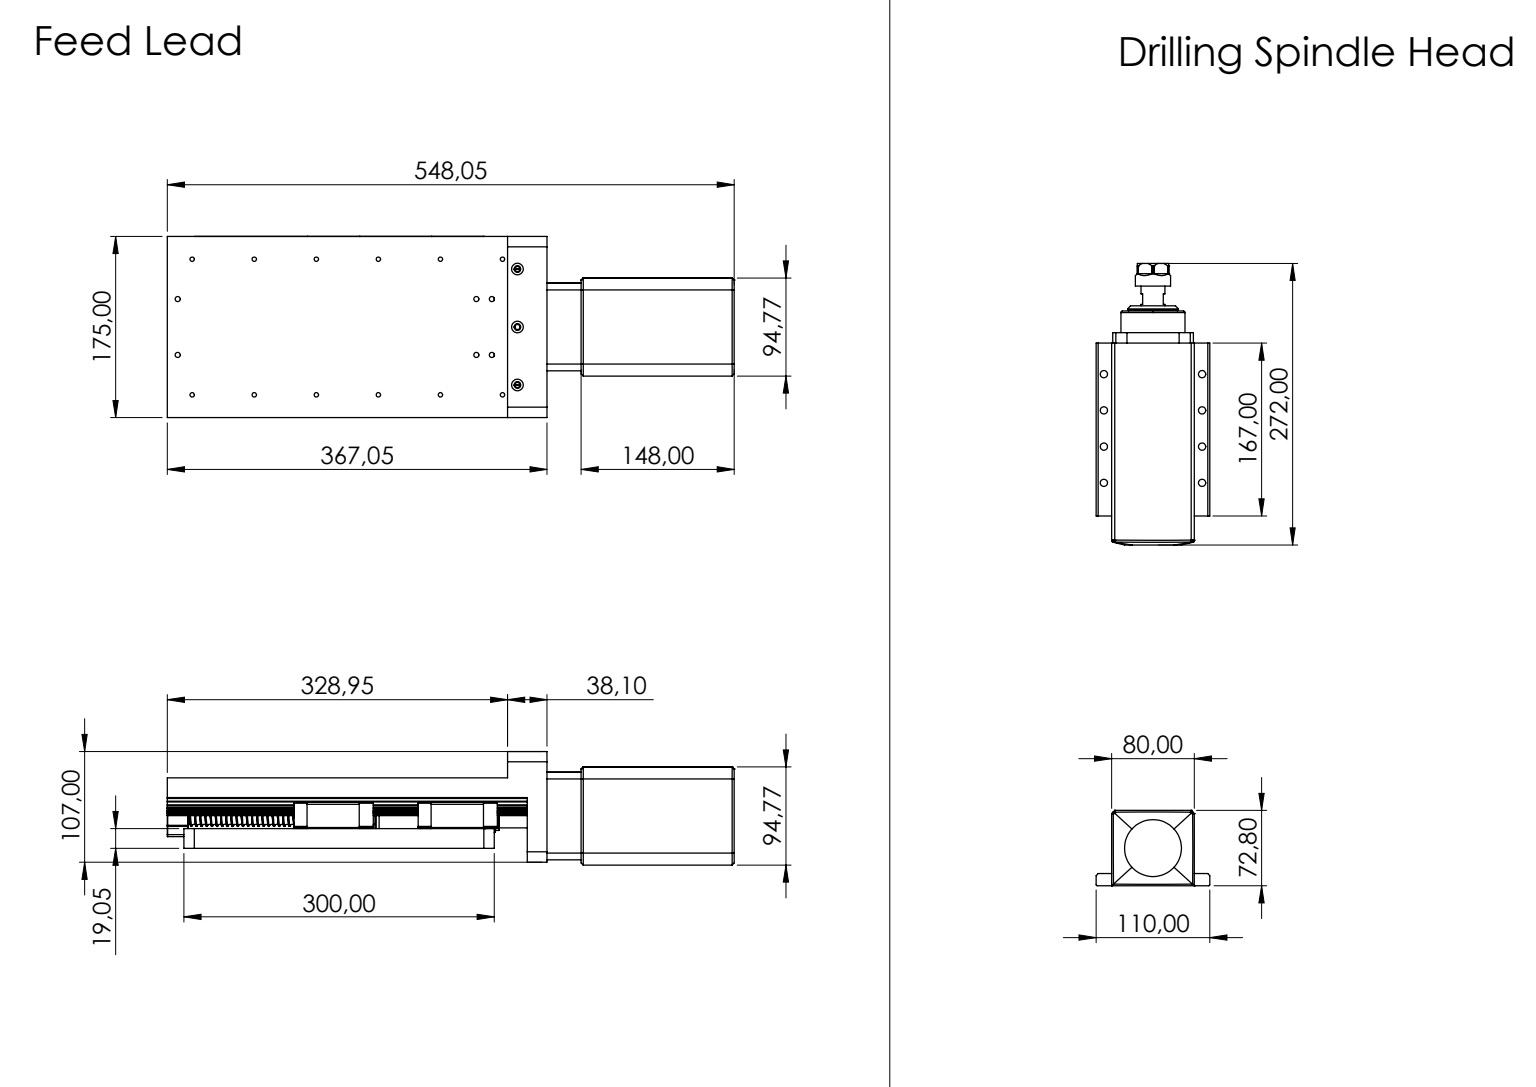
ISO-10303-21;
HEADER;
FILE_DESCRIPTION (('STEP AP214'),
    '1' );
FILE_NAME ('Feed Lead.step',
    '2026-10-07T11:37:37',
    ( '' ),
    ( '' ),
    'SwSTEP 2.0',
    'SolidWorks 2020',
    '' );
FILE_SCHEMA (( 'AUTOMOTIVE_DESIGN' ));
ENDSEC;

DATA;
#1=CARTESIAN_POINT ( 'NONE',  ( 98.82205551832399237, -39.36200594543229414, 279.3785665600675543 ) ) ;
#2=VECTOR ( 'NONE', #11114, 1000.000000000000000 ) ;
#4=CARTESIAN_POINT ( 'NONE',  ( 105.4244293397738659, -47.72525222749325735, 147.4584824187689662 ) ) ;
#7=DIRECTION ( 'NONE',  ( 0.000000000000000000, 1.000000000000000000, 0.000000000000000000 ) ) ;
#10=CARTESIAN_POINT ( 'NONE',  ( 112.4341072229889136, -46.44469865882210513, 248.9661014663869878 ) ) ;
#13=ORIENTED_EDGE ( 'NONE', *, *, #80261, .T. ) ;
#16=CARTESIAN_POINT ( 'NONE',  ( 97.53157056845665807, -31.04763954905634193, 126.9108633711489915 ) ) ;
#17=CARTESIAN_POINT ( 'NONE',  ( 83.56670559755357885, -36.73837296219067383, 249.5838068554176630 ) ) ;
#20=ORIENTED_EDGE ( 'NONE', *, *, #86122, .T. ) ;
#22=DIRECTION ( 'NONE',  ( 0.000000000000000000, 0.000000000000000000, -1.000000000000000000 ) ) ;
#23=LINE ( 'NONE', #20915, #47197 ) ;
#25=CARTESIAN_POINT ( 'NONE',  ( 179.7974245136208253, -36.32844715993472562, 237.4678068554150059 ) ) ;
#26=CARTESIAN_POINT ( 'NONE',  ( 108.8610815749077574, -28.26302276435299987, 182.7404713219719667 ) ) ;
#27=CARTESIAN_POINT ( 'NONE',  ( 118.1260584382194025, -36.12034675239389259, 269.8822919425776945 ) ) ;
#28=DIRECTION ( 'NONE',  ( 0.7071067811865491270, -0.7071067811865459074, 7.071067811865492096E-16 ) ) ;
#29=EDGE_LOOP ( 'NONE', ( #51270, #35552, #65434, #23515 ) ) ;
#34=ORIENTED_EDGE ( 'NONE', *, *, #61854, .T. ) ;
#35=EDGE_CURVE ( 'NONE', #22057, #40854, #8280, .T. ) ;
#37=DIRECTION ( 'NONE',  ( 0.000000000000000000, 0.000000000000000000, 1.000000000000000000 ) ) ;
#38=LINE ( 'NONE', #47715, #64581 ) ;
#39=CARTESIAN_POINT ( 'NONE',  ( 20.03715912545644073, -24.42818131006202265, 129.9678068554150627 ) ) ;
#42=CARTESIAN_POINT ( 'NONE',  ( 112.8494018163660968, -30.44343212223953543, 198.9067055423629711 ) ) ;
#43=CARTESIAN_POINT ( 'NONE',  ( 116.1621043582934902, -29.05491297703968101, 74.38419670448293175 ) ) ;
#44=CARTESIAN_POINT ( 'NONE',  ( 140.9629299006807059, -46.47944715994099596, -5.074374724088994704 ) ) ;
#45=VERTEX_POINT ( 'NONE', #80264 ) ;
#46=DIRECTION ( 'NONE',  ( 0.000000000000000000, 0.000000000000000000, -1.000000000000000000 ) ) ;
#47=ORIENTED_EDGE ( 'NONE', *, *, #89162, .T. ) ;
#50=LINE ( 'NONE', #6413, #88589 ) ;
#51=CARTESIAN_POINT ( 'NONE',  ( 151.0371591254573502, -24.42818131005592974, 249.9678068554149490 ) ) ;
#52=DIRECTION ( 'NONE',  ( 0.000000000000000000, 0.000000000000000000, -1.000000000000000000 ) ) ;
#53=AXIS2_PLACEMENT_3D ( 'NONE', #43663, #9164, #36861 ) ;
#54=CARTESIAN_POINT ( 'NONE',  ( 50.56670390244699576, -22.48495420874030515, 342.9256252759119548 ) ) ;
#56=CARTESIAN_POINT ( 'NONE',  ( 117.9477513149503523, -41.48675964724572651, 58.49848241876792798 ) ) ;
#59=LINE ( 'NONE', #15039, #77144 ) ;
#60=CARTESIAN_POINT ( 'NONE',  ( 131.4961476553978912, -17.75123073100106552, 2.855912073278314534 ) ) ;
#63=CIRCLE ( 'NONE', #39212, 3.250000000000002665 ) ;
#68=CIRCLE ( 'NONE', #26139, 0.1499999999999965528 ) ;
#69=CARTESIAN_POINT ( 'NONE',  ( 163.2449138992999735, -32.11662333284611748, -5.074374724088000832 ) ) ;
#70=VERTEX_POINT ( 'NONE', #52061 ) ;
#71=CARTESIAN_POINT ( 'NONE',  ( 98.28804800891427362, -28.73186473263583807, 76.73848241876795839 ) ) ;
#74=CARTESIAN_POINT ( 'NONE',  ( 151.0371591254582881, -46.82818131005593187, 249.9678068554149490 ) ) ;
#78=ORIENTED_EDGE ( 'NONE', *, *, #28035, .F. ) ;
#79=CARTESIAN_POINT ( 'NONE',  ( 116.1942131220465768, -33.21547736372282600, 135.1184824187679396 ) ) ;
#81=VECTOR ( 'NONE', #81815, 1000.000000000000000 ) ;
#82=PLANE ( 'NONE',  #68963 ) ;
#83=ORIENTED_EDGE ( 'NONE', *, *, #76173, .T. ) ;
#84=CARTESIAN_POINT ( 'NONE',  ( 95.25611604350974915, -37.33230102880721546, 267.3670538473395482 ) ) ;
#89=CARTESIAN_POINT ( 'NONE',  ( 19.56648329127400032, 0.2215528400590013880, 342.9256252759119548 ) ) ;
#90=DIRECTION ( 'NONE',  ( 0.000000000000000000, 0.000000000000000000, 1.000000000000000000 ) ) ;
#92=VECTOR ( 'NONE', #88319, 1000.000000000000000 ) ;
#93=CARTESIAN_POINT ( 'NONE',  ( 102.2986265273211188, -45.30740241592388884, 187.1727681330549729 ) ) ;
#94=ORIENTED_EDGE ( 'NONE', *, *, #21602, .F. ) ;
#96=CARTESIAN_POINT ( 'NONE',  ( 102.7360552222912418, -45.06754756083040547, 163.6149166392309837 ) ) ;
#97=CARTESIAN_POINT ( 'NONE',  ( 41.56648329127398966, -27.82844715994070484, 78.92562527591199739 ) ) ;
#98=CARTESIAN_POINT ( 'NONE',  ( 110.5196960824274868, -45.46740155661881033, 19.31967854399191253 ) ) ;
#100=VECTOR ( 'NONE', #56288, 1000.000000000000000 ) ;
#101=CARTESIAN_POINT ( 'NONE',  ( 97.80969231062213964, -40.51824920587227297, 266.6357212253427633 ) ) ;
#102=CARTESIAN_POINT ( 'NONE',  ( 107.3303934170485405, -25.27334761448656764, 321.8751915430112263 ) ) ;
#103=CIRCLE ( 'NONE', #55178, 11.45913725231036118 ) ;
#106=CARTESIAN_POINT ( 'NONE',  ( 117.3910620576583312, -35.19077923515891371, 218.9441967044829482 ) ) ;
#112=CARTESIAN_POINT ( 'NONE',  ( 98.04125204931517601, -41.04130019950920172, 122.6806003489451342 ) ) ;
#114=VECTOR ( 'NONE', #52134, 1000.000000000000114 ) ;
#115=ADVANCED_FACE ( 'NONE', ( #66606 ), #81165, .T. ) ;
#118=CARTESIAN_POINT ( 'NONE',  ( 109.6225776363756950, -25.10716277166327615, 25.90419670448196143 ) ) ;
#120=CARTESIAN_POINT ( 'NONE',  ( 116.8850244782298091, -41.80638879970206290, 243.4346728949589647 ) ) ;
#123=CARTESIAN_POINT ( 'NONE',  ( 48.16670390244701139, -28.27351298637280408, 342.9256252759109884 ) ) ;
#124=CARTESIAN_POINT ( 'NONE',  ( 116.9882021585877823, -35.34044312313820058, 168.9370952240663257 ) ) ;
#125=CARTESIAN_POINT ( 'NONE',  ( 103.0685998583681311, -29.61280089403793525, 58.30237608387695047 ) ) ;
#126=CARTESIAN_POINT ( 'NONE',  ( 103.0413726597163446, -26.41035368485499646, 166.3603871806729444 ) ) ;
#128=DIRECTION ( 'NONE',  ( 1.000000000000000000, 4.163336342344333240E-14, 0.000000000000000000 ) ) ;
#131=ORIENTED_EDGE ( 'NONE', *, *, #64159, .T. ) ;
#133=ORIENTED_EDGE ( 'NONE', *, *, #51168, .F. ) ;
#137=VERTEX_POINT ( 'NONE', #67956 ) ;
#138=DIRECTION ( 'NONE',  ( 0.000000000000000000, 0.000000000000000000, -1.000000000000000000 ) ) ;
#139=CARTESIAN_POINT ( 'NONE',  ( 114.8228036748933079, -33.15234975719755539, 103.5924198280769843 ) ) ;
#140=VECTOR ( 'NONE', #87504, 1000.000000000000000 ) ;
#141=CARTESIAN_POINT ( 'NONE',  ( 96.49566810458604493, -31.31724962161759507, 245.9499109901969689 ) ) ;
#142=CARTESIAN_POINT ( 'NONE',  ( 116.8369567342160451, -40.30247308064095790, 218.5470538473399529 ) ) ;
#143=CARTESIAN_POINT ( 'NONE',  ( 114.8031991714176741, -43.68443766454699073, 34.24419670448197905 ) ) ;
#145=CARTESIAN_POINT ( 'NONE',  ( 116.7940250750810804, -39.39174829627296504, 94.61447052041835093 ) ) ;
#146=VECTOR ( 'NONE', #83071, 1000.000000000000000 ) ;
#147=EDGE_CURVE ( 'NONE', #87632, #64364, #18910, .T. ) ;
#148=ORIENTED_EDGE ( 'NONE', *, *, #76335, .T. ) ;
#150=CARTESIAN_POINT ( 'NONE',  ( 98.15811136316399654, -31.42099212808717468, 130.9108633711499863 ) ) ;
#151=CARTESIAN_POINT ( 'NONE',  ( 106.8402339230401452, -48.62808610490878891, 77.56133956162491927 ) ) ;
#152=CARTESIAN_POINT ( 'NONE',  ( 104.8318391505165010, -26.46503486849124087, 260.2470538473397710 ) ) ;
#154=CARTESIAN_POINT ( 'NONE',  ( 115.5175571194294122, -29.60495148624196204, 224.3718157521009573 ) ) ;
#156=CARTESIAN_POINT ( 'NONE',  ( 107.0664832912739399, -36.72944715994095333, 293.9356252759109793 ) ) ;
#158=DIRECTION ( 'NONE',  ( -1.000000000000000078E-15, 0.000000000000000000, 1.000000000000000000 ) ) ;
#159=CARTESIAN_POINT ( 'NONE',  ( 167.2371591254543262, -47.82818131005522844, 249.9678068554149775 ) ) ;
#160=CARTESIAN_POINT ( 'NONE',  ( 41.56670390244777735, -36.32844715994104234, 300.4678068554150059 ) ) ;
#164=CARTESIAN_POINT ( 'NONE',  ( 88.17226027475679473, -58.72944715994100306, 239.5838068554174924 ) ) ;
#169=ORIENTED_EDGE ( 'NONE', *, *, #32648, .T. ) ;
#171=CARTESIAN_POINT ( 'NONE',  ( 96.89273651078235616, -34.20293982824353662, 276.1327681330536734 ) ) ;
#172=CARTESIAN_POINT ( 'NONE',  ( 117.0331605330187728, -30.31849857022486816, 140.2813395616249750 ) ) ;
#173=CARTESIAN_POINT ( 'NONE',  ( 106.2234015700748699, -47.79681864418333959, 263.5280062282922131 ) ) ;
#174=CARTESIAN_POINT ( 'NONE',  ( 51.56670390244799762, -33.35206098992650681, -5.074374724088000832 ) ) ;
#175=CIRCLE ( 'NONE', #23415, 3.000000000000002665 ) ;
#177=LINE ( 'NONE', #49653, #51558 ) ;
#178=CARTESIAN_POINT ( 'NONE',  ( 164.9212702847350158, -29.73316016639540749, -5.074374724088000832 ) ) ;
#179=CARTESIAN_POINT ( 'NONE',  ( 84.06648329127399677, -18.82844715994099971, 93.42562527591199739 ) ) ;
#180=VECTOR ( 'NONE', #42235, 1000.000000000000000 ) ;
#181=ORIENTED_EDGE ( 'NONE', *, *, #13082, .F. ) ;
#183=EDGE_LOOP ( 'NONE', ( #41737, #81659, #77262, #76610 ) ) ;
#184=CARTESIAN_POINT ( 'NONE',  ( 104.1791519563360993, -28.66003454886012136, 189.7724198280769770 ) ) ;
#185=EDGE_CURVE ( 'NONE', #48213, #31965, #19881, .T. ) ;
#186=CARTESIAN_POINT ( 'NONE',  ( 112.0622504009905356, -45.49043716283868832, 187.9900270775093247 ) ) ;
#187=ORIENTED_EDGE ( 'NONE', *, *, #67758, .F. ) ;
#189=CARTESIAN_POINT ( 'NONE',  ( 103.8142050530422864, -26.84757730287823563, 161.3299109901969643 ) ) ;
#190=DIRECTION ( 'NONE',  ( 0.000000000000000000, 1.000000000000000000, 0.000000000000000000 ) ) ;
#192=DIRECTION ( 'NONE',  ( 1.000000000000000000, 0.000000000000000000, 2.283216351027200160E-14 ) ) ;
#193=DIRECTION ( 'NONE',  ( 0.7071067811865779928, -0.7071067811865171526, 7.071067811865786933E-16 ) ) ;
#195=LINE ( 'NONE', #54679, #27346 ) ;
#196=CARTESIAN_POINT ( 'NONE',  ( 31.78666935232898894, -29.62846900982320264, -5.074374724088000832 ) ) ;
#197=CARTESIAN_POINT ( 'NONE',  ( 97.28369645613162220, -37.51102008256657427, 101.3899109901979472 ) ) ;
#199=ORIENTED_EDGE ( 'NONE', *, *, #77128, .T. ) ;
#202=CARTESIAN_POINT ( 'NONE',  ( 106.1501016865858844, -27.91533782510476058, 46.59015473446797984 ) ) ;
#203=DIRECTION ( 'NONE',  ( 5.512527431108029424E-15, -1.000000000000000000, 0.000000000000000000 ) ) ;
#204=CARTESIAN_POINT ( 'NONE',  ( 104.6152064257953640, -27.26083179018629465, 196.2784824187679362 ) ) ;
#206=DIRECTION ( 'NONE',  ( 0.000000000000000000, 0.000000000000000000, -1.000000000000000000 ) ) ;
#208=VECTOR ( 'NONE', #84296, 1000.000000000000000 ) ;
#209=CARTESIAN_POINT ( 'NONE',  ( 37.06648329127298780, 12.92155284005730387, 361.9756252759109998 ) ) ;
#210=CARTESIAN_POINT ( 'NONE',  ( 41.56670390244777735, -36.32844715994104234, 300.4678068554150059 ) ) ;
#212=CARTESIAN_POINT ( 'NONE',  ( 107.3333893024683903, -26.32957087652219741, 120.0556252759109555 ) ) ;
#213=EDGE_LOOP ( 'NONE', ( #60741, #6929, #76892, #6396, #4910, #86505 ) ) ;
#215=ORIENTED_EDGE ( 'NONE', *, *, #58002, .F. ) ;
#219=CARTESIAN_POINT ( 'NONE',  ( 98.44383420958352815, -35.98725590436672661, 184.0642808457819797 ) ) ;
#221=CARTESIAN_POINT ( 'NONE',  ( 104.4907063090252848, -26.97860099647315835, 26.28081536904196014 ) ) ;
#223=VERTEX_POINT ( 'NONE', #60677 ) ;
#224=ORIENTED_EDGE ( 'NONE', *, *, #76975, .F. ) ;
#225=AXIS2_PLACEMENT_3D ( 'NONE', #81195, #12130, #54323 ) ;
#226=CARTESIAN_POINT ( 'NONE',  ( 136.6090958654750978, -19.77717416134860073, 2.822018739140460308 ) ) ;
#227=ORIENTED_EDGE ( 'NONE', *, *, #86908, .T. ) ;
#228=VERTEX_POINT ( 'NONE', #75677 ) ;
#229=DIRECTION ( 'NONE',  ( 0.7071067811989784069, -0.7071067811741166276, 2.899137802813994686E-29 ) ) ;
#230=CARTESIAN_POINT ( 'NONE',  ( 115.9278856700424143, -36.79130581669468825, 260.2530118773256049 ) ) ;
#231=VERTEX_POINT ( 'NONE', #46142 ) ;
#232=VECTOR ( 'NONE', #61372, 1000.000000000000000 ) ;
#233=DIRECTION ( 'NONE',  ( 0.000000000000000000, 0.000000000000000000, 1.000000000000000000 ) ) ;
#235=ORIENTED_EDGE ( 'NONE', *, *, #62757, .T. ) ;
#236=ORIENTED_EDGE ( 'NONE', *, *, #27432, .F. ) ;
#239=FACE_OUTER_BOUND ( 'NONE', #13018, .T. ) ;
#240=ORIENTED_EDGE ( 'NONE', *, *, #81916, .T. ) ;
#241=VERTEX_POINT ( 'NONE', #73874 ) ;
#243=CARTESIAN_POINT ( 'NONE',  ( 102.1978417368446657, -43.31572210571547998, 254.8880903695915947 ) ) ;
#245=CARTESIAN_POINT ( 'NONE',  ( 117.7016330746719035, -39.82606306527180351, 138.5889586092439743 ) ) ;
#246=CARTESIAN_POINT ( 'NONE',  ( 109.7644292386350457, -47.42453529627131559, 92.78514908543495210 ) ) ;
#248=DIRECTION ( 'NONE',  ( 0.000000000000000000, 1.000000000000000000, 0.000000000000000000 ) ) ;
#249=CARTESIAN_POINT ( 'NONE',  ( 118.0406971908402340, -35.41012545131285094, 234.9337205140059552 ) ) ;
#250=PLANE ( 'NONE',  #16765 ) ;
#251=CARTESIAN_POINT ( 'NONE',  ( 97.07202379341690346, -35.37891260357572776, 127.2189961379345533 ) ) ;
#252=ORIENTED_EDGE ( 'NONE', *, *, #45616, .F. ) ;
#257=EDGE_CURVE ( 'NONE', #42008, #10149, #60224, .T. ) ;
#258=EDGE_LOOP ( 'NONE', ( #12072, #35059, #37559, #82671 ) ) ;
#260=EDGE_CURVE ( 'NONE', #76240, #83594, #40692, .T. ) ;
#261=EDGE_CURVE ( 'NONE', #85910, #25889, #5287, .T. ) ;
#263=AXIS2_PLACEMENT_3D ( 'NONE', #9661, #10113, #65519 ) ;
#264=CARTESIAN_POINT ( 'NONE',  ( 113.9865487620526920, -28.11017913222394071, 119.5261014663869474 ) ) ;
#266=ADVANCED_FACE ( 'NONE', ( #53845 ), #12696, .T. ) ;
#270=CARTESIAN_POINT ( 'NONE',  ( 97.84728005659533778, -40.60342492179871954, 56.64262628539218269 ) ) ;
#271=CARTESIAN_POINT ( 'NONE',  ( 107.2427983594548948, -47.16656068249876910, 208.5899109901969837 ) ) ;
#272=LINE ( 'NONE', #64302, #50971 ) ;
#273=CARTESIAN_POINT ( 'NONE',  ( 73.06648329127396835, -8.729447159941065237, 14.67562527591093513 ) ) ;
#276=CARTESIAN_POINT ( 'NONE',  ( 25.56670390244797275, -62.87844715994099687, 262.0928068554150059 ) ) ;
#277=EDGE_CURVE ( 'NONE', #55396, #20871, #38896, .T. ) ;
#279=CARTESIAN_POINT ( 'NONE',  ( 25.56670390244797275, -62.87844715994099687, 173.2178068554149775 ) ) ;
#282=CARTESIAN_POINT ( 'NONE',  ( 97.18209604296552584, -40.28622700274314639, 266.6013395616253661 ) ) ;
#283=EDGE_LOOP ( 'NONE', ( #66370, #22379, #4924, #25013 ) ) ;
#285=CARTESIAN_POINT ( 'NONE',  ( 102.0403423364015509, -46.60028036886249225, 172.2137205140059564 ) ) ;
#286=CARTESIAN_POINT ( 'NONE',  ( 96.65901483881968659, -33.00673566691533978, 22.06514908543494258 ) ) ;
#287=CARTESIAN_POINT ( 'NONE',  ( 102.8263616157396854, -46.30098559033366001, 173.2441967044829596 ) ) ;
#288=DIRECTION ( 'NONE',  ( 0.000000000000000000, 1.000000000000000000, 1.541976423090495239E-15 ) ) ;
#289=CARTESIAN_POINT ( 'NONE',  ( 194.0667039024482392, -40.32844715993407192, 129.9678068554150343 ) ) ;
#290=DIRECTION ( 'NONE',  ( 1.000000000000000000, 6.897260540483778545E-11, 0.000000000000000000 ) ) ;
#291=DIRECTION ( 'NONE',  ( -0.9254794337955623007, -0.3787978585227819162, 0.000000000000000000 ) ) ;
#292=CARTESIAN_POINT ( 'NONE',  ( 102.0670550211478940, -27.97049802524514561, 190.4897919370553723 ) ) ;
#294=ORIENTED_EDGE ( 'NONE', *, *, #45450, .F. ) ;
#297=ORIENTED_EDGE ( 'NONE', *, *, #22548, .T. ) ;
#298=EDGE_CURVE ( 'NONE', #22750, #69972, #67790, .T. ) ;
#300=CARTESIAN_POINT ( 'NONE',  ( 108.9812119692459049, -46.95502683147942236, 78.72419670448194040 ) ) ;
#302=EDGE_CURVE ( 'NONE', #30540, #70341, #82951, .T. ) ;
#304=CARTESIAN_POINT ( 'NONE',  ( 113.7066566934868348, -44.24661119772650864, 118.1542348793510797 ) ) ;
#305=CARTESIAN_POINT ( 'NONE',  ( 114.3743266858445935, -29.18402207539437399, 170.4641967044829585 ) ) ;
#306=EDGE_CURVE ( 'NONE', #30320, #66948, #55191, .T. ) ;
#307=CIRCLE ( 'NONE', #48127, 2.500000000000002220 ) ;
#308=CARTESIAN_POINT ( 'NONE',  ( 106.3786087989843736, -45.75936958534449417, 266.9505150661723860 ) ) ;
#310=EDGE_LOOP ( 'NONE', ( #10446, #4525, #31738, #66778 ) ) ;
#311=VERTEX_POINT ( 'NONE', #89763 ) ;
#315=CARTESIAN_POINT ( 'NONE',  ( 105.8005616001767919, -26.72389448867465589, 20.17631252315041124 ) ) ;
#317=LINE ( 'NONE', #34380, #47959 ) ;
#318=FACE_OUTER_BOUND ( 'NONE', #73984, .T. ) ;
#319=DIRECTION ( 'NONE',  ( 0.000000000000000000, 0.000000000000000000, -1.000000000000000000 ) ) ;
#320=CARTESIAN_POINT ( 'NONE',  ( 116.7068942081672276, -31.36975501082240569, 29.24229194257799236 ) ) ;
#322=AXIS2_PLACEMENT_3D ( 'NONE', #12515, #67464, #82472 ) ;
#323=EDGE_LOOP ( 'NONE', ( #9517, #37915, #44390, #42427, #11200 ) ) ;
#325=DIRECTION ( 'NONE',  ( 0.000000000000000000, 0.000000000000000000, 1.000000000000000000 ) ) ;
#326=CARTESIAN_POINT ( 'NONE',  ( 115.3104451506078192, -40.98773602117310588, 91.26523322673496352 ) ) ;
#329=CARTESIAN_POINT ( 'NONE',  ( 188.5667039024483529, -48.82844715993431350, 293.2178068554150059 ) ) ;
#331=DIRECTION ( 'NONE',  ( -1.000000000000000000, -4.299999999999999979E-14, -1.000000000000000078E-15 ) ) ;
#332=ORIENTED_EDGE ( 'NONE', *, *, #80901, .T. ) ;
#336=ORIENTED_EDGE ( 'NONE', *, *, #71330, .T. ) ;
#338=CARTESIAN_POINT ( 'NONE',  ( 105.5787418010314695, -46.69191849206237066, 143.8901547344689789 ) ) ;
#339=DIRECTION ( 'NONE',  ( 0.000000000000000000, 0.000000000000000000, -1.000000000000000000 ) ) ;
#340=CARTESIAN_POINT ( 'NONE',  ( 108.5410322698540853, -26.38715707682645117, 100.9641967044829727 ) ) ;
#342=ORIENTED_EDGE ( 'NONE', *, *, #66737, .T. ) ;
#344=( BOUNDED_CURVE ( )  B_SPLINE_CURVE ( 3, ( #44, #89538, #6404, #82288 ),
 .UNSPECIFIED., .F., .F. ) 
 B_SPLINE_CURVE_WITH_KNOTS ( ( 4, 4 ),
 ( 1.570796326796012332, 3.141592653591100071 ),
 .UNSPECIFIED. ) 
 CURVE ( )  GEOMETRIC_REPRESENTATION_ITEM ( )  RATIONAL_B_SPLINE_CURVE ( ( 1.000000000000000000, 0.8047378541243199734, 0.8047378541243199734, 1.000000000000000000 ) ) 
 REPRESENTATION_ITEM ( '' )  );
#347=EDGE_CURVE ( 'NONE', #71530, #74616, #28405, .T. ) ;
#348=EDGE_CURVE ( 'NONE', #63582, #58541, #14803, .T. ) ;
#349=EDGE_CURVE ( 'NONE', #47011, #27495, #88110, .T. ) ;
#350=AXIS2_PLACEMENT_3D ( 'NONE', #71260, #57605, #29916 ) ;
#353=CARTESIAN_POINT ( 'NONE',  ( 99.85651329992167291, -30.12038005267077878, 275.7356252759109907 ) ) ;
#354=CARTESIAN_POINT ( 'NONE',  ( 102.3028228262999164, -26.72980997527264790, 136.4422919425779526 ) ) ;
#355=DIRECTION ( 'NONE',  ( 1.000000000000000078E-15, 1.000000000000000083E-30, -1.000000000000000000 ) ) ;
#357=CARTESIAN_POINT ( 'NONE',  ( 103.8413319783160489, -46.68031304110885316, 78.32705384733995402 ) ) ;
#358=CARTESIAN_POINT ( 'NONE',  ( 113.1782937855189175, -44.75186858143347024, 263.0939586106779871 ) ) ;
#359=ORIENTED_EDGE ( 'NONE', *, *, #83740, .T. ) ;
#362=ADVANCED_FACE ( 'NONE', ( #20710 ), #6627, .T. ) ;
#363=CYLINDRICAL_SURFACE ( 'NONE', #49100, 2.517500000000005844 ) ;
#368=CARTESIAN_POINT ( 'NONE',  ( 106.5180884070038161, -25.68959433010697779, 45.12800622829193742 ) ) ;
#372=CARTESIAN_POINT ( 'NONE',  ( 115.7849560329669316, -41.79918665415381440, 93.40735705935379940 ) ) ;
#373=CARTESIAN_POINT ( 'NONE',  ( 113.6564618781686704, -45.68400828401192371, 33.08133956162595268 ) ) ;
#374=CARTESIAN_POINT ( 'NONE',  ( 123.6837132603319560, -55.86395651782485317, 239.5838068554170377 ) ) ;
#375=CARTESIAN_POINT ( 'NONE',  ( 116.9011659702703270, -33.23038410113878882, 110.0984824187679578 ) ) ;
#380=LINE ( 'NONE', #54868, #23274 ) ;
#383=AXIS2_PLACEMENT_3D ( 'NONE', #79227, #30612, #36545 ) ;
#384=EDGE_CURVE ( 'NONE', #62636, #60868, #42469, .T. ) ;
#385=CARTESIAN_POINT ( 'NONE',  ( 97.81305373959743577, -40.51655628150228949, 62.63606721061723448 ) ) ;
#386=CARTESIAN_POINT ( 'NONE',  ( 113.7136498174399577, -45.61921998050937077, 188.0994347997199725 ) ) ;
#388=DIRECTION ( 'NONE',  ( 0.000000000000000000, 0.000000000000000000, 1.000000000000000000 ) ) ;
#389=CARTESIAN_POINT ( 'NONE',  ( 116.3968524479345348, -41.42853965253563331, 199.4556252759109611 ) ) ;
#392=ADVANCED_FACE ( 'NONE', ( #48831 ), #55637, .F. ) ;
#394=VERTEX_POINT ( 'NONE', #62925 ) ;
#395=CIRCLE ( 'NONE', #51150, 2.029999999999997140 ) ;
#397=VERTEX_POINT ( 'NONE', #70200 ) ;
#398=EDGE_LOOP ( 'NONE', ( #88242, #56816, #40923, #15353 ) ) ;
#400=B_SPLINE_CURVE_WITH_KNOTS ( 'NONE', 3,
 ( #74384, #34379, #5797, #83006, #53452, #62087, #20761, #48432, #41187, #82114, #19868, #6241, #39844, #69366, #89822, #68914, #6681, #20327 ),
 .UNSPECIFIED., .F., .F.,
 ( 4, 2, 2, 2, 2, 2, 2, 2, 4 ),
 ( 0.000000000000000000, 0.06249223058255102409, 0.1249844611651020482, 0.1874766917476530792, 0.2499689223302040963, 0.3124611529127551135, 0.3749533834953061584, 0.4374456140778571478, 0.4999378446604081927 ),
 .UNSPECIFIED. ) ;
#401=ORIENTED_EDGE ( 'NONE', *, *, #80513, .F. ) ;
#403=CARTESIAN_POINT ( 'NONE',  ( 100.7501737310821994, -45.80018108968007340, 233.0803871806729717 ) ) ;
#404=CARTESIAN_POINT ( 'NONE',  ( 107.0664832912739399, -36.72944715994095333, 293.6356252759106837 ) ) ;
#406=EDGE_CURVE ( 'NONE', #68641, #20681, #82800, .T. ) ;
#410=LINE ( 'NONE', #49435, #25440 ) ;
#411=CARTESIAN_POINT ( 'NONE',  ( 96.66715014961923202, -32.91509328854561289, 21.03467289495897319 ) ) ;
#414=CARTESIAN_POINT ( 'NONE',  ( 89.10937460273881072, -56.62589376934804619, 14.92562527591089072 ) ) ;
#416=CARTESIAN_POINT ( 'NONE',  ( 104.3638673426610950, -27.29495504168068365, 221.2984824187679465 ) ) ;
#420=CARTESIAN_POINT ( 'NONE',  ( 112.4472966703648780, -46.45872411559670212, 98.97848241876694431 ) ) ;
#421=CARTESIAN_POINT ( 'NONE',  ( 97.81193015299326987, -40.51731617131004271, 31.63594527021773573 ) ) ;
#422=CARTESIAN_POINT ( 'NONE',  ( 99.09526974470551863, -30.55101700259475095, 21.80228081981730526 ) ) ;
#423=ORIENTED_EDGE ( 'NONE', *, *, #49489, .T. ) ;
#427=EDGE_LOOP ( 'NONE', ( #4062, #28838, #78754, #43787 ) ) ;
#429=CARTESIAN_POINT ( 'NONE',  ( 114.5810018449060834, -31.08954144758037685, 260.7825356868496556 ) ) ;
#432=CARTESIAN_POINT ( 'NONE',  ( 164.7830935719630361, -29.99615139349950965, 193.9678068554150059 ) ) ;
#433=DIRECTION ( 'NONE',  ( 0.000000000000000000, 0.000000000000000000, -1.000000000000000000 ) ) ;
#434=CARTESIAN_POINT ( 'NONE',  ( 105.8694971003958614, -26.37070548771162493, 321.6188579224977389 ) ) ;
#437=DIRECTION ( 'NONE',  ( 3.999999999999999995E-14, -1.000000000000000000, 4.100000000000000342E-29 ) ) ;
#438=CARTESIAN_POINT ( 'NONE',  ( 101.9929361239610586, -45.44564905068737914, 183.1569278323868275 ) ) ;
#439=ORIENTED_EDGE ( 'NONE', *, *, #54997, .F. ) ;
#440=CARTESIAN_POINT ( 'NONE',  ( 103.5987056385471448, -46.56110768157568458, 57.30705384733997221 ) ) ;
#441=ORIENTED_EDGE ( 'NONE', *, *, #18893, .T. ) ;
#442=CARTESIAN_POINT ( 'NONE',  ( 110.7250417795893611, -29.43255185136001728, 277.5252332267342581 ) ) ;
#443=DIRECTION ( 'NONE',  ( 0.000000000000000000, 0.000000000000000000, -1.000000000000000000 ) ) ;
#444=CARTESIAN_POINT ( 'NONE',  ( 113.3375292005774639, -44.23527279707086279, 193.1299109901969757 ) ) ;
#446=DIRECTION ( 'NONE',  ( 1.000000000000000000, 8.843517682682131024E-16, 1.000000000000000078E-15 ) ) ;
#448=CARTESIAN_POINT ( 'NONE',  ( 57.56670390244832447, -48.82844715994039575, 257.2178068554150627 ) ) ;
#449=EDGE_CURVE ( 'NONE', #89731, #57212, #70727, .T. ) ;
#450=CARTESIAN_POINT ( 'NONE',  ( 100.8224507837568638, -45.17634439094529597, 253.0699109901969450 ) ) ;
#451=CARTESIAN_POINT ( 'NONE',  ( 108.4288913835557935, -46.66050271621784873, 117.6868369591917798 ) ) ;
#452=ORIENTED_EDGE ( 'NONE', *, *, #80459, .T. ) ;
#455=CARTESIAN_POINT ( 'NONE',  ( 117.6520138419322734, -33.39117794972031561, 125.0575300378149706 ) ) ;
#457=AXIS2_PLACEMENT_3D ( 'NONE', #40016, #13662, #12778 ) ;
#460=EDGE_CURVE ( 'NONE', #23716, #59746, #25705, .T. ) ;
#462=VERTEX_POINT ( 'NONE', #5128 ) ;
#463=LINE ( 'NONE', #21362, #81231 ) ;
#464=ADVANCED_FACE ( 'NONE', ( #20109, #60985 ), #12393, .T. ) ;
#465=DIRECTION ( 'NONE',  ( 1.000000000000000078E-15, -1.000000000000000083E-30, -1.000000000000000000 ) ) ;
#466=DIRECTION ( 'NONE',  ( 9.351236661543306751E-17, -3.725950533538267725E-29, -1.000000000000000000 ) ) ;
#467=CARTESIAN_POINT ( 'NONE',  ( 46.03715912545432332, -48.62818131006086020, 249.9678068554150343 ) ) ;
#468=CARTESIAN_POINT ( 'NONE',  ( 165.2748236753145079, -30.08671355699731720, 313.9678068554149490 ) ) ;
#469=CARTESIAN_POINT ( 'NONE',  ( 114.5787023362084085, -39.92261033116096058, 166.3252332267339852 ) ) ;
#470=CARTESIAN_POINT ( 'NONE',  ( 99.31704471179752147, -28.81544643672065220, 266.7051490854347549 ) ) ;
#471=CARTESIAN_POINT ( 'NONE',  ( 181.9694315774339941, -34.03355364505720360, -5.074374724088000832 ) ) ;
#472=ORIENTED_EDGE ( 'NONE', *, *, #66905, .F. ) ;
#474=EDGE_CURVE ( 'NONE', #57694, #54558, #12854, .T. ) ;
#475=DIRECTION ( 'NONE',  ( 0.000000000000000000, 1.000000000000000000, 0.000000000000000000 ) ) ;
#476=ORIENTED_EDGE ( 'NONE', *, *, #40956, .T. ) ;
#477=ORIENTED_EDGE ( 'NONE', *, *, #19060, .T. ) ;
#478=ADVANCED_FACE ( 'NONE', ( #33732 ), #15616, .T. ) ;
#483=LINE ( 'NONE', #35438, #14390 ) ;
#484=CARTESIAN_POINT ( 'NONE',  ( 125.0664851986225159, -56.72944715994101728, 14.67562527591098842 ) ) ;
#485=EDGE_CURVE ( 'NONE', #9163, #84782, #46440, .T. ) ;
#486=CARTESIAN_POINT ( 'NONE',  ( 113.4141308401190287, -30.97102092343966007, 208.8352769709339896 ) ) ;
#487=CARTESIAN_POINT ( 'NONE',  ( 115.7653496281367325, -43.62456195820889349, 48.30514908543492680 ) ) ;
#488=ORIENTED_EDGE ( 'NONE', *, *, #73147, .F. ) ;
#491=AXIS2_PLACEMENT_3D ( 'NONE', #81875, #41838, #63202 ) ;
#494=CARTESIAN_POINT ( 'NONE',  ( 100.9540432847708757, -28.70751825035962668, 261.5939957165031728 ) ) ;
#495=ORIENTED_EDGE ( 'NONE', *, *, #3649, .T. ) ;
#496=DIRECTION ( 'NONE',  ( 0.000000000000000000, 1.000000000000000000, 0.000000000000000000 ) ) ;
#497=DIRECTION ( 'NONE',  ( 0.7071067811864661934, 0.7071067811866289521, 7.071067811864654918E-16 ) ) ;
#500=DIRECTION ( 'NONE',  ( 0.000000000000000000, 0.000000000000000000, 1.000000000000000000 ) ) ;
#502=CARTESIAN_POINT ( 'NONE',  ( 117.0750736332619937, -31.98354782443029620, 64.19086337114899266 ) ) ;
#505=CARTESIAN_POINT ( 'NONE',  ( 123.0664832912757021, -36.72944715993921960, 13.92562527591098487 ) ) ;
#506=CARTESIAN_POINT ( 'NONE',  ( 132.5731111080376081, -16.41810224486803449, 1.981704920701433448 ) ) ;
#507=ORIENTED_EDGE ( 'NONE', *, *, #40768, .T. ) ;
#512=CARTESIAN_POINT ( 'NONE',  ( 114.0955628336689500, -44.50577255156974843, 129.1613395616249704 ) ) ;
#515=EDGE_CURVE ( 'NONE', #85162, #7841, #6469, .T. ) ;
#516=DIRECTION ( 'NONE',  ( 0.000000000000000000, -1.000000000000000000, 0.000000000000000000 ) ) ;
#518=CARTESIAN_POINT ( 'NONE',  ( 162.8595971212720031, -23.19206098994050436, -5.074374724088000832 ) ) ;
#519=CARTESIAN_POINT ( 'NONE',  ( 97.33998274022617636, -37.75834089694784979, 122.4099109901959679 ) ) ;
#522=CARTESIAN_POINT ( 'NONE',  ( 115.0380569359701326, -30.04493676975927485, 265.3813395616251682 ) ) ;
#524=FACE_OUTER_BOUND ( 'NONE', #14285, .T. ) ;
#527=CARTESIAN_POINT ( 'NONE',  ( 48.16670390244701139, -26.71338133339251542, -5.074374724088000832 ) ) ;
#528=DIRECTION ( 'NONE',  ( 0.000000000000000000, 0.000000000000000000, 1.000000000000000000 ) ) ;
#529=CARTESIAN_POINT ( 'NONE',  ( 108.1128363339379632, -46.45408497333518483, 202.6613395616259652 ) ) ;
#530=ORIENTED_EDGE ( 'NONE', *, *, #45775, .T. ) ;
#532=CARTESIAN_POINT ( 'NONE',  ( 113.1755435565086998, -43.14875213554007161, 154.6130118773249649 ) ) ;
#533=EDGE_CURVE ( 'NONE', #28842, #89511, #38792, .T. ) ;
#535=CARTESIAN_POINT ( 'NONE',  ( 31.89136050872263439, -31.76306994223845948, 237.4678068554150059 ) ) ;
#536=CARTESIAN_POINT ( 'NONE',  ( 98.24278011039416469, -41.58876472015902692, 23.15872616303999010 ) ) ;
#538=CARTESIAN_POINT ( 'NONE',  ( 69.26949937496598864, -71.54137415153812185, 361.9756252759101471 ) ) ;
#539=DIRECTION ( 'NONE',  ( 1.000000000000000078E-15, 1.000000000000000083E-30, -1.000000000000000000 ) ) ;
#541=AXIS2_PLACEMENT_3D ( 'NONE', #19415, #46652, #5344 ) ;
#542=CARTESIAN_POINT ( 'NONE',  ( 193.0371591254572934, -23.42818131005411786, 237.4678068554150059 ) ) ;
#543=CYLINDRICAL_SURFACE ( 'NONE', #74912, 9.999999999999998224 ) ;
#544=CARTESIAN_POINT ( 'NONE',  ( 115.4997179687694882, -29.61999039777954579, 224.3718157521009573 ) ) ;
#546=ORIENTED_EDGE ( 'NONE', *, *, #43939, .F. ) ;
#548=CARTESIAN_POINT ( 'NONE',  ( 98.30753417703368768, -41.72887546760895106, 86.73979194043660357 ) ) ;
#549=CARTESIAN_POINT ( 'NONE',  ( 82.81647637678409524, -18.77596264856125430, 6.749779334551668342 ) ) ;
#550=CARTESIAN_POINT ( 'NONE',  ( 113.1793785465512201, -44.75106650107741046, 124.0924085711809965 ) ) ;
#551=CARTESIAN_POINT ( 'NONE',  ( 25.56670390244797275, -67.87844715994100397, 262.0928068554150059 ) ) ;
#554=FACE_OUTER_BOUND ( 'NONE', #32275, .T. ) ;
#555=CARTESIAN_POINT ( 'NONE',  ( 118.1077515449285613, -36.21032982800684152, 268.8518157521015723 ) ) ;
#556=EDGE_CURVE ( 'NONE', #40009, #71950, #88711, .T. ) ;
#558=EDGE_CURVE ( 'NONE', #50481, #68206, #62341, .T. ) ;
#559=CARTESIAN_POINT ( 'NONE',  ( 107.0664832912739968, -36.72944715994100306, 287.6356252759109680 ) ) ;
#560=FACE_BOUND ( 'NONE', #57673, .T. ) ;
#561=ADVANCED_FACE ( 'NONE', ( #55484, #43213 ), #64129, .F. ) ;
#563=CARTESIAN_POINT ( 'NONE',  ( 107.1962421797556289, -28.07588791089852265, 77.89475703625792846 ) ) ;
#564=CARTESIAN_POINT ( 'NONE',  ( 113.5786777234211939, -44.94349119991360197, 164.1099109901969655 ) ) ;
#565=LINE ( 'NONE', #61440, #85629 ) ;
#567=EDGE_CURVE ( 'NONE', #27001, #32371, #2511, .T. ) ;
#568=DIRECTION ( 'NONE',  ( 4.237773401492740281E-14, -1.000000000000000000, 0.000000000000000000 ) ) ;
#569=EDGE_LOOP ( 'NONE', ( #65281, #35010, #45549, #63195, #36234, #78377 ) ) ;
#570=ORIENTED_EDGE ( 'NONE', *, *, #83826, .F. ) ;
#573=ORIENTED_EDGE ( 'NONE', *, *, #24287, .F. ) ;
#576=AXIS2_PLACEMENT_3D ( 'NONE', #61805, #46, #41357 ) ;
#577=CARTESIAN_POINT ( 'NONE',  ( 106.9471680199217332, -25.26948335760882713, 320.5674069059367639 ) ) ;
#578=EDGE_CURVE ( 'NONE', #82390, #82238, #27804, .T. ) ;
#579=CARTESIAN_POINT ( 'NONE',  ( 113.7032067727884197, -42.10625226631949403, 87.70670554236198768 ) ) ;
#580=CARTESIAN_POINT ( 'NONE',  ( 106.8511556536399780, -47.80415145147887301, 227.5489586092439538 ) ) ;
#581=CARTESIAN_POINT ( 'NONE',  ( 103.3114313307233658, -27.02747569519249993, 215.3699109901969848 ) ) ;
#582=CARTESIAN_POINT ( 'NONE',  ( 112.1705331031350283, -27.62378402076942763, 30.66991099019694644 ) ) ;
#583=CARTESIAN_POINT ( 'NONE',  ( 41.56648329127399677, 0.2215528400590013880, 76.80862527591200717 ) ) ;
#585=EDGE_LOOP ( 'NONE', ( #73914, #36571, #16667, #18856, #51645, #20721, #25049, #39551, #67761, #8021, #890, #9072, #69488, #83607, #32589, #87543 ) ) ;
#589=CARTESIAN_POINT ( 'NONE',  ( 96.20363159075253634, -34.36081134307595164, 106.1556252759109640 ) ) ;
#590=CARTESIAN_POINT ( 'NONE',  ( 101.6881215347969345, -27.70586588967184483, 85.50419670448295051 ) ) ;
#591=CARTESIAN_POINT ( 'NONE',  ( 106.8354617269136497, -47.19621815579884583, 272.5584824187680510 ) ) ;
#592=VECTOR ( 'NONE', #33740, 1000.000000000000000 ) ;
#593=VERTEX_POINT ( 'NONE', #57292 ) ;
#594=UNCERTAINTY_MEASURE_WITH_UNIT (LENGTH_MEASURE( 1.000000000000000082E-05 ), #15036, 'distance_accuracy_value', 'NONE');
#595=CARTESIAN_POINT ( 'NONE',  ( 101.6505379212622699, -45.63756515480785225, 247.1413395616249602 ) ) ;
#596=DIRECTION ( 'NONE',  ( 0.000000000000000000, 0.000000000000000000, 1.000000000000000000 ) ) ;
#597=VECTOR ( 'NONE', #60325, 1000.000000000000000 ) ;
#600=CARTESIAN_POINT ( 'NONE',  ( 49.16670390244654243, -28.27351298637376686, 193.9678068554150911 ) ) ;
#601=DIRECTION ( 'NONE',  ( 0.000000000000000000, 0.000000000000000000, 1.000000000000000000 ) ) ;
#603=DIRECTION ( 'NONE',  ( 1.000000000000000078E-15, -1.000000000000000083E-30, -1.000000000000000000 ) ) ;
#606=VECTOR ( 'NONE', #21628, 1000.000000000000000 ) ;
#608=LINE ( 'NONE', #29227, #58991 ) ;
#610=CARTESIAN_POINT ( 'NONE',  ( 98.34985889676497095, -31.65658483615705521, 260.9064586116816145 ) ) ;
#611=VERTEX_POINT ( 'NONE', #50480 ) ;
#613=CARTESIAN_POINT ( 'NONE',  ( 96.99510461011969653, -33.95209312647379818, 251.1127681330538337 ) ) ;
#614=CARTESIAN_POINT ( 'NONE',  ( 99.10138041440774259, -45.50374834597938900, 152.9899109901969894 ) ) ;
#615=CARTESIAN_POINT ( 'NONE',  ( 101.3723308891022157, -27.97080072976544685, 21.53562527591096298 ) ) ;
#616=LINE ( 'NONE', #21531, #83843 ) ;
#617=DIRECTION ( 'NONE',  ( 0.000000000000000000, 0.000000000000000000, -1.000000000000000000 ) ) ;
#618=CARTESIAN_POINT ( 'NONE',  ( 82.31780288914308130, -35.14744377621693161, 7.339349742403836530 ) ) ;
#619=EDGE_CURVE ( 'NONE', #6607, #89473, #22352, .T. ) ;
#620=CARTESIAN_POINT ( 'NONE',  ( 116.3231543710223121, -32.93883412237410369, 190.1356252759109680 ) ) ;
#623=VERTEX_POINT ( 'NONE', #20999 ) ;
#626=CARTESIAN_POINT ( 'NONE',  ( 102.7266122873206768, -44.08618886718738139, 161.5752769709339702 ) ) ;
#627=CARTESIAN_POINT ( 'NONE',  ( 193.5667039024483529, -48.82844715993410034, 300.4678068554149490 ) ) ;
#628=VERTEX_POINT ( 'NONE', #14642 ) ;
#630=CARTESIAN_POINT ( 'NONE',  ( 116.9962961068553113, -33.62662860631130712, 170.0670538473399631 ) ) ;
#631=CARTESIAN_POINT ( 'NONE',  ( 162.7131505118551047, -33.70561438051486647, 313.9678068554149490 ) ) ;
#633=CARTESIAN_POINT ( 'NONE',  ( 111.4434818239271436, -27.72135023051140834, 85.71645798515046977 ) ) ;
#636=CARTESIAN_POINT ( 'NONE',  ( 112.1775644307544013, -28.39036538331624726, 94.63848241876893042 ) ) ;
#637=ORIENTED_EDGE ( 'NONE', *, *, #20066, .T. ) ;
#640=VECTOR ( 'NONE', #25417, 1000.000000000000000 ) ;
#641=CARTESIAN_POINT ( 'NONE',  ( 115.2933828064165311, -33.43605939358163681, 50.56158330589693861 ) ) ;
#642=EDGE_CURVE ( 'NONE', #45558, #61357, #53228, .T. ) ;
#644=CARTESIAN_POINT ( 'NONE',  ( 107.5349099188610893, -47.08895302312297559, 188.6003871806719587 ) ) ;
#648=DIRECTION ( 'NONE',  ( 3.999999999999999995E-14, -1.000000000000000000, 4.100000000000000342E-29 ) ) ;
#649=DIRECTION ( 'NONE',  ( -2.900000000000000265E-14, 2.000000000000000155E-15, -1.000000000000000000 ) ) ;
#652=CARTESIAN_POINT ( 'NONE',  ( 114.0075736764523100, -28.98025818340840942, 114.4956252759109816 ) ) ;
#653=ORIENTED_EDGE ( 'NONE', *, *, #73659, .T. ) ;
#654=ORIENTED_EDGE ( 'NONE', *, *, #48753, .F. ) ;
#658=CARTESIAN_POINT ( 'NONE',  ( 102.0659489093014685, -27.97114065885338263, 130.4898948659551365 ) ) ;
#659=DIRECTION ( 'NONE',  ( 1.000000000000000000, 3.930900487435134677E-14, 0.000000000000000000 ) ) ;
#660=CARTESIAN_POINT ( 'NONE',  ( 112.1932604131138760, -43.70204218538222563, 180.8871379886389832 ) ) ;
#664=VECTOR ( 'NONE', #62185, 1000.000000000000000 ) ;
#666=CARTESIAN_POINT ( 'NONE',  ( 83.06670390244796920, -61.87844715994100397, 204.3338068554149913 ) ) ;
#667=VERTEX_POINT ( 'NONE', #62769 ) ;
#668=ORIENTED_EDGE ( 'NONE', *, *, #40170, .F. ) ;
#669=ORIENTED_EDGE ( 'NONE', *, *, #45253, .F. ) ;
#670=VECTOR ( 'NONE', #88324, 1000.000000000000000 ) ;
#671=CIRCLE ( 'NONE', #54333, 1.000000000000000888 ) ;
#674=EDGE_LOOP ( 'NONE', ( #44663, #41328, #16227, #43214 ) ) ;
#677=CARTESIAN_POINT ( 'NONE',  ( 104.8088860400571463, -27.60915219823615985, 236.6892023535159808 ) ) ;
#680=CYLINDRICAL_SURFACE ( 'NONE', #60979, 2.750000000000002665 ) ;
#682=ORIENTED_EDGE ( 'NONE', *, *, #19511, .F. ) ;
#685=EDGE_LOOP ( 'NONE', ( #78794, #39701 ) ) ;
#686=VERTEX_POINT ( 'NONE', #72289 ) ;
#689=CARTESIAN_POINT ( 'NONE',  ( 106.1481202089414637, -44.86820639808929201, 280.3052332267342877 ) ) ;
#690=CARTESIAN_POINT ( 'NONE',  ( 102.3026241189005532, -26.72939285866361914, 140.4422919425769578 ) ) ;
#691=CARTESIAN_POINT ( 'NONE',  ( 98.47671751366513604, -30.86049585540210671, 120.8499109901969604 ) ) ;
#692=CARTESIAN_POINT ( 'NONE',  ( 97.81168895331838087, -40.51742574516882200, 287.6356252759109680 ) ) ;
#693=ADVANCED_FACE ( 'NONE', ( #58200 ), #71402, .F. ) ;
#695=CARTESIAN_POINT ( 'NONE',  ( 109.9601702690906677, -48.22123515106449787, 238.7727681330539724 ) ) ;
#697=CARTESIAN_POINT ( 'NONE',  ( 142.8698897858160706, -0.9167816978817300289, 542.9756252759101471 ) ) ;
#699=DIRECTION ( 'NONE',  ( -1.000000000000000000, -4.299999999999999979E-14, -1.000000000000000078E-15 ) ) ;
#700=ORIENTED_EDGE ( 'NONE', *, *, #62620, .T. ) ;
#704=CARTESIAN_POINT ( 'NONE',  ( 115.7771187221315898, -31.78005509801509021, 135.2375939364552266 ) ) ;
#705=ORIENTED_EDGE ( 'NONE', *, *, #10479, .F. ) ;
#706=CARTESIAN_POINT ( 'NONE',  ( 98.45613130301506999, -42.66979608177781813, 126.8070538473389490 ) ) ;
#707=CARTESIAN_POINT ( 'NONE',  ( 120.6562317954107328, -37.89495061977655155, 302.6356252759109680 ) ) ;
#708=AXIS2_PLACEMENT_3D ( 'NONE', #61591, #89328, #88881 ) ;
#709=FACE_OUTER_BOUND ( 'NONE', #24326, .T. ) ;
#712=CARTESIAN_POINT ( 'NONE',  ( 102.0553424010809351, -45.40300992569917327, 57.15924359062986326 ) ) ;
#713=CARTESIAN_POINT ( 'NONE',  ( 100.8363305107023820, -45.83159080358277748, 238.1108633711489517 ) ) ;
#715=DIRECTION ( 'NONE',  ( 1.000000000000000078E-15, -1.000000000000000083E-30, -1.000000000000000000 ) ) ;
#718=FACE_OUTER_BOUND ( 'NONE', #75674, .T. ) ;
#721=CARTESIAN_POINT ( 'NONE',  ( 172.5664832912740110, 0.2215528400590013880, 318.9256252759120116 ) ) ;
#722=EDGE_LOOP ( 'NONE', ( #23623, #15028, #2356, #87724 ) ) ;
#724=CARTESIAN_POINT ( 'NONE',  ( 101.9611696646907433, -46.55956485693801028, 167.1832443235299763 ) ) ;
#725=CARTESIAN_POINT ( 'NONE',  ( 115.7285985590555129, -43.59543139906921283, 44.30514908543492680 ) ) ;
#726=CARTESIAN_POINT ( 'NONE',  ( 109.8676264040644526, -26.64249633179236909, 170.8613395616249591 ) ) ;
#727=CARTESIAN_POINT ( 'NONE',  ( 97.33784125381592389, -34.07106473404611080, 32.11479195932787434 ) ) ;
#728=DIRECTION ( 'NONE',  ( 1.000000000000000000, 0.000000000000000000, 9.462128050782575008E-16 ) ) ;
#731=DIRECTION ( 'NONE',  ( -0.000000000000000000, -0.000000000000000000, 1.000000000000000000 ) ) ;
#732=DIRECTION ( 'NONE',  ( 0.000000000000000000, 0.000000000000000000, 1.000000000000000000 ) ) ;
#733=VERTEX_POINT ( 'NONE', #85930 ) ;
#735=CIRCLE ( 'NONE', #25428, 2.117000000000000881 ) ;
#736=VECTOR ( 'NONE', #34922, 1000.000000000000000 ) ;
#741=ORIENTED_EDGE ( 'NONE', *, *, #80273, .F. ) ;
#743=CIRCLE ( 'NONE', #67453, 0.5000000000000004441 ) ;
#744=DIRECTION ( 'NONE',  ( 0.000000000000000000, -1.000000000000000000, 0.000000000000000000 ) ) ;
#746=CARTESIAN_POINT ( 'NONE',  ( 112.7479404651553949, -27.97242311821442584, 65.61848241876793963 ) ) ;
#747=DIRECTION ( 'NONE',  ( -0.9068632946707808618, 0.4214249218767877059, 0.000000000000000000 ) ) ;
#748=CARTESIAN_POINT ( 'NONE',  ( 165.6738106836045006, -28.98061976758433289, 237.4678068554150059 ) ) ;
#749=CARTESIAN_POINT ( 'NONE',  ( 113.7785824165150643, -44.76317014998476651, 189.1299109901969757 ) ) ;
#750=AXIS2_PLACEMENT_3D ( 'NONE', #24215, #59157, #1983 ) ;
#751=CARTESIAN_POINT ( 'NONE',  ( 97.36980136507975203, -37.22440909395530184, 270.7895626852197779 ) ) ;
#752=VERTEX_POINT ( 'NONE', #65897 ) ;
#757=DIRECTION ( 'NONE',  ( -2.999999999999999839E-15, 1.000000000000000000, -2.999999999999999900E-30 ) ) ;
#758=DIRECTION ( 'NONE',  ( -4.237773401492740281E-14, 1.000000000000000000, 0.000000000000000000 ) ) ;
#759=CARTESIAN_POINT ( 'NONE',  ( 97.31585577103271589, -39.30600539877234922, 162.5314611377484084 ) ) ;
#760=CARTESIAN_POINT ( 'NONE',  ( 112.1393456390005952, -28.01282277954388888, 74.65645860948981749 ) ) ;
#761=VECTOR ( 'NONE', #1970, 1000.000000000000000 ) ;
#763=CYLINDRICAL_SURFACE ( 'NONE', #81462, 13.16666666666669627 ) ;
#764=EDGE_CURVE ( 'NONE', #26493, #14667, #50932, .T. ) ;
#767=CARTESIAN_POINT ( 'NONE',  ( 96.71096103112829212, -32.93116260832594122, 21.03467289495897319 ) ) ;
#770=VERTEX_POINT ( 'NONE', #57750 ) ;
#772=DIRECTION ( 'NONE',  ( 0.000000000000000000, 1.000000000000000000, 0.000000000000000000 ) ) ;
#773=CARTESIAN_POINT ( 'NONE',  ( 41.56648329127398966, -18.82844715994071194, 258.9256252759120116 ) ) ;
#774=CARTESIAN_POINT ( 'NONE',  ( 100.6392880577574687, -41.80624237711439406, 89.67666179816296790 ) ) ;
#775=ADVANCED_FACE ( 'NONE', ( #86365 ), #65018, .T. ) ;
#776=B_SPLINE_CURVE_WITH_KNOTS ( 'NONE', 3,
 ( #76928, #55545, #48739, #1068, #42379, #61936, #14706, #7433, #21978, #76474, #29230, #13800, #610, #13359, #49645, #42826, #76023, #34679 ),
 .UNSPECIFIED., .F., .F.,
 ( 4, 2, 2, 2, 2, 2, 2, 2, 4 ),
 ( 0.000000000000000000, 0.06250000008602163426, 0.1250000001720432685, 0.1875000002580649028, 0.2500000003440865370, 0.3125000004301081713, 0.3750000005161298056, 0.4375000006021514398, 0.5000000006881730741 ),
 .UNSPECIFIED. ) ;
#777=AXIS2_PLACEMENT_3D ( 'NONE', #25052, #40017, #47268 ) ;
#778=VECTOR ( 'NONE', #6983, 1000.000000000000000 ) ;
#781=CARTESIAN_POINT ( 'NONE',  ( 116.3212776292271258, -32.94146857470711609, 44.13562527591097506 ) ) ;
#782=ORIENTED_EDGE ( 'NONE', *, *, #58682, .T. ) ;
#783=VERTEX_POINT ( 'NONE', #55463 ) ;
#784=DIRECTION ( 'NONE',  ( 1.000000000000000000, -1.000000000000000078E-15, 0.000000000000000000 ) ) ;
#788=CARTESIAN_POINT ( 'NONE',  ( 104.0080147226004925, -45.04654038386073012, 138.7272975916119435 ) ) ;
#790=CARTESIAN_POINT ( 'NONE',  ( 117.8979321085648877, -39.04567734339117635, 104.6708633711489824 ) ) ;
#791=DIRECTION ( 'NONE',  ( -0.7071067811865779928, 0.7071067811865171526, -7.071067811865785947E-16 ) ) ;
#792=EDGE_LOOP ( 'NONE', ( #87956, #8143, #70608, #66324, #45131 ) ) ;
#794=VECTOR ( 'NONE', #12046, 1000.000000000000000 ) ;
#795=TOROIDAL_SURFACE ( 'NONE', #87816, 11.75000000000000000, 2.125000000000000000 ) ;
#796=ORIENTED_EDGE ( 'NONE', *, *, #68724, .F. ) ;
#798=CIRCLE ( 'NONE', #70252, 3.000000000000002665 ) ;
#800=FACE_OUTER_BOUND ( 'NONE', #89670, .T. ) ;
#801=ORIENTED_EDGE ( 'NONE', *, *, #59322, .T. ) ;
#802=CARTESIAN_POINT ( 'NONE',  ( 97.51798386322114709, -31.03399775848789233, 280.8984824187687082 ) ) ;
#803=CARTESIAN_POINT ( 'NONE',  ( 106.9748050991984059, -47.17592283179411083, 183.5699109901969734 ) ) ;
#806=CARTESIAN_POINT ( 'NONE',  ( 101.9928297044944543, -45.44558343088166907, 128.1563855231297850 ) ) ;
#807=CARTESIAN_POINT ( 'NONE',  ( 113.8434436840914117, -28.76112614263219669, 135.5156252759109634 ) ) ;
#808=CYLINDRICAL_SURFACE ( 'NONE', #21880, 9.999999999999998224 ) ;
#809=EDGE_CURVE ( 'NONE', #84681, #23299, #69575, .T. ) ;
#810=VERTEX_POINT ( 'NONE', #35943 ) ;
#812=CARTESIAN_POINT ( 'NONE',  ( 144.8664832912740223, -71.52944715994085811, 394.9756252759100903 ) ) ;
#814=DIRECTION ( 'NONE',  ( 0.000000000000000000, 0.000000000000000000, 1.000000000000000000 ) ) ;
#815=AXIS2_PLACEMENT_3D ( 'NONE', #55356, #35825, #83549 ) ;
#816=ORIENTED_EDGE ( 'NONE', *, *, #29499, .T. ) ;
#819=CARTESIAN_POINT ( 'NONE',  ( 99.76197604230684135, -44.21744263965017296, 21.96133956162593748 ) ) ;
#821=CIRCLE ( 'NONE', #18255, 0.4999999999999976685 ) ;
#822=PLANE ( 'NONE',  #31862 ) ;
#823=CARTESIAN_POINT ( 'NONE',  ( 105.7154773393596372, -46.72385839336168090, 73.46895860995762462 ) ) ;
#824=CARTESIAN_POINT ( 'NONE',  ( 104.7983354006062058, -46.84845355260645761, 27.38895860924495196 ) ) ;
#825=CARTESIAN_POINT ( 'NONE',  ( 97.53201903585136279, -39.74950769135491413, 111.5705769356003287 ) ) ;
#826=CARTESIAN_POINT ( 'NONE',  ( 117.5859182825551983, -33.41202194707546624, 125.0575300378149706 ) ) ;
#828=CARTESIAN_POINT ( 'NONE',  ( 172.5664832912740110, -9.303447159940999356, 201.0426252759120018 ) ) ;
#829=VERTEX_POINT ( 'NONE', #27783 ) ;
#831=FACE_BOUND ( 'NONE', #32263, .T. ) ;
#833=VECTOR ( 'NONE', #85571, 1000.000000000000000 ) ;
#834=VERTEX_POINT ( 'NONE', #56373 ) ;
#836=CARTESIAN_POINT ( 'NONE',  ( 108.3716159000525039, -47.75258262280652843, 162.6822919425769669 ) ) ;
#837=VERTEX_POINT ( 'NONE', #15063 ) ;
#838=CARTESIAN_POINT ( 'NONE',  ( 41.56670390244688207, -36.32844715994109208, 193.9678068554150911 ) ) ;
#839=CARTESIAN_POINT ( 'NONE',  ( 114.6212291911790402, -29.51397259194560263, 230.4327681330539690 ) ) ;
#840=CARTESIAN_POINT ( 'NONE',  ( 99.26130681012091372, -43.75918647830361863, 52.90991099019698396 ) ) ;
#842=DIRECTION ( 'NONE',  ( -1.000000000000000000, -4.299999999999999979E-14, 1.230419385187874527E-43 ) ) ;
#843=VECTOR ( 'NONE', #71770, 1000.000000000000000 ) ;
#844=FACE_OUTER_BOUND ( 'NONE', #84054, .T. ) ;
#846=AXIS2_PLACEMENT_3D ( 'NONE', #32859, #19245, #80142 ) ;
#848=ORIENTED_EDGE ( 'NONE', *, *, #1891, .F. ) ;
#850=CARTESIAN_POINT ( 'NONE',  ( 41.56648329127499153, -27.82844715994070484, 83.67562527591201160 ) ) ;
#851=CARTESIAN_POINT ( 'NONE',  ( 115.7761331719916171, -31.00018137778016936, 250.2899109901966028 ) ) ;
#852=CARTESIAN_POINT ( 'NONE',  ( 33.91903122894440514, -35.91149509761246605, 193.9678068554150911 ) ) ;
#853=CARTESIAN_POINT ( 'NONE',  ( 136.1684221027214790, -16.94667169169761678, 2.376609173410517695 ) ) ;
#854=CARTESIAN_POINT ( 'NONE',  ( 125.0664851986225159, -56.72944715994101728, 14.92562527591098842 ) ) ;
#855=DIRECTION ( 'NONE',  ( -1.000000000000000000, 0.000000000000000000, 0.000000000000000000 ) ) ;
#856=DIRECTION ( 'NONE',  ( -7.723290606088049820E-15, 0.000000000000000000, -1.000000000000000000 ) ) ;
#857=CARTESIAN_POINT ( 'NONE',  ( 109.6484814735558189, -46.85267042889636002, 47.77562527591094721 ) ) ;
#858=ORIENTED_EDGE ( 'NONE', *, *, #68817, .T. ) ;
#859=AXIS2_PLACEMENT_3D ( 'NONE', #84695, #41975, #69709 ) ;
#860=ORIENTED_EDGE ( 'NONE', *, *, #37022, .F. ) ;
#861=VECTOR ( 'NONE', #43079, 1000.000000000000000 ) ;
#862=EDGE_CURVE ( 'NONE', #52251, #6347, #68681, .T. ) ;
#863=DIRECTION ( 'NONE',  ( 1.000000000000000000, 4.237773401492740281E-14, 0.000000000000000000 ) ) ;
#864=AXIS2_PLACEMENT_3D ( 'NONE', #1232, #17420, #79664 ) ;
#865=CARTESIAN_POINT ( 'NONE',  ( 97.81483072311490901, -40.51614641965803543, 17.63529977666319937 ) ) ;
#867=CARTESIAN_POINT ( 'NONE',  ( 101.6507727546967743, -27.01955209951630010, 251.4813395616246510 ) ) ;
#868=CARTESIAN_POINT ( 'NONE',  ( 193.0371591254586860, -47.82818131005411999, 117.4678068554150627 ) ) ;
#870=CARTESIAN_POINT ( 'NONE',  ( 116.7039036015865037, -32.90075090702275418, 95.13943479971997874 ) ) ;
#872=CARTESIAN_POINT ( 'NONE',  ( 103.2786946225953244, -27.47457500332495783, 21.38560984476657367 ) ) ;
#873=EDGE_CURVE ( 'NONE', #43897, #27298, #82327, .T. ) ;
#876=ADVANCED_FACE ( 'NONE', ( #524 ), #35485, .F. ) ;
#878=ORIENTED_EDGE ( 'NONE', *, *, #89050, .T. ) ;
#882=CARTESIAN_POINT ( 'NONE',  ( 106.2775494337459037, -46.09182447052010190, 258.9292023535161889 ) ) ;
#884=CARTESIAN_POINT ( 'NONE',  ( 116.7951252649886555, -39.38782981628543922, 193.6147919404536992 ) ) ;
#888=DIRECTION ( 'NONE',  ( 1.000000000000000000, -1.000000000000000078E-15, 0.000000000000000000 ) ) ;
#890=ORIENTED_EDGE ( 'NONE', *, *, #36462, .T. ) ;
#891=DIRECTION ( 'NONE',  ( 0.1858654558203195195, -0.9825752044157765042, 0.000000000000000000 ) ) ;
#893=VERTEX_POINT ( 'NONE', #76385 ) ;
#894=CARTESIAN_POINT ( 'NONE',  ( 110.3719962439868425, -47.27708535874812412, 52.80610146638697699 ) ) ;
#895=ORIENTED_EDGE ( 'NONE', *, *, #68923, .F. ) ;
#896=CARTESIAN_POINT ( 'NONE',  ( 101.0819131387675611, -42.86434890131523900, 21.38384839950496641 ) ) ;
#897=ADVANCED_FACE ( 'NONE', ( #76834 ), #14164, .T. ) ;
#898=CYLINDRICAL_SURFACE ( 'NONE', #14088, 4.749999999999976907 ) ;
#899=CARTESIAN_POINT ( 'NONE',  ( 116.4500618263486444, -39.48841239489308919, 183.5984824187689526 ) ) ;
#902=DIRECTION ( 'NONE',  ( 1.000000000000000000, 4.163336342344333240E-14, 0.000000000000000000 ) ) ;
#904=CARTESIAN_POINT ( 'NONE',  ( 109.2209341577003698, -48.43284210327079364, 273.7213395616253706 ) ) ;
#906=ORIENTED_EDGE ( 'NONE', *, *, #59103, .T. ) ;
#907=CARTESIAN_POINT ( 'NONE',  ( 48.45959712129000252, -28.98061976758940617, -5.074374724088000832 ) ) ;
#909=CARTESIAN_POINT ( 'NONE',  ( 117.9015171282527916, -39.13767059441630636, 99.64038718067195077 ) ) ;
#912=DIRECTION ( 'NONE',  ( 0.000000000000000000, 0.000000000000000000, -1.000000000000000000 ) ) ;
#914=VERTEX_POINT ( 'NONE', #980 ) ;
#915=DIRECTION ( 'NONE',  ( -0.7071067811865475727, 0.7071067811865475727, 0.000000000000000000 ) ) ;
#918=CARTESIAN_POINT ( 'NONE',  ( 50.56670390244759972, -18.82844715994099971, -5.074374724088000832 ) ) ;
#919=FACE_OUTER_BOUND ( 'NONE', #24563, .T. ) ;
#920=CARTESIAN_POINT ( 'NONE',  ( 100.4792253034169960, -27.85352395805916359, 31.59657765686396758 ) ) ;
#923=ORIENTED_EDGE ( 'NONE', *, *, #29698, .F. ) ;
#926=VECTOR ( 'NONE', #24690, 1000.000000000000000 ) ;
#927=DIRECTION ( 'NONE',  ( 1.000000000000000000, 4.299999999999999979E-14, 1.000000000000000078E-15 ) ) ;
#928=ORIENTED_EDGE ( 'NONE', *, *, #2414, .T. ) ;
#929=EDGE_LOOP ( 'NONE', ( #3602, #48230, #57007, #56048 ) ) ;
#932=CARTESIAN_POINT ( 'NONE',  ( 25.56670390244797275, -48.82844715994099971, 293.2178068554150627 ) ) ;
#933=VECTOR ( 'NONE', #68373, 1000.000000000000000 ) ;
#934=CARTESIAN_POINT ( 'NONE',  ( 19.56648329127400032, 0.2215528400590083269, 323.8756252759109202 ) ) ;
#935=CARTESIAN_POINT ( 'NONE',  ( 97.12554568906318764, -37.99677948043573394, 16.42730063705512578 ) ) ;
#939=CARTESIAN_POINT ( 'NONE',  ( 98.04376085404715013, -35.95281974173802553, 185.6686103042669629 ) ) ;
#941=CARTESIAN_POINT ( 'NONE',  ( 102.5390659930443746, -27.28968240376552501, 95.43276813305395478 ) ) ;
#943=CARTESIAN_POINT ( 'NONE',  ( 132.1198940698264153, -20.67261125153088841, 7.590611884327144843 ) ) ;
#944=VERTEX_POINT ( 'NONE', #22782 ) ;
#946=ORIENTED_EDGE ( 'NONE', *, *, #71953, .T. ) ;
#947=CARTESIAN_POINT ( 'NONE',  ( 116.3212776292270973, -32.94146857470704504, 49.13562527591097506 ) ) ;
#948=EDGE_LOOP ( 'NONE', ( #39295, #50309, #44340, #82075, #28155, #33375, #36970, #41977, #80232, #84882, #47381, #79009, #7396, #61225 ) ) ;
#955=CARTESIAN_POINT ( 'NONE',  ( 110.4638204314202881, -47.27238515144596676, 57.83657765686300678 ) ) ;
#956=CARTESIAN_POINT ( 'NONE',  ( 116.3201356630459884, -32.94258242523766711, 69.13562527591093954 ) ) ;
#959=CARTESIAN_POINT ( 'NONE',  ( 131.8592257737627449, -17.08568546291111190, 2.471387922376312218 ) ) ;
#961=CARTESIAN_POINT ( 'NONE',  ( 77.31648329127399677, -36.72944715994107412, 14.92562527591094046 ) ) ;
#962=CARTESIAN_POINT ( 'NONE',  ( 104.4899545134221910, -26.97880756921290413, 155.2814586042531459 ) ) ;
#963=CARTESIAN_POINT ( 'NONE',  ( 107.0664832912739399, -49.89611382660763184, 308.7195067599733420 ) ) ;
#964=CARTESIAN_POINT ( 'NONE',  ( 103.1973475860487639, -46.47157139977531415, 113.2756252759109827 ) ) ;
#965=CARTESIAN_POINT ( 'NONE',  ( 162.9033555647770015, -33.89581943344391135, -5.074374724088000832 ) ) ;
#966=CARTESIAN_POINT ( 'NONE',  ( 48.86082318535700608, -35.55794170701751256, -5.074374724088000832 ) ) ;
#971=EDGE_CURVE ( 'NONE', #54474, #73652, #20012, .T. ) ;
#973=EDGE_CURVE ( 'NONE', #19682, #50715, #60572, .T. ) ;
#974=CARTESIAN_POINT ( 'NONE',  ( 98.36735121233628831, -42.37464764417345719, 142.7965776568629508 ) ) ;
#976=VERTEX_POINT ( 'NONE', #80758 ) ;
#977=EDGE_CURVE ( 'NONE', #57623, #62556, #57271, .T. ) ;
#978=CARTESIAN_POINT ( 'NONE',  ( 115.6373213143783545, -30.77082676042347487, 275.3099109901965562 ) ) ;
#979=CARTESIAN_POINT ( 'NONE',  ( 194.0371591254572934, -24.42818131005417825, 300.4678068554149490 ) ) ;
#980=CARTESIAN_POINT ( 'NONE',  ( 51.03742451361310373, -23.42844715994068849, 193.9678068554150911 ) ) ;
#982=CARTESIAN_POINT ( 'NONE',  ( 80.06648329127399677, -8.350947159940998787, 293.6356252759119911 ) ) ;
#986=VECTOR ( 'NONE', #84387, 1000.000000000000000 ) ;
#987=CARTESIAN_POINT ( 'NONE',  ( 116.1939227058878714, -40.33550099034470549, 193.5270538473399426 ) ) ;
#988=ORIENTED_EDGE ( 'NONE', *, *, #73179, .F. ) ;
#989=ORIENTED_EDGE ( 'NONE', *, *, #13021, .F. ) ;
#990=CARTESIAN_POINT ( 'NONE',  ( 107.8658914883948512, -27.90296577952642210, 151.4358690201829631 ) ) ;
#992=VECTOR ( 'NONE', #4749, 1000.000000000000000 ) ;
#993=CARTESIAN_POINT ( 'NONE',  ( 51.42025729302798709, -31.94127993907680718, -5.074374724088000832 ) ) ;
#994=AXIS2_PLACEMENT_3D ( 'NONE', #60875, #53588, #6362 ) ;
#995=CARTESIAN_POINT ( 'NONE',  ( 117.6440909798951253, -33.30491947301820232, 280.0756252759109657 ) ) ;
#997=ADVANCED_FACE ( 'NONE', ( #45744 ), #73028, .F. ) ;
#999=CARTESIAN_POINT ( 'NONE',  ( 107.3241674272228892, -25.27320757387406402, 321.5865679059475610 ) ) ;
#1001=CARTESIAN_POINT ( 'NONE',  ( 131.0667039024480118, -67.87844715994100397, 207.5838068554149913 ) ) ;
#1002=CARTESIAN_POINT ( 'NONE',  ( 112.4430884738663821, -45.67687932769439385, 238.0070538473389377 ) ) ;
#1003=DIRECTION ( 'NONE',  ( 1.000000000000000078E-15, -1.000000000000000083E-30, -1.000000000000000000 ) ) ;
#1007=CARTESIAN_POINT ( 'NONE',  ( 99.04406184276894010, -42.84125761936532939, 86.84395860719635607 ) ) ;
#1008=CARTESIAN_POINT ( 'NONE',  ( 82.81058719979510840, -18.91414947189774409, 6.758631288823465866 ) ) ;
#1009=DIRECTION ( 'NONE',  ( -0.9254794337955620787, -0.3787978585227822492, 0.000000000000000000 ) ) ;
#1010=FACE_OUTER_BOUND ( 'NONE', #74696, .T. ) ;
#1011=VECTOR ( 'NONE', #20035, 1000.000000000000000 ) ;
#1012=CARTESIAN_POINT ( 'NONE',  ( 114.3402351757609097, -43.26825200597433962, 34.24419670448197905 ) ) ;
#1014=CLOSED_SHELL ( 'NONE', ( #3243, #64982, #6193, #64038, #15469, #48042, #25476 ) ) ;
#1015=ORIENTED_EDGE ( 'NONE', *, *, #78887, .F. ) ;
#1016=CARTESIAN_POINT ( 'NONE',  ( 112.1383799374394670, -26.85658479980368440, 15.71086337114896381 ) ) ;
#1017=DIRECTION ( 'NONE',  ( 0.000000000000000000, 1.000000000000000000, 0.000000000000000000 ) ) ;
#1019=CARTESIAN_POINT ( 'NONE',  ( 112.4118754778678380, -46.40445981238691076, 252.9661014663871583 ) ) ;
#1021=B_SPLINE_CURVE_WITH_KNOTS ( 'NONE', 3,
 ( #71671, #64846, #73436, #24410, #51194, #87082, #18468, #18022, #72989, #59353, #45705, #3069, #87525, #9885, #58898, #73886, #65723, #17148 ),
 .UNSPECIFIED., .F., .F.,
 ( 4, 2, 2, 2, 2, 2, 2, 2, 4 ),
 ( 0.000000000000000000, 0.06249843191113654828, 0.1249968638222730966, 0.1874952957334096448, 0.2499937276445461931, 0.3124921595556827691, 0.3749905914668192897, 0.4374890233779558102, 0.4999874552890923862 ),
 .UNSPECIFIED. ) ;
#1022=CARTESIAN_POINT ( 'NONE',  ( 77.74802179993278628, -38.20859666167125113, 7.273989459505274091 ) ) ;
#1024=DIRECTION ( 'NONE',  ( -4.237773401492740281E-14, 1.000000000000000000, 0.000000000000000000 ) ) ;
#1025=CARTESIAN_POINT ( 'NONE',  ( 98.46239236780679960, -37.66247686286469332, 79.21856656006798403 ) ) ;
#1026=CARTESIAN_POINT ( 'NONE',  ( 102.0405519839503086, -46.59986864225058412, 168.2137205140059564 ) ) ;
#1030=FACE_OUTER_BOUND ( 'NONE', #20809, .T. ) ;
#1031=ORIENTED_EDGE ( 'NONE', *, *, #56201, .F. ) ;
#1032=ORIENTED_EDGE ( 'NONE', *, *, #44128, .F. ) ;
#1033=CARTESIAN_POINT ( 'NONE',  ( 107.0667039024482818, -36.72944715994103149, 249.5838068554170093 ) ) ;
#1037=CARTESIAN_POINT ( 'NONE',  ( 112.1857315011839802, -29.85591823435125747, 103.9895626852199655 ) ) ;
#1038=CARTESIAN_POINT ( 'NONE',  ( 118.1310582692406257, -36.20923403681121044, 268.8518157521014587 ) ) ;
#1039=CARTESIAN_POINT ( 'NONE',  ( 194.5667039024482960, -47.82844715993405771, 300.4678068554149490 ) ) ;
#1040=DIRECTION ( 'NONE',  ( 0.000000000000000000, 0.000000000000000000, -1.000000000000000000 ) ) ;
#1041=ADVANCED_FACE ( 'NONE', ( #85016 ), #1147, .F. ) ;
#1044=DIRECTION ( 'NONE',  ( -1.000000000000000000, -2.756263715554006823E-15, 0.000000000000000000 ) ) ;
#1046=CYLINDRICAL_SURFACE ( 'NONE', #15910, 2.999999999999999112 ) ;
#1048=CARTESIAN_POINT ( 'NONE',  ( 117.2073019650709256, -38.89799087863980276, 108.6708633711499772 ) ) ;
#1049=EDGE_CURVE ( 'NONE', #77857, #70798, #9839, .T. ) ;
#1050=CARTESIAN_POINT ( 'NONE',  ( 98.26918992425659383, -28.71468409831775404, 80.73848241876795839 ) ) ;
#1052=CARTESIAN_POINT ( 'NONE',  ( 99.30039714715974242, -28.79844535499942637, 270.7051490854347549 ) ) ;
#1055=CARTESIAN_POINT ( 'NONE',  ( 98.83914287153486100, -29.34771585412822859, 235.7565776568629872 ) ) ;
#1057=CIRCLE ( 'NONE', #69269, 2.500000000000002220 ) ;
#1059=PLANE ( 'NONE',  #8576 ) ;
#1061=DIRECTION ( 'NONE',  ( 0.000000000000000000, 0.000000000000000000, 1.000000000000000000 ) ) ;
#1066=DIRECTION ( 'NONE',  ( 0.000000000000000000, 0.000000000000000000, 1.000000000000000000 ) ) ;
#1068=CARTESIAN_POINT ( 'NONE',  ( 113.2454986924611831, -28.75867294014850017, 259.5522919431510331 ) ) ;
#1069=VERTEX_POINT ( 'NONE', #73932 ) ;
#1070=CARTESIAN_POINT ( 'NONE',  ( 116.3212776292296127, -32.94146857471318413, 9.635625275910941312 ) ) ;
#1071=CARTESIAN_POINT ( 'NONE',  ( 110.9007760261032871, -26.97308707819648887, 269.7784824187680783 ) ) ;
#1072=CARTESIAN_POINT ( 'NONE',  ( 113.8434436840914117, -28.76112614263219669, 135.5156252759109634 ) ) ;
#1073=CARTESIAN_POINT ( 'NONE',  ( 97.08395347075709481, -39.80944164022105980, 17.56419670448195092 ) ) ;
#1075=DIRECTION ( 'NONE',  ( 0.000000000000000000, 0.000000000000000000, -1.000000000000000000 ) ) ;
#1077=CARTESIAN_POINT ( 'NONE',  ( 82.81181082189971221, -36.54506369576082392, 6.756870619999560290 ) ) ;
#1078=CARTESIAN_POINT ( 'NONE',  ( 80.06648329127399677, -8.729447159940999512, 308.6356252759119911 ) ) ;
#1081=EDGE_CURVE ( 'NONE', #311, #15646, #50008, .T. ) ;
#1083=ORIENTED_EDGE ( 'NONE', *, *, #51612, .F. ) ;
#1084=EDGE_CURVE ( 'NONE', #81584, #10240, #66415, .T. ) ;
#1085=CARTESIAN_POINT ( 'NONE',  ( 115.8434954054525292, -34.49858887834006538, 168.4590864947439854 ) ) ;
#1086=DIRECTION ( 'NONE',  ( -4.299999999999999979E-14, 1.000000000000000000, -4.400000000000000367E-29 ) ) ;
#1087=ORIENTED_EDGE ( 'NONE', *, *, #37246, .T. ) ;
#1088=CARTESIAN_POINT ( 'NONE',  ( 69.25757238336807120, -1.944390235229864539, 361.9756252759101471 ) ) ;
#1089=EDGE_CURVE ( 'NONE', #82238, #52360, #8707, .T. ) ;
#1090=CARTESIAN_POINT ( 'NONE',  ( 107.6517678568360452, -47.10594642807011923, 148.6213395616249784 ) ) ;
#1092=CARTESIAN_POINT ( 'NONE',  ( 100.9550073947607416, -28.70676405461405878, 150.5943758343188676 ) ) ;
#1095=EDGE_CURVE ( 'NONE', #23005, #54148, #34462, .T. ) ;
#1097=CARTESIAN_POINT ( 'NONE',  ( 97.87212830949604836, -31.93334231290197067, 90.93181575210196854 ) ) ;
#1098=AXIS2_PLACEMENT_3D ( 'NONE', #46225, #82143, #67591 ) ;
#1100=EDGE_LOOP ( 'NONE', ( #17602, #31733, #14707, #68615 ) ) ;
#1101=VECTOR ( 'NONE', #3865, 1000.000000000000000 ) ;
#1103=CARTESIAN_POINT ( 'NONE',  ( 104.4962338114797262, -45.76661171243296877, 63.79967854399193072 ) ) ;
#1105=CARTESIAN_POINT ( 'NONE',  ( 97.38117110781249153, -35.36630255995241612, 177.2156252759109805 ) ) ;
#1106=CARTESIAN_POINT ( 'NONE',  ( 117.0718954832505148, -35.46248234554022360, 38.92729194342982879 ) ) ;
#1107=CARTESIAN_POINT ( 'NONE',  ( 98.35008263532775175, -31.65619168214967871, 55.90512834145738452 ) ) ;
#1109=ADVANCED_FACE ( 'NONE', ( #1881 ), #58941, .F. ) ;
#1111=DIRECTION ( 'NONE',  ( 0.000000000000000000, 0.000000000000000000, 1.000000000000000000 ) ) ;
#1112=DIRECTION ( 'NONE',  ( 4.299999999999999979E-14, -1.000000000000000000, 0.000000000000000000 ) ) ;
#1113=CARTESIAN_POINT ( 'NONE',  ( 96.05093434719793777, -37.29646042206077539, 121.3794347997209684 ) ) ;
#1114=ORIENTED_EDGE ( 'NONE', *, *, #42132, .T. ) ;
#1115=EDGE_LOOP ( 'NONE', ( #85274, #9415 ) ) ;
#1120=FACE_OUTER_BOUND ( 'NONE', #51217, .T. ) ;
#1122=CARTESIAN_POINT ( 'NONE',  ( 102.0328030160422230, -28.93470572416599751, 218.3509475124479593 ) ) ;
#1123=VECTOR ( 'NONE', #70345, 1000.000000000000000 ) ;
#1126=CARTESIAN_POINT ( 'NONE',  ( 116.3283240494693160, -32.94276334974209419, 64.13562527591099638 ) ) ;
#1127=CARTESIAN_POINT ( 'NONE',  ( 128.2586590417343473, -60.54728653293321372, 394.9756252759100903 ) ) ;
#1128=ORIENTED_EDGE ( 'NONE', *, *, #82632, .T. ) ;
#1132=CARTESIAN_POINT ( 'NONE',  ( 172.5664832912740110, 0.2215528400590013880, 261.0426252759119734 ) ) ;
#1133=ORIENTED_EDGE ( 'NONE', *, *, #3086, .T. ) ;
#1134=VERTEX_POINT ( 'NONE', #61189 ) ;
#1135=CARTESIAN_POINT ( 'NONE',  ( 80.06648281188262217, -21.47944715903999224, 8.225259175037979986 ) ) ;
#1136=CARTESIAN_POINT ( 'NONE',  ( 105.1749981762835802, -28.04127050161159218, 256.6787261630399826 ) ) ;
#1138=CARTESIAN_POINT ( 'NONE',  ( 105.7154763623905325, -46.72385826930020158, 272.4689585321721097 ) ) ;
#1139=ORIENTED_EDGE ( 'NONE', *, *, #52392, .F. ) ;
#1140=VECTOR ( 'NONE', #9711, 1000.000000000000000 ) ;
#1142=EDGE_CURVE ( 'NONE', #55592, #16504, #81665, .T. ) ;
#1143=FACE_OUTER_BOUND ( 'NONE', #20323, .T. ) ;
#1145=VERTEX_POINT ( 'NONE', #33486 ) ;
#1146=ORIENTED_EDGE ( 'NONE', *, *, #46506, .T. ) ;
#1147=CONICAL_SURFACE ( 'NONE', #80912, 1.571100913904360796, 1.047197551196591414 ) ;
#1148=DIRECTION ( 'NONE',  ( 1.000000000000000078E-15, 1.000000000000000083E-30, -1.000000000000000000 ) ) ;
#1149=EDGE_LOOP ( 'NONE', ( #68518, #70003, #30605, #37059 ) ) ;
#1151=EDGE_CURVE ( 'NONE', #29300, #69198, #38864, .T. ) ;
#1152=CARTESIAN_POINT ( 'NONE',  ( 98.99928044157054785, -35.48447157832033128, 264.0223760838769635 ) ) ;
#1153=CARTESIAN_POINT ( 'NONE',  ( 101.9737040637596124, -45.89197751792076474, 187.1727681330539781 ) ) ;
#1154=CARTESIAN_POINT ( 'NONE',  ( 102.3122812202564376, -27.43633205498510108, 120.4527681330539792 ) ) ;
#1155=LINE ( 'NONE', #58661, #6547 ) ;
#1156=CARTESIAN_POINT ( 'NONE',  ( 193.0371591254586008, -47.82818131005421236, 193.9678068554150343 ) ) ;
#1157=CARTESIAN_POINT ( 'NONE',  ( 117.4126858048608000, -35.18755665659306686, 214.9441967044829767 ) ) ;
#1161=DIRECTION ( 'NONE',  ( 0.000000000000000000, 0.000000000000000000, -1.000000000000000000 ) ) ;
#1163=EDGE_LOOP ( 'NONE', ( #74376, #83384, #75990, #89814 ) ) ;
#1166=CIRCLE ( 'NONE', #18523, 2.117000000000000881 ) ;
#1167=DIRECTION ( 'NONE',  ( 1.000000000000000000, 4.443626637970137948E-14, 0.000000000000000000 ) ) ;
#1169=ORIENTED_EDGE ( 'NONE', *, *, #25991, .T. ) ;
#1170=CARTESIAN_POINT ( 'NONE',  ( 117.2382404677042729, -39.01746902538002360, 148.6499109901969859 ) ) ;
#1173=DIRECTION ( 'NONE',  ( 0.000000000000000000, 0.000000000000000000, -1.000000000000000000 ) ) ;
#1174=CARTESIAN_POINT ( 'NONE',  ( 142.8824340801165249, -74.11588153691421610, 540.9756252759101471 ) ) ;
#1176=CARTESIAN_POINT ( 'NONE',  ( 115.7579298488886224, -31.01215564512775558, 250.2899109901966028 ) ) ;
#1183=DIRECTION ( 'NONE',  ( -0.9254794337955620787, -0.3787978585227822492, 0.000000000000000000 ) ) ;
#1184=CARTESIAN_POINT ( 'NONE',  ( 110.9088526855213388, -26.95253601363527807, 269.7784824187680783 ) ) ;
#1186=PLANE ( 'NONE',  #3121 ) ;
#1187=CARTESIAN_POINT ( 'NONE',  ( 97.65468660891812647, -41.26425114427870255, 171.6841967044819626 ) ) ;
#1188=CARTESIAN_POINT ( 'NONE',  ( 115.6731346838618464, -43.66482979471727077, 39.27467289495895386 ) ) ;
#1189=CARTESIAN_POINT ( 'NONE',  ( 112.2265052985635236, -45.83807782717671131, 208.9870538473389558 ) ) ;
#1190=VECTOR ( 'NONE', #44932, 1000.000000000000000 ) ;
#1191=CARTESIAN_POINT ( 'NONE',  ( 105.7995183767597211, -26.72403497849174059, 31.17729195139352427 ) ) ;
#1192=FACE_OUTER_BOUND ( 'NONE', #57543, .T. ) ;
#1193=CYLINDRICAL_SURFACE ( 'NONE', #21742, 2.030000000001311644 ) ;
#1194=CARTESIAN_POINT ( 'NONE',  ( 51.06670390244799762, -33.35206098992630075, -5.074374724088000832 ) ) ;
#1195=DIRECTION ( 'NONE',  ( -3.999999999999999995E-14, 1.000000000000000000, -4.100000000000000342E-29 ) ) ;
#1200=CIRCLE ( 'NONE', #15728, 6.571100913904396990 ) ;
#1203=EDGE_CURVE ( 'NONE', #37163, #33963, #54349, .T. ) ;
#1205=CYLINDRICAL_SURFACE ( 'NONE', #12500, 10.00000000000000711 ) ;
#1206=ORIENTED_EDGE ( 'NONE', *, *, #46372, .T. ) ;
#1207=CARTESIAN_POINT ( 'NONE',  ( 101.0787430638809496, -27.46603582566407908, 66.54514908543495721 ) ) ;
#1208=CARTESIAN_POINT ( 'NONE',  ( 63.03715912545643363, -24.42818131006017168, 129.9678068554150911 ) ) ;
#1212=CARTESIAN_POINT ( 'NONE',  ( 117.8238795360118445, -33.99523349031771602, 165.0365776568629315 ) ) ;
#1216=CARTESIAN_POINT ( 'NONE',  ( 116.1088647163993386, -36.23144265813309772, 273.3048007804578674 ) ) ;
#1218=ORIENTED_EDGE ( 'NONE', *, *, #74092, .F. ) ;
#1219=ORIENTED_EDGE ( 'NONE', *, *, #23918, .F. ) ;
#1221=CARTESIAN_POINT ( 'NONE',  ( 116.3212776292267989, -32.94146857470629186, 109.1356252759109680 ) ) ;
#1224=CARTESIAN_POINT ( 'NONE',  ( 109.7248659172085468, -27.00080517855199602, 74.86479194292134309 ) ) ;
#1227=EDGE_CURVE ( 'NONE', #46193, #83432, #400, .T. ) ;
#1228=CARTESIAN_POINT ( 'NONE',  ( 51.42025729304100423, -33.70561438051981185, 313.9678068554150059 ) ) ;
#1229=CARTESIAN_POINT ( 'NONE',  ( 168.0371591254546217, -48.62818131005519007, 129.9678068554150059 ) ) ;
#1230=EDGE_CURVE ( 'NONE', #47280, #23292, #33932, .T. ) ;
#1231=CARTESIAN_POINT ( 'NONE',  ( 114.0759046727996093, -46.25395340493279406, 33.08133956162495792 ) ) ;
#1232=CARTESIAN_POINT ( 'NONE',  ( 41.56648329127499153, -32.07844715994070839, 18.92562527591200094 ) ) ;
#1233=VERTEX_POINT ( 'NONE', #53904 ) ;
#1234=CARTESIAN_POINT ( 'NONE',  ( 109.7248663305506824, -27.00080529972676402, 269.8647919088584786 ) ) ;
#1235=CIRCLE ( 'NONE', #78146, 5.599999999999994316 ) ;
#1237=CARTESIAN_POINT ( 'NONE',  ( 99.02147155855831784, -38.11057432192225747, 89.27951894101998676 ) ) ;
#1238=VECTOR ( 'NONE', #55571, 1000.000000000000000 ) ;
#1239=DIRECTION ( 'NONE',  ( 0.000000000000000000, 0.000000000000000000, -1.000000000000000000 ) ) ;
#1240=FACE_OUTER_BOUND ( 'NONE', #74366, .T. ) ;
#1243=CARTESIAN_POINT ( 'NONE',  ( 116.3195061320206207, -32.94150711290046729, 139.1356252759109680 ) ) ;
#1244=ORIENTED_EDGE ( 'NONE', *, *, #63545, .T. ) ;
#1246=CARTESIAN_POINT ( 'NONE',  ( 113.3535730310440215, -29.74740315656111989, 155.9368214011359726 ) ) ;
#1249=CARTESIAN_POINT ( 'NONE',  ( 117.6173583669683040, -42.17933576662011319, 89.44705384733997278 ) ) ;
#1250=LINE ( 'NONE', #55720, #50250 ) ;
#1253=EDGE_LOOP ( 'NONE', ( #76808, #30804, #21641, #56351 ) ) ;
#1255=ADVANCED_FACE ( 'NONE', ( #13946 ), #5345, .T. ) ;
#1258=ORIENTED_EDGE ( 'NONE', *, *, #10802, .T. ) ;
#1259=CARTESIAN_POINT ( 'NONE',  ( 111.0379167980823496, -47.01981040405703993, 17.85753003781598380 ) ) ;
#1260=CARTESIAN_POINT ( 'NONE',  ( 109.3632651814324817, -25.89385771158341853, 180.9222919425779708 ) ) ;
#1262=LINE ( 'NONE', #28968, #50442 ) ;
#1263=CARTESIAN_POINT ( 'NONE',  ( 117.5808906079046352, -33.32045621506634347, 130.0880062282919880 ) ) ;
#1264=DIRECTION ( 'NONE',  ( -0.04216478779797398074, 0.9991106698809455455, 0.000000000000000000 ) ) ;
#1265=ORIENTED_EDGE ( 'NONE', *, *, #51238, .T. ) ;
#1267=DIRECTION ( 'NONE',  ( -1.000000000000000078E-15, 1.000000000000000083E-30, 1.000000000000000000 ) ) ;
#1269=AXIS2_PLACEMENT_3D ( 'NONE', #52081, #59360, #60251 ) ;
#1270=CARTESIAN_POINT ( 'NONE',  ( 100.8874142568969887, -44.70019346635132962, 133.0531993215868454 ) ) ;
#1271=ORIENTED_EDGE ( 'NONE', *, *, #74088, .F. ) ;
#1272=ORIENTED_EDGE ( 'NONE', *, *, #67656, .T. ) ;
#1275=CARTESIAN_POINT ( 'NONE',  ( 95.25894796463062164, -35.71821259427313322, 36.25848241876794731 ) ) ;
#1276=FACE_OUTER_BOUND ( 'NONE', #42259, .T. ) ;
#1277=CARTESIAN_POINT ( 'NONE',  ( 192.5667039024473013, -23.42844715993434335, 249.9678068554149775 ) ) ;
#1278=CARTESIAN_POINT ( 'NONE',  ( 109.6430121376341731, -46.48008673325654883, 73.78145860982388626 ) ) ;
#1279=CARTESIAN_POINT ( 'NONE',  ( 110.1676348244934616, -46.62498374987622896, 52.80610146638697699 ) ) ;
#1280=CARTESIAN_POINT ( 'NONE',  ( 37.03715912545347777, -48.62818131006128652, 129.9678068554150911 ) ) ;
#1281=CARTESIAN_POINT ( 'NONE',  ( 102.0922439024871551, -27.59239485085799970, 141.4727681330539895 ) ) ;
#1282=FACE_OUTER_BOUND ( 'NONE', #76067, .T. ) ;
#1283=DIRECTION ( 'NONE',  ( -0.08544974978095701279, -0.9963424814100680926, 0.000000000000000000 ) ) ;
#1285=VECTOR ( 'NONE', #59340, 1000.000000000000000 ) ;
#1287=PLANE ( 'NONE',  #62261 ) ;
#1288=LINE ( 'NONE', #22190, #77551 ) ;
#1290=ADVANCED_FACE ( 'NONE', ( #75283 ), #32583, .F. ) ;
#1292=CARTESIAN_POINT ( 'NONE',  ( 101.9629764938643035, -45.91127772325894085, 187.1727681330539781 ) ) ;
#1293=ORIENTED_EDGE ( 'NONE', *, *, #65322, .F. ) ;
#1294=LINE ( 'NONE', #23102, #82825 ) ;
#1295=CARTESIAN_POINT ( 'NONE',  ( 96.65238424151439744, -35.53540495314400260, 202.2356252759109623 ) ) ;
#1296=CARTESIAN_POINT ( 'NONE',  ( 101.7337754387761635, -26.99498644972499051, 96.46324432352997746 ) ) ;
#1297=CARTESIAN_POINT ( 'NONE',  ( 119.5435152932140284, -31.57448135767196362, 293.6356252759107974 ) ) ;
#1298=CARTESIAN_POINT ( 'NONE',  ( 107.0664832912739968, -36.72944715994100306, 287.6356252759109680 ) ) ;
#1299=AXIS2_PLACEMENT_3D ( 'NONE', #44643, #72376, #1552 ) ;
#1302=EDGE_CURVE ( 'NONE', #71592, #61394, #60732, .T. ) ;
#1305=VERTEX_POINT ( 'NONE', #40299 ) ;
#1306=DIRECTION ( 'NONE',  ( 1.907762142705490052E-15, 7.167082501179359715E-16, -1.000000000000000000 ) ) ;
#1307=CARTESIAN_POINT ( 'NONE',  ( 118.6539291974399219, -39.21253252500506647, 254.6584824187681022 ) ) ;
#1308=LINE ( 'NONE', #36273, #19986 ) ;
#1310=ADVANCED_FACE ( 'NONE', ( #70258 ), #78437, .F. ) ;
#1313=CARTESIAN_POINT ( 'NONE',  ( 86.06670390244796920, -58.35344715994099829, 10.91780685541479734 ) ) ;
#1315=CARTESIAN_POINT ( 'NONE',  ( 115.9104104090373539, -31.16785412357883800, 34.27276813305396530 ) ) ;
#1316=ORIENTED_EDGE ( 'NONE', *, *, #15848, .F. ) ;
#1317=CIRCLE ( 'NONE', #82579, 0.5000000000000004441 ) ;
#1318=VECTOR ( 'NONE', #65684, 1000.000000000000000 ) ;
#1319=ORIENTED_EDGE ( 'NONE', *, *, #57624, .F. ) ;
#1320=CARTESIAN_POINT ( 'NONE',  ( 97.07210785868812764, -35.37808982346257380, 17.22062569094285678 ) ) ;
#1321=CARTESIAN_POINT ( 'NONE',  ( 104.7413546109693527, -27.22895552020974108, 281.2670538473389570 ) ) ;
#1322=CARTESIAN_POINT ( 'NONE',  ( 181.5667039024459939, -18.82844715994031048, -5.074374724088000832 ) ) ;
#1323=EDGE_CURVE ( 'NONE', #68582, #48583, #42528, .T. ) ;
#1324=CIRCLE ( 'NONE', #86910, 2.999999999999919176 ) ;
#1325=CARTESIAN_POINT ( 'NONE',  ( 102.6065612795740805, -27.36740250608086100, 136.4422919425769578 ) ) ;
#1328=EDGE_CURVE ( 'NONE', #38211, #27387, #71169, .T. ) ;
#1329=AXIS2_PLACEMENT_3D ( 'NONE', #73383, #39311, #72509 ) ;
#1330=CARTESIAN_POINT ( 'NONE',  ( 108.5946222506355952, -26.81343367791396659, 20.95493592026397778 ) ) ;
#1333=CARTESIAN_POINT ( 'NONE',  ( 134.0664832912740110, -8.729447159940999512, 2.408125275911999097 ) ) ;
#1334=EDGE_CURVE ( 'NONE', #8126, #49439, #57738, .T. ) ;
#1339=CARTESIAN_POINT ( 'NONE',  ( 105.8471956337337190, -45.50678253122700312, 253.8987261630398677 ) ) ;
#1340=DIRECTION ( 'NONE',  ( 0.000000000000000000, 0.000000000000000000, -1.000000000000000000 ) ) ;
#1342=LINE ( 'NONE', #15426, #49019 ) ;
#1343=CIRCLE ( 'NONE', #68054, 13.44999999999999396 ) ;
#1345=VERTEX_POINT ( 'NONE', #4344 ) ;
#1347=FACE_OUTER_BOUND ( 'NONE', #6550, .T. ) ;
#1349=CARTESIAN_POINT ( 'NONE',  ( 112.5143773164265184, -27.84083190490108706, 94.63848241876793566 ) ) ;
#1351=CARTESIAN_POINT ( 'NONE',  ( 105.0857350373783561, -45.56626257478142605, 26.81146744712498275 ) ) ;
#1352=CARTESIAN_POINT ( 'NONE',  ( 116.8165727570488741, -34.15080317556459732, 129.0313754411595824 ) ) ;
#1353=CARTESIAN_POINT ( 'NONE',  ( 116.7860849611261500, -31.33117650353035799, 179.2299109901969700 ) ) ;
#1355=CARTESIAN_POINT ( 'NONE',  ( 87.06648329127403940, -46.72944715994105280, -4.824374724089049771 ) ) ;
#1358=VECTOR ( 'NONE', #26134, 1000.000000000000000 ) ;
#1359=CARTESIAN_POINT ( 'NONE',  ( 116.1774319148507573, -31.53050193741562524, 285.2384824187680579 ) ) ;
#1360=CARTESIAN_POINT ( 'NONE',  ( 110.4730404891439832, -46.15996163262695973, 117.8541770027330529 ) ) ;
#1362=CARTESIAN_POINT ( 'NONE',  ( 136.7660003837311535, -37.25405382162939105, 6.823682607504132136 ) ) ;
#1364=CARTESIAN_POINT ( 'NONE',  ( 101.4776230940428832, -27.87746311998561666, 106.5241967044819944 ) ) ;
#1366=VERTEX_POINT ( 'NONE', #25221 ) ;
#1368=EDGE_CURVE ( 'NONE', #40826, #8807, #66105, .T. ) ;
#1370=CARTESIAN_POINT ( 'NONE',  ( 99.04406175382935373, -42.84125750402932908, 121.8439585956957103 ) ) ;
#1371=LINE ( 'NONE', #6828, #59327 ) ;
#1373=CARTESIAN_POINT ( 'NONE',  ( 179.1667039024476082, -26.71338133338671028, 193.9678068554150059 ) ) ;
#1375=CARTESIAN_POINT ( 'NONE',  ( 116.3364580279229301, -41.54664843801584340, 284.4441967044824082 ) ) ;
#1376=DIRECTION ( 'NONE',  ( -1.000000000000000000, -2.756263715554006823E-15, 0.000000000000000000 ) ) ;
#1377=ORIENTED_EDGE ( 'NONE', *, *, #75271, .F. ) ;
#1378=FACE_OUTER_BOUND ( 'NONE', #72636, .T. ) ;
#1379=CIRCLE ( 'NONE', #11547, 4.750000000000004441 ) ;
#1380=DIRECTION ( 'NONE',  ( -0.7071067811865187069, -0.7071067811865764385, -7.071067811865181482E-16 ) ) ;
#1382=VERTEX_POINT ( 'NONE', #52449 ) ;
#1383=CIRCLE ( 'NONE', #83926, 4.874999999999990230 ) ;
#1385=CARTESIAN_POINT ( 'NONE',  ( 161.4809174648183330, -48.32844715993547879, 300.4678068554149490 ) ) ;
#1387=CARTESIAN_POINT ( 'NONE',  ( 106.5131950068454216, -24.24167068730766417, 320.8164078654934315 ) ) ;
#1390=DIRECTION ( 'NONE',  ( -0.02150753337723538411, -0.0009076677972193728959, -0.9997682742251812194 ) ) ;
#1391=CARTESIAN_POINT ( 'NONE',  ( 100.6939357996894557, -31.04202505589751837, 190.1695626852199439 ) ) ;
#1392=LINE ( 'NONE', #63611, #18562 ) ;
#1394=CARTESIAN_POINT ( 'NONE',  ( 114.5992475275822784, -44.05128143045557465, 98.21276813305395592 ) ) ;
#1396=CARTESIAN_POINT ( 'NONE',  ( 71.24189083761808661, -0.9290567490904538817, 542.9756252759101471 ) ) ;
#1398=AXIS2_PLACEMENT_3D ( 'NONE', #85405, #71315, #36783 ) ;
#1399=EDGE_CURVE ( 'NONE', #84277, #89309, #85337, .T. ) ;
#1401=CARTESIAN_POINT ( 'NONE',  ( 103.2832162603179285, -27.47272535187759956, 276.3852211716737202 ) ) ;
#1402=ORIENTED_EDGE ( 'NONE', *, *, #53008, .T. ) ;
#1404=EDGE_CURVE ( 'NONE', #77239, #78071, #17527, .T. ) ;
#1405=CARTESIAN_POINT ( 'NONE',  ( 152.4532656103850172, -72.54314042502360849, 542.9756252759101471 ) ) ;
#1406=ORIENTED_EDGE ( 'NONE', *, *, #28026, .F. ) ;
#1407=CARTESIAN_POINT ( 'NONE',  ( 188.5667039024484950, -48.82844715993430640, 139.7178068554150059 ) ) ;
#1410=EDGE_CURVE ( 'NONE', #78226, #87811, #22759, .T. ) ;
#1411=CARTESIAN_POINT ( 'NONE',  ( 172.5664832912740110, -36.32844715994070839, 194.1756252759119832 ) ) ;
#1413=CARTESIAN_POINT ( 'NONE',  ( 98.07775226919108036, -31.40506188283435307, 85.90133956162493689 ) ) ;
#1415=CARTESIAN_POINT ( 'NONE',  ( 99.09538940105012728, -30.55084863300459475, 165.8023339492073944 ) ) ;
#1418=CARTESIAN_POINT ( 'NONE',  ( 107.0664832912730020, -36.72944715994189835, 342.9256252759109884 ) ) ;
#1419=ORIENTED_EDGE ( 'NONE', *, *, #29735, .F. ) ;
#1420=ADVANCED_FACE ( 'NONE', ( #38399 ), #3890, .F. ) ;
#1421=CARTESIAN_POINT ( 'NONE',  ( 131.3164832912739826, -36.72944715994100306, 14.92562527591099553 ) ) ;
#1422=DIRECTION ( 'NONE',  ( 0.000000000000000000, 1.000000000000000000, 0.000000000000000000 ) ) ;
#1423=EDGE_CURVE ( 'NONE', #44341, #74855, #9375, .T. ) ;
#1425=CARTESIAN_POINT ( 'NONE',  ( 113.0894857754661587, -28.19359922731340262, 125.5870538473399591 ) ) ;
#1427=CARTESIAN_POINT ( 'NONE',  ( 141.0667039024479834, -50.82844715994100682, 198.9178068554149945 ) ) ;
#1429=VECTOR ( 'NONE', #18753, 1000.000000000000000 ) ;
#1430=VERTEX_POINT ( 'NONE', #64784 ) ;
#1432=CARTESIAN_POINT ( 'NONE',  ( 116.5394839232219510, -34.29517225379352396, 120.0270538473389479 ) ) ;
#1436=EDGE_CURVE ( 'NONE', #65478, #55247, #52010, .T. ) ;
#1437=CARTESIAN_POINT ( 'NONE',  ( 117.5198883501232103, -40.51604253736888950, 19.54991099019698453 ) ) ;
#1438=FACE_OUTER_BOUND ( 'NONE', #32979, .T. ) ;
#1440=CARTESIAN_POINT ( 'NONE',  ( 151.0371591254572934, -24.42818131005592974, 300.4678068554149490 ) ) ;
#1441=EDGE_CURVE ( 'NONE', #36268, #46468, #45639, .T. ) ;
#1442=CARTESIAN_POINT ( 'NONE',  ( 151.0371591254575208, -24.42818131005592264, 180.4678068554149775 ) ) ;
#1443=EDGE_CURVE ( 'NONE', #65895, #81510, #3004, .T. ) ;
#1444=DIRECTION ( 'NONE',  ( -0.7071067811865634489, 0.7071067811865315855, -7.071067811865641980E-16 ) ) ;
#1446=ADVANCED_FACE ( 'NONE', ( #51138, #11142 ), #86131, .T. ) ;
#1447=CARTESIAN_POINT ( 'NONE',  ( 104.1325824198641499, -27.39908484284267587, 250.3184824187684683 ) ) ;
#1449=ORIENTED_EDGE ( 'NONE', *, *, #60949, .F. ) ;
#1450=CARTESIAN_POINT ( 'NONE',  ( 113.3955173535308063, -30.52198670013464010, 145.8758690201829609 ) ) ;
#1451=AXIS2_PLACEMENT_3D ( 'NONE', #77132, #55746, #63036 ) ;
#1453=CARTESIAN_POINT ( 'NONE',  ( 105.0114852080080254, -45.89751720821543302, 23.82063092494396273 ) ) ;
#1455=CARTESIAN_POINT ( 'NONE',  ( 134.0664832912739826, -18.72944715994100306, -5.074374724089001809 ) ) ;
#1458=DIRECTION ( 'NONE',  ( 1.000000000000000078E-15, 0.000000000000000000, -1.000000000000000000 ) ) ;
#1461=CARTESIAN_POINT ( 'NONE',  ( 116.0363244534468805, -41.99923036749497385, 238.4041967044829562 ) ) ;
#1463=VERTEX_POINT ( 'NONE', #58402 ) ;
#1464=ORIENTED_EDGE ( 'NONE', *, *, #37003, .T. ) ;
#1467=VECTOR ( 'NONE', #23210, 1000.000000000000000 ) ;
#1468=CARTESIAN_POINT ( 'NONE',  ( 97.82696674394188108, -40.55455350847689289, 122.6383624784102722 ) ) ;
#1469=DIRECTION ( 'NONE',  ( 0.000000000000000000, 0.000000000000000000, 1.000000000000000000 ) ) ;
#1470=CARTESIAN_POINT ( 'NONE',  ( 106.6352542858682284, -26.36832623700844280, 36.09753003781596448 ) ) ;
#1471=LINE ( 'NONE', #42765, #9304 ) ;
#1473=CARTESIAN_POINT ( 'NONE',  ( 110.2975601020867202, -46.68703778808450267, 8.827053847339950465 ) ) ;
#1474=CARTESIAN_POINT ( 'NONE',  ( 61.56670390244634916, -23.42844715994023375, 180.4678068554151196 ) ) ;
#1475=CARTESIAN_POINT ( 'NONE',  ( 97.61519122654028990, -41.12945951998310790, 256.6727681330537507 ) ) ;
#1478=CARTESIAN_POINT ( 'NONE',  ( 77.40528906089568295, -37.42303004212706696, 6.877070700249887203 ) ) ;
#1479=CARTESIAN_POINT ( 'NONE',  ( 73.06670390244801183, -50.82844715994100682, 10.91780685541510110 ) ) ;
#1480=FACE_OUTER_BOUND ( 'NONE', #2476, .T. ) ;
#1481=CARTESIAN_POINT ( 'NONE',  ( 108.0475348069766284, -44.83298120013808585, 115.4909475124489830 ) ) ;
#1482=CARTESIAN_POINT ( 'NONE',  ( 110.7038792373522824, -48.03394190404919328, 203.8241967044819489 ) ) ;
#1483=CARTESIAN_POINT ( 'NONE',  ( 31.56670390244800828, -32.29483332968611364, -5.074374724088000832 ) ) ;
#1484=VERTEX_POINT ( 'NONE', #23906 ) ;
#1485=CARTESIAN_POINT ( 'NONE',  ( 130.3998166246070127, 12.92155284005802685, 349.2756252759110680 ) ) ;
#1486=VECTOR ( 'NONE', #6356, 1000.000000000000000 ) ;
#1489=CARTESIAN_POINT ( 'NONE',  ( 141.8664832912729992, -1.929447159941394263, 361.9756252759109998 ) ) ;
#1490=EDGE_LOOP ( 'NONE', ( #21592, #40625, #23212, #44186 ) ) ;
#1491=ORIENTED_EDGE ( 'NONE', *, *, #3137, .F. ) ;
#1492=DIRECTION ( 'NONE',  ( 1.000000000000000000, 6.145690160522439356E-16, 0.000000000000000000 ) ) ;
#1496=CARTESIAN_POINT ( 'NONE',  ( 100.3410792892688761, -42.04179533522079026, 91.28099125664796532 ) ) ;
#1497=CARTESIAN_POINT ( 'NONE',  ( 108.0161133123553725, -24.89170165127225332, 265.0127681330534415 ) ) ;
#1498=EDGE_CURVE ( 'NONE', #17889, #3581, #82453, .T. ) ;
#1502=AXIS2_PLACEMENT_3D ( 'NONE', #54107, #67766, #39599 ) ;
#1505=DIRECTION ( 'NONE',  ( 0.000000000000000000, 1.000000000000000000, 0.000000000000000000 ) ) ;
#1509=ADVANCED_FACE ( 'NONE', ( #61970, #32925 ), #67902, .T. ) ;
#1510=CARTESIAN_POINT ( 'NONE',  ( 97.33998274022607688, -37.75834089694785689, 126.4099109901969626 ) ) ;
#1511=CARTESIAN_POINT ( 'NONE',  ( 102.2821109723304431, -27.37735778705684098, 120.4527681330539792 ) ) ;
#1512=CARTESIAN_POINT ( 'NONE',  ( 116.3563860081925725, -41.55700552044970664, 288.4441967044822945 ) ) ;
#1513=ORIENTED_EDGE ( 'NONE', *, *, #16568, .T. ) ;
#1514=CARTESIAN_POINT ( 'NONE',  ( 113.2201423986613520, -45.14488000985961946, 228.0784824187679760 ) ) ;
#1515=CARTESIAN_POINT ( 'NONE',  ( 83.06670390244804025, -42.97311385574013798, 207.5838068554169809 ) ) ;
#1517=DIRECTION ( 'NONE',  ( 1.000000000000000078E-15, -1.000000000000000083E-30, -1.000000000000000000 ) ) ;
#1521=CARTESIAN_POINT ( 'NONE',  ( 141.8545562996768012, -1.932463243632623229, 394.9756252759100903 ) ) ;
#1522=CARTESIAN_POINT ( 'NONE',  ( 131.3881603334745307, -37.35482103167609580, 6.853567712192067951 ) ) ;
#1523=CIRCLE ( 'NONE', #72707, 11.45913725231036118 ) ;
#1526=CARTESIAN_POINT ( 'NONE',  ( 107.0664832912739968, -36.72944715994100306, 287.6356252759109680 ) ) ;
#1527=EDGE_CURVE ( 'NONE', #55604, #83594, #25669, .T. ) ;
#1528=LINE ( 'NONE', #63747, #61685 ) ;
#1529=VERTEX_POINT ( 'NONE', #54239 ) ;
#1530=DIRECTION ( 'NONE',  ( -1.000000000000000000, 0.000000000000000000, 2.900000000000000265E-14 ) ) ;
#1531=CARTESIAN_POINT ( 'NONE',  ( 100.8351866834200337, -45.15911532695984931, 257.0699109901966608 ) ) ;
#1532=CARTESIAN_POINT ( 'NONE',  ( 102.6835365363430981, -27.27046913952221985, 176.4213395616249898 ) ) ;
#1533=CARTESIAN_POINT ( 'NONE',  ( 100.4654578171049337, -27.83497312075872188, 31.59657765686396758 ) ) ;
#1536=CARTESIAN_POINT ( 'NONE',  ( 81.36335724984412821, -34.30134337669328914, 7.962481652686962619 ) ) ;
#1537=CARTESIAN_POINT ( 'NONE',  ( 97.92333446084529669, -40.78093374296712881, 137.6583996970876456 ) ) ;
#1540=FACE_OUTER_BOUND ( 'NONE', #74364, .T. ) ;
#1541=ORIENTED_EDGE ( 'NONE', *, *, #69904, .T. ) ;
#1542=VECTOR ( 'NONE', #76999, 1000.000000000000000 ) ;
#1543=CARTESIAN_POINT ( 'NONE',  ( 115.6043783821399558, -39.74888713174190968, 177.9905150661719802 ) ) ;
#1548=CARTESIAN_POINT ( 'NONE',  ( 102.0615167388205293, -46.55869598106821883, 168.2137205140059564 ) ) ;
#1549=DIRECTION ( 'NONE',  ( 1.000000000000000078E-15, 0.000000000000000000, 1.000000000000000000 ) ) ;
#1550=FACE_BOUND ( 'NONE', #55978, .T. ) ;
#1551=CARTESIAN_POINT ( 'NONE',  ( 110.8974114899633463, -27.49234298998610271, 85.76376216369907013 ) ) ;
#1552=DIRECTION ( 'NONE',  ( 1.000000000000000000, 0.000000000000000000, 0.000000000000000000 ) ) ;
#1553=CARTESIAN_POINT ( 'NONE',  ( 97.82527667066705135, -40.55047884729894747, 96.63846944729883148 ) ) ;
#1554=EDGE_CURVE ( 'NONE', #74158, #31761, #61083, .T. ) ;
#1555=CARTESIAN_POINT ( 'NONE',  ( 96.76615086495793605, -37.93025403122317130, 86.43086337114897333 ) ) ;
#1556=ORIENTED_EDGE ( 'NONE', *, *, #26606, .T. ) ;
#1557=AXIS2_PLACEMENT_3D ( 'NONE', #77427, #56968, #20674 ) ;
#1558=EDGE_LOOP ( 'NONE', ( #88400, #79193, #56424, #64076 ) ) ;
#1559=CARTESIAN_POINT ( 'NONE',  ( 97.94737569220006890, -41.00876738043628222, 58.10729759161198160 ) ) ;
#1560=DIRECTION ( 'NONE',  ( -1.000000000000000078E-15, -1.000000000000000083E-30, 1.000000000000000000 ) ) ;
#1561=CARTESIAN_POINT ( 'NONE',  ( 98.96845470676157674, -30.25173782105014197, 191.7775300378149836 ) ) ;
#1562=CARTESIAN_POINT ( 'NONE',  ( 100.8874679703711195, -44.70022144079540993, 37.05229195109952656 ) ) ;
#1563=LINE ( 'NONE', #29264, #27555 ) ;
#1564=CARTESIAN_POINT ( 'NONE',  ( 46.32460016641643108, -48.34074026909789268, 129.9678068554150911 ) ) ;
#1568=CARTESIAN_POINT ( 'NONE',  ( 108.3168256696638281, -47.05733704442519638, 117.6727681330539639 ) ) ;
#1570=ORIENTED_EDGE ( 'NONE', *, *, #83036, .T. ) ;
#1572=CIRCLE ( 'NONE', #49391, 13.44999999999999396 ) ;
#1575=CARTESIAN_POINT ( 'NONE',  ( 51.24204729617298426, -31.76306994223730840, 237.4678068554150059 ) ) ;
#1576=LINE ( 'NONE', #36087, #46456 ) ;
#1578=CARTESIAN_POINT ( 'NONE',  ( 102.6495774910181780, -44.17201850306531696, 204.9804713219729706 ) ) ;
#1580=ADVANCED_FACE ( 'NONE', ( #61521 ), #47438, .T. ) ;
#1581=PLANE ( 'NONE',  #53701 ) ;
#1582=B_SPLINE_CURVE_WITH_KNOTS ( 'NONE', 3,
 ( #68511, #27613, #81707, #33969, #19908, #40789, #13541, #28053, #41225, #34870, #68955, #6278, #61672, #54394, #20805, #13988, #47590, #34421 ),
 .UNSPECIFIED., .F., .F.,
 ( 4, 2, 2, 2, 2, 2, 2, 2, 4 ),
 ( 0.5000000002310567293, 0.5625000002021746104, 0.6250000001732924915, 0.6875000001444104836, 0.7500000001155283647, 0.8125000000866462457, 0.8750000000577642378, 0.9375000000288821189, 1.000000000000000000 ),
 .UNSPECIFIED. ) ;
#1583=CARTESIAN_POINT ( 'NONE',  ( 97.74620163809125017, -42.67179083687646823, 141.7661014663869707 ) ) ;
#1584=CARTESIAN_POINT ( 'NONE',  ( 165.6738106836043585, -28.98061976758451053, 237.4678068554150059 ) ) ;
#1587=ORIENTED_EDGE ( 'NONE', *, *, #52130, .F. ) ;
#1588=AXIS2_PLACEMENT_3D ( 'NONE', #9865, #37126, #79814 ) ;
#1590=ORIENTED_EDGE ( 'NONE', *, *, #84891, .F. ) ;
#1591=ORIENTED_EDGE ( 'NONE', *, *, #56835, .F. ) ;
#1594=CARTESIAN_POINT ( 'NONE',  ( 98.31940232332729579, -40.15947632561638869, 243.0434880678019738 ) ) ;
#1595=DIRECTION ( 'NONE',  ( -0.000000000000000000, -0.000000000000000000, -1.000000000000000000 ) ) ;
#1596=ORIENTED_EDGE ( 'NONE', *, *, #78100, .F. ) ;
#1597=CARTESIAN_POINT ( 'NONE',  ( 100.0187664783711483, -40.62989960760008046, 9.635625275910943088 ) ) ;
#1598=DIRECTION ( 'NONE',  ( -4.299999999999999979E-14, 1.000000000000000000, -4.400000000000000367E-29 ) ) ;
#1600=ORIENTED_EDGE ( 'NONE', *, *, #21100, .T. ) ;
#1607=CARTESIAN_POINT ( 'NONE',  ( 115.7114656938015429, -36.32299383444259888, 266.6699951314962505 ) ) ;
#1608=CARTESIAN_POINT ( 'NONE',  ( 117.5094658089964241, -40.42262428419060427, 178.5680062282919778 ) ) ;
#1609=AXIS2_PLACEMENT_3D ( 'NONE', #15949, #58595, #43631 ) ;
#1611=CARTESIAN_POINT ( 'NONE',  ( 97.59110611908489830, -31.08311649095515250, 130.9108633711489915 ) ) ;
#1613=CARTESIAN_POINT ( 'NONE',  ( 20.56670390244748603, -48.82844715994200158, 129.9678068554150627 ) ) ;
#1614=CARTESIAN_POINT ( 'NONE',  ( 115.8552077933167794, -44.67884570232850194, 229.2413395616249545 ) ) ;
#1615=DIRECTION ( 'NONE',  ( 1.000000000000000000, 4.299999999999999979E-14, 1.000000000000000078E-15 ) ) ;
#1618=VERTEX_POINT ( 'NONE', #88813 ) ;
#1619=CARTESIAN_POINT ( 'NONE',  ( 164.5667039024479834, -50.82844715994100682, 10.91780685541479734 ) ) ;
#1620=ORIENTED_EDGE ( 'NONE', *, *, #59322, .F. ) ;
#1622=ORIENTED_EDGE ( 'NONE', *, *, #61664, .T. ) ;
#1623=AXIS2_PLACEMENT_3D ( 'NONE', #46896, #47349, #54597 ) ;
#1624=EDGE_CURVE ( 'NONE', #49936, #14756, #19759, .T. ) ;
#1626=CARTESIAN_POINT ( 'NONE',  ( 113.7136498174399577, -45.61921998050937077, 188.0994347997199725 ) ) ;
#1628=CARTESIAN_POINT ( 'NONE',  ( 102.3603858057123972, -46.03211757857948783, 127.2041967044829960 ) ) ;
#1629=CARTESIAN_POINT ( 'NONE',  ( 97.81399847929220925, -40.51646572127298640, 256.6355814287313137 ) ) ;
#1630=CARTESIAN_POINT ( 'NONE',  ( 135.9194882200285690, -34.69035895458431185, 7.660272404649855815 ) ) ;
#1631=DIRECTION ( 'NONE',  ( 0.000000000000000000, 0.000000000000000000, -1.000000000000000000 ) ) ;
#1632=CARTESIAN_POINT ( 'NONE',  ( 143.9834832912729894, -71.52944715994142655, 352.4506252759077825 ) ) ;
#1634=CARTESIAN_POINT ( 'NONE',  ( 113.7851844261089695, -26.99768152489570738, 235.5956252759109759 ) ) ;
#1636=DIRECTION ( 'NONE',  ( -4.299999999999999979E-14, 1.000000000000000000, 0.000000000000000000 ) ) ;
#1637=EDGE_CURVE ( 'NONE', #12195, #79540, #27020, .T. ) ;
#1638=DIRECTION ( 'NONE',  ( -0.7071067811865475727, 0.7071067811865475727, 0.000000000000000000 ) ) ;
#1639=CARTESIAN_POINT ( 'NONE',  ( 134.0664832912740110, -8.729447159940999512, 4.925625275911999168 ) ) ;
#1640=CARTESIAN_POINT ( 'NONE',  ( 117.0608945241952483, -38.08045311458047877, 259.7189586097406391 ) ) ;
#1641=CARTESIAN_POINT ( 'NONE',  ( 107.0664832912740394, -56.47944715994103149, -4.824374724089029343 ) ) ;
#1643=CARTESIAN_POINT ( 'NONE',  ( 117.5355484441921163, -36.80252840376058288, 263.8213395616250523 ) ) ;
#1644=ORIENTED_EDGE ( 'NONE', *, *, #23752, .F. ) ;
#1646=CARTESIAN_POINT ( 'NONE',  ( 99.08440026364779385, -45.52245356036965518, 156.9899109901969609 ) ) ;
#1647=CARTESIAN_POINT ( 'NONE',  ( 97.35162482889903401, -32.85093483786611301, 37.02419670448292521 ) ) ;
#1648=CARTESIAN_POINT ( 'NONE',  ( 117.3342495501102007, -34.51337161069084658, 179.9956252759109532 ) ) ;
#1650=CARTESIAN_POINT ( 'NONE',  ( 152.0368932755770857, -23.42844715993588522, 249.9678068554149490 ) ) ;
#1651=FACE_OUTER_BOUND ( 'NONE', #25600, .T. ) ;
#1652=DIRECTION ( 'NONE',  ( 0.000000000000000000, 0.000000000000000000, 1.000000000000000000 ) ) ;
#1653=DIRECTION ( 'NONE',  ( 0.000000000000000000, 0.000000000000000000, 1.000000000000000000 ) ) ;
#1654=LINE ( 'NONE', #56123, #5955 ) ;
#1655=EDGE_LOOP ( 'NONE', ( #58719, #47475, #58604, #81433 ) ) ;
#1656=AXIS2_PLACEMENT_3D ( 'NONE', #65732, #23978, #4421 ) ;
#1658=EDGE_LOOP ( 'NONE', ( #89720, #70654, #32040, #47006 ) ) ;
#1660=CONICAL_SURFACE ( 'NONE', #16179, 9.571100913904340146, 0.7853981633974539411 ) ;
#1661=CARTESIAN_POINT ( 'NONE',  ( 41.56648329127499153, -27.82844715994070484, 203.6756252759119832 ) ) ;
#1663=CARTESIAN_POINT ( 'NONE',  ( 98.60777729073579678, -43.80857954853289016, 67.86895860924497015 ) ) ;
#1666=CARTESIAN_POINT ( 'NONE',  ( 71.24189083761808661, -0.9290567490904538817, 542.9756252759101471 ) ) ;
#1667=CARTESIAN_POINT ( 'NONE',  ( 96.00793635059680753, -35.77758691827158799, 182.2461014663869889 ) ) ;
#1668=EDGE_CURVE ( 'NONE', #27718, #55509, #54582, .T. ) ;
#1669=CARTESIAN_POINT ( 'NONE',  ( 100.8732324256648951, -44.32512360075851632, 12.03276813305398463 ) ) ;
#1672=VERTEX_POINT ( 'NONE', #14747 ) ;
#1674=FACE_OUTER_BOUND ( 'NONE', #5073, .T. ) ;
#1675=DIRECTION ( 'NONE',  ( 4.299999999999999979E-14, -1.000000000000000000, 4.400000000000000367E-29 ) ) ;
#1680=CARTESIAN_POINT ( 'NONE',  ( 130.3998166246059895, 12.92155284005730387, 358.9756252759109998 ) ) ;
#1681=CARTESIAN_POINT ( 'NONE',  ( 117.4903696573864522, -37.28369426754697002, 18.78419670448294809 ) ) ;
#1682=ORIENTED_EDGE ( 'NONE', *, *, #11573, .T. ) ;
#1686=CARTESIAN_POINT ( 'NONE',  ( 98.42009728606723229, -37.10485906011713553, 114.1671379886389559 ) ) ;
#1687=CIRCLE ( 'NONE', #19050, 10.04999999999999361 ) ;
#1688=ADVANCED_FACE ( 'NONE', ( #70144 ), #28818, .F. ) ;
#1689=CARTESIAN_POINT ( 'NONE',  ( 90.44969454456403923, -17.59493780205715652, 229.5838068554169809 ) ) ;
#1690=CARTESIAN_POINT ( 'NONE',  ( 118.5256205435843526, -36.72944715994100306, 394.9756252759102040 ) ) ;
#1692=ORIENTED_EDGE ( 'NONE', *, *, #42690, .T. ) ;
#1693=CARTESIAN_POINT ( 'NONE',  ( 99.50491052054114505, -43.30599679329080942, 136.8954324092491959 ) ) ;
#1694=ORIENTED_EDGE ( 'NONE', *, *, #55189, .F. ) ;
#1695=ORIENTED_EDGE ( 'NONE', *, *, #73004, .F. ) ;
#1696=CIRCLE ( 'NONE', #74241, 1.499999999999987788 ) ;
#1697=CARTESIAN_POINT ( 'NONE',  ( 103.3528332358002331, -45.35993549251112711, 133.6968214011349403 ) ) ;
#1699=CARTESIAN_POINT ( 'NONE',  ( 117.3602503114455402, -32.64000144215158628, 95.13943479972097350 ) ) ;
#1700=AXIS2_PLACEMENT_3D ( 'NONE', #61047, #54207, #6539 ) ;
#1701=CARTESIAN_POINT ( 'NONE',  ( 112.4304735641928374, -45.18349285385466629, 18.02636112242024424 ) ) ;
#1705=EDGE_CURVE ( 'NONE', #27930, #72137, #18994, .T. ) ;
#1707=CARTESIAN_POINT ( 'NONE',  ( 98.28768183251310120, -28.73153112808589427, 80.73848241876795839 ) ) ;
#1710=CARTESIAN_POINT ( 'NONE',  ( 111.5675350091857325, -45.45035926415926752, 272.9556252759110180 ) ) ;
#1711=CARTESIAN_POINT ( 'NONE',  ( 107.6557286256638264, -47.79009794008123890, 193.6308633711489620 ) ) ;
#1712=DIRECTION ( 'NONE',  ( 0.000000000000000000, 0.000000000000000000, -1.000000000000000000 ) ) ;
#1715=CARTESIAN_POINT ( 'NONE',  ( 98.20239980326637408, -43.33262854484335946, 107.8480062282919647 ) ) ;
#1716=AXIS2_PLACEMENT_3D ( 'NONE', #66058, #16155, #51094 ) ;
#1717=CARTESIAN_POINT ( 'NONE',  ( 107.0664832912739968, -36.72944715994100306, 287.6356252759109680 ) ) ;
#1719=DIRECTION ( 'NONE',  ( -0.7071067811865765496, 0.7071067811865185959, -7.071067811865773128E-16 ) ) ;
#1720=EDGE_CURVE ( 'NONE', #34717, #38575, #50130, .T. ) ;
#1721=EDGE_LOOP ( 'NONE', ( #9907, #28709, #20435, #18619 ) ) ;
#1726=CARTESIAN_POINT ( 'NONE',  ( 79.06648329127300201, -36.72944715994189835, 361.9756252759109998 ) ) ;
#1727=CARTESIAN_POINT ( 'NONE',  ( 115.8917813183058740, -31.17956921574393903, 34.27276813305396530 ) ) ;
#1731=CARTESIAN_POINT ( 'NONE',  ( 112.3909220325769667, -27.83061929752856400, 54.65943479972096242 ) ) ;
#1733=CARTESIAN_POINT ( 'NONE',  ( 99.43809884604152671, -27.69271567064635065, 146.6356252759109395 ) ) ;
#1735=DIRECTION ( 'NONE',  ( 0.000000000000000000, 0.000000000000000000, -1.000000000000000000 ) ) ;
#1737=ORIENTED_EDGE ( 'NONE', *, *, #19258, .F. ) ;
#1739=AXIS2_PLACEMENT_3D ( 'NONE', #45180, #80628, #79299 ) ;
#1740=DIRECTION ( 'NONE',  ( 0.000000000000000000, 0.000000000000000000, 1.000000000000000000 ) ) ;
#1743=CYLINDRICAL_SURFACE ( 'NONE', #8533, 2.500000000000002220 ) ;
#1744=CARTESIAN_POINT ( 'NONE',  ( 113.6419851944692425, -45.67235822675655754, 183.0689586092439640 ) ) ;
#1746=DIRECTION ( 'NONE',  ( 1.000000000000000000, 0.000000000000000000, 9.462128050782575008E-16 ) ) ;
#1747=CARTESIAN_POINT ( 'NONE',  ( 116.5464386332369600, -41.20266105201044127, 224.4756252759109714 ) ) ;
#1748=CARTESIAN_POINT ( 'NONE',  ( 96.04171114508396556, -38.01470880000633201, 82.43086337114895912 ) ) ;
#1749=CARTESIAN_POINT ( 'NONE',  ( 115.0921083526524313, -30.62179339271783007, 250.3457344079624818 ) ) ;
#1750=AXIS2_PLACEMENT_3D ( 'NONE', #28533, #56229, #83979 ) ;
#1752=FACE_OUTER_BOUND ( 'NONE', #52042, .T. ) ;
#1753=ORIENTED_EDGE ( 'NONE', *, *, #85215, .T. ) ;
#1754=AXIS2_PLACEMENT_3D ( 'NONE', #6182, #33870, #20258 ) ;
#1755=ORIENTED_EDGE ( 'NONE', *, *, #60357, .T. ) ;
#1757=VERTEX_POINT ( 'NONE', #62426 ) ;
#1759=CARTESIAN_POINT ( 'NONE',  ( 100.6563598938200812, -44.95093154396422364, 228.0499109901969348 ) ) ;
#1760=CARTESIAN_POINT ( 'NONE',  ( 142.8821648370248170, -72.54478064608022692, 542.9756252759101471 ) ) ;
#1761=DIRECTION ( 'NONE',  ( 1.000000000000000000, 0.000000000000000000, 0.000000000000000000 ) ) ;
#1762=AXIS2_PLACEMENT_3D ( 'NONE', #40307, #88483, #18978 ) ;
#1763=CARTESIAN_POINT ( 'NONE',  ( 192.5667039024474434, -23.42844715993433624, 180.4678068554150343 ) ) ;
#1767=CARTESIAN_POINT ( 'NONE',  ( 102.7461184130007581, -25.66741906146929253, 20.37276813305294354 ) ) ;
#1770=VERTEX_POINT ( 'NONE', #49230 ) ;
#1771=ORIENTED_EDGE ( 'NONE', *, *, #45505, .T. ) ;
#1773=DIRECTION ( 'NONE',  ( 1.000000000000000000, 8.673617379883546378E-16, 9.757819552368989676E-16 ) ) ;
#1774=CARTESIAN_POINT ( 'NONE',  ( 105.7995771162975416, -24.27178701759104840, 322.4846826458744431 ) ) ;
#1776=CARTESIAN_POINT ( 'NONE',  ( 117.4208826025846690, -36.15918394849474282, 269.8822919425771829 ) ) ;
#1778=PLANE ( 'NONE',  #32775 ) ;
#1779=CARTESIAN_POINT ( 'NONE',  ( 116.9564367646782728, -33.61053620760072391, 125.0575300378159795 ) ) ;
#1784=CARTESIAN_POINT ( 'NONE',  ( 97.60787293175452817, -39.98237518918260491, 57.59005031470000091 ) ) ;
#1789=CARTESIAN_POINT ( 'NONE',  ( 115.9514134386872826, -36.57345012324869060, 285.2730118773255867 ) ) ;
#1790=ADVANCED_FACE ( 'NONE', ( #15185 ), #15640, .F. ) ;
#1791=DIRECTION ( 'NONE',  ( 0.000000000000000000, -1.000000000000000000, 0.000000000000000000 ) ) ;
#1792=DIRECTION ( 'NONE',  ( 1.000000000000000078E-15, 1.000000000000000083E-30, -1.000000000000000000 ) ) ;
#1793=CARTESIAN_POINT ( 'NONE',  ( 116.3186249068845939, -32.94868901192853627, 254.1356252759109395 ) ) ;
#1795=CARTESIAN_POINT ( 'NONE',  ( 29.56648329127400388, 15.62155284005900491, 328.6381252759109088 ) ) ;
#1796=CARTESIAN_POINT ( 'NONE',  ( 152.0371591254582881, -47.82818131005588214, 300.4678068554149490 ) ) ;
#1797=CIRCLE ( 'NONE', #52519, 2.517500000000005844 ) ;
#1798=ORIENTED_EDGE ( 'NONE', *, *, #78237, .T. ) ;
#1799=CARTESIAN_POINT ( 'NONE',  ( 97.22546204445637841, -31.69621874537715556, 95.96229194257799122 ) ) ;
#1800=ORIENTED_EDGE ( 'NONE', *, *, #20414, .T. ) ;
#1801=CARTESIAN_POINT ( 'NONE',  ( 110.6296508234850222, -44.49217663217273611, 27.34099125664796048 ) ) ;
#1802=EDGE_CURVE ( 'NONE', #74993, #84792, #81200, .T. ) ;
#1803=CARTESIAN_POINT ( 'NONE',  ( 99.04451456929375297, -42.84186625629031653, 126.8437268382981387 ) ) ;
#1804=CARTESIAN_POINT ( 'NONE',  ( 97.98063455390165188, -41.72806076336413383, 176.7146728949589658 ) ) ;
#1805=LINE ( 'NONE', #30840, #53471 ) ;
#1807=CARTESIAN_POINT ( 'NONE',  ( 116.3212776292296127, -32.94146857471318413, 287.6356252759109680 ) ) ;
#1808=AXIS2_PLACEMENT_3D ( 'NONE', #24429, #39384, #67089 ) ;
#1810=CARTESIAN_POINT ( 'NONE',  ( 116.3557873595856336, -41.55669258580370951, 284.4441967044824082 ) ) ;
#1811=CARTESIAN_POINT ( 'NONE',  ( 106.4460240858017528, -46.73159911271572753, 117.5290179274728075 ) ) ;
#1812=ORIENTED_EDGE ( 'NONE', *, *, #43102, .T. ) ;
#1815=CARTESIAN_POINT ( 'NONE',  ( 117.7233698349432132, -39.83239211553974712, 134.5889586092439743 ) ) ;
#1816=PLANE ( 'NONE',  #74416 ) ;
#1818=ORIENTED_EDGE ( 'NONE', *, *, #12913, .F. ) ;
#1819=EDGE_LOOP ( 'NONE', ( #40428, #80947 ) ) ;
#1821=CARTESIAN_POINT ( 'NONE',  ( 21.03715912545824551, -47.82818131006186491, 300.4678068554150059 ) ) ;
#1824=FACE_OUTER_BOUND ( 'NONE', #7569, .T. ) ;
#1825=DIRECTION ( 'NONE',  ( 0.000000000000000000, 0.000000000000000000, 1.000000000000000000 ) ) ;
#1826=EDGE_CURVE ( 'NONE', #68103, #39224, #1563, .T. ) ;
#1827=CARTESIAN_POINT ( 'NONE',  ( 106.6068465219953794, -25.68577410589699994, 36.09753003781596448 ) ) ;
#1830=VERTEX_POINT ( 'NONE', #17415 ) ;
#1832=CARTESIAN_POINT ( 'NONE',  ( 32.25690895537100289, -33.54226604285010893, -5.074374724088000832 ) ) ;
#1833=EDGE_LOOP ( 'NONE', ( #81821, #34815, #69385, #52376 ) ) ;
#1836=CARTESIAN_POINT ( 'NONE',  ( 80.06648329127399677, -21.47944715994105991, 1.625625275910943746 ) ) ;
#1837=DIRECTION ( 'NONE',  ( -0.7071067811874389708, 0.7071067811856560636, 0.000000000000000000 ) ) ;
#1838=CARTESIAN_POINT ( 'NONE',  ( 162.5667039024470171, -32.29483332968611364, -5.074374724088000832 ) ) ;
#1840=DIRECTION ( 'NONE',  ( -1.000000000000000000, -2.756263715554006823E-15, 0.000000000000000000 ) ) ;
#1841=CARTESIAN_POINT ( 'NONE',  ( 103.9834678596679538, -28.76382429851063449, 214.7924198280769872 ) ) ;
#1843=DIRECTION ( 'NONE',  ( -4.237773401492740281E-14, 1.000000000000000000, 0.000000000000000000 ) ) ;
#1845=CARTESIAN_POINT ( 'NONE',  ( 104.2019728789896078, -25.17854340234507760, 90.26991099019693365 ) ) ;
#1846=ORIENTED_EDGE ( 'NONE', *, *, #60116, .T. ) ;
#1847=CYLINDRICAL_SURFACE ( 'NONE', #68361, 0.4999999999999976685 ) ;
#1849=EDGE_LOOP ( 'NONE', ( #88194, #34939, #52622, #61995 ) ) ;
#1852=LINE ( 'NONE', #29548, #70283 ) ;
#1853=ORIENTED_EDGE ( 'NONE', *, *, #7488, .F. ) ;
#1858=DIRECTION ( 'NONE',  ( 1.000000000000000078E-15, 0.000000000000000000, -1.000000000000000000 ) ) ;
#1860=CARTESIAN_POINT ( 'NONE',  ( 106.8407094991504209, -48.60307516909384873, 77.56133956162491927 ) ) ;
#1861=CARTESIAN_POINT ( 'NONE',  ( 97.75839927879950153, -40.38492254185889863, 166.6242597985468308 ) ) ;
#1862=LINE ( 'NONE', #43169, #22040 ) ;
#1865=AXIS2_PLACEMENT_3D ( 'NONE', #58280, #51884, #79640 ) ;
#1866=CARTESIAN_POINT ( 'NONE',  ( 172.5664832912740110, -36.32844715994070839, 23.67562527591200094 ) ) ;
#1869=CARTESIAN_POINT ( 'NONE',  ( 106.0743987232105212, -48.56321320874933889, 108.5099109901969712 ) ) ;
#1870=DIRECTION ( 'NONE',  ( 1.000000000000000078E-15, -1.000000000000000083E-30, -1.000000000000000000 ) ) ;
#1871=DIRECTION ( 'NONE',  ( -0.7071067811865192621, -0.7071067811865758834, -7.071067811865186413E-16 ) ) ;
#1874=ORIENTED_EDGE ( 'NONE', *, *, #12701, .T. ) ;
#1875=DIRECTION ( 'NONE',  ( 0.000000000000000000, 1.000000000000000000, 0.000000000000000000 ) ) ;
#1876=CARTESIAN_POINT ( 'NONE',  ( 98.02110346605356028, -41.80092515478911963, 177.7451490854339795 ) ) ;
#1877=FACE_OUTER_BOUND ( 'NONE', #3764, .T. ) ;
#1878=ORIENTED_EDGE ( 'NONE', *, *, #63667, .T. ) ;
#1879=CARTESIAN_POINT ( 'NONE',  ( 110.8002664325828164, -46.40403567634503901, 13.85753003781498016 ) ) ;
#1880=CARTESIAN_POINT ( 'NONE',  ( 94.06648329127393993, -36.72944715994095333, 294.6356252759106837 ) ) ;
#1881=FACE_OUTER_BOUND ( 'NONE', #1933, .T. ) ;
#1882=CARTESIAN_POINT ( 'NONE',  ( 163.5667039024460223, -18.82844715994111340, -5.074374724088000832 ) ) ;
#1884=DIRECTION ( 'NONE',  ( -0.000000000000000000, 1.000000000000000000, 0.000000000000000000 ) ) ;
#1885=CARTESIAN_POINT ( 'NONE',  ( 118.0655259830059265, -38.35211242607485360, 223.7099109901979546 ) ) ;
#1886=VERTEX_POINT ( 'NONE', #45098 ) ;
#1888=CARTESIAN_POINT ( 'NONE',  ( 115.7036244402283529, -40.42759782077664710, 209.9482499725639855 ) ) ;
#1889=CONICAL_SURFACE ( 'NONE', #88912, 1.258750000000002922, 1.029744258676650093 ) ;
#1890=DIRECTION ( 'NONE',  ( -2.108538789381372925E-16, 0.5150380749100580413, 0.8571673007021100021 ) ) ;
#1891=EDGE_CURVE ( 'NONE', #43116, #66809, #65233, .T. ) ;
#1892=CARTESIAN_POINT ( 'NONE',  ( 116.2961902049681697, -40.76469377450285947, 54.93015473446794061 ) ) ;
#1894=VECTOR ( 'NONE', #46363, 1000.000000000000000 ) ;
#1896=CARTESIAN_POINT ( 'NONE',  ( 29.56670390244857316, -48.82844715994099971, 300.4678068554149490 ) ) ;
#1897=ADVANCED_FACE ( 'NONE', ( #72386, #45530 ), #51033, .F. ) ;
#1898=CARTESIAN_POINT ( 'NONE',  ( 160.7738106836351051, -48.62134037874900372, 129.9678068554149775 ) ) ;
#1899=CARTESIAN_POINT ( 'NONE',  ( 194.5667039024479834, -67.87844715994100397, 300.9178068554150514 ) ) ;
#1901=CARTESIAN_POINT ( 'NONE',  ( 96.83034234600413015, -40.83861266248845823, 251.6422919425777138 ) ) ;
#1903=ORIENTED_EDGE ( 'NONE', *, *, #34266, .T. ) ;
#1908=CARTESIAN_POINT ( 'NONE',  ( 107.3241674272228892, -25.27320757387406402, 321.5865679059475610 ) ) ;
#1910=CARTESIAN_POINT ( 'NONE',  ( 115.0382812869126923, -42.90717343850143806, 124.3008843337145493 ) ) ;
#1911=LINE ( 'NONE', #44558, #57846 ) ;
#1912=EDGE_CURVE ( 'NONE', #54183, #19039, #23242, .T. ) ;
#1913=CARTESIAN_POINT ( 'NONE',  ( 106.0550521757682816, -27.00111521709629514, 46.15848241876796720 ) ) ;
#1916=CARTESIAN_POINT ( 'NONE',  ( 115.6092852924205943, -42.78035731602705027, 49.33562527591095659 ) ) ;
#1918=TOROIDAL_SURFACE ( 'NONE', #52641, 11.75000000000000000, 2.550000000000000266 ) ;
#1919=EDGE_CURVE ( 'NONE', #28582, #4939, #58727, .T. ) ;
#1920=CARTESIAN_POINT ( 'NONE',  ( 109.9602307476630330, -48.22147533147688847, 242.7727681330539724 ) ) ;
#1921=ORIENTED_EDGE ( 'NONE', *, *, #75931, .T. ) ;
#1922=CIRCLE ( 'NONE', #42546, 4.749999999999976907 ) ;
#1924=CARTESIAN_POINT ( 'NONE',  ( 116.7956705048818833, -39.38589551711255865, 19.61517315323455080 ) ) ;
#1926=ADVANCED_FACE ( 'NONE', ( #30152 ), #2454, .F. ) ;
#1927=CARTESIAN_POINT ( 'NONE',  ( 99.91476266851738330, -32.73750773393640401, 108.7395189410199663 ) ) ;
#1928=CARTESIAN_POINT ( 'NONE',  ( 113.1681127151884141, -26.54159316308081173, 200.6470538473399756 ) ) ;
#1932=VERTEX_POINT ( 'NONE', #22906 ) ;
#1933=EDGE_LOOP ( 'NONE', ( #38657, #38106, #30690, #37524 ) ) ;
#1935=CARTESIAN_POINT ( 'NONE',  ( 83.06670390244808289, -58.72944715994108122, 207.5838068554169809 ) ) ;
#1936=ORIENTED_EDGE ( 'NONE', *, *, #27418, .F. ) ;
#1937=VERTEX_POINT ( 'NONE', #23798 ) ;
#1938=DIRECTION ( 'NONE',  ( -6.524622321627019585E-16, -4.013151879589939944E-16, -1.000000000000000000 ) ) ;
#1939=CARTESIAN_POINT ( 'NONE',  ( 97.12553659991493760, -37.99670770671464481, 42.42725359356597181 ) ) ;
#1940=CARTESIAN_POINT ( 'NONE',  ( 103.4870123794286059, -45.04810440550495798, 136.6876579233149300 ) ) ;
#1941=CARTESIAN_POINT ( 'NONE',  ( 105.6290166497307581, -47.07739640705644035, 257.4670538473392298 ) ) ;
#1942=EDGE_CURVE ( 'NONE', #34565, #32370, #37863, .T. ) ;
#1943=EDGE_CURVE ( 'NONE', #50013, #35318, #85140, .T. ) ;
#1944=CARTESIAN_POINT ( 'NONE',  ( 126.8164832912740110, -46.47944715994101017, 14.92562527591099020 ) ) ;
#1950=DIRECTION ( 'NONE',  ( 0.000000000000000000, 0.000000000000000000, -1.000000000000000000 ) ) ;
#1953=CARTESIAN_POINT ( 'NONE',  ( 114.5992475275822784, -44.05128143045557465, 98.21276813305395592 ) ) ;
#1955=ORIENTED_EDGE ( 'NONE', *, *, #57171, .T. ) ;
#1956=CARTESIAN_POINT ( 'NONE',  ( 96.53679867426635042, -40.09171982297686299, 281.5603871806728762 ) ) ;
#1961=LINE ( 'NONE', #35113, #15568 ) ;
#1962=CARTESIAN_POINT ( 'NONE',  ( 57.56670390244744340, -48.82844715994040286, 170.7178068554150911 ) ) ;
#1963=CARTESIAN_POINT ( 'NONE',  ( 167.6524903400755875, -49.32844715993520879, 180.4678068554150059 ) ) ;
#1964=CARTESIAN_POINT ( 'NONE',  ( 188.5667039024484097, -48.82844715993431350, 257.2178068554150059 ) ) ;
#1966=DIRECTION ( 'NONE',  ( 0.000000000000000000, 0.000000000000000000, 1.000000000000000000 ) ) ;
#1968=CARTESIAN_POINT ( 'NONE',  ( 97.81168843500762478, -40.51741166756562507, 12.63579318495451176 ) ) ;
#1969=CARTESIAN_POINT ( 'NONE',  ( 21.03689327557613709, -23.42844715994197813, 193.9678068554150627 ) ) ;
#1970=DIRECTION ( 'NONE',  ( -0.9254794337955621897, -0.3787978585227821382, 0.000000000000000000 ) ) ;
#1972=CARTESIAN_POINT ( 'NONE',  ( 36.23715912545429063, -47.82818131006125384, 249.9678068554150343 ) ) ;
#1973=CARTESIAN_POINT ( 'NONE',  ( 116.3368571269942464, -41.54685706111320087, 288.4441967044822945 ) ) ;
#1974=CARTESIAN_POINT ( 'NONE',  ( 95.91002759172351944, -32.73343517516348555, 172.0527681330539735 ) ) ;
#1975=CARTESIAN_POINT ( 'NONE',  ( 102.3596500697202174, -47.65578173298946751, 283.2527681330539053 ) ) ;
#1976=DIRECTION ( 'NONE',  ( 1.000000000000000000, 0.000000000000000000, 0.000000000000000000 ) ) ;
#1977=DIRECTION ( 'NONE',  ( 0.000000000000000000, 0.000000000000000000, -1.000000000000000000 ) ) ;
#1979=EDGE_LOOP ( 'NONE', ( #57902, #80804, #1590, #27732, #34775 ) ) ;
#1980=CARTESIAN_POINT ( 'NONE',  ( 71.25614885437424562, -84.12815644128085069, 540.9756252759101471 ) ) ;
#1982=CARTESIAN_POINT ( 'NONE',  ( 98.65123886609836745, -31.74476095556103061, 81.90133956162493689 ) ) ;
#1983=DIRECTION ( 'NONE',  ( 4.299999999999999979E-14, -1.000000000000000000, 4.400000000000000367E-29 ) ) ;
#1985=AXIS2_PLACEMENT_3D ( 'NONE', #70024, #47761, #75044 ) ;
#1987=CARTESIAN_POINT ( 'NONE',  ( 96.87985868497426623, -34.61725761836213167, 212.1641967044819808 ) ) ;
#1988=FACE_OUTER_BOUND ( 'NONE', #21891, .T. ) ;
#1989=CARTESIAN_POINT ( 'NONE',  ( 110.8549113655039378, -45.98405751658768992, 147.8856630510708214 ) ) ;
#1993=CARTESIAN_POINT ( 'NONE',  ( 116.0282290876930773, -41.23944930189807678, 98.45557829630303104 ) ) ;
#1994=CARTESIAN_POINT ( 'NONE',  ( 118.1720832024965802, -36.20253795304678590, 118.8641967044829784 ) ) ;
#1995=VERTEX_POINT ( 'NONE', #9708 ) ;
#1996=ORIENTED_EDGE ( 'NONE', *, *, #71175, .F. ) ;
#1997=AXIS2_PLACEMENT_3D ( 'NONE', #48456, #76195, #47125 ) ;
#1998=CARTESIAN_POINT ( 'NONE',  ( 98.44769980935930676, -38.78975051229773641, 52.94444044875496047 ) ) ;
#1999=CARTESIAN_POINT ( 'NONE',  ( 119.2637946045970097, -42.39761235918182081, 3.024967495036162912 ) ) ;
#2000=CARTESIAN_POINT ( 'NONE',  ( 99.40370404213548738, -29.74227323812501211, 226.7261014663869503 ) ) ;
#2003=DIRECTION ( 'NONE',  ( 1.000000000000000078E-15, -1.000000000000000000, 0.000000000000000000 ) ) ;
#2004=EDGE_CURVE ( 'NONE', #55608, #6226, #43488, .T. ) ;
#2009=CARTESIAN_POINT ( 'NONE',  ( 117.0023065291009061, -39.93004192841232936, 158.5784824187679476 ) ) ;
#2012=VERTEX_POINT ( 'NONE', #80102 ) ;
#2014=EDGE_CURVE ( 'NONE', #42554, #76542, #40577, .T. ) ;
#2017=CARTESIAN_POINT ( 'NONE',  ( 97.70664598133903667, -40.25154286292865891, 131.6128750669620047 ) ) ;
#2018=CARTESIAN_POINT ( 'NONE',  ( 98.15069168346546746, -41.26105110007194554, 102.7006730368125886 ) ) ;
#2019=CARTESIAN_POINT ( 'NONE',  ( 115.6671688226974197, -35.76553148137116267, 231.7214237029249659 ) ) ;
#2020=EDGE_CURVE ( 'NONE', #49604, #54780, #78350, .T. ) ;
#2021=VECTOR ( 'NONE', #60130, 1000.000000000000000 ) ;
#2022=CARTESIAN_POINT ( 'NONE',  ( 76.24325998657069192, -5.906223855237660914, -4.824374724089060429 ) ) ;
#2025=CARTESIAN_POINT ( 'NONE',  ( 102.9133425085070712, -27.12904003091135152, 155.4013395616249795 ) ) ;
#2026=DIRECTION ( 'NONE',  ( 0.000000000000000000, 1.000000000000000000, 0.000000000000000000 ) ) ;
#2028=ORIENTED_EDGE ( 'NONE', *, *, #46820, .T. ) ;
#2034=CARTESIAN_POINT ( 'NONE',  ( 131.5359215223094793, -35.65293368213150416, 7.043713522540487659 ) ) ;
#2035=EDGE_CURVE ( 'NONE', #3324, #86462, #81453, .T. ) ;
#2036=CARTESIAN_POINT ( 'NONE',  ( 110.1825742734413609, -44.80353631977761353, 15.67570941721097100 ) ) ;
#2038=ORIENTED_EDGE ( 'NONE', *, *, #67864, .T. ) ;
#2039=CARTESIAN_POINT ( 'NONE',  ( 116.4162535572406227, -39.30367360901732354, 9.635625275910939536 ) ) ;
#2040=EDGE_CURVE ( 'NONE', #19992, #80451, #49255, .T. ) ;
#2044=CIRCLE ( 'NONE', #42603, 2.517500000000005844 ) ;
#2045=CARTESIAN_POINT ( 'NONE',  ( 109.6431318019857741, -46.48005661577610681, 112.7814924369443048 ) ) ;
#2046=CIRCLE ( 'NONE', #73144, 0.2999999999999943823 ) ;
#2047=ORIENTED_EDGE ( 'NONE', *, *, #41980, .T. ) ;
#2049=VECTOR ( 'NONE', #49400, 999.9999999999998863 ) ;
#2050=CARTESIAN_POINT ( 'NONE',  ( 99.35983957736841887, -39.50259174935074213, 264.4195189410201579 ) ) ;
#2051=AXIS2_PLACEMENT_3D ( 'NONE', #14860, #42527, #7586 ) ;
#2052=CARTESIAN_POINT ( 'NONE',  ( 118.9428397581607442, -36.92852597549882177, 153.8127681330539644 ) ) ;
#2053=CARTESIAN_POINT ( 'NONE',  ( 108.2752786314947429, -47.69320359391970499, 157.6518157521019532 ) ) ;
#2054=LINE ( 'NONE', #1156, #52467 ) ;
#2055=CARTESIAN_POINT ( 'NONE',  ( 98.03678599612689482, -44.40402742967116723, 222.8870538473399563 ) ) ;
#2061=EDGE_CURVE ( 'NONE', #51053, #60205, #12385, .T. ) ;
#2063=ADVANCED_FACE ( 'NONE', ( #20103 ), #73913, .F. ) ;
#2064=CARTESIAN_POINT ( 'NONE',  ( 97.01576029581003979, -41.44069443601846814, 211.6632443235299945 ) ) ;
#2066=CARTESIAN_POINT ( 'NONE',  ( 97.95630822081318456, -30.46975087157407458, 165.8594347997199634 ) ) ;
#2068=DIRECTION ( 'NONE',  ( 0.000000000000000000, 0.000000000000000000, 1.000000000000000000 ) ) ;
#2069=FACE_OUTER_BOUND ( 'NONE', #72844, .T. ) ;
#2070=DIRECTION ( 'NONE',  ( -1.000000000000000000, 1.000000000000000078E-15, 0.000000000000000000 ) ) ;
#2071=CARTESIAN_POINT ( 'NONE',  ( 99.48017111314335637, -43.25549976577509881, 56.89151756084950762 ) ) ;
#2072=CARTESIAN_POINT ( 'NONE',  ( 99.55514648348079731, -29.48070623161996551, 246.7156252759109520 ) ) ;
#2073=DIRECTION ( 'NONE',  ( 0.000000000000000000, 0.000000000000000000, -1.000000000000000000 ) ) ;
#2075=DIRECTION ( 'NONE',  ( 0.000000000000000000, 0.000000000000000000, -1.000000000000000000 ) ) ;
#2078=LINE ( 'NONE', #21180, #28830 ) ;
#2079=CARTESIAN_POINT ( 'NONE',  ( 102.8854998099173628, -43.62190156306392197, 195.5838068554170945 ) ) ;
#2080=ORIENTED_EDGE ( 'NONE', *, *, #9388, .F. ) ;
#2082=CARTESIAN_POINT ( 'NONE',  ( 98.26213988389305598, -31.03978702703054537, 145.8699109901969848 ) ) ;
#2083=CARTESIAN_POINT ( 'NONE',  ( 117.9887704088505274, -38.42580343310776669, 64.69181575210097890 ) ) ;
#2084=CARTESIAN_POINT ( 'NONE',  ( 96.63066398506619237, -35.53291458860860530, 202.2356252759109623 ) ) ;
#2085=CARTESIAN_POINT ( 'NONE',  ( 33.92127028473601769, -29.73316016639540749, 342.9256252759119548 ) ) ;
#2086=CARTESIAN_POINT ( 'NONE',  ( 36.65249034007530327, -49.32844715994124130, 300.4678068554150059 ) ) ;
#2087=DIRECTION ( 'NONE',  ( 0.000000000000000000, 0.000000000000000000, 1.000000000000000000 ) ) ;
#2088=CARTESIAN_POINT ( 'NONE',  ( 163.2569089553700223, -33.54226604285010893, -5.074374724088000832 ) ) ;
#2089=CARTESIAN_POINT ( 'NONE',  ( 107.0664832912739399, -36.72944715994096754, 300.2406250056037038 ) ) ;
#2091=VERTEX_POINT ( 'NONE', #5122 ) ;
#2094=DIRECTION ( 'NONE',  ( 0.000000000000000000, 0.000000000000000000, -1.000000000000000000 ) ) ;
#2097=ORIENTED_EDGE ( 'NONE', *, *, #65777, .F. ) ;
#2099=VERTEX_POINT ( 'NONE', #68251 ) ;
#2100=CARTESIAN_POINT ( 'NONE',  ( 114.0075736764522389, -28.98025818340847692, 110.4956252759109816 ) ) ;
#2101=CARTESIAN_POINT ( 'NONE',  ( 36.65249034007526063, -48.32844715994123419, 300.4678068554150059 ) ) ;
#2103=DIRECTION ( 'NONE',  ( -4.237773401492740281E-14, 1.000000000000000000, 0.000000000000000000 ) ) ;
#2104=CARTESIAN_POINT ( 'NONE',  ( 104.4155842956043614, -46.14412563975625403, 22.35848241876892217 ) ) ;
#2110=AXIS2_PLACEMENT_3D ( 'NONE', #73687, #36936, #64637 ) ;
#2113=CARTESIAN_POINT ( 'NONE',  ( 33.78129701732233059, -35.65087443489924368, 117.4678068554150485 ) ) ;
#2114=CARTESIAN_POINT ( 'NONE',  ( 97.07207206033048408, -35.37844118961633910, 117.2189586084917465 ) ) ;
#2115=AXIS2_PLACEMENT_3D ( 'NONE', #72445, #25624, #25172 ) ;
#2116=FACE_OUTER_BOUND ( 'NONE', #56016, .T. ) ;
#2117=CARTESIAN_POINT ( 'NONE',  ( 161.4809174648185603, -49.32844715993547169, 180.4678068554150059 ) ) ;
#2118=EDGE_CURVE ( 'NONE', #43566, #38211, #79774, .T. ) ;
#2120=ADVANCED_FACE ( 'NONE', ( #74606 ), #13043, .F. ) ;
#2125=CARTESIAN_POINT ( 'NONE',  ( 107.0664832912739968, -36.72944715994100306, 277.6356252759110248 ) ) ;
#2126=CARTESIAN_POINT ( 'NONE',  ( 96.70769389551958284, -42.43415482991314036, 26.72705384733997747 ) ) ;
#2128=EDGE_CURVE ( 'NONE', #83421, #73910, #72499, .T. ) ;
#2129=DIRECTION ( 'NONE',  ( 0.000000000000000000, 0.000000000000000000, 1.000000000000000000 ) ) ;
#2131=CARTESIAN_POINT ( 'NONE',  ( 108.5685384152640864, -45.25263643686804471, 120.5214237029249915 ) ) ;
#2132=EDGE_CURVE ( 'NONE', #7741, #13694, #46432, .T. ) ;
#2133=CARTESIAN_POINT ( 'NONE',  ( 97.53201689872335578, -39.74949948161557955, 96.57057676354683906 ) ) ;
#2134=ADVANCED_FACE ( 'NONE', ( #19203 ), #19642, .F. ) ;
#2135=CARTESIAN_POINT ( 'NONE',  ( 25.56670390244832447, -48.82844715994168183, 257.2178068554150059 ) ) ;
#2137=VERTEX_POINT ( 'NONE', #87793 ) ;
#2138=LINE ( 'NONE', #28949, #75783 ) ;
#2139=ORIENTED_EDGE ( 'NONE', *, *, #23065, .T. ) ;
#2140=VERTEX_POINT ( 'NONE', #25558 ) ;
#2142=CARTESIAN_POINT ( 'NONE',  ( 115.8989637469753831, -39.93316602039875107, 169.9692023535169483 ) ) ;
#2143=DIRECTION ( 'NONE',  ( 0.000000000000000000, 1.000000000000000000, 0.000000000000000000 ) ) ;
#2144=CARTESIAN_POINT ( 'NONE',  ( 102.5487710710870033, -27.30991770518087591, 91.43276813305395478 ) ) ;
#2146=CARTESIAN_POINT ( 'NONE',  ( 111.2589507039926673, -45.80977664277359196, 17.92067989835221553 ) ) ;
#2147=ORIENTED_EDGE ( 'NONE', *, *, #60736, .T. ) ;
#2150=ORIENTED_EDGE ( 'NONE', *, *, #60777, .T. ) ;
#2151=CARTESIAN_POINT ( 'NONE',  ( 100.0385306026334717, -40.93546354753772221, 159.5738046553059917 ) ) ;
#2152=CARTESIAN_POINT ( 'NONE',  ( 117.4695374193713775, -37.69008693337416815, 78.75276813305399060 ) ) ;
#2154=CARTESIAN_POINT ( 'NONE',  ( 104.4960957391109417, -46.84663716100912012, 47.37848241876796607 ) ) ;
#2155=CARTESIAN_POINT ( 'NONE',  ( 102.8351866564443924, -46.28106417705388509, 173.2441967044829596 ) ) ;
#2156=DIRECTION ( 'NONE',  ( -0.000000000000000000, 1.000000000000000000, 0.000000000000000000 ) ) ;
#2158=CARTESIAN_POINT ( 'NONE',  ( 114.0221110621602492, -28.96402831996850225, 110.4956252759109816 ) ) ;
#2159=CARTESIAN_POINT ( 'NONE',  ( 48.45959712127231711, -26.00627455219176554, 313.9678068554150059 ) ) ;
#2163=CARTESIAN_POINT ( 'NONE',  ( 107.0664832912739399, -36.72944715994096754, 300.2406250056037038 ) ) ;
#2167=CONICAL_SURFACE ( 'NONE', #38393, 1.258750000000002922, 1.029744258676650093 ) ;
#2169=AXIS2_PLACEMENT_3D ( 'NONE', #19405, #25766, #87556 ) ;
#2170=VECTOR ( 'NONE', #76166, 1000.000000000000000 ) ;
#2171=CARTESIAN_POINT ( 'NONE',  ( 123.6837132603320413, -56.64645651782490177, 239.5838068554164693 ) ) ;
#2172=CARTESIAN_POINT ( 'NONE',  ( 99.06573214631099233, -44.35618096740151373, 36.92038718067297509 ) ) ;
#2173=CARTESIAN_POINT ( 'NONE',  ( 75.31670390244798341, -50.82844715994100682, 88.43480685541499042 ) ) ;
#2174=AXIS2_PLACEMENT_3D ( 'NONE', #70061, #41881, #83254 ) ;
#2175=CYLINDRICAL_SURFACE ( 'NONE', #5758, 0.5000000000000004441 ) ;
#2177=CARTESIAN_POINT ( 'NONE',  ( 101.5079035968563943, -28.64143341885324290, 50.55562527591095545 ) ) ;
#2179=CARTESIAN_POINT ( 'NONE',  ( 109.1969564574039282, -26.54663071456431211, 135.9127681330539872 ) ) ;
#2180=CYLINDRICAL_SURFACE ( 'NONE', #26274, 0.5000000000000104361 ) ;
#2182=ORIENTED_EDGE ( 'NONE', *, *, #45449, .F. ) ;
#2183=LINE ( 'NONE', #38465, #64338 ) ;
#2187=EDGE_LOOP ( 'NONE', ( #30572, #48799, #30481, #67896 ) ) ;
#2188=LINE ( 'NONE', #29442, #60705 ) ;
#2189=EDGE_CURVE ( 'NONE', #28049, #56291, #13728, .T. ) ;
#2190=CARTESIAN_POINT ( 'NONE',  ( 96.69933951777882442, -35.27033920508573317, 181.2156252759109805 ) ) ;
#2191=ORIENTED_EDGE ( 'NONE', *, *, #58584, .F. ) ;
#2193=CARTESIAN_POINT ( 'NONE',  ( 118.6781471654015689, -39.21772221756580734, 254.6584824187681022 ) ) ;
#2194=CARTESIAN_POINT ( 'NONE',  ( 101.6557087385557736, -27.03816153323032268, 101.4937205140059575 ) ) ;
#2195=CARTESIAN_POINT ( 'NONE',  ( 102.0693260774676077, -27.96916680133194788, 251.4954626382068170 ) ) ;
#2196=DIRECTION ( 'NONE',  ( 4.299999999999999979E-14, -1.000000000000000000, 4.400000000000000367E-29 ) ) ;
#2197=AXIS2_PLACEMENT_3D ( 'NONE', #49101, #70021, #56815 ) ;
#2199=EDGE_LOOP ( 'NONE', ( #46345, #19487, #45707, #60891 ) ) ;
#2200=EDGE_CURVE ( 'NONE', #24293, #72149, #60865, .T. ) ;
#2201=CIRCLE ( 'NONE', #32644, 2.029999999999997140 ) ;
#2202=EDGE_LOOP ( 'NONE', ( #9887, #66284, #10875, #64176 ) ) ;
#2204=ORIENTED_EDGE ( 'NONE', *, *, #24360, .F. ) ;
#2206=CARTESIAN_POINT ( 'NONE',  ( 106.5673366543293383, -47.17799660047543853, 243.5384824187679556 ) ) ;
#2208=CARTESIAN_POINT ( 'NONE',  ( 131.5918432679227692, -35.51852171454133611, 2.740177351677670625 ) ) ;
#2210=DIRECTION ( 'NONE',  ( 0.000000000000000000, 0.000000000000000000, 1.000000000000000000 ) ) ;
#2211=DIRECTION ( 'NONE',  ( 0.9834602067019598826, 0.1811243270069988198, 0.000000000000000000 ) ) ;
#2212=CARTESIAN_POINT ( 'NONE',  ( 99.04884357002234196, -44.37228004027687689, 36.92038718067297509 ) ) ;
#2214=VERTEX_POINT ( 'NONE', #82791 ) ;
#2217=CARTESIAN_POINT ( 'NONE',  ( 107.0664832912739968, -36.72944715994100306, 293.2242906452868851 ) ) ;
#2219=DIRECTION ( 'NONE',  ( 0.8758084860610321210, 0.03696114963002913867, 0.4812414873652411940 ) ) ;
#2220=CARTESIAN_POINT ( 'NONE',  ( 113.3415799102510277, -29.55617248177381740, 285.5032443235294863 ) ) ;
#2223=CARTESIAN_POINT ( 'NONE',  ( 103.4152017835536270, -27.65577212482034497, 126.3813395616249835 ) ) ;
#2225=CARTESIAN_POINT ( 'NONE',  ( 105.7148859710100339, -46.72376874668114510, 27.46891152066978847 ) ) ;
#2227=LINE ( 'NONE', #35832, #3709 ) ;
#2228=EDGE_CURVE ( 'NONE', #8503, #22291, #18794, .T. ) ;
#2229=CARTESIAN_POINT ( 'NONE',  ( 101.1158614047228070, -28.69863163947533735, 195.5838086201111992 ) ) ;
#2232=CARTESIAN_POINT ( 'NONE',  ( 104.9598549460505126, -28.12176414095025834, 281.6987261630399644 ) ) ;
#2233=VECTOR ( 'NONE', #17843, 1000.000000000000114 ) ;
#2235=AXIS2_PLACEMENT_3D ( 'NONE', #81438, #46860, #26447 ) ;
#2236=DIRECTION ( 'NONE',  ( 0.000000000000000000, 0.000000000000000000, 1.000000000000000000 ) ) ;
#2239=EDGE_CURVE ( 'NONE', #23384, #56843, #21449, .T. ) ;
#2240=CYLINDRICAL_SURFACE ( 'NONE', #2429, 2.517500000000005844 ) ;
#2243=CARTESIAN_POINT ( 'NONE',  ( 29.77381068363512995, -48.62134037875389936, 180.4678068554150911 ) ) ;
#2244=DIRECTION ( 'NONE',  ( -1.000000000000000078E-15, -1.000000000000000083E-30, 1.000000000000000000 ) ) ;
#2245=VERTEX_POINT ( 'NONE', #15076 ) ;
#2246=CARTESIAN_POINT ( 'NONE',  ( 98.64717563880898865, -43.89145428829765194, 76.89943479971999807 ) ) ;
#2247=EDGE_LOOP ( 'NONE', ( #64116, #5451, #68628, #29875 ) ) ;
#2248=CARTESIAN_POINT ( 'NONE',  ( 116.6246688045503248, -35.02307164793359107, 48.38956268521998538 ) ) ;
#2250=CARTESIAN_POINT ( 'NONE',  ( 117.1137397764925794, -36.70408575741609525, 89.82803621957074824 ) ) ;
#2251=CARTESIAN_POINT ( 'NONE',  ( 99.76930146980365066, -30.21680002102808515, 190.7470538473399415 ) ) ;
#2252=CARTESIAN_POINT ( 'NONE',  ( 83.56670390244801183, -35.47069715994107497, 218.8274735512160589 ) ) ;
#2253=DIRECTION ( 'NONE',  ( 0.000000000000000000, 0.000000000000000000, 1.000000000000000000 ) ) ;
#2255=VECTOR ( 'NONE', #7789, 1000.000000000000000 ) ;
#2256=CARTESIAN_POINT ( 'NONE',  ( 116.5760347145385367, -42.45360038892302157, 274.3832443235299365 ) ) ;
#2257=VERTEX_POINT ( 'NONE', #538 ) ;
#2258=CYLINDRICAL_SURFACE ( 'NONE', #76327, 0.5000000000000172085 ) ;
#2260=CARTESIAN_POINT ( 'NONE',  ( 108.6553284749260229, -25.75107874774626993, 145.9737205140069420 ) ) ;
#2265=ORIENTED_EDGE ( 'NONE', *, *, #2519, .F. ) ;
#2266=CARTESIAN_POINT ( 'NONE',  ( 107.0664832912739399, -36.72944715994095333, 302.4856252759109907 ) ) ;
#2268=CARTESIAN_POINT ( 'NONE',  ( 117.2610056464983899, -34.82931580038571440, 203.9851490854349549 ) ) ;
#2271=DIRECTION ( 'NONE',  ( 0.000000000000000000, 1.000000000000000000, 0.000000000000000000 ) ) ;
#2272=CARTESIAN_POINT ( 'NONE',  ( 117.5122013968931327, -37.28485508719111863, 14.78419670448294454 ) ) ;
#2275=CARTESIAN_POINT ( 'NONE',  ( 97.39132285814163481, -39.27863230505913350, 172.5314464909690173 ) ) ;
#2277=EDGE_CURVE ( 'NONE', #8532, #10148, #83228, .T. ) ;
#2278=EDGE_LOOP ( 'NONE', ( #26146, #60774, #48811, #5437, #49983, #10714, #79016, #72653, #66355, #63648, #52989, #54495, #41268, #18003 ) ) ;
#2279=ORIENTED_EDGE ( 'NONE', *, *, #48571, .T. ) ;
#2280=CIRCLE ( 'NONE', #86442, 2.117000000000007987 ) ;
#2283=CARTESIAN_POINT ( 'NONE',  ( 110.6887065042383256, -47.98678726807249006, 207.8241967044819489 ) ) ;
#2284=CONICAL_SURFACE ( 'NONE', #26902, 13.31607168056649115, 0.1047197551196538678 ) ;
#2287=CYLINDRICAL_SURFACE ( 'NONE', #65139, 2.117000000000000881 ) ;
#2288=FACE_OUTER_BOUND ( 'NONE', #45660, .T. ) ;
#2289=CARTESIAN_POINT ( 'NONE',  ( 98.10212974493634874, -35.44374275293071008, 225.6476579233149948 ) ) ;
#2291=CARTESIAN_POINT ( 'NONE',  ( 118.7081646409640427, -34.65111545711814500, 44.96705384733895272 ) ) ;
#2293=CARTESIAN_POINT ( 'NONE',  ( 117.4914506980151572, -37.69211045134998272, 78.75276813305399060 ) ) ;
#2294=ORIENTED_EDGE ( 'NONE', *, *, #64461, .F. ) ;
#2295=LINE ( 'NONE', #56326, #17593 ) ;
#2296=VERTEX_POINT ( 'NONE', #76402 ) ;
#2297=DIRECTION ( 'NONE',  ( 0.000000000000000000, 0.000000000000000000, -1.000000000000000000 ) ) ;
#2299=CARTESIAN_POINT ( 'NONE',  ( 100.9524021217529111, -28.70875815854373769, 276.5941401920176190 ) ) ;
#2301=CARTESIAN_POINT ( 'NONE',  ( 71.06648329127399677, -8.729447159940999512, 323.8756252759120002 ) ) ;
#2304=CARTESIAN_POINT ( 'NONE',  ( 163.1639762274590169, -34.03355364505800651, 193.9678068554150059 ) ) ;
#2306=VECTOR ( 'NONE', #60851, 1000.000000000000000 ) ;
#2308=EDGE_CURVE ( 'NONE', #9456, #67515, #7262, .T. ) ;
#2309=CARTESIAN_POINT ( 'NONE',  ( 114.5834136592134200, -44.03589093681723909, 98.21276813305395592 ) ) ;
#2311=VECTOR ( 'NONE', #86354, 1000.000000000000000 ) ;
#2314=CARTESIAN_POINT ( 'NONE',  ( 134.0664832912740110, -46.72944715994100306, 4.925625275910997303 ) ) ;
#2316=CARTESIAN_POINT ( 'NONE',  ( 127.1498166246069985, 12.92155284005802685, 349.2756252759110680 ) ) ;
#2317=VERTEX_POINT ( 'NONE', #76849 ) ;
#2318=CARTESIAN_POINT ( 'NONE',  ( 115.9999835663602425, -32.15690669870756579, 120.2027918068147869 ) ) ;
#2320=DIRECTION ( 'NONE',  ( 0.000000000000000000, 1.000000000000000000, 0.000000000000000000 ) ) ;
#2321=DIRECTION ( 'NONE',  ( 0.000000000000000000, 0.000000000000000000, -1.000000000000000000 ) ) ;
#2322=CYLINDRICAL_SURFACE ( 'NONE', #12343, 9.999999999999998224 ) ;
#2323=FACE_OUTER_BOUND ( 'NONE', #74053, .T. ) ;
#2326=AXIS2_PLACEMENT_3D ( 'NONE', #9134, #51327, #50895 ) ;
#2328=CARTESIAN_POINT ( 'NONE',  ( 112.4269750522866076, -44.91043508143932428, 174.0384824187679556 ) ) ;
#2329=EDGE_CURVE ( 'NONE', #89894, #9402, #88512, .T. ) ;
#2331=ORIENTED_EDGE ( 'NONE', *, *, #77422, .F. ) ;
#2332=CARTESIAN_POINT ( 'NONE',  ( 111.1466539572837320, -45.61852150024213870, 23.91848241876692782 ) ) ;
#2333=LINE ( 'NONE', #57726, #3410 ) ;
#2334=CARTESIAN_POINT ( 'NONE',  ( 110.8544976311862627, -45.98422686449477936, 52.88562747957674048 ) ) ;
#2335=ADVANCED_FACE ( 'NONE', ( #70491 ), #27351, .F. ) ;
#2336=CARTESIAN_POINT ( 'NONE',  ( 168.0371591254543944, -48.62818131005519717, 249.9678068554149775 ) ) ;
#2339=CARTESIAN_POINT ( 'NONE',  ( 98.06605190618643064, -40.64173669134676459, 231.6527681330539679 ) ) ;
#2340=ORIENTED_EDGE ( 'NONE', *, *, #72951, .F. ) ;
#2342=CARTESIAN_POINT ( 'NONE',  ( 102.9614994733801439, -44.58294233512814486, 208.6244404487539725 ) ) ;
#2343=CARTESIAN_POINT ( 'NONE',  ( 117.0713428532484244, -35.45787740602197857, 54.92720707917401768 ) ) ;
#2344=CARTESIAN_POINT ( 'NONE',  ( 114.4295241859595933, -42.56572631025478870, 44.73682140113599814 ) ) ;
#2349=ORIENTED_EDGE ( 'NONE', *, *, #6584, .T. ) ;
#2351=DIRECTION ( 'NONE',  ( 0.000000000000000000, 1.000000000000000000, 0.000000000000000000 ) ) ;
#2353=CARTESIAN_POINT ( 'NONE',  ( 97.63514171170966449, -41.12017164899860688, 256.6727681330537507 ) ) ;
#2355=ORIENTED_EDGE ( 'NONE', *, *, #75957, .T. ) ;
#2356=ORIENTED_EDGE ( 'NONE', *, *, #15049, .T. ) ;
#2357=DIRECTION ( 'NONE',  ( 1.000000000000000000, 3.999999999999999995E-14, 1.000000000000000078E-15 ) ) ;
#2358=DIRECTION ( 'NONE',  ( 0.9999999853157766072, 0.0001713722456143218888, 0.000000000000000000 ) ) ;
#2359=DIRECTION ( 'NONE',  ( 1.000000000000000000, 0.000000000000000000, 0.000000000000000000 ) ) ;
#2360=CARTESIAN_POINT ( 'NONE',  ( 99.99294959284291906, -33.44233276930008714, 9.425625275910963552 ) ) ;
#2361=VECTOR ( 'NONE', #14084, 1000.000000000000000 ) ;
#2362=CARTESIAN_POINT ( 'NONE',  ( 103.0217603822331398, -26.37318333953113836, 16.37276813305293999 ) ) ;
#2364=DIRECTION ( 'NONE',  ( 0.000000000000000000, 1.000000000000000000, 0.000000000000000000 ) ) ;
#2366=CIRCLE ( 'NONE', #31386, 0.5000000000000004441 ) ;
#2367=CARTESIAN_POINT ( 'NONE',  ( 118.7813114821712901, -34.63805691389952557, 44.96705384733895272 ) ) ;
#2368=VECTOR ( 'NONE', #76069, 1000.000000000000000 ) ;
#2369=DIRECTION ( 'NONE',  ( -0.7071067811864676367, -0.7071067811866273978, -7.071067811864669709E-16 ) ) ;
#2370=AXIS2_PLACEMENT_3D ( 'NONE', #51800, #58622, #16865 ) ;
#2371=CARTESIAN_POINT ( 'NONE',  ( 105.0216316738932107, -25.86677467614671500, 280.2365776568631759 ) ) ;
#2372=ORIENTED_EDGE ( 'NONE', *, *, #78459, .F. ) ;
#2373=CARTESIAN_POINT ( 'NONE',  ( 82.57637212004242144, -17.60518726036903203, 2.783021291305785905 ) ) ;
#2374=CARTESIAN_POINT ( 'NONE',  ( 97.81863755922226744, -40.53440256270629760, 17.63675073572146346 ) ) ;
#2375=CARTESIAN_POINT ( 'NONE',  ( 160.7738106836350482, -48.62134037874900372, 180.4678068554150059 ) ) ;
#2376=CARTESIAN_POINT ( 'NONE',  ( 99.60924227704973077, -33.40991670024246218, 98.81094751244894780 ) ) ;
#2377=CARTESIAN_POINT ( 'NONE',  ( 99.06932979199925171, -29.95266829982950441, 211.7670538473399517 ) ) ;
#2378=FACE_OUTER_BOUND ( 'NONE', #26754, .T. ) ;
#2379=ORIENTED_EDGE ( 'NONE', *, *, #6516, .F. ) ;
#2381=DIRECTION ( 'NONE',  ( 0.7071067811861589947, -0.7071067811869361508, 0.000000000000000000 ) ) ;
#2382=ORIENTED_EDGE ( 'NONE', *, *, #13447, .T. ) ;
#2383=EDGE_LOOP ( 'NONE', ( #3491, #12437, #2480, #38867, #9258 ) ) ;
#2384=CARTESIAN_POINT ( 'NONE',  ( 95.60734603896358408, -36.72944715994100306, 300.2406250056037038 ) ) ;
#2385=VERTEX_POINT ( 'NONE', #5011 ) ;
#2386=ORIENTED_EDGE ( 'NONE', *, *, #75745, .F. ) ;
#2391=CARTESIAN_POINT ( 'NONE',  ( 112.1370707133610551, -28.01151978404558207, 24.65666564914236858 ) ) ;
#2392=CARTESIAN_POINT ( 'NONE',  ( 100.0120368033278311, -41.59636475471172901, 126.2295626852199746 ) ) ;
#2393=CARTESIAN_POINT ( 'NONE',  ( 111.7490138926534797, -27.39026733005105640, 279.7070538473396937 ) ) ;
#2398=DIRECTION ( 'NONE',  ( 0.000000000000000000, 1.000000000000000000, 0.000000000000000000 ) ) ;
#2404=PRODUCT_DEFINITION_CONTEXT ( 'detailed design', #26055, 'design' ) ;
#2405=CARTESIAN_POINT ( 'NONE',  ( 108.0141129856239957, -24.91663700320364327, 265.0127681330535552 ) ) ;
#2406=CARTESIAN_POINT ( 'NONE',  ( 96.67145939589113368, -37.96898657530446997, 37.42133956162496844 ) ) ;
#2408=CARTESIAN_POINT ( 'NONE',  ( 123.6837132603318992, -16.81243780205710436, 239.5838068554165545 ) ) ;
#2411=CYLINDRICAL_SURFACE ( 'NONE', #66983, 2.500000000000002220 ) ;
#2413=LINE ( 'NONE', #16050, #15526 ) ;
#2414=EDGE_CURVE ( 'NONE', #34580, #72320, #63, .T. ) ;
#2416=FACE_OUTER_BOUND ( 'NONE', #34062, .T. ) ;
#2417=ADVANCED_FACE ( 'NONE', ( #39969 ), #32256, .T. ) ;
#2418=DIRECTION ( 'NONE',  ( 0.7071067811865187069, 0.7071067811865764385, 7.071067811865181482E-16 ) ) ;
#2419=CARTESIAN_POINT ( 'NONE',  ( 97.19579330311479737, -33.30690068839255957, 286.0613395616251751 ) ) ;
#2420=CARTESIAN_POINT ( 'NONE',  ( 103.5424053135282634, -26.88047730603072694, 186.3499109901969746 ) ) ;
#2421=CARTESIAN_POINT ( 'NONE',  ( 104.6438654950096350, -47.53759819287119370, 23.38895860924494841 ) ) ;
#2422=VECTOR ( 'NONE', #86944, 1000.000000000000000 ) ;
#2423=CARTESIAN_POINT ( 'NONE',  ( 61.56670390244634916, -23.42844715994043270, 180.4678068554151196 ) ) ;
#2425=CARTESIAN_POINT ( 'NONE',  ( 41.56648329127399677, -18.82844715994099971, 16.80862527591200006 ) ) ;
#2426=CIRCLE ( 'NONE', #50253, 3.299999999999997158 ) ;
#2429=AXIS2_PLACEMENT_3D ( 'NONE', #71288, #17648, #29491 ) ;
#2430=EDGE_CURVE ( 'NONE', #52659, #76993, #18186, .T. ) ;
#2434=CARTESIAN_POINT ( 'NONE',  ( 116.8058161338297509, -37.62879752186919546, 74.75276813305298163 ) ) ;
#2435=CARTESIAN_POINT ( 'NONE',  ( 31.90335556477753087, -33.89581943344372661, 117.4678068554150485 ) ) ;
#2436=ORIENTED_EDGE ( 'NONE', *, *, #62322, .T. ) ;
#2437=FACE_OUTER_BOUND ( 'NONE', #38144, .T. ) ;
#2438=CARTESIAN_POINT ( 'NONE',  ( 97.42226921825846375, -40.63044708855864684, 202.6327681330539860 ) ) ;
#2440=CARTESIAN_POINT ( 'NONE',  ( 152.0371591254585155, -47.82818131005588214, 193.9678068554149775 ) ) ;
#2441=DIRECTION ( 'NONE',  ( 1.000000000000000000, 4.299999999999999979E-14, 1.000000000000000078E-15 ) ) ;
#2443=CARTESIAN_POINT ( 'NONE',  ( 107.0664832912739399, -36.72944715994095333, 302.6356252759109680 ) ) ;
#2445=CARTESIAN_POINT ( 'NONE',  ( 101.9926790296990617, -45.44549198893967201, 97.15644839471165994 ) ) ;
#2446=CARTESIAN_POINT ( 'NONE',  ( 114.2951562036313646, -44.16484043540982185, 118.2022919425779719 ) ) ;
#2447=ORIENTED_EDGE ( 'NONE', *, *, #64197, .F. ) ;
#2448=ORIENTED_EDGE ( 'NONE', *, *, #1323, .T. ) ;
#2449=CARTESIAN_POINT ( 'NONE',  ( 98.70151408295986073, -32.45115127476004346, 92.39396425827794701 ) ) ;
#2450=CLOSED_SHELL ( 'NONE', ( #67978, #44873, #65919, #73944, #9506, #75828, #29716, #45419, #66834, #4528 ) ) ;
#2451=DIRECTION ( 'NONE',  ( -1.000000000000000000, -4.299999999999999979E-14, -1.000000000000000078E-15 ) ) ;
#2452=CARTESIAN_POINT ( 'NONE',  ( 104.0204373342842814, -47.42213563049708824, 213.3556252759109668 ) ) ;
#2454=CYLINDRICAL_SURFACE ( 'NONE', #20307, 2.500000000000002220 ) ;
#2457=EDGE_CURVE ( 'NONE', #48113, #52443, #27414, .T. ) ;
#2460=EDGE_CURVE ( 'NONE', #38655, #6628, #78419, .T. ) ;
#2461=CARTESIAN_POINT ( 'NONE',  ( 97.76587557681018836, -42.65924729906321744, 141.7661014663869707 ) ) ;
#2462=VERTEX_POINT ( 'NONE', #84014 ) ;
#2463=ORIENTED_EDGE ( 'NONE', *, *, #46767, .F. ) ;
#2464=ORIENTED_EDGE ( 'NONE', *, *, #38378, .T. ) ;
#2465=ADVANCED_FACE ( 'NONE', ( #40860 ), #14970, .F. ) ;
#2469=CARTESIAN_POINT ( 'NONE',  ( 172.5664832912728457, -27.82844715994070484, 141.9256252759119832 ) ) ;
#2470=CARTESIAN_POINT ( 'NONE',  ( 98.38024141146789248, -41.69495811671281160, 102.7397364358299683 ) ) ;
#2471=CARTESIAN_POINT ( 'NONE',  ( 115.6591437269271694, -35.69643618062379176, 236.7518998934009460 ) ) ;
#2472=TOROIDAL_SURFACE ( 'NONE', #43088, 13.50000000000000000, 0.5000000000000000000 ) ;
#2474=CARTESIAN_POINT ( 'NONE',  ( 104.5625478726873894, -48.31265885861421339, 182.4070538473399665 ) ) ;
#2475=FACE_OUTER_BOUND ( 'NONE', #4820, .T. ) ;
#2476=EDGE_LOOP ( 'NONE', ( #82219, #32746, #88557, #78259, #36525, #35506, #87850, #66493, #83455, #35952, #23042, #13862, #17754, #32156, #54995, #34490 ) ) ;
#2477=EDGE_LOOP ( 'NONE', ( #89283, #43761, #21479, #6064, #55922 ) ) ;
#2478=ORIENTED_EDGE ( 'NONE', *, *, #80459, .F. ) ;
#2480=ORIENTED_EDGE ( 'NONE', *, *, #65974, .F. ) ;
#2483=CARTESIAN_POINT ( 'NONE',  ( 133.6902059199614143, -33.99866847873242648, 8.209451181318698332 ) ) ;
#2484=CARTESIAN_POINT ( 'NONE',  ( 106.3528233092926740, -46.09786297945525035, 263.9596785439923678 ) ) ;
#2485=CARTESIAN_POINT ( 'NONE',  ( 116.3114837287122754, -32.94280867712679850, 274.1356252759109680 ) ) ;
#2488=AXIS2_PLACEMENT_3D ( 'NONE', #42561, #63024, #42126 ) ;
#2489=CARTESIAN_POINT ( 'NONE',  ( 114.0969355440510355, -42.17668752783679054, 9.635625275910941312 ) ) ;
#2490=FACE_BOUND ( 'NONE', #213, .T. ) ;
#2491=VERTEX_POINT ( 'NONE', #20881 ) ;
#2493=VECTOR ( 'NONE', #56354, 1000.000000000000000 ) ;
#2494=VECTOR ( 'NONE', #83577, 1000.000000000000000 ) ;
#2495=DIRECTION ( 'NONE',  ( 0.000000000000000000, 0.000000000000000000, -1.000000000000000000 ) ) ;
#2496=AXIS2_PLACEMENT_3D ( 'NONE', #9728, #36987, #56519 ) ;
#2497=ORIENTED_EDGE ( 'NONE', *, *, #86925, .T. ) ;
#2498=ORIENTED_EDGE ( 'NONE', *, *, #31190, .T. ) ;
#2500=CARTESIAN_POINT ( 'NONE',  ( 114.7745679063646378, -33.04956858091291139, 18.60384839950496172 ) ) ;
#2501=CARTESIAN_POINT ( 'NONE',  ( 117.0895389762686136, -39.67643183956238317, 183.5984824187679578 ) ) ;
#2502=CARTESIAN_POINT ( 'NONE',  ( 97.76587557681018836, -42.65924729906321744, 141.7661014663869707 ) ) ;
#2503=CARTESIAN_POINT ( 'NONE',  ( 182.5667039024459939, -19.82844715994031759, 342.9256252759109884 ) ) ;
#2504=CARTESIAN_POINT ( 'NONE',  ( 115.9598434605651107, -30.16574962093465828, 255.3203871806729524 ) ) ;
#2505=DIRECTION ( 'NONE',  ( 1.000000000000000000, 0.000000000000000000, 0.000000000000000000 ) ) ;
#2509=VERTEX_POINT ( 'NONE', #14062 ) ;
#2510=AXIS2_PLACEMENT_3D ( 'NONE', #86283, #13549, #13115 ) ;
#2511=CIRCLE ( 'NONE', #89528, 0.5000000000000004441 ) ;
#2512=CARTESIAN_POINT ( 'NONE',  ( 109.4554010020096513, -25.88943074854985227, 179.8918157521019339 ) ) ;
#2513=ORIENTED_EDGE ( 'NONE', *, *, #76054, .F. ) ;
#2515=CARTESIAN_POINT ( 'NONE',  ( 111.4173512164996254, -47.75262429423162303, 172.8756252759109771 ) ) ;
#2517=CARTESIAN_POINT ( 'NONE',  ( 136.5173892390752712, -35.48112160756611644, 7.135585143040955813 ) ) ;
#2518=CARTESIAN_POINT ( 'NONE',  ( 51.06648329127330044, -0.7548456658612000547, 331.7756252759120343 ) ) ;
#2519=EDGE_CURVE ( 'NONE', #38575, #4939, #34813, .T. ) ;
#2520=CARTESIAN_POINT ( 'NONE',  ( 98.00595362218291484, -39.44849273793310829, 277.6356252759110248 ) ) ;
#2521=CARTESIAN_POINT ( 'NONE',  ( 90.44969454456413871, -53.34645651782494724, 239.5838068554169809 ) ) ;
#2522=CARTESIAN_POINT ( 'NONE',  ( 96.79764630557892247, -40.75620882907055176, 242.6118157521009664 ) ) ;
#2523=LINE ( 'NONE', #57915, #19075 ) ;
#2524=DIRECTION ( 'NONE',  ( 0.000000000000000000, 0.000000000000000000, 1.000000000000000000 ) ) ;
#2525=DIRECTION ( 'NONE',  ( 0.000000000000000000, 1.000000000000000000, 0.000000000000000000 ) ) ;
#2526=EDGE_CURVE ( 'NONE', #8195, #79540, #13099, .T. ) ;
#2527=CARTESIAN_POINT ( 'NONE',  ( 107.0664832912739399, -36.72944715994096754, 299.5704287327187103 ) ) ;
#2528=CARTESIAN_POINT ( 'NONE',  ( 176.7738106835694225, -48.62134037881071436, 249.9678068554149775 ) ) ;
#2529=EDGE_CURVE ( 'NONE', #54739, #53364, #18864, .T. ) ;
#2530=CARTESIAN_POINT ( 'NONE',  ( 73.06670390244801183, -58.72944715994112386, 198.9178068554149945 ) ) ;
#2531=CARTESIAN_POINT ( 'NONE',  ( 114.8835829893441911, -32.52868086562086347, 195.5838068554168103 ) ) ;
#2535=CARTESIAN_POINT ( 'NONE',  ( 107.5668325082694139, -47.79493819276859057, 192.6003871806729535 ) ) ;
#2536=CARTESIAN_POINT ( 'NONE',  ( 98.64735160015825954, -43.89130460420365409, 72.89943479972099283 ) ) ;
#2537=CARTESIAN_POINT ( 'NONE',  ( 98.34346157482828232, -29.86603762143552032, 196.8080062282919869 ) ) ;
#2538=DIRECTION ( 'NONE',  ( 0.000000000000000000, 0.000000000000000000, 1.000000000000000000 ) ) ;
#2540=LINE ( 'NONE', #62954, #23247 ) ;
#2542=CARTESIAN_POINT ( 'NONE',  ( 115.0889047250496304, -30.61763668164335428, 69.34395860908813347 ) ) ;
#2543=DIRECTION ( 'NONE',  ( -0.000000000000000000, -0.000000000000000000, 1.000000000000000000 ) ) ;
#2545=VECTOR ( 'NONE', #22991, 1000.000000000000000 ) ;
#2546=ADVANCED_FACE ( 'NONE', ( #57172 ), #77642, .F. ) ;
#2547=DIRECTION ( 'NONE',  ( 0.000000000000000000, 0.000000000000000000, 1.000000000000000000 ) ) ;
#2548=EDGE_CURVE ( 'NONE', #85262, #26105, #68216, .T. ) ;
#2549=VERTEX_POINT ( 'NONE', #51694 ) ;
#2551=CARTESIAN_POINT ( 'NONE',  ( 114.8228036748933079, -33.15234975719755539, 103.5924198280769843 ) ) ;
#2554=CARTESIAN_POINT ( 'NONE',  ( 115.2499566122392736, -44.12502604085369029, 79.25372051400697160 ) ) ;
#2555=CARTESIAN_POINT ( 'NONE',  ( 123.6837132603319560, -53.34645651782485487, 229.5838068554170093 ) ) ;
#2556=EDGE_CURVE ( 'NONE', #76619, #84501, #79441, .T. ) ;
#2557=DIRECTION ( 'NONE',  ( 1.000000000000000000, 3.999999999999999995E-14, 1.000000000000000078E-15 ) ) ;
#2558=DIRECTION ( 'NONE',  ( 0.000000000000000000, 0.000000000000000000, 1.000000000000000000 ) ) ;
#2560=CARTESIAN_POINT ( 'NONE',  ( 106.6352542858682284, -26.36832623700835398, 40.09753003781596448 ) ) ;
#2561=ORIENTED_EDGE ( 'NONE', *, *, #35543, .T. ) ;
#2562=ORIENTED_EDGE ( 'NONE', *, *, #7027, .T. ) ;
#2563=ORIENTED_EDGE ( 'NONE', *, *, #89281, .T. ) ;
#2565=AXIS2_PLACEMENT_3D ( 'NONE', #44897, #9954, #78999 ) ;
#2566=LINE ( 'NONE', #87458, #12345 ) ;
#2570=DIRECTION ( 'NONE',  ( 0.7071067811868672059, 0.7071067811862279395, 6.612322855857878503E-17 ) ) ;
#2571=CARTESIAN_POINT ( 'NONE',  ( 97.78477890316482046, -40.45109945164446685, 52.62952827575012549 ) ) ;
#2574=CARTESIAN_POINT ( 'NONE',  ( 114.3378803067696765, -44.16957155219879638, 73.19276813305397411 ) ) ;
#2576=ADVANCED_FACE ( 'NONE', ( #43542 ), #65345, .F. ) ;
#2578=CARTESIAN_POINT ( 'NONE',  ( 102.0670556523651129, -27.97049767320797642, 270.4897918799564422 ) ) ;
#2580=EDGE_CURVE ( 'NONE', #65668, #43936, #65776, .T. ) ;
#2581=VECTOR ( 'NONE', #41232, 1000.000000000000000 ) ;
#2583=CARTESIAN_POINT ( 'NONE',  ( 114.7692409103599687, -39.43078961860824450, 131.3766617981629565 ) ) ;
#2584=AXIS2_PLACEMENT_3D ( 'NONE', #60286, #27574, #40741 ) ;
#2585=CARTESIAN_POINT ( 'NONE',  ( 97.80804003460494300, -40.50849928945232392, 96.63485748601286218 ) ) ;
#2586=DIRECTION ( 'NONE',  ( 0.7071067811739204512, -0.7071067811991745833, 0.000000000000000000 ) ) ;
#2588=ORIENTED_EDGE ( 'NONE', *, *, #74749, .T. ) ;
#2590=ORIENTED_EDGE ( 'NONE', *, *, #8065, .T. ) ;
#2591=VERTEX_POINT ( 'NONE', #16310 ) ;
#2592=CARTESIAN_POINT ( 'NONE',  ( 99.50276801249795255, -32.11225214635365433, 167.3215833058969793 ) ) ;
#2594=CARTESIAN_POINT ( 'NONE',  ( 97.81677459100555438, -31.87350772351088679, 131.9413395616259947 ) ) ;
#2595=CARTESIAN_POINT ( 'NONE',  ( 97.31584367109211087, -39.30597582529259171, 121.5314585950798403 ) ) ;
#2597=CARTESIAN_POINT ( 'NONE',  ( 117.0897445426788295, -37.64026809670689744, 18.75396567128554892 ) ) ;
#2598=ORIENTED_EDGE ( 'NONE', *, *, #57285, .F. ) ;
#2599=ORIENTED_EDGE ( 'NONE', *, *, #69975, .F. ) ;
#2601=CARTESIAN_POINT ( 'NONE',  ( 102.5899018517108772, -44.13627803831183627, 199.9499951314959674 ) ) ;
#2602=CARTESIAN_POINT ( 'NONE',  ( 104.7546666864753320, -46.91776733316893200, 72.39848241876795498 ) ) ;
#2603=VERTEX_POINT ( 'NONE', #29488 ) ;
#2604=CARTESIAN_POINT ( 'NONE',  ( 115.5933672690474765, -28.53551910654237389, 39.43562527591099354 ) ) ;
#2605=CARTESIAN_POINT ( 'NONE',  ( 104.4482647075962518, -26.61598136914473400, 196.2784824187679362 ) ) ;
#2606=DIRECTION ( 'NONE',  ( 0.000000000000000000, -9.999999999999953445E-16, 1.000000000000000000 ) ) ;
#2607=CARTESIAN_POINT ( 'NONE',  ( 97.81168569434709070, -40.51740311210409828, 127.6359003399277441 ) ) ;
#2608=CARTESIAN_POINT ( 'NONE',  ( 108.2766895582742848, -26.33922418024667422, 125.9841967044819597 ) ) ;
#2610=ORIENTED_EDGE ( 'NONE', *, *, #83767, .T. ) ;
#2612=AXIS2_PLACEMENT_3D ( 'NONE', #50412, #86290, #24070 ) ;
#2614=DIRECTION ( 'NONE',  ( 0.000000000000000000, 0.000000000000000000, 1.000000000000000000 ) ) ;
#2618=CARTESIAN_POINT ( 'NONE',  ( 116.3259679314843282, -32.93868236591013243, 264.1356252759109680 ) ) ;
#2619=AXIS2_PLACEMENT_3D ( 'NONE', #65973, #78755, #30135 ) ;
#2620=CARTESIAN_POINT ( 'NONE',  ( 107.0664832912739968, 19.62155284005901024, 330.1506252759110680 ) ) ;
#2621=CARTESIAN_POINT ( 'NONE',  ( 96.92686062739846875, -39.15330414739766240, 56.51276813305394597 ) ) ;
#2622=DIRECTION ( 'NONE',  ( 0.7071067811866516006, -0.7071067811864434338, 0.000000000000000000 ) ) ;
#2624=DIRECTION ( 'NONE',  ( -4.237773401492740281E-14, 1.000000000000000000, 0.000000000000000000 ) ) ;
#2626=ADVANCED_FACE ( 'NONE', ( #43089 ), #43987, .F. ) ;
#2627=CARTESIAN_POINT ( 'NONE',  ( 113.0644005321300511, -46.09090919705352718, 68.02991099019695298 ) ) ;
#2628=CARTESIAN_POINT ( 'NONE',  ( 181.8884939055946575, -32.11662333283960180, 237.4678068554150059 ) ) ;
#2629=CARTESIAN_POINT ( 'NONE',  ( 98.00553567079155926, -41.84099229931889852, 132.7356252759109623 ) ) ;
#2632=ORIENTED_EDGE ( 'NONE', *, *, #298, .T. ) ;
#2633=DIRECTION ( 'NONE',  ( 0.000000000000000000, 0.000000000000000000, -1.000000000000000000 ) ) ;
#2635=EDGE_CURVE ( 'NONE', #72873, #48257, #4414, .T. ) ;
#2637=CARTESIAN_POINT ( 'NONE',  ( 25.56670390244797275, -62.87844715994099687, 137.2178068554150059 ) ) ;
#2638=VECTOR ( 'NONE', #4954, 1000.000000000000000 ) ;
#2639=EDGE_CURVE ( 'NONE', #28741, #49561, #9054, .T. ) ;
#2640=DIRECTION ( 'NONE',  ( -1.000000000000000078E-15, 1.000000000000000083E-30, 1.000000000000000000 ) ) ;
#2641=CARTESIAN_POINT ( 'NONE',  ( 99.05215007911658631, -29.93811023049936892, 215.7670538473399517 ) ) ;
#2642=ORIENTED_EDGE ( 'NONE', *, *, #1443, .F. ) ;
#2643=CARTESIAN_POINT ( 'NONE',  ( 33.78309357196258844, -29.99615139349924675, 342.9256252759109884 ) ) ;
#2644=CARTESIAN_POINT ( 'NONE',  ( 96.75123844313058896, -34.86533355485506291, 237.1841967044819626 ) ) ;
#2645=CARTESIAN_POINT ( 'NONE',  ( 96.74875621672018156, -38.50074266403909462, 87.46133956162493917 ) ) ;
#2646=CIRCLE ( 'NONE', #25835, 4.875000000000017764 ) ;
#2647=CARTESIAN_POINT ( 'NONE',  ( 194.0667039024479834, -40.32844715993407902, 300.4678068554149490 ) ) ;
#2649=CARTESIAN_POINT ( 'NONE',  ( 99.09497285450953541, -30.55141387270104048, 191.8022096076827552 ) ) ;
#2650=CARTESIAN_POINT ( 'NONE',  ( 115.7831076721481764, -41.80230950652948252, 78.40645860958801450 ) ) ;
#2651=ORIENTED_EDGE ( 'NONE', *, *, #41288, .F. ) ;
#2652=EDGE_CURVE ( 'NONE', #77917, #64042, #85371, .T. ) ;
#2653=ORIENTED_EDGE ( 'NONE', *, *, #88370, .F. ) ;
#2654=ADVANCED_FACE ( 'NONE', ( #29943 ), #51246, .T. ) ;
#2655=VERTEX_POINT ( 'NONE', #78554 ) ;
#2657=EDGE_LOOP ( 'NONE', ( #68451, #82652, #40751, #53725 ) ) ;
#2659=CARTESIAN_POINT ( 'NONE',  ( 105.3240584539683482, -26.47319898023377149, 11.20991099019697046 ) ) ;
#2661=CARTESIAN_POINT ( 'NONE',  ( 131.3164832912740110, -36.72944715994100306, 3.101481641215535046 ) ) ;
#2662=EDGE_CURVE ( 'NONE', #35967, #46977, #71833, .T. ) ;
#2663=DIRECTION ( 'NONE',  ( 1.000000000000000000, 4.299999999999999979E-14, 1.000000000000000078E-15 ) ) ;
#2665=CARTESIAN_POINT ( 'NONE',  ( 179.8585841295800094, -30.08671355700241179, -5.074374724088000832 ) ) ;
#2666=CARTESIAN_POINT ( 'NONE',  ( 115.0373743241724327, -39.87857374794037923, 192.9495626852199450 ) ) ;
#2667=ORIENTED_EDGE ( 'NONE', *, *, #22230, .F. ) ;
#2670=VERTEX_POINT ( 'NONE', #86691 ) ;
#2671=CARTESIAN_POINT ( 'NONE',  ( 110.8549203045407978, -45.98405385848638360, 182.8856638173630529 ) ) ;
#2672=CARTESIAN_POINT ( 'NONE',  ( 112.1541913332956284, -45.76570811864959154, 253.9965776568629110 ) ) ;
#2673=CARTESIAN_POINT ( 'NONE',  ( 97.81168895331838087, -40.51742574516882200, 287.6356252759109680 ) ) ;
#2675=ORIENTED_EDGE ( 'NONE', *, *, #74928, .F. ) ;
#2676=AXIS2_PLACEMENT_3D ( 'NONE', #78933, #16698, #44380 ) ;
#2681=CARTESIAN_POINT ( 'NONE',  ( 111.5476492967639359, -29.48535330821865941, 286.0672975916113501 ) ) ;
#2682=CIRCLE ( 'NONE', #50511, 2.500000000000002220 ) ;
#2683=AXIS2_PLACEMENT_3D ( 'NONE', #52529, #5317, #32552 ) ;
#2685=CARTESIAN_POINT ( 'NONE',  ( 25.56670390244797275, -58.35344715994099829, 173.2178068554149775 ) ) ;
#2692=CARTESIAN_POINT ( 'NONE',  ( 109.6839073351967642, -47.46854297047285343, 87.75467289495897205 ) ) ;
#2693=EDGE_LOOP ( 'NONE', ( #48499, #38481 ) ) ;
#2694=CARTESIAN_POINT ( 'NONE',  ( 114.9815630121539272, -32.32897180620768296, 28.66480078045796631 ) ) ;
#2695=CIRCLE ( 'NONE', #66468, 2.500000000000002220 ) ;
#2697=CARTESIAN_POINT ( 'NONE',  ( 112.4011824308993397, -28.99526907646757934, 86.03967854399191140 ) ) ;
#2699=CARTESIAN_POINT ( 'NONE',  ( 116.8176351461798816, -34.15490266430645505, 15.03129702300762638 ) ) ;
#2700=CARTESIAN_POINT ( 'NONE',  ( 91.27445496092437338, -35.37506862591278889, 302.6356252759109680 ) ) ;
#2701=CIRCLE ( 'NONE', #7039, 0.5000000000000004441 ) ;
#2703=CARTESIAN_POINT ( 'NONE',  ( 117.5626006132557535, -36.54510529939036445, 284.8413395616253752 ) ) ;
#2705=VERTEX_POINT ( 'NONE', #19426 ) ;
#2706=EDGE_CURVE ( 'NONE', #5970, #80043, #52218, .T. ) ;
#2708=EDGE_LOOP ( 'NONE', ( #58431, #17831, #43894, #14719 ) ) ;
#2709=CARTESIAN_POINT ( 'NONE',  ( 105.7148016331714757, -24.90641244965552659, 156.1670538473399574 ) ) ;
#2710=CARTESIAN_POINT ( 'NONE',  ( 79.69020591994394920, -21.46022584114962939, 1.641799370505243827 ) ) ;
#2711=EDGE_LOOP ( 'NONE', ( #29510, #40676, #50421, #40816 ) ) ;
#2712=ORIENTED_EDGE ( 'NONE', *, *, #40555, .F. ) ;
#2713=EDGE_LOOP ( 'NONE', ( #7717, #89123 ) ) ;
#2715=DIRECTION ( 'NONE',  ( -0.7071067811865192621, -0.7071067811865758834, -7.071067811865186413E-16 ) ) ;
#2717=CARTESIAN_POINT ( 'NONE',  ( 96.12852455334814294, -38.72269610271991525, 201.4699109901969791 ) ) ;
#2718=CARTESIAN_POINT ( 'NONE',  ( 144.8664832912739939, -71.52944715994085811, 361.9756252759100335 ) ) ;
#2719=DIRECTION ( 'NONE',  ( 0.000000000000000000, 1.000000000000000000, 0.000000000000000000 ) ) ;
#2720=DIRECTION ( 'NONE',  ( 1.000000000000000000, 4.299999999999999979E-14, 1.000000000000000078E-15 ) ) ;
#2721=CARTESIAN_POINT ( 'NONE',  ( 117.5407444095047111, -36.54548251031545192, 284.8413395616252615 ) ) ;
#2722=DIRECTION ( 'NONE',  ( 1.000000000000000000, 4.163336342344333240E-14, 0.000000000000000000 ) ) ;
#2723=VERTEX_POINT ( 'NONE', #18524 ) ;
#2724=CARTESIAN_POINT ( 'NONE',  ( 97.79627733347969354, -40.47956530005762232, 172.6323719911590899 ) ) ;
#2726=VECTOR ( 'NONE', #73705, 1000.000000000000000 ) ;
#2728=DIRECTION ( 'NONE',  ( 0.000000000000000000, 0.000000000000000000, 1.000000000000000000 ) ) ;
#2730=CARTESIAN_POINT ( 'NONE',  ( 112.4780167374716058, -46.34085331822173970, 257.9965776568635647 ) ) ;
#2733=PLANE ( 'NONE',  #44835 ) ;
#2734=CARTESIAN_POINT ( 'NONE',  ( 184.5664832912729878, -81.37844715994266664, 361.9756252759109998 ) ) ;
#2735=ADVANCED_FACE ( 'NONE', ( #88485 ), #26242, .F. ) ;
#2736=CARTESIAN_POINT ( 'NONE',  ( 98.89771913768545630, -40.63891803577419637, 216.1162293518859485 ) ) ;
#2738=CARTESIAN_POINT ( 'NONE',  ( 117.4328057974122714, -37.95573561897357706, 49.73276813305393773 ) ) ;
#2740=CARTESIAN_POINT ( 'NONE',  ( 109.0807882705640139, -47.64528240413121551, 127.7337205140059382 ) ) ;
#2741=ORIENTED_EDGE ( 'NONE', *, *, #83393, .F. ) ;
#2746=CARTESIAN_POINT ( 'NONE',  ( 110.2240687061785707, -27.20640067271266460, 275.8215515107314104 ) ) ;
#2747=EDGE_LOOP ( 'NONE', ( #68008, #47012, #36592, #22120 ) ) ;
#2751=ORIENTED_EDGE ( 'NONE', *, *, #56201, .T. ) ;
#2752=PLANE ( 'NONE',  #5918 ) ;
#2753=DIRECTION ( 'NONE',  ( 4.299999999999999979E-14, -1.000000000000000000, 4.400000000000000367E-29 ) ) ;
#2754=AXIS2_PLACEMENT_3D ( 'NONE', #84563, #50902, #49098 ) ;
#2755=LINE ( 'NONE', #78623, #59670 ) ;
#2757=AXIS2_PLACEMENT_3D ( 'NONE', #23707, #65023, #56851 ) ;
#2758=EDGE_CURVE ( 'NONE', #66915, #46344, #79890, .T. ) ;
#2759=CARTESIAN_POINT ( 'NONE',  ( 95.46334413863738177, -34.19939227723602926, 106.1556252759109640 ) ) ;
#2760=CARTESIAN_POINT ( 'NONE',  ( 97.80795155074446257, -40.50828509696400914, 166.6348390368860635 ) ) ;
#2762=CARTESIAN_POINT ( 'NONE',  ( 104.4081006369549982, -46.45808913368724546, 142.3647919406123208 ) ) ;
#2764=EDGE_CURVE ( 'NONE', #51166, #61833, #7332, .T. ) ;
#2770=CIRCLE ( 'NONE', #60767, 2.517500000000005844 ) ;
#2771=DIRECTION ( 'NONE',  ( 1.000000000000000000, 4.163336342344333240E-14, 0.000000000000000000 ) ) ;
#2773=DIRECTION ( 'NONE',  ( 0.000000000000000000, 0.000000000000000000, 1.000000000000000000 ) ) ;
#2774=ORIENTED_EDGE ( 'NONE', *, *, #57742, .T. ) ;
#2775=CARTESIAN_POINT ( 'NONE',  ( 116.3130905035090876, -32.93898513502411163, 35.13562527591096796 ) ) ;
#2776=CARTESIAN_POINT ( 'NONE',  ( 111.1483613326457629, -47.07112276671751516, 168.8756252759109486 ) ) ;
#2778=FACE_OUTER_BOUND ( 'NONE', #78792, .T. ) ;
#2779=ORIENTED_EDGE ( 'NONE', *, *, #75020, .T. ) ;
#2780=CARTESIAN_POINT ( 'NONE',  ( 97.33063402535807995, -33.15845140301009053, 17.03467289495797132 ) ) ;
#2781=DIRECTION ( 'NONE',  ( 0.000000000000000000, 1.000000000000000000, 0.000000000000000000 ) ) ;
#2782=CARTESIAN_POINT ( 'NONE',  ( 101.9935131536830255, -45.44600547682843938, 52.15652309846547752 ) ) ;
#2784=EDGE_LOOP ( 'NONE', ( #26357, #21741, #19433, #87508 ) ) ;
#2786=CARTESIAN_POINT ( 'NONE',  ( 116.7732407090126827, -35.28285290846962141, 218.9441967044829482 ) ) ;
#2787=VERTEX_POINT ( 'NONE', #50598 ) ;
#2789=EDGE_CURVE ( 'NONE', #9116, #25721, #63798, .T. ) ;
#2790=AXIS2_PLACEMENT_3D ( 'NONE', #76630, #62543, #83010 ) ;
#2791=CARTESIAN_POINT ( 'NONE',  ( 117.1060311394199402, -37.55296641157723769, 185.1930118773259437 ) ) ;
#2793=CARTESIAN_POINT ( 'NONE',  ( 107.5258121372104227, -46.79223613538503912, 39.04444044875393871 ) ) ;
#2795=CARTESIAN_POINT ( 'NONE',  ( 31.78666935232998725, -36.02818131005891189, 342.9256252759119548 ) ) ;
#2800=CARTESIAN_POINT ( 'NONE',  ( 101.3060704567421197, -26.40153104436172526, 255.4813395616251626 ) ) ;
#2802=ORIENTED_EDGE ( 'NONE', *, *, #18081, .T. ) ;
#2803=AXIS2_PLACEMENT_3D ( 'NONE', #76364, #49979, #28655 ) ;
#2804=CARTESIAN_POINT ( 'NONE',  ( 33.96670390244744198, -28.27351298637434240, 313.9678068554150059 ) ) ;
#2806=CARTESIAN_POINT ( 'NONE',  ( 188.5667039024483529, -48.82844715993431350, 290.7178068554150059 ) ) ;
#2808=CARTESIAN_POINT ( 'NONE',  ( 109.4546162266722575, -25.87086512622489920, 25.90419670448196143 ) ) ;
#2811=AXIS2_PLACEMENT_3D ( 'NONE', #73164, #46336, #10941 ) ;
#2813=EDGE_CURVE ( 'NONE', #19234, #64957, #57658, .T. ) ;
#2814=CARTESIAN_POINT ( 'NONE',  ( 110.4707641138770668, -47.29393344369797347, 53.83657765686300678 ) ) ;
#2815=CARTESIAN_POINT ( 'NONE',  ( 118.3411383306134468, -33.07924694129162901, 284.0756252759109657 ) ) ;
#2817=VECTOR ( 'NONE', #5606, 1000.000000000000000 ) ;
#2818=DIRECTION ( 'NONE',  ( -1.000000000000000078E-15, 1.000000000000000083E-30, 1.000000000000000000 ) ) ;
#2819=CARTESIAN_POINT ( 'NONE',  ( 97.82709414970555883, -40.55490225695719175, 17.63852738896761707 ) ) ;
#2822=CARTESIAN_POINT ( 'NONE',  ( 107.4866789999374390, -28.54983079893278486, 92.85380465530596439 ) ) ;
#2823=CARTESIAN_POINT ( 'NONE',  ( 108.1840971438632550, -47.11637154254925974, 198.6613395616249989 ) ) ;
#2824=CARTESIAN_POINT ( 'NONE',  ( 51.06670390244899238, -32.29483332968430886, -5.074374724088000832 ) ) ;
#2825=DIRECTION ( 'NONE',  ( 0.000000000000000000, 0.000000000000000000, 1.000000000000000000 ) ) ;
#2826=EDGE_LOOP ( 'NONE', ( #73856, #10535, #25706, #5708 ) ) ;
#2827=VECTOR ( 'NONE', #16599, 1000.000000000000000 ) ;
#2828=CYLINDRICAL_SURFACE ( 'NONE', #17543, 2.116999999999993776 ) ;
#2829=ORIENTED_EDGE ( 'NONE', *, *, #27986, .T. ) ;
#2830=ORIENTED_EDGE ( 'NONE', *, *, #67015, .T. ) ;
#2832=ORIENTED_EDGE ( 'NONE', *, *, #43523, .T. ) ;
#2835=CARTESIAN_POINT ( 'NONE',  ( 102.0670447425352165, -27.97050339635270788, 41.48976872766033352 ) ) ;
#2836=EDGE_CURVE ( 'NONE', #20875, #48555, #1576, .T. ) ;
#2837=VECTOR ( 'NONE', #22180, 1000.000000000000000 ) ;
#2838=CARTESIAN_POINT ( 'NONE',  ( 99.43039265704440766, -41.59799905411310306, 141.1886103042669731 ) ) ;
#2839=CARTESIAN_POINT ( 'NONE',  ( 118.1265197682042327, -36.12032134488166690, 273.8822919425775808 ) ) ;
#2840=ADVANCED_FACE ( 'NONE', ( #82131 ), #47563, .T. ) ;
#2842=ADVANCED_FACE ( 'NONE', ( #63343, #1120 ), #40759, .F. ) ;
#2844=CARTESIAN_POINT ( 'NONE',  ( 104.5600616111754562, -27.04296758930388833, 136.2779522869518303 ) ) ;
#2845=EDGE_CURVE ( 'NONE', #12768, #20192, #22930, .T. ) ;
#2847=DIRECTION ( 'NONE',  ( 1.000000000000000000, 4.510281037539788691E-14, 0.000000000000000000 ) ) ;
#2851=VERTEX_POINT ( 'NONE', #52353 ) ;
#2852=CARTESIAN_POINT ( 'NONE',  ( 96.80868943730629894, -40.84730494075294871, 251.6422919425777138 ) ) ;
#2853=CARTESIAN_POINT ( 'NONE',  ( 117.5312049024071257, -37.01681686833584450, 39.80419670448193159 ) ) ;
#2854=CARTESIAN_POINT ( 'NONE',  ( 113.1782937674814491, -44.75186859554625585, 119.0939586088680500 ) ) ;
#2855=DIRECTION ( 'NONE',  ( -1.000000000000000078E-15, 0.000000000000000000, 1.000000000000000000 ) ) ;
#2856=DIRECTION ( 'NONE',  ( 0.7071067811866377228, -0.7071067811864573116, 0.000000000000000000 ) ) ;
#2857=DIRECTION ( 'NONE',  ( 1.000000000000000000, -3.885780586187990841E-13, 0.000000000000000000 ) ) ;
#2859=CARTESIAN_POINT ( 'NONE',  ( 131.7480217999342926, -38.20859666167535096, 7.273989459506820410 ) ) ;
#2861=EDGE_CURVE ( 'NONE', #38542, #32624, #25126, .T. ) ;
#2862=DIRECTION ( 'NONE',  ( -0.1858654557293184517, 0.9825752044329902901, 0.000000000000000000 ) ) ;
#2863=CARTESIAN_POINT ( 'NONE',  ( 115.7834167274817503, -41.80178756718994748, 163.4063445344124261 ) ) ;
#2864=DIRECTION ( 'NONE',  ( 0.000000000000000000, 1.000000000000000000, 0.000000000000000000 ) ) ;
#2865=AXIS2_PLACEMENT_3D ( 'NONE', #73796, #80184, #86552 ) ;
#2866=CARTESIAN_POINT ( 'NONE',  ( 49.35031423293201414, -29.99615139349890569, 313.9678068554150059 ) ) ;
#2867=CARTESIAN_POINT ( 'NONE',  ( 116.5566381636777322, -42.44192488244189576, 278.3832443235297660 ) ) ;
#2868=CARTESIAN_POINT ( 'NONE',  ( 103.8073934974285066, -26.82688076304711444, 161.3299109901969643 ) ) ;
#2869=CARTESIAN_POINT ( 'NONE',  ( 96.31605362642591217, -41.77429727756310740, 57.67562527591096710 ) ) ;
#2870=PLANE ( 'NONE',  #50830 ) ;
#2871=DIRECTION ( 'NONE',  ( 0.7071067811865758834, -0.7071067811865192621, 7.071067811865766226E-16 ) ) ;
#2872=CARTESIAN_POINT ( 'NONE',  ( 82.80042800423679239, -36.38432671277497832, 3.076561810303515276 ) ) ;
#2873=AXIS2_PLACEMENT_3D ( 'NONE', #63355, #56978, #84719 ) ;
#2876=VERTEX_POINT ( 'NONE', #66452 ) ;
#2877=CARTESIAN_POINT ( 'NONE',  ( 103.6990349130722677, -26.13358598113153164, 51.32133956162493149 ) ) ;
#2878=AXIS2_PLACEMENT_3D ( 'NONE', #86496, #67361, #11063 ) ;
#2879=DIRECTION ( 'NONE',  ( 1.000000000000000078E-15, -1.000000000000000083E-30, -1.000000000000000000 ) ) ;
#2880=VERTEX_POINT ( 'NONE', #73267 ) ;
#2881=CARTESIAN_POINT ( 'NONE',  ( 99.04401119945882215, -42.84118153451598943, 47.84395147023094097 ) ) ;
#2882=CARTESIAN_POINT ( 'NONE',  ( 110.4916936757735186, -26.90617889774112825, 205.8099109901969541 ) ) ;
#2883=CARTESIAN_POINT ( 'NONE',  ( 32.06670390244764945, -33.35206098992742341, 313.9678068554150059 ) ) ;
#2886=CARTESIAN_POINT ( 'NONE',  ( 97.06107109957150669, -37.99641198294513345, 47.42729194408147464 ) ) ;
#2887=CARTESIAN_POINT ( 'NONE',  ( 194.5667039024479834, -48.82844715994099971, 310.9178068554150514 ) ) ;
#2888=CARTESIAN_POINT ( 'NONE',  ( 99.08956738544915765, -42.79550390363951351, 96.84396446119878021 ) ) ;
#2889=AXIS2_PLACEMENT_3D ( 'NONE', #48360, #76095, #49273 ) ;
#2890=CARTESIAN_POINT ( 'NONE',  ( 111.8077268321493563, -46.78591733285071541, 137.9270538473399768 ) ) ;
#2891=EDGE_LOOP ( 'NONE', ( #4565, #87707, #60253, #39963 ) ) ;
#2894=CARTESIAN_POINT ( 'NONE',  ( 115.7982244386701609, -33.26055366603426933, 95.57110711542094350 ) ) ;
#2895=DIRECTION ( 'NONE',  ( 0.000000000000000000, 1.000000000000000000, 0.000000000000000000 ) ) ;
#2896=CARTESIAN_POINT ( 'NONE',  ( 111.8874393434637682, -45.23954810143637673, 208.9870538473389558 ) ) ;
#2898=DIRECTION ( 'NONE',  ( 9.351236661543306751E-17, -3.725950533538267725E-29, -1.000000000000000000 ) ) ;
#2900=EDGE_CURVE ( 'NONE', #30367, #30159, #57865, .T. ) ;
#2901=AXIS2_PLACEMENT_3D ( 'NONE', #33441, #54750, #19371 ) ;
#2906=CARTESIAN_POINT ( 'NONE',  ( 116.6407469026009238, -40.79910830432095281, 168.5070538473399608 ) ) ;
#2907=ORIENTED_EDGE ( 'NONE', *, *, #43181, .F. ) ;
#2908=VERTEX_POINT ( 'NONE', #31048 ) ;
#2911=DIRECTION ( 'NONE',  ( 0.000000000000000000, 1.000000000000000000, 0.000000000000000000 ) ) ;
#2912=CARTESIAN_POINT ( 'NONE',  ( 97.81186694083565669, -40.51786060332464956, 102.6356630628624060 ) ) ;
#2913=CARTESIAN_POINT ( 'NONE',  ( 116.2459175369934172, -38.08366948007849118, 221.5280903695909842 ) ) ;
#2917=CARTESIAN_POINT ( 'NONE',  ( 98.37959078170875671, -29.89446464491232192, 200.8080062282919869 ) ) ;
#2919=VERTEX_POINT ( 'NONE', #2469 ) ;
#2920=VERTEX_POINT ( 'NONE', #45110 ) ;
#2922=AXIS2_PLACEMENT_3D ( 'NONE', #15425, #58514, #9487 ) ;
#2924=DIRECTION ( 'NONE',  ( -0.9963424814100678706, 0.08544974978095865037, 0.000000000000000000 ) ) ;
#2925=CARTESIAN_POINT ( 'NONE',  ( 172.5664832912740110, -36.32844715994070839, 18.92562527591200094 ) ) ;
#2926=CARTESIAN_POINT ( 'NONE',  ( 114.1852310984691883, -41.65497984893937655, 11.17475703625792072 ) ) ;
#2928=CARTESIAN_POINT ( 'NONE',  ( 115.7831074623854590, -41.80230988274058035, 273.4064585755251642 ) ) ;
#2930=CARTESIAN_POINT ( 'NONE',  ( 116.3422999134539566, -39.38573384602094052, 9.635625275910941312 ) ) ;
#2931=CYLINDRICAL_SURFACE ( 'NONE', #70630, 2.500000000000002220 ) ;
#2932=VERTEX_POINT ( 'NONE', #45541 ) ;
#2933=CIRCLE ( 'NONE', #73985, 0.5000000000000004441 ) ;
#2934=ORIENTED_EDGE ( 'NONE', *, *, #46666, .F. ) ;
#2935=CYLINDRICAL_SURFACE ( 'NONE', #19748, 9.999999999999998224 ) ;
#2936=ORIENTED_EDGE ( 'NONE', *, *, #82900, .T. ) ;
#2938=CARTESIAN_POINT ( 'NONE',  ( 110.3949268851355328, -45.15168757608171290, 22.31051506617198754 ) ) ;
#2939=VECTOR ( 'NONE', #80924, 1000.000000000000000 ) ;
#2940=CARTESIAN_POINT ( 'NONE',  ( 103.0412047595748959, -26.40992324271003966, 170.3603871806729444 ) ) ;
#2941=CARTESIAN_POINT ( 'NONE',  ( 103.1828028919049558, -27.07824557232541807, 130.3813395616259925 ) ) ;
#2942=DIRECTION ( 'NONE',  ( -1.000000000000000078E-15, 1.000000000000000083E-30, 1.000000000000000000 ) ) ;
#2943=CARTESIAN_POINT ( 'NONE',  ( 99.14341341762981585, -43.50528616620496791, 31.88991099019594699 ) ) ;
#2944=CARTESIAN_POINT ( 'NONE',  ( 115.3234718241651535, -45.22984455807579707, 264.1899109901965517 ) ) ;
#2946=EDGE_CURVE ( 'NONE', #42715, #65869, #30164, .T. ) ;
#2947=DIRECTION ( 'NONE',  ( 3.360405532702990443E-14, -1.000000000000000000, 0.000000000000000000 ) ) ;
#2950=VERTEX_POINT ( 'NONE', #78782 ) ;
#2952=CARTESIAN_POINT ( 'NONE',  ( 96.69933951777882442, -35.27033920508573317, 181.2156252759109805 ) ) ;
#2954=CARTESIAN_POINT ( 'NONE',  ( 98.00691293156391737, -30.39673331971502179, 160.8289586092449497 ) ) ;
#2955=CARTESIAN_POINT ( 'NONE',  ( 97.80969231062213964, -40.51824920587227297, 266.6357212253427633 ) ) ;
#2959=FACE_OUTER_BOUND ( 'NONE', #48584, .T. ) ;
#2960=CARTESIAN_POINT ( 'NONE',  ( 110.9847977634195928, -46.36662828626490551, 278.8841967044824059 ) ) ;
#2961=CARTESIAN_POINT ( 'NONE',  ( 33.78309357196401663, -29.99615139349950965, 313.9678068554150059 ) ) ;
#2962=FACE_OUTER_BOUND ( 'NONE', #41421, .T. ) ;
#2963=AXIS2_PLACEMENT_3D ( 'NONE', #80579, #60548, #88735 ) ;
#2964=CARTESIAN_POINT ( 'NONE',  ( 109.7212149768267437, -26.99983785526716318, 270.8646645069375722 ) ) ;
#2966=CARTESIAN_POINT ( 'NONE',  ( 32.25690895537100289, -33.54226604285010893, 342.9256252759119548 ) ) ;
#2967=ADVANCED_FACE ( 'NONE', ( #44669 ), #44213, .F. ) ;
#2968=CARTESIAN_POINT ( 'NONE',  ( 98.30753420875569759, -41.72887552247058096, 257.7397919454337512 ) ) ;
#2969=CARTESIAN_POINT ( 'NONE',  ( 104.1015251979861773, -44.20529628163873781, 195.5838068554170661 ) ) ;
#2971=CARTESIAN_POINT ( 'NONE',  ( 83.56670559755343675, -40.03837296219064967, 239.5838068554176914 ) ) ;
#2972=CARTESIAN_POINT ( 'NONE',  ( 117.3133064751534249, -34.51789172102134984, 183.9956252759109532 ) ) ;
#2973=CARTESIAN_POINT ( 'NONE',  ( 112.7598396812348369, -27.95408244994987967, 65.61848241876793963 ) ) ;
#2974=CARTESIAN_POINT ( 'NONE',  ( 117.9939971868874125, -34.78344139941312108, 194.9546728949589749 ) ) ;
#2976=DIRECTION ( 'NONE',  ( 1.000000000000000000, 4.163336342344333240E-14, 0.000000000000000000 ) ) ;
#2977=CONICAL_SURFACE ( 'NONE', #5894, 1.571100913904333041, 1.047197551196591858 ) ;
#2978=CARTESIAN_POINT ( 'NONE',  ( 80.06648329127402519, -46.42944715994105565, 4.925625275910944012 ) ) ;
#2979=CARTESIAN_POINT ( 'NONE',  ( 116.9975143198770269, -38.00265672266952066, 39.72466762246843786 ) ) ;
#2980=DIRECTION ( 'NONE',  ( 1.000000000000000000, 1.261617073437676668E-15, 9.462128050782575008E-16 ) ) ;
#2981=FACE_OUTER_BOUND ( 'NONE', #28946, .T. ) ;
#2983=CARTESIAN_POINT ( 'NONE',  ( 97.12553845659432739, -37.99676787625246988, 66.42808859729984761 ) ) ;
#2984=ORIENTED_EDGE ( 'NONE', *, *, #3400, .F. ) ;
#2986=CARTESIAN_POINT ( 'NONE',  ( 103.1631342820178929, -29.09950819311272951, 119.8752769709339816 ) ) ;
#2987=VECTOR ( 'NONE', #10602, 1000.000000000000000 ) ;
#2989=ORIENTED_EDGE ( 'NONE', *, *, #21081, .F. ) ;
#2990=CARTESIAN_POINT ( 'NONE',  ( 96.66103594285313250, -37.56076609107801545, 97.38991099019594344 ) ) ;
#2991=DIRECTION ( 'NONE',  ( 1.000000000000000078E-15, -1.000000000000000083E-30, -1.000000000000000000 ) ) ;
#2993=CARTESIAN_POINT ( 'NONE',  ( 77.40046754268362861, -18.03188136815523279, 6.871351212842800926 ) ) ;
#2995=CARTESIAN_POINT ( 'NONE',  ( 105.4283229756613309, -27.08692670426131954, 15.20991099019697401 ) ) ;
#2996=ORIENTED_EDGE ( 'NONE', *, *, #11015, .T. ) ;
#2997=ORIENTED_EDGE ( 'NONE', *, *, #62383, .T. ) ;
#2998=VECTOR ( 'NONE', #39579, 1000.000000000000000 ) ;
#3000=CARTESIAN_POINT ( 'NONE',  ( 125.0235919798090833, -56.62589376934764118, -5.074374724088935196 ) ) ;
#3001=DIRECTION ( 'NONE',  ( 1.000000000000000000, 8.673617379883546378E-16, 9.757819552368989676E-16 ) ) ;
#3004=LINE ( 'NONE', #85694, #39287 ) ;
#3005=CARTESIAN_POINT ( 'NONE',  ( 97.79626992864577062, -40.47954699870867756, 52.63196278063107769 ) ) ;
#3008=CARTESIAN_POINT ( 'NONE',  ( 72.06648329127396835, -9.729447159941065237, 14.92562527591093691 ) ) ;
#3010=CARTESIAN_POINT ( 'NONE',  ( 99.14404768239418786, -44.40400490628097430, 41.95086337114900488 ) ) ;
#3015=CARTESIAN_POINT ( 'NONE',  ( 114.5297761857384415, -31.21626383854846765, 107.1509475124489654 ) ) ;
#3018=CARTESIAN_POINT ( 'NONE',  ( 97.78499608817705280, -40.45164102492867642, 96.62997540673826791 ) ) ;
#3026=ORIENTED_EDGE ( 'NONE', *, *, #12789, .T. ) ;
#3029=CARTESIAN_POINT ( 'NONE',  ( 99.82831888057269509, -43.73513634207608902, 188.3701547344689686 ) ) ;
#3030=EDGE_CURVE ( 'NONE', #45213, #82293, #20566, .T. ) ;
#3033=CARTESIAN_POINT ( 'NONE',  ( 96.00479252368074867, -37.29883552165912874, 117.3794347997199594 ) ) ;
#3034=LINE ( 'NONE', #23930, #39994 ) ;
#3035=EDGE_CURVE ( 'NONE', #54987, #56697, #11507, .T. ) ;
#3036=CARTESIAN_POINT ( 'NONE',  ( 104.4076680213851489, -46.45796240592144244, 17.36483092543189244 ) ) ;
#3037=ORIENTED_EDGE ( 'NONE', *, *, #67402, .T. ) ;
#3038=EDGE_CURVE ( 'NONE', #23716, #49134, #19215, .T. ) ;
#3041=ORIENTED_EDGE ( 'NONE', *, *, #54810, .F. ) ;
#3043=CARTESIAN_POINT ( 'NONE',  ( 109.9085748933103162, -45.56225229135190347, 205.6423760838769681 ) ) ;
#3044=CARTESIAN_POINT ( 'NONE',  ( 100.9280588457464489, -46.89575235069233372, 52.14419670448194921 ) ) ;
#3045=ORIENTED_EDGE ( 'NONE', *, *, #2639, .T. ) ;
#3046=CARTESIAN_POINT ( 'NONE',  ( 97.79189512308828114, -32.01662636557816199, 50.95276813305294183 ) ) ;
#3047=CARTESIAN_POINT ( 'NONE',  ( 98.30744901804703773, -41.72866419761319179, 251.7400428627262272 ) ) ;
#3048=CARTESIAN_POINT ( 'NONE',  ( 107.0664832912739968, 19.62155284005901024, 333.4006252759110112 ) ) ;
#3049=DIRECTION ( 'NONE',  ( 1.000000000000000000, 4.012088370409549976E-14, 0.000000000000000000 ) ) ;
#3050=CARTESIAN_POINT ( 'NONE',  ( 116.8065287754011337, -43.47971597432173496, 159.3441967044829539 ) ) ;
#3051=EDGE_CURVE ( 'NONE', #58818, #51146, #39200, .T. ) ;
#3054=CARTESIAN_POINT ( 'NONE',  ( 184.3595971212631071, -48.62134037874749026, 129.9678068554150059 ) ) ;
#3055=CIRCLE ( 'NONE', #46533, 5.599999999999994316 ) ;
#3057=DIRECTION ( 'NONE',  ( 4.299999999999999979E-14, -1.000000000000000000, 4.400000000000000367E-29 ) ) ;
#3062=CARTESIAN_POINT ( 'NONE',  ( 98.72235591169328472, -42.97945265871884857, 66.83848241876793850 ) ) ;
#3065=DIRECTION ( 'NONE',  ( 0.000000000000000000, 0.000000000000000000, -1.000000000000000000 ) ) ;
#3066=CARTESIAN_POINT ( 'NONE',  ( 98.34688518126456813, -32.29864090244028318, 50.95276813305393659 ) ) ;
#3068=CARTESIAN_POINT ( 'NONE',  ( 114.1099639442525699, -29.07320488188167218, 195.4841967044819739 ) ) ;
#3069=CARTESIAN_POINT ( 'NONE',  ( 99.09461421399829817, -30.55189217855991757, 60.80243564339674833 ) ) ;
#3071=ORIENTED_EDGE ( 'NONE', *, *, #17294, .F. ) ;
#3073=CARTESIAN_POINT ( 'NONE',  ( 134.0664832912739826, -36.72944715994100306, 14.92562527591099908 ) ) ;
#3074=EDGE_CURVE ( 'NONE', #25046, #85174, #31586, .T. ) ;
#3076=EDGE_CURVE ( 'NONE', #39961, #13820, #74179, .T. ) ;
#3080=DIRECTION ( 'NONE',  ( 0.000000000000000000, 1.000000000000000000, 0.000000000000000000 ) ) ;
#3081=CARTESIAN_POINT ( 'NONE',  ( 117.9786848761844453, -34.69554937534774552, 203.9851490854349549 ) ) ;
#3083=CARTESIAN_POINT ( 'NONE',  ( 105.7993243576699740, -26.72405701148164425, 145.1773073154230929 ) ) ;
#3084=CARTESIAN_POINT ( 'NONE',  ( 118.1046235831494755, -32.34975429571041161, 245.1270538473389706 ) ) ;
#3085=CARTESIAN_POINT ( 'NONE',  ( 108.0381942455320967, -25.67262681319542494, 105.9946728949589811 ) ) ;
#3086=EDGE_CURVE ( 'NONE', #59810, #59306, #11959, .T. ) ;
#3087=CARTESIAN_POINT ( 'NONE',  ( 97.33812840985710579, -34.06989766951477350, 252.1185538372223789 ) ) ;
#3090=CARTESIAN_POINT ( 'NONE',  ( 113.1776118851075523, -44.75237816312386485, 264.0940798895346688 ) ) ;
#3091=VERTEX_POINT ( 'NONE', #53698 ) ;
#3092=ORIENTED_EDGE ( 'NONE', *, *, #87930, .T. ) ;
#3093=VERTEX_POINT ( 'NONE', #81465 ) ;
#3094=CIRCLE ( 'NONE', #14702, 2.117000000000000881 ) ;
#3095=ORIENTED_EDGE ( 'NONE', *, *, #80064, .T. ) ;
#3096=CARTESIAN_POINT ( 'NONE',  ( 116.3212776292269837, -32.94146857470673240, 74.13562527591093954 ) ) ;
#3097=CARTESIAN_POINT ( 'NONE',  ( 106.2269110120561635, -47.75074920971118075, 263.5280062282920994 ) ) ;
#3103=AXIS2_PLACEMENT_3D ( 'NONE', #79956, #38152, #4076 ) ;
#3104=CARTESIAN_POINT ( 'NONE',  ( 115.3915529780678781, -40.29397869100746021, 212.9390864947429804 ) ) ;
#3106=ORIENTED_EDGE ( 'NONE', *, *, #1441, .F. ) ;
#3107=VERTEX_POINT ( 'NONE', #74619 ) ;
#3108=AXIS2_PLACEMENT_3D ( 'NONE', #72090, #44361, #64381 ) ;
#3109=FACE_BOUND ( 'NONE', #78919, .T. ) ;
#3110=CARTESIAN_POINT ( 'NONE',  ( 98.38056673804321406, -41.69552625526764444, 181.7398107738224553 ) ) ;
#3111=CARTESIAN_POINT ( 'NONE',  ( 105.2300248619054344, -26.52326248388681051, 271.2061014663865990 ) ) ;
#3112=DIRECTION ( 'NONE',  ( 1.000000000000000078E-15, -1.000000000000000083E-30, -1.000000000000000000 ) ) ;
#3113=DIRECTION ( 'NONE',  ( -1.000000000000000078E-15, 1.000000000000000000, 0.000000000000000000 ) ) ;
#3114=CARTESIAN_POINT ( 'NONE',  ( 141.0667039024479834, -50.82844715994100682, 310.9178068554150514 ) ) ;
#3115=VECTOR ( 'NONE', #25222, 1000.000000000000000 ) ;
#3116=ORIENTED_EDGE ( 'NONE', *, *, #65169, .T. ) ;
#3117=CARTESIAN_POINT ( 'NONE',  ( 97.33759702722761631, -34.07205617727079527, 57.11479585955967764 ) ) ;
#3120=CARTESIAN_POINT ( 'NONE',  ( 110.1825742734413609, -44.80353631977761353, 15.67570941721097100 ) ) ;
#3121=AXIS2_PLACEMENT_3D ( 'NONE', #15266, #48855, #55656 ) ;
#3122=DIRECTION ( 'NONE',  ( 1.000000000000000078E-15, 0.000000000000000000, -1.000000000000000000 ) ) ;
#3124=EDGE_CURVE ( 'NONE', #26617, #74993, #5594, .T. ) ;
#3125=DIRECTION ( 'NONE',  ( 4.299999999999999979E-14, -1.000000000000000000, 4.400000000000000367E-29 ) ) ;
#3127=CARTESIAN_POINT ( 'NONE',  ( 31.90335556477812773, -33.89581943344378345, 342.9256252759109884 ) ) ;
#3129=FACE_OUTER_BOUND ( 'NONE', #76203, .T. ) ;
#3130=EDGE_CURVE ( 'NONE', #73516, #22726, #80355, .T. ) ;
#3131=CARTESIAN_POINT ( 'NONE',  ( 107.0664832912750057, -36.72944715993903486, 3.024967495036150922 ) ) ;
#3132=ORIENTED_EDGE ( 'NONE', *, *, #63384, .F. ) ;
#3133=CARTESIAN_POINT ( 'NONE',  ( 97.28826076399516865, -33.11373220042904109, 66.04419670448297097 ) ) ;
#3134=ORIENTED_EDGE ( 'NONE', *, *, #36753, .F. ) ;
#3135=CARTESIAN_POINT ( 'NONE',  ( 112.8214380862813755, -44.54936551000075440, 32.50384839950498872 ) ) ;
#3137=EDGE_CURVE ( 'NONE', #87926, #55506, #28713, .T. ) ;
#3138=PLANE ( 'NONE',  #51795 ) ;
#3139=CARTESIAN_POINT ( 'NONE',  ( 97.72568451978753501, -37.74236564027221874, 77.83205949637394383 ) ) ;
#3141=ADVANCED_FACE ( 'NONE', ( #63232 ), #49129, .F. ) ;
#3144=CARTESIAN_POINT ( 'NONE',  ( 116.4070807376042609, -31.97209126034463011, 40.20133956162496958 ) ) ;
#3147=ORIENTED_EDGE ( 'NONE', *, *, #23047, .F. ) ;
#3148=DIRECTION ( 'NONE',  ( 0.000000000000000000, 0.000000000000000000, 1.000000000000000000 ) ) ;
#3150=CARTESIAN_POINT ( 'NONE',  ( 111.8139374584311554, -25.81739915606283375, 130.7499109901969518 ) ) ;
#3151=CARTESIAN_POINT ( 'NONE',  ( 79.00802158143517318, -21.26771232012923463, 1.799893082726899740 ) ) ;
#3153=ORIENTED_EDGE ( 'NONE', *, *, #55507, .T. ) ;
#3154=ADVANCED_FACE ( 'NONE', ( #14648 ), #84594, .T. ) ;
#3155=AXIS2_PLACEMENT_3D ( 'NONE', #31336, #37271, #57706 ) ;
#3158=CARTESIAN_POINT ( 'NONE',  ( 109.1965444620390571, -27.18343884754219886, 224.9013395616259459 ) ) ;
#3159=CARTESIAN_POINT ( 'NONE',  ( 172.5664832912740110, -9.303447159940999356, 138.9256252759119832 ) ) ;
#3160=CARTESIAN_POINT ( 'NONE',  ( 130.3998166246070127, 12.92155284005802685, 349.2756252759110680 ) ) ;
#3161=CARTESIAN_POINT ( 'NONE',  ( 97.81170999498195329, -40.51745678363457159, 187.6351607544849287 ) ) ;
#3162=CARTESIAN_POINT ( 'NONE',  ( 97.28846512631339749, -33.11380776793520653, 62.04419670448196911 ) ) ;
#3164=CARTESIAN_POINT ( 'NONE',  ( 98.04129921502178036, -41.04139788470866534, 42.68115173508382298 ) ) ;
#3165=ORIENTED_EDGE ( 'NONE', *, *, #82118, .T. ) ;
#3166=CARTESIAN_POINT ( 'NONE',  ( 105.0192423035563678, -26.92869720746245576, 171.2403743890392320 ) ) ;
#3170=ORIENTED_EDGE ( 'NONE', *, *, #16091, .F. ) ;
#3172=DIRECTION ( 'NONE',  ( 0.7071067811865784369, -0.7071067811865165975, 7.071067811865791864E-16 ) ) ;
#3174=CARTESIAN_POINT ( 'NONE',  ( 104.3301552612371381, -26.04411461992200927, 245.2880062282919482 ) ) ;
#3177=DIRECTION ( 'NONE',  ( -0.04216478779797398074, 0.9991106698809455455, 0.000000000000000000 ) ) ;
#3178=CARTESIAN_POINT ( 'NONE',  ( 100.3258375188005402, -30.68160747159130963, 235.1790864947439559 ) ) ;
#3179=DIRECTION ( 'NONE',  ( -1.000000000000000000, -4.299999999999999979E-14, -1.000000000000000078E-15 ) ) ;
#3180=CARTESIAN_POINT ( 'NONE',  ( 103.9639062230919251, -47.31423993612432355, 58.33753003781600199 ) ) ;
#3182=CARTESIAN_POINT ( 'NONE',  ( 102.6790914627476070, -46.92570513279398625, 137.2651490854349561 ) ) ;
#3184=CARTESIAN_POINT ( 'NONE',  ( 179.7974245136200011, -36.32844715994040996, 342.9256252759119548 ) ) ;
#3185=ORIENTED_EDGE ( 'NONE', *, *, #57679, .F. ) ;
#3187=FACE_OUTER_BOUND ( 'NONE', #7952, .T. ) ;
#3188=CARTESIAN_POINT ( 'NONE',  ( 115.8332703014196312, -31.75044964869108810, 275.2380515835822052 ) ) ;
#3195=EDGE_CURVE ( 'NONE', #66655, #15446, #15088, .T. ) ;
#3196=DIRECTION ( 'NONE',  ( 0.000000000000000000, 0.000000000000000000, 1.000000000000000000 ) ) ;
#3198=CARTESIAN_POINT ( 'NONE',  ( 141.0667039024479834, -48.82844715994099971, 250.9178068554160461 ) ) ;
#3199=ORIENTED_EDGE ( 'NONE', *, *, #89002, .T. ) ;
#3200=VECTOR ( 'NONE', #39348, 1000.000000000000114 ) ;
#3201=CARTESIAN_POINT ( 'NONE',  ( 101.6994268497411724, -27.72483345503921370, 85.50419670448295051 ) ) ;
#3203=CARTESIAN_POINT ( 'NONE',  ( 97.78490694950903617, -40.45141876997547570, 166.6299563115132116 ) ) ;
#3205=CARTESIAN_POINT ( 'NONE',  ( 105.7154773070653704, -46.72385838926080481, 142.4689586073946543 ) ) ;
#3206=ORIENTED_EDGE ( 'NONE', *, *, #39653, .T. ) ;
#3211=CARTESIAN_POINT ( 'NONE',  ( 71.06648329127399677, -8.729447159940999512, -5.074374724088000832 ) ) ;
#3213=CARTESIAN_POINT ( 'NONE',  ( 117.1057691840046147, -37.46862480412959684, 249.7680016665607354 ) ) ;
#3214=PLANE ( 'NONE',  #31191 ) ;
#3217=EDGE_LOOP ( 'NONE', ( #66937, #30175 ) ) ;
#3218=LINE ( 'NONE', #45850, #54897 ) ;
#3219=CARTESIAN_POINT ( 'NONE',  ( 112.1511370651176662, -26.84216853020821958, 165.6984824187679521 ) ) ;
#3220=CARTESIAN_POINT ( 'NONE',  ( 144.4409906766500455, -0.9165124547899898833, 540.9756252759101471 ) ) ;
#3221=EDGE_LOOP ( 'NONE', ( #56278, #7392, #79586 ) ) ;
#3222=CARTESIAN_POINT ( 'NONE',  ( 116.2977993645975232, -41.52656014244012539, 284.4441967044824082 ) ) ;
#3223=CARTESIAN_POINT ( 'NONE',  ( 79.56670390244796920, -50.82844715994100682, 104.9178068554150087 ) ) ;
#3224=CARTESIAN_POINT ( 'NONE',  ( 98.54782847511336286, -41.97726656945443580, 51.76585797866146521 ) ) ;
#3225=FACE_BOUND ( 'NONE', #50152, .T. ) ;
#3227=CARTESIAN_POINT ( 'NONE',  ( 102.0677619940791914, -27.97008352907843687, 30.48995469929853286 ) ) ;
#3228=ORIENTED_EDGE ( 'NONE', *, *, #59103, .F. ) ;
#3229=VECTOR ( 'NONE', #9904, 1000.000000000000000 ) ;
#3231=EDGE_CURVE ( 'NONE', #61365, #36567, #8275, .T. ) ;
#3232=CARTESIAN_POINT ( 'NONE',  ( 109.9841060568515729, -28.36190534590500434, 206.2415833058969667 ) ) ;
#3233=VECTOR ( 'NONE', #6596, 1000.000000000000000 ) ;
#3234=DIRECTION ( 'NONE',  ( -1.000000000000000000, 1.011922027653136551E-15, 0.000000000000000000 ) ) ;
#3235=CARTESIAN_POINT ( 'NONE',  ( 99.19755098026091389, -30.44051964901187191, 42.22158330589692810 ) ) ;
#3237=EDGE_CURVE ( 'NONE', #33634, #13721, #35974, .T. ) ;
#3238=ADVANCED_FACE ( 'NONE', ( #41867 ), #15543, .F. ) ;
#3239=CARTESIAN_POINT ( 'NONE',  ( 108.4174892568073005, -26.73503592836434706, 79.96895860887276797 ) ) ;
#3240=CYLINDRICAL_SURFACE ( 'NONE', #58938, 9.999999999999998224 ) ;
#3241=ORIENTED_EDGE ( 'NONE', *, *, #60322, .F. ) ;
#3243=ADVANCED_FACE ( 'NONE', ( #79113 ), #10501, .F. ) ;
#3245=VERTEX_POINT ( 'NONE', #2806 ) ;
#3246=CARTESIAN_POINT ( 'NONE',  ( 117.4695305279094981, -36.80206755349689729, 263.8213395616251660 ) ) ;
#3248=VERTEX_POINT ( 'NONE', #3687 ) ;
#3251=CARTESIAN_POINT ( 'NONE',  ( 116.8171228667533796, -34.15291832118845150, 84.03145860919784127 ) ) ;
#3255=CARTESIAN_POINT ( 'NONE',  ( 96.60079736239889314, -36.47965167166085365, 192.3070538473399438 ) ) ;
#3258=EDGE_LOOP ( 'NONE', ( #10676, #48610 ) ) ;
#3259=CIRCLE ( 'NONE', #74314, 3.000000000000002665 ) ;
#3260=CARTESIAN_POINT ( 'NONE',  ( 112.9878179797879909, -28.09632633057573159, 40.59848241876795782 ) ) ;
#3261=DIRECTION ( 'NONE',  ( 2.900000000000000265E-14, -2.000000000000000155E-15, 1.000000000000000000 ) ) ;
#3262=CARTESIAN_POINT ( 'NONE',  ( 111.7391504816189212, -27.40993963462091543, 279.7070538473396937 ) ) ;
#3264=ADVANCED_FACE ( 'NONE', ( #51813 ), #9609, .T. ) ;
#3267=CARTESIAN_POINT ( 'NONE',  ( 105.7160904893042783, -46.72395770272043336, 18.46948113466270769 ) ) ;
#3268=DIRECTION ( 'NONE',  ( 0.000000000000000000, 0.000000000000000000, 1.000000000000000000 ) ) ;
#3269=CARTESIAN_POINT ( 'NONE',  ( 114.8246268090051245, -34.19154740317726038, 86.89666179816296676 ) ) ;
#3270=CARTESIAN_POINT ( 'NONE',  ( 98.24294948823698803, -42.32252413779357170, 182.7756252759109543 ) ) ;
#3272=ORIENTED_EDGE ( 'NONE', *, *, #5036, .F. ) ;
#3275=ORIENTED_EDGE ( 'NONE', *, *, #16027, .F. ) ;
#3277=( BOUNDED_CURVE ( )  B_SPLINE_CURVE ( 3, ( #1908, #7374, #21913, #28711 ),
 .UNSPECIFIED., .F., .T. ) 
 B_SPLINE_CURVE_WITH_KNOTS ( ( 4, 4 ),
 ( 1.506129919829842123, 1.572423208257343274 ),
 .UNSPECIFIED. ) 
 CURVE ( )  GEOMETRIC_REPRESENTATION_ITEM ( )  RATIONAL_B_SPLINE_CURVE ( ( 1.000000000000000000, 0.9996338001896092340, 0.9996338001896092340, 1.000000000000000000 ) ) 
 REPRESENTATION_ITEM ( '' )  );
#3278=ORIENTED_EDGE ( 'NONE', *, *, #8194, .F. ) ;
#3280=CARTESIAN_POINT ( 'NONE',  ( 112.0675020739599006, -45.48750542127923779, 168.9906668250784776 ) ) ;
#3281=CARTESIAN_POINT ( 'NONE',  ( 99.09569553996823288, -30.55044851293582653, 41.80222573704838851 ) ) ;
#3282=CARTESIAN_POINT ( 'NONE',  ( 98.01892258562502036, -37.12227740767932715, 115.7714674471239675 ) ) ;
#3283=B_SPLINE_CURVE_WITH_KNOTS ( 'NONE', 3,
 ( #20790, #13973, #42112, #69838, #69391 ),
 .UNSPECIFIED., .F., .F.,
 ( 4, 1, 4 ),
 ( 0.000000000000000000, 0.5713596581863561452, 1.000000000000000000 ),
 .UNSPECIFIED. ) ;
#3284=CARTESIAN_POINT ( 'NONE',  ( 105.4140021367065003, -47.06753073853725056, 37.44991099019695469 ) ) ;
#3285=VECTOR ( 'NONE', #50335, 1000.000000000000000 ) ;
#3287=ORIENTED_EDGE ( 'NONE', *, *, #64697, .T. ) ;
#3288=CARTESIAN_POINT ( 'NONE',  ( 103.2790154487345688, -27.47444377515469682, 136.3855822504286266 ) ) ;
#3290=CARTESIAN_POINT ( 'NONE',  ( 80.06648329127401098, -41.22944715994105280, 4.925625275910944012 ) ) ;
#3291=CARTESIAN_POINT ( 'NONE',  ( 117.0605793477646444, -38.08267519577708526, 33.71899569443299782 ) ) ;
#3292=ADVANCED_FACE ( 'NONE', ( #87259 ), #30504, .F. ) ;
#3293=DIRECTION ( 'NONE',  ( -1.000000000000000000, -3.999999999999999995E-14, -1.000000000000000078E-15 ) ) ;
#3294=VECTOR ( 'NONE', #20015, 1000.000000000000000 ) ;
#3297=CARTESIAN_POINT ( 'NONE',  ( 115.6554515427140473, -30.75822225795367970, 279.3099109901966131 ) ) ;
#3298=CARTESIAN_POINT ( 'NONE',  ( 104.2291421067619694, -46.80627582718438617, 18.35848241876792031 ) ) ;
#3300=CARTESIAN_POINT ( 'NONE',  ( 90.44969454456415292, -53.34645651782494724, 229.5838068554169809 ) ) ;
#3301=CARTESIAN_POINT ( 'NONE',  ( 76.24325998657069192, -5.906223855237660914, -5.074374724089060429 ) ) ;
#3302=DIRECTION ( 'NONE',  ( 0.000000000000000000, 0.000000000000000000, -1.000000000000000000 ) ) ;
#3304=CARTESIAN_POINT ( 'NONE',  ( 83.06670390244796920, -67.87844715994100397, 201.9838068554149970 ) ) ;
#3305=CARTESIAN_POINT ( 'NONE',  ( 51.06670390244799762, -33.35206098992630075, 342.9256252759119548 ) ) ;
#3306=FACE_OUTER_BOUND ( 'NONE', #82321, .T. ) ;
#3307=CARTESIAN_POINT ( 'NONE',  ( 99.04410099017079006, -42.84131659189329611, 161.8437698291777735 ) ) ;
#3308=AXIS2_PLACEMENT_3D ( 'NONE', #22031, #8389, #659 ) ;
#3309=DIRECTION ( 'NONE',  ( 1.000000000000000078E-15, -1.000000000000000083E-30, -1.000000000000000000 ) ) ;
#3310=CARTESIAN_POINT ( 'NONE',  ( 111.7836659179374408, -46.75466717335095268, 287.9146728949587555 ) ) ;
#3311=CARTESIAN_POINT ( 'NONE',  ( 109.3584748782654401, -25.91645705315499981, 180.9222919425779708 ) ) ;
#3312=CARTESIAN_POINT ( 'NONE',  ( 106.6058858729755201, -25.66269263286424263, 36.09753003781596448 ) ) ;
#3314=PLANE ( 'NONE',  #39955 ) ;
#3315=CARTESIAN_POINT ( 'NONE',  ( 81.97596355239819843, -34.74831825238398864, 2.232988539021949492 ) ) ;
#3316=AXIS2_PLACEMENT_3D ( 'NONE', #89644, #6080, #54627 ) ;
#3317=EDGE_CURVE ( 'NONE', #45463, #28588, #11335, .T. ) ;
#3318=ORIENTED_EDGE ( 'NONE', *, *, #88036, .T. ) ;
#3319=FACE_OUTER_BOUND ( 'NONE', #48560, .T. ) ;
#3321=AXIS2_PLACEMENT_3D ( 'NONE', #11100, #2524, #79282 ) ;
#3322=CARTESIAN_POINT ( 'NONE',  ( 114.7602587138392209, -43.68247563549507362, 79.25372051400597684 ) ) ;
#3324=VERTEX_POINT ( 'NONE', #9172 ) ;
#3326=CARTESIAN_POINT ( 'NONE',  ( 101.4371718687638406, -46.21494532752021200, 203.1622919425779514 ) ) ;
#3328=CARTESIAN_POINT ( 'NONE',  ( 105.7153080974451882, -46.72383283222870887, 147.4690131811856872 ) ) ;
#3329=DIRECTION ( 'NONE',  ( 0.000000000000000000, -1.000000000000000000, 0.000000000000000000 ) ) ;
#3330=DIRECTION ( 'NONE',  ( -6.831565154159360295E-14, 1.000000000000000000, 0.000000000000000000 ) ) ;
#3333=CARTESIAN_POINT ( 'NONE',  ( 111.3489484856832235, -45.76813167571804541, 97.92856849314694045 ) ) ;
#3334=CARTESIAN_POINT ( 'NONE',  ( 108.9483104351207317, -46.92736419409159510, 127.7337205140069472 ) ) ;
#3335=ORIENTED_EDGE ( 'NONE', *, *, #973, .T. ) ;
#3336=VERTEX_POINT ( 'NONE', #37770 ) ;
#3337=CARTESIAN_POINT ( 'NONE',  ( 107.2073525216087120, -27.33494443775582639, 76.50824997256394511 ) ) ;
#3338=CARTESIAN_POINT ( 'NONE',  ( 31.56670390244800828, -32.29483332968611364, -5.074374724088000832 ) ) ;
#3339=CARTESIAN_POINT ( 'NONE',  ( 101.2091419812965256, -45.28691980162477648, 238.1108633711489517 ) ) ;
#3340=DIRECTION ( 'NONE',  ( 0.000000000000000000, 0.000000000000000000, -1.000000000000000000 ) ) ;
#3341=CARTESIAN_POINT ( 'NONE',  ( 25.56670390244797275, -62.87844715994099687, 293.2178068554150627 ) ) ;
#3342=CARTESIAN_POINT ( 'NONE',  ( 179.4595971212889935, -28.98061976758940617, -5.074374724088000832 ) ) ;
#3343=B_SPLINE_CURVE_WITH_KNOTS ( 'NONE', 3,
 ( #16058, #84658, #1077, #27878, #76937, #8804, #50100, #15158, #35131, #56469, #71476, #50554, #64206, #14266, #84217, #55553, #42834, #28789, #618, #21987, #9238, #49203, #21073, #43286, #70571, #7443, #41939, #14715, #48749, #57368, #63300, #8345, #1536, #62842, #28315, #77836, #85109 ),
 .UNSPECIFIED., .F., .F.,
 ( 4, 2, 2, 1, 2, 2, 2, 1, 1, 2, 2, 2, 2, 1, 2, 2, 2, 1, 1, 1, 2, 4 ),
 ( 0.6666501603264138875, 0.6874845253060100081, 0.6926931165509091493, 0.6979017077958082904, 0.7083188902856059066, 0.7499876202447992579, 0.7525919158672497167, 0.7551962114897000644, 0.7604048027346009819, 0.7708219852244027059, 0.7916563502040085964, 0.8124907151836144870, 0.8176993064285161816, 0.8229078976734178763, 0.8333250801632203775, 0.8749938101224256082, 0.8775981057448752898, 0.8802024013673249714, 0.8854109926122243346, 0.8958281751020222838, 0.9166625400816181823, 1.000000000000000000 ),
 .UNSPECIFIED. ) ;
#3344=ADVANCED_FACE ( 'NONE', ( #86813 ), #10940, .F. ) ;
#3346=DIRECTION ( 'NONE',  ( -1.387778780781444413E-14, -1.000000000000000000, 0.000000000000000000 ) ) ;
#3349=ADVANCED_FACE ( 'NONE', ( #72732, #43672 ), #85936, .F. ) ;
#3351=CARTESIAN_POINT ( 'NONE',  ( 102.0922439024870982, -27.59239485085791088, 145.4727681330539610 ) ) ;
#3357=CARTESIAN_POINT ( 'NONE',  ( 97.33784134183721903, -34.07106442030320892, 152.1147919335942333 ) ) ;
#3359=CARTESIAN_POINT ( 'NONE',  ( 97.86644802266228282, -40.64892155565895848, 102.6469608634411372 ) ) ;
#3361=CARTESIAN_POINT ( 'NONE',  ( 108.3334346252740517, -46.73486118540429857, 268.6772908713167567 ) ) ;
#3362=CARTESIAN_POINT ( 'NONE',  ( 102.9670468844020235, -26.46427747797763175, 175.3908633711489813 ) ) ;
#3363=CYLINDRICAL_SURFACE ( 'NONE', #34239, 9.999999999999998224 ) ;
#3364=ORIENTED_EDGE ( 'NONE', *, *, #17294, .T. ) ;
#3365=ORIENTED_EDGE ( 'NONE', *, *, #29121, .T. ) ;
#3368=CARTESIAN_POINT ( 'NONE',  ( 97.90457037977253663, -40.73788048421130981, 62.65513217813478519 ) ) ;
#3369=DIRECTION ( 'NONE',  ( 0.000000000000000000, 1.000000000000000000, 0.000000000000000000 ) ) ;
#3371=CARTESIAN_POINT ( 'NONE',  ( 114.0851551000824600, -43.95502333027237540, 264.6215833058971043 ) ) ;
#3372=LINE ( 'NONE', #66469, #46346 ) ;
#3373=ORIENTED_EDGE ( 'NONE', *, *, #13817, .T. ) ;
#3374=CARTESIAN_POINT ( 'NONE',  ( 110.3061846121042464, -44.54875278746831668, 9.635625275910943088 ) ) ;
#3375=CARTESIAN_POINT ( 'NONE',  ( 163.0664832912739826, -0.7548456658610993575, 333.4006252759120343 ) ) ;
#3377=VERTEX_POINT ( 'NONE', #50938 ) ;
#3378=VECTOR ( 'NONE', #53973, 1000.000000000000000 ) ;
#3379=CARTESIAN_POINT ( 'NONE',  ( 116.5693234920293406, -33.54757666135687089, 114.0835099680320468 ) ) ;
#3380=ORIENTED_EDGE ( 'NONE', *, *, #47014, .T. ) ;
#3382=FACE_OUTER_BOUND ( 'NONE', #82012, .T. ) ;
#3383=VECTOR ( 'NONE', #82830, 1000.000000000000000 ) ;
#3384=CARTESIAN_POINT ( 'NONE',  ( 105.7183000297088284, -45.16381338481517815, 36.87241982807598362 ) ) ;
#3385=CARTESIAN_POINT ( 'NONE',  ( 96.16820482414080118, -32.01123326506838396, 211.0013395616249738 ) ) ;
#3386=CARTESIAN_POINT ( 'NONE',  ( 95.33621695423326514, -38.27597901479985865, 151.4299109901969871 ) ) ;
#3388=CARTESIAN_POINT ( 'NONE',  ( 105.1090458072749527, -25.85091697680629608, 271.2061014663872243 ) ) ;
#3389=CARTESIAN_POINT ( 'NONE',  ( 141.8664832912729992, -71.52944715994142655, 352.4506252759077825 ) ) ;
#3392=VERTEX_POINT ( 'NONE', #17764 ) ;
#3394=CARTESIAN_POINT ( 'NONE',  ( 115.0114139542580318, -28.97761122332106964, 194.4537205140059370 ) ) ;
#3395=VERTEX_POINT ( 'NONE', #59523 ) ;
#3396=CARTESIAN_POINT ( 'NONE',  ( 95.90979441981569664, -32.73335165780250122, 176.0527681330539735 ) ) ;
#3397=CARTESIAN_POINT ( 'NONE',  ( 116.3259679314843282, -32.93868236591013243, 264.1356252759109680 ) ) ;
#3400=EDGE_CURVE ( 'NONE', #19567, #38055, #1235, .T. ) ;
#3402=CARTESIAN_POINT ( 'NONE',  ( 32.09598329127712901, -23.42844715994121785, 237.4678068554150059 ) ) ;
#3403=LINE ( 'NONE', #58358, #84123 ) ;
#3405=CARTESIAN_POINT ( 'NONE',  ( 100.1919508713739759, -45.35525880799009713, 268.0289586092443415 ) ) ;
#3406=CARTESIAN_POINT ( 'NONE',  ( 71.25529199314600248, -79.12815651470191369, 394.9756252759101471 ) ) ;
#3407=DIRECTION ( 'NONE',  ( 0.000000000000000000, 0.000000000000000000, -1.000000000000000000 ) ) ;
#3409=CARTESIAN_POINT ( 'NONE',  ( 97.07198150990221563, -35.37932431885204210, 272.2185945074161282 ) ) ;
#3410=VECTOR ( 'NONE', #78654, 1000.000000000000000 ) ;
#3413=CARTESIAN_POINT ( 'NONE',  ( 97.81169182074827972, -40.51741433969252881, 77.63574375254798099 ) ) ;
#3414=CARTESIAN_POINT ( 'NONE',  ( 114.5003034259403876, -40.32092683139836709, 195.5838068554168103 ) ) ;
#3415=ORIENTED_EDGE ( 'NONE', *, *, #59729, .T. ) ;
#3416=CARTESIAN_POINT ( 'NONE',  ( 136.4532669483820086, -20.09809895853697626, 7.205238605735853952 ) ) ;
#3417=CARTESIAN_POINT ( 'NONE',  ( 113.1683672335202431, -26.54116819535108363, 204.6470538473399756 ) ) ;
#3418=CARTESIAN_POINT ( 'NONE',  ( 110.4565933333529699, -47.24995733706104062, 53.83657765686300678 ) ) ;
#3419=CARTESIAN_POINT ( 'NONE',  ( 110.2692182064865420, -26.72542277727598403, 230.8299109901969643 ) ) ;
#3420=CARTESIAN_POINT ( 'NONE',  ( 71.06648329127399677, -18.82844715994099971, -5.074374724088000832 ) ) ;
#3421=FACE_OUTER_BOUND ( 'NONE', #44834, .T. ) ;
#3422=CARTESIAN_POINT ( 'NONE',  ( 37.06648329127400388, 12.92155284005802685, 335.5992267699910485 ) ) ;
#3423=CARTESIAN_POINT ( 'NONE',  ( 99.03269296098446262, -42.71672268585848542, 37.83590083622135580 ) ) ;
#3425=DIRECTION ( 'NONE',  ( 1.000000000000000000, 0.000000000000000000, 0.000000000000000000 ) ) ;
#3426=VECTOR ( 'NONE', #74195, 1000.000000000000000 ) ;
#3427=CARTESIAN_POINT ( 'NONE',  ( 97.53191058446375905, -39.74916629817411717, 66.57112017202103971 ) ) ;
#3428=EDGE_CURVE ( 'NONE', #10086, #80351, #7057, .T. ) ;
#3430=ORIENTED_EDGE ( 'NONE', *, *, #49161, .F. ) ;
#3431=CARTESIAN_POINT ( 'NONE',  ( 115.5032561769494066, -38.06248691838574416, 113.1238483995059596 ) ) ;
#3432=FACE_OUTER_BOUND ( 'NONE', #89510, .T. ) ;
#3434=CARTESIAN_POINT ( 'NONE',  ( 103.3702027031294648, -47.12181610991854086, 98.31657765686297523 ) ) ;
#3436=CARTESIAN_POINT ( 'NONE',  ( 78.64593636902102958, -16.36767598605628393, 7.908804215164068729 ) ) ;
#3438=CARTESIAN_POINT ( 'NONE',  ( 105.5226833586260682, -46.38761039419750176, 37.44991099019695469 ) ) ;
#3440=ORIENTED_EDGE ( 'NONE', *, *, #73892, .F. ) ;
#3441=VERTEX_POINT ( 'NONE', #73616 ) ;
#3444=DIRECTION ( 'NONE',  ( 1.000000000000000078E-15, 1.000000000000000083E-30, -1.000000000000000000 ) ) ;
#3448=CARTESIAN_POINT ( 'NONE',  ( 130.5667039024479834, -36.72944715994100306, 239.5838068554162987 ) ) ;
#3449=CARTESIAN_POINT ( 'NONE',  ( 109.7256116747375785, -27.00100285621926233, 50.86608334895753813 ) ) ;
#3453=CARTESIAN_POINT ( 'NONE',  ( 112.7298150101557894, -27.26422151970076158, 54.65943479971996055 ) ) ;
#3455=EDGE_CURVE ( 'NONE', #79347, #59817, #19546, .T. ) ;
#3456=ORIENTED_EDGE ( 'NONE', *, *, #348, .T. ) ;
#3459=FACE_BOUND ( 'NONE', #49722, .T. ) ;
#3460=CARTESIAN_POINT ( 'NONE',  ( 98.14730025337767927, -34.17130281729839680, 138.9223760838769692 ) ) ;
#3461=VECTOR ( 'NONE', #53125, 1000.000000000000000 ) ;
#3462=AXIS2_PLACEMENT_3D ( 'NONE', #13486, #56133, #747 ) ;
#3463=CARTESIAN_POINT ( 'NONE',  ( 34.27258461953899626, -35.55794170701810941, -5.074374724088000832 ) ) ;
#3466=EDGE_CURVE ( 'NONE', #51387, #71603, #40435, .T. ) ;
#3467=CARTESIAN_POINT ( 'NONE',  ( 151.0371591254575776, -24.42818131005592974, 117.4678068554150485 ) ) ;
#3468=CIRCLE ( 'NONE', #15079, 16.00000000000000000 ) ;
#3470=ORIENTED_EDGE ( 'NONE', *, *, #14907, .F. ) ;
#3473=CARTESIAN_POINT ( 'NONE',  ( 102.8032110495234264, -45.10208326393837552, 168.6453928297069353 ) ) ;
#3474=FACE_OUTER_BOUND ( 'NONE', #11009, .T. ) ;
#3477=VERTEX_POINT ( 'NONE', #5028 ) ;
#3478=ORIENTED_EDGE ( 'NONE', *, *, #38035, .F. ) ;
#3480=CARTESIAN_POINT ( 'NONE',  ( 104.4487311862825578, -28.48030787377049577, 203.1271379886389639 ) ) ;
#3481=CARTESIAN_POINT ( 'NONE',  ( 98.62940354253828446, -43.90657238178356181, 76.89943479971999807 ) ) ;
#3482=CARTESIAN_POINT ( 'NONE',  ( 96.70769389551958284, -42.43415482991314036, 26.72705384733997747 ) ) ;
#3483=CARTESIAN_POINT ( 'NONE',  ( 64.68306507141296890, -72.55818180160879649, 361.9756252759101471 ) ) ;
#3484=CARTESIAN_POINT ( 'NONE',  ( 182.5667039024478413, -32.29483332967956244, 193.9678068554150059 ) ) ;
#3485=CARTESIAN_POINT ( 'NONE',  ( 98.16828830165673025, -31.29763223543249850, 166.8899109901969950 ) ) ;
#3486=LINE ( 'NONE', #30751, #59578 ) ;
#3488=CARTESIAN_POINT ( 'NONE',  ( 116.3212776292270973, -32.94146857470704504, 49.13562527591097506 ) ) ;
#3490=FACE_OUTER_BOUND ( 'NONE', #41059, .T. ) ;
#3491=ORIENTED_EDGE ( 'NONE', *, *, #4004, .F. ) ;
#3492=ORIENTED_EDGE ( 'NONE', *, *, #83767, .F. ) ;
#3494=DIRECTION ( 'NONE',  ( -0.000000000000000000, 0.000000000000000000, -1.000000000000000000 ) ) ;
#3496=CARTESIAN_POINT ( 'NONE',  ( 101.1408812403245747, -27.39851324166288649, 65.51467289495799662 ) ) ;
#3497=CARTESIAN_POINT ( 'NONE',  ( 86.06670390244796920, -48.82844715994099971, 310.9178068554150514 ) ) ;
#3499=EDGE_CURVE ( 'NONE', #67881, #66948, #40876, .T. ) ;
#3500=DIRECTION ( 'NONE',  ( 4.299999999999999979E-14, -1.000000000000000000, 4.400000000000000367E-29 ) ) ;
#3502=CARTESIAN_POINT ( 'NONE',  ( 107.8187922529720026, -26.97765417004747945, 70.01562527591099183 ) ) ;
#3503=FACE_OUTER_BOUND ( 'NONE', #64211, .T. ) ;
#3504=CARTESIAN_POINT ( 'NONE',  ( 116.7748712849171255, -40.56502120445009751, 189.5270538473389479 ) ) ;
#3508=FACE_OUTER_BOUND ( 'NONE', #6204, .T. ) ;
#3509=DIRECTION ( 'NONE',  ( 0.000000000000000000, 0.000000000000000000, -1.000000000000000000 ) ) ;
#3510=CARTESIAN_POINT ( 'NONE',  ( 97.60821144546386563, -39.98336359112931859, 136.5904942992093538 ) ) ;
#3511=CARTESIAN_POINT ( 'NONE',  ( 177.0371591254545365, -48.62818131005479927, 193.9678068554150059 ) ) ;
#3512=CARTESIAN_POINT ( 'NONE',  ( 116.8989603263487567, -40.32514756444775372, 218.5470538473399529 ) ) ;
#3513=ORIENTED_EDGE ( 'NONE', *, *, #36390, .F. ) ;
#3514=CARTESIAN_POINT ( 'NONE',  ( 97.80413494325495094, -40.49892049533512051, 146.6340343114085840 ) ) ;
#3515=CARTESIAN_POINT ( 'NONE',  ( 111.6179861195847849, -46.13269558042843244, 243.9356252759109509 ) ) ;
#3516=CARTESIAN_POINT ( 'NONE',  ( 104.9540660161283370, -25.01839229886434524, 121.2184824187679766 ) ) ;
#3518=CARTESIAN_POINT ( 'NONE',  ( 82.49755700851245876, -38.01506174167302987, 7.157201688890673985 ) ) ;
#3519=CARTESIAN_POINT ( 'NONE',  ( 128.5492039024480277, -51.22944715994093912, 231.5838068554170093 ) ) ;
#3520=DIRECTION ( 'NONE',  ( 1.000000000000000078E-15, -1.000000000000000083E-30, -1.000000000000000000 ) ) ;
#3521=EDGE_LOOP ( 'NONE', ( #36204, #39976, #27229, #43307, #43469 ) ) ;
#3522=VECTOR ( 'NONE', #75529, 999.9999999999998863 ) ;
#3525=AXIS2_PLACEMENT_3D ( 'NONE', #13100, #56185, #40783 ) ;
#3526=AXIS2_PLACEMENT_3D ( 'NONE', #32532, #10753, #86632 ) ;
#3527=VERTEX_POINT ( 'NONE', #39985 ) ;
#3530=CIRCLE ( 'NONE', #26738, 2.117000000000007987 ) ;
#3533=CARTESIAN_POINT ( 'NONE',  ( 97.21679027376985971, -33.31418093018012172, 282.0613395616252888 ) ) ;
#3535=CARTESIAN_POINT ( 'NONE',  ( 131.9692527705847169, -34.94806367531011659, 2.376725340804888731 ) ) ;
#3536=ADVANCED_FACE ( 'NONE', ( #68604 ), #67700, .T. ) ;
#3537=ADVANCED_FACE ( 'NONE', ( #26804 ), #33627, .T. ) ;
#3538=DIRECTION ( 'NONE',  ( 1.000000000000000000, 4.163336342344333240E-14, 0.000000000000000000 ) ) ;
#3540=CARTESIAN_POINT ( 'NONE',  ( 115.9692459539148643, -35.07008363779494431, 203.4076579233149573 ) ) ;
#3541=ORIENTED_EDGE ( 'NONE', *, *, #83553, .T. ) ;
#3542=ORIENTED_EDGE ( 'NONE', *, *, #71061, .T. ) ;
#3544=LINE ( 'NONE', #10796, #16633 ) ;
#3545=CARTESIAN_POINT ( 'NONE',  ( 105.7152538737207834, -46.72382489312290943, 182.4690088981411407 ) ) ;
#3546=ADVANCED_FACE ( 'NONE', ( #87699 ), #13193, .T. ) ;
#3547=DIRECTION ( 'NONE',  ( 1.000000000000000000, 0.000000000000000000, 0.000000000000000000 ) ) ;
#3548=CARTESIAN_POINT ( 'NONE',  ( 116.4309197881342612, -37.49355097060504249, 35.20539282970796791 ) ) ;
#3550=CARTESIAN_POINT ( 'NONE',  ( 193.0371591254585155, -47.82818131005411999, 180.4678068554150343 ) ) ;
#3552=DIRECTION ( 'NONE',  ( 0.000000000000000000, 0.000000000000000000, -1.000000000000000000 ) ) ;
#3555=ORIENTED_EDGE ( 'NONE', *, *, #9128, .T. ) ;
#3556=CARTESIAN_POINT ( 'NONE',  ( 172.5667039024480687, -36.32844715993499563, 129.9678068554150059 ) ) ;
#3557=CARTESIAN_POINT ( 'NONE',  ( 105.2414988608755522, -45.18937368885499950, 30.23761417911497063 ) ) ;
#3559=CARTESIAN_POINT ( 'NONE',  ( 89.06648138392553449, -56.72944715994104570, -5.074374724089047106 ) ) ;
#3561=CARTESIAN_POINT ( 'NONE',  ( 172.5664832912740110, -32.07844715994070839, 194.1756252759119832 ) ) ;
#3562=FACE_OUTER_BOUND ( 'NONE', #19344, .T. ) ;
#3564=CARTESIAN_POINT ( 'NONE',  ( 71.24189083761808661, -0.9290567490904538817, 540.9756252759101471 ) ) ;
#3567=ORIENTED_EDGE ( 'NONE', *, *, #18617, .T. ) ;
#3568=CARTESIAN_POINT ( 'NONE',  ( 117.3389957193927131, -32.64844533837379004, 99.13943479972098771 ) ) ;
#3569=ORIENTED_EDGE ( 'NONE', *, *, #67007, .T. ) ;
#3570=EDGE_CURVE ( 'NONE', #32266, #69245, #75200, .T. ) ;
#3571=CARTESIAN_POINT ( 'NONE',  ( 114.7034172354883168, -32.83980166744527196, 43.62384839950495063 ) ) ;
#3572=EDGE_CURVE ( 'NONE', #54506, #83131, #72295, .T. ) ;
#3573=CARTESIAN_POINT ( 'NONE',  ( 102.0492436467375654, -45.42708556363530192, 88.15966356583727759 ) ) ;
#3574=CARTESIAN_POINT ( 'NONE',  ( 105.1055546886446308, -45.37138199117224957, 68.83015473446796761 ) ) ;
#3579=CARTESIAN_POINT ( 'NONE',  ( 109.6483737747080198, -46.85224817473300618, 43.77562527591094721 ) ) ;
#3580=CARTESIAN_POINT ( 'NONE',  ( 22.49541547940750164, -78.44951497180814215, 342.9256252759109884 ) ) ;
#3581=VERTEX_POINT ( 'NONE', #53591 ) ;
#3585=CARTESIAN_POINT ( 'NONE',  ( 48.79742451362098166, -36.32844715994040996, -5.074374724088000832 ) ) ;
#3586=VECTOR ( 'NONE', #16838, 1000.000000000000000 ) ;
#3590=VERTEX_POINT ( 'NONE', #46335 ) ;
#3591=CIRCLE ( 'NONE', #55758, 1.000000000000000888 ) ;
#3593=AXIS2_PLACEMENT_3D ( 'NONE', #24118, #38620, #37292 ) ;
#3594=CARTESIAN_POINT ( 'NONE',  ( 115.3120223323506792, -44.18753462406608179, 233.2413395616259493 ) ) ;
#3595=CARTESIAN_POINT ( 'NONE',  ( 101.0140741488528846, -28.73402828939939369, 125.5909382567238453 ) ) ;
#3597=CARTESIAN_POINT ( 'NONE',  ( 100.9432064590905469, -28.29215089373294489, 71.57562527591099411 ) ) ;
#3598=CARTESIAN_POINT ( 'NONE',  ( 98.15075042664197724, -41.26116664859105043, 42.70068335180353358 ) ) ;
#3599=ORIENTED_EDGE ( 'NONE', *, *, #13625, .F. ) ;
#3600=CARTESIAN_POINT ( 'NONE',  ( 97.78478760265450376, -40.45112112471975507, 172.6299302010647239 ) ) ;
#3601=CARTESIAN_POINT ( 'NONE',  ( 63.56670390244745050, -47.82844715994014706, 129.9678068554150911 ) ) ;
#3602=ORIENTED_EDGE ( 'NONE', *, *, #89579, .F. ) ;
#3605=CARTESIAN_POINT ( 'NONE',  ( 107.5091008941355994, -47.12332782054438951, 237.6099109901969655 ) ) ;
#3606=CARTESIAN_POINT ( 'NONE',  ( 164.9212702847350158, -29.73316016639540749, -5.074374724088000832 ) ) ;
#3608=LINE ( 'NONE', #58999, #12955 ) ;
#3609=CARTESIAN_POINT ( 'NONE',  ( 97.81413906161476746, -40.51632882248723888, 267.6361360915977343 ) ) ;
#3610=CARTESIAN_POINT ( 'NONE',  ( 114.8173571680961231, -40.38677627709480333, 227.8981341137909453 ) ) ;
#3611=DIRECTION ( 'NONE',  ( 0.7071067811866377228, -0.7071067811864573116, 0.000000000000000000 ) ) ;
#3612=CARTESIAN_POINT ( 'NONE',  ( 104.0490797691970073, -47.33883444496879633, 63.36800622829197494 ) ) ;
#3614=CARTESIAN_POINT ( 'NONE',  ( 114.0157635323931515, -28.07379075743241259, 119.5261014663869474 ) ) ;
#3616=CARTESIAN_POINT ( 'NONE',  ( 133.3151861768397168, -21.40257939794838293, 8.160477455083581688 ) ) ;
#3618=DIRECTION ( 'NONE',  ( -6.524622321627019585E-16, -3.741823817616790462E-31, -1.000000000000000000 ) ) ;
#3619=DIRECTION ( 'NONE',  ( -0.9254794337955623007, -0.3787978585227819162, 0.000000000000000000 ) ) ;
#3620=DIRECTION ( 'NONE',  ( 0.000000000000000000, 0.000000000000000000, -1.000000000000000000 ) ) ;
#3621=ORIENTED_EDGE ( 'NONE', *, *, #78173, .F. ) ;
#3622=CARTESIAN_POINT ( 'NONE',  ( 97.79834681188958712, -40.48468739506365210, 51.63281160315436580 ) ) ;
#3623=CARTESIAN_POINT ( 'NONE',  ( 104.0952645214482430, -46.76829794407347407, 107.3470538473389411 ) ) ;
#3624=ORIENTED_EDGE ( 'NONE', *, *, #67742, .T. ) ;
#3625=LINE ( 'NONE', #25407, #53791 ) ;
#3626=LINE ( 'NONE', #36818, #72255 ) ;
#3627=AXIS2_PLACEMENT_3D ( 'NONE', #24939, #15904, #71322 ) ;
#3629=VERTEX_POINT ( 'NONE', #81360 ) ;
#3630=CARTESIAN_POINT ( 'NONE',  ( 116.9427733469681385, -33.21558069166144378, 114.0984824187679720 ) ) ;
#3631=EDGE_CURVE ( 'NONE', #50606, #71390, #83912, .T. ) ;
#3632=CIRCLE ( 'NONE', #54360, 2.517500000000000071 ) ;
#3635=CARTESIAN_POINT ( 'NONE',  ( 32.09598329127609873, -23.42844715994129956, 193.9678068554150911 ) ) ;
#3637=CARTESIAN_POINT ( 'NONE',  ( 116.3212776292272537, -32.94146857470742162, 144.1356252759109680 ) ) ;
#3638=ORIENTED_EDGE ( 'NONE', *, *, #88566, .F. ) ;
#3640=EDGE_LOOP ( 'NONE', ( #24121, #11356, #56768, #63460 ) ) ;
#3642=DIRECTION ( 'NONE',  ( 1.000000000000000078E-15, 1.000000000000000083E-30, -1.000000000000000000 ) ) ;
#3644=EDGE_CURVE ( 'NONE', #41573, #70760, #28139, .T. ) ;
#3645=ADVANCED_FACE ( 'NONE', ( #55830 ), #67932, .T. ) ;
#3647=CARTESIAN_POINT ( 'NONE',  ( 93.79772160076439036, -35.59147263058779487, 299.5704287327187103 ) ) ;
#3648=DIRECTION ( 'NONE',  ( 9.912705577010326536E-16, 1.000000000000000000, 0.000000000000000000 ) ) ;
#3649=EDGE_CURVE ( 'NONE', #24119, #5757, #31685, .T. ) ;
#3650=EDGE_CURVE ( 'NONE', #623, #79790, #41762, .T. ) ;
#3652=EDGE_LOOP ( 'NONE', ( #65461, #50322, #39157, #72622 ) ) ;
#3653=AXIS2_PLACEMENT_3D ( 'NONE', #38063, #36731, #64432 ) ;
#3654=VECTOR ( 'NONE', #59725, 1000.000000000000000 ) ;
#3655=AXIS2_PLACEMENT_3D ( 'NONE', #13751, #6936, #28260 ) ;
#3656=FACE_OUTER_BOUND ( 'NONE', #37612, .T. ) ;
#3657=EDGE_CURVE ( 'NONE', #35758, #26375, #76305, .T. ) ;
#3658=CARTESIAN_POINT ( 'NONE',  ( 99.36405074150921735, -30.70139697576588134, 151.7984824187679465 ) ) ;
#3659=DIRECTION ( 'NONE',  ( 0.9999999853157766072, 0.0001713722456134502174, 0.000000000000000000 ) ) ;
#3660=ORIENTED_EDGE ( 'NONE', *, *, #21086, .F. ) ;
#3661=CARTESIAN_POINT ( 'NONE',  ( 98.38136461969652657, -29.78821554292439444, 41.78991099019696520 ) ) ;
#3662=DIRECTION ( 'NONE',  ( 1.000000000000000078E-15, -1.000000000000000083E-30, -1.000000000000000000 ) ) ;
#3663=CARTESIAN_POINT ( 'NONE',  ( 172.5664832912729878, -27.82844715994070484, 318.9256252759120116 ) ) ;
#3668=ORIENTED_EDGE ( 'NONE', *, *, #67409, .F. ) ;
#3669=ORIENTED_EDGE ( 'NONE', *, *, #1328, .T. ) ;
#3671=CARTESIAN_POINT ( 'NONE',  ( 112.1289716242999361, -44.03925847519028025, 199.4901547344690016 ) ) ;
#3672=CYLINDRICAL_SURFACE ( 'NONE', #73405, 2.030000000001869864 ) ;
#3674=AXIS2_PLACEMENT_3D ( 'NONE', #56916, #83748, #70562 ) ;
#3677=EDGE_LOOP ( 'NONE', ( #25344, #41434 ) ) ;
#3679=CARTESIAN_POINT ( 'NONE',  ( 116.3130905035090876, -32.93898513502411163, 35.13562527591096796 ) ) ;
#3681=CARTESIAN_POINT ( 'NONE',  ( 106.2286657330468103, -47.72771449247521502, 267.5280062282920994 ) ) ;
#3684=EDGE_CURVE ( 'NONE', #59373, #41311, #73765, .T. ) ;
#3687=CARTESIAN_POINT ( 'NONE',  ( 182.4202572930269923, -31.94127993907680718, -5.074374724088000832 ) ) ;
#3689=EDGE_CURVE ( 'NONE', #31817, #11027, #21806, .T. ) ;
#3691=CARTESIAN_POINT ( 'NONE',  ( 102.2170635254687454, -46.00716819922848799, 208.1927681330539599 ) ) ;
#3694=CARTESIAN_POINT ( 'NONE',  ( 97.03360904796217312, -33.74039811955494628, 27.09562527591097236 ) ) ;
#3695=CARTESIAN_POINT ( 'NONE',  ( 72.06648329127399677, -9.729447159941065237, -4.824374724089063982 ) ) ;
#3696=VECTOR ( 'NONE', #13797, 1000.000000000000000 ) ;
#3697=CARTESIAN_POINT ( 'NONE',  ( 116.5821416419259435, -42.35362450032752690, 283.4137205140060587 ) ) ;
#3698=ORIENTED_EDGE ( 'NONE', *, *, #86343, .T. ) ;
#3699=CARTESIAN_POINT ( 'NONE',  ( 81.12494507884962047, -16.19118199975293848, 1.799893109327372009 ) ) ;
#3700=CARTESIAN_POINT ( 'NONE',  ( 98.04140782067196369, -41.04162603110138718, 17.68090933045322899 ) ) ;
#3702=CARTESIAN_POINT ( 'NONE',  ( 114.7692409103599687, -39.43078961860824450, 131.3766617981629565 ) ) ;
#3703=CARTESIAN_POINT ( 'NONE',  ( 116.6256809191353909, -40.94358996305180654, 249.4956252759109532 ) ) ;
#3705=ORIENTED_EDGE ( 'NONE', *, *, #4708, .F. ) ;
#3706=CARTESIAN_POINT ( 'NONE',  ( 135.5598545223519693, -39.04079274305309610, 1.981704437697082488 ) ) ;
#3708=EDGE_LOOP ( 'NONE', ( #86674, #58448, #5739, #63634 ) ) ;
#3709=VECTOR ( 'NONE', #70823, 1000.000000000000114 ) ;
#3712=AXIS2_PLACEMENT_3D ( 'NONE', #39625, #80999, #88702 ) ;
#3716=VECTOR ( 'NONE', #8640, 1000.000000000000000 ) ;
#3717=CARTESIAN_POINT ( 'NONE',  ( 100.9535868929799989, -28.70787548350885388, 25.59406758372123392 ) ) ;
#3718=CARTESIAN_POINT ( 'NONE',  ( 99.50386058399449496, -32.75919911893461034, 135.3638483995049739 ) ) ;
#3719=VECTOR ( 'NONE', #61055, 1000.000000000000000 ) ;
#3720=CARTESIAN_POINT ( 'NONE',  ( 99.10996421577944204, -43.53389204880360097, 31.88991099019594699 ) ) ;
#3721=VERTEX_POINT ( 'NONE', #69497 ) ;
#3724=AXIS2_PLACEMENT_3D ( 'NONE', #82886, #32914, #40629 ) ;
#3725=FACE_OUTER_BOUND ( 'NONE', #16206, .T. ) ;
#3727=DIRECTION ( 'NONE',  ( 0.000000000000000000, 0.000000000000000000, 1.000000000000000000 ) ) ;
#3728=DIRECTION ( 'NONE',  ( -0.04216478779797398074, 0.9991106698809455455, 0.000000000000000000 ) ) ;
#3729=DIRECTION ( 'NONE',  ( 1.000000000000000078E-15, -1.000000000000000083E-30, -1.000000000000000000 ) ) ;
#3731=EDGE_CURVE ( 'NONE', #26105, #85262, #8497, .T. ) ;
#3732=DIRECTION ( 'NONE',  ( 0.000000000000000000, 0.000000000000000000, -1.000000000000000000 ) ) ;
#3733=VERTEX_POINT ( 'NONE', #69944 ) ;
#3734=CARTESIAN_POINT ( 'NONE',  ( 100.1774089044720881, -45.37350532423673144, 272.0289586092443415 ) ) ;
#3735=CARTESIAN_POINT ( 'NONE',  ( 111.1459338097010914, -47.05202348217205355, 18.88800622829195319 ) ) ;
#3738=EDGE_CURVE ( 'NONE', #68582, #12535, #85414, .T. ) ;
#3740=DIRECTION ( 'NONE',  ( 2.900000000000000265E-14, -2.000000000000000155E-15, 1.000000000000000000 ) ) ;
#3741=CARTESIAN_POINT ( 'NONE',  ( 107.0664832912730020, -36.72944715994189835, 361.9756252759109998 ) ) ;
#3744=CARTESIAN_POINT ( 'NONE',  ( 83.06670390244796920, -64.87844715994098976, 231.5838068554150198 ) ) ;
#3746=PLANE ( 'NONE',  #6882 ) ;
#3748=DIRECTION ( 'NONE',  ( 0.000000000000000000, 0.000000000000000000, -1.000000000000000000 ) ) ;
#3749=EDGE_CURVE ( 'NONE', #86967, #73636, #69045, .T. ) ;
#3750=CARTESIAN_POINT ( 'NONE',  ( 111.1461885285858671, -47.05266801877174032, 22.88800622829195675 ) ) ;
#3751=CARTESIAN_POINT ( 'NONE',  ( 110.1374552785425323, -26.11139123911904036, 210.8403871806729626 ) ) ;
#3752=CARTESIAN_POINT ( 'NONE',  ( 96.89995799317335923, -32.33320227283598314, 57.01372051400599616 ) ) ;
#3753=CARTESIAN_POINT ( 'NONE',  ( 137.0667039024479834, -50.82844715994100682, 10.91780685541479734 ) ) ;
#3754=FACE_OUTER_BOUND ( 'NONE', #40941, .T. ) ;
#3755=DIRECTION ( 'NONE',  ( 1.000000000000000078E-15, -1.000000000000000083E-30, -1.000000000000000000 ) ) ;
#3759=CARTESIAN_POINT ( 'NONE',  ( 97.06107108242123616, -37.99641184083684919, 187.4272919328122953 ) ) ;
#3761=ADVANCED_FACE ( 'NONE', ( #54931 ), #8166, .T. ) ;
#3762=CARTESIAN_POINT ( 'NONE',  ( 97.55373691267115532, -39.00345059616618215, 52.51276813305294411 ) ) ;
#3764=EDGE_LOOP ( 'NONE', ( #73099, #42268, #13323, #10176 ) ) ;
#3765=DIRECTION ( 'NONE',  ( -1.000000000000000000, 0.000000000000000000, 0.000000000000000000 ) ) ;
#3766=CARTESIAN_POINT ( 'NONE',  ( 103.8265608274144398, -48.10271009292816302, 213.3556252759109668 ) ) ;
#3767=CARTESIAN_POINT ( 'NONE',  ( 163.0667039024478697, -33.35206098992140511, 193.9678068554149775 ) ) ;
#3768=LINE ( 'NONE', #2440, #5172 ) ;
#3769=DIRECTION ( 'NONE',  ( 1.000000000000000000, 4.163336342344333240E-14, 0.000000000000000000 ) ) ;
#3770=CARTESIAN_POINT ( 'NONE',  ( 95.60734603896362671, -36.72944715994100306, 312.6356252759112522 ) ) ;
#3771=ADVANCED_FACE ( 'NONE', ( #84492 ), #77658, .T. ) ;
#3772=CARTESIAN_POINT ( 'NONE',  ( 131.6146038194004007, -37.97617057399416751, 2.716753174567031692 ) ) ;
#3774=CARTESIAN_POINT ( 'NONE',  ( 96.37928053093608582, -33.66421044892479131, 141.1041967044829732 ) ) ;
#3775=ORIENTED_EDGE ( 'NONE', *, *, #28084, .F. ) ;
#3776=ORIENTED_EDGE ( 'NONE', *, *, #52717, .T. ) ;
#3777=VECTOR ( 'NONE', #65567, 1000.000000000000000 ) ;
#3778=CARTESIAN_POINT ( 'NONE',  ( 102.5524010923236915, -28.48932656383806972, 96.89491663923000431 ) ) ;
#3779=AXIS2_PLACEMENT_3D ( 'NONE', #86414, #78718, #10103 ) ;
#3780=LINE ( 'NONE', #66438, #13834 ) ;
#3781=AXIS2_PLACEMENT_3D ( 'NONE', #47669, #88590, #75403 ) ;
#3782=CARTESIAN_POINT ( 'NONE',  ( 116.5994914424365021, -40.81117973626238893, 209.5165776568629497 ) ) ;
#3783=CARTESIAN_POINT ( 'NONE',  ( 41.56648329127399677, -9.303447159940999356, 78.92562527591199739 ) ) ;
#3791=CARTESIAN_POINT ( 'NONE',  ( 103.4759237351580623, -46.49349013887667326, 142.2956252759109645 ) ) ;
#3795=DIRECTION ( 'NONE',  ( 0.000000000000000000, 0.000000000000000000, 1.000000000000000000 ) ) ;
#3797=LINE ( 'NONE', #31484, #16345 ) ;
#3801=( BOUNDED_CURVE ( )  B_SPLINE_CURVE ( 3, ( #64744, #24307, #51973, #79731 ),
 .UNSPECIFIED., .F., .T. ) 
 B_SPLINE_CURVE_WITH_KNOTS ( ( 4, 4 ),
 ( 1.570796326793645337, 3.141592653589136308 ),
 .UNSPECIFIED. ) 
 CURVE ( )  GEOMETRIC_REPRESENTATION_ITEM ( )  RATIONAL_B_SPLINE_CURVE ( ( 1.000000000000000000, 0.8047378541242249383, 0.8047378541242249383, 1.000000000000000000 ) ) 
 REPRESENTATION_ITEM ( '' )  );
#3802=CIRCLE ( 'NONE', #21247, 1.000000000000000888 ) ;
#3803=CARTESIAN_POINT ( 'NONE',  ( 102.6834449319766378, -27.27027144519976787, 180.4213395616249898 ) ) ;
#3805=ORIENTED_EDGE ( 'NONE', *, *, #17430, .T. ) ;
#3806=ORIENTED_EDGE ( 'NONE', *, *, #71834, .F. ) ;
#3807=ORIENTED_EDGE ( 'NONE', *, *, #50702, .T. ) ;
#3808=CARTESIAN_POINT ( 'NONE',  ( 111.1351804138767108, -45.89630524753858509, 63.90945011243512397 ) ) ;
#3810=CARTESIAN_POINT ( 'NONE',  ( 131.3165190107491185, -36.55810522840583587, 6.749822759741316069 ) ) ;
#3811=CARTESIAN_POINT ( 'NONE',  ( 105.3283384058428851, -27.49606390364131414, 276.6682499725636717 ) ) ;
#3813=EDGE_LOOP ( 'NONE', ( #88115, #39666, #14670, #13222 ) ) ;
#3814=EDGE_CURVE ( 'NONE', #87871, #80786, #55383, .T. ) ;
#3816=DIRECTION ( 'NONE',  ( -0.02150753337723812844, -0.0009076677972192511400, -0.9997682742251809973 ) ) ;
#3817=ORIENTED_EDGE ( 'NONE', *, *, #71946, .T. ) ;
#3818=ORIENTED_EDGE ( 'NONE', *, *, #35470, .T. ) ;
#3819=ADVANCED_FACE ( 'NONE', ( #17221, #78119 ), #17661, .F. ) ;
#3821=ORIENTED_EDGE ( 'NONE', *, *, #37455, .T. ) ;
#3822=ORIENTED_EDGE ( 'NONE', *, *, #13507, .F. ) ;
#3823=CARTESIAN_POINT ( 'NONE',  ( 104.4882991616644290, -26.97926274729164575, 156.2813675130791751 ) ) ;
#3824=CARTESIAN_POINT ( 'NONE',  ( 114.2970346969270565, -32.18244176163005221, 33.69527697093299423 ) ) ;
#3825=CARTESIAN_POINT ( 'NONE',  ( 98.36125384756333290, -29.88003685912757490, 200.8080062282919869 ) ) ;
#3826=CARTESIAN_POINT ( 'NONE',  ( 115.0229693000241156, -29.09019634776596419, 189.4232443235299570 ) ) ;
#3827=CARTESIAN_POINT ( 'NONE',  ( 63.06670390244707392, -40.32844715994016838, 180.4678068554151196 ) ) ;
#3828=CARTESIAN_POINT ( 'NONE',  ( 96.77613930368880801, -40.76464245898888095, 242.6118157521009664 ) ) ;
#3830=DIRECTION ( 'NONE',  ( 0.000000000000000000, 1.000000000000000000, 0.000000000000000000 ) ) ;
#3833=VECTOR ( 'NONE', #60083, 1000.000000000000000 ) ;
#3835=CARTESIAN_POINT ( 'NONE',  ( 107.0664832912739399, -36.72944715994096754, 296.0306255462182321 ) ) ;
#3836=CARTESIAN_POINT ( 'NONE',  ( 99.72210660708088881, -29.26842865273154004, 225.6956252759109702 ) ) ;
#3837=VERTEX_POINT ( 'NONE', #24482 ) ;
#3839=CARTESIAN_POINT ( 'NONE',  ( 117.7793243111075157, -34.00655811778471360, 169.0365776568629599 ) ) ;
#3840=PLANE ( 'NONE',  #10867 ) ;
#3845=EDGE_CURVE ( 'NONE', #87253, #75711, #50372, .T. ) ;
#3846=DIRECTION ( 'NONE',  ( 0.000000000000000000, 0.000000000000000000, -1.000000000000000000 ) ) ;
#3847=DIRECTION ( 'NONE',  ( -0.000000000000000000, -0.000000000000000000, 1.000000000000000000 ) ) ;
#3848=CARTESIAN_POINT ( 'NONE',  ( 95.25611604350974915, -37.33230102880721546, 267.3670538473395482 ) ) ;
#3852=CARTESIAN_POINT ( 'NONE',  ( 99.09464024186620179, -30.55185734355772098, 271.8020006611150734 ) ) ;
#3855=DIRECTION ( 'NONE',  ( 1.000000000000000000, 4.510281037539819615E-14, 0.000000000000000000 ) ) ;
#3856=CARTESIAN_POINT ( 'NONE',  ( 97.07207206141239908, -35.37844118198271559, 77.21895860788390564 ) ) ;
#3857=CARTESIAN_POINT ( 'NONE',  ( 98.71706140474314850, -34.42688893107280990, 195.5838068554172366 ) ) ;
#3860=CYLINDRICAL_SURFACE ( 'NONE', #81467, 3.300000000000000711 ) ;
#3861=CARTESIAN_POINT ( 'NONE',  ( 95.88624405714097065, -32.72491640434669335, 176.0527681330539735 ) ) ;
#3862=CARTESIAN_POINT ( 'NONE',  ( 107.9456208643995012, -25.71123053419755422, 111.0251490854349754 ) ) ;
#3863=CARTESIAN_POINT ( 'NONE',  ( 98.80492496406409941, -29.31701487593723598, 231.7565776568629587 ) ) ;
#3864=CARTESIAN_POINT ( 'NONE',  ( 163.2449138993005988, -32.11662333284040471, 313.9678068554149490 ) ) ;
#3865=DIRECTION ( 'NONE',  ( 1.907762142705490052E-15, 7.167082501179359715E-16, -1.000000000000000000 ) ) ;
#3866=CIRCLE ( 'NONE', #73486, 2.116999999999993776 ) ;
#3868=CARTESIAN_POINT ( 'NONE',  ( 116.9761379366299536, -35.34627962053155414, 39.93653275092082566 ) ) ;
#3870=DIRECTION ( 'NONE',  ( 1.000000000000000078E-15, -1.000000000000000083E-30, -1.000000000000000000 ) ) ;
#3871=CARTESIAN_POINT ( 'NONE',  ( 107.0664832912739968, -36.72944715994100306, 287.6356252759109680 ) ) ;
#3872=VERTEX_POINT ( 'NONE', #85386 ) ;
#3873=EDGE_LOOP ( 'NONE', ( #7907, #32328, #73171, #70582 ) ) ;
#3874=EDGE_CURVE ( 'NONE', #75709, #88176, #47359, .T. ) ;
#3875=CARTESIAN_POINT ( 'NONE',  ( 99.91372553312717741, -41.39787175238471661, 101.2095626852199644 ) ) ;
#3878=CARTESIAN_POINT ( 'NONE',  ( 117.0854383170105564, -39.53109055650221393, 94.60991099019693706 ) ) ;
#3880=CARTESIAN_POINT ( 'NONE',  ( 78.15700282949597977, -16.74831852143626776, 7.618261863063606754 ) ) ;
#3881=DIRECTION ( 'NONE',  ( 1.639958061481212836E-42, -4.100000000000000342E-29, -1.000000000000000000 ) ) ;
#3882=CARTESIAN_POINT ( 'NONE',  ( 97.35451824726682446, -37.88753622196094994, 41.42133956162496844 ) ) ;
#3883=ORIENTED_EDGE ( 'NONE', *, *, #74025, .T. ) ;
#3884=EDGE_LOOP ( 'NONE', ( #55485, #43005, #50208, #1541 ) ) ;
#3885=ORIENTED_EDGE ( 'NONE', *, *, #60743, .T. ) ;
#3887=CARTESIAN_POINT ( 'NONE',  ( 96.70615320395842218, -37.17927570127480408, 112.3489586092439652 ) ) ;
#3888=CARTESIAN_POINT ( 'NONE',  ( 73.06648329127402519, -46.72944715994106701, -4.824374724089063982 ) ) ;
#3889=CARTESIAN_POINT ( 'NONE',  ( 97.33784131355466229, -34.07106452111344908, 117.1147919418627197 ) ) ;
#3890=CYLINDRICAL_SURFACE ( 'NONE', #71207, 3.299999999999997158 ) ;
#3891=CARTESIAN_POINT ( 'NONE',  ( 97.81452210549078075, -40.51628237377364883, 52.63520911028864901 ) ) ;
#3892=FACE_OUTER_BOUND ( 'NONE', #68733, .T. ) ;
#3895=CARTESIAN_POINT ( 'NONE',  ( 97.30890135812528285, -33.12136451854834007, 66.04419670448297097 ) ) ;
#3896=VERTEX_POINT ( 'NONE', #30396 ) ;
#3899=DIRECTION ( 'NONE',  ( 1.639958061481212836E-42, -4.100000000000000342E-29, -1.000000000000000000 ) ) ;
#3900=CONICAL_SURFACE ( 'NONE', #54630, 1.624999999999987566, 1.029744258676650093 ) ;
#3903=CARTESIAN_POINT ( 'NONE',  ( 101.0810522191901981, -29.63898995574150419, 148.4538046553059587 ) ) ;
#3904=VECTOR ( 'NONE', #25181, 1000.000000000000000 ) ;
#3906=AXIS2_PLACEMENT_3D ( 'NONE', #3463, #72069, #79341 ) ;
#3908=CARTESIAN_POINT ( 'NONE',  ( 33.96670390244699433, -28.27351298637401200, -5.074374724088000832 ) ) ;
#3910=ORIENTED_EDGE ( 'NONE', *, *, #54882, .T. ) ;
#3912=ORIENTED_EDGE ( 'NONE', *, *, #71345, .F. ) ;
#3914=CARTESIAN_POINT ( 'NONE',  ( 141.0667039024479834, -58.72944715994110254, 250.9178068554160461 ) ) ;
#3915=CARTESIAN_POINT ( 'NONE',  ( 112.6322303140947838, -44.29905650357037672, 179.5006309249449430 ) ) ;
#3916=FACE_BOUND ( 'NONE', #1115, .T. ) ;
#3919=FACE_BOUND ( 'NONE', #68705, .T. ) ;
#3924=ORIENTED_EDGE ( 'NONE', *, *, #7846, .T. ) ;
#3925=ORIENTED_EDGE ( 'NONE', *, *, #49577, .T. ) ;
#3926=CARTESIAN_POINT ( 'NONE',  ( 98.43814749271325582, -36.05658283995993685, 189.0947570362579597 ) ) ;
#3927=CARTESIAN_POINT ( 'NONE',  ( 101.4890226443523744, -27.89551843606815495, 110.5241967044819944 ) ) ;
#3928=CARTESIAN_POINT ( 'NONE',  ( 114.8031991714177451, -43.68443766454706889, 38.24419670448192221 ) ) ;
#3929=CARTESIAN_POINT ( 'NONE',  ( 117.0602230546818703, -38.08518235923209971, 253.7190022475310229 ) ) ;
#3931=CARTESIAN_POINT ( 'NONE',  ( 163.0664832912739826, 19.62155284005901024, 327.8006252759110453 ) ) ;
#3932=CARTESIAN_POINT ( 'NONE',  ( 102.9671325615611437, -26.46449201736525225, 171.3908633711489813 ) ) ;
#3933=CARTESIAN_POINT ( 'NONE',  ( 107.0664832912739968, -36.72944715994100306, 287.6356252759109680 ) ) ;
#3936=VERTEX_POINT ( 'NONE', #2700 ) ;
#3938=CARTESIAN_POINT ( 'NONE',  ( 97.81461822720238786, -40.51595288653417981, 132.6359866545674890 ) ) ;
#3939=ORIENTED_EDGE ( 'NONE', *, *, #36113, .T. ) ;
#3940=ORIENTED_EDGE ( 'NONE', *, *, #6641, .T. ) ;
#3941=AXIS2_PLACEMENT_3D ( 'NONE', #44606, #87647, #23751 ) ;
#3944=CARTESIAN_POINT ( 'NONE',  ( 116.3212776292296127, -32.94146857471318413, 287.6356252759109680 ) ) ;
#3945=CARTESIAN_POINT ( 'NONE',  ( 113.4596546395850680, -46.70781606211470205, 68.02991099019695298 ) ) ;
#3946=CARTESIAN_POINT ( 'NONE',  ( 51.23005224011622261, -33.89581943344351345, 193.9678068554150911 ) ) ;
#3947=CARTESIAN_POINT ( 'NONE',  ( 46.83715912545429916, -47.82818131006083462, 237.4678068554150059 ) ) ;
#3949=CARTESIAN_POINT ( 'NONE',  ( 109.9668656698224822, -46.07028316908886723, 97.81562527591097478 ) ) ;
#3950=CARTESIAN_POINT ( 'NONE',  ( 72.17003668186727339, -45.68655394112764156, 14.92562527591097776 ) ) ;
#3951=CARTESIAN_POINT ( 'NONE',  ( 117.4355769707882473, -40.49052663852277334, 169.5375300378159693 ) ) ;
#3953=EDGE_CURVE ( 'NONE', #84928, #42564, #84934, .T. ) ;
#3954=LINE ( 'NONE', #37593, #32226 ) ;
#3957=EDGE_CURVE ( 'NONE', #17048, #13307, #32851, .T. ) ;
#3958=CARTESIAN_POINT ( 'NONE',  ( 31.71315051185421297, -33.70561438052095582, 193.9678068554150911 ) ) ;
#3959=EDGE_CURVE ( 'NONE', #53860, #137, #64472, .T. ) ;
#3961=FACE_OUTER_BOUND ( 'NONE', #27959, .T. ) ;
#3962=CARTESIAN_POINT ( 'NONE',  ( 96.14524839136181811, -32.00129468986670389, 211.0013395616249738 ) ) ;
#3963=ORIENTED_EDGE ( 'NONE', *, *, #73004, .T. ) ;
#3966=CARTESIAN_POINT ( 'NONE',  ( 116.2377588530493995, -41.80555791324388082, 259.4241967044827106 ) ) ;
#3967=CARTESIAN_POINT ( 'NONE',  ( 117.2518684062627727, -39.29770432102194633, 119.6299109901969615 ) ) ;
#3969=CARTESIAN_POINT ( 'NONE',  ( 193.0371591254572365, -23.42818131005412496, 300.4678068554149490 ) ) ;
#3970=CARTESIAN_POINT ( 'NONE',  ( 82.10313645209993183, -38.57950990140825098, 7.523361336351456430 ) ) ;
#3971=CARTESIAN_POINT ( 'NONE',  ( 172.5664832912740110, -9.303447159940999356, 18.92562527591200094 ) ) ;
#3972=CARTESIAN_POINT ( 'NONE',  ( 164.7812970173289955, -35.65087443492610930, 193.9678068554150059 ) ) ;
#3976=VECTOR ( 'NONE', #24362, 1000.000000000000000 ) ;
#3977=EDGE_LOOP ( 'NONE', ( #36622, #51457, #49224, #77566 ) ) ;
#3979=EDGE_CURVE ( 'NONE', #70069, #39961, #44453, .T. ) ;
#3982=CARTESIAN_POINT ( 'NONE',  ( 104.5881800117806932, -26.60309611811081254, 281.2670538473395823 ) ) ;
#3988=CARTESIAN_POINT ( 'NONE',  ( 104.9258105463076873, -28.46061097091046577, 199.7009912566479386 ) ) ;
#3989=EDGE_LOOP ( 'NONE', ( #47707, #62457 ) ) ;
#3991=ORIENTED_EDGE ( 'NONE', *, *, #40474, .F. ) ;
#3993=DIRECTION ( 'NONE',  ( 1.000000000000000000, 0.000000000000000000, 0.000000000000000000 ) ) ;
#3994=CARTESIAN_POINT ( 'NONE',  ( 104.4079088469246130, -46.45803334375896299, 182.3648505240071245 ) ) ;
#3996=CARTESIAN_POINT ( 'NONE',  ( 113.0371668699568204, -44.84250099658410704, 29.51301187732496700 ) ) ;
#3998=CYLINDRICAL_SURFACE ( 'NONE', #11467, 0.9999999999991942001 ) ;
#4000=VERTEX_POINT ( 'NONE', #58530 ) ;
#4001=DIRECTION ( 'NONE',  ( 0.000000000000000000, 0.000000000000000000, 1.000000000000000000 ) ) ;
#4002=ORIENTED_EDGE ( 'NONE', *, *, #27222, .T. ) ;
#4003=CARTESIAN_POINT ( 'NONE',  ( 83.56670559755343675, -40.03837296219067099, 249.5838068554176630 ) ) ;
#4004=EDGE_CURVE ( 'NONE', #21043, #43807, #26692, .T. ) ;
#4005=CARTESIAN_POINT ( 'NONE',  ( 99.12746238500623974, -38.62725459667914407, 54.33094751244893672 ) ) ;
#4006=AXIS2_PLACEMENT_3D ( 'NONE', #62057, #27544, #85664 ) ;
#4007=CARTESIAN_POINT ( 'NONE',  ( 135.5068622967207830, -16.38644903112292894, 7.895285856717910278 ) ) ;
#4009=CYLINDRICAL_SURFACE ( 'NONE', #78061, 2.750000000000002665 ) ;
#4011=ORIENTED_EDGE ( 'NONE', *, *, #16740, .F. ) ;
#4012=LINE ( 'NONE', #59851, #114 ) ;
#4014=VERTEX_POINT ( 'NONE', #38537 ) ;
#4015=CARTESIAN_POINT ( 'NONE',  ( 97.54218415029114908, -32.48978251111615378, 100.9927681330539713 ) ) ;
#4016=ORIENTED_EDGE ( 'NONE', *, *, #35881, .T. ) ;
#4017=CARTESIAN_POINT ( 'NONE',  ( 100.6982016950751699, -42.46504578929962292, 56.33241982807696502 ) ) ;
#4018=CARTESIAN_POINT ( 'NONE',  ( 142.8687636814962616, 5.654319119531167281, 361.9756252759100335 ) ) ;
#4019=CARTESIAN_POINT ( 'NONE',  ( 99.62013013265574557, -29.94545647671011679, 77.17015473446797102 ) ) ;
#4020=CARTESIAN_POINT ( 'NONE',  ( 123.6837132603319418, -53.34645651782485487, 239.5838068554170377 ) ) ;
#4022=VECTOR ( 'NONE', #18685, 1000.000000000000000 ) ;
#4024=CARTESIAN_POINT ( 'NONE',  ( 110.5624684038761814, -46.61161715960605534, 33.84705384733993583 ) ) ;
#4025=CYLINDRICAL_SURFACE ( 'NONE', #58292, 0.4999999999999933387 ) ;
#4028=CIRCLE ( 'NONE', #56198, 2.117000000000007987 ) ;
#4029=ORIENTED_EDGE ( 'NONE', *, *, #80806, .F. ) ;
#4031=EDGE_CURVE ( 'NONE', #78275, #57034, #51709, .T. ) ;
#4036=AXIS2_PLACEMENT_3D ( 'NONE', #47451, #20670, #82910 ) ;
#4037=ORIENTED_EDGE ( 'NONE', *, *, #51338, .F. ) ;
#4038=CARTESIAN_POINT ( 'NONE',  ( 116.5994914424366016, -40.81117973626242446, 213.5165776568640013 ) ) ;
#4039=CARTESIAN_POINT ( 'NONE',  ( 98.47266077831692144, -31.55723625645210362, 125.8945218809075470 ) ) ;
#4040=FACE_OUTER_BOUND ( 'NONE', #569, .T. ) ;
#4041=CARTESIAN_POINT ( 'NONE',  ( 112.8177273059790764, -27.29031728650405597, 45.62895860924398761 ) ) ;
#4042=CARTESIAN_POINT ( 'NONE',  ( 143.0664832912740110, -8.729447159940999512, -5.074374724088000832 ) ) ;
#4043=ORIENTED_EDGE ( 'NONE', *, *, #87102, .T. ) ;
#4044=FACE_OUTER_BOUND ( 'NONE', #20744, .T. ) ;
#4047=AXIS2_PLACEMENT_3D ( 'NONE', #28872, #44145, #71886 ) ;
#4050=LINE ( 'NONE', #10863, #30063 ) ;
#4052=CARTESIAN_POINT ( 'NONE',  ( 98.91597900623158068, -29.29754952351876796, 230.7261014663869503 ) ) ;
#4054=EDGE_CURVE ( 'NONE', #8960, #63665, #52584, .T. ) ;
#4055=DIRECTION ( 'NONE',  ( 9.351236661543306751E-17, -3.725950533538267725E-29, -1.000000000000000000 ) ) ;
#4056=CARTESIAN_POINT ( 'NONE',  ( 77.85525873416882803, -38.37463194330737082, 2.472581811079971104 ) ) ;
#4057=CARTESIAN_POINT ( 'NONE',  ( 114.2024335102360908, -32.03537151136463734, 253.7124198280768042 ) ) ;
#4058=DIRECTION ( 'NONE',  ( 1.000000000000000078E-15, -1.000000000000000083E-30, -1.000000000000000000 ) ) ;
#4059=CARTESIAN_POINT ( 'NONE',  ( 104.7644060343265551, -46.87484541886965417, 68.39848241876794077 ) ) ;
#4061=CARTESIAN_POINT ( 'NONE',  ( 97.89382931228060158, -31.60946541130721954, 110.9213395616259703 ) ) ;
#4062=ORIENTED_EDGE ( 'NONE', *, *, #65190, .F. ) ;
#4064=ORIENTED_EDGE ( 'NONE', *, *, #48198, .F. ) ;
#4067=CARTESIAN_POINT ( 'NONE',  ( 19.56648329127303043, -18.82844715994100326, 342.9256252759109884 ) ) ;
#4070=CARTESIAN_POINT ( 'NONE',  ( 97.12558208529860337, -37.99706834861481042, 51.42732375708717996 ) ) ;
#4071=CARTESIAN_POINT ( 'NONE',  ( 97.50197496249766971, -32.47188371672483242, 100.9927681330539713 ) ) ;
#4073=DIRECTION ( 'NONE',  ( 1.000000000000000078E-15, -1.000000000000000083E-30, -1.000000000000000000 ) ) ;
#4074=CARTESIAN_POINT ( 'NONE',  ( 147.9050922409201121, -0.9159188039171800577, 542.9756252759101471 ) ) ;
#4075=VECTOR ( 'NONE', #69517, 1000.000000000000114 ) ;
#4076=DIRECTION ( 'NONE',  ( -1.000000000000000000, -2.756263715554006823E-15, 0.000000000000000000 ) ) ;
#4077=ORIENTED_EDGE ( 'NONE', *, *, #86797, .F. ) ;
#4078=CARTESIAN_POINT ( 'NONE',  ( 108.2792694979413568, -26.31707411447196421, 129.9841967044819739 ) ) ;
#4080=CARTESIAN_POINT ( 'NONE',  ( 168.5667039024480687, -48.82844715993517326, 300.4678068554149490 ) ) ;
#4084=ORIENTED_EDGE ( 'NONE', *, *, #37132, .F. ) ;
#4087=LINE ( 'NONE', #31788, #80241 ) ;
#4088=EDGE_CURVE ( 'NONE', #60868, #9815, #53023, .T. ) ;
#4090=EDGE_CURVE ( 'NONE', #62556, #26370, #60766, .T. ) ;
#4093=CARTESIAN_POINT ( 'NONE',  ( 41.56648329127399677, -18.82844715994099971, 256.8086252759120498 ) ) ;
#4098=CARTESIAN_POINT ( 'NONE',  ( 97.71246005893831921, -41.20616857227587815, 212.6937205140059461 ) ) ;
#4099=CARTESIAN_POINT ( 'NONE',  ( 105.8259002483207922, -25.33766151058717142, 321.6188579224977389 ) ) ;
#4101=VECTOR ( 'NONE', #45439, 1000.000000000000000 ) ;
#4102=CARTESIAN_POINT ( 'NONE',  ( 97.89279369561094768, -33.33727167892453735, 62.04419670448196911 ) ) ;
#4103=CARTESIAN_POINT ( 'NONE',  ( 108.3332121129147225, -46.73488633077575827, 52.67731614845624932 ) ) ;
#4104=CARTESIAN_POINT ( 'NONE',  ( 97.81168895331838087, -40.51742574516882200, 11.63562527591094309 ) ) ;
#4105=VECTOR ( 'NONE', #79320, 1000.000000000000000 ) ;
#4106=CARTESIAN_POINT ( 'NONE',  ( 173.8164832912740110, 12.92155284005802685, 349.2756252759111248 ) ) ;
#4107=ORIENTED_EDGE ( 'NONE', *, *, #65605, .T. ) ;
#4109=VECTOR ( 'NONE', #17206, 1000.000000000000000 ) ;
#4110=AXIS2_PLACEMENT_3D ( 'NONE', #71347, #36370, #58144 ) ;
#4112=EDGE_LOOP ( 'NONE', ( #48740, #73787, #79436, #49787 ) ) ;
#4113=CARTESIAN_POINT ( 'NONE',  ( 100.2828564484647274, -30.98100942051235052, 212.1987261630399360 ) ) ;
#4114=CARTESIAN_POINT ( 'NONE',  ( 105.7167024970128608, -46.72405552150465269, 53.46869760484980816 ) ) ;
#4118=AXIS2_PLACEMENT_3D ( 'NONE', #12771, #68181, #83166 ) ;
#4119=DIRECTION ( 'NONE',  ( 0.000000000000000000, 0.000000000000000000, -1.000000000000000000 ) ) ;
#4121=DIRECTION ( 'NONE',  ( 1.000000000000000000, 2.999999999999999839E-15, 1.000000000000000078E-15 ) ) ;
#4124=CARTESIAN_POINT ( 'NONE',  ( 96.68905559037375497, -32.92312794843576995, 21.03467289495897319 ) ) ;
#4127=CARTESIAN_POINT ( 'NONE',  ( 99.04406185070456559, -42.84125762965616957, 81.84395860822249347 ) ) ;
#4128=DIRECTION ( 'NONE',  ( 0.7071067811865758834, -0.7071067811865192621, 7.071067811865765240E-16 ) ) ;
#4129=CARTESIAN_POINT ( 'NONE',  ( 83.73314995793998605, 12.92155284005730387, 355.9756252759109998 ) ) ;
#4131=VECTOR ( 'NONE', #28596, 1000.000000000000114 ) ;
#4133=CARTESIAN_POINT ( 'NONE',  ( 98.50201126197670476, -30.70924794336980668, 201.8384824187679385 ) ) ;
#4135=VERTEX_POINT ( 'NONE', #88501 ) ;
#4136=CARTESIAN_POINT ( 'NONE',  ( 115.2006710226633004, -43.31943727361606733, 84.28419670448195689 ) ) ;
#4138=DIRECTION ( 'NONE',  ( 1.000000000000000078E-15, -1.000000000000000083E-30, -1.000000000000000000 ) ) ;
#4141=EDGE_CURVE ( 'NONE', #52360, #19111, #12186, .T. ) ;
#4143=ADVANCED_FACE ( 'NONE', ( #5369 ), #33516, .F. ) ;
#4144=CARTESIAN_POINT ( 'NONE',  ( 78.49243656059439900, -38.98954602991467056, 7.829737348688145637 ) ) ;
#4145=CARTESIAN_POINT ( 'NONE',  ( 141.0664832912740110, -8.729447159940995959, -4.824374724088991151 ) ) ;
#4146=CARTESIAN_POINT ( 'NONE',  ( 112.0636451658066193, -45.48965997882522316, 152.9902778487048636 ) ) ;
#4147=CARTESIAN_POINT ( 'NONE',  ( 110.7682021097048306, -28.22102727396991284, 132.5680903695919710 ) ) ;
#4148=CARTESIAN_POINT ( 'NONE',  ( 110.2625522973084600, -26.74624433126517076, 230.8299109901969643 ) ) ;
#4149=EDGE_CURVE ( 'NONE', #45090, #23101, #11262, .T. ) ;
#4152=VECTOR ( 'NONE', #34784, 1000.000000000000000 ) ;
#4153=EDGE_CURVE ( 'NONE', #35419, #51043, #47124, .T. ) ;
#4154=CARTESIAN_POINT ( 'NONE',  ( 135.2499137886250935, -39.21189172703900994, 1.845048092479758095 ) ) ;
#4156=VERTEX_POINT ( 'NONE', #40321 ) ;
#4158=AXIS2_PLACEMENT_3D ( 'NONE', #33701, #54554, #69120 ) ;
#4159=ADVANCED_FACE ( 'NONE', ( #70277 ), #56177, .F. ) ;
#4161=EDGE_LOOP ( 'NONE', ( #16368, #78238, #47634, #25917 ) ) ;
#4162=ORIENTED_EDGE ( 'NONE', *, *, #87447, .F. ) ;
#4163=DIRECTION ( 'NONE',  ( 0.7071067811865784369, -0.7071067811865165975, 7.071067811865480264E-16 ) ) ;
#4164=DIRECTION ( 'NONE',  ( 0.7071067811865431318, -0.7071067811865517916, 7.071067811865425043E-16 ) ) ;
#4165=EDGE_CURVE ( 'NONE', #1484, #54987, #83927, .T. ) ;
#4166=LINE ( 'NONE', #59110, #4022 ) ;
#4167=CARTESIAN_POINT ( 'NONE',  ( 105.6324958909751075, -46.33196107771311745, 146.8809912566479738 ) ) ;
#4168=CARTESIAN_POINT ( 'NONE',  ( 97.06250871634010480, -39.81605817309107920, 21.56419670448195092 ) ) ;
#4169=ORIENTED_EDGE ( 'NONE', *, *, #2189, .T. ) ;
#4170=AXIS2_PLACEMENT_3D ( 'NONE', #13419, #41103, #42887 ) ;
#4171=EDGE_CURVE ( 'NONE', #43699, #82504, #79437, .T. ) ;
#4175=VECTOR ( 'NONE', #18293, 1000.000000000000000 ) ;
#4176=LINE ( 'NONE', #52725, #54794 ) ;
#4178=CARTESIAN_POINT ( 'NONE',  ( 97.74156636318205926, -40.34206866484610288, 167.6208556024714653 ) ) ;
#4180=FACE_OUTER_BOUND ( 'NONE', #6599, .T. ) ;
#4181=CARTESIAN_POINT ( 'NONE',  ( 97.81556180715350024, -40.52687500387260400, 131.6364377373729440 ) ) ;
#4182=LINE ( 'NONE', #45048, #56706 ) ;
#4183=ORIENTED_EDGE ( 'NONE', *, *, #13488, .T. ) ;
#4184=CARTESIAN_POINT ( 'NONE',  ( 101.5973605122076862, -47.27098594307553725, 17.19562527591095247 ) ) ;
#4185=CARTESIAN_POINT ( 'NONE',  ( 115.9822161205003397, -42.21601869724081268, 14.38705384733995984 ) ) ;
#4186=FACE_OUTER_BOUND ( 'NONE', #25960, .T. ) ;
#4188=CARTESIAN_POINT ( 'NONE',  ( 112.1393585966182656, -28.01283025110964786, 145.6568144398399340 ) ) ;
#4189=DIRECTION ( 'NONE',  ( -1.000000000000000000, -4.299999999999999979E-14, -1.000000000000000078E-15 ) ) ;
#4190=LINE ( 'NONE', #60937, #70232 ) ;
#4192=EDGE_CURVE ( 'NONE', #61394, #71543, #77107, .T. ) ;
#4193=CARTESIAN_POINT ( 'NONE',  ( 113.2454986892643802, -28.75867293750068043, 10.55229194345644039 ) ) ;
#4195=EDGE_CURVE ( 'NONE', #27163, #62031, #66364, .T. ) ;
#4197=CARTESIAN_POINT ( 'NONE',  ( 96.88405369895032493, -39.16353706000892032, 56.51276813305394597 ) ) ;
#4198=CARTESIAN_POINT ( 'NONE',  ( 101.2007021600770855, -45.34774740814643934, 193.1013395616249682 ) ) ;
#4199=CARTESIAN_POINT ( 'NONE',  ( 99.96594057013267332, -44.39231554709003547, 42.98133956162492098 ) ) ;
#4200=ADVANCED_FACE ( 'NONE', ( #89847 ), #13527, .T. ) ;
#4202=CARTESIAN_POINT ( 'NONE',  ( 151.0371591254573787, -24.95799193692592866, 249.9678068554149490 ) ) ;
#4203=DIRECTION ( 'NONE',  ( 0.000000000000000000, 1.000000000000000000, 0.000000000000000000 ) ) ;
#4204=AXIS2_PLACEMENT_3D ( 'NONE', #83664, #90, #27340 ) ;
#4206=CARTESIAN_POINT ( 'NONE',  ( 172.5664832912740110, -32.07844715994070839, 258.9256252759120116 ) ) ;
#4208=CARTESIAN_POINT ( 'NONE',  ( 107.8912859324307192, -26.39220933555703752, 111.0251490854339806 ) ) ;
#4212=CARTESIAN_POINT ( 'NONE',  ( 110.8089421659425540, -26.35361831834165969, 245.7889586092439629 ) ) ;
#4213=CARTESIAN_POINT ( 'NONE',  ( 163.0664832912739826, 12.92155284005902516, 336.6506252759110112 ) ) ;
#4214=PLANE ( 'NONE',  #89922 ) ;
#4215=DIRECTION ( 'NONE',  ( 1.000000000000000078E-15, 0.000000000000000000, 1.000000000000000000 ) ) ;
#4216=CARTESIAN_POINT ( 'NONE',  ( 116.1804594027163517, -40.96476762480074996, 9.425625275910979539 ) ) ;
#4217=VECTOR ( 'NONE', #69205, 1000.000000000000000 ) ;
#4220=CARTESIAN_POINT ( 'NONE',  ( 103.2204921605863888, -27.09891563476508836, 175.3908633711489813 ) ) ;
#4221=ORIENTED_EDGE ( 'NONE', *, *, #34620, .F. ) ;
#4223=AXIS2_PLACEMENT_3D ( 'NONE', #40840, #62186, #20423 ) ;
#4224=CARTESIAN_POINT ( 'NONE',  ( 103.2343105203340201, -28.73928255177903068, 91.86444044875396742 ) ) ;
#4225=DIRECTION ( 'NONE',  ( -0.7071067811865784369, 0.7071067811865165975, -7.071067811865480264E-16 ) ) ;
#4226=CARTESIAN_POINT ( 'NONE',  ( 110.8764511561472119, -27.72125199330416478, 240.7584824187679544 ) ) ;
#4228=DIRECTION ( 'NONE',  ( 1.000000000000000078E-15, 0.000000000000000000, -1.000000000000000000 ) ) ;
#4229=LINE ( 'NONE', #83118, #49579 ) ;
#4233=DIRECTION ( 'NONE',  ( 1.639958061481212836E-42, -4.100000000000000342E-29, -1.000000000000000000 ) ) ;
#4234=CARTESIAN_POINT ( 'NONE',  ( 31.56670390244800828, -33.35206098992711077, 237.4678068554150059 ) ) ;
#4235=AXIS2_PLACEMENT_3D ( 'NONE', #11559, #63500, #66051 ) ;
#4236=CARTESIAN_POINT ( 'NONE',  ( 110.6887065042383256, -47.98678726807249006, 207.8241967044819489 ) ) ;
#4237=EDGE_LOOP ( 'NONE', ( #60350, #14798 ) ) ;
#4240=CARTESIAN_POINT ( 'NONE',  ( 108.4174892996514075, -26.73503593485758145, 150.9689586054618360 ) ) ;
#4241=VECTOR ( 'NONE', #29666, 1000.000000000000000 ) ;
#4244=ORIENTED_EDGE ( 'NONE', *, *, #4944, .F. ) ;
#4245=CARTESIAN_POINT ( 'NONE',  ( 99.04404884010753563, -42.84124075760115602, 267.8439569258346751 ) ) ;
#4246=EDGE_CURVE ( 'NONE', #43807, #18476, #3283, .T. ) ;
#4247=CARTESIAN_POINT ( 'NONE',  ( 109.3585227812971539, -25.91623105973918939, 184.9222919425779708 ) ) ;
#4248=EDGE_CURVE ( 'NONE', #29169, #86897, #7611, .T. ) ;
#4250=ORIENTED_EDGE ( 'NONE', *, *, #78426, .T. ) ;
#4251=ORIENTED_EDGE ( 'NONE', *, *, #30489, .F. ) ;
#4253=AXIS2_PLACEMENT_3D ( 'NONE', #41794, #20931, #49057 ) ;
#4256=CARTESIAN_POINT ( 'NONE',  ( 188.5667039024479834, -67.87844715994100397, 173.2178068554149775 ) ) ;
#4257=CARTESIAN_POINT ( 'NONE',  ( 97.81555538561684671, -40.52686194202485837, 166.6364365798628171 ) ) ;
#4258=CARTESIAN_POINT ( 'NONE',  ( 115.2261106523039444, -36.95351711827176899, 41.62237608387797394 ) ) ;
#4259=EDGE_CURVE ( 'NONE', #83807, #51539, #49605, .T. ) ;
#4260=DIRECTION ( 'NONE',  ( 0.7071067811571474238, 0.7071067812159476107, 0.000000000000000000 ) ) ;
#4263=CIRCLE ( 'NONE', #15885, 2.500000000000002220 ) ;
#4264=DIRECTION ( 'NONE',  ( -0.04216478779797398074, 0.9991106698809455455, 1.084202172485504434E-19 ) ) ;
#4265=EDGE_LOOP ( 'NONE', ( #76368, #16996, #77568, #21622 ) ) ;
#4266=EDGE_LOOP ( 'NONE', ( #24443, #28092, #88300, #78688 ) ) ;
#4267=ADVANCED_FACE ( 'NONE', ( #64810 ), #23048, .F. ) ;
#4269=EDGE_LOOP ( 'NONE', ( #55960, #32869, #57323, #66768 ) ) ;
#4270=EDGE_LOOP ( 'NONE', ( #6902, #9144, #40909, #60507, #65679 ) ) ;
#4273=CARTESIAN_POINT ( 'NONE',  ( 102.0495883242188171, -29.81664044981240025, 74.99813411379096806 ) ) ;
#4274=CARTESIAN_POINT ( 'NONE',  ( 108.1841437630847338, -47.11680481413669952, 202.6613395616249704 ) ) ;
#4276=CARTESIAN_POINT ( 'NONE',  ( 113.6717327907684165, -45.56316108038149082, 188.0994347997199725 ) ) ;
#4277=LINE ( 'NONE', #33320, #46100 ) ;
#4278=CARTESIAN_POINT ( 'NONE',  ( 118.1029919389229406, -36.12161712796727642, 269.8822919425776945 ) ) ;
#4283=VECTOR ( 'NONE', #60707, 999.9999999999998863 ) ;
#4285=ADVANCED_FACE ( 'NONE', ( #3474 ), #15774, .T. ) ;
#4289=CARTESIAN_POINT ( 'NONE',  ( 99.05215007911658631, -29.93811023049936892, 215.7670538473399517 ) ) ;
#4291=CARTESIAN_POINT ( 'NONE',  ( 103.6385507868184277, -26.22095696399066966, 210.3394347997209763 ) ) ;
#4292=DIRECTION ( 'NONE',  ( 1.000000000000000078E-15, 0.000000000000000000, -1.000000000000000000 ) ) ;
#4296=CARTESIAN_POINT ( 'NONE',  ( 97.86360378202594745, -40.49644234972143408, 277.6356252759112522 ) ) ;
#4298=CARTESIAN_POINT ( 'NONE',  ( 96.58568816239609589, -40.17018292043292860, 282.5908633711490552 ) ) ;
#4306=CARTESIAN_POINT ( 'NONE',  ( 97.81168883536605563, -40.51740680051663190, 96.63562987897269352 ) ) ;
#4308=DIRECTION ( 'NONE',  ( 1.000000000000000078E-15, 0.000000000000000000, -1.000000000000000000 ) ) ;
#4309=VERTEX_POINT ( 'NONE', #31165 ) ;
#4310=CARTESIAN_POINT ( 'NONE',  ( 194.5667039024479834, -67.87844715994100397, 20.91780685541479912 ) ) ;
#4311=CARTESIAN_POINT ( 'NONE',  ( 106.9748012750099946, -47.17635858745483546, 187.5699109901969734 ) ) ;
#4312=CARTESIAN_POINT ( 'NONE',  ( 113.9169062821921727, -28.05502007051373070, 120.5565776568639507 ) ) ;
#4313=CARTESIAN_POINT ( 'NONE',  ( 104.1737878132142043, -26.63141132829087354, 221.2984824187679465 ) ) ;
#4316=CARTESIAN_POINT ( 'NONE',  ( 37.06648329127298780, 12.92155284005730387, 355.9756252759109998 ) ) ;
#4319=CARTESIAN_POINT ( 'NONE',  ( 107.0664832912739968, -36.72944715994100306, 287.6356252759109680 ) ) ;
#4320=CARTESIAN_POINT ( 'NONE',  ( 150.5667039024473297, -25.42844715993594562, 300.4678068554149490 ) ) ;
#4321=CARTESIAN_POINT ( 'NONE',  ( 131.4004675426834865, -19.42701295172721387, 2.979899338979302037 ) ) ;
#4325=AXIS2_PLACEMENT_3D ( 'NONE', #31197, #60237, #38904 ) ;
#4326=CARTESIAN_POINT ( 'NONE',  ( 97.58007606596183336, -34.66094392094686327, 105.5781341137909664 ) ) ;
#4329=CARTESIAN_POINT ( 'NONE',  ( 105.3199149336540046, -48.42511963160323774, 143.4584824187689662 ) ) ;
#4331=DIRECTION ( 'NONE',  ( 9.351236661543306751E-17, -3.725950533538267725E-29, -1.000000000000000000 ) ) ;
#4332=EDGE_CURVE ( 'NONE', #26394, #5757, #44344, .T. ) ;
#4334=CARTESIAN_POINT ( 'NONE',  ( 116.3212776292293569, -32.94146857471253753, 110.1356252759109822 ) ) ;
#4335=CARTESIAN_POINT ( 'NONE',  ( 112.4622727538958884, -27.87370092883236694, 49.62895860924398761 ) ) ;
#4336=ORIENTED_EDGE ( 'NONE', *, *, #74635, .T. ) ;
#4339=EDGE_LOOP ( 'NONE', ( #37405, #61513 ) ) ;
#4342=CARTESIAN_POINT ( 'NONE',  ( 98.40655050692429029, -32.18313002855528993, 131.9413395616250000 ) ) ;
#4343=DIRECTION ( 'NONE',  ( 0.000000000000000000, 1.000000000000000000, 0.000000000000000000 ) ) ;
#4344=CARTESIAN_POINT ( 'NONE',  ( 182.4202572930400095, -33.70561438051981185, -5.074374724088000832 ) ) ;
#4345=CARTESIAN_POINT ( 'NONE',  ( 33.78309357195740859, -29.99615139352333060, 193.9678068554150911 ) ) ;
#4346=DIRECTION ( 'NONE',  ( 2.900000000000000265E-14, -2.000000000000000155E-15, 1.000000000000000000 ) ) ;
#4349=DIRECTION ( 'NONE',  ( -1.000000000000000000, -1.000000000000000078E-15, -1.000000000000000078E-15 ) ) ;
#4350=CARTESIAN_POINT ( 'NONE',  ( 96.73636544059188225, -37.96124694896867169, 41.42133956162496844 ) ) ;
#4352=ORIENTED_EDGE ( 'NONE', *, *, #69221, .T. ) ;
#4353=CIRCLE ( 'NONE', #30423, 4.750000000000004441 ) ;
#4356=PLANE ( 'NONE',  #322 ) ;
#4357=CARTESIAN_POINT ( 'NONE',  ( 115.0306645585770298, -38.52089976383655312, 146.4680903695919767 ) ) ;
#4361=CARTESIAN_POINT ( 'NONE',  ( 87.17003668186721654, -54.68655584847608964, -5.074374724089126154 ) ) ;
#4362=ORIENTED_EDGE ( 'NONE', *, *, #88052, .F. ) ;
#4364=CIRCLE ( 'NONE', #88475, 0.3000000000000062617 ) ;
#4371=CARTESIAN_POINT ( 'NONE',  ( 104.2245914675057321, -27.77399204033938318, 201.7406309249449521 ) ) ;
#4374=AXIS2_PLACEMENT_3D ( 'NONE', #33557, #87196, #52627 ) ;
#4378=ORIENTED_EDGE ( 'NONE', *, *, #71601, .T. ) ;
#4382=EDGE_CURVE ( 'NONE', #77354, #40177, #81552, .T. ) ;
#4383=CARTESIAN_POINT ( 'NONE',  ( 104.3071780974205183, -29.01783752938878180, 188.1680903695909706 ) ) ;
#4384=CARTESIAN_POINT ( 'NONE',  ( 110.1645224859485808, -46.70684747839494833, 97.81562527591097478 ) ) ;
#4385=CARTESIAN_POINT ( 'NONE',  ( 108.9812119692459049, -46.95502683147942236, 82.72419670448194040 ) ) ;
#4386=CARTESIAN_POINT ( 'NONE',  ( 104.4065072340926577, -46.45762169397040964, 252.3649774052962300 ) ) ;
#4388=LINE ( 'NONE', #3484, #79459 ) ;
#4389=CARTESIAN_POINT ( 'NONE',  ( 117.8006386470660658, -34.09280371250640940, 160.0061014663869798 ) ) ;
#4391=VERTEX_POINT ( 'NONE', #67035 ) ;
#4392=DIRECTION ( 'NONE',  ( 0.000000000000000000, 1.000000000000000000, 0.000000000000000000 ) ) ;
#4393=VERTEX_POINT ( 'NONE', #80679 ) ;
#4394=EDGE_LOOP ( 'NONE', ( #9420, #41528, #9038, #63812, #54045 ) ) ;
#4395=DIRECTION ( 'NONE',  ( 1.000000000000000078E-15, 0.000000000000000000, -1.000000000000000000 ) ) ;
#4397=AXIS2_PLACEMENT_3D ( 'NONE', #18884, #77203, #891 ) ;
#4401=CARTESIAN_POINT ( 'NONE',  ( 111.8884855208196569, -27.93222315804501932, 130.6774218487876453 ) ) ;
#4402=CARTESIAN_POINT ( 'NONE',  ( 107.6031522308233974, -26.28253885536559764, 95.03562527591097364 ) ) ;
#4403=CARTESIAN_POINT ( 'NONE',  ( 103.7793689006360580, -43.80298085837112154, 0.4256252759109674932 ) ) ;
#4404=B_SPLINE_CURVE_WITH_KNOTS ( 'NONE', 3,
 ( #4877, #17175, #31227, #44858, #38057, #32568, #59818, #58922, #45295, #25759, #73015, #73457, #10784, #59375, #38487, #66187, #52541, #3096 ),
 .UNSPECIFIED., .F., .F.,
 ( 4, 2, 2, 2, 2, 2, 2, 2, 4 ),
 ( 0.4999999996252184609, 0.5624999996720660977, 0.6249999997189138456, 0.6874999997657615936, 0.7499999998126092304, 0.8124999998594568673, 0.8749999999063046152, 0.9374999999531523631, 1.000000000000000000 ),
 .UNSPECIFIED. ) ;
#4405=CARTESIAN_POINT ( 'NONE',  ( 132.3254539024480323, -42.97311385573998876, 207.5838068554170377 ) ) ;
#4407=CARTESIAN_POINT ( 'NONE',  ( 97.87212830949604836, -31.93334231290197067, 90.93181575210196854 ) ) ;
#4408=CARTESIAN_POINT ( 'NONE',  ( 89.06648138392553449, -56.72944715994104570, -4.824374724089047106 ) ) ;
#4409=CARTESIAN_POINT ( 'NONE',  ( 113.6005200848514107, -45.61596423689125146, 179.0689586092439640 ) ) ;
#4410=LINE ( 'NONE', #86190, #87171 ) ;
#4411=CARTESIAN_POINT ( 'NONE',  ( 51.27381068362094396, -23.19206098993945275, 342.9256252759109884 ) ) ;
#4412=ORIENTED_EDGE ( 'NONE', *, *, #30964, .F. ) ;
#4413=CARTESIAN_POINT ( 'NONE',  ( 51.06670390244799762, -33.35206098992630075, -5.074374724088000832 ) ) ;
#4414=CIRCLE ( 'NONE', #65297, 29.00000000000000000 ) ;
#4415=B_SPLINE_CURVE_WITH_KNOTS ( 'NONE', 3,
 ( #19740, #33815, #75610, #73809, #88798, #52865, #47424, #61065, #4772, #18847, #46968, #75151, #54673, #25203, #53781, #74263, #39284, #32456 ),
 .UNSPECIFIED., .F., .F.,
 ( 4, 2, 2, 2, 2, 2, 2, 2, 4 ),
 ( 0.000000000000000000, 0.06249238482208734763, 0.1249847696441746953, 0.1874771544662620359, 0.2499695392883493905, 0.3124619241104367173, 0.3749543089325240719, 0.4374466937546114265, 0.4999390785766987810 ),
 .UNSPECIFIED. ) ;
#4416=DIRECTION ( 'NONE',  ( -1.000000000000000000, 6.036837696399408848E-13, 0.000000000000000000 ) ) ;
#4417=AXIS2_PLACEMENT_3D ( 'NONE', #29238, #57367, #1976 ) ;
#4419=CARTESIAN_POINT ( 'NONE',  ( 103.2876017065440664, -26.96590681778891252, 215.3699109901969848 ) ) ;
#4421=DIRECTION ( 'NONE',  ( 9.912705577010326536E-16, 1.000000000000000000, 0.000000000000000000 ) ) ;
#4422=CARTESIAN_POINT ( 'NONE',  ( 96.54178838847580835, -40.18459672615917100, 282.5908633711491120 ) ) ;
#4423=CARTESIAN_POINT ( 'NONE',  ( 114.8035609388329021, -44.68778416175712920, 114.2022919425779719 ) ) ;
#4424=CARTESIAN_POINT ( 'NONE',  ( 172.5667039024480687, -42.82844715993500273, 300.4678068554149490 ) ) ;
#4425=EDGE_CURVE ( 'NONE', #29546, #38331, #73848, .T. ) ;
#4429=ORIENTED_EDGE ( 'NONE', *, *, #69265, .T. ) ;
#4431=ORIENTED_EDGE ( 'NONE', *, *, #31694, .F. ) ;
#4432=ORIENTED_EDGE ( 'NONE', *, *, #58954, .T. ) ;
#4433=ORIENTED_EDGE ( 'NONE', *, *, #63334, .F. ) ;
#4434=LINE ( 'NONE', #80740, #50896 ) ;
#4435=CARTESIAN_POINT ( 'NONE',  ( 105.0216744116726630, -25.86700170375123520, 276.2365776568634033 ) ) ;
#4436=LINE ( 'NONE', #76035, #20054 ) ;
#4438=DIRECTION ( 'NONE',  ( -4.299999999999999979E-14, 1.000000000000000000, -4.400000000000000367E-29 ) ) ;
#4440=CARTESIAN_POINT ( 'NONE',  ( 104.2579841207466984, -28.11985932224000351, 209.7619436376009787 ) ) ;
#4441=ORIENTED_EDGE ( 'NONE', *, *, #23065, .F. ) ;
#4444=EDGE_CURVE ( 'NONE', #2908, #18234, #5259, .T. ) ;
#4446=B_SPLINE_CURVE_WITH_KNOTS ( 'NONE', 3,
 ( #23982, #71246, #85775, #29902, #29450, #51656, #2649, #58473, #64416, #23107, #36717, #57130, #42599, #8562, #30347, #15383, #70335, #71685 ),
 .UNSPECIFIED., .F., .F.,
 ( 4, 2, 2, 2, 2, 2, 2, 2, 4 ),
 ( 0.5000275190869877262, 0.5625240792011142466, 0.6250206393152407669, 0.6875171994293673983, 0.7500137595434939186, 0.8125103196576204390, 0.8750068797717469593, 0.9375034398858734797, 1.000000000000000000 ),
 .UNSPECIFIED. ) ;
#4448=DIRECTION ( 'NONE',  ( 0.000000000000000000, 0.000000000000000000, 1.000000000000000000 ) ) ;
#4449=CARTESIAN_POINT ( 'NONE',  ( 114.6135591410776016, -41.37377328621888495, 14.81872616303997425 ) ) ;
#4452=CIRCLE ( 'NONE', #18971, 2.750000000000002665 ) ;
#4453=DIRECTION ( 'NONE',  ( 0.000000000000000000, 0.000000000000000000, 1.000000000000000000 ) ) ;
#4454=CARTESIAN_POINT ( 'NONE',  ( 109.7813264909552515, -47.51098736074730766, 242.7727681330539724 ) ) ;
#4456=VERTEX_POINT ( 'NONE', #74308 ) ;
#4457=DIRECTION ( 'NONE',  ( -0.7071067811865692221, -0.7071067811865259234, -7.071067811865685367E-16 ) ) ;
#4458=AXIS2_PLACEMENT_3D ( 'NONE', #38524, #25342, #5361 ) ;
#4459=PLANE ( 'NONE',  #6046 ) ;
#4460=CARTESIAN_POINT ( 'NONE',  ( 100.9805754248354788, -42.21072563198327998, 54.72809036959092310 ) ) ;
#4461=CARTESIAN_POINT ( 'NONE',  ( 136.5173892390865831, -17.48112160758304867, 7.135585143028393418 ) ) ;
#4462=CARTESIAN_POINT ( 'NONE',  ( 182.2420472961719895, -31.76306994223730840, -5.074374724088000832 ) ) ;
#4465=ORIENTED_EDGE ( 'NONE', *, *, #80244, .T. ) ;
#4467=DIRECTION ( 'NONE',  ( -1.000000000000000000, -4.299999999999999979E-14, -1.000000000000000078E-15 ) ) ;
#4468=EDGE_CURVE ( 'NONE', #87925, #48525, #81139, .T. ) ;
#4469=ORIENTED_EDGE ( 'NONE', *, *, #25900, .F. ) ;
#4470=CARTESIAN_POINT ( 'NONE',  ( 101.7558625676976618, -27.03530485730228250, 100.4632443235299633 ) ) ;
#4471=ORIENTED_EDGE ( 'NONE', *, *, #81841, .T. ) ;
#4472=ADVANCED_FACE ( 'NONE', ( #18432 ), #25697, .T. ) ;
#4473=CARTESIAN_POINT ( 'NONE',  ( 115.2492312947614437, -32.84933048162275071, 63.61337220902895950 ) ) ;
#4474=VECTOR ( 'NONE', #75714, 1000.000000000000000 ) ;
#4475=CARTESIAN_POINT ( 'NONE',  ( 116.8171228655006075, -34.15291831812996293, 70.03145860946138157 ) ) ;
#4476=CARTESIAN_POINT ( 'NONE',  ( 116.3507336416864746, -38.17139756410392692, 65.12348806780198629 ) ) ;
#4480=CARTESIAN_POINT ( 'NONE',  ( 118.0985323217624057, -37.71894194680212564, 29.74324432352998215 ) ) ;
#4481=VECTOR ( 'NONE', #89437, 1000.000000000000000 ) ;
#4482=CARTESIAN_POINT ( 'NONE',  ( 130.5667039024481255, -40.02944715994100022, 239.5838068554162987 ) ) ;
#4484=DIRECTION ( 'NONE',  ( -4.093947403305260305E-16, 1.000000000000000000, -6.162975822039159109E-32 ) ) ;
#4485=ORIENTED_EDGE ( 'NONE', *, *, #24366, .F. ) ;
#4486=CARTESIAN_POINT ( 'NONE',  ( 77.71552635665730691, -20.16021090639628710, 2.608895778936489940 ) ) ;
#4487=ORIENTED_EDGE ( 'NONE', *, *, #59743, .F. ) ;
#4488=ORIENTED_EDGE ( 'NONE', *, *, #36368, .F. ) ;
#4490=VECTOR ( 'NONE', #50742, 1000.000000000000000 ) ;
#4493=CARTESIAN_POINT ( 'NONE',  ( 110.0587659310071729, -27.38278898179161658, 234.8299109901969643 ) ) ;
#4494=CARTESIAN_POINT ( 'NONE',  ( 97.80136889829883273, -40.49211973435467371, 126.6329963442747442 ) ) ;
#4495=CARTESIAN_POINT ( 'NONE',  ( 98.30753412580686756, -41.72887537901419108, 187.7397919323684334 ) ) ;
#4496=CARTESIAN_POINT ( 'NONE',  ( 116.2315886754559386, -31.76121500512346074, 65.22133956162595325 ) ) ;
#4500=CARTESIAN_POINT ( 'NONE',  ( 109.7248998095299868, -27.00080582534542017, 114.8665783998315533 ) ) ;
#4502=EDGE_LOOP ( 'NONE', ( #18058, #89019, #52076, #26220 ) ) ;
#4503=DIRECTION ( 'NONE',  ( -2.900000000000000265E-14, 2.000000000000000155E-15, -1.000000000000000000 ) ) ;
#4504=CARTESIAN_POINT ( 'NONE',  ( 98.30746919718092158, -41.72870820425139726, 112.7403801342047416 ) ) ;
#4505=CARTESIAN_POINT ( 'NONE',  ( 118.0279888096068390, -35.50094427011355691, 233.9032443235299752 ) ) ;
#4507=LINE ( 'NONE', #32196, #82601 ) ;
#4508=CARTESIAN_POINT ( 'NONE',  ( 79.11888855178027313, -39.31186128672827351, 1.764000668897422130 ) ) ;
#4510=CARTESIAN_POINT ( 'NONE',  ( 111.5095219758393483, -44.62071306430618023, 257.4190864947434534 ) ) ;
#4511=CARTESIAN_POINT ( 'NONE',  ( 182.3467384525657167, -29.62846900981657683, 193.9678068554150059 ) ) ;
#4512=CARTESIAN_POINT ( 'NONE',  ( 99.51750086509218818, -43.88776608678588786, 77.92991099019597812 ) ) ;
#4514=CARTESIAN_POINT ( 'NONE',  ( 117.7240352459720043, -39.83258586197658246, 138.5889586092439743 ) ) ;
#4516=CARTESIAN_POINT ( 'NONE',  ( 132.3477924061144222, -20.87777042261643601, 7.743969477060447026 ) ) ;
#4519=CIRCLE ( 'NONE', #53815, 4.750000000000004441 ) ;
#4521=DIRECTION ( 'NONE',  ( 0.000000000000000000, 0.000000000000000000, -1.000000000000000000 ) ) ;
#4524=CARTESIAN_POINT ( 'NONE',  ( 108.9929891821633134, -47.66111943275755181, 122.7032443235299723 ) ) ;
#4525=ORIENTED_EDGE ( 'NONE', *, *, #43523, .F. ) ;
#4526=DIRECTION ( 'NONE',  ( 0.000000000000000000, 1.000000000000000000, 0.000000000000000000 ) ) ;
#4528=ADVANCED_FACE ( 'NONE', ( #3916, #60197 ), #73397, .T. ) ;
#4529=DIRECTION ( 'NONE',  ( 0.000000000000000000, 0.000000000000000000, -1.000000000000000000 ) ) ;
#4530=VERTEX_POINT ( 'NONE', #72952 ) ;
#4531=AXIS2_PLACEMENT_3D ( 'NONE', #49039, #35424, #76772 ) ;
#4532=CARTESIAN_POINT ( 'NONE',  ( 109.0765542020472907, -47.62233732142709641, 127.7337205140059382 ) ) ;
#4535=CARTESIAN_POINT ( 'NONE',  ( 31.89136050872173911, -31.76306994223854119, 117.4678068554150485 ) ) ;
#4536=DIRECTION ( 'NONE',  ( 0.000000000000000000, 0.000000000000000000, 1.000000000000000000 ) ) ;
#4537=ORIENTED_EDGE ( 'NONE', *, *, #34187, .F. ) ;
#4539=CARTESIAN_POINT ( 'NONE',  ( 41.56648329127399677, 0.2215528400590013880, 21.04262527591200183 ) ) ;
#4541=CARTESIAN_POINT ( 'NONE',  ( 63.03715912545825262, -46.82818131006018092, 249.9678068554150343 ) ) ;
#4542=CARTESIAN_POINT ( 'NONE',  ( 112.0659115677942310, -45.48839629263709128, 157.9897919375864603 ) ) ;
#4544=AXIS2_PLACEMENT_3D ( 'NONE', #29708, #2003, #57399 ) ;
#4545=CARTESIAN_POINT ( 'NONE',  ( 104.4897549782674417, -26.97886241702974885, 105.2814749527903615 ) ) ;
#4548=AXIS2_PLACEMENT_3D ( 'NONE', #56114, #28896, #21642 ) ;
#4550=EDGE_CURVE ( 'NONE', #79544, #60263, #66127, .T. ) ;
#4551=DIRECTION ( 'NONE',  ( -1.000000000000000000, 9.376883653928684652E-16, 1.500301384628589584E-15 ) ) ;
#4552=CARTESIAN_POINT ( 'NONE',  ( 111.8874393434637682, -45.23954810143637673, 208.9870538473389558 ) ) ;
#4555=ORIENTED_EDGE ( 'NONE', *, *, #88789, .F. ) ;
#4556=CARTESIAN_POINT ( 'NONE',  ( 115.6651410650258214, -32.06827565682262815, 65.22133956162495849 ) ) ;
#4557=CARTESIAN_POINT ( 'NONE',  ( 117.0519585894030001, -35.94438672013124858, 53.88895366790352881 ) ) ;
#4560=DIRECTION ( 'NONE',  ( 1.000000000000000000, -1.709087168450053042E-15, 0.000000000000000000 ) ) ;
#4561=ADVANCED_FACE ( 'NONE', ( #31612 ), #52477, .T. ) ;
#4562=ORIENTED_EDGE ( 'NONE', *, *, #34291, .F. ) ;
#4563=PLANE ( 'NONE',  #15329 ) ;
#4565=ORIENTED_EDGE ( 'NONE', *, *, #73775, .F. ) ;
#4566=CARTESIAN_POINT ( 'NONE',  ( 98.23953817868523686, -35.94630056370082372, 227.6872975916109567 ) ) ;
#4568=DIRECTION ( 'NONE',  ( 0.000000000000000000, 0.000000000000000000, 1.000000000000000000 ) ) ;
#4570=CARTESIAN_POINT ( 'NONE',  ( 115.7831076496464249, -41.80230954688622091, 154.4064586059346595 ) ) ;
#4571=DIRECTION ( 'NONE',  ( 0.000000000000000000, 0.000000000000000000, -1.000000000000000000 ) ) ;
#4576=ORIENTED_EDGE ( 'NONE', *, *, #69295, .F. ) ;
#4577=CARTESIAN_POINT ( 'NONE',  ( 96.34404753607181249, -39.41381804822120216, 16.53372051400597798 ) ) ;
#4579=EDGE_CURVE ( 'NONE', #82504, #43699, #67548, .T. ) ;
#4581=CARTESIAN_POINT ( 'NONE',  ( 106.8863607564096725, -44.89016293055450291, 270.3766617981627860 ) ) ;
#4582=CARTESIAN_POINT ( 'NONE',  ( 31.56670390244800828, -33.35206098992711077, 342.9256252759119548 ) ) ;
#4584=CARTESIAN_POINT ( 'NONE',  ( 20.03715912545739997, -46.82818131006202123, 129.9678068554150627 ) ) ;
#4585=DIRECTION ( 'NONE',  ( -0.7071067811578587436, 0.7071067812152364018, 0.000000000000000000 ) ) ;
#4587=CARTESIAN_POINT ( 'NONE',  ( 117.2394727393827765, -34.25896837304814113, 205.0156252759109634 ) ) ;
#4591=CARTESIAN_POINT ( 'NONE',  ( 106.8402480490632342, -48.62734320582506342, 73.56133956162497611 ) ) ;
#4592=CARTESIAN_POINT ( 'NONE',  ( 32.25690895537100289, -33.54226604285010893, -5.074374724088000832 ) ) ;
#4593=ORIENTED_EDGE ( 'NONE', *, *, #1423, .F. ) ;
#4594=ORIENTED_EDGE ( 'NONE', *, *, #37798, .F. ) ;
#4595=EDGE_LOOP ( 'NONE', ( #78765, #27282, #59296, #21833 ) ) ;
#4596=ADVANCED_FACE ( 'NONE', ( #31457 ), #57834, .T. ) ;
#4598=DIRECTION ( 'NONE',  ( 0.000000000000000000, 1.000000000000000000, 0.000000000000000000 ) ) ;
#4599=EDGE_CURVE ( 'NONE', #70197, #22586, #3768, .T. ) ;
#4600=CYLINDRICAL_SURFACE ( 'NONE', #42180, 2.116999999999980009 ) ;
#4601=CARTESIAN_POINT ( 'NONE',  ( 103.3362113047044772, -29.43782462767379116, 118.2709475124489842 ) ) ;
#4602=CARTESIAN_POINT ( 'NONE',  ( 97.14909927861904748, -40.01315743934404878, 237.5813395616249579 ) ) ;
#4603=VECTOR ( 'NONE', #73253, 1000.000000000000000 ) ;
#4605=ORIENTED_EDGE ( 'NONE', *, *, #46308, .F. ) ;
#4606=FACE_OUTER_BOUND ( 'NONE', #12495, .T. ) ;
#4607=ORIENTED_EDGE ( 'NONE', *, *, #23186, .F. ) ;
#4608=AXIS2_PLACEMENT_3D ( 'NONE', #71908, #72353, #9666 ) ;
#4610=CARTESIAN_POINT ( 'NONE',  ( 107.0664832912739541, -36.72944715994095333, 305.7008218191032256 ) ) ;
#4612=VERTEX_POINT ( 'NONE', #86890 ) ;
#4613=CARTESIAN_POINT ( 'NONE',  ( 20.03715912545733602, -46.82818131006202123, 193.9678068554150627 ) ) ;
#4614=DIRECTION ( 'NONE',  ( 0.7071067811865473507, 0.000000000000000000, -0.7071067811865476838 ) ) ;
#4615=CARTESIAN_POINT ( 'NONE',  ( 97.06112373929039450, -37.99668619498721256, 26.42731374779140197 ) ) ;
#4616=CARTESIAN_POINT ( 'NONE',  ( 99.64399296875224366, -31.54106566633107533, 160.2514674471249521 ) ) ;
#4617=AXIS2_PLACEMENT_3D ( 'NONE', #51747, #55317, #83073 ) ;
#4618=CARTESIAN_POINT ( 'NONE',  ( 105.1555015486555078, -47.05240725173535310, 12.42991099019596923 ) ) ;
#4622=AXIS2_PLACEMENT_3D ( 'NONE', #87415, #16593, #72009 ) ;
#4624=CARTESIAN_POINT ( 'NONE',  ( 131.0667039024480118, -58.35344715994099829, 231.5838068554150198 ) ) ;
#4626=CARTESIAN_POINT ( 'NONE',  ( 99.16350003447738004, -30.55523068857526070, 166.7982118921487142 ) ) ;
#4628=CARTESIAN_POINT ( 'NONE',  ( 99.08970013401406618, -42.79568349143557526, 131.8439815248826221 ) ) ;
#4630=ORIENTED_EDGE ( 'NONE', *, *, #42086, .T. ) ;
#4631=CARTESIAN_POINT ( 'NONE',  ( 96.66715014961923202, -32.91509328854561289, 21.03467289495897319 ) ) ;
#4632=CARTESIAN_POINT ( 'NONE',  ( 109.6537587170975030, -46.87336088289573865, 43.77562527591094721 ) ) ;
#4635=EDGE_CURVE ( 'NONE', #11339, #44492, #58712, .T. ) ;
#4636=CARTESIAN_POINT ( 'NONE',  ( 104.4899661847896368, -26.97880442220879260, 146.2818772940478596 ) ) ;
#4637=CARTESIAN_POINT ( 'NONE',  ( 106.6019379103756535, -25.27972995136449441, 322.9014499992877631 ) ) ;
#4639=CARTESIAN_POINT ( 'NONE',  ( 85.24325998657072034, -58.55267046464445002, 14.67562527591094756 ) ) ;
#4642=CARTESIAN_POINT ( 'NONE',  ( 99.95068698205643898, -44.40877713917536340, 46.98133956162592284 ) ) ;
#4643=CARTESIAN_POINT ( 'NONE',  ( 103.7231914492017637, -26.19396519929847145, 201.3089586092439731 ) ) ;
#4644=CARTESIAN_POINT ( 'NONE',  ( 112.7717388973142647, -27.93574178168534061, 65.61848241876793963 ) ) ;
#4646=FACE_OUTER_BOUND ( 'NONE', #63564, .T. ) ;
#4647=CARTESIAN_POINT ( 'NONE',  ( 149.4409906032288973, -0.9156555935619370423, 394.9756252759100903 ) ) ;
#4648=FACE_OUTER_BOUND ( 'NONE', #61663, .T. ) ;
#4651=ORIENTED_EDGE ( 'NONE', *, *, #30926, .F. ) ;
#4652=DIRECTION ( 'NONE',  ( 0.000000000000000000, 0.000000000000000000, -1.000000000000000000 ) ) ;
#4653=ORIENTED_EDGE ( 'NONE', *, *, #60973, .F. ) ;
#4654=CARTESIAN_POINT ( 'NONE',  ( 97.42673588038243793, -38.38435052442952866, 87.46133956162493917 ) ) ;
#4657=EDGE_LOOP ( 'NONE', ( #47184, #42725, #74552, #10877 ) ) ;
#4658=CARTESIAN_POINT ( 'NONE',  ( 107.5091008941355994, -47.12332782054429714, 233.6099109901969655 ) ) ;
#4659=DIRECTION ( 'NONE',  ( -4.237773401492740281E-14, 1.000000000000000000, 0.000000000000000000 ) ) ;
#4660=CARTESIAN_POINT ( 'NONE',  ( 80.06648329127399677, -8.729447159940999512, 4.925625275911999168 ) ) ;
#4661=DIRECTION ( 'NONE',  ( -1.000000000000000078E-15, 1.000000000000000000, 0.000000000000000000 ) ) ;
#4662=CARTESIAN_POINT ( 'NONE',  ( 115.0889047255370770, -30.61763668237492908, 80.34395860901999242 ) ) ;
#4663=EDGE_CURVE ( 'NONE', #18701, #8408, #30583, .T. ) ;
#4665=EDGE_CURVE ( 'NONE', #20875, #15623, #55915, .T. ) ;
#4667=CARTESIAN_POINT ( 'NONE',  ( 37.56670390244833158, -48.82844715994119866, 249.9678068554150343 ) ) ;
#4668=CARTESIAN_POINT ( 'NONE',  ( 116.7860849611261500, -31.33117650353035799, 179.2299109901969700 ) ) ;
#4669=EDGE_LOOP ( 'NONE', ( #51025, #88414, #58517, #70659 ) ) ;
#4671=VECTOR ( 'NONE', #61175, 1000.000000000000000 ) ;
#4673=CARTESIAN_POINT ( 'NONE',  ( 116.0040243724562146, -33.83170925634997417, 130.5196785439929670 ) ) ;
#4676=CARTESIAN_POINT ( 'NONE',  ( 115.3604274781776411, -30.50455558986046256, 260.3508633711485345 ) ) ;
#4677=DIRECTION ( 'NONE',  ( -5.551115123125777653E-14, -1.000000000000000000, 0.000000000000000000 ) ) ;
#4678=CARTESIAN_POINT ( 'NONE',  ( 179.4595971212889935, -28.98061976758940617, -5.074374724088000832 ) ) ;
#4679=ADVANCED_FACE ( 'NONE', ( #51885 ), #37398, .T. ) ;
#4680=CARTESIAN_POINT ( 'NONE',  ( 51.06648329127400388, -18.82844715994099971, 333.4006252759120343 ) ) ;
#4681=VECTOR ( 'NONE', #26631, 1000.000000000000000 ) ;
#4683=DIRECTION ( 'NONE',  ( -0.9254794337955620787, -0.3787978585227822492, 0.000000000000000000 ) ) ;
#4686=CARTESIAN_POINT ( 'NONE',  ( 117.1710321396411416, -41.15233254730030410, 208.4861014663869696 ) ) ;
#4688=VECTOR ( 'NONE', #77267, 1000.000000000000000 ) ;
#4689=EDGE_CURVE ( 'NONE', #65816, #49816, #85505, .T. ) ;
#4690=ORIENTED_EDGE ( 'NONE', *, *, #46902, .T. ) ;
#4692=LINE ( 'NONE', #60525, #5547 ) ;
#4693=CARTESIAN_POINT ( 'NONE',  ( 108.4182250531618763, -26.73512938305734110, 184.9693472879707201 ) ) ;
#4695=CARTESIAN_POINT ( 'NONE',  ( 115.8229818292872295, -31.72577650744706901, 94.24017908913180008 ) ) ;
#4698=CARTESIAN_POINT ( 'NONE',  ( 97.05801352979682406, -41.42088835504144839, 211.6632443235299945 ) ) ;
#4699=LINE ( 'NONE', #80121, #3833 ) ;
#4702=ADVANCED_FACE ( 'NONE', ( #39613 ), #33259, .F. ) ;
#4703=VECTOR ( 'NONE', #56703, 1000.000000000000000 ) ;
#4704=CARTESIAN_POINT ( 'NONE',  ( 108.8069666745183639, -46.61095096727596143, 63.71573676758425364 ) ) ;
#4707=CARTESIAN_POINT ( 'NONE',  ( 98.04152846853264691, -41.04187693203201093, 166.6812038652217041 ) ) ;
#4708=EDGE_CURVE ( 'NONE', #70, #58818, #82663, .T. ) ;
#4709=CARTESIAN_POINT ( 'NONE',  ( 105.7780793485435851, -44.78982812472496988, 35.26809036959094357 ) ) ;
#4710=CARTESIAN_POINT ( 'NONE',  ( 117.2433672581536968, -42.84935593481555571, 124.3956252759109731 ) ) ;
#4713=EDGE_CURVE ( 'NONE', #40161, #80487, #36214, .T. ) ;
#4714=CARTESIAN_POINT ( 'NONE',  ( 49.21213752016101495, -29.73316016639650172, 313.9678068554150059 ) ) ;
#4715=CARTESIAN_POINT ( 'NONE',  ( 97.95250717983365973, -32.49412669507731266, 25.56312527591095929 ) ) ;
#4716=ORIENTED_EDGE ( 'NONE', *, *, #41987, .F. ) ;
#4718=VECTOR ( 'NONE', #60646, 1000.000000000000000 ) ;
#4720=EDGE_LOOP ( 'NONE', ( #2642, #2588, #42246, #5622 ) ) ;
#4721=ORIENTED_EDGE ( 'NONE', *, *, #7417, .T. ) ;
#4723=CARTESIAN_POINT ( 'NONE',  ( 104.1257281832662613, -27.47619977921510781, 54.74384839950496939 ) ) ;
#4724=CARTESIAN_POINT ( 'NONE',  ( 110.1440020323170330, -26.08875547494869451, 214.8403871806729342 ) ) ;
#4725=CARTESIAN_POINT ( 'NONE',  ( 112.7681627534586681, -45.43114336468926950, 178.0384824187679556 ) ) ;
#4726=CARTESIAN_POINT ( 'NONE',  ( 97.81938603920509934, -40.53623202280513738, 21.63691838182942107 ) ) ;
#4727=CARTESIAN_POINT ( 'NONE',  ( 100.5643946202652756, -27.81952766013699119, 26.56610146638793779 ) ) ;
#4730=VERTEX_POINT ( 'NONE', #60499 ) ;
#4731=VECTOR ( 'NONE', #76980, 1000.000000000000000 ) ;
#4732=ORIENTED_EDGE ( 'NONE', *, *, #77938, .T. ) ;
#4734=DIRECTION ( 'NONE',  ( -0.000000000000000000, -0.000000000000000000, -1.000000000000000000 ) ) ;
#4735=CARTESIAN_POINT ( 'NONE',  ( 110.1504846022309607, -26.06634163003500859, 214.8403871806729342 ) ) ;
#4736=ORIENTED_EDGE ( 'NONE', *, *, #73574, .F. ) ;
#4737=CARTESIAN_POINT ( 'NONE',  ( 113.7507820938996872, -44.72989589602062210, 193.1299109901969757 ) ) ;
#4739=DIRECTION ( 'NONE',  ( 1.000000000000000078E-15, 1.000000000000000083E-30, -1.000000000000000000 ) ) ;
#4740=CARTESIAN_POINT ( 'NONE',  ( 181.8764988495240118, -33.54226604284930602, -5.074374724088000832 ) ) ;
#4741=CARTESIAN_POINT ( 'NONE',  ( 70.06202783732101125, -36.73691869758536654, 361.9756252759101471 ) ) ;
#4742=CARTESIAN_POINT ( 'NONE',  ( 113.7157087630704240, -42.06174584507512293, 277.6356252759110816 ) ) ;
#4744=CARTESIAN_POINT ( 'NONE',  ( 29.56648329127298069, 25.62155284005700295, 361.9756252759109998 ) ) ;
#4745=CARTESIAN_POINT ( 'NONE',  ( 149.4532656544376721, -72.54365454176046057, 361.9756252759100335 ) ) ;
#4749=DIRECTION ( 'NONE',  ( -2.981567257902526681E-15, 0.8571673007021100021, 0.5150380749100580413 ) ) ;
#4750=CARTESIAN_POINT ( 'NONE',  ( 105.7995184961486217, -26.72403496493496888, 76.17729194189745101 ) ) ;
#4752=VERTEX_POINT ( 'NONE', #53670 ) ;
#4753=CARTESIAN_POINT ( 'NONE',  ( 41.56670390244689628, -36.32844715994109208, 180.4678068554150911 ) ) ;
#4754=CARTESIAN_POINT ( 'NONE',  ( 101.3926005705062749, -45.54394758209068073, 222.1213395616249784 ) ) ;
#4755=CARTESIAN_POINT ( 'NONE',  ( 96.03574380810476896, -41.06042880536169548, 92.62419670448296927 ) ) ;
#4756=CARTESIAN_POINT ( 'NONE',  ( 116.9258602667948566, -41.82750404599077854, 239.4346728949589647 ) ) ;
#4757=CARTESIAN_POINT ( 'NONE',  ( 107.0664832912750057, -36.72944715993903486, 4.925625275910970657 ) ) ;
#4758=CARTESIAN_POINT ( 'NONE',  ( 116.3212776292296127, -32.94146857471318413, 287.6356252759109680 ) ) ;
#4760=CARTESIAN_POINT ( 'NONE',  ( 103.6593828106357904, -46.19869665420930005, 38.30169458292214557 ) ) ;
#4761=CARTESIAN_POINT ( 'NONE',  ( 179.7974245136200011, -36.32844715994040996, 193.9678068554150059 ) ) ;
#4763=ADVANCED_FACE ( 'NONE', ( #12370, #81437 ), #4214, .F. ) ;
#4766=ORIENTED_EDGE ( 'NONE', *, *, #28796, .T. ) ;
#4767=CARTESIAN_POINT ( 'NONE',  ( 115.6810990589499397, -33.93640840262257541, 133.5105150661719620 ) ) ;
#4768=ADVANCED_FACE ( 'NONE', ( #45517 ), #25099, .T. ) ;
#4770=ORIENTED_EDGE ( 'NONE', *, *, #12341, .F. ) ;
#4771=VECTOR ( 'NONE', #45623, 1000.000000000000000 ) ;
#4772=CARTESIAN_POINT ( 'NONE',  ( 104.4898545173444973, -26.97883498049986883, 90.27984912381337779 ) ) ;
#4773=CARTESIAN_POINT ( 'NONE',  ( 98.00553567079155926, -41.84099229931889852, 132.7356252759109623 ) ) ;
#4774=DIRECTION ( 'NONE',  ( 1.000000000000000078E-15, 0.000000000000000000, 1.000000000000000000 ) ) ;
#4775=CARTESIAN_POINT ( 'NONE',  ( 77.96454488115479364, -16.94667115355656151, 7.474641677899402481 ) ) ;
#4777=EDGE_CURVE ( 'NONE', #3721, #89894, #60048, .T. ) ;
#4779=DIRECTION ( 'NONE',  ( 1.000000000000000078E-15, 1.000000000000000083E-30, -1.000000000000000000 ) ) ;
#4780=CARTESIAN_POINT ( 'NONE',  ( 116.8058161338298504, -37.62879752186918836, 78.75276813305399060 ) ) ;
#4781=VERTEX_POINT ( 'NONE', #26446 ) ;
#4782=ORIENTED_EDGE ( 'NONE', *, *, #27446, .T. ) ;
#4783=VERTEX_POINT ( 'NONE', #80526 ) ;
#4784=EDGE_CURVE ( 'NONE', #86805, #69972, #74151, .T. ) ;
#4785=VECTOR ( 'NONE', #4138, 1000.000000000000000 ) ;
#4787=CARTESIAN_POINT ( 'NONE',  ( 102.3610132369663432, -45.97051510703448685, 168.2137205140059564 ) ) ;
#4791=DIRECTION ( 'NONE',  ( 0.000000000000000000, 0.000000000000000000, 1.000000000000000000 ) ) ;
#4793=CARTESIAN_POINT ( 'NONE',  ( 41.56648329127499153, -36.32844715994070839, 83.67562527591201160 ) ) ;
#4794=DIRECTION ( 'NONE',  ( -1.000000000000000078E-15, 0.000000000000000000, 1.000000000000000000 ) ) ;
#4795=CARTESIAN_POINT ( 'NONE',  ( 116.1047473792920357, -29.10330858331343151, 74.38419670448293175 ) ) ;
#4796=ORIENTED_EDGE ( 'NONE', *, *, #22027, .T. ) ;
#4798=EDGE_LOOP ( 'NONE', ( #83931, #169 ) ) ;
#4799=CARTESIAN_POINT ( 'NONE',  ( 162.7866693523299944, -36.02818131005322044, 193.9678068554149775 ) ) ;
#4801=LINE ( 'NONE', #19772, #49644 ) ;
#4802=CARTESIAN_POINT ( 'NONE',  ( 98.92690986002996567, -36.11615286530263091, 144.0852332267349709 ) ) ;
#4804=CIRCLE ( 'NONE', #70087, 5.599999999999994316 ) ;
#4806=CARTESIAN_POINT ( 'NONE',  ( 136.8164806451551669, -18.72944715939129523, 6.749772901088581634 ) ) ;
#4808=ORIENTED_EDGE ( 'NONE', *, *, #31445, .F. ) ;
#4810=ORIENTED_EDGE ( 'NONE', *, *, #76659, .T. ) ;
#4811=ORIENTED_EDGE ( 'NONE', *, *, #56951, .T. ) ;
#4812=LINE ( 'NONE', #75198, #66583 ) ;
#4813=EDGE_CURVE ( 'NONE', #4000, #21358, #40122, .T. ) ;
#4814=CARTESIAN_POINT ( 'NONE',  ( 98.38943151359886485, -34.93026649658274607, 212.5958690201829597 ) ) ;
#4816=ADVANCED_FACE ( 'NONE', ( #18798 ), #87397, .T. ) ;
#4817=PLANE ( 'NONE',  #38563 ) ;
#4820=EDGE_LOOP ( 'NONE', ( #70863, #83092, #88200, #13402 ) ) ;
#4823=EDGE_LOOP ( 'NONE', ( #86998, #19685, #65029, #53257 ) ) ;
#4824=CARTESIAN_POINT ( 'NONE',  ( 115.6671688226974197, -35.76553148137116267, 231.7214237029249659 ) ) ;
#4825=VECTOR ( 'NONE', #4659, 1000.000000000000000 ) ;
#4826=CARTESIAN_POINT ( 'NONE',  ( 114.5834136592134200, -44.03589093681723909, 98.21276813305395592 ) ) ;
#4827=CARTESIAN_POINT ( 'NONE',  ( 98.60777729073571152, -43.80857954853296121, 71.86895860924397539 ) ) ;
#4828=CARTESIAN_POINT ( 'NONE',  ( 109.6404665629360267, -46.48072720445416195, 252.7816004336761466 ) ) ;
#4830=DIRECTION ( 'NONE',  ( 1.000000000000000078E-15, -1.000000000000000083E-30, -1.000000000000000000 ) ) ;
#4831=CARTESIAN_POINT ( 'NONE',  ( 103.0497676667862947, -26.43187579209836002, 166.3603871806729444 ) ) ;
#4833=ORIENTED_EDGE ( 'NONE', *, *, #81603, .T. ) ;
#4834=FACE_OUTER_BOUND ( 'NONE', #32177, .T. ) ;
#4835=ORIENTED_EDGE ( 'NONE', *, *, #9659, .F. ) ;
#4836=ORIENTED_EDGE ( 'NONE', *, *, #10479, .T. ) ;
#4837=CYLINDRICAL_SURFACE ( 'NONE', #41834, 2.517500000000005844 ) ;
#4839=ORIENTED_EDGE ( 'NONE', *, *, #54784, .T. ) ;
#4840=VECTOR ( 'NONE', #4779, 1000.000000000000000 ) ;
#4841=ADVANCED_FACE ( 'NONE', ( #33322 ), #74219, .T. ) ;
#4842=CARTESIAN_POINT ( 'NONE',  ( 107.0664832912739968, -8.979447159941031487, -5.074374724089029343 ) ) ;
#4843=VERTEX_POINT ( 'NONE', #68299 ) ;
#4844=CARTESIAN_POINT ( 'NONE',  ( 115.7831076647344588, -41.80230951982593979, 178.4064586084813016 ) ) ;
#4845=CARTESIAN_POINT ( 'NONE',  ( 96.07744114619573850, -37.92110155076959899, 81.40038718067299328 ) ) ;
#4847=DIRECTION ( 'NONE',  ( 0.000000000000000000, 0.000000000000000000, 1.000000000000000000 ) ) ;
#4850=CARTESIAN_POINT ( 'NONE',  ( 97.40233316251689644, -42.04621543282986096, 172.7146728949589942 ) ) ;
#4851=FACE_OUTER_BOUND ( 'NONE', #27361, .T. ) ;
#4852=LINE ( 'NONE', #68427, #33726 ) ;
#4854=CARTESIAN_POINT ( 'NONE',  ( 107.0664832912739541, -36.72944715994095333, 307.1356252759109680 ) ) ;
#4856=DIRECTION ( 'NONE',  ( 0.9834602067019604377, 0.1811243270069963496, 0.000000000000000000 ) ) ;
#4857=CARTESIAN_POINT ( 'NONE',  ( 32.56670390244712365, -18.82844715994099616, -5.074374724088000832 ) ) ;
#4858=CARTESIAN_POINT ( 'NONE',  ( 118.1283360304583994, -32.34034571477864262, 249.1270538473389706 ) ) ;
#4861=CARTESIAN_POINT ( 'NONE',  ( 97.48672026426986292, -32.61689163886055809, 12.00419670448293985 ) ) ;
#4862=CARTESIAN_POINT ( 'NONE',  ( 116.9629591039797845, -33.20839883953882321, 110.0984824187679578 ) ) ;
#4865=EDGE_CURVE ( 'NONE', #76536, #26931, #52822, .T. ) ;
#4866=FACE_OUTER_BOUND ( 'NONE', #12549, .T. ) ;
#4867=DIRECTION ( 'NONE',  ( -2.981567257902526681E-15, 0.8571673007021100021, 0.5150380749100580413 ) ) ;
#4868=ORIENTED_EDGE ( 'NONE', *, *, #862, .F. ) ;
#4870=AXIS2_PLACEMENT_3D ( 'NONE', #47714, #75453, #20492 ) ;
#4871=ADVANCED_FACE ( 'NONE', ( #61022 ), #88750, .T. ) ;
#4876=VERTEX_POINT ( 'NONE', #60112 ) ;
#4877=CARTESIAN_POINT ( 'NONE',  ( 97.81169150544869240, -40.51741169384158781, 71.63577594787710723 ) ) ;
#4878=CARTESIAN_POINT ( 'NONE',  ( 104.4960957391109559, -46.84663716100901354, 43.37848241876896083 ) ) ;
#4879=CARTESIAN_POINT ( 'NONE',  ( 72.26648329127297643, -1.929447159941394263, 342.9256252759109884 ) ) ;
#4883=CARTESIAN_POINT ( 'NONE',  ( 101.8145705177301892, -43.46543587290290134, 231.4724198280769940 ) ) ;
#4884=ORIENTED_EDGE ( 'NONE', *, *, #77980, .T. ) ;
#4885=ORIENTED_EDGE ( 'NONE', *, *, #8686, .F. ) ;
#4886=ORIENTED_EDGE ( 'NONE', *, *, #76905, .T. ) ;
#4889=DIRECTION ( 'NONE',  ( 0.0001211784769810529054, -0.7071067708032295895, 0.7071067811865515695 ) ) ;
#4890=CIRCLE ( 'NONE', #6317, 1.000000000000000888 ) ;
#4891=CARTESIAN_POINT ( 'NONE',  ( 116.8170317996813736, -34.15256532312115212, 104.0313894407264996 ) ) ;
#4894=CARTESIAN_POINT ( 'NONE',  ( 98.24278011039416469, -41.58876472015902692, 23.15872616303999010 ) ) ;
#4895=EDGE_CURVE ( 'NONE', #87481, #34970, #11079, .T. ) ;
#4899=CARTESIAN_POINT ( 'NONE',  ( 100.6696166679599003, -29.33055989933767904, 260.6441967044828516 ) ) ;
#4900=PLANE ( 'NONE',  #42862 ) ;
#4903=PLANE ( 'NONE',  #5472 ) ;
#4904=CARTESIAN_POINT ( 'NONE',  ( 80.06648329127399677, -8.350947159940998787, 308.6356252759119911 ) ) ;
#4905=CARTESIAN_POINT ( 'NONE',  ( 114.3647906391003630, -33.01227106732497418, 42.01951894101996032 ) ) ;
#4906=VECTOR ( 'NONE', #50613, 1000.000000000000114 ) ;
#4907=DIRECTION ( 'NONE',  ( -0.000000000000000000, 1.000000000000000000, 0.000000000000000000 ) ) ;
#4909=DIRECTION ( 'NONE',  ( -0.8571673007021084478, -0.5150380749100604838, -8.571673007021083688E-16 ) ) ;
#4910=ORIENTED_EDGE ( 'NONE', *, *, #61291, .T. ) ;
#4911=DIRECTION ( 'NONE',  ( 1.000000000000000078E-15, 0.000000000000000000, 1.000000000000000000 ) ) ;
#4913=EDGE_LOOP ( 'NONE', ( #17845, #82775, #14973, #80685 ) ) ;
#4914=CARTESIAN_POINT ( 'NONE',  ( 98.45854724665603896, -30.84808103350501085, 120.8499109901969604 ) ) ;
#4916=CARTESIAN_POINT ( 'NONE',  ( 100.8685319560204050, -42.60665150962044123, 81.35241982807694683 ) ) ;
#4917=DIRECTION ( 'NONE',  ( 0.000000000000000000, 0.000000000000000000, -1.000000000000000000 ) ) ;
#4918=CARTESIAN_POINT ( 'NONE',  ( 112.8895349442155265, -29.35594087158844445, 120.9882499725639633 ) ) ;
#4919=CARTESIAN_POINT ( 'NONE',  ( 131.0667039024480118, -67.87844715994100397, 231.5838068554150198 ) ) ;
#4922=CARTESIAN_POINT ( 'NONE',  ( 99.74686247383996829, -44.23293585951837059, 17.96133956162493206 ) ) ;
#4923=CARTESIAN_POINT ( 'NONE',  ( 97.07208394142573127, -35.37832485732319299, 182.2194452067948873 ) ) ;
#4924=ORIENTED_EDGE ( 'NONE', *, *, #30752, .F. ) ;
#4925=VECTOR ( 'NONE', #31546, 999.9999999999998863 ) ;
#4926=DIRECTION ( 'NONE',  ( 0.000000000000000000, 1.000000000000000000, 0.000000000000000000 ) ) ;
#4930=ORIENTED_EDGE ( 'NONE', *, *, #6167, .T. ) ;
#4931=VERTEX_POINT ( 'NONE', #73761 ) ;
#4933=ORIENTED_EDGE ( 'NONE', *, *, #78641, .T. ) ;
#4934=CARTESIAN_POINT ( 'NONE',  ( 101.2091419812964830, -45.28691980162484754, 242.1108633711499465 ) ) ;
#4935=CARTESIAN_POINT ( 'NONE',  ( 97.61330010463601070, -39.99285327795418254, 126.5905029351318802 ) ) ;
#4936=FACE_OUTER_BOUND ( 'NONE', #10175, .T. ) ;
#4937=CARTESIAN_POINT ( 'NONE',  ( 110.3719271596222882, -47.27686491584164941, 48.80610146638797175 ) ) ;
#4939=VERTEX_POINT ( 'NONE', #39239 ) ;
#4940=CARTESIAN_POINT ( 'NONE',  ( 182.2300522401169758, -33.89581943343728199, 313.9678068554149490 ) ) ;
#4942=LINE ( 'NONE', #88072, #23024 ) ;
#4944=EDGE_CURVE ( 'NONE', #1484, #88413, #60565, .T. ) ;
#4946=CARTESIAN_POINT ( 'NONE',  ( 193.0374249753377001, -23.42844715993431848, 129.9678068554150343 ) ) ;
#4947=CARTESIAN_POINT ( 'NONE',  ( 34.67381068362062280, -26.00627455219358453, 342.9256252759109884 ) ) ;
#4948=CARTESIAN_POINT ( 'NONE',  ( 117.4695305279094981, -36.80206755349689729, 263.8213395616251660 ) ) ;
#4952=LINE ( 'NONE', #32647, #1190 ) ;
#4953=CARTESIAN_POINT ( 'NONE',  ( 113.0872481101271205, -29.11229423309321618, 273.9667055423626039 ) ) ;
#4954=DIRECTION ( 'NONE',  ( 0.000000000000000000, 0.000000000000000000, 1.000000000000000000 ) ) ;
#4955=CARTESIAN_POINT ( 'NONE',  ( 113.4926247784320452, -28.54816540729044405, 75.54705384733995288 ) ) ;
#4957=CARTESIAN_POINT ( 'NONE',  ( 95.96722792477895325, -36.58315769931292749, 156.3280062282919687 ) ) ;
#4960=VERTEX_POINT ( 'NONE', #81500 ) ;
#4963=DIRECTION ( 'NONE',  ( 1.000000000000000078E-15, 1.000000000000000083E-30, -1.000000000000000000 ) ) ;
#4966=DIRECTION ( 'NONE',  ( 1.000000000000000000, 0.000000000000000000, 9.351236661543306751E-17 ) ) ;
#4967=CARTESIAN_POINT ( 'NONE',  ( 114.2838679902333610, -44.31336211532283897, 158.1813395616249807 ) ) ;
#4969=CARTESIAN_POINT ( 'NONE',  ( 19.56670390244643443, -25.42844715994203852, 180.4678068554150911 ) ) ;
#4974=CARTESIAN_POINT ( 'NONE',  ( 97.96720171806632038, -41.86261760143219846, 136.7356252759109623 ) ) ;
#4978=ORIENTED_EDGE ( 'NONE', *, *, #38037, .F. ) ;
#4979=EDGE_CURVE ( 'NONE', #61259, #7662, #85767, .T. ) ;
#4982=LINE ( 'NONE', #30118, #27812 ) ;
#4986=EDGE_CURVE ( 'NONE', #68369, #33468, #71336, .T. ) ;
#4987=LINE ( 'NONE', #47189, #82819 ) ;
#4989=CARTESIAN_POINT ( 'NONE',  ( 113.2454463666727946, -28.75862960087268405, 179.5522973137137228 ) ) ;
#4990=VECTOR ( 'NONE', #29562, 1000.000000000000114 ) ;
#4991=VERTEX_POINT ( 'NONE', #23204 ) ;
#4992=EDGE_CURVE ( 'NONE', #36895, #11918, #7408, .T. ) ;
#4994=LINE ( 'NONE', #61727, #28812 ) ;
#4995=CARTESIAN_POINT ( 'NONE',  ( 103.8504807240353500, -26.87063827031099450, 206.3394347997199816 ) ) ;
#4996=EDGE_CURVE ( 'NONE', #49134, #63259, #6000, .T. ) ;
#4998=ORIENTED_EDGE ( 'NONE', *, *, #79153, .T. ) ;
#4999=CARTESIAN_POINT ( 'NONE',  ( 97.00151786184787284, -41.45262973156711439, 57.67562527591096710 ) ) ;
#5000=CYLINDRICAL_SURFACE ( 'NONE', #35672, 9.999999999999998224 ) ;
#5002=CARTESIAN_POINT ( 'NONE',  ( 97.75828313668286285, -40.38462675027328430, 22.62423254407919160 ) ) ;
#5003=ORIENTED_EDGE ( 'NONE', *, *, #65300, .T. ) ;
#5005=ORIENTED_EDGE ( 'NONE', *, *, #88470, .T. ) ;
#5006=VERTEX_POINT ( 'NONE', #35900 ) ;
#5007=CARTESIAN_POINT ( 'NONE',  ( 106.9593448401346620, -46.12439510495315886, 229.0111071154209696 ) ) ;
#5011=CARTESIAN_POINT ( 'NONE',  ( 184.5664832912729878, 25.62155284005700295, 361.9756252759109998 ) ) ;
#5012=CIRCLE ( 'NONE', #16636, 4.874999999999990230 ) ;
#5013=CARTESIAN_POINT ( 'NONE',  ( 116.7951252642580329, -39.38782981925626103, 154.6147919402135642 ) ) ;
#5014=CARTESIAN_POINT ( 'NONE',  ( 82.81648329127399677, -36.72944715994106701, 3.101481641215461327 ) ) ;
#5015=AXIS2_PLACEMENT_3D ( 'NONE', #1963, #35567, #83738 ) ;
#5016=ORIENTED_EDGE ( 'NONE', *, *, #50973, .T. ) ;
#5017=FACE_OUTER_BOUND ( 'NONE', #21001, .T. ) ;
#5019=CARTESIAN_POINT ( 'NONE',  ( 116.3212776292269268, -32.94146857470660450, 84.13562527591095375 ) ) ;
#5021=CARTESIAN_POINT ( 'NONE',  ( 99.76197604230684135, -44.21744263965017296, 21.96133956162593748 ) ) ;
#5022=ORIENTED_EDGE ( 'NONE', *, *, #6422, .F. ) ;
#5024=CARTESIAN_POINT ( 'NONE',  ( 114.7541070161690158, -40.70454043057743121, 241.2528522743529606 ) ) ;
#5025=PLANE ( 'NONE',  #6821 ) ;
#5026=CARTESIAN_POINT ( 'NONE',  ( 113.8091913586854531, -43.81457933525494042, 158.1813395616259754 ) ) ;
#5027=DIRECTION ( 'NONE',  ( 0.000000000000000000, 0.000000000000000000, 1.000000000000000000 ) ) ;
#5028=CARTESIAN_POINT ( 'NONE',  ( 177.8371591254545194, -47.82818131005477369, 180.4678068554150343 ) ) ;
#5031=CARTESIAN_POINT ( 'NONE',  ( 110.0644950372451945, -26.04256623378434554, 215.8708633711489711 ) ) ;
#5033=ORIENTED_EDGE ( 'NONE', *, *, #23143, .T. ) ;
#5034=CARTESIAN_POINT ( 'NONE',  ( 118.0477628396966310, -38.34468641101997122, 69.72229194257801055 ) ) ;
#5035=CARTESIAN_POINT ( 'NONE',  ( 116.3183303039212291, -32.94226276200836878, 104.1356252759109680 ) ) ;
#5036=EDGE_CURVE ( 'NONE', #85840, #76619, #8207, .T. ) ;
#5037=ORIENTED_EDGE ( 'NONE', *, *, #82023, .F. ) ;
#5039=ORIENTED_EDGE ( 'NONE', *, *, #17313, .F. ) ;
#5041=CARTESIAN_POINT ( 'NONE',  ( 105.7976818973178581, -26.72428486692769312, 160.1772091339258282 ) ) ;
#5044=CARTESIAN_POINT ( 'NONE',  ( 99.63185314732805864, -32.29918761127225224, 128.7290427505439823 ) ) ;
#5045=CARTESIAN_POINT ( 'NONE',  ( 96.75123844313058896, -34.86533355485506291, 237.1841967044819626 ) ) ;
#5050=VERTEX_POINT ( 'NONE', #22742 ) ;
#5051=ORIENTED_EDGE ( 'NONE', *, *, #38184, .T. ) ;
#5052=AXIS2_PLACEMENT_3D ( 'NONE', #3871, #64324, #86109 ) ;
#5055=ORIENTED_EDGE ( 'NONE', *, *, #764, .T. ) ;
#5056=ORIENTED_EDGE ( 'NONE', *, *, #20635, .T. ) ;
#5057=CARTESIAN_POINT ( 'NONE',  ( 152.5667039024472160, -23.42844715993585325, 129.9678068554149775 ) ) ;
#5060=DIRECTION ( 'NONE',  ( 0.1811243268507098381, -0.9834602067307437467, 0.000000000000000000 ) ) ;
#5061=CARTESIAN_POINT ( 'NONE',  ( 99.60253261678104764, -31.60088882024776780, 165.2819436375999658 ) ) ;
#5062=CARTESIAN_POINT ( 'NONE',  ( 101.3600985487617692, -27.95198515609010315, 25.53562527591096654 ) ) ;
#5063=CARTESIAN_POINT ( 'NONE',  ( 109.7229095233572878, -27.00028666605756555, 125.8649514782447199 ) ) ;
#5064=VERTEX_POINT ( 'NONE', #5411 ) ;
#5065=DIRECTION ( 'NONE',  ( -1.000000000000000000, 9.376883653928684652E-16, 1.500301384628589584E-15 ) ) ;
#5068=ORIENTED_EDGE ( 'NONE', *, *, #67811, .F. ) ;
#5069=CARTESIAN_POINT ( 'NONE',  ( 31.89136050872121331, -31.76306994223872238, 193.9678068554150911 ) ) ;
#5071=CARTESIAN_POINT ( 'NONE',  ( 117.0922404263411778, -37.60051096986498465, 133.7571228985926552 ) ) ;
#5072=FACE_OUTER_BOUND ( 'NONE', #24791, .T. ) ;
#5073=EDGE_LOOP ( 'NONE', ( #25165, #17668, #3430, #31072 ) ) ;
#5074=CARTESIAN_POINT ( 'NONE',  ( 107.1956731390977779, -26.28293224109629733, 35.06705384733893283 ) ) ;
#5076=CARTESIAN_POINT ( 'NONE',  ( 111.9491823805485922, -27.46919719833538309, 55.68991099019693536 ) ) ;
#5077=AXIS2_PLACEMENT_3D ( 'NONE', #83899, #21670, #28458 ) ;
#5080=LINE ( 'NONE', #12348, #15836 ) ;
#5082=LINE ( 'NONE', #26426, #8983 ) ;
#5083=DIRECTION ( 'NONE',  ( 0.000000000000000000, 0.000000000000000000, -1.000000000000000000 ) ) ;
#5084=PLANE ( 'NONE',  #36834 ) ;
#5085=ADVANCED_FACE ( 'NONE', ( #82176 ), #7200, .F. ) ;
#5086=AXIS2_PLACEMENT_3D ( 'NONE', #62727, #62275, #55888 ) ;
#5087=CARTESIAN_POINT ( 'NONE',  ( 51.23005224011598102, -33.89581943344511217, 342.9256252759109884 ) ) ;
#5088=EDGE_CURVE ( 'NONE', #4730, #54028, #14006, .T. ) ;
#5090=ORIENTED_EDGE ( 'NONE', *, *, #17976, .F. ) ;
#5091=CARTESIAN_POINT ( 'NONE',  ( 97.31040724827032307, -32.83447933365327742, 41.02419670448193045 ) ) ;
#5092=CARTESIAN_POINT ( 'NONE',  ( 117.9325828832643026, -34.70414220975756336, 199.9851490854349549 ) ) ;
#5093=CARTESIAN_POINT ( 'NONE',  ( 114.5831001172654595, -44.03558617456690172, 94.21276813305395592 ) ) ;
#5094=EDGE_CURVE ( 'NONE', #74091, #88572, #10334, .T. ) ;
#5095=CARTESIAN_POINT ( 'NONE',  ( 194.0371591254572934, -24.89890238294407965, 300.4678068554149490 ) ) ;
#5096=CARTESIAN_POINT ( 'NONE',  ( 25.56670390244745050, -48.82844715994178841, 170.7178068554150627 ) ) ;
#5098=AXIS2_PLACEMENT_3D ( 'NONE', #70473, #83656, #35937 ) ;
#5099=AXIS2_PLACEMENT_3D ( 'NONE', #721, #20727, #22528 ) ;
#5101=ORIENTED_EDGE ( 'NONE', *, *, #61889, .F. ) ;
#5102=CARTESIAN_POINT ( 'NONE',  ( 117.1895451461016648, -38.97942580829903392, 99.64038718067195077 ) ) ;
#5106=CARTESIAN_POINT ( 'NONE',  ( 118.0177608886752836, -35.41288285714062312, 234.9337205140059552 ) ) ;
#5107=DIRECTION ( 'NONE',  ( 0.000000000000000000, -1.000000000000000000, 0.000000000000000000 ) ) ;
#5108=DIRECTION ( 'NONE',  ( 0.000000000000000000, 0.000000000000000000, -1.000000000000000000 ) ) ;
#5109=ADVANCED_FACE ( 'NONE', ( #89426 ), #33550, .F. ) ;
#5110=DIRECTION ( 'NONE',  ( 1.000000000000000000, 0.000000000000000000, 0.000000000000000000 ) ) ;
#5111=CARTESIAN_POINT ( 'NONE',  ( 105.7995185016981026, -26.72403496430482406, 81.17729194145603344 ) ) ;
#5112=CARTESIAN_POINT ( 'NONE',  ( 131.8552587341645221, -38.37463194330769767, 2.472581811083949255 ) ) ;
#5114=CARTESIAN_POINT ( 'NONE',  ( 98.25516505653058630, -40.97492784622586015, 171.6841967044829573 ) ) ;
#5116=ORIENTED_EDGE ( 'NONE', *, *, #14443, .T. ) ;
#5117=CARTESIAN_POINT ( 'NONE',  ( 115.5384384484689804, -31.27996107247446744, 140.7130118773259539 ) ) ;
#5118=LINE ( 'NONE', #5579, #18233 ) ;
#5119=CARTESIAN_POINT ( 'NONE',  ( 97.63766479707265944, -34.12929003103651127, 247.1127681330529811 ) ) ;
#5122=CARTESIAN_POINT ( 'NONE',  ( 149.4512091874902922, -60.54365471797113685, 361.9756252759100335 ) ) ;
#5124=PLANE ( 'NONE',  #24094 ) ;
#5125=CARTESIAN_POINT ( 'NONE',  ( 168.0371591254546217, -48.62818131005518296, 117.4678068554150485 ) ) ;
#5127=CARTESIAN_POINT ( 'NONE',  ( 107.5647246096319236, -47.74832088493825211, 192.6003871806729535 ) ) ;
#5128=CARTESIAN_POINT ( 'NONE',  ( 49.21213752016101495, -29.73316016639650172, 237.4678068554150059 ) ) ;
#5129=ORIENTED_EDGE ( 'NONE', *, *, #57413, .F. ) ;
#5130=VERTEX_POINT ( 'NONE', #27187 ) ;
#5132=CARTESIAN_POINT ( 'NONE',  ( 53.56670390244828184, -48.82844715994055917, 300.4678068554150059 ) ) ;
#5134=CARTESIAN_POINT ( 'NONE',  ( 31.56670390244800828, -33.35206098992711077, -5.074374724088000832 ) ) ;
#5135=VECTOR ( 'NONE', #38406, 1000.000000000000000 ) ;
#5136=FACE_OUTER_BOUND ( 'NONE', #78983, .T. ) ;
#5137=VERTEX_POINT ( 'NONE', #54862 ) ;
#5138=CIRCLE ( 'NONE', #42858, 13.00000000000000355 ) ;
#5139=CARTESIAN_POINT ( 'NONE',  ( 99.04388118832164878, -42.84098620836660132, 61.84393314859575241 ) ) ;
#5140=CIRCLE ( 'NONE', #5211, 2.999999999999933387 ) ;
#5141=VECTOR ( 'NONE', #32143, 1000.000000000000000 ) ;
#5142=EDGE_CURVE ( 'NONE', #28975, #81967, #53804, .T. ) ;
#5143=CARTESIAN_POINT ( 'NONE',  ( 96.85831052012196096, -34.61278962133658155, 216.1641967044819808 ) ) ;
#5144=DIRECTION ( 'NONE',  ( 0.000000000000000000, 0.000000000000000000, -1.000000000000000000 ) ) ;
#5146=CIRCLE ( 'NONE', #74789, 4.749999999999976907 ) ;
#5149=CARTESIAN_POINT ( 'NONE',  ( 72.17003668186724497, -9.772340378754513779, 14.92562527591103461 ) ) ;
#5150=CARTESIAN_POINT ( 'NONE',  ( 105.1735626975883662, -45.17443245699572429, 25.20713798863899413 ) ) ;
#5151=CARTESIAN_POINT ( 'NONE',  ( 102.3506485400807975, -46.05136549539959390, 123.2041967044829818 ) ) ;
#5153=DIRECTION ( 'NONE',  ( 0.7071067811864661934, 0.7071067811866289521, 7.071067811864654918E-16 ) ) ;
#5155=CIRCLE ( 'NONE', #815, 3.299999999999999822 ) ;
#5156=DIRECTION ( 'NONE',  ( 0.9068632946707807507, -0.4214249218767880945, 9.080193194566099635E-16 ) ) ;
#5157=CARTESIAN_POINT ( 'NONE',  ( 82.81648124396200217, -18.63640413217068925, 6.749771997051031036 ) ) ;
#5159=ORIENTED_EDGE ( 'NONE', *, *, #12701, .F. ) ;
#5160=ADVANCED_FACE ( 'NONE', ( #81283 ), #26290, .F. ) ;
#5162=ORIENTED_EDGE ( 'NONE', *, *, #61363, .T. ) ;
#5163=ORIENTED_EDGE ( 'NONE', *, *, #6131, .T. ) ;
#5165=AXIS2_PLACEMENT_3D ( 'NONE', #51868, #50994, #16492 ) ;
#5166=CARTESIAN_POINT ( 'NONE',  ( 102.0478764085966361, -45.04113848309104640, 51.56670554236298187 ) ) ;
#5167=CARTESIAN_POINT ( 'NONE',  ( 114.1397626436471171, -29.04081378529519597, 199.4841967044819739 ) ) ;
#5168=CARTESIAN_POINT ( 'NONE',  ( 98.10941331148539746, -42.08998169807674117, 161.7556252759109725 ) ) ;
#5169=CARTESIAN_POINT ( 'NONE',  ( 97.87036982965192067, -40.65816500629669150, 21.64744875867875251 ) ) ;
#5170=CARTESIAN_POINT ( 'NONE',  ( 115.9265467165007379, -42.18176083994490000, 14.38705384733995984 ) ) ;
#5172=VECTOR ( 'NONE', #43299, 1000.000000000000000 ) ;
#5173=CARTESIAN_POINT ( 'NONE',  ( 188.5667039024479834, -62.87844715994099687, 137.2178068554150059 ) ) ;
#5177=ORIENTED_EDGE ( 'NONE', *, *, #32590, .T. ) ;
#5178=CIRCLE ( 'NONE', #55924, 1.000000000000000888 ) ;
#5179=CYLINDRICAL_SURFACE ( 'NONE', #41512, 13.00000000000000355 ) ;
#5180=CARTESIAN_POINT ( 'NONE',  ( 113.1256532486054880, -46.02994946121840769, 223.0480062282919675 ) ) ;
#5182=CARTESIAN_POINT ( 'NONE',  ( 117.1973380236488111, -34.26920065746595867, 209.0156252759109634 ) ) ;
#5183=CARTESIAN_POINT ( 'NONE',  ( 100.9546727506802455, -28.70702577259136135, 35.59395861520961546 ) ) ;
#5187=LINE ( 'NONE', #41035, #37729 ) ;
#5189=CARTESIAN_POINT ( 'NONE',  ( 115.1018088917358426, -38.78897616956993488, 277.6356252759109680 ) ) ;
#5190=CARTESIAN_POINT ( 'NONE',  ( 188.5667039024479834, -62.87844715994099687, 257.2178068554150059 ) ) ;
#5191=CARTESIAN_POINT ( 'NONE',  ( 101.9933622192556015, -45.44592330270667446, 173.1564353148846465 ) ) ;
#5192=DIRECTION ( 'NONE',  ( 0.7071067811989762975, -0.7071067811741188480, 2.899137802814003655E-29 ) ) ;
#5193=CARTESIAN_POINT ( 'NONE',  ( 19.56670390244643443, -25.42844715994203852, 180.4678068554150911 ) ) ;
#5194=LINE ( 'NONE', #27416, #34155 ) ;
#5195=DIRECTION ( 'NONE',  ( 1.000000000000000000, 4.163336342344333240E-14, 0.000000000000000000 ) ) ;
#5196=EDGE_CURVE ( 'NONE', #72082, #39122, #33106, .T. ) ;
#5197=DIRECTION ( 'NONE',  ( -1.000000000000000000, 0.000000000000000000, 1.094868876412250136E-15 ) ) ;
#5198=DIRECTION ( 'NONE',  ( -0.000000000000000000, -0.000000000000000000, -1.000000000000000000 ) ) ;
#5199=ORIENTED_EDGE ( 'NONE', *, *, #31953, .T. ) ;
#5200=PLANE ( 'NONE',  #7466 ) ;
#5201=CARTESIAN_POINT ( 'NONE',  ( 118.8150946519381250, -38.46269469016341702, 223.7099109901969598 ) ) ;
#5202=CARTESIAN_POINT ( 'NONE',  ( 114.7260775003150712, -43.80144150384058577, 119.2327681330539804 ) ) ;
#5203=CARTESIAN_POINT ( 'NONE',  ( 118.1491249375158645, -36.11907637682050165, 269.8822919425776945 ) ) ;
#5204=DIRECTION ( 'NONE',  ( 1.000000000000000000, 4.163336342344333240E-14, 0.000000000000000000 ) ) ;
#5205=DIRECTION ( 'NONE',  ( 0.000000000000000000, 0.000000000000000000, -1.000000000000000000 ) ) ;
#5206=FACE_OUTER_BOUND ( 'NONE', #62465, .T. ) ;
#5207=DIRECTION ( 'NONE',  ( 0.000000000000000000, 0.000000000000000000, -1.000000000000000000 ) ) ;
#5208=PLANE ( 'NONE',  #34085 ) ;
#5211=AXIS2_PLACEMENT_3D ( 'NONE', #74162, #11938, #49566 ) ;
#5212=CIRCLE ( 'NONE', #19732, 0.5000000000000004441 ) ;
#5214=VERTEX_POINT ( 'NONE', #19029 ) ;
#5215=CARTESIAN_POINT ( 'NONE',  ( 104.1185212827848545, -44.74603268130591971, 141.7181341137909669 ) ) ;
#5218=ORIENTED_EDGE ( 'NONE', *, *, #19222, .T. ) ;
#5220=CARTESIAN_POINT ( 'NONE',  ( 113.0643619202157453, -28.22920495858477352, 125.5870538473399591 ) ) ;
#5221=DIRECTION ( 'NONE',  ( 0.000000000000000000, 0.000000000000000000, 1.000000000000000000 ) ) ;
#5222=EDGE_CURVE ( 'NONE', #10055, #87762, #62150, .T. ) ;
#5223=EDGE_CURVE ( 'NONE', #89871, #64817, #41244, .T. ) ;
#5226=CARTESIAN_POINT ( 'NONE',  ( 97.81169789812091153, -40.51742632959496859, 107.6355761348045519 ) ) ;
#5227=EDGE_CURVE ( 'NONE', #72723, #16229, #68530, .T. ) ;
#5229=CARTESIAN_POINT ( 'NONE',  ( 116.4719273984281784, -32.36179259691358823, 59.16038718067295576 ) ) ;
#5230=VERTEX_POINT ( 'NONE', #13559 ) ;
#5231=ORIENTED_EDGE ( 'NONE', *, *, #85702, .F. ) ;
#5233=LINE ( 'NONE', #32922, #8062 ) ;
#5234=CARTESIAN_POINT ( 'NONE',  ( 113.2097911582632292, -29.11871762112829032, 160.5356252759109736 ) ) ;
#5240=DIRECTION ( 'NONE',  ( 0.0001484127182026448726, -0.8660253910675250744, -0.5000000000000052180 ) ) ;
#5241=DIRECTION ( 'NONE',  ( -4.237773401492740281E-14, 1.000000000000000000, 0.000000000000000000 ) ) ;
#5242=CARTESIAN_POINT ( 'NONE',  ( 97.64212626138829876, -32.24102647341085515, 75.97276813305397525 ) ) ;
#5244=ORIENTED_EDGE ( 'NONE', *, *, #6536, .F. ) ;
#5246=DIRECTION ( 'NONE',  ( 1.000000000000000000, 0.000000000000000000, 0.000000000000000000 ) ) ;
#5247=CARTESIAN_POINT ( 'NONE',  ( 107.0664832912739257, -50.22944715994095333, 312.1356252759112522 ) ) ;
#5248=CARTESIAN_POINT ( 'NONE',  ( 102.2276451341571999, -43.90295244235954897, 149.9099951314959753 ) ) ;
#5249=B_SPLINE_CURVE_WITH_KNOTS ( 'NONE', 3,
 ( #421, #69921, #7686, #31875, #66846, #30098, #30983, #23310, #25064, #85973, #57797, #80050, #11442, #79605, #3291, #58670, #17805, #51408 ),
 .UNSPECIFIED., .F., .F.,
 ( 4, 2, 2, 2, 2, 2, 2, 2, 4 ),
 ( 0.5000352890896443414, 0.5625308779534388126, 0.6250264668172332838, 0.6875220556810277550, 0.7500176445448221152, 0.8125132334086166974, 0.8750088222724110576, 0.9375044111362055288, 1.000000000000000000 ),
 .UNSPECIFIED. ) ;
#5252=ORIENTED_EDGE ( 'NONE', *, *, #17423, .T. ) ;
#5254=CARTESIAN_POINT ( 'NONE',  ( 107.0664832912739399, -36.72944715994095333, 311.6356252759109680 ) ) ;
#5255=ORIENTED_EDGE ( 'NONE', *, *, #11778, .F. ) ;
#5256=ORIENTED_EDGE ( 'NONE', *, *, #32648, .F. ) ;
#5257=CARTESIAN_POINT ( 'NONE',  ( 77.42411991178802566, -19.49143581486272225, 6.902478035881912000 ) ) ;
#5258=CARTESIAN_POINT ( 'NONE',  ( 111.4343887032284783, -44.43980907907789657, 209.4187261630399632 ) ) ;
#5259=LINE ( 'NONE', #59315, #77191 ) ;
#5262=AXIS2_PLACEMENT_3D ( 'NONE', #49235, #6578, #70148 ) ;
#5263=EDGE_LOOP ( 'NONE', ( #87268, #44025, #39183, #38550 ) ) ;
#5265=AXIS2_PLACEMENT_3D ( 'NONE', #68587, #61743, #89479 ) ;
#5266=ADVANCED_FACE ( 'NONE', ( #1282 ), #77583, .F. ) ;
#5267=AXIS2_PLACEMENT_3D ( 'NONE', #84018, #63105, #69933 ) ;
#5269=ORIENTED_EDGE ( 'NONE', *, *, #50579, .F. ) ;
#5271=CARTESIAN_POINT ( 'NONE',  ( 99.55502339443899018, -39.99451353983162960, 229.4709475124479638 ) ) ;
#5272=EDGE_CURVE ( 'NONE', #87926, #37760, #43933, .T. ) ;
#5273=CARTESIAN_POINT ( 'NONE',  ( 115.1840797895677611, -43.30599572718466561, 88.28419670448195689 ) ) ;
#5274=CARTESIAN_POINT ( 'NONE',  ( 109.6783822832554449, -47.44587409406599932, 87.75467289495897205 ) ) ;
#5275=CARTESIAN_POINT ( 'NONE',  ( 111.1802904571995896, -44.25639671664211505, 249.5838068554169524 ) ) ;
#5276=B_SPLINE_SURFACE_WITH_KNOTS ( 'NONE', 3, 3, ( 
 ( #34173, #27817, #21466, #63692, #1473, #69611, #62335, #56858, #55493, #49135, #82810, #35515, #70056, #21923, #42325, #89613, #76419, #1016, #20571, #41874, #28721, #6930, #83249, #48687, #84148, #27370, #49589, #15094, #8283, #48240, #84599, #35979, #22362, #41430, #69159, #34631, #118, #80017, #3694, #9616, #51374, #37776, #43680, #71415, #30951, #10507, #31387, #17332, #23712, #9177, #44564, #79119, #10070, #15998, #16885, #72740, #59082, #72300, #78690, #65473, #86820, #58213, #44113, #65030, #3260, #58640, #17771, #78239, #57763, #64585, #85500, #36877, #2367, #38212, #16437, #86374, #65908, #24587, #22818, #24147, #1916, #51819, #79570, #30068, #23281, #85942, #45010, #52252, #64142, #2814, #50945, #71853, #37326, #29613, #30509, #45445, #85048, #8741, #36442, #57302, #50492, #74970, #18662, #10946, #59972, #38651, #45892, #74521, #61326, #66352, #68162, #39095, #73169, #66804, #53599, #33636, #89049, #54041, #46341, #5034, #39992, #32733, #60425, #26810, #5944, #59528, #4591, #31836, #5492, #11854, #87266, #26372, #32276, #54491, #82255, #20014, #39547, #88173, #25930, #87705, #74069, #25472, #53142, #19108, #25030, #81365, #4136, #60887, #11401, #67250, #80914, #46790, #81800, #88616, #52693, #12300, #19552, #67708, #33188, #80452, #47242, #18211, #12756, #40442, #73625, #83149, #76313, #28607, #69955, #82705, #49484, #21354, #7722, #6373, #68612, #909, #54939, #40885, #77221, #70401, #13640, #89505, #49027, #27716, #27265, #42663, #7282, #63129, #1364, #84502, #20463, #55393, #35411, #21815, #63585, #76763, #34523, #34063, #62682, #48579, #61767, #56294, #48135, #75869, #41324, #42225, #84038, #14087, #69052, #20906, #14993, #8175, #55839, #35867, #29067, #75426, #56755, #41771, #14548, #47691, #34968, #6820, #62230, #455, #28149, #69506, #13200, #16, #83589, #49932, #43569, #16778, #58104, #30405, #3150, #85837, #22710, #15447, #65368, #58538, #23171, #1815, #29514, #23609, #84944, #85395, #8633, #36328, #64037, #57196, #77667, #71307, #9076, #70861, #50381, #78129, #51715, #51267, #44459, #36776, #43117, #15890, #64478, #2260, #37219, #30849, #29963, #37671, #57651, #22261, #79010, #50842, #78580, #16332, #44009, #86263, #71745, #72190, #9515, #9966, #64923, #2709, #24045, #69803, #49783, #22559, #7126, #7575, #42962, #70696, #48875, #41615, #8476, #34821, #76615, #62075, #77068, #49335, #1212, #42072, #57045, #55677, #14396, #89811, #83429, #21204, #76158, #62530, #305, #28002, #13489, #28452, #63425, #77511, #41174, #63889, #28918, #83891, #15293, #34365, #14848, #35261, #84790, #36173, #62970, #56136, #42516, #48421, #13937, #35713, #1667, #29368, #22114, #21663, #69353, #70245, #8019, #56603, #20749, #84348, #50233, #68904, #6670, #749, #27563, #55243, #82995, #39090, #66801, #3255, #25026, #60421, #59968, #10503, #45442, #31383, #38208, #53136, #87701, #25927, #73165, #25469, #31831, #59078, #53594, #32273, #67246, #4133, #52689, #10943, #17766, #38646, #80910, #4587, #17327, #24582, #52249, #45007, #86817, #3691, #80013, #72297, #87262, #18659, #46337, #10065, #32729, #74066, #80449, #11850, #30948, #73621, #66348, #81362, #5031, #59525, #18207, #11398, #72735, #65905, #39543, #88168, #19103, #37772, #45887, #65469, #58637, #86371, #24142, #79567, #51816, #20901, #7276, #61763, #26807, #20459, #34963, #41766, #54935, #13196, #12751, #13635, #55834, #26368, #5941, #40439, #33632, #74966, #68156, #76308, #54488, #6815, #48574, #62675, #60882, #75863, #39989, #34518, #48129, #81796, #61323, #34059, #62225, #69501, #12297, #40881, #89045, #54037, #19549, #67703, #82251, #20010, #33184, #47687, #47239, #83584, #10, #14081, #75422, #74517, #68608, #5488, #6368, #41320, #450, #88613, #28142, #89500, #46786, #27261, #82699, #69048, #27710, #55387, #83142, #43110, #7715, #22705, #69949, #36771, #29508, #64474, #77661, #57645, #30400, #14987, #15442, #50836, #78575, #56750, #49479, #16326, #42656, #84496, #35405, #84939, #57190, #9071, #49926, #64918, #63580, #22255, #63123, #904, #2256, #50377, #29959, #70856, #85390, #58097, #70396, #8628, #44003, #71739, #36322, #77216, #9510, #8169, #64032, #28601, #78124, #15886, #23165, #1810, #2703, #1359, #43564, #56289 ),
 ( #84033, #21809, #37214, #35861, #71303, #29061, #21348, #49022, #76758, #14542, #42220, #18543, #72184, #51710, #44454, #18093, #24484, #9961, #38985, #79461, #80793, #4922, #46228, #52146, #45339, #73059, #10398, #58970, #72633, #52586, #80344, #16773, #38540, #73963, #73509, #24040, #86707, #44904, #17224, #66694, #11280, #39439, #79908, #4480, #10834, #38103, #67141, #45782, #11740, #17663, #66234, #4024, #31276, #31727, #32168, #59863, #30843, #87595, #59425, #25353, #37665, #65362, #53025, #3144, #79004, #32612, #85832, #65793, #58532, #87156, #3579, #86257, #23603, #24923, #51261, #13975, #7170, #5371, #68045, #20351, #34408, #76196, #89395, #47126, #81250, #75310, #61220, #53485, #41211, #33519, #74863, #27155, #54828, #19000, #13089, #48457, #48024, #88505, #88941, #19443, #26257, #68938, #75760, #41654, #26694, #13529, #19895, #12637, #69392, #6708, #55280, #82146, #40774, #54376, #5831, #47576, #62116, #82594, #33069, #89850, #33955, #27600, #46684, #74414, #83039, #67594, #12188, #20792, #60313, #53935, #39873, #61654, #40324, #60769, #88049, #68499, #25812, #81693, #6265, #69840, #42551, #84825, #8967, #50725, #63923, #21700, #55718, #49821, #35751, #28040, #15775, #14437, #21242, #83465, #29404, #43452, #1249, #35295, #70279, #36665, #2144, #43000, #64369, #78006, #62565, #71192, #28956, #1699, #8513, #84385, #48912, #49374, #22154, #15327, #8056, #78463, #57083, #63464, #340, #77108, #29851, #22592, #50266, #85278, #57539, #790, #76651, #23049, #16222, #77546, #42114, #7612, #43900, #63008, #56638, #28489, #56178, #71634, #70739, #36210, #34860, #83928, #14886, #65255, #57988, #32848, #37992, #23496, #53713, #3033, #5612, #19674, #33304, #65688, #60090, #87826, #23929, #78902, #85721, #30290, #5151, #19231, #4710, #9851, #44798, #74637, #67820, #18778, #40104, #81480, #37108, #46907, #32388, #39660, #74198, #25590, #2594, #51602, #53263, #81033, #72526, #26486, #60543, #46461, #64813, #79352, #12414, #88291, #26046, #61002, #88731, #30732, #51161, #54159, #81921, #11976, #16660, #72079, #47356, #37555, #67360, #44345, #58427, #9399, #86154, #17113, #10287, #7832, #61439, #41001, #33750, #7389, #13754, #89169, #28263, #68721, #70064, #84159, #35527, #41439, #34642, #62346, #89623, #48249, #61891, #41885, #69621, #6062, #27826, #63251, #62787, #13315, #75981, #34185, #6487, #55958, #564, #28729, #69169, #83702, #126, #27379, #56416, #35080, #1026, #6940, #55504, #83257, #20582, #21018, #21473, #49147, #20132, #76883, #48696, #14664, #26939, #54607, #42334, #82367, #68281, #21933, #75085, #55057, #47805, #76426, #82818, #75542, #12876, #14205, #40561, #3270, #86383, #84612, #57312, #9628, #23722, #65484, #78698, #36450, #70521, #64596, #50504, #42778, #30520, #64155, #77784, #15562, #79131, #85059, #37334, #51382, #30961, #63702, #16447, #8292, #65039, #23290, #22370, #8750, #36887, #2823, #44576, #15103, #43688, #1928, #29182, #50047, #35988, #29624, #22826, #1482, #43235, #56870, #49602, #58222, #16897, #78250, #77328, #16007, #70977, #71425, #50953, #37785, #9190, #72308, #2377, #30077, #57771, #85512, #10081, #58648, #85951, #44124, #71863, #10518, #25483, #72749, #39558, #32286, #67261, #80464, #60439, #33198, #17780, #18223, #53609, #81375, #59541, #52261, #19120, #45458, #87275, #38223, #87714, #59984, #11866, #52704, #67718, #66361, #25041, #65916, #4148, #31848, #86829, #73178, #10956, #38661, #24159, #39108, #74083, #88183, #51829, #74534, #5045, #4602, #25939, #45021, #53154, #45903, #5504, #46801, #73634, #66817, #80923, #59093, #24598, #46352, #12310, #40003, #32743, #18671, #80026, #60899, #79580, #17341, #31396, #3703, #11410, #49042, #13653, #68622, #62240, #76776, #83601, #6834, #54950, #54504, #55406, #7735, #68175, #47701, #82267, #75441, #75881, #76323, #21368, #54055, #82717, #13212, #5957, #33646, #81814, #6386, #34075, #74982, #20025, #61337, #35426, #14102, #470, #61780, #26382, #40895, #19565, #89064, #27, #14564, #47253, #42238, #89519, #88628, #27275, #69064, #69966, #12766, #69519, #20478, #48146, #40455, #27727, #26823, #41783, #34537, #7295, #41335, #34980, #83161, #20919, #48590, #28164, #55851, #62693, #1375, #2721, #56766, #36340, #21827 ),
 ( #78141, #23185, #37230, #63142, #23620, #78592, #43580, #9529, #84051, #64496, #29527, #44471, #58116, #64049, #15900, #2272, #8186, #35879, #85410, #64935, #85848, #71761, #71319, #63596, #9087, #36788, #29974, #70417, #57665, #30419, #51278, #50853, #43129, #16344, #79025, #16791, #44022, #57210, #29079, #72202, #9977, #42677, #22271, #84514, #49946, #77678, #15460, #920, #70872, #28620, #56306, #49497, #77231, #15003, #8643, #1827, #84954, #22720, #50396, #37682, #31290, #18112, #88065, #53499, #18559, #73076, #59439, #24056, #39000, #86277, #53042, #45797, #80809, #4041, #73977, #46698, #58983, #31743, #67155, #4937, #10855, #65809, #32632, #86724, #38554, #51725, #11297, #73523, #25374, #66249, #81265, #79923, #87170, #79478, #17677, #45356, #10414, #24497, #52159, #24936, #65382, #52600, #87610, #11757, #3162, #25830, #46242, #66710, #39454, #58548, #4496, #80361, #19013, #60330, #32181, #59877, #74429, #72648, #38117, #30860, #17238, #44917, #3597, #27168, #74877, #48040, #82608, #13542, #19460, #20367, #76213, #62581, #54843, #82160, #75775, #357, #7183, #41226, #68512, #68061, #68956, #21256, #81709, #61234, #5846, #88956, #40343, #33534, #41670, #19909, #62131, #13989, #28054, #26273, #6725, #5388, #89864, #34422, #47144, #26710, #89410, #27614, #34871, #67609, #6280, #54395, #12652, #47591, #33087, #75326, #13106, #88519, #40790, #33970, #48926, #55296, #69408, #61674, #39892, #83054, #60785, #20806, #48470, #55734, #53949, #83482, #12203, #35764, #8073, #63476, #76669, #1715, #36682, #50741, #14451, #37125, #2158, #57095, #23069, #7625, #78022, #43015, #58005, #71651, #77560, #29417, #15790, #21715, #49386, #8982, #78476, #9413, #85293, #84838, #77121, #22608, #50280, #43465, #83944, #71206, #16239, #64826, #64383, #56652, #29867, #2608, #30309, #57551, #70753, #42562, #43915, #85738, #56191, #1263, #70295, #28969, #14898, #84399, #23512, #22166, #42127, #69854, #35311, #807, #63025, #28500, #49833, #15345, #8527, #36225, #63935, #38889, #46135, #16678, #45248, #10304, #30749, #86170, #44363, #31180, #58879, #37571, #44812, #58441, #87951, #66597, #52927, #86616, #78917, #38010, #72092, #23944, #52492, #39345, #9864, #73866, #17127, #51176, #72540, #31630, #11651, #67051, #32076, #24389, #72968, #65271, #80255, #3050, #4389, #59333, #59772, #17567, #87503, #60215, #65704, #10735, #80698, #18447, #52052, #79368, #4831, #3485, #79813, #51622, #24827, #87061, #25261, #38439, #32514, #66145, #3932, #18000, #45681, #73414, #11186, #34316, #82051, #26170, #61129, #89755, #82942, #33872, #55182, #68849, #53389, #62021, #19805, #54737, #89303, #75218, #18903, #40230, #12999, #6184, #88857, #41566, #47929, #54287, #81157, #67948, #27506, #13439, #75670, #76104, #41125, #81608, #46588, #48370, #69301, #40686, #32974, #88409, #6620, #53838, #47485, #67491, #5279, #82500, #68406, #61567, #7072, #13883, #12094, #19358, #74325, #20703, #27067, #39778, #34770, #47030, #62473, #25716, #60670, #20260, #74765, #12544, #5737, #26611, #33427, #56998, #84741, #21152, #42910, #78374, #77913, #28398, #63375, #49284, #56086, #71106, #15690, #43812, #1157, #43362, #49734, #77014, #71552, #50176, #85187, #22064, #70649, #28862, #35662, #56551, #8881, #22500, #35207, #2055, #63835, #36580, #48824, #76561, #64283, #7518, #83378, #29760, #22958, #83834, #42021, #1614, #70191, #69749, #50632, #77457, #57445, #9314, #37015, #62917, #7963, #16136, #249, #27952, #29315, #14795, #14342, #15235, #84293, #695, #55630, #21609, #42462, #8423, #36119, #78816, #3828, #57897, #24720, #38341, #9758, #23844, #51949, #52384, #59665, #30203, #58774, #51512, #44254, #37461, #85634, #44704, #72432, #51076, #58342, #71988, #11543, #80147, #66490, #10200, #2504, #79259, #23409, #65160, #66039, #52821, #16576, #87396, #30646, #64720, #86071, #45142, #25156, #80594, #45578, #37906, #86514, #2944, #31521, #17021, #17897, #72867, #73304, #31081, #11078, #73760, #65607, #24283, #4278, #31971, #3388, #79707, #18340, #17462, #10637, #59226, #86955, #38784, #46026, #67840, #82836, #81499, #40121, #87845, #19251, #46924, #11992, #88307, #60564, #26065, #39238, #54179, #89194, #13331, #66945, #89642, #54625, #19693, #75563, #60111 ),
 ( #75104, #47373, #40580, #46481, #12892, #41018, #27395, #81942, #74659, #68298, #55074, #34207, #6078, #5631, #5170, #33767, #48263, #18797, #53733, #32864, #12432, #67381, #33321, #68740, #61021, #26958, #6510, #61909, #20597, #88749, #81051, #61460, #26507, #74218, #75997, #82386, #20150, #4727, #32406, #39678, #47823, #25608, #53282, #30879, #44040, #582, #34658, #29995, #15919, #6958, #85865, #83272, #143, #62361, #9546, #23635, #71335, #14226, #50416, #79042, #72221, #23203, #44489, #58133, #41458, #51295, #9107, #71775, #78608, #64511, #27841, #29541, #2291, #85428, #78159, #58563, #37251, #43596, #69186, #57226, #16807, #2738, #64954, #65400, #30438, #69636, #55520, #37701, #86293, #57685, #21039, #76443, #9992, #41902, #36803, #48713, #7405, #3180, #50870, #16363, #24073, #51743, #35096, #62803, #84971, #13774, #22741, #3612, #32651, #73094, #74446, #88535, #12221, #18129, #39017, #66727, #4059, #52619, #66268, #46258, #73994, #10432, #32200, #67626, #67173, #17695, #80380, #38570, #45375, #60347, #4955, #33105, #45813, #88085, #4512, #31758, #60802, #39470, #39909, #11316, #59897, #73542, #24952, #87629, #25848, #11773, #24512, #81282, #53059, #53514, #38135, #65827, #19028, #86741, #72665, #80829, #31307, #46715, #25393, #5410, #18578, #26289, #79493, #10872, #17255, #44935, #59003, #52176, #59454, #79939, #87188, #27186, #12672, #27633, #89882, #41689, #82626, #7643, #6297, #54861, #40363, #33988, #61690, #26729, #13123, #75344, #40807, #53966, #68974, #14005, #28070, #81726, #14466, #69424, #34440, #375, #74894, #55314, #20387, #35332, #48944, #48057, #6741, #83070, #88973, #54412, #76231, #55753, #76686, #62599, #62149, #82175, #20824, #48489, #7199, #61251, #34889, #83500, #42143, #21271, #89425, #69871, #63044, #826, #19478, #75792, #19930, #47161, #68077, #33549, #68529, #47611, #13558, #41243, #5864, #58023, #36244, #78497, #2629, #44381, #42582, #57571, #21731, #16257, #2179, #63496, #77582, #15810, #43932, #23531, #83960, #22629, #15367, #8092, #1281, #49403, #8546, #63954, #14916, #22184, #35782, #65292, #71670, #30331, #1733, #56209, #43032, #77139, #28986, #29888, #16699, #70317, #51193, #84416, #28516, #49853, #8999, #78934, #72110, #9433, #29434, #50302, #56672, #70774, #85315, #23088, #57114, #71227, #9884, #37144, #84860, #78042, #43483, #36700, #64845, #85759, #37591, #64401, #50762, #52513, #79833, #74341, #52950, #87972, #24847, #45704, #3951, #38461, #31652, #73885, #25285, #38030, #4850, #66618, #80718, #51641, #23964, #46156, #10326, #86189, #32536, #25734, #58897, #44831, #4409, #72988, #72559, #53409, #80278, #18467, #46608, #39795, #65722, #10756, #11672, #67071, #18922, #32095, #17589, #79385, #18021, #59352, #17147, #39365, #3504, #31201, #86635, #87524, #60241, #87081, #24409, #66165, #81176, #12112, #11208, #3068, #30769, #58459, #52073, #73435, #59792, #45271, #38908, #60689, #82072, #54754, #47946, #40702, #83397, #89774, #6201, #32991, #19822, #13902, #55204, #27525, #27968, #82961, #33445, #88427, #271, #21172, #27085, #74784, #40251, #20718, #5754, #89322, #19375, #47050, #34334, #82519, #20281, #48841, #55646, #53856, #61148, #26188, #48388, #33888, #81625, #76122, #88873, #62492, #76581, #14362, #61585, #75687, #13456, #47503, #68425, #75240, #41584, #69318, #7092, #67512, #34786, #26629, #12564, #5302, #67968, #41142, #54305, #13015, #68866, #6638, #62040, #83852, #21629, #8898, #63851, #1634, #85649, #64738, #28420, #7982, #713, #64301, #70666, #56104, #85209, #35682, #37032, #51093, #2522, #8441, #29334, #57014, #56570, #15256, #28881, #36599, #2072, #62934, #84756, #30223, #29777, #70212, #42929, #1176, #63395, #22975, #57468, #23427, #36138, #50650, #22519, #84313, #78831, #78392, #57914, #50199, #77932, #15706, #77474, #43381, #16154, #43829, #77035, #71568, #71123, #9329, #49302, #14813, #42040, #42480, #35228, #69767, #7539, #22084, #49749, #3848, #3405, #30662, #31988, #17479, #80167, #80611, #46045, #86087, #31096, #52401, #38804, #25175, #31542, #10217, #9775, #72884, #86535, #37479, #73325, #58360, #65181, #2960, #86975, #11098, #51967, #51530, #58790, #66509, #4298, #38357, #59682, #17914, #44271, #87414, #79723, #59245 ),
 ( #23858, #79280, #17040, #24736, #24301, #44720, #45593, #72449, #52837, #18360, #16592, #45161, #10651, #66057, #72008, #37922, #65622, #64582, #2362, #28718, #50489, #85938, #85495, #35976, #70964, #56854, #63687, #78686, #23277, #51371, #8738, #50941, #57299, #84596, #79116, #57759, #2808, #29610, #78233, #36438, #43222, #64138, #16434, #30065, #42764, #9611, #71411, #44110, #56402, #84145, #71850, #15091, #1012, #37322, #30506, #1470, #49585, #9174, #77768, #77316, #58208, #85043, #65027, #16880, #44560, #70504, #15547, #23709, #7821, #35512, #36874, #22359, #21919, #22814, #1913, #8278, #63234, #29167, #50033, #15995, #43676, #51443, #71919, #30131, #2877, #65970, #3762, #9683, #64646, #31451, #57828, #37392, #85118, #10132, #72365, #24214, #65094, #80078, #78752, #30576, #22886, #16505, #44184, #9245, #85564, #23342, #51009, #36509, #79194, #86447, #10570, #64213, #86884, #51880, #16951, #72803, #57376, #37841, #58275, #17833, #59156, #86006, #44631, #38274, #79634, #58706, #24647, #17393, #2434, #50562, #52314, #45510, #23778, #43747, #36941, #45075, #65539, #3322, #78303, #16066, #31014, #73232, #1982, #29681, #71484, #87330, #66872, #59592, #33254, #39607, #25092, #54114, #4654, #6013, #20082, #33704, #67313, #60493, #88239, #25536, #74145, #87774, #67773, #5562, #31901, #53664, #89124, #88684, #39169, #11920, #60041, #32340, #81870, #26441, #54556, #5102, #19621, #25995, #53211, #82322, #60955, #61395, #32798, #81431, #19183, #46410, #46854, #47308, #75039, #45958, #12826, #74585, #40511, #52756, #80520, #68231, #18274, #4208, #26883, #47757, #80980, #73695, #12365, #18728, #11472, #11011, #40054, #38716, #66419, #22321, #20533, #83211, #35478, #49548, #1432, #14614, #62293, #6443, #519, #76380, #68676, #56366, #55004, #61835, #34137, #69569, #62743, #7343, #35936, #20972, #77281, #42730, #83655, #15057, #28678, #13264, #84108, #35032, #42286, #49099, #28216, #89571, #79, #55907, #21426, #48649, #29134, #7788, #14159, #40953, #27777, #41833, #21879, #63198, #48201, #70472, #76828, #974, #27330, #82772, #8241, #75935, #13707, #63651, #56814, #41393, #69122, #70019, #55458, #6887, #84564, #75493, #34589, #3658, #86781, #85010, #57721, #10032, #24112, #65867, #79082, #36839, #70928, #64991, #50904, #43185, #30912, #29574, #36401, #8701, #44079, #37284, #71812, #10472, #85462, #51779, #17293, #58171, #79531, #3219, #77737, #58602, #9582, #16845, #23674, #2776, #64105, #64549, #30472, #85901, #23239, #31352, #72258, #78650, #15511, #2328, #86334, #37739, #65437, #38174, #44973, #15956, #1876, #72706, #59043, #51335, #57263, #22777, #50000, #78197, #44523, #50451, #43637, #71375, #9142, #30028, #16401, #47199, #10909, #80415, #73130, #46753, #53102, #38615, #67670, #18169, #19515, #33593, #74935, #80868, #74034, #11814, #39059, #87668, #11358, #81325, #19068, #45411, #67210, #12714, #12256, #52657, #25433, #73584, #45852, #5449, #39951, #68118, #18623, #33145, #39511, #66766, #5899, #74485, #40405, #46301, #4995, #32695, #59936, #88128, #59492, #4552, #60390, #60840, #61288, #79980, #25887, #32238, #4098, #87225, #17734, #53558, #88575, #66310, #26331, #31798, #24551, #54004, #81763, #52214, #24994, #75826, #26770, #61729, #416, #77179, #82216, #84001, #54902, #89012, #82666, #69466, #49444, #14956, #69916, #34481, #20864, #75386, #28108, #47653, #14508, #7240, #35824, #42182, #14050, #62187, #20424, #55355, #28564, #56250, #89925, #27221, #21775, #48094, #27676, #13160, #62642, #34930, #76726, #83107, #42624, #41283, #48533, #40842, #69016, #6782, #89465, #13600, #76274, #41732, #54453, #55793, #48987, #63085, #19972, #70360, #7682, #83548, #35373, #68572, #21313, #867, #8134, #6335, #34026, #16296, #2672, #8591, #36287, #85799, #65333, #86229, #72154, #78541, #63999, #9475, #43975, #64891, #70815, #71709, #37635, #24008, #37184, #43529, #30372, #51683, #58503, #58066, #29931, #29475, #23572, #72604, #43076, #22674, #57155, #50347, #1776, #84904, #3111, #71271, #51233, #30810, #79430, #77625, #78977, #56714, #16741, #44420, #17190, #44876, #9930, #9042, #85358, #49894, #10369, #22219, #63541, #1321, #29028, #84458, #15410, #36742, #78086, #57616, #15849, #64442, #2220, #23129 ),
 ( #50802, #59392, #87122, #38072, #52994, #88017, #12158, #65761, #88473, #53453, #18512, #74385, #58942, #39407, #4449, #19417, #33040, #38954, #80760, #67113, #73029, #10800, #60287, #39845, #60734, #46654, #46197, #38505, #73933, #11713, #4894, #45312, #32584, #67564, #26226, #25779, #18064, #81221, #53905, #81666, #18968, #32137, #3996, #5346, #47097, #17633, #24892, #31696, #52558, #66206, #80318, #74833, #45746, #3548, #31243, #86680, #52114, #24451, #79878, #73478, #11252, #66663, #59835, #25327, #87567, #8828, #68013, #7910, #62866, #83327, #48776, #5799, #83783, #21555, #202, #7468, #21099, #50578, #29260, #15635, #49226, #40300, #641, #33487, #76507, #15180, #1998, #61190, #36527, #69699, #12611, #35155, #76958, #27902, #77404, #49680, #1559, #42412, #57392, #56035, #14743, #55579, #70140, #35608, #14290, #28340, #63325, #1103, #41963, #28813, #63782, #77860, #56496, #64227, #56943, #84239, #50123, #22009, #42857, #70595, #85135, #29700, #8368, #36067, #84685, #22447, #43309, #71054, #22902, #11029, #86900, #3337, #51028, #24229, #58722, #79654, #85581, #86464, #52332, #38733, #31031, #58291, #51895, #66437, #73248, #17411, #44650, #44198, #45093, #87347, #57845, #37407, #71934, #65110, #16523, #9702, #17848, #86022, #38289, #80097, #4224, #2449, #72818, #71500, #65987, #10584, #23357, #2894, #65555, #3778, #31916, #43764, #72382, #30592, #78767, #23794, #9261, #51460, #79208, #64664, #16966, #10150, #25108, #31467, #45525, #37858, #16084, #59172, #36955, #24667, #59611, #78318, #30148, #47773, #18743, #52771, #46428, #33269, #13279, #68691, #33720, #88255, #74602, #39184, #54127, #11488, #68247, #60972, #89589, #6029, #67789, #26012, #74160, #19198, #82338, #20099, #53681, #80997, #75508, #11936, #75056, #87788, #54571, #26457, #12843, #66887, #73711, #61410, #60057, #45976, #40969, #6459, #39624, #4673, #81884, #32813, #32354, #34151, #12380, #89139, #61850, #80535, #25551, #60509, #40526, #26897, #18288, #19637, #67328, #53227, #5577, #81448, #5117, #46867, #40071, #88700, #47324, #21445, #14629, #49114, #77750, #62758, #1450, #84577, #35493, #56829, #70486, #55022, #35954, #76844, #56385, #990, #42302, #20548, #41848, #70035, #7802, #532, #43200, #49564, #55925, #82787, #69587, #63668, #15071, #77296, #15524, #42746, #83223, #48215, #50015, #70944, #63213, #34607, #96, #8254, #55472, #28697, #69137, #6903, #84124, #21893, #29148, #8717, #36419, #13724, #20988, #75950, #22335, #83671, #41409, #64119, #48666, #27347, #62310, #27793, #76396, #14175, #7358, #35048, #28231, #78664, #58614, #86353, #22791, #44538, #79994, #79546, #30042, #65007, #50919, #57737, #72718, #17309, #45423, #2791, #44987, #51351, #16415, #73142, #51792, #86795, #23687, #72276, #30487, #37300, #58186, #10484, #71391, #44090, #85476, #71826, #23252, #9594, #31366, #85916, #38185, #65879, #17748, #15971, #30925, #85023, #3671, #65450, #36850, #79097, #16858, #59055, #24564, #57280, #10046, #37752, #9153, #64563, #50467, #3232, #24123, #78211, #52230, #2342, #38627, #10924, #1888, #29587, #43653, #53115, #4113, #39072, #67683, #54467, #59506, #61304, #32253, #66326, #59948, #46764, #26781, #82232, #47218, #11827, #88141, #52669, #5462, #25007, #81774, #74496, #13172, #19526, #81342, #39523, #87679, #32708, #5917, #33608, #67225, #4566, #89023, #25448, #5007, #80427, #39966, #12271, #54016, #60402, #19985, #18638, #25904, #18184, #46318, #74046, #66779, #80883, #53572, #19081, #31811, #33160, #26348, #40418, #87242, #47668, #74947, #60856, #12727, #45865, #88588, #68132, #75401, #73597, #11378, #83561, #69929, #75840, #13612, #63095, #42635, #63553, #49455, #55806, #41297, #76738, #21327, #42198, #48106, #48998, #14968, #1339, #14520, #20877, #7695, #29041, #35837, #35383, #7255, #6792, #882, #49906, #41742, #84012, #429, #27689, #22235, #28576, #56726, #62655, #56265, #69479, #76289, #34942, #21787, #77196, #69028, #70370, #8146, #84472, #89477, #61742, #77637, #34492, #34036, #40857, #68585, #62204, #82678, #6349, #48545, #20437, #27236, #28118, #54915, #55098, #55367, #83119, #14060, #65343, #79439, #31253, #44430, #2232, #36303, #30380, #16309, #8605, #86239, #84915, #1789, #64011, #9483, #2681 ),
 ( #43985, #58951, #57626, #71718, #29486, #85367, #23141, #78095, #64451, #36752, #29942, #15422, #58075, #3120, #17202, #43087, #65773, #30822, #85811, #51692, #57169, #16749, #37196, #86688, #10378, #64899, #23582, #72165, #50356, #15863, #37645, #44885, #38081, #24016, #51244, #43541, #78985, #9940, #58513, #22686, #72615, #3557, #24460, #52127, #50816, #70830, #71283, #9053, #78552, #46208, #45757, #46663, #88926, #59402, #38965, #73488, #66674, #18072, #11264, #19425, #87578, #39855, #10811, #4905, #80772, #73038, #60746, #87136, #66217, #38514, #73945, #67124, #11723, #40308, #25335, #53915, #47108, #88026, #74843, #33048, #17643, #88484, #39417, #18980, #53462, #32594, #4005, #4460, #60295, #25790, #53002, #5813, #12171, #18522, #45321, #32149, #26240, #67574, #5355, #68022, #81675, #59846, #31705, #12622, #33500, #81233, #24904, #52569, #61201, #74394, #26680, #80327, #79889, #21227, #76181, #13957, #8039, #77094, #40756, #20338, #13069, #76637, #83017, #68478, #7599, #48004, #49358, #63451, #14873, #20774, #41640, #69376, #68924, #27587, #41199, #48900, #14418, #75293, #7151, #42539, #42099, #82578, #55265, #13513, #75741, #35283, #69826, #35735, #48442, #62993, #34846, #6690, #1237, #774, #70268, #62552, #326, #28023, #89834, #55703, #28473, #56166, #89375, #83915, #83450, #21684, #6252, #33942, #54357, #61638, #47562, #82126, #19880, #34391, #27140, #54814, #62101, #8499, #23917, #78448, #44329, #72512, #65674, #63911, #36652, #78888, #3015, #44783, #57968, #15762, #22580, #36196, #28940, #72062, #30718, #64353, #56625, #43434, #84369, #1686, #30279, #17099, #22141, #51589, #84813, #49807, #50252, #9385, #79334, #10274, #9837, #2131, #50708, #15315, #85706, #77536, #37543, #37094, #42981, #65241, #43887, #29836, #77990, #85267, #58413, #86141, #57524, #57069, #37976, #71180, #23032, #70726, #2583, #64795, #16648, #16210, #29388, #8954, #71620, #23481, #51149, #73385, #66117, #52466, #24797, #80223, #3460, #18417, #53362, #67466, #31155, #53810, #18875, #73836, #39751, #24358, #4802, #59742, #74737, #88382, #4357, #46106, #32487, #38414, #3903, #25683, #5248, #26143, #12064, #11623, #31600, #39313, #67020, #60186, #10707, #87918, #32938, #81576, #81128, #11155, #46559, #19323, #46999, #74292, #87476, #59300, #60641, #12516, #72935, #17969, #87032, #45653, #38863, #66567, #40196, #32047, #58851, #86586, #52025, #17542, #79784, #45219, #25232, #52895, #80668, #27036, #55150, #55597, #62884, #33397, #61987, #54705, #47455, #12966, #61098, #47897, #75641, #54251, #48339, #14309, #88827, #69264, #34283, #49244, #660, #68818, #20672, #7041, #40655, #68376, #219, #69719, #28367, #76525, #82912, #6154, #13853, #76072, #34737, #75187, #41534, #41985, #56055, #62444, #13411, #27920, #83802, #21577, #83348, #89727, #33843, #21121, #76981, #61534, #82473, #89271, #20227, #41095, #6589, #7491, #27476, #48794, #35173, #14764, #82020, #67918, #26579, #5705, #19773, #77425, #1578, #29722, #30166, #37429, #7929, #36546, #29280, #22032, #15198, #35631, #22469, #50145, #28834, #36089, #49702, #80444, #57867, #44215, #77878, #70157, #56965, #63345, #42880, #43783, #30613, #1122, #65131, #8390, #42434, #63801, #22920, #2913, #58315, #23379, #15653, #64245, #56515, #71519, #84258, #85600, #50600, #70613, #51048, #57417, #43333, #84706, #8848, #71959, #9724, #71074, #2019, #86042, #85152, #78341, #16104, #9278, #36978, #78785, #64689, #25020, #2471, #16540, #52684, #60415, #88159, #80900, #67241, #39537, #5024, #18200, #33176, #68147, #82244, #45879, #68599, #33622, #39085, #19542, #74511, #89491, #13188, #19095, #60872, #47231, #53130, #18651, #40431, #19999, #40871, #26799, #88604, #46331, #54029, #26361, #74958, #25463, #81788, #47680, #6361, #12741, #25919, #5932, #34052, #61755, #61316, #12291, #74060, #89038, #27251, #87696, #32722, #11841, #53585, #81356, #46778, #75414, #39981, #54481, #54927, #73611, #32267, #11391, #66794, #4581, #59962, #67696, #5478, #69940, #70386, #77653, #48120, #76750, #41756, #62217, #27701, #75854, #62666, #442, #69041, #76301, #1, #29500, #8161, #84487, #28134, #20450, #69492, #13626, #55379, #84025, #70845, #41312, #15434, #48564, #82690, #14072, #63114, #43101 ),
 ( #22248, #49918, #55825, #20892, #8618, #7268, #83575, #6805, #56279, #28590, #35851, #21340, #36314, #34954, #49013, #34508, #14534, #42212, #83134, #7707, #35397, #896, #21800, #49470, #42648, #56741, #77208, #64024, #63568, #14979, #29054, #1351, #1801, #86700, #24476, #2694, #85381, #52139, #50828, #30392, #15877, #30836, #3135, #44896, #85825, #10827, #9501, #58089, #43554, #37209, #64910, #29953, #16320, #78566, #43997, #57183, #72177, #17216, #31268, #84929, #17655, #72625, #37657, #3571, #78113, #58525, #23595, #38531, #79899, #51255, #9952, #86251, #2248, #57637, #79453, #58963, #45332, #65787, #65354, #23156, #24032, #51703, #10390, #64466, #38095, #73051, #66228, #4017, #78998, #22697, #50368, #71295, #9064, #16764, #71732, #36763, #44446, #45774, #87589, #32162, #25347, #4473, #59857, #19437, #18535, #67588, #53929, #68036, #80338, #74408, #24916, #5366, #18993, #11275, #53018, #60307, #33061, #47121, #87147, #67136, #80787, #73502, #38979, #59417, #46221, #73957, #18086, #11734, #66687, #61213, #60761, #81687, #39432, #52580, #4916, #32606, #88042, #46677, #40318, #25805, #74856, #53477, #31719, #12631, #81244, #12183, #39867, #88497, #26251, #5824, #33512, #24324, #71594, #38382, #31122, #59707, #66084, #37947, #58385, #37511, #59270, #10677, #45187, #73353, #72909, #78861, #43860, #45619, #66536, #72477, #30249, #85675, #3875, #51118, #44748, #64765, #2551, #79750, #10242, #65646, #4326, #11123, #9355, #16618, #37062, #31566, #51559, #57942, #86999, #44299, #17940, #32012, #38831, #79306, #3431, #58822, #65210, #86113, #9801, #17507, #24761, #23453, #86559, #23002, #52431, #72032, #23887, #2986, #30688, #80191, #50679, #78418, #17064, #16180, #51991, #74260, #68786, #47421, #82434, #19293, #40162, #88349, #32908, #26108, #68339, #19736, #32453, #89237, #61062, #75147, #46068, #18384, #40623, #4767, #80636, #27002, #20193, #53325, #39281, #88795, #67426, #66986, #47868, #46965, #12933, #41061, #34252, #60150, #5215, #6120, #61502, #13376, #26547, #12032, #73805, #12482, #53778, #11591, #33811, #87888, #25651, #81093, #81543, #74699, #67883, #75607, #60607, #54669, #6553, #5672, #87442, #25199, #52862, #18844, #33363, #54220, #81982, #46525, #39716, #76491, #49210, #42397, #35139, #77845, #84223, #626, #27439, #41502, #56930, #21539, #77387, #15621, #8812, #7002, #69680, #21993, #36049, #43293, #1085, #48761, #82880, #76943, #62849, #55117, #42841, #69234, #48305, #20641, #56018, #14723, #83768, #22432, #7451, #63765, #29245, #70122, #1543, #15163, #89687, #70580, #7894, #28797, #35593, #63310, #76038, #14273, #56478, #49662, #28325, #71035, #8353, #84666, #13818, #41947, #50107, #61953, #34698, #62406, #184, #27887, #55562, #83313, #21082, #44867, #2666, #64883, #72148, #66653, #80310, #86223, #38064, #24442, #30365, #58060, #17624, #87114, #18057, #3988, #10361, #85790, #31234, #65752, #86671, #23563, #3540, #59382, #45735, #58930, #65327, #52104, #73466, #11244, #79870, #51673, #51226, #45304, #4440, #78971, #44410, #16732, #9922, #37627, #3104, #24883, #30801, #73021, #52549, #38946, #9465, #10791, #78532, #38495, #66195, #58494, #24000, #72596, #31687, #32128, #50794, #79422, #17182, #85352, #23122, #16288, #43968, #71703, #37174, #53443, #67103, #6673, #75276, #61621, #5336, #87557, #88462, #40733, #82106, #4883, #89356, #33478, #19856, #18504, #80747, #13051, #32575, #52985, #27118, #82557, #25768, #11704, #61181, #39835, #39397, #54795, #19406, #68459, #13491, #59826, #60277, #67553, #47544, #33923, #75720, #88908, #46644, #46189, #74822, #60723, #73923, #6233, #88006, #81210, #18960, #53896, #47087, #81657, #20319, #33031, #47985, #41177, #68004, #68906, #25320, #74375, #12147, #12600, #26661, #54340, #40292, #26218, #5787, #21664, #14850, #7577, #50235, #56605, #62971, #89813, #48877, #70699, #22116, #84349, #84791, #49784, #308, #55246, #57046, #77967, #83894, #62079, #42517, #751, #62531, #56140, #76162, #13939, #1216, #49337, #77069, #15742, #22561, #20751, #28003, #82998, #77512, #28453, #48423, #15296, #55678, #29370, #43415, #71160, #70247, #8020, #35714, #76618, #35263, #21206, #28919, #42963, #41620, #63428, #34369, #8479, #83431, #36175, #14397, #42073 ),
 ( #63890, #27565, #1669, #69357, #7128, #34823, #69804, #86123, #2995, #59280, #44309, #72916, #66096, #17072, #38389, #52001, #36634, #17518, #30696, #37955, #72486, #58393, #2104, #23461, #23894, #79314, #72039, #24774, #31132, #37522, #64334, #51129, #45199, #86567, #58831, #87006, #24333, #64775, #29816, #31575, #52442, #51568, #57505, #44761, #65221, #37071, #10254, #50686, #78428, #65654, #3438, #79760, #80204, #17948, #85245, #2560, #23013, #10684, #3882, #16191, #45627, #30262, #8936, #43868, #71602, #9363, #57949, #85684, #78869, #9812, #16626, #40175, #67893, #4335, #26120, #61512, #61075, #11601, #46537, #32464, #39293, #54229, #88806, #27012, #74272, #26558, #32917, #60163, #54681, #33372, #68350, #5229, #53788, #12041, #18853, #39728, #81991, #5684, #18393, #75161, #46974, #19749, #32022, #59720, #47431, #80647, #66547, #12945, #6133, #66996, #25212, #74711, #53336, #52871, #33822, #60617, #40632, #82444, #20207, #46081, #81108, #89246, #73363, #11134, #12493, #87898, #87453, #38839, #4780, #73816, #25660, #67437, #88361, #81555, #19303, #76502, #76049, #69693, #89699, #27451, #14737, #7463, #35151, #1555, #70591, #34262, #13827, #6563, #70135, #14284, #61962, #1097, #41513, #42851, #56940, #8363, #41959, #62861, #636, #62417, #21094, #34714, #42408, #7905, #68795, #28335, #36062, #35603, #69243, #48772, #7012, #197, #28808, #63321, #29256, #56031, #56492, #83778, #27898, #84680, #84234, #63778, #21551, #49222, #76953, #83323, #22004, #49675, #77399, #82890, #15175, #47877, #75617, #55128, #20651, #13386, #48315, #41074, #55573, #45089, #78315, #64224, #86019, #2446, #1994, #17408, #71930, #37854, #65983, #59167, #57388, #30144, #72378, #86460, #38286, #51456, #9257, #43305, #37404, #23354, #15631, #3334, #29695, #8824, #71051, #16519, #9698, #44195, #72814, #57840, #24226, #79649, #30588, #51890, #65551, #50119, #31028, #65107, #79205, #23791, #2890, #36523, #36952, #58287, #16963, #85578, #3774, #44645, #51024, #77856, #64660, #58718, #10147, #10581, #31464, #22443, #85132, #22897, #50574, #16080, #78764, #43760, #71497, #60054, #12837, #19195, #25547, #52328, #11485, #33265, #74598, #46864, #47320, #12376, #52767, #17844, #19633, #40522, #46425, #24663, #67325, #53224, #25105, #18739, #38730, #66432, #53678, #74157, #11932, #68244, #75053, #73244, #80531, #45522, #40067, #80993, #11025, #67785, #18285, #81881, #6026, #33716, #39620, #5114, #32808, #39181, #87784, #73707, #81444, #5572, #4220, #60506, #86896, #60969, #45973, #88250, #66883, #4668, #88696, #26454, #80093, #26008, #54124, #31913, #32351, #59607, #87344, #56381, #83220, #14172, #62306, #6900, #93, #42298, #83667, #6456, #63209, #35044, #21442, #20095, #82335, #14626, #68687, #54568, #987, #84120, #27342, #13275, #62754, #41405, #40966, #21890, #20985, #76840, #15068, #8251, #34147, #69133, #49110, #35490, #77293, #529, #48212, #47768, #76393, #27788, #75505, #70032, #61846, #89586, #55018, #55469, #48661, #41844, #49560, #34603, #28693, #42742, #69583, #70482, #7798, #89136, #61407, #26893, #82783, #20544, #7355, #28228, #55921, #75947, #13720, #22787, #2786, #30484, #56825, #78659, #25330, #23684, #64115, #9150, #85020, #1885, #16855, #51348, #80764, #36847, #79093, #85472, #50464, #18516, #85912, #32142, #57733, #16412, #64559, #71387, #2339, #44535, #58182, #70940, #38957, #9591, #72273, #84574, #22332, #11257, #43197, #29145, #66668, #59840, #29584, #77746, #37297, #15968, #15521, #87571, #23249, #4454, #46202, #73938, #8713, #43649, #52997, #35951, #63663, #65004, #78207, #50012, #50916, #30039, #36416, #1447, #57277, #44087, #71822, #5805, #88920, #33492, #62094, #47102, #75733, #68918, #19872, #41194, #54808, #39410, #20332, #61195, #40747, #75286, #26675, #4899, #26233, #54352, #82120, #74837, #27579, #33936, #40303, #67118, #53908, #47998, #89368, #61633, #89827, #27132, #67567, #32587, #34383, #55259, #47555, #60290, #13063, #68016, #39849, #68471, #53456, #81227, #6247, #82570, #13506, #83011, #20767, #88020, #5349, #25782, #6685, #48436, #18973, #11717, #33043, #46657, #74389, #12164, #60738, #88477, #81670, #19420, #12614, #71176, #84363, #42532, #42092, #42976, #85261, #55696, #35278, #69820 ),
 ( #63443, #63905, #8948, #41634, #70263, #62988, #83444, #21221, #69370, #56158, #83908, #62544, #7591, #48892, #23027, #1681, #77983, #21678, #13950, #767, #7144, #76631, #77529, #64349, #34840, #36647, #28466, #76176, #49352, #56619, #2126, #29831, #57064, #77087, #8034, #320, #15310, #28018, #29384, #22134, #14413, #84808, #1231, #14866, #35728, #28933, #15755, #43428, #49801, #70716, #57517, #8493, #36191, #22574, #50247, #86579, #38407, #79327, #4350, #3010, #51581, #9381, #30711, #58406, #23474, #9829, #72055, #37536, #50701, #65667, #10700, #24790, #78442, #11148, #66111, #31149, #10268, #57963, #30275, #65235, #32039, #45646, #17089, #3453, #79776, #85699, #51144, #72929, #52458, #73377, #59294, #58844, #78883, #24349, #52018, #17534, #16644, #86136, #44323, #23912, #44776, #72503, #80217, #37969, #3895, #17963, #66560, #64789, #45212, #43881, #31591, #87024, #38853, #59734, #87468, #16205, #71616, #37089, #2574, #74285, #4795, #60180, #80661, #5242, #32931, #11615, #18867, #32479, #61978, #40646, #27028, #60633, #52888, #12057, #18407, #87912, #26571, #13401, #46097, #20220, #81122, #25226, #46551, #5697, #75632, #41088, #6146, #88374, #46991, #39307, #54244, #73829, #68366, #33387, #67012, #33835, #40188, #26136, #39744, #81568, #54696, #82462, #53802, #53352, #47891, #67457, #19317, #25674, #88818, #61090, #12959, #74729, #68810, #12508, #67909, #82010, #19765, #47444, #75177, #61526, #89262, #6579, #34276, #14755, #49693, #63792, #89716, #50135, #15190, #70149, #49236, #7030, #69257, #76516, #71066, #84697, #652, #42424, #28824, #34729, #62434, #22022, #1568, #22459, #8379, #7921, #212, #35621, #63336, #1113, #27913, #56506, #29270, #77871, #84248, #69710, #77415, #15645, #43322, #42870, #56047, #55589, #70605, #8837, #83339, #36079, #56955, #36537, #21112, #27467, #55142, #82904, #20664, #7480, #48330, #76065, #13844, #41526, #83792, #48786, #14301, #41976, #35165, #62876, #28355, #21566, #76970, #2461, #3791, #71949, #24240, #38301, #80110, #78331, #3351, #57405, #51908, #37870, #9270, #23369, #51471, #79667, #59182, #29713, #58305, #51040, #43775, #36968, #85145, #44208, #9716, #50589, #57857, #71510, #11044, #17424, #65999, #37419, #2009, #78777, #22912, #64679, #65568, #52345, #16095, #86915, #30157, #64237, #85592, #44662, #24679, #17861, #45104, #65122, #86035, #16532, #31043, #2906, #72830, #72396, #30604, #10597, #79221, #23804, #16979, #10161, #31478, #45536, #58733, #86477, #73260, #32368, #11951, #87361, #12392, #74612, #26468, #67339, #82349, #81009, #39636, #25121, #18755, #46439, #11501, #87800, #60068, #25566, #38745, #53691, #88710, #12853, #66447, #89148, #54138, #19209, #88266, #45989, #18303, #53240, #20108, #33731, #5127, #81458, #67800, #73721, #39195, #60984, #40539, #61421, #47338, #46881, #81896, #26026, #74172, #47785, #19648, #26910, #60520, #40084, #32827, #5587, #33282, #75066, #68261, #66902, #6042, #54586, #75520, #52782, #59623, #4236, #4686, #31930, #80548, #35965, #69148, #55035, #76858, #83237, #82799, #8268, #62768, #28706, #56841, #50023, #48228, #20998, #63225, #77308, #29157, #42313, #106, #34161, #28243, #14185, #6468, #84136, #20559, #89600, #61865, #7370, #544, #35057, #63676, #48674, #15082, #70496, #21454, #42756, #56393, #40982, #21906, #55936, #70045, #14641, #83681, #27358, #27803, #49122, #7813, #76407, #84587, #35503, #41859, #68702, #55483, #49574, #1002, #1461, #22351, #13292, #6915, #75963, #13733, #41418, #34617, #62324, #69599, #16427, #15985, #9603, #29601, #57291, #44549, #37313, #65017, #31375, #10495, #64128, #43665, #36429, #10056, #44103, #1901, #30940, #71401, #72727, #86806, #38200, #71839, #2800, #30498, #2353, #50931, #64572, #72288, #37764, #8727, #58199, #65896, #65462, #9166, #78675, #36863, #30054, #58628, #3246, #59068, #85929, #22804, #50479, #86364, #79557, #3681, #24134, #23700, #78223, #51364, #79109, #16870, #85033, #51805, #17320, #24573, #44998, #57749, #77759, #15537, #43212, #70954, #85486, #23267, #19092, #61314, #31821, #11388, #18197, #39082, #80441, #45876, #81786, #59959, #12288, #26358, #68145, #66338, #81353, #45435, #39977, #25916, #87254, #66791, #39533, #67693, #47229, #17758, #46328 ),
 ( #74956, #11838, #5475, #5930, #89036, #25017, #87693, #33173, #54027, #33619, #46775, #4577, #73158, #67238, #53127, #10934, #60869, #59517, #38636, #4124, #74057, #5021, #32718, #12739, #25459, #19539, #40429, #60412, #52242, #88600, #80004, #52681, #88156, #74507, #53582, #73608, #32264, #80897, #18648, #7266, #2943, #42646, #49011, #55377, #82242, #41310, #63112, #14530, #76748, #77206, #42210, #82688, #47678, #49467, #70384, #76299, #54478, #34952, #83132, #54925, #48561, #68596, #6359, #83572, #14070, #69039, #27699, #13623, #21338, #69938, #75412, #69489, #14977, #7705, #20448, #20890, #75852, #48118, #35395, #894, #8159, #41754, #28587, #62664, #6803, #35849, #56277, #21798, #440, #28132, #55823, #62215, #84023, #63565, #26797, #61753, #19997, #13186, #40869, #34050, #89488, #27249, #34505, #84484, #3133, #24030, #57181, #71730, #78563, #57635, #85379, #86249, #50826, #16762, #44894, #38093, #36312, #9062, #51253, #65352, #17214, #30390, #78110, #22246, #16318, #2246, #49916, #72175, #70843, #77651, #15432, #23154, #43995, #9498, #51701, #36761, #30834, #58522, #37207, #79450, #44443, #29052, #9950, #64908, #58087, #2692, #85823, #43099, #15875, #23592, #78996, #64463, #72623, #37654, #29951, #56739, #43551, #10388, #1349, #8615, #64022, #1799, #84927, #29497, #22695, #50366, #71293, #3568, #46219, #4470, #4015, #87587, #17653, #45330, #32604, #25345, #53016, #19434, #88494, #52137, #31717, #24473, #88039, #32160, #79897, #18991, #59414, #60759, #74854, #26249, #59855, #80785, #18532, #53927, #25803, #87145, #86698, #81685, #47119, #73955, #31266, #11732, #39429, #24914, #67134, #73049, #10825, #60305, #4914, #53474, #12629, #65785, #38528, #52578, #66226, #81242, #46675, #80336, #74405, #18084, #58961, #45772, #73499, #12181, #39865, #67586, #11273, #38977, #66685, #5364, #33059, #61211, #83030, #29729, #29284, #68489, #13522, #89386, #6259, #22473, #56970, #85156, #41205, #84709, #89843, #27149, #22925, #1583, #36549, #62110, #20785, #68932, #75752, #6701, #50149, #63804, #75303, #43335, #13969, #77882, #88935, #26688, #15657, #47569, #33509, #71077, #64250, #33949, #48450, #27594, #34400, #55273, #2025, #76190, #8851, #50602, #78344, #13080, #48014, #57420, #40316, #68034, #69386, #54821, #54368, #41649, #7163, #82139, #5822, #19888, #40766, #61647, #34854, #82587, #20345, #66458, #51484, #80120, #73276, #24250, #45545, #59194, #43785, #24689, #10172, #45115, #79678, #65579, #9283, #30616, #3362, #86487, #79232, #31944, #38313, #44674, #71523, #58317, #52357, #3803, #66011, #86929, #85602, #2474, #36986, #37880, #31052, #58745, #4247, #16993, #17871, #11054, #51921, #38756, #59635, #64692, #87371, #17434, #72841, #10605, #31489, #30171, #86045, #25132, #52792, #72408, #16106, #57870, #23382, #51050, #23815, #78788, #16545, #44222, #71964, #9727, #37433, #65134, #2917, #34176, #40097, #18317, #60995, #19221, #18769, #12406, #32380, #60082, #47350, #67813, #5600, #61883, #13306, #66918, #46452, #39207, #12868, #46898, #4698, #33743, #74186, #75532, #89614, #40994, #74627, #33295, #88723, #5143, #53705, #67352, #75079, #40551, #11512, #26479, #68715, #68274, #11966, #81471, #39649, #32841, #61433, #6055, #27371, #54151, #89161, #81913, #60533, #80562, #26930, #6481, #19664, #54598, #82361, #26038, #20124, #47798, #45999, #25579, #73733, #87817, #53254, #81023, #88281, #8285, #62338, #48241, #56861, #77778, #21012, #35518, #42326, #21467, #49137, #50040, #14655, #70512, #8743, #1920, #120, #62780, #15097, #29174, #70971, #84151, #41876, #75975, #70058, #55951, #13748, #76875, #21926, #28723, #7826, #41433, #69612, #63244, #1019, #28256, #36444, #77321, #83696, #20572, #7383, #1475, #42772, #35982, #15553, #63694, #48690, #69161, #43228, #64145, #56408, #82811, #49591, #84602, #83250, #22364, #6932, #34632, #55050, #27818, #55494, #76420, #14197, #35072, #555, #50494, #37778, #37328, #16000, #58642, #30071, #72742, #31390, #10509, #65033, #30511, #58215, #50947, #71856, #23283, #10073, #72302, #22820, #85944, #38215, #3262, #2371, #9620, #85502, #57765, #86377, #30954, #3697, #2815, #24151, #23715, #78692, #59085, #65475, #45013, #51376, #79123, #16890, #44116, #44566, #51822 ),
 ( #79572, #17334, #65910, #29615, #57306, #85053, #78241, #16440, #43682, #71417, #9181, #36880, #64588, #7677, #41725, #35817, #21769, #14044, #1767, #411, #7235, #69458, #14950, #8125, #42619, #71264, #56244, #84895, #78079, #29023, #50340, #63992, #48524, #29467, #69908, #42177, #35368, #20856, #63533, #70807, #22665, #76265, #9035, #36281, #1315, #70352, #28102, #55785, #63078, #2212, #15840, #49437, #56708, #49889, #83537, #21307, #43069, #43521, #36734, #57149, #84450, #48981, #22214, #77618, #15401, #76719, #8581, #64434, #29920, #57609, #857, #34925, #62635, #14502, #28555, #77173, #83995, #15339, #3044, #29861, #77554, #50734, #36674, #43459, #58435, #65265, #31175, #78470, #30742, #37119, #64377, #58874, #37565, #72534, #9407, #30303, #16233, #23061, #43909, #86164, #9859, #22602, #79363, #51170, #23938, #36219, #8521, #51614, #84832, #70746, #17121, #10298, #71200, #57998, #64820, #71643, #2602, #38004, #85731, #44807, #86609, #24384, #50274, #85287, #65697, #3481, #43008, #16670, #2152, #63929, #23506, #78911, #1707, #29411, #57089, #78015, #15783, #44357, #72086, #8976, #57545, #87498, #26165, #19353, #60210, #81602, #5273, #79808, #60664, #46130, #81152, #25710, #11645, #45243, #66590, #39339, #32509, #25256, #67943, #74320, #80693, #53384, #67046, #72963, #4384, #4826, #87945, #52922, #5731, #12089, #18443, #17562, #32071, #88403, #39773, #67486, #12538, #32969, #17995, #10730, #74760, #33422, #18898, #38434, #46581, #73860, #80250, #53833, #3927, #31623, #47025, #40225, #61123, #88852, #52047, #66140, #45676, #59328, #87056, #24822, #52487, #73409, #11181, #38885, #59767, #49279, #55177, #76100, #13879, #41121, #89751, #13435, #83375, #21148, #47480, #54282, #42017, #68845, #26605, #27501, #75665, #82496, #7514, #14338, #70187, #82938, #69745, #41561, #6615, #7959, #76556, #21604, #48366, #69297, #20698, #62017, #7068, #35203, #48820, #61562, #28394, #245, #62913, #75213, #12994, #690, #33867, #19799, #56082, #77009, #20255, #34765, #62468, #27948, #55625, #14791, #83831, #42458, #35657, #63371, #89299, #34312, #82046, #40679, #68400, #6179, #27063, #54733, #47924, #2052, #84288, #71985, #70644, #77453, #22060, #85184, #78370, #22955, #51508, #36575, #65157, #58339, #9312, #30641, #44251, #28858, #9755, #50628, #30200, #16132, #8420, #29757, #77909, #56995, #15686, #29312, #84738, #86068, #8877, #51073, #2940, #17018, #15231, #57894, #49730, #78813, #64717, #36115, #50172, #43810, #16572, #23840, #56545, #71549, #43358, #63830, #1608, #42907, #71104, #64279, #22497, #57442, #37012, #37902, #37458, #2501, #85630, #23405, #79256, #44701, #72429, #10197, #1153, #58771, #60559, #31517, #65603, #59223, #46023, #26061, #81494, #46477, #11075, #87393, #51946, #66941, #24280, #81048, #73757, #12429, #18793, #80590, #38780, #86952, #31968, #5167, #32861, #66486, #3825, #88304, #24717, #4274, #79704, #39235, #11538, #53279, #59661, #19248, #17894, #25153, #17459, #45574, #73301, #38337, #52380, #80144, #52817, #3385, #18337, #25604, #39675, #31078, #53730, #74214, #4724, #32403, #72864, #45138, #60107, #46921, #74655, #87842, #11989, #67377, #10633, #66036, #86510, #41899, #62801, #48711, #55070, #12889, #75995, #20595, #41455, #47370, #48261, #14223, #580, #82834, #20147, #13771, #28280, #35094, #69184, #6506, #6075, #49165, #55973, #68737, #89638, #27392, #54622, #13327, #26954, #6954, #34656, #61018, #67836, #55518, #82382, #40118, #41015, #89190, #33764, #21036, #27839, #83715, #34204, #83270, #62358, #47819, #21490, #141, #76896, #61905, #76440, #69633, #75560, #7403, #5628, #33317, #75100, #88745, #26503, #54176, #81937, #19690, #40576, #68295, #61456, #16462, #37350, #70537, #85074, #1941, #70992, #8764, #9643, #64171, #30091, #58238, #51399, #49616, #22386, #64609, #78711, #30537, #43704, #1497, #35546, #29638, #15578, #7848, #85529, #84175, #1038, #63264, #36465, #57330, #22840, #65056, #50065, #44141, #71879, #50521, #2839, #57786, #42348, #23303, #78264, #71440, #16022, #9207, #28746, #29202, #36900, #2393, #77799, #85965, #50969, #43249, #70078, #56882, #23736, #14680, #56432, #21947, #77342, #8306, #15119, #42796, #36003, #63717, #84626, #59555, #17794, #17356 ),
 ( #72765, #74103, #39571, #4618, #87292, #38675, #86403, #58664, #65932, #60457, #11883, #80042, #31864, #18240, #24176, #51842, #11428, #80940, #67278, #87731, #4168, #79596, #25055, #52719, #80482, #45036, #45918, #53171, #5062, #73648, #59112, #39130, #32762, #88199, #66832, #45474, #10534, #10973, #38237, #73194, #3720, #31410, #86845, #24613, #52277, #18687, #66377, #32302, #46369, #25958, #3284, #60000, #72325, #25503, #79152, #16912, #44589, #10096, #37800, #65501, #30976, #47720, #12784, #33217, #88645, #19143, #33665, #61354, #40021, #47274, #60918, #487, #69087, #89083, #54968, #26840, #89537, #81392, #26403, #82735, #41797, #46815, #48606, #19582, #53625, #75000, #34096, #14121, #69534, #34552, #54523, #75460, #67736, #20499, #12328, #6851, #61800, #74548, #62257, #68638, #82287, #40476, #20043, #83176, #20934, #13229, #81829, #76343, #68193, #40916, #5524, #27294, #48166, #41353, #6403, #7311, #5975, #75899, #54075, #13667, #43, #27742, #55426, #34996, #62709, #28178, #43150, #78161, #2293, #55868, #36359, #84531, #84072, #49963, #7752, #29098, #15020, #21844, #42694, #56324, #49514, #57687, #35901, #15921, #29997, #44042, #42254, #57228, #21386, #43598, #1845, #63159, #77250, #15481, #71337, #23205, #83619, #22288, #70435, #35443, #941, #49060, #8208, #63613, #14579, #1394, #28638, #64956, #9109, #56782, #29543, #77697, #64069, #76792, #70891, #84973, #16365, #69983, #50872, #8661, #22743, #50418, #36805, #78610, #71777, #64513, #85430, #9548, #37253, #4061, #51297, #18131, #10874, #39472, #45815, #17697, #38137, #86295, #59005, #32202, #59899, #65830, #30881, #87631, #24075, #3614, #79044, #66270, #38572, #80382, #31309, #46260, #44937, #86743, #16809, #72667, #10434, #65402, #51745, #79495, #17257, #2740, #45377, #52621, #66729, #30440, #53061, #73544, #73096, #52178, #9994, #72223, #24514, #73996, #25395, #79941, #31760, #59456, #37703, #3182, #24954, #4514, #80831, #11318, #87190, #58565, #39019, #18580, #11775, #58135, #85867, #23637, #44491, #82177, #47163, #40809, #55316, #62151, #40365, #83072, #89427, #5866, #32653, #81728, #13560, #54863, #27188, #27635, #82628, #33107, #88087, #89884, #20826, #26731, #4957, #47613, #33551, #5412, #88975, #19030, #46717, #33990, #54414, #19932, #48491, #76233, #53516, #60804, #25850, #20389, #61253, #81284, #48059, #88537, #14007, #67175, #60349, #75346, #13125, #68531, #19480, #68079, #53968, #61692, #75794, #74448, #12223, #41245, #74896, #39911, #6299, #26291, #12674, #68976, #6743, #67628, #34442, #86078, #2512, #29768, #24292, #2952, #37914, #64729, #85641, #43821, #78383, #71560, #23850, #65172, #77924, #44712, #16584, #30654, #1626, #63843, #51521, #50188, #36130, #72439, #65613, #8890, #23418, #30214, #9321, #37023, #3394, #57906, #58351, #86524, #79714, #15698, #50642, #79269, #17032, #58780, #71998, #57456, #29326, #51085, #78822, #57006, #10208, #22508, #84748, #43372, #44262, #9767, #37469, #31087, #16146, #51958, #41691, #69426, #7201, #71115, #36591, #64291, #2064, #85200, #22967, #66955, #10642, #31979, #4735, #87853, #4289, #88756, #67387, #12441, #39247, #60119, #18349, #52828, #46036, #88315, #39684, #52390, #19261, #81059, #5180, #66046, #38347, #60574, #24727, #3836, #46933, #40129, #73314, #25617, #32412, #73768, #11555, #67851, #53293, #32873, #61027, #54186, #80157, #25164, #26074, #81509, #33330, #46488, #59673, #31533, #18806, #74227, #59236, #53739, #86966, #17904, #45584, #12002, #74665, #5638, #26515, #80601, #17468, #45151, #72875, #11088, #38794, #66500, #87403, #76005, #21050, #55529, #41467, #75114, #6519, #69197, #62370, #55082, #7859, #14239, #20605, #47380, #34215, #28293, #69647, #41915, #42360, #7415, #47834, #12899, #14690, #35559, #6971, #19698, #152, #48271, #20159, #13781, #33774, #61468, #48722, #34665, #27852, #63275, #70089, #68303, #75572, #40588, #35107, #83280, #6087, #62815, #13342, #76911, #1052, #28760, #76456, #591, #55985, #61919, #82845, #68748, #83729, #21507, #89202, #26968, #49177, #89652, #81950, #54634, #41029, #27402, #82397, #44150, #10106, #57341, #9652, #16035, #43714, #63730, #36018, #43262, #37813, #51411, #85083, #9216, #85536, #1512, #29214, #78721, #58248, #79164 ) ),
 .UNSPECIFIED., .F., .F., .F.,
 ( 4, 3, 1, 1, 1, 3, 4 ),
 ( 4, 1, 1, 1, 1, 1, 1, 1, 1, 1, 1, 1, 1, 1, 1, 1, 1, 1, 1, 1, 1, 1, 1, 1, 1, 1, 1, 1, 1, 1, 1, 1, 1, 1, 1, 1, 1, 1, 1, 1, 1, 1, 1, 1, 1, 1, 1, 1, 1, 1, 1, 1, 1, 1, 1, 1, 1, 1, 1, 1, 1, 1, 1, 1, 1, 1, 1, 1, 1, 1, 1, 1, 1, 1, 1, 1, 1, 1, 1, 1, 1, 1, 1, 1, 1, 1, 1, 1, 1, 1, 1, 1, 1, 1, 1, 1, 1, 1, 1, 1, 1, 1, 1, 1, 1, 1, 1, 1, 1, 1, 1, 1, 1, 1, 1, 1, 1, 1, 1, 1, 1, 1, 1, 1, 1, 1, 1, 1, 1, 1, 1, 1, 1, 1, 1, 1, 1, 1, 1, 1, 1, 1, 1, 1, 1, 1, 1, 1, 1, 1, 1, 1, 1, 1, 1, 1, 1, 1, 1, 1, 1, 1, 1, 1, 1, 1, 1, 1, 1, 1, 1, 1, 1, 1, 1, 1, 1, 1, 1, 1, 1, 1, 1, 1, 1, 1, 1, 1, 1, 1, 1, 1, 1, 1, 1, 1, 1, 1, 1, 1, 1, 1, 1, 1, 1, 1, 1, 1, 1, 1, 1, 1, 1, 1, 1, 1, 1, 1, 1, 1, 1, 1, 1, 1, 1, 1, 1, 1, 1, 1, 1, 1, 1, 1, 1, 1, 1, 1, 1, 1, 1, 1, 1, 1, 1, 1, 1, 1, 1, 1, 1, 1, 1, 1, 1, 1, 1, 1, 1, 1, 1, 1, 1, 1, 1, 1, 1, 1, 1, 1, 1, 1, 1, 1, 1, 1, 1, 1, 1, 1, 1, 1, 1, 1, 1, 1, 1, 1, 1, 1, 1, 1, 1, 1, 1, 1, 1, 1, 1, 1, 1, 1, 1, 1, 1, 1, 1, 1, 1, 1, 1, 1, 1, 1, 1, 1, 1, 1, 1, 1, 1, 1, 1, 1, 1, 1, 1, 1, 1, 1, 1, 1, 1, 1, 1, 1, 1, 1, 1, 1, 1, 1, 1, 1, 1, 1, 1, 1, 1, 1, 1, 1, 1, 1, 1, 1, 1, 1, 1, 1, 1, 1, 1, 1, 1, 1, 1, 1, 1, 1, 1, 1, 1, 1, 1, 1, 1, 1, 1, 1, 1, 1, 1, 1, 1, 1, 1, 1, 1, 1, 1, 1, 1, 1, 1, 1, 1, 1, 1, 1, 1, 1, 1, 1, 1, 1, 1, 1, 1, 1, 1, 1, 1, 1, 1, 1, 1, 1, 1, 1, 1, 1, 1, 1, 1, 1, 1, 1, 1, 1, 1, 1, 1, 1, 1, 1, 1, 1, 1, 1, 1, 1, 1, 1, 1, 1, 1, 1, 1, 1, 1, 1, 1, 1, 1, 1, 1, 1, 1, 1, 1, 1, 1, 1, 1, 1, 1, 1, 1, 1, 1, 1, 1, 1, 1, 1, 1, 1, 1, 1, 1, 1, 1, 1, 1, 1, 1, 1, 1, 1, 1, 1, 1, 1, 1, 1, 1, 1, 1, 1, 1, 1, 1, 1, 1, 1, 1, 1, 1, 1, 1, 1, 1, 1, 1, 1, 1, 1, 1, 1, 1, 1, 1, 1, 1, 4 ),
 ( -1.602212253331664948, -1.570796326795749875, -0.6731984257695950991, -0.2243994752565149908, 0.6731984257696440599, 1.570796326795800057, 1.602526412597075067 ),
 ( 0.000000000000000000, 0.4990644329702639825, 0.9981288659405289643, 1.497193298910790116, 1.996257731881059927, 2.994386597821590001, 3.992515463762110084, 4.491579896732379673, 4.990644329702639936, 5.489708762672909970, 5.988773195643170233, 6.986902061583700529, 7.985030927524229938, 8.484095360494489313, 8.983159793464759346, 9.482224226435020498, 9.981288659405290531, 10.97941752534580040, 11.97754639128630139, 12.47661082425659984, 12.97567525722690007, 13.47473969019709905, 13.97380412316740106, 14.97193298910790027, 15.97006185504850073, 16.46912628801869971, 16.96819072098899994, 17.46725515395930017, 17.96631958692950093, 18.96444845286999836, 19.96257731881059883, 20.46164175178079958, 20.96070618475109981, 21.45977061772140004, 21.95883505069160080, 22.95696391663220126, 23.95509278257270225, 24.45415721554289945, 24.95322164851319968, 25.45228608148349991, 25.95135051445370067, 26.94947938039430113, 27.94760824633480212, 28.44667267930509880, 28.94573711227529955, 29.44480154524559978, 29.94386597821590001, 30.94199484415640100, 31.94012371009690199, 32.43918814306720577, 32.93825257603739942, 33.43731700900769965, 33.93638144197799988, 34.93451030791850087, 35.93263917385900186, 36.43170360682930209, 36.93076803979960232, 37.42983247276980308, 37.92889690574009620, 38.92702577168060429, 39.92515463762109817, 40.42421907059139841, 40.92328350356169864, 41.42234793653189939, 41.92141236950219962, 42.91954123544270061, 43.91767010138330107, 44.41673453435349472, 44.91579896732380206, 45.41486340029400282, 45.91392783326430305, 46.91205669920479693, 47.91018556514539739, 48.40924999811559815, 48.90831443108589838, 49.40737886405619861, 49.90644329702639936, 50.90457216296699983, 51.90270102890750081, 52.40176546187770157, 52.90082989484799469, 53.39989432781830203, 53.89895876078850279, 54.89708762672909614, 55.89521649266960424, 56.39428092563989736, 56.89334535861009812, 57.39240979158039835, 57.89147422455069858, 58.88960309049119957, 59.88773195643170055, 60.38679638940200078, 60.88586082237220154, 61.38492525534249467, 61.88398968831280200, 62.88211855425329588, 63.88024742019380398, 64.37931185316409710, 64.87837628613441154, 65.37744071910459809, 65.87650515207489832, 66.87463401801539931, 67.87276288395590029, 68.37182731692620052, 68.87089174989650076, 69.36995618286670151, 69.86902061583700174, 70.86714948177750273, 71.86527834771810319, 72.36434278068828974, 72.86340721365860418, 73.36247164662880493, 73.86153607959910516, 74.85966494553959194, 75.85779381148019240, 76.35685824445040737, 76.85592267742069339, 77.35498711039100783, 77.85405154336119438, 78.85218040930179484, 79.85030927524229583, 80.34937370821249658, 80.84843814118279681, 81.34750257415311125, 81.84656700712329780, 82.84469587306389826, 83.84282473900439925, 84.34188917197469948, 84.84095360494490023, 85.34001803791520047, 85.83908247088550070, 86.83721133682600168, 87.83534020276650267, 88.33440463573680290, 88.83346906870698945, 89.33253350167728968, 89.83159793464760412, 90.82972680058810511, 91.82785566652860609, 92.32692009949890632, 92.82598453246910708, 93.32504896543939310, 93.82411339840969333, 94.82224226435020853, 95.82037113029070952, 96.31943556326099554, 96.81849999623130998, 97.31756442920149652, 97.81662886217179675, 98.81475772811229774, 99.81288659405289820, 100.3119510270229995, 100.8110154599930013, 101.3100798929639978, 101.8091443259339997, 102.8072731918740033, 103.8054020578150016, 104.3044664907849892, 104.8035309237550052, 105.3025953567259876, 105.8016597896960036, 106.7997886556370020, 107.7979175215769914, 108.2969819545470074, 108.7960463875180039, 109.2951108204880057, 109.7941752534579933, 110.7923041193989917, 111.7904329853389953, 112.2894974183089971, 112.7885618512799937, 113.2876262842500097, 113.7866907172199973, 114.7848195831609956, 115.7829484491009993, 116.2820128820720100, 116.7810773150420118, 117.2801417480119994, 117.7792061809820012, 118.7773350469229996, 119.7754639128630032, 120.2745283458339998, 120.7735927788040016, 121.2726572117740034, 121.7717216447440052, 122.7698505106850035, 123.7679793766259877, 124.2670438095959895, 124.7661082425660055, 125.2651726755359931, 125.7642371085070039, 126.7623659744470075, 127.7604948403880059, 128.2595592733580077, 128.7586237063279953, 129.2576881392979828, 129.7567525722689936, 130.7548814382089972, 131.7530103041499956, 132.2520747371200116, 132.7511391700899992, 133.2502036030609815, 133.7492680360309976, 134.7473969019710012, 135.7455257679119995, 136.2445902008820156, 136.7436546338520031, 137.2427190668229855, 137.7417834997930015, 138.7399123657329767, 139.7380412316740035, 140.2371056646440195, 140.7361700976149734, 141.2352345305849894, 141.7342989635550055, 142.7324278294960038, 143.7305566954360074, 144.2296211284059950, 144.7286855613770058, 145.2277499943469934, 145.7268144273169810, 146.7249432932580078, 147.7230721591979830, 148.2221365921679990, 148.7212010251390097, 149.2202654581089973, 149.7193298910789849, 150.7174587570200117, 151.7155876229599869, 152.2146520559309977, 152.7137164889010137, 153.2127809218710013, 153.7118453548409889, 154.7099742207820157, 155.7081030867219908, 156.2071675196930016, 156.7062319526630176, 157.2052963856329768, 157.7043608186039876, 158.7024896845440196, 159.7006185504849896, 160.1996829834550056, 160.6987474164249932, 161.1978118493950092, 161.6968762823659915, 162.6950051483059951, 163.6931340142469935, 164.1921984472169811, 164.6912628801869971, 165.1903273131570131, 165.6893917461279955, 166.6875206120679991, 167.6856494780089974, 168.1847139109789850, 168.6837783439490011, 169.1828427769200118, 169.6819072098899994, 170.6800360758300030, 171.6781649417710014, 172.1772293747409890, 172.6762938077110050, 173.1753582406820158, 173.6744226736520034, 174.6725515395920070, 175.6706804055330053, 176.6688092714740037, 177.1678737044439913, 177.6669381374140073, 178.6650670033550057, 179.6631958692950093, 180.1622603022650253, 180.6613247352360077, 181.1603891682059952, 181.6594536011760113, 182.6575824671170096, 183.6557113330570132, 184.1547757660279956, 184.6538401989979832, 185.1529046319679992, 185.6519690649380152, 186.6500979308789852, 187.6482267968190172, 188.1472912297899995, 188.6463556627599871, 189.1454200957300031, 189.6444845286999907, 190.6426133946409891, 191.6407422605809927, 192.1398066935519751, 192.6388711265219911, 193.1379355594920071, 193.6369999924630179, 194.6351288584029930, 195.6332577243439914, 196.1323221573140074, 196.6313865902839950, 197.1304510232539826, 197.6295154562249934, 198.6276443221649970, 199.6257731881059954, 200.1248376210760114, 200.6239020540459990, 201.1229664870159866, 201.6220309199869973, 202.6201597859270009, 203.6182886518679993, 204.1173530848380153, 204.6164175178080029, 205.1154819507789853, 205.6145463837490013, 206.6126752496890049, 207.6108041156300033, 208.1098685485999908, 208.6089329815700069, 209.1079974145409892, 209.6070618475110052, 210.6051907134520036, 211.6033195793920072, 212.1023840123619948, 212.6014484453330056, 213.1005128783029932, 213.5995773112729808, 214.5977061772140075, 215.5958350431539827, 216.0948994761239987, 216.5939639090950095, 217.0930283420649971, 217.5920927750350131, 218.5902216409760115, 219.5883505069159867, 220.0874149398869974, 220.5864793728569850, 221.0855438058270011, 221.5846082387970171, 222.5827371047380154, 223.5808659706779906, 224.0799304036490014, 224.5789948366189890, 225.0780592695890050, 225.5771237025589926, 226.5752525685000194, 227.5733814344410177, 228.0724458674109769, 228.5715103003809929, 229.0705747333509805, 229.5696391663219913, 230.5677680322619949, 231.5658968982030217, 232.0649613311730093, 232.5640257641429969, 233.0630901971129845, 233.5621546300839952, 234.5602834960239989, 235.5584123619649972, 236.0574767949350132, 236.5565412279050008, 237.0556056608760116, 237.5546700938459992, 238.5527989597860028, 239.5509278257270012, 240.0499922586970172, 240.5490566916670048, 241.0481211246380155, 241.5471855576080031, 242.5453144235479783, 243.5434432894890051, 244.0425077224589927, 244.5415721554290087, 245.0406365884000195, 245.5397010213700071, 246.5378298873109770, 247.5359587532509806, 248.0350231862209966, 248.5340876191920074, 249.0331520521619950, 249.5322164851320110, 250.5303453510730094, 251.5284742170129846, 252.0275386499830006, 252.5266030829539829, 253.0256675159239990, 253.5247319488940150, 254.5228608148350133, 255.5209896807749885, 256.0200541137460277, 256.5191185467160153, 257.0181829796860029, 257.5172474126559905, 258.5153762785969889, 259.5135051445370209, 260.0125695775079748, 260.5116340104780193, 261.0106984434480069, 261.5097628764180513, 262.5078917423589928, 263.5060206082999912, 264.0050850412700356, 264.5041494742399664, 265.0032139072100108, 265.5022783401809647, 266.5004072061209968, 267.4985360720619951, 267.9976005050319827, 268.4966649380020272, 268.9957293709719579, 269.4947938039430255, 270.4929226698830007, 271.4910515358239991, 271.9901159687939867, 272.4891804017639743, 272.9882448347349850, 273.4873092677049726, 274.4854381336450047, 275.4835669995860030, 275.9826314325560475, 276.4816958655259782, 276.9807602984969890, 277.4798247314670334, 278.4779535974070086, 279.4760824633480070, 279.9751468963179946, 280.4742113292880390, 280.9732757622589929, 281.4723401952289805, 282.4704690611699789, 283.4685979271100109, 283.9676623600799985, 284.4667267930510093, 284.9657912260209969, 285.4648556589909845, 286.4629845249319828, 287.4611133908720149, 287.9601778238429688, 288.4592422568130132, 288.9583066897830008, 289.4573711227530453, 290.4554999886939868, 291.4536288546339620, 291.9526932876050296, 292.4517577205749603, 292.9508221535450048, 293.4498865865149924, 294.4480154524559907, 295.4461443183960228, 295.9452087513669767, 296.4442731843370211, 296.9433376173070087, 297.4424020502780195, 298.4405309162180515, 299.4386597821589930, 299.9377242151289806, 300.4367886480989682, 300.9358530810690127, 301.4349175140399666, 302.4330463799799986, 303.4311752459209970, 303.9302396788909846, 304.4293041118610290, 304.9283685448309598, 305.4274329778020274, 306.4255618437420026, 307.4236907096830009, 307.9227551426529885, 308.4218195756230330, 308.9208840085939869, 309.4199484415639745, 310.4180773075040065, 311.4162061734450049, 311.9152706064150493, 312.4143350393849801, 312.9133994723560477, 313.4124639053259784, 314.4105927712660105, 315.4087216372070088, 315.9077860701769964, 316.4068505031480072, 316.9059149361179948, 317.4049793690880392, 318.4031082350289807, 319.4012371009689559, 319.9003015339390004, 320.3993659669100111, 320.8984303998799987, 321.3974948328499863, 322.3956236987909847, 323.3937525647310167, 323.8928169977019706, 324.3918814306720151, 324.8909458636420027, 325.3900102966119903, 326.3881391625530455, 327.3862680284929638, 327.8853324614640314, 328.3843968944339622, 328.8834613274040066, 329.3825257603739942, 330.3806546263149926, 331.3787834922550246, 331.8778479252259785, 332.3769123581960230, 332.8759767911659537, 333.3750412241370213, 334.3731700900769965, 335.3712989560180517, 335.8703633889879825, 336.3694278219579701, 336.8684922549280145, 337.3675566878989684, 338.3656855538390005, 339.3638144197799988, 339.8628788527500433, 340.3619432857199740, 340.8610077186899616, 341.3600721516610292, 342.3582010176010044, 343.3563298835420028, 343.8553943165119904, 344.3544587494820348, 344.8535231824529887, 345.3525876154230332, 346.3507164813629515, 347.3488453473040067, 347.8479097802739943, 348.3469742132439819, 348.8460386462150495, 349.3451030791849803 ),
 .UNSPECIFIED. ) ;
#5277=FACE_OUTER_BOUND ( 'NONE', #63993, .T. ) ;
#5278=CARTESIAN_POINT ( 'NONE',  ( 108.0837332833436903, -25.31555065790283976, 321.9052427074753382 ) ) ;
#5279=CARTESIAN_POINT ( 'NONE',  ( 109.6058369744873886, -26.58188510553521056, 195.8813395616249977 ) ) ;
#5281=EDGE_LOOP ( 'NONE', ( #69172, #68289, #3335, #46454, #66843 ) ) ;
#5284=ORIENTED_EDGE ( 'NONE', *, *, #3572, .F. ) ;
#5286=ORIENTED_EDGE ( 'NONE', *, *, #48110, .T. ) ;
#5287=LINE ( 'NONE', #32981, #77861 ) ;
#5288=AXIS2_PLACEMENT_3D ( 'NONE', #1935, #65050, #8299 ) ;
#5290=ADVANCED_FACE ( 'NONE', ( #70318 ), #2180, .T. ) ;
#5293=CARTESIAN_POINT ( 'NONE',  ( 109.7217209985873723, -26.99997186863735621, 90.86504839370768138 ) ) ;
#5294=CARTESIAN_POINT ( 'NONE',  ( 104.1077555235347631, -46.72609462085661391, 107.3470538473389411 ) ) ;
#5296=AXIS2_PLACEMENT_3D ( 'NONE', #5890, #744, #63420 ) ;
#5298=CARTESIAN_POINT ( 'NONE',  ( 107.0664832912730020, -36.72944715994189835, 342.9256252759109884 ) ) ;
#5299=CARTESIAN_POINT ( 'NONE',  ( 51.24204729617298426, -31.76306994223730840, -5.074374724088000832 ) ) ;
#5302=CARTESIAN_POINT ( 'NONE',  ( 115.8368392028493190, -44.66223131803943858, 229.2413395616249545 ) ) ;
#5305=ORIENTED_EDGE ( 'NONE', *, *, #67681, .F. ) ;
#5306=FACE_OUTER_BOUND ( 'NONE', #17306, .T. ) ;
#5307=EDGE_CURVE ( 'NONE', #37024, #29858, #42184, .T. ) ;
#5308=CARTESIAN_POINT ( 'NONE',  ( 128.5492039024480562, -43.72944715994093912, 207.5838068554170377 ) ) ;
#5309=CARTESIAN_POINT ( 'NONE',  ( 97.31323396095949363, -38.96131870160394328, 136.5057903769251482 ) ) ;
#5312=CARTESIAN_POINT ( 'NONE',  ( 103.0736367338192139, -47.94042275923426644, 252.3041967044822798 ) ) ;
#5313=ORIENTED_EDGE ( 'NONE', *, *, #53539, .F. ) ;
#5314=LINE ( 'NONE', #75699, #87222 ) ;
#5315=CARTESIAN_POINT ( 'NONE',  ( 113.7700232194324883, -29.06831460768450626, 285.5032443235299979 ) ) ;
#5316=CARTESIAN_POINT ( 'NONE',  ( 95.97749374758174667, -37.21091289986100037, 112.3489586092449599 ) ) ;
#5317=DIRECTION ( 'NONE',  ( 0.7071067811865969777, -0.7071067811864980568, 0.000000000000000000 ) ) ;
#5319=AXIS2_PLACEMENT_3D ( 'NONE', #71737, #9507, #9957 ) ;
#5320=CARTESIAN_POINT ( 'NONE',  ( 177.0371591254543944, -48.62818131005480637, 237.4678068554150059 ) ) ;
#5323=CARTESIAN_POINT ( 'NONE',  ( 73.17003668186727339, -8.979447159941065237, 14.92562527591093691 ) ) ;
#5327=VERTEX_POINT ( 'NONE', #64402 ) ;
#5329=CARTESIAN_POINT ( 'NONE',  ( 100.6111884388667335, -28.52632756463412633, 11.60705384733995515 ) ) ;
#5330=CARTESIAN_POINT ( 'NONE',  ( 134.0664832912740110, 0.2215528400590013880, 293.6356252759119911 ) ) ;
#5331=ADVANCED_FACE ( 'NONE', ( #9000 ), #15811, .F. ) ;
#5332=DIRECTION ( 'NONE',  ( -1.000000000000000000, 0.000000000000000000, 0.000000000000000000 ) ) ;
#5333=LINE ( 'NONE', #80744, #20661 ) ;
#5334=CARTESIAN_POINT ( 'NONE',  ( 41.56648329127398966, -27.57844715994070484, 261.9256252759120116 ) ) ;
#5335=EDGE_CURVE ( 'NONE', #4752, #31084, #1021, .T. ) ;
#5336=CARTESIAN_POINT ( 'NONE',  ( 113.9432952986174854, -30.83689873488770061, 228.8248007804579629 ) ) ;
#5337=ORIENTED_EDGE ( 'NONE', *, *, #39900, .F. ) ;
#5338=ORIENTED_EDGE ( 'NONE', *, *, #9361, .T. ) ;
#5339=ORIENTED_EDGE ( 'NONE', *, *, #25665, .F. ) ;
#5340=AXIS2_PLACEMENT_3D ( 'NONE', #51972, #10657, #87868 ) ;
#5342=VECTOR ( 'NONE', #33504, 1000.000000000000114 ) ;
#5344=DIRECTION ( 'NONE',  ( -0.7071067811865475727, 0.000000000000000000, -0.7071067811865475727 ) ) ;
#5345=PLANE ( 'NONE',  #15680 ) ;
#5346=CARTESIAN_POINT ( 'NONE',  ( 116.4244759746951985, -37.56879123375174601, 30.17491663923099665 ) ) ;
#5348=CARTESIAN_POINT ( 'NONE',  ( 107.0667039024467186, -36.72944715994091069, 195.5838068554169809 ) ) ;
#5349=CARTESIAN_POINT ( 'NONE',  ( 115.9511604156667772, -42.07746527209881293, 278.3832443235305618 ) ) ;
#5350=DIRECTION ( 'NONE',  ( 0.000000000000000000, 1.000000000000000000, 0.000000000000000000 ) ) ;
#5351=EDGE_LOOP ( 'NONE', ( #75429, #65487 ) ) ;
#5353=AXIS2_PLACEMENT_3D ( 'NONE', #20928, #55418, #33209 ) ;
#5355=CARTESIAN_POINT ( 'NONE',  ( 109.9854453146643039, -44.35239847312019634, 60.68523322673397047 ) ) ;
#5358=CARTESIAN_POINT ( 'NONE',  ( 107.0664832912739399, -36.72944715994095333, 311.6343304127839815 ) ) ;
#5361=DIRECTION ( 'NONE',  ( -1.000000000000000000, 0.000000000000000000, 0.000000000000000000 ) ) ;
#5364=CARTESIAN_POINT ( 'NONE',  ( 102.6160711382646156, -46.84739750188308705, 132.2346728949579528 ) ) ;
#5365=ORIENTED_EDGE ( 'NONE', *, *, #34693, .F. ) ;
#5366=CARTESIAN_POINT ( 'NONE',  ( 111.7311378220509255, -29.53965576977622831, 69.04099125664797043 ) ) ;
#5367=FACE_OUTER_BOUND ( 'NONE', #29897, .T. ) ;
#5368=CARTESIAN_POINT ( 'NONE',  ( 102.4863184357179051, -28.52587382674474981, 101.9253928297069791 ) ) ;
#5369=FACE_OUTER_BOUND ( 'NONE', #18449, .T. ) ;
#5370=CARTESIAN_POINT ( 'NONE',  ( 177.8371591254545478, -47.82818131005477369, 117.4678068554150485 ) ) ;
#5371=CARTESIAN_POINT ( 'NONE',  ( 96.17045672112728028, -38.71987694442820782, 47.48229194257797303 ) ) ;
#5372=AXIS2_PLACEMENT_3D ( 'NONE', #9450, #16273, #43500 ) ;
#5373=LINE ( 'NONE', #19001, #23693 ) ;
#5374=CARTESIAN_POINT ( 'NONE',  ( 163.0664832912739826, -0.7548456658610993575, 333.4006252759120343 ) ) ;
#5375=VERTEX_POINT ( 'NONE', #86636 ) ;
#5379=EDGE_CURVE ( 'NONE', #12604, #2603, #52514, .T. ) ;
#5380=ADVANCED_FACE ( 'NONE', ( #11209 ), #38031, .F. ) ;
#5383=ORIENTED_EDGE ( 'NONE', *, *, #7749, .T. ) ;
#5384=CARTESIAN_POINT ( 'NONE',  ( 116.8464009251322153, -35.91275531464980020, 253.8927681330545454 ) ) ;
#5385=CARTESIAN_POINT ( 'NONE',  ( 117.6028659061361736, -33.31333136338176359, 130.0880062282919880 ) ) ;
#5386=CARTESIAN_POINT ( 'NONE',  ( 102.8734617018388633, -27.62276334107901121, 125.4186639751545869 ) ) ;
#5387=CARTESIAN_POINT ( 'NONE',  ( 116.8181881254705274, -34.15704652260703966, 130.0311224560221035 ) ) ;
#5388=CARTESIAN_POINT ( 'NONE',  ( 109.7700798034136511, -47.44693503648352362, 88.78514908543493789 ) ) ;
#5389=CARTESIAN_POINT ( 'NONE',  ( 107.0664832912750057, -36.72944715993903486, 4.925625275910970657 ) ) ;
#5394=VECTOR ( 'NONE', #75774, 999.9999999999998863 ) ;
#5399=CYLINDRICAL_SURFACE ( 'NONE', #47471, 2.517499999999998739 ) ;
#5402=CARTESIAN_POINT ( 'NONE',  ( 97.57986484199619781, -43.79006170206860560, 261.8356252759109566 ) ) ;
#5405=DIRECTION ( 'NONE',  ( -0.000000000000000000, -0.000000000000000000, 1.000000000000000000 ) ) ;
#5406=LINE ( 'NONE', #32197, #63549 ) ;
#5408=CARTESIAN_POINT ( 'NONE',  ( 98.80150335516665905, -38.88496061976939444, 275.9524198280767564 ) ) ;
#5409=CARTESIAN_POINT ( 'NONE',  ( 116.3121618740066623, -32.93870344941997530, 39.13562527591096796 ) ) ;
#5410=CARTESIAN_POINT ( 'NONE',  ( 107.6020193903983966, -26.30459096080998904, 91.03562527591097364 ) ) ;
#5411=CARTESIAN_POINT ( 'NONE',  ( 20.56670390244748603, -48.82844715994200158, 129.9678068554150627 ) ) ;
#5412=CARTESIAN_POINT ( 'NONE',  ( 114.2838679902333610, -44.31336211532283897, 158.1813395616249807 ) ) ;
#5417=DIRECTION ( 'NONE',  ( 0.000000000000000000, 0.000000000000000000, -1.000000000000000000 ) ) ;
#5418=CARTESIAN_POINT ( 'NONE',  ( 135.1249450788490378, -34.19118199975285677, 1.799893109327216578 ) ) ;
#5419=ORIENTED_EDGE ( 'NONE', *, *, #61560, .T. ) ;
#5420=EDGE_CURVE ( 'NONE', #8128, #25485, #13252, .T. ) ;
#5421=AXIS2_PLACEMENT_3D ( 'NONE', #13118, #37584, #16252 ) ;
#5422=CARTESIAN_POINT ( 'NONE',  ( 97.06098165937136457, -37.99585007323931762, 62.42765791910697715 ) ) ;
#5423=CARTESIAN_POINT ( 'NONE',  ( 102.6790914627476070, -46.92570513279398625, 137.2651490854349561 ) ) ;
#5424=ORIENTED_EDGE ( 'NONE', *, *, #4996, .T. ) ;
#5428=AXIS2_PLACEMENT_3D ( 'NONE', #54403, #53957, #68965 ) ;
#5429=CARTESIAN_POINT ( 'NONE',  ( 108.3334480883274722, -46.73485935487656917, 118.6772919420508430 ) ) ;
#5430=CARTESIAN_POINT ( 'NONE',  ( 99.04406186696009229, -42.84125765073620329, 76.84395861032450625 ) ) ;
#5431=ORIENTED_EDGE ( 'NONE', *, *, #86780, .F. ) ;
#5433=SHAPE_DEFINITION_REPRESENTATION ( #46585, #64293 ) ;
#5434=DIRECTION ( 'NONE',  ( 0.000000000000000000, 0.000000000000000000, -1.000000000000000000 ) ) ;
#5436=ORIENTED_EDGE ( 'NONE', *, *, #4444, .T. ) ;
#5437=ORIENTED_EDGE ( 'NONE', *, *, #25200, .T. ) ;
#5438=CARTESIAN_POINT ( 'NONE',  ( 172.5664832912729878, -27.82844715994070484, 18.92562527591200094 ) ) ;
#5440=DIRECTION ( 'NONE',  ( 0.000000000000000000, 1.000000000000000000, 0.000000000000000000 ) ) ;
#5441=CARTESIAN_POINT ( 'NONE',  ( 172.5664832912729878, -27.82844715994070484, 258.9256252759120116 ) ) ;
#5442=DIRECTION ( 'NONE',  ( 3.999999999999999995E-14, -1.000000000000000000, 4.100000000000000342E-29 ) ) ;
#5444=EDGE_CURVE ( 'NONE', #38655, #86561, #29205, .T. ) ;
#5447=VERTEX_POINT ( 'NONE', #66619 ) ;
#5448=LINE ( 'NONE', #12255, #10007 ) ;
#5449=CARTESIAN_POINT ( 'NONE',  ( 112.7790632652331482, -27.19118669266625687, 200.6470538473389809 ) ) ;
#5451=ORIENTED_EDGE ( 'NONE', *, *, #41175, .T. ) ;
#5452=CARTESIAN_POINT ( 'NONE',  ( 106.0550521757682816, -27.00111521709629514, 46.15848241876796720 ) ) ;
#5456=VERTEX_POINT ( 'NONE', #58460 ) ;
#5457=EDGE_CURVE ( 'NONE', #5214, #37298, #4410, .T. ) ;
#5458=DIRECTION ( 'NONE',  ( -1.175184669632759901E-16, 1.000000000000000000, 2.000000000000003705E-15 ) ) ;
#5460=ORIENTED_EDGE ( 'NONE', *, *, #62886, .F. ) ;
#5462=CARTESIAN_POINT ( 'NONE',  ( 114.2499829074921820, -30.67355260991839216, 220.8034880678019647 ) ) ;
#5463=EDGE_CURVE ( 'NONE', #5997, #54334, #32096, .T. ) ;
#5465=CARTESIAN_POINT ( 'NONE',  ( 98.54763758010979302, -41.97696078833845235, 52.76539822096258803 ) ) ;
#5466=VECTOR ( 'NONE', #63769, 1000.000000000000000 ) ;
#5469=DIRECTION ( 'NONE',  ( 0.000000000000000000, 0.000000000000000000, -1.000000000000000000 ) ) ;
#5470=ORIENTED_EDGE ( 'NONE', *, *, #67338, .T. ) ;
#5472=AXIS2_PLACEMENT_3D ( 'NONE', #33497, #40305, #55262 ) ;
#5475=CARTESIAN_POINT ( 'NONE',  ( 100.4652087429556815, -44.82591848225601439, 12.03276813305398463 ) ) ;
#5476=EDGE_LOOP ( 'NONE', ( #76093, #83527 ) ) ;
#5477=ORIENTED_EDGE ( 'NONE', *, *, #60787, .T. ) ;
#5478=CARTESIAN_POINT ( 'NONE',  ( 115.7079196686036653, -36.25352450022288764, 271.7004713219723726 ) ) ;
#5479=AXIS2_PLACEMENT_3D ( 'NONE', #36802, #16362, #57225 ) ;
#5480=FACE_BOUND ( 'NONE', #70811, .T. ) ;
#5481=CARTESIAN_POINT ( 'NONE',  ( 104.0088209277215583, -27.43890701233894092, 165.3299109901969643 ) ) ;
#5483=DIRECTION ( 'NONE',  ( 1.000000000000000000, 4.163336342344333240E-14, 0.000000000000000000 ) ) ;
#5484=VECTOR ( 'NONE', #51037, 1000.000000000000000 ) ;
#5485=CYLINDRICAL_SURFACE ( 'NONE', #37631, 0.5000000000000104361 ) ;
#5486=AXIS2_PLACEMENT_3D ( 'NONE', #42470, #70203, #30980 ) ;
#5488=CARTESIAN_POINT ( 'NONE',  ( 101.2698767154569168, -26.33663883357058921, 251.4813395616249920 ) ) ;
#5489=CARTESIAN_POINT ( 'NONE',  ( 51.06648329127400388, 25.62155284005901379, 339.0006252759110339 ) ) ;
#5491=EDGE_LOOP ( 'NONE', ( #48251, #44791, #53737, #18869 ) ) ;
#5492=CARTESIAN_POINT ( 'NONE',  ( 117.4907998085504062, -37.69205034685562339, 74.75276813305397638 ) ) ;
#5494=ORIENTED_EDGE ( 'NONE', *, *, #78133, .T. ) ;
#5495=ORIENTED_EDGE ( 'NONE', *, *, #33810, .T. ) ;
#5497=EDGE_CURVE ( 'NONE', #28392, #34697, #51642, .T. ) ;
#5498=ORIENTED_EDGE ( 'NONE', *, *, #89800, .T. ) ;
#5501=CYLINDRICAL_SURFACE ( 'NONE', #79080, 4.750000000000004441 ) ;
#5502=CARTESIAN_POINT ( 'NONE',  ( 25.56670390244808289, -42.82844715994167473, 257.2178068554150059 ) ) ;
#5503=CARTESIAN_POINT ( 'NONE',  ( 99.80647774793122551, -41.44074323372286273, 144.6147570362579415 ) ) ;
#5504=CARTESIAN_POINT ( 'NONE',  ( 115.2688234373398046, -30.20251741173218818, 240.3613395616249875 ) ) ;
#5505=LINE ( 'NONE', #54057, #81 ) ;
#5506=ORIENTED_EDGE ( 'NONE', *, *, #84263, .F. ) ;
#5508=EDGE_CURVE ( 'NONE', #783, #78421, #13313, .T. ) ;
#5510=CARTESIAN_POINT ( 'NONE',  ( 136.6493805748345665, -37.67376371870763307, 2.871651383882680708 ) ) ;
#5512=VECTOR ( 'NONE', #27725, 1000.000000000000000 ) ;
#5515=FACE_OUTER_BOUND ( 'NONE', #85195, .T. ) ;
#5516=EDGE_LOOP ( 'NONE', ( #41606, #76428, #2590 ) ) ;
#5517=ORIENTED_EDGE ( 'NONE', *, *, #7445, .T. ) ;
#5518=CARTESIAN_POINT ( 'NONE',  ( 107.0664832912739541, -36.72944715994095333, 307.1356252759109680 ) ) ;
#5520=LINE ( 'NONE', #78815, #30719 ) ;
#5523=CARTESIAN_POINT ( 'NONE',  ( 109.0154912191213583, -27.88557705556195998, 179.3143245899819647 ) ) ;
#5524=CARTESIAN_POINT ( 'NONE',  ( 116.2704737988580206, -31.74013610724590961, 69.22133956162495849 ) ) ;
#5525=ORIENTED_EDGE ( 'NONE', *, *, #2836, .F. ) ;
#5526=CARTESIAN_POINT ( 'NONE',  ( 164.9190312289439930, -35.91149509761220315, -5.074374724088000832 ) ) ;
#5529=VERTEX_POINT ( 'NONE', #68867 ) ;
#5530=LINE ( 'NONE', #80047, #43196 ) ;
#5531=ORIENTED_EDGE ( 'NONE', *, *, #51235, .F. ) ;
#5532=CARTESIAN_POINT ( 'NONE',  ( 99.64972233663489476, -29.98183745677715351, 166.7387298538411073 ) ) ;
#5533=AXIS2_PLACEMENT_3D ( 'NONE', #85862, #29992, #8204 ) ;
#5535=CARTESIAN_POINT ( 'NONE',  ( 116.7444820060442083, -34.14078160163364828, 134.0345115328372856 ) ) ;
#5536=CIRCLE ( 'NONE', #37430, 4.875000000000017764 ) ;
#5538=VERTEX_POINT ( 'NONE', #55205 ) ;
#5539=AXIS2_PLACEMENT_3D ( 'NONE', #16821, #3196, #79506 ) ;
#5540=CARTESIAN_POINT ( 'NONE',  ( 100.5368863760760973, -27.78183265877541430, 30.56610146638794134 ) ) ;
#5541=CARTESIAN_POINT ( 'NONE',  ( 104.7499416563296961, -46.93859083614567140, 68.39848241876794077 ) ) ;
#5544=DIRECTION ( 'NONE',  ( 0.7071067811865473507, 0.7071067811865476838, 0.000000000000000000 ) ) ;
#5545=CARTESIAN_POINT ( 'NONE',  ( 116.3212776292293569, -32.94146857471253753, 110.1356252759109822 ) ) ;
#5546=FACE_BOUND ( 'NONE', #55591, .T. ) ;
#5547=VECTOR ( 'NONE', #47790, 1000.000000000000000 ) ;
#5549=CIRCLE ( 'NONE', #37518, 10.00000000000000711 ) ;
#5550=CARTESIAN_POINT ( 'NONE',  ( 95.35945913470564506, -35.72541260001472097, 298.1356252759109680 ) ) ;
#5551=ORIENTED_EDGE ( 'NONE', *, *, #29206, .T. ) ;
#5552=CARTESIAN_POINT ( 'NONE',  ( 114.1203865811702087, -46.31439608500644312, 33.08133956162495792 ) ) ;
#5553=CARTESIAN_POINT ( 'NONE',  ( 118.0249073071387471, -38.34132458482030614, 69.72229194257801055 ) ) ;
#5556=CARTESIAN_POINT ( 'NONE',  ( 99.50511838765265793, -43.30624115933716922, 171.8947509423747135 ) ) ;
#5557=CARTESIAN_POINT ( 'NONE',  ( 141.0664832912740110, -8.729447159940995959, -4.824374724088991151 ) ) ;
#5562=CARTESIAN_POINT ( 'NONE',  ( 103.5129713284350146, -46.47169217660395191, 93.28610146638693834 ) ) ;
#5564=ORIENTED_EDGE ( 'NONE', *, *, #80802, .F. ) ;
#5565=CARTESIAN_POINT ( 'NONE',  ( 96.70388795518327640, -35.81005419191409089, 227.2556252759109725 ) ) ;
#5566=CARTESIAN_POINT ( 'NONE',  ( 105.7144241109852345, -46.72372135719457020, 253.4708212861533241 ) ) ;
#5567=CARTESIAN_POINT ( 'NONE',  ( 115.0663604721750488, -42.78498363884347810, 148.3107124467303777 ) ) ;
#5569=CARTESIAN_POINT ( 'NONE',  ( 97.81169817874256012, -40.51742791483425776, 82.63555527327814332 ) ) ;
#5570=LINE ( 'NONE', #33263, #12897 ) ;
#5572=CARTESIAN_POINT ( 'NONE',  ( 109.6835627966675162, -27.30531164764922991, 174.8613395616259822 ) ) ;
#5575=VERTEX_POINT ( 'NONE', #32992 ) ;
#5576=VECTOR ( 'NONE', #2103, 1000.000000000000000 ) ;
#5577=CARTESIAN_POINT ( 'NONE',  ( 112.3917779585437131, -43.81249117439911345, 139.5215833058969679 ) ) ;
#5578=ADVANCED_FACE ( 'NONE', ( #4851 ), #48389, .F. ) ;
#5579=CARTESIAN_POINT ( 'NONE',  ( 188.5667039024479834, -58.35344715994099829, 259.9678068554150059 ) ) ;
#5580=CARTESIAN_POINT ( 'NONE',  ( 106.8506556707825013, -46.50783423188139665, 268.5584824187674258 ) ) ;
#5581=CARTESIAN_POINT ( 'NONE',  ( 71.24076473329807868, 5.642044068322332961, 361.9756252759101471 ) ) ;
#5582=CARTESIAN_POINT ( 'NONE',  ( 41.56648329127398966, -27.57844715994070484, 201.9256252759119832 ) ) ;
#5584=LINE ( 'NONE', #61862, #61796 ) ;
#5587=CARTESIAN_POINT ( 'NONE',  ( 108.1794352217186344, -47.07304438381573419, 202.6613395616249704 ) ) ;
#5588=DIRECTION ( 'NONE',  ( 0.7071067811874244269, -0.7071067811856707186, 7.071067811874251411E-16 ) ) ;
#5589=ORIENTED_EDGE ( 'NONE', *, *, #22322, .T. ) ;
#5590=ORIENTED_EDGE ( 'NONE', *, *, #16353, .T. ) ;
#5591=AXIS2_PLACEMENT_3D ( 'NONE', #65291, #17146, #23963 ) ;
#5594=LINE ( 'NONE', #40546, #75139 ) ;
#5595=DIRECTION ( 'NONE',  ( 0.000000000000000000, 0.000000000000000000, -1.000000000000000000 ) ) ;
#5597=CARTESIAN_POINT ( 'NONE',  ( 34.96670390244699433, -26.71338133339301635, -5.074374724088000832 ) ) ;
#5599=CARTESIAN_POINT ( 'NONE',  ( 107.0664832912739968, -36.72944715994100306, 287.6356252759109680 ) ) ;
#5600=CARTESIAN_POINT ( 'NONE',  ( 101.4252639664679094, -46.23501037223531540, 207.1622919425779514 ) ) ;
#5601=DIRECTION ( 'NONE',  ( 9.351236661543306751E-17, -3.725950533538267725E-29, -1.000000000000000000 ) ) ;
#5602=ADVANCED_FACE ( 'NONE', ( #13016 ), #74342, .T. ) ;
#5603=VERTEX_POINT ( 'NONE', #60690 ) ;
#5606=DIRECTION ( 'NONE',  ( -1.000000000000000000, -4.299999999999999979E-14, -1.000000000000000078E-15 ) ) ;
#5607=LINE ( 'NONE', #47353, #10128 ) ;
#5609=CARTESIAN_POINT ( 'NONE',  ( 100.8872380539724247, -44.70003101589365713, 163.0522683080627075 ) ) ;
#5610=CARTESIAN_POINT ( 'NONE',  ( 111.0712550167563677, -29.58490437025668740, 32.48809036959193719 ) ) ;
#5611=AXIS2_PLACEMENT_3D ( 'NONE', #4511, #32199, #59896 ) ;
#5612=CARTESIAN_POINT ( 'NONE',  ( 99.66919142226757344, -46.01935155626545537, 118.0413395616259606 ) ) ;
#5615=EDGE_CURVE ( 'NONE', #23299, #61548, #26189, .T. ) ;
#5618=CARTESIAN_POINT ( 'NONE',  ( 82.31780288913714116, -17.14744377620639781, 7.339349742409305044 ) ) ;
#5620=ORIENTED_EDGE ( 'NONE', *, *, #89388, .T. ) ;
#5621=DIRECTION ( 'NONE',  ( -0.7071067811865274777, 0.7071067811865675568, -7.071067811864971448E-16 ) ) ;
#5622=ORIENTED_EDGE ( 'NONE', *, *, #18355, .F. ) ;
#5624=DIRECTION ( 'NONE',  ( -4.237773401492740281E-14, 1.000000000000000000, 0.000000000000000000 ) ) ;
#5625=EDGE_CURVE ( 'NONE', #59703, #76619, #81626, .T. ) ;
#5626=CIRCLE ( 'NONE', #73755, 16.00000000000000000 ) ;
#5627=CARTESIAN_POINT ( 'NONE',  ( 109.3970511370136904, -44.97690468586920787, 72.21813411379096692 ) ) ;
#5628=CARTESIAN_POINT ( 'NONE',  ( 110.8247753047693749, -26.30972152642112150, 249.7889586092445882 ) ) ;
#5629=CARTESIAN_POINT ( 'NONE',  ( 96.76471471792625323, -35.27954033865438532, 181.2156252759109805 ) ) ;
#5630=PLANE ( 'NONE',  #78054 ) ;
#5631=CARTESIAN_POINT ( 'NONE',  ( 111.0379167980822928, -47.01981040405694756, 13.85753003781498016 ) ) ;
#5632=CARTESIAN_POINT ( 'NONE',  ( 106.0039306387646860, -11.55185827894094786, 322.0356252759110021 ) ) ;
#5633=FACE_OUTER_BOUND ( 'NONE', #85283, .T. ) ;
#5634=ORIENTED_EDGE ( 'NONE', *, *, #80248, .T. ) ;
#5635=B_SPLINE_CURVE_WITH_KNOTS ( 'NONE', 3,
 ( #56799, #54983, #35915, #82753, #20516, #15037, #15496, #70453, #8225, #69103, #63629, #1415, #68655, #84546, #44060, #85884, #72241, #78181, #15939, #65421, #44955, #9124, #1861, #3203, #72690, #8680, #2760, #64531, #36824 ),
 .UNSPECIFIED., .F., .F.,
 ( 4, 2, 2, 2, 2, 2, 2, 2, 2, 2, 1, 1, 1, 1, 1, 2, 4 ),
 ( 0.000000000000000000, 0.06250185081845154034, 0.1250037016369030807, 0.1875055524553546071, 0.2500074032738061613, 0.3125092540922577156, 0.3750111049107092143, 0.4375129557291607685, 0.4687638811383865733, 0.4843893438429994203, 0.4922020751953060658, 0.4961084408714594440, 0.4980616237095359944, 0.4990382151285742696, 0.4995265108380935182, 0.4997706586928529204, 0.5000148065476123227 ),
 .UNSPECIFIED. ) ;
#5636=AXIS2_PLACEMENT_3D ( 'NONE', #37638, #3113, #10803 ) ;
#5637=LINE ( 'NONE', #31978, #54533 ) ;
#5638=CARTESIAN_POINT ( 'NONE',  ( 97.12779447186500192, -40.02021159927672755, 241.5813395616249863 ) ) ;
#5640=CARTESIAN_POINT ( 'NONE',  ( 98.43480628652092435, -29.82486610537253569, 195.7775300378159784 ) ) ;
#5641=PLANE ( 'NONE',  #28235 ) ;
#5642=DIRECTION ( 'NONE',  ( 1.000000000000000000, 0.000000000000000000, 0.000000000000000000 ) ) ;
#5643=CARTESIAN_POINT ( 'NONE',  ( 180.3521107875639871, -35.65087443492551245, -5.074374724088000832 ) ) ;
#5644=PLANE ( 'NONE',  #39818 ) ;
#5645=CARTESIAN_POINT ( 'NONE',  ( 114.2883772398465538, -33.13574786571706454, 277.6356252759109680 ) ) ;
#5646=CARTESIAN_POINT ( 'NONE',  ( 25.56670390244797275, -67.87844715994100397, 293.2178068554150627 ) ) ;
#5654=ORIENTED_EDGE ( 'NONE', *, *, #24887, .F. ) ;
#5655=VECTOR ( 'NONE', #66396, 1000.000000000000000 ) ;
#5656=CYLINDRICAL_SURFACE ( 'NONE', #56794, 6.571100913904396990 ) ;
#5657=CARTESIAN_POINT ( 'NONE',  ( 97.03688691280343903, -41.43079139552996537, 211.6632443235299945 ) ) ;
#5658=CARTESIAN_POINT ( 'NONE',  ( 114.5674230198705317, -44.02034806205370643, 94.21276813305395592 ) ) ;
#5659=CARTESIAN_POINT ( 'NONE',  ( 111.0094172226674374, -46.42718045843506047, 278.8841967044824059 ) ) ;
#5660=DIRECTION ( 'NONE',  ( 0.000000000000000000, 0.000000000000000000, -1.000000000000000000 ) ) ;
#5663=CARTESIAN_POINT ( 'NONE',  ( 50.96943157743499597, -34.03355364505720360, -5.074374724088000832 ) ) ;
#5665=CARTESIAN_POINT ( 'NONE',  ( 31.89136050872298966, -31.76306994223740432, -5.074374724088000832 ) ) ;
#5666=CARTESIAN_POINT ( 'NONE',  ( 132.6459363690182158, -21.09121833381622935, 1.942446336659213513 ) ) ;
#5667=AXIS2_PLACEMENT_3D ( 'NONE', #7135, #22567, #50241 ) ;
#5669=EDGE_CURVE ( 'NONE', #78421, #12031, #11821, .T. ) ;
#5670=ORIENTED_EDGE ( 'NONE', *, *, #9489, .F. ) ;
#5672=CARTESIAN_POINT ( 'NONE',  ( 116.7762654731291860, -36.89220852042034693, 153.2352769709339668 ) ) ;
#5673=AXIS2_PLACEMENT_3D ( 'NONE', #27722, #7289, #22 ) ;
#5675=ORIENTED_EDGE ( 'NONE', *, *, #4665, .F. ) ;
#5677=CARTESIAN_POINT ( 'NONE',  ( 113.8292797163801851, -28.77778007523028947, 135.5156252759109634 ) ) ;
#5679=VECTOR ( 'NONE', #66892, 1000.000000000000000 ) ;
#5680=DIRECTION ( 'NONE',  ( -6.524622321627019585E-16, -4.013151879589939944E-16, -1.000000000000000000 ) ) ;
#5681=LINE ( 'NONE', #66543, #62102 ) ;
#5683=VECTOR ( 'NONE', #87533, 1000.000000000000114 ) ;
#5684=CARTESIAN_POINT ( 'NONE',  ( 104.1495640007033217, -46.68084741754461220, 62.33753003781600199 ) ) ;
#5685=EDGE_LOOP ( 'NONE', ( #59721, #87560, #42855, #18953 ) ) ;
#5687=ORIENTED_EDGE ( 'NONE', *, *, #20576, .T. ) ;
#5688=ADVANCED_FACE ( 'NONE', ( #82520 ), #60242, .T. ) ;
#5689=DIRECTION ( 'NONE',  ( -1.000000000000000000, -3.999999999999999995E-14, -1.000000000000000078E-15 ) ) ;
#5690=CARTESIAN_POINT ( 'NONE',  ( 96.69720940280909360, -36.59277893904148726, 152.3280062282909739 ) ) ;
#5694=DIRECTION ( 'NONE',  ( 0.000000000000000000, 0.000000000000000000, -1.000000000000000000 ) ) ;
#5696=CARTESIAN_POINT ( 'NONE',  ( 101.9935007850360620, -45.44599742214800386, 178.1564475108619945 ) ) ;
#5697=CARTESIAN_POINT ( 'NONE',  ( 96.11054930851071276, -38.00668368623060189, 86.43086337114897333 ) ) ;
#5698=ORIENTED_EDGE ( 'NONE', *, *, #39851, .T. ) ;
#5699=ORIENTED_EDGE ( 'NONE', *, *, #26616, .T. ) ;
#5700=ORIENTED_EDGE ( 'NONE', *, *, #78720, .T. ) ;
#5701=EDGE_CURVE ( 'NONE', #44803, #41711, #82073, .T. ) ;
#5705=CARTESIAN_POINT ( 'NONE',  ( 100.3885320853208896, -32.03533449533603772, 203.6566617981629577 ) ) ;
#5708=ORIENTED_EDGE ( 'NONE', *, *, #64246, .F. ) ;
#5709=ORIENTED_EDGE ( 'NONE', *, *, #23596, .F. ) ;
#5711=CARTESIAN_POINT ( 'NONE',  ( 70.14948329127297200, -71.52944715994141234, 342.9256252759110453 ) ) ;
#5712=CARTESIAN_POINT ( 'NONE',  ( 135.1908702341724506, -21.23918067504807894, 1.822998012174642968 ) ) ;
#5713=ORIENTED_EDGE ( 'NONE', *, *, #8156, .F. ) ;
#5714=VERTEX_POINT ( 'NONE', #27526 ) ;
#5716=EDGE_CURVE ( 'NONE', #19751, #49481, #75635, .T. ) ;
#5717=CARTESIAN_POINT ( 'NONE',  ( 116.3029726692365813, -35.00788115540211010, 200.4168214011349676 ) ) ;
#5718=AXIS2_PLACEMENT_3D ( 'NONE', #62512, #13036, #27546 ) ;
#5722=ORIENTED_EDGE ( 'NONE', *, *, #71101, .F. ) ;
#5723=AXIS2_PLACEMENT_3D ( 'NONE', #20898, #38872, #77213 ) ;
#5724=ORIENTED_EDGE ( 'NONE', *, *, #558, .F. ) ;
#5725=DIRECTION ( 'NONE',  ( -0.9963424814100680926, 0.08544974978095698503, 0.000000000000000000 ) ) ;
#5726=ORIENTED_EDGE ( 'NONE', *, *, #88491, .F. ) ;
#5727=EDGE_LOOP ( 'NONE', ( #35153, #3045, #53805 ) ) ;
#5728=ADVANCED_FACE ( 'NONE', ( #63396 ), #83398, .T. ) ;
#5729=CARTESIAN_POINT ( 'NONE',  ( 113.4754094548699186, -31.62960856676687982, 242.1795189410199782 ) ) ;
#5730=VECTOR ( 'NONE', #10618, 1000.000000000000000 ) ;
#5731=CARTESIAN_POINT ( 'NONE',  ( 111.0910783018720025, -25.55641485417826431, 99.80133956162498521 ) ) ;
#5732=CARTESIAN_POINT ( 'NONE',  ( 98.66494773507966443, -43.87633619481174918, 76.89943479971999807 ) ) ;
#5733=CARTESIAN_POINT ( 'NONE',  ( 115.7727261665505836, -40.42085123866506535, 249.5838068554168103 ) ) ;
#5734=EDGE_CURVE ( 'NONE', #89264, #76080, #272, .T. ) ;
#5735=CARTESIAN_POINT ( 'NONE',  ( 133.1862368104802670, -16.12360705087672130, 8.106403045237987826 ) ) ;
#5736=CARTESIAN_POINT ( 'NONE',  ( 105.8320912101120399, -25.33698730529098953, 321.9074507037550461 ) ) ;
#5737=CARTESIAN_POINT ( 'NONE',  ( 103.6386224297199163, -26.22117658871400181, 206.3394347997209763 ) ) ;
#5739=ORIENTED_EDGE ( 'NONE', *, *, #86797, .T. ) ;
#5741=ORIENTED_EDGE ( 'NONE', *, *, #46269, .F. ) ;
#5742=VERTEX_POINT ( 'NONE', #36600 ) ;
#5743=AXIS2_PLACEMENT_3D ( 'NONE', #21977, #36492, #62833 ) ;
#5744=CARTESIAN_POINT ( 'NONE',  ( 45.76696975232771081, -48.62818131006091704, 180.4678068554150911 ) ) ;
#5745=ORIENTED_EDGE ( 'NONE', *, *, #42698, .F. ) ;
#5746=CARTESIAN_POINT ( 'NONE',  ( 97.75827573275111604, -40.38460791318124166, 137.6242309511203246 ) ) ;
#5747=CARTESIAN_POINT ( 'NONE',  ( 98.34920873643025629, -31.65775108644640312, 91.90656420394297754 ) ) ;
#5748=CARTESIAN_POINT ( 'NONE',  ( 111.0826007845189736, -25.57995003598136208, 99.80133956162498521 ) ) ;
#5750=DIRECTION ( 'NONE',  ( 0.000000000000000000, -1.000000000000000000, 0.000000000000000000 ) ) ;
#5751=CARTESIAN_POINT ( 'NONE',  ( 149.4409906032288973, -0.9156555935619370423, 394.9756252759100903 ) ) ;
#5752=CARTESIAN_POINT ( 'NONE',  ( 19.56670390244734747, -25.42844715994192129, 300.4678068554150059 ) ) ;
#5754=CARTESIAN_POINT ( 'NONE',  ( 99.10268845779070546, -29.98093639561600909, 211.7670538473399517 ) ) ;
#5757=VERTEX_POINT ( 'NONE', #49303 ) ;
#5758=AXIS2_PLACEMENT_3D ( 'NONE', #71666, #49849, #36240 ) ;
#5759=DIRECTION ( 'NONE',  ( 1.000000000000000000, 4.163336342344333240E-14, 0.000000000000000000 ) ) ;
#5761=CARTESIAN_POINT ( 'NONE',  ( 131.0667039024480118, -64.87844715994098976, 207.5838068554149913 ) ) ;
#5762=DIRECTION ( 'NONE',  ( -0.7071067811865506814, 0.7071067811865443531, -7.071067811865500971E-16 ) ) ;
#5763=CARTESIAN_POINT ( 'NONE',  ( 116.9671346634708442, -41.74840980516093936, 248.4651490854349731 ) ) ;
#5764=VERTEX_POINT ( 'NONE', #13903 ) ;
#5765=CARTESIAN_POINT ( 'NONE',  ( 111.1917831817336975, -27.58851263026131306, 194.7389780491331521 ) ) ;
#5766=CARTESIAN_POINT ( 'NONE',  ( 96.89316087236547048, -34.20304521249558150, 272.1327681330539576 ) ) ;
#5767=CARTESIAN_POINT ( 'NONE',  ( 95.96792091384095613, -36.58316683298836125, 152.3280062282919971 ) ) ;
#5768=CARTESIAN_POINT ( 'NONE',  ( 97.81169952324414396, -40.51743120087827776, 141.6355106266202313 ) ) ;
#5769=CARTESIAN_POINT ( 'NONE',  ( 97.39129596614627360, -39.27853438940273634, 102.5314386769556876 ) ) ;
#5770=VECTOR ( 'NONE', #32365, 1000.000000000000000 ) ;
#5771=LINE ( 'NONE', #33011, #4283 ) ;
#5774=CARTESIAN_POINT ( 'NONE',  ( 71.06648329127399677, -8.729447159940999512, 342.9256252759119548 ) ) ;
#5775=ORIENTED_EDGE ( 'NONE', *, *, #46372, .F. ) ;
#5778=ORIENTED_EDGE ( 'NONE', *, *, #35823, .F. ) ;
#5779=AXIS2_PLACEMENT_3D ( 'NONE', #31921, #16971, #10590 ) ;
#5780=ORIENTED_EDGE ( 'NONE', *, *, #24270, .T. ) ;
#5781=FACE_OUTER_BOUND ( 'NONE', #14219, .T. ) ;
#5782=CARTESIAN_POINT ( 'NONE',  ( 104.2468583329775811, -46.74335657891433726, 18.35848241876792031 ) ) ;
#5784=AXIS2_PLACEMENT_3D ( 'NONE', #2978, #23876, #44736 ) ;
#5786=CARTESIAN_POINT ( 'NONE',  ( 36.65249034007450746, -49.32844715994130524, 129.9678068554150911 ) ) ;
#5787=CARTESIAN_POINT ( 'NONE',  ( 105.2433400634091925, -28.35518594498741507, 259.6695626852197734 ) ) ;
#5788=ORIENTED_EDGE ( 'NONE', *, *, #15223, .T. ) ;
#5789=ORIENTED_EDGE ( 'NONE', *, *, #65411, .T. ) ;
#5790=CIRCLE ( 'NONE', #75224, 2.029999999999997140 ) ;
#5791=CIRCLE ( 'NONE', #85559, 2.124999999999994227 ) ;
#5793=EDGE_CURVE ( 'NONE', #16304, #57152, #43382, .T. ) ;
#5795=CARTESIAN_POINT ( 'NONE',  ( 98.15101130392974937, -41.26167982539337942, 101.7011238567067011 ) ) ;
#5796=DIRECTION ( 'NONE',  ( -1.000000000000000078E-15, 0.000000000000000000, 1.000000000000000000 ) ) ;
#5797=CARTESIAN_POINT ( 'NONE',  ( 115.0859250807818910, -30.61377459442804039, 274.3439221958257690 ) ) ;
#5799=CARTESIAN_POINT ( 'NONE',  ( 114.4295241859595933, -42.56572631025478870, 44.73682140113599814 ) ) ;
#5800=DIRECTION ( 'NONE',  ( 0.000000000000000000, -1.000000000000000000, 0.000000000000000000 ) ) ;
#5801=AXIS2_PLACEMENT_3D ( 'NONE', #51830, #31849, #23724 ) ;
#5803=CARTESIAN_POINT ( 'NONE',  ( 83.56670390244799762, -36.72944715994108122, 229.5838068554169524 ) ) ;
#5805=CARTESIAN_POINT ( 'NONE',  ( 103.3362402991319442, -47.20309360805218546, 252.3041967044827913 ) ) ;
#5806=LINE ( 'NONE', #27580, #71941 ) ;
#5807=EDGE_CURVE ( 'NONE', #83951, #5456, #42041, .T. ) ;
#5808=ORIENTED_EDGE ( 'NONE', *, *, #45188, .F. ) ;
#5811=CIRCLE ( 'NONE', #76866, 5.599999999999994316 ) ;
#5812=CARTESIAN_POINT ( 'NONE',  ( 25.56670390244797275, -62.87844715994099687, 142.0928068554150059 ) ) ;
#5813=CARTESIAN_POINT ( 'NONE',  ( 114.9159532999967723, -33.08434830970520579, 56.97856656006794651 ) ) ;
#5817=CARTESIAN_POINT ( 'NONE',  ( 57.56670390244718760, -42.82844715994040996, 170.7178068554150911 ) ) ;
#5818=LINE ( 'NONE', #39860, #5342 ) ;
#5819=EDGE_LOOP ( 'NONE', ( #59355, #48354 ) ) ;
#5822=CARTESIAN_POINT ( 'NONE',  ( 117.8008629928215782, -34.09274860618955216, 164.0061014663869798 ) ) ;
#5823=ORIENTED_EDGE ( 'NONE', *, *, #87919, .T. ) ;
#5824=CARTESIAN_POINT ( 'NONE',  ( 112.2084326156563066, -29.27471527533065299, 89.03051506617198640 ) ) ;
#5826=LINE ( 'NONE', #4018, #46016 ) ;
#5827=CARTESIAN_POINT ( 'NONE',  ( 117.1284314671335665, -36.25205438732766083, 115.2958690201829626 ) ) ;
#5828=DIRECTION ( 'NONE',  ( 0.7071067811985215501, -0.7071067811745735954, 0.000000000000000000 ) ) ;
#5829=DIRECTION ( 'NONE',  ( 1.000000000000000078E-15, -1.000000000000000083E-30, -1.000000000000000000 ) ) ;
#5830=AXIS2_PLACEMENT_3D ( 'NONE', #67234, #32715, #52678 ) ;
#5831=CARTESIAN_POINT ( 'NONE',  ( 95.32466046839788021, -34.95410283156319053, 67.20705384733894050 ) ) ;
#5832=DIRECTION ( 'NONE',  ( 0.7071067708032310328, 0.0001211784769794162209, 0.7071067811865502373 ) ) ;
#5833=DIRECTION ( 'NONE',  ( -0.9999999853157766072, -0.0001713722456120069274, 0.000000000000000000 ) ) ;
#5835=CARTESIAN_POINT ( 'NONE',  ( 77.55659459556798652, -19.85370728022772013, 2.783021134847694089 ) ) ;
#5838=EDGE_CURVE ( 'NONE', #52709, #40784, #55647, .T. ) ;
#5841=CARTESIAN_POINT ( 'NONE',  ( 97.44287158780957725, -40.59272077381807975, 251.6422919425783675 ) ) ;
#5842=CARTESIAN_POINT ( 'NONE',  ( 117.3314307007336481, -34.78826007317788083, 154.9756252759109714 ) ) ;
#5845=DIRECTION ( 'NONE',  ( 0.000000000000000000, -1.000000000000000000, 0.000000000000000000 ) ) ;
#5846=CARTESIAN_POINT ( 'NONE',  ( 100.2987399830848432, -46.45735886148204941, 83.09276813305294240 ) ) ;
#5849=ORIENTED_EDGE ( 'NONE', *, *, #60743, .F. ) ;
#5850=DIRECTION ( 'NONE',  ( 4.299999999999999979E-14, -1.000000000000000000, 0.000000000000000000 ) ) ;
#5851=VECTOR ( 'NONE', #66411, 1000.000000000000000 ) ;
#5853=CARTESIAN_POINT ( 'NONE',  ( 80.48314995793998605, 12.92155284005802862, 355.9756252759109998 ) ) ;
#5854=ORIENTED_EDGE ( 'NONE', *, *, #63910, .T. ) ;
#5857=CARTESIAN_POINT ( 'NONE',  ( 149.4409906032289257, -0.9156555935619231645, 543.8623766218582887 ) ) ;
#5858=CARTESIAN_POINT ( 'NONE',  ( 116.5166575185069462, -42.41785904284980546, 278.3832443235298797 ) ) ;
#5859=LINE ( 'NONE', #61246, #43133 ) ;
#5860=CARTESIAN_POINT ( 'NONE',  ( 25.56670390244748248, -48.82844715994178841, 137.2178068554150627 ) ) ;
#5862=CARTESIAN_POINT ( 'NONE',  ( 101.7353989658528661, -28.52926574610319932, 25.53562527591096654 ) ) ;
#5864=CARTESIAN_POINT ( 'NONE',  ( 111.7842945758856246, -25.88553347519915349, 130.7499109901969518 ) ) ;
#5865=CARTESIAN_POINT ( 'NONE',  ( 138.0667039024479550, -14.72944715994091069, 199.5838068554170093 ) ) ;
#5866=CARTESIAN_POINT ( 'NONE',  ( 117.1686558484209826, -33.85615284218268073, 149.0470538473389581 ) ) ;
#5872=DIRECTION ( 'NONE',  ( 3.999999999999999995E-14, -1.000000000000000000, 4.100000000000000342E-29 ) ) ;
#5873=CARTESIAN_POINT ( 'NONE',  ( 177.4809174648215730, -48.32844715993478246, 129.9678068554150059 ) ) ;
#5874=ORIENTED_EDGE ( 'NONE', *, *, #70925, .T. ) ;
#5875=CARTESIAN_POINT ( 'NONE',  ( 109.7274606350641903, -27.00149574038083955, 60.86486693327666586 ) ) ;
#5876=CARTESIAN_POINT ( 'NONE',  ( 103.4531379826000261, -46.55545292317445671, 142.2956252759109645 ) ) ;
#5877=ORIENTED_EDGE ( 'NONE', *, *, #45802, .T. ) ;
#5880=DIRECTION ( 'NONE',  ( -0.7071067812123270624, -0.7071067811607679721, 0.000000000000000000 ) ) ;
#5882=ORIENTED_EDGE ( 'NONE', *, *, #80979, .T. ) ;
#5883=EDGE_LOOP ( 'NONE', ( #43237, #15243 ) ) ;
#5884=AXIS2_PLACEMENT_3D ( 'NONE', #62901, #41110, #42896 ) ;
#5886=CIRCLE ( 'NONE', #77010, 7.499999999999996447 ) ;
#5889=CARTESIAN_POINT ( 'NONE',  ( 107.8867142951287974, -26.70539886071778923, 250.0113088905621623 ) ) ;
#5890=CARTESIAN_POINT ( 'NONE',  ( 41.56648329127399677, 0.2215528400590013880, 258.9256252759120116 ) ) ;
#5891=CARTESIAN_POINT ( 'NONE',  ( 115.8252488141339427, -31.72970135207203057, 104.2398208576954630 ) ) ;
#5892=LINE ( 'NONE', #45844, #22545 ) ;
#5894=AXIS2_PLACEMENT_3D ( 'NONE', #3564, #31263, #10821 ) ;
#5895=ORIENTED_EDGE ( 'NONE', *, *, #65706, .T. ) ;
#5896=FACE_OUTER_BOUND ( 'NONE', #83381, .T. ) ;
#5897=LINE ( 'NONE', #88573, #28871 ) ;
#5898=EDGE_CURVE ( 'NONE', #2880, #34477, #35022, .T. ) ;
#5899=CARTESIAN_POINT ( 'NONE',  ( 116.5663773505004315, -40.88766770462209621, 204.4861014663869696 ) ) ;
#5900=DIRECTION ( 'NONE',  ( 1.000000000000000078E-15, 1.000000000000000083E-30, -1.000000000000000000 ) ) ;
#5901=ORIENTED_EDGE ( 'NONE', *, *, #50920, .F. ) ;
#5902=ADVANCED_FACE ( 'NONE', ( #85650 ), #23428, .T. ) ;
#5903=CARTESIAN_POINT ( 'NONE',  ( 108.4470127171751983, -27.04659769318761775, 100.9641967044819779 ) ) ;
#5904=CARTESIAN_POINT ( 'NONE',  ( 151.0371591254572934, -24.42818131005592974, 313.9678068554149490 ) ) ;
#5905=DIRECTION ( 'NONE',  ( 0.000000000000000000, 0.000000000000000000, 1.000000000000000000 ) ) ;
#5906=AXIS2_PLACEMENT_3D ( 'NONE', #42863, #7472, #206 ) ;
#5907=CARTESIAN_POINT ( 'NONE',  ( 162.7866693523298522, -36.02818131005322755, 237.4678068554150059 ) ) ;
#5908=VECTOR ( 'NONE', #36831, 1000.000000000000000 ) ;
#5909=EDGE_CURVE ( 'NONE', #2603, #55318, #48041, .T. ) ;
#5912=ADVANCED_FACE ( 'NONE', ( #25176 ), #23859, .T. ) ;
#5914=ORIENTED_EDGE ( 'NONE', *, *, #62547, .F. ) ;
#5915=ORIENTED_EDGE ( 'NONE', *, *, #38752, .T. ) ;
#5916=B_SPLINE_CURVE_WITH_KNOTS ( 'NONE', 3,
 ( #41503, #7003, #29246, #14274, #84224, #34701, #62407, #84668, #21994, #186, #55563, #83314, #22433, #41949, #50109, #77846, #16952, #37393 ),
 .UNSPECIFIED., .F., .F.,
 ( 4, 2, 2, 2, 2, 2, 2, 2, 4 ),
 ( 0.5000699581767007462, 0.5625612134046131807, 0.6250524686325256152, 0.6875437238604379386, 0.7500349790883503731, 0.8125262343162628076, 0.8750174895441751310, 0.9375087447720875655, 1.000000000000000000 ),
 .UNSPECIFIED. ) ;
#5917=CARTESIAN_POINT ( 'NONE',  ( 114.2010777387499587, -30.61601215110631458, 225.8339642582779447 ) ) ;
#5918=AXIS2_PLACEMENT_3D ( 'NONE', #23646, #43608, #8217 ) ;
#5919=EDGE_CURVE ( 'NONE', #1069, #69462, #2523, .T. ) ;
#5923=CARTESIAN_POINT ( 'NONE',  ( 109.6430120555397707, -46.48008675582220661, 153.7814586030977466 ) ) ;
#5924=CIRCLE ( 'NONE', #47977, 15.69999999999999574 ) ;
#5925=CARTESIAN_POINT ( 'NONE',  ( 83.73314995794051185, 12.92155284005802685, 335.5992267699911054 ) ) ;
#5926=VERTEX_POINT ( 'NONE', #3406 ) ;
#5927=CARTESIAN_POINT ( 'NONE',  ( 179.4595971212723100, -26.00627455218570461, 313.9678068554149490 ) ) ;
#5928=CARTESIAN_POINT ( 'NONE',  ( 172.5664832912740110, 0.2215528400590013880, 318.9256252759120116 ) ) ;
#5930=CARTESIAN_POINT ( 'NONE',  ( 105.1635383257858507, -47.00901688944614421, 12.42991099019596923 ) ) ;
#5931=VERTEX_POINT ( 'NONE', #65623 ) ;
#5932=CARTESIAN_POINT ( 'NONE',  ( 101.7278717236064836, -30.55458258274888905, 258.4623760838770750 ) ) ;
#5935=CARTESIAN_POINT ( 'NONE',  ( 97.29384000864233428, -37.12803473146956890, 161.3584824187679487 ) ) ;
#5937=CARTESIAN_POINT ( 'NONE',  ( 107.0664832912739968, -36.72944715994100306, 287.6356252759109680 ) ) ;
#5938=CARTESIAN_POINT ( 'NONE',  ( 165.2748236753140247, -30.08671355700301575, -5.074374724088000832 ) ) ;
#5939=CARTESIAN_POINT ( 'NONE',  ( 25.56670390244797275, -48.82844715994099971, 293.2178068554150627 ) ) ;
#5941=CARTESIAN_POINT ( 'NONE',  ( 98.80492496406409941, -29.31701487593723598, 231.7565776568629587 ) ) ;
#5944=CARTESIAN_POINT ( 'NONE',  ( 96.61310803562074057, -37.29506674262550803, 72.36991099019596163 ) ) ;
#5945=CARTESIAN_POINT ( 'NONE',  ( 87.06648329127401098, -46.72944715994105280, 14.67562527591094934 ) ) ;
#5946=ORIENTED_EDGE ( 'NONE', *, *, #11065, .F. ) ;
#5948=ORIENTED_EDGE ( 'NONE', *, *, #50388, .T. ) ;
#5949=CIRCLE ( 'NONE', #33488, 13.00000000000000355 ) ;
#5951=CARTESIAN_POINT ( 'NONE',  ( 98.34940958104101583, -31.65739082969338369, 160.9063178345361962 ) ) ;
#5952=DIRECTION ( 'NONE',  ( -1.000000000000000000, 0.000000000000000000, 1.071939472051879986E-15 ) ) ;
#5953=PLANE ( 'NONE',  #79958 ) ;
#5954=FACE_BOUND ( 'NONE', #68854, .T. ) ;
#5955=VECTOR ( 'NONE', #8460, 1000.000000000000000 ) ;
#5956=CARTESIAN_POINT ( 'NONE',  ( 114.6928066196564515, -42.01481596195104373, 161.1623760838769783 ) ) ;
#5957=CARTESIAN_POINT ( 'NONE',  ( 99.38090234834324121, -28.75341736348360655, 261.6746728949589169 ) ) ;
#5958=CARTESIAN_POINT ( 'NONE',  ( 112.0640897386794563, -45.48941479919412245, 58.98962357542096413 ) ) ;
#5962=ADVANCED_FACE ( 'NONE', ( #72450 ), #59246, .F. ) ;
#5963=CARTESIAN_POINT ( 'NONE',  ( 41.56648329127398966, -27.82844715994070484, 18.92562527591200094 ) ) ;
#5964=CIRCLE ( 'NONE', #17554, 2.500000000000002220 ) ;
#5969=VERTEX_POINT ( 'NONE', #2961 ) ;
#5970=VERTEX_POINT ( 'NONE', #30663 ) ;
#5972=CARTESIAN_POINT ( 'NONE',  ( 128.5492039024480846, -58.72944715994093201, 207.5838068554170377 ) ) ;
#5973=DIRECTION ( 'NONE',  ( -1.000000000000000000, 1.011922027653136551E-15, 0.000000000000000000 ) ) ;
#5974=CARTESIAN_POINT ( 'NONE',  ( 112.9548150380649503, -42.91681406074877003, 157.6038483995049830 ) ) ;
#5975=CARTESIAN_POINT ( 'NONE',  ( 104.7497970125497204, -46.93922829031851762, 72.39848241876795498 ) ) ;
#5976=CARTESIAN_POINT ( 'NONE',  ( 25.56670390244828539, -48.82844715994168183, 295.7178068554150059 ) ) ;
#5977=EDGE_LOOP ( 'NONE', ( #88634, #62408 ) ) ;
#5979=ORIENTED_EDGE ( 'NONE', *, *, #87623, .T. ) ;
#5982=ORIENTED_EDGE ( 'NONE', *, *, #85735, .T. ) ;
#5983=DIRECTION ( 'NONE',  ( 1.000000000000000000, 8.673617379883546378E-16, 9.757819552368989676E-16 ) ) ;
#5985=FACE_OUTER_BOUND ( 'NONE', #54548, .T. ) ;
#5986=AXIS2_PLACEMENT_3D ( 'NONE', #7656, #14927, #35344 ) ;
#5987=ADVANCED_FACE ( 'NONE', ( #44721 ), #10218, .T. ) ;
#5988=CYLINDRICAL_SURFACE ( 'NONE', #36500, 0.9999999999999731326 ) ;
#5989=ORIENTED_EDGE ( 'NONE', *, *, #47000, .T. ) ;
#5990=CARTESIAN_POINT ( 'NONE',  ( 99.27722696178533113, -43.74484797918319856, 56.90991099019593236 ) ) ;
#5991=CARTESIAN_POINT ( 'NONE',  ( 106.8402480490632342, -48.62734320582506342, 73.56133956162497611 ) ) ;
#5994=FACE_OUTER_BOUND ( 'NONE', #22245, .T. ) ;
#5995=CARTESIAN_POINT ( 'NONE',  ( 107.0664832912739399, -36.72944715994096754, 296.5517437918485939 ) ) ;
#5997=VERTEX_POINT ( 'NONE', #73326 ) ;
#5998=CIRCLE ( 'NONE', #22017, 4.875000000000017764 ) ;
#5999=DIRECTION ( 'NONE',  ( 9.351236661543306751E-17, -3.725950533538267725E-29, -1.000000000000000000 ) ) ;
#6000=CIRCLE ( 'NONE', #69800, 7.499999999999996447 ) ;
#6001=CARTESIAN_POINT ( 'NONE',  ( 107.0664832912750057, -36.72944715993903486, 9.125625275910969947 ) ) ;
#6002=DIRECTION ( 'NONE',  ( 0.000000000000000000, 1.000000000000000000, 0.000000000000000000 ) ) ;
#6003=VERTEX_POINT ( 'NONE', #79724 ) ;
#6004=CARTESIAN_POINT ( 'NONE',  ( 97.20510023974232183, -31.68580462152881339, 91.96229194257693962 ) ) ;
#6007=CYLINDRICAL_SURFACE ( 'NONE', #84289, 2.749999999999974687 ) ;
#6008=EDGE_CURVE ( 'NONE', #86967, #60336, #52402, .T. ) ;
#6011=ORIENTED_EDGE ( 'NONE', *, *, #6855, .T. ) ;
#6012=EDGE_CURVE ( 'NONE', #17169, #71916, #56867, .T. ) ;
#6013=CARTESIAN_POINT ( 'NONE',  ( 99.36524671511907059, -42.81259845621065807, 87.85848241876792031 ) ) ;
#6017=EDGE_CURVE ( 'NONE', #11918, #36895, #80112, .T. ) ;
#6018=CARTESIAN_POINT ( 'NONE',  ( 117.4525030917817645, -36.13006561810995976, 224.8727681330539667 ) ) ;
#6020=CARTESIAN_POINT ( 'NONE',  ( 116.5687119429383642, -33.54617018878323620, 149.0836319459096728 ) ) ;
#6021=FACE_OUTER_BOUND ( 'NONE', #49369, .T. ) ;
#6022=CARTESIAN_POINT ( 'NONE',  ( 109.7248659309123013, -27.00080518256924478, 80.86479194179250385 ) ) ;
#6024=ADVANCED_FACE ( 'NONE', ( #10652 ), #38358, .F. ) ;
#6026=CARTESIAN_POINT ( 'NONE',  ( 103.2980200187117390, -27.06831524915186904, 170.3603871806729444 ) ) ;
#6027=ORIENTED_EDGE ( 'NONE', *, *, #49419, .T. ) ;
#6028=ORIENTED_EDGE ( 'NONE', *, *, #41359, .T. ) ;
#6029=CARTESIAN_POINT ( 'NONE',  ( 97.68334685095105385, -37.21243378447991290, 117.8111071154209526 ) ) ;
#6031=CIRCLE ( 'NONE', #58270, 5.599999999999994316 ) ;
#6032=DIRECTION ( 'NONE',  ( 1.000000000000000000, 0.000000000000000000, 0.000000000000000000 ) ) ;
#6033=CARTESIAN_POINT ( 'NONE',  ( 100.0046238269857639, -29.91446987444276928, 246.7156252759109520 ) ) ;
#6034=DIRECTION ( 'NONE',  ( 4.299999999999999979E-14, -1.000000000000000000, 4.400000000000000367E-29 ) ) ;
#6035=DIRECTION ( 'NONE',  ( -1.000000000000000078E-15, 0.000000000000000000, 1.000000000000000000 ) ) ;
#6037=DIRECTION ( 'NONE',  ( 0.000000000000000000, 1.000000000000000000, 0.000000000000000000 ) ) ;
#6042=CARTESIAN_POINT ( 'NONE',  ( 103.7301789885933658, -26.21598454391059363, 205.3089586092439731 ) ) ;
#6044=EDGE_LOOP ( 'NONE', ( #76094, #26745 ) ) ;
#6046=AXIS2_PLACEMENT_3D ( 'NONE', #3556, #53001, #61637 ) ;
#6047=DIRECTION ( 'NONE',  ( 0.000000000000000000, 0.000000000000000000, -1.000000000000000000 ) ) ;
#6048=CARTESIAN_POINT ( 'NONE',  ( 79.31510987520707090, -16.05633243510678554, 1.690787911858472770 ) ) ;
#6050=CARTESIAN_POINT ( 'NONE',  ( 36.65249034007535300, -49.32844715994124130, 249.9678068554150343 ) ) ;
#6051=AXIS2_PLACEMENT_3D ( 'NONE', #88438, #81637, #18938 ) ;
#6052=CARTESIAN_POINT ( 'NONE',  ( 25.56670390244797275, -58.35344715994099829, 134.4678068554150059 ) ) ;
#6053=ORIENTED_EDGE ( 'NONE', *, *, #84154, .F. ) ;
#6054=CARTESIAN_POINT ( 'NONE',  ( 100.8869726253045513, -44.69981113982900922, 62.05224101154388450 ) ) ;
#6055=CARTESIAN_POINT ( 'NONE',  ( 118.7903470546216482, -38.45904373001069843, 223.7099109901969598 ) ) ;
#6056=VERTEX_POINT ( 'NONE', #4744 ) ;
#6060=DIRECTION ( 'NONE',  ( -4.237773401492740281E-14, 1.000000000000000000, 0.000000000000000000 ) ) ;
#6061=CARTESIAN_POINT ( 'NONE',  ( 109.0595394021483742, -27.66723669546327358, 27.72237608387795404 ) ) ;
#6062=CARTESIAN_POINT ( 'NONE',  ( 116.8268856436350518, -43.49382415615948361, 159.3441967044829539 ) ) ;
#6064=ORIENTED_EDGE ( 'NONE', *, *, #6716, .T. ) ;
#6065=EDGE_CURVE ( 'NONE', #73752, #73831, #6095, .T. ) ;
#6066=DIRECTION ( 'NONE',  ( -2.108538789381372925E-16, 0.5150380749100580413, 0.8571673007021100021 ) ) ;
#6067=CARTESIAN_POINT ( 'NONE',  ( 115.6377686515996999, -42.05128457402461351, 68.38507870720354731 ) ) ;
#6069=EDGE_LOOP ( 'NONE', ( #19306, #40053, #46832, #51115 ) ) ;
#6072=ORIENTED_EDGE ( 'NONE', *, *, #38605, .T. ) ;
#6074=CARTESIAN_POINT ( 'NONE',  ( 109.1774539423994952, -45.00591588954721800, 47.19813411379097801 ) ) ;
#6075=CARTESIAN_POINT ( 'NONE',  ( 97.45268567403179816, -40.90835349962023315, 231.6527681330539679 ) ) ;
#6076=CARTESIAN_POINT ( 'NONE',  ( 97.93839266929572318, -41.72010113774609152, 221.7241967044819546 ) ) ;
#6077=LINE ( 'NONE', #33766, #20000 ) ;
#6078=CARTESIAN_POINT ( 'NONE',  ( 101.6204011159890541, -47.22657592904984369, 13.19562527591094891 ) ) ;
#6079=DIRECTION ( 'NONE',  ( 0.000000000000000000, 1.000000000000000000, 0.000000000000000000 ) ) ;
#6080=DIRECTION ( 'NONE',  ( 0.000000000000000000, 1.000000000000000000, 0.000000000000000000 ) ) ;
#6081=ORIENTED_EDGE ( 'NONE', *, *, #80766, .T. ) ;
#6082=VECTOR ( 'NONE', #11793, 1000.000000000000000 ) ;
#6083=AXIS2_PLACEMENT_3D ( 'NONE', #79258, #54520, #62255 ) ;
#6084=CARTESIAN_POINT ( 'NONE',  ( 97.28369645613162220, -37.51102008256657427, 101.3899109901979472 ) ) ;
#6086=CARTESIAN_POINT ( 'NONE',  ( 113.3690198962888758, -27.59211078819982887, 89.60800622829195561 ) ) ;
#6087=CARTESIAN_POINT ( 'NONE',  ( 118.1543649935527185, -36.20813824561556515, 268.8518157521014587 ) ) ;
#6089=CARTESIAN_POINT ( 'NONE',  ( 96.85831052012196096, -34.61278962133658155, 216.1641967044819808 ) ) ;
#6090=CARTESIAN_POINT ( 'NONE',  ( 107.0664832912739968, -36.72944715994100306, 287.6356252759109680 ) ) ;
#6091=CARTESIAN_POINT ( 'NONE',  ( 99.50458969558927436, -43.30562421865187872, 22.89600243872639140 ) ) ;
#6092=LINE ( 'NONE', #12449, #22404 ) ;
#6093=CARTESIAN_POINT ( 'NONE',  ( 114.7357040289479642, -40.07855725538382075, 277.6356252759111953 ) ) ;
#6095=LINE ( 'NONE', #18361, #87295 ) ;
#6096=DIRECTION ( 'NONE',  ( 1.000000000000000078E-15, -1.000000000000000083E-30, -1.000000000000000000 ) ) ;
#6098=DIRECTION ( 'NONE',  ( 0.000000000000000000, 1.000000000000000000, 0.000000000000000000 ) ) ;
#6102=CARTESIAN_POINT ( 'NONE',  ( 101.1435383712028511, -28.73162758398862238, 195.5838068554171514 ) ) ;
#6103=ORIENTED_EDGE ( 'NONE', *, *, #36413, .F. ) ;
#6104=CYLINDRICAL_SURFACE ( 'NONE', #64082, 0.4999999999999982236 ) ;
#6105=CARTESIAN_POINT ( 'NONE',  ( 100.7367085078155640, -45.81951824476916357, 237.0803871806729717 ) ) ;
#6106=CARTESIAN_POINT ( 'NONE',  ( 103.1746689306972939, -27.05803214298817849, 126.3813395616259783 ) ) ;
#6107=CARTESIAN_POINT ( 'NONE',  ( 101.2698767154569168, -26.33663883357058921, 251.4813395616249920 ) ) ;
#6109=FACE_OUTER_BOUND ( 'NONE', #40985, .T. ) ;
#6111=DIRECTION ( 'NONE',  ( 1.000000000000000000, -5.337610695313248426E-16, 0.000000000000000000 ) ) ;
#6113=AXIS2_PLACEMENT_3D ( 'NONE', #34013, #61714, #14494 ) ;
#6115=VECTOR ( 'NONE', #1267, 1000.000000000000000 ) ;
#6117=ORIENTED_EDGE ( 'NONE', *, *, #29807, .T. ) ;
#6118=EDGE_CURVE ( 'NONE', #686, #19911, #65828, .T. ) ;
#6120=CARTESIAN_POINT ( 'NONE',  ( 108.3145574644059224, -45.20850512633867169, 142.1152769709339907 ) ) ;
#6125=CARTESIAN_POINT ( 'NONE',  ( 96.72090476913471946, -37.82382852467499390, 122.4099109901969626 ) ) ;
#6126=CARTESIAN_POINT ( 'NONE',  ( 105.7137884042412139, -46.72360237654041271, 148.4694629689294061 ) ) ;
#6127=ADVANCED_FACE ( 'NONE', ( #34225 ), #74235, .T. ) ;
#6128=AXIS2_PLACEMENT_3D ( 'NONE', #20061, #25977, #47294 ) ;
#6129=DIRECTION ( 'NONE',  ( -0.000000000000000000, 1.000000000000000000, 0.000000000000000000 ) ) ;
#6130=LINE ( 'NONE', #74709, #43288 ) ;
#6131=EDGE_CURVE ( 'NONE', #43708, #22746, #39694, .T. ) ;
#6133=CARTESIAN_POINT ( 'NONE',  ( 113.0644005321300511, -46.09090919705352718, 68.02991099019695298 ) ) ;
#6134=ORIENTED_EDGE ( 'NONE', *, *, #75777, .T. ) ;
#6135=VERTEX_POINT ( 'NONE', #80612 ) ;
#6136=ORIENTED_EDGE ( 'NONE', *, *, #29617, .T. ) ;
#6138=CARTESIAN_POINT ( 'NONE',  ( 114.0663967180212950, -29.08153105160607410, 150.4746728949579619 ) ) ;
#6139=DIRECTION ( 'NONE',  ( 0.000000000000000000, 1.000000000000000000, 0.000000000000000000 ) ) ;
#6141=CARTESIAN_POINT ( 'NONE',  ( 182.4202572930258839, -31.94127993907126140, 237.4678068554150059 ) ) ;
#6142=ADVANCED_FACE ( 'NONE', ( #60128 ), #60583, .T. ) ;
#6143=CARTESIAN_POINT ( 'NONE',  ( 86.06670390244796920, -50.82844715994100682, 250.9178068554150514 ) ) ;
#6145=CYLINDRICAL_SURFACE ( 'NONE', #12475, 2.517499999999998739 ) ;
#6146=CARTESIAN_POINT ( 'NONE',  ( 115.1498815335951491, -43.27828968249936992, 88.28419670448195689 ) ) ;
#6148=VERTEX_POINT ( 'NONE', #81517 ) ;
#6150=CARTESIAN_POINT ( 'NONE',  ( 51.06648329127400388, 19.62155284005901024, 333.4006252759110112 ) ) ;
#6154=CARTESIAN_POINT ( 'NONE',  ( 116.3142130228717264, -37.48801553205211690, 186.5795189410199555 ) ) ;
#6155=CIRCLE ( 'NONE', #56895, 2.517500000000005844 ) ;
#6156=CARTESIAN_POINT ( 'NONE',  ( 97.07209691576048272, -35.37819998029382162, 27.21882120925108239 ) ) ;
#6157=EDGE_LOOP ( 'NONE', ( #84451, #51196, #64072, #13535 ) ) ;
#6158=ORIENTED_EDGE ( 'NONE', *, *, #70057, .F. ) ;
#6160=DIRECTION ( 'NONE',  ( -1.000000000000000078E-15, 1.000000000000000083E-30, 1.000000000000000000 ) ) ;
#6161=CARTESIAN_POINT ( 'NONE',  ( 134.0664832912739826, -21.47944715994100306, 1.625625275910997480 ) ) ;
#6162=VERTEX_POINT ( 'NONE', #21059 ) ;
#6163=ORIENTED_EDGE ( 'NONE', *, *, #33409, .T. ) ;
#6164=CARTESIAN_POINT ( 'NONE',  ( 77.43469508765193154, -19.52719034724596270, 6.916533740477924574 ) ) ;
#6166=CARTESIAN_POINT ( 'NONE',  ( 106.8838381269920745, -46.12323054477403161, 223.9806309249449612 ) ) ;
#6167=EDGE_CURVE ( 'NONE', #20535, #26172, #16240, .T. ) ;
#6172=AXIS2_PLACEMENT_3D ( 'NONE', #87194, #24958, #10438 ) ;
#6173=CARTESIAN_POINT ( 'NONE',  ( 107.0667039024479834, -36.72944715994100306, 239.5838068554170093 ) ) ;
#6175=ORIENTED_EDGE ( 'NONE', *, *, #43855, .F. ) ;
#6178=CARTESIAN_POINT ( 'NONE',  ( 102.8259602516037177, -43.70423678882019658, 244.9595189410199794 ) ) ;
#6179=CARTESIAN_POINT ( 'NONE',  ( 95.28658997325378266, -38.28252189325972665, 151.4299109901969871 ) ) ;
#6180=CARTESIAN_POINT ( 'NONE',  ( 110.4495079430909641, -47.22796928374267367, 57.83657765686300678 ) ) ;
#6181=CARTESIAN_POINT ( 'NONE',  ( 112.3819288266831933, -43.64340785303151904, 249.5838068554168956 ) ) ;
#6182=CARTESIAN_POINT ( 'NONE',  ( 188.5667039024479834, -65.37844715994100397, 173.2178068554149775 ) ) ;
#6183=CARTESIAN_POINT ( 'NONE',  ( 108.0878824955162969, -25.31592121169968479, 322.1035414506763459 ) ) ;
#6184=CARTESIAN_POINT ( 'NONE',  ( 106.9749963086187279, -47.15413504876184447, 183.5699109901969734 ) ) ;
#6185=DIRECTION ( 'NONE',  ( -1.000000000000000078E-15, 1.000000000000000083E-30, 1.000000000000000000 ) ) ;
#6186=ORIENTED_EDGE ( 'NONE', *, *, #1081, .F. ) ;
#6188=ORIENTED_EDGE ( 'NONE', *, *, #16385, .F. ) ;
#6189=ORIENTED_EDGE ( 'NONE', *, *, #87977, .F. ) ;
#6191=ORIENTED_EDGE ( 'NONE', *, *, #64163, .T. ) ;
#6193=ADVANCED_FACE ( 'NONE', ( #82854 ), #14248, .T. ) ;
#6194=( BOUNDED_CURVE ( )  B_SPLINE_CURVE ( 3, ( #77075, #51572, #3000, #72921 ),
 .UNSPECIFIED., .F., .F. ) 
 B_SPLINE_CURVE_WITH_KNOTS ( ( 4, 4 ),
 ( 3.141592653593537232, 4.712388980388810822 ),
 .UNSPECIFIED. ) 
 CURVE ( )  GEOMETRIC_REPRESENTATION_ITEM ( )  RATIONAL_B_SPLINE_CURVE ( ( 1.000000000000000000, 0.8047378541242761196, 0.8047378541242761196, 1.000000000000000000 ) ) 
 REPRESENTATION_ITEM ( '' )  );
#6195=CARTESIAN_POINT ( 'NONE',  ( 102.5580992528948912, -27.32936716964785262, 95.43276813305395478 ) ) ;
#6198=PLANE ( 'NONE',  #52814 ) ;
#6199=DIRECTION ( 'NONE',  ( 0.000000000000000000, 0.000000000000000000, -1.000000000000000000 ) ) ;
#6200=LINE ( 'NONE', #12563, #31077 ) ;
#6201=CARTESIAN_POINT ( 'NONE',  ( 101.4371718687638406, -46.21494532752021200, 203.1622919425779514 ) ) ;
#6202=DIRECTION ( 'NONE',  ( 1.000000000000000078E-15, -1.000000000000000083E-30, -1.000000000000000000 ) ) ;
#6204=EDGE_LOOP ( 'NONE', ( #70066, #3026, #55067, #82122 ) ) ;
#6205=FACE_OUTER_BOUND ( 'NONE', #16900, .T. ) ;
#6206=VECTOR ( 'NONE', #17621, 1000.000000000000000 ) ;
#6208=DIRECTION ( 'NONE',  ( 1.000000000000000078E-15, -1.000000000000000083E-30, -1.000000000000000000 ) ) ;
#6210=CARTESIAN_POINT ( 'NONE',  ( 100.2192867603235840, -28.80968922735345927, 260.6441967044821695 ) ) ;
#6211=ORIENTED_EDGE ( 'NONE', *, *, #47633, .F. ) ;
#6213=CARTESIAN_POINT ( 'NONE',  ( 117.4513846513745960, -35.59318846168486772, 274.9127681330539872 ) ) ;
#6214=CARTESIAN_POINT ( 'NONE',  ( 114.5432832596865325, -29.39626808186021378, 145.4441967044819819 ) ) ;
#6216=CARTESIAN_POINT ( 'NONE',  ( 97.80494262393504812, -40.50090711907665764, 102.6342054156130246 ) ) ;
#6218=PLANE ( 'NONE',  #57329 ) ;
#6219=CARTESIAN_POINT ( 'NONE',  ( 134.0664832912740110, -46.72944715994100306, 4.925625275910997303 ) ) ;
#6222=CIRCLE ( 'NONE', #81646, 2.500000000000002220 ) ;
#6223=ORIENTED_EDGE ( 'NONE', *, *, #82792, .T. ) ;
#6225=EDGE_CURVE ( 'NONE', #59810, #42074, #66992, .T. ) ;
#6226=VERTEX_POINT ( 'NONE', #42370 ) ;
#6228=CARTESIAN_POINT ( 'NONE',  ( 116.4547782460826255, -32.24742764444982157, 15.18133956162492915 ) ) ;
#6229=CARTESIAN_POINT ( 'NONE',  ( 164.9667039024475059, -28.27351298636832766, 237.4678068554150059 ) ) ;
#6230=ADVANCED_FACE ( 'NONE', ( #55093 ), #76016, .T. ) ;
#6231=DIRECTION ( 'NONE',  ( -0.000000000000000000, -0.000000000000000000, -1.000000000000000000 ) ) ;
#6232=CARTESIAN_POINT ( 'NONE',  ( 182.4202572930400095, -33.70561438051981185, -5.074374724088000832 ) ) ;
#6233=CARTESIAN_POINT ( 'NONE',  ( 116.0913394378304702, -33.14858145062638073, 248.5495626852199678 ) ) ;
#6235=ORIENTED_EDGE ( 'NONE', *, *, #28451, .T. ) ;
#6236=EDGE_LOOP ( 'NONE', ( #15494, #3095, #25016, #35416 ) ) ;
#6238=CARTESIAN_POINT ( 'NONE',  ( 34.67381068360400320, -28.98061976758901892, -5.074374724088000832 ) ) ;
#6239=CARTESIAN_POINT ( 'NONE',  ( 105.7155907543573790, -46.72387588654685686, 102.4688864389793110 ) ) ;
#6240=DIRECTION ( 'NONE',  ( 6.524622321627019585E-16, 3.741823817616790462E-31, 1.000000000000000000 ) ) ;
#6241=CARTESIAN_POINT ( 'NONE',  ( 99.09464024186353015, -30.55185734356122396, 275.8020006352290352 ) ) ;
#6247=CARTESIAN_POINT ( 'NONE',  ( 105.2300248619626757, -26.52326248392216357, 275.2061014663877927 ) ) ;
#6248=DIRECTION ( 'NONE',  ( 4.299999999999999979E-14, -1.000000000000000000, 4.400000000000000367E-29 ) ) ;
#6250=LINE ( 'NONE', #68921, #12940 ) ;
#6251=DIRECTION ( 'NONE',  ( 1.000000000000000078E-15, 1.000000000000000083E-30, -1.000000000000000000 ) ) ;
#6252=CARTESIAN_POINT ( 'NONE',  ( 114.9276189159122907, -38.92769025571944042, 96.42809036959192781 ) ) ;
#6254=CARTESIAN_POINT ( 'NONE',  ( 97.81169160209351787, -40.51741184665055329, 67.63577596198375375 ) ) ;
#6255=ORIENTED_EDGE ( 'NONE', *, *, #19055, .F. ) ;
#6256=CARTESIAN_POINT ( 'NONE',  ( 78.35735255115685050, -34.57277629267482411, 7.749696248610925764 ) ) ;
#6259=CARTESIAN_POINT ( 'NONE',  ( 97.98636869442889008, -41.85180495037556625, 136.7356252759109623 ) ) ;
#6261=CARTESIAN_POINT ( 'NONE',  ( 41.56648329127499153, -32.07844715994070839, 263.6756252759120116 ) ) ;
#6262=CARTESIAN_POINT ( 'NONE',  ( 98.20536012454746810, -36.63577306554869750, 107.7501547344689783 ) ) ;
#6263=CARTESIAN_POINT ( 'NONE',  ( 63.03715912545826683, -46.82818131006018092, 236.4678068554150343 ) ) ;
#6265=CARTESIAN_POINT ( 'NONE',  ( 118.8673094125028200, -35.40175986820349152, 79.91562527591095488 ) ) ;
#6267=CARTESIAN_POINT ( 'NONE',  ( 172.5667039024480687, -36.32844715993499563, 129.9678068554150059 ) ) ;
#6270=ORIENTED_EDGE ( 'NONE', *, *, #26131, .F. ) ;
#6271=ORIENTED_EDGE ( 'NONE', *, *, #25926, .T. ) ;
#6273=DIRECTION ( 'NONE',  ( 0.000000000000000000, 0.000000000000000000, 1.000000000000000000 ) ) ;
#6274=ORIENTED_EDGE ( 'NONE', *, *, #68447, .F. ) ;
#6275=CARTESIAN_POINT ( 'NONE',  ( 97.83217745605946902, -40.05230289513916375, 266.6013395616258776 ) ) ;
#6276=CARTESIAN_POINT ( 'NONE',  ( 95.28708132950120557, -38.28245711228485959, 147.4299109901969871 ) ) ;
#6278=CARTESIAN_POINT ( 'NONE',  ( 108.4174892569846946, -26.73503592839110610, 140.9689586088591966 ) ) ;
#6279=B_SPLINE_CURVE_WITH_KNOTS ( 'NONE', 3,
 ( #22716, #36336, #35422, #84047, #70413, #14097, #41777, #63592, #43125, #64045, #49942, #56302, #69513, #34975, #14999, #41330, #42673, #84950 ),
 .UNSPECIFIED., .F., .F.,
 ( 4, 2, 2, 2, 2, 2, 2, 2, 4 ),
 ( 0.5000003672892693318, 0.5625003213781106792, 0.6250002754669520266, 0.6875002295557932630, 0.7500001836446346104, 0.8125001377334759578, 0.8750000918223173052, 0.9375000459111586526, 1.000000000000000000 ),
 .UNSPECIFIED. ) ;
#6280=CARTESIAN_POINT ( 'NONE',  ( 110.1579320793587442, -46.68562272277494429, 93.81562527591097478 ) ) ;
#6281=CARTESIAN_POINT ( 'NONE',  ( 108.4209149160002710, -26.73547159001482498, 95.96804306659618078 ) ) ;
#6284=CARTESIAN_POINT ( 'NONE',  ( 112.0662701423777463, -45.48819631686011888, 158.9896538191669606 ) ) ;
#6289=CYLINDRICAL_SURFACE ( 'NONE', #80350, 4.749999999999976907 ) ;
#6290=CARTESIAN_POINT ( 'NONE',  ( 100.2615012876617726, -45.41023301258256595, 277.0594347997204636 ) ) ;
#6291=DIRECTION ( 'NONE',  ( -0.7071067811864634178, 0.7071067811866316166, -7.071067811864330499E-16 ) ) ;
#6292=AXIS2_PLACEMENT_3D ( 'NONE', #14676, #55969, #6952 ) ;
#6295=CARTESIAN_POINT ( 'NONE',  ( 103.0217603569634690, -26.37318327779222216, 20.37276813305394185 ) ) ;
#6296=CARTESIAN_POINT ( 'NONE',  ( 97.79849751320908524, -40.48507364506422590, 101.6332966594512754 ) ) ;
#6297=CARTESIAN_POINT ( 'NONE',  ( 108.5348814579965904, -26.43029805172858460, 100.9641967044829727 ) ) ;
#6298=CARTESIAN_POINT ( 'NONE',  ( 48.79742451362098166, -36.32844715994040996, -5.074374724088000832 ) ) ;
#6299=CARTESIAN_POINT ( 'NONE',  ( 102.9497400982657069, -26.42094052169726837, 175.3908633711489813 ) ) ;
#6301=VERTEX_POINT ( 'NONE', #8786 ) ;
#6302=LINE ( 'NONE', #80835, #13495 ) ;
#6303=CARTESIAN_POINT ( 'NONE',  ( 83.06670390244796920, -67.87844715994100397, 231.5838068554150198 ) ) ;
#6304=DIRECTION ( 'NONE',  ( 1.000000000000000078E-15, -1.000000000000000000, 0.000000000000000000 ) ) ;
#6305=ORIENTED_EDGE ( 'NONE', *, *, #50819, .T. ) ;
#6306=ADVANCED_FACE ( 'NONE', ( #35116 ), #69207, .T. ) ;
#6307=EDGE_CURVE ( 'NONE', #63968, #39230, #35592, .T. ) ;
#6308=CARTESIAN_POINT ( 'NONE',  ( 98.35048176673211628, -31.65547862740807616, 61.90667382029496935 ) ) ;
#6309=CARTESIAN_POINT ( 'NONE',  ( 109.5188487141873850, -46.90749067903785630, 132.7641967044819751 ) ) ;
#6311=CYLINDRICAL_SURFACE ( 'NONE', #45112, 4.750000000000004441 ) ;
#6313=CARTESIAN_POINT ( 'NONE',  ( 90.44969454456405344, -20.11243780205715481, 229.5838068554169809 ) ) ;
#6317=AXIS2_PLACEMENT_3D ( 'NONE', #6229, #12594, #18957 ) ;
#6318=EDGE_CURVE ( 'NONE', #86212, #51499, #17372, .T. ) ;
#6319=ORIENTED_EDGE ( 'NONE', *, *, #2845, .F. ) ;
#6321=EDGE_LOOP ( 'NONE', ( #5256, #65707, #58201, #18689 ) ) ;
#6322=FACE_OUTER_BOUND ( 'NONE', #62638, .T. ) ;
#6324=FACE_OUTER_BOUND ( 'NONE', #47432, .T. ) ;
#6327=CARTESIAN_POINT ( 'NONE',  ( 102.0669035284297479, -27.97058685607146700, 105.4898057718093156 ) ) ;
#6328=CARTESIAN_POINT ( 'NONE',  ( 116.3212776292296127, -32.94146857471318413, 287.6356252759109680 ) ) ;
#6330=ORIENTED_EDGE ( 'NONE', *, *, #3953, .T. ) ;
#6335=CARTESIAN_POINT ( 'NONE',  ( 98.19951187208815213, -40.85743130997446571, 252.6727681330533812 ) ) ;
#6338=CARTESIAN_POINT ( 'NONE',  ( 118.1148702536303290, -35.48641528967803538, 79.91562527591095488 ) ) ;
#6340=EDGE_CURVE ( 'NONE', #88945, #59559, #10994, .T. ) ;
#6342=CARTESIAN_POINT ( 'NONE',  ( 111.0271110396046765, -27.49575338583956352, 20.75426942819767362 ) ) ;
#6344=LINE ( 'NONE', #34032, #80630 ) ;
#6345=EDGE_CURVE ( 'NONE', #38746, #26493, #23513, .T. ) ;
#6346=ORIENTED_EDGE ( 'NONE', *, *, #29504, .T. ) ;
#6347=VERTEX_POINT ( 'NONE', #73214 ) ;
#6348=CARTESIAN_POINT ( 'NONE',  ( 34.27482367531500529, -30.08671355700301575, -5.074374724088000832 ) ) ;
#6349=CARTESIAN_POINT ( 'NONE',  ( 108.8902037297786762, -46.63625027785658972, 274.1530118773256390 ) ) ;
#6350=AXIS2_PLACEMENT_3D ( 'NONE', #37482, #65185, #65626 ) ;
#6351=DIRECTION ( 'NONE',  ( -0.9254794337955623007, -0.3787978585227819162, 0.000000000000000000 ) ) ;
#6352=CARTESIAN_POINT ( 'NONE',  ( 100.9544641706648065, -28.70718897609401665, 140.5939795459164543 ) ) ;
#6353=CARTESIAN_POINT ( 'NONE',  ( 97.07207206064353500, -35.37844118740781596, 81.21895860831540404 ) ) ;
#6356=DIRECTION ( 'NONE',  ( -0.9999999853157766072, -0.0001713722456143214551, 0.000000000000000000 ) ) ;
#6359=CARTESIAN_POINT ( 'NONE',  ( 117.4878618838608872, -37.01562663403593234, 43.80419670448293346 ) ) ;
#6361=CARTESIAN_POINT ( 'NONE',  ( 114.0298635175061008, -31.59016113260716097, 257.1385665600676589 ) ) ;
#6362=DIRECTION ( 'NONE',  ( 1.000000000000000000, 0.000000000000000000, 0.000000000000000000 ) ) ;
#6363=CARTESIAN_POINT ( 'NONE',  ( 98.64540312569886282, -41.76920806142285159, 161.7556252759109725 ) ) ;
#6365=CARTESIAN_POINT ( 'NONE',  ( 131.0667039024480118, -61.87844715994100397, 207.5838068554149913 ) ) ;
#6366=DIRECTION ( 'NONE',  ( -0.7071067811571960515, 0.7071067812158990940, 0.000000000000000000 ) ) ;
#6368=CARTESIAN_POINT ( 'NONE',  ( 96.22287284433019749, -34.36014117848482385, 252.1432443235303538 ) ) ;
#6371=VECTOR ( 'NONE', #84925, 1000.000000000000000 ) ;
#6372=EDGE_LOOP ( 'NONE', ( #67957, #41774, #73157, #58921, #62892 ) ) ;
#6373=CARTESIAN_POINT ( 'NONE',  ( 103.3469782872468130, -47.18711328981185460, 98.31657765686297523 ) ) ;
#6375=VECTOR ( 'NONE', #19609, 1000.000000000000000 ) ;
#6376=AXIS2_PLACEMENT_3D ( 'NONE', #40699, #82958, #27082 ) ;
#6377=ORIENTED_EDGE ( 'NONE', *, *, #69578, .F. ) ;
#6380=CIRCLE ( 'NONE', #2051, 4.874999999999990230 ) ;
#6381=CARTESIAN_POINT ( 'NONE',  ( 116.3214453605167478, -32.94026287388232532, 159.1356252759109680 ) ) ;
#6383=DIRECTION ( 'NONE',  ( 1.000000000000000078E-15, -1.000000000000000083E-30, -1.000000000000000000 ) ) ;
#6384=DIRECTION ( 'NONE',  ( -4.237773401492740281E-14, 1.000000000000000000, 0.000000000000000000 ) ) ;
#6385=CARTESIAN_POINT ( 'NONE',  ( 102.9190449779222405, -43.75998617602524376, 159.9709475124489586 ) ) ;
#6386=CARTESIAN_POINT ( 'NONE',  ( 100.1243021666677606, -44.53607127582347402, 262.9984824187678782 ) ) ;
#6387=CARTESIAN_POINT ( 'NONE',  ( 104.4069165777156059, -46.45774650464046829, 58.36469172372787284 ) ) ;
#6390=CARTESIAN_POINT ( 'NONE',  ( 138.8167039024479834, -67.87844715994100397, 60.91780685541480267 ) ) ;
#6391=ORIENTED_EDGE ( 'NONE', *, *, #54427, .F. ) ;
#6392=ORIENTED_EDGE ( 'NONE', *, *, #65080, .F. ) ;
#6393=LINE ( 'NONE', #81820, #60443 ) ;
#6394=EDGE_CURVE ( 'NONE', #32539, #79573, #52493, .T. ) ;
#6396=ORIENTED_EDGE ( 'NONE', *, *, #81332, .T. ) ;
#6398=CARTESIAN_POINT ( 'NONE',  ( 182.0667039024476139, -32.29483332967959086, 313.9678068554149490 ) ) ;
#6399=EDGE_CURVE ( 'NONE', #20410, #16018, #14820, .T. ) ;
#6400=LINE ( 'NONE', #34093, #11517 ) ;
#6402=CARTESIAN_POINT ( 'NONE',  ( 115.3626348109362425, -40.36077478062563983, 207.9086103042679667 ) ) ;
#6403=CARTESIAN_POINT ( 'NONE',  ( 95.29943635023701631, -34.95028898632038050, 71.20705384733993526 ) ) ;
#6404=CARTESIAN_POINT ( 'NONE',  ( 141.0664832912740394, -46.72944715994108122, -4.970821333495771377 ) ) ;
#6405=ORIENTED_EDGE ( 'NONE', *, *, #13290, .T. ) ;
#6406=ADVANCED_FACE ( 'NONE', ( #57353, #85094 ), #22863, .T. ) ;
#6409=ADVANCED_FACE ( 'NONE', ( #64626 ), #57807, .F. ) ;
#6412=VERTEX_POINT ( 'NONE', #44163 ) ;
#6413=CARTESIAN_POINT ( 'NONE',  ( 143.9834832912729894, -1.929447159941392931, 352.4506252759079530 ) ) ;
#6415=CARTESIAN_POINT ( 'NONE',  ( 112.4849986523878442, -45.14882631497925303, 133.0314946533368925 ) ) ;
#6416=ADVANCED_FACE ( 'NONE', ( #71902 ), #9660, .T. ) ;
#6418=FACE_BOUND ( 'NONE', #41890, .T. ) ;
#6420=CARTESIAN_POINT ( 'NONE',  ( 115.6914824993820901, -43.67961476919119690, 43.27467289495795200 ) ) ;
#6421=VECTOR ( 'NONE', #10000, 1000.000000000000000 ) ;
#6422=EDGE_CURVE ( 'NONE', #25932, #4530, #65075, .T. ) ;
#6424=PLANE ( 'NONE',  #52955 ) ;
#6426=CARTESIAN_POINT ( 'NONE',  ( 131.6688901780889296, -17.37024878623243751, 2.654395752964755051 ) ) ;
#6430=PLANE ( 'NONE',  #48709 ) ;
#6432=ORIENTED_EDGE ( 'NONE', *, *, #60162, .F. ) ;
#6433=CARTESIAN_POINT ( 'NONE',  ( 108.9892323659770170, -46.99785963944585632, 78.72419670448194040 ) ) ;
#6436=CARTESIAN_POINT ( 'NONE',  ( 193.0371591254583734, -47.82818131005411999, 313.9678068554149490 ) ) ;
#6438=VECTOR ( 'NONE', #47304, 1000.000000000000000 ) ;
#6443=CARTESIAN_POINT ( 'NONE',  ( 98.20106483660288177, -31.34956418181673854, 121.8803871806729546 ) ) ;
#6444=CARTESIAN_POINT ( 'NONE',  ( 97.80792351950141494, -40.51905676813210988, 116.6359120812046939 ) ) ;
#6446=AXIS2_PLACEMENT_3D ( 'NONE', #51966, #17478, #52400 ) ;
#6447=CARTESIAN_POINT ( 'NONE',  ( 116.1995025514323316, -41.78438384397597360, 259.4241967044825969 ) ) ;
#6448=CARTESIAN_POINT ( 'NONE',  ( 97.86619352455458909, -40.64832413407319933, 252.6469055415188620 ) ) ;
#6451=CARTESIAN_POINT ( 'NONE',  ( 87.31648329127401098, -46.47944715994105280, 14.92562527591095112 ) ) ;
#6455=EDGE_CURVE ( 'NONE', #3936, #783, #48170, .T. ) ;
#6456=CARTESIAN_POINT ( 'NONE',  ( 118.1473594538626486, -37.63838399483783093, 188.7613395616259595 ) ) ;
#6458=ORIENTED_EDGE ( 'NONE', *, *, #37422, .F. ) ;
#6459=CARTESIAN_POINT ( 'NONE',  ( 113.0289363901617889, -43.32575541760495241, 129.5930118773259778 ) ) ;
#6460=LINE ( 'NONE', #46868, #60231 ) ;
#6461=CARTESIAN_POINT ( 'NONE',  ( 115.3146942856800337, -32.23016485065021897, 20.64348806780197521 ) ) ;
#6462=LINE ( 'NONE', #13283, #5679 ) ;
#6463=DIRECTION ( 'NONE',  ( 0.000000000000000000, 0.000000000000000000, -1.000000000000000000 ) ) ;
#6467=DIRECTION ( 'NONE',  ( 0.000000000000000000, 0.000000000000000000, -1.000000000000000000 ) ) ;
#6468=CARTESIAN_POINT ( 'NONE',  ( 96.16101635903902434, -35.07578045570937775, 221.1946728949589840 ) ) ;
#6469=LINE ( 'NONE', #61422, #27205 ) ;
#6470=ORIENTED_EDGE ( 'NONE', *, *, #70535, .T. ) ;
#6471=ORIENTED_EDGE ( 'NONE', *, *, #60434, .F. ) ;
#6473=CARTESIAN_POINT ( 'NONE',  ( 82.31791107858144585, -20.31136518418547965, 7.339178645752261865 ) ) ;
#6474=CARTESIAN_POINT ( 'NONE',  ( 116.3216177720312317, -32.94249360885015676, 184.1356252759109680 ) ) ;
#6475=CARTESIAN_POINT ( 'NONE',  ( 172.5664832912740110, -18.82844715994099971, 81.04262527591200183 ) ) ;
#6477=CARTESIAN_POINT ( 'NONE',  ( 194.5667039024480403, -40.82844715993405771, 249.9678068554149775 ) ) ;
#6481=CARTESIAN_POINT ( 'NONE',  ( 113.2201423986613520, -45.14488000985961946, 228.0784824187679760 ) ) ;
#6482=VERTEX_POINT ( 'NONE', #5545 ) ;
#6484=DIRECTION ( 'NONE',  ( 1.000000000000000000, 3.999999999999999995E-14, 1.000000000000000078E-15 ) ) ;
#6486=CARTESIAN_POINT ( 'NONE',  ( 112.1086029179114547, -30.31019831854434443, 77.36523322673394887 ) ) ;
#6487=CARTESIAN_POINT ( 'NONE',  ( 101.9613826146451885, -46.55915482862852173, 163.1832443235299763 ) ) ;
#6488=CARTESIAN_POINT ( 'NONE',  ( 105.8444747722200674, -25.33565403619829226, 322.4846826458744431 ) ) ;
#6492=CARTESIAN_POINT ( 'NONE',  ( 99.42197401388541778, -43.20727476509772202, 66.88677594099895884 ) ) ;
#6493=VERTEX_POINT ( 'NONE', #45937 ) ;
#6494=ORIENTED_EDGE ( 'NONE', *, *, #9824, .T. ) ;
#6495=AXIS2_PLACEMENT_3D ( 'NONE', #68455, #47983, #67550 ) ;
#6496=CIRCLE ( 'NONE', #2169, 13.49999999999999822 ) ;
#6498=AXIS2_PLACEMENT_3D ( 'NONE', #7238, #40403, #54900 ) ;
#6502=CIRCLE ( 'NONE', #10905, 4.749999999999976907 ) ;
#6503=EDGE_CURVE ( 'NONE', #23851, #2670, #11453, .T. ) ;
#6504=EDGE_CURVE ( 'NONE', #40777, #74550, #22090, .T. ) ;
#6505=CARTESIAN_POINT ( 'NONE',  ( 102.6785256587874926, -29.36752282311925200, 84.92670554236298130 ) ) ;
#6506=CARTESIAN_POINT ( 'NONE',  ( 96.66004714996478242, -35.80616453621266970, 231.2556252759109725 ) ) ;
#6507=ADVANCED_FACE ( 'NONE', ( #75476 ), #88220, .T. ) ;
#6508=CARTESIAN_POINT ( 'NONE',  ( 113.7366723824214887, -44.71300795807898965, 193.1299109901969757 ) ) ;
#6509=DIRECTION ( 'NONE',  ( -1.000000000000000000, 0.000000000000000000, 0.000000000000000000 ) ) ;
#6510=CARTESIAN_POINT ( 'NONE',  ( 111.3142535964730371, -27.23286288913599051, 20.74133956162494030 ) ) ;
#6513=EDGE_CURVE ( 'NONE', #89449, #64543, #37532, .T. ) ;
#6514=EDGE_LOOP ( 'NONE', ( #45341, #3807, #52181, #75038 ) ) ;
#6515=ORIENTED_EDGE ( 'NONE', *, *, #54234, .T. ) ;
#6516=EDGE_CURVE ( 'NONE', #55655, #87716, #5082, .T. ) ;
#6517=CARTESIAN_POINT ( 'NONE',  ( 118.1148702536304427, -35.48641528967804248, 83.91562527591095488 ) ) ;
#6518=CARTESIAN_POINT ( 'NONE',  ( 102.9537058647788967, -46.35710148923402585, 92.25562527591097250 ) ) ;
#6519=CARTESIAN_POINT ( 'NONE',  ( 110.8326918741827711, -26.28777313046090569, 249.7889586092445882 ) ) ;
#6521=CARTESIAN_POINT ( 'NONE',  ( 107.5100371804366688, -47.14531440222233272, 237.6099109901969655 ) ) ;
#6522=CARTESIAN_POINT ( 'NONE',  ( 99.09570902266669634, -30.55043182097106680, 35.80229194939514059 ) ) ;
#6524=DIRECTION ( 'NONE',  ( 1.000000000000000078E-15, -1.000000000000000083E-30, -1.000000000000000000 ) ) ;
#6525=CARTESIAN_POINT ( 'NONE',  ( 117.0407245441959816, -35.29532848343978202, 29.94117331857431807 ) ) ;
#6527=CARTESIAN_POINT ( 'NONE',  ( 112.6803783697433516, -30.99839248778516776, 277.6356252759110248 ) ) ;
#6528=DIRECTION ( 'NONE',  ( 0.000000000000000000, 0.000000000000000000, 1.000000000000000000 ) ) ;
#6529=CARTESIAN_POINT ( 'NONE',  ( 117.0719014705369716, -35.46251353140062434, 174.9272894658773509 ) ) ;
#6530=LINE ( 'NONE', #61036, #10569 ) ;
#6533=CARTESIAN_POINT ( 'NONE',  ( 151.5667039024483245, -48.82844715993591223, 300.4678068554149490 ) ) ;
#6534=CARTESIAN_POINT ( 'NONE',  ( 116.3121618740066623, -32.93870344941997530, 39.13562527591096796 ) ) ;
#6535=CARTESIAN_POINT ( 'NONE',  ( 51.03742451361635091, -23.42844715994068849, 117.4678068554150485 ) ) ;
#6536=EDGE_CURVE ( 'NONE', #3590, #7607, #59773, .T. ) ;
#6539=DIRECTION ( 'NONE',  ( 1.000000000000000000, -4.163336342344333240E-14, 0.000000000000000000 ) ) ;
#6540=CARTESIAN_POINT ( 'NONE',  ( 117.2187229798756363, -34.26400738748503727, 209.0156252759109634 ) ) ;
#6541=CARTESIAN_POINT ( 'NONE',  ( 95.77906782739819391, -40.33899944578667629, 127.5727681330539554 ) ) ;
#6542=CARTESIAN_POINT ( 'NONE',  ( 105.0131270392176646, -25.82159629633810738, 276.2365776568634033 ) ) ;
#6543=CARTESIAN_POINT ( 'NONE',  ( 97.81171236172070849, -40.51746256574213589, 261.6350867226296941 ) ) ;
#6544=CARTESIAN_POINT ( 'NONE',  ( 116.3212776292296127, -32.94146857471318413, 287.6356252759109680 ) ) ;
#6545=CARTESIAN_POINT ( 'NONE',  ( 83.06670390244796920, -58.72944715994093912, 207.5838068554149913 ) ) ;
#6547=VECTOR ( 'NONE', #22499, 1000.000000000000000 ) ;
#6548=CARTESIAN_POINT ( 'NONE',  ( 72.25757238336808541, -1.944390235229867425, 361.9756252759101471 ) ) ;
#6550=EDGE_LOOP ( 'NONE', ( #12801, #8970, #77761, #49075 ) ) ;
#6553=CARTESIAN_POINT ( 'NONE',  ( 112.9437820074331569, -43.62348782359368471, 152.5733722090289746 ) ) ;
#6555=VERTEX_POINT ( 'NONE', #61379 ) ;
#6557=CARTESIAN_POINT ( 'NONE',  ( 99.11802762103509679, -45.48540990049882282, 152.9899109901969894 ) ) ;
#6558=CARTESIAN_POINT ( 'NONE',  ( 104.4066719782816790, -46.45767031374273870, 148.3653026159171588 ) ) ;
#6561=LINE ( 'NONE', #76048, #86108 ) ;
#6562=EDGE_CURVE ( 'NONE', #27190, #49111, #31884, .T. ) ;
#6563=CARTESIAN_POINT ( 'NONE',  ( 116.7176835877704946, -38.50936494796418685, 88.68133956162593279 ) ) ;
#6565=ORIENTED_EDGE ( 'NONE', *, *, #41456, .F. ) ;
#6566=VERTEX_POINT ( 'NONE', #25521 ) ;
#6567=CIRCLE ( 'NONE', #76198, 2.517499999999998739 ) ;
#6570=CARTESIAN_POINT ( 'NONE',  ( 97.31342953368671544, -35.99458159538090030, 142.2670538473389570 ) ) ;
#6572=VECTOR ( 'NONE', #68618, 1000.000000000000000 ) ;
#6575=AXIS2_PLACEMENT_3D ( 'NONE', #39383, #17608, #59808 ) ;
#6576=FACE_OUTER_BOUND ( 'NONE', #74868, .T. ) ;
#6577=CARTESIAN_POINT ( 'NONE',  ( 194.5664832912739826, 0.2215528400590013880, -5.074374724088000832 ) ) ;
#6578=DIRECTION ( 'NONE',  ( -4.237773401492740281E-14, 1.000000000000000000, 0.000000000000000000 ) ) ;
#6579=CARTESIAN_POINT ( 'NONE',  ( 98.16825066461156268, -43.24752039522714142, 106.8175300378159704 ) ) ;
#6582=ORIENTED_EDGE ( 'NONE', *, *, #67116, .F. ) ;
#6584=EDGE_CURVE ( 'NONE', #7678, #6003, #53191, .T. ) ;
#6586=DIRECTION ( 'NONE',  ( 0.000000000000000000, 0.000000000000000000, 1.000000000000000000 ) ) ;
#6587=DIRECTION ( 'NONE',  ( 4.299999999999999979E-14, -1.000000000000000000, 4.400000000000000367E-29 ) ) ;
#6589=CARTESIAN_POINT ( 'NONE',  ( 100.2649065926023297, -31.37786052998579223, 198.6261856076869776 ) ) ;
#6590=EDGE_CURVE ( 'NONE', #87925, #55605, #83194, .T. ) ;
#6591=CIRCLE ( 'NONE', #5099, 2.116999999999980009 ) ;
#6593=EDGE_LOOP ( 'NONE', ( #52539, #85685, #2712 ) ) ;
#6594=EDGE_LOOP ( 'NONE', ( #20081, #79463, #81931, #87329, #17183 ) ) ;
#6595=ORIENTED_EDGE ( 'NONE', *, *, #78349, .F. ) ;
#6596=DIRECTION ( 'NONE',  ( 1.000000000000000078E-15, -1.000000000000000083E-30, -1.000000000000000000 ) ) ;
#6598=ORIENTED_EDGE ( 'NONE', *, *, #1368, .T. ) ;
#6599=EDGE_LOOP ( 'NONE', ( #29196, #73199 ) ) ;
#6601=CARTESIAN_POINT ( 'NONE',  ( 115.4123442176498173, -41.04489973583525142, 239.8663452106589773 ) ) ;
#6603=PLANE ( 'NONE',  #69679 ) ;
#6604=VECTOR ( 'NONE', #10866, 1000.000000000000000 ) ;
#6607=VERTEX_POINT ( 'NONE', #505 ) ;
#6608=PLANE ( 'NONE',  #72525 ) ;
#6609=AXIS2_PLACEMENT_3D ( 'NONE', #50543, #35571, #56456 ) ;
#6614=CARTESIAN_POINT ( 'NONE',  ( 109.5637425988213636, -28.92903792723274847, 232.6480903695909603 ) ) ;
#6615=CARTESIAN_POINT ( 'NONE',  ( 95.75500511041516916, -40.34669435480882527, 131.5727681330539554 ) ) ;
#6616=EDGE_CURVE ( 'NONE', #54796, #20434, #35014, .T. ) ;
#6617=CARTESIAN_POINT ( 'NONE',  ( 116.5135284680788175, -32.37261310794432490, 104.1699109901969535 ) ) ;
#6618=CARTESIAN_POINT ( 'NONE',  ( 101.9411125306454124, -42.93772781322726217, 249.5838068554172366 ) ) ;
#6619=CARTESIAN_POINT ( 'NONE',  ( 133.3217830637516101, -16.08035908359601152, 8.141856907853265213 ) ) ;
#6620=CARTESIAN_POINT ( 'NONE',  ( 107.6544996609965352, -47.76702919738148267, 193.6308633711489620 ) ) ;
#6621=CARTESIAN_POINT ( 'NONE',  ( 46.48091746482130304, -49.32844715994084339, 300.4678068554150059 ) ) ;
#6624=ORIENTED_EDGE ( 'NONE', *, *, #76370, .F. ) ;
#6626=ORIENTED_EDGE ( 'NONE', *, *, #45969, .T. ) ;
#6627=CYLINDRICAL_SURFACE ( 'NONE', #11176, 9.999999999999998224 ) ;
#6628=VERTEX_POINT ( 'NONE', #20952 ) ;
#6631=CARTESIAN_POINT ( 'NONE',  ( 95.67500926166044906, -33.46221576448694890, 141.1041967044829732 ) ) ;
#6635=LINE ( 'NONE', #61582, #51356 ) ;
#6636=CARTESIAN_POINT ( 'NONE',  ( 51.24204729617191845, -31.76306994223763880, 193.9678068554150911 ) ) ;
#6638=CARTESIAN_POINT ( 'NONE',  ( 95.31970492887387536, -38.09378048407035777, 232.4184824187679794 ) ) ;
#6639=CARTESIAN_POINT ( 'NONE',  ( 107.0664832912739541, -20.87944715994095546, 302.7856252759109452 ) ) ;
#6640=CARTESIAN_POINT ( 'NONE',  ( 107.0664832912739399, -36.72944715994096754, 296.0306255462182321 ) ) ;
#6641=EDGE_CURVE ( 'NONE', #88962, #75252, #59, .T. ) ;
#6642=ORIENTED_EDGE ( 'NONE', *, *, #79967, .T. ) ;
#6643=DIRECTION ( 'NONE',  ( 1.000000000000000000, 0.000000000000000000, 0.000000000000000000 ) ) ;
#6646=VECTOR ( 'NONE', #89694, 1000.000000000000000 ) ;
#6647=CARTESIAN_POINT ( 'NONE',  ( 194.0371591254582881, -46.82818131005407736, 237.4678068554150059 ) ) ;
#6648=CARTESIAN_POINT ( 'NONE',  ( 112.6874404347162084, -45.56185944854193792, 263.0270538473394026 ) ) ;
#6649=ORIENTED_EDGE ( 'NONE', *, *, #66403, .T. ) ;
#6650=CARTESIAN_POINT ( 'NONE',  ( 105.9948944823395891, -26.75816435948428307, 195.1613249903887493 ) ) ;
#6651=CARTESIAN_POINT ( 'NONE',  ( 96.58491273044850800, -36.88769195468244533, 136.3384824187679385 ) ) ;
#6652=CARTESIAN_POINT ( 'NONE',  ( 115.4446095375818970, -42.99269977972175383, 24.31562527591096767 ) ) ;
#6653=CARTESIAN_POINT ( 'NONE',  ( 113.5922599384962552, -44.96062289245586641, 164.1099109901969655 ) ) ;
#6655=CARTESIAN_POINT ( 'NONE',  ( 36.65249034007446483, -48.32844715994130524, 129.9678068554150911 ) ) ;
#6656=AXIS2_PLACEMENT_3D ( 'NONE', #73585, #5900, #45412 ) ;
#6658=CARTESIAN_POINT ( 'NONE',  ( 25.56670390244797275, -62.87844715994099687, 252.3428068554150059 ) ) ;
#6659=DIRECTION ( 'NONE',  ( 0.7071067811866279529, -0.7071067811864671926, 7.071067811866286874E-16 ) ) ;
#6661=EDGE_LOOP ( 'NONE', ( #50660, #37749, #10474, #55160 ) ) ;
#6665=ORIENTED_EDGE ( 'NONE', *, *, #9732, .F. ) ;
#6666=CARTESIAN_POINT ( 'NONE',  ( 49.35031423293201414, -29.99615139349890569, -5.074374724088000832 ) ) ;
#6667=CARTESIAN_POINT ( 'NONE',  ( 106.8416606513710008, -48.55305329746386178, 73.56133956162497611 ) ) ;
#6668=CARTESIAN_POINT ( 'NONE',  ( 156.5667039024480971, -42.82844715993568485, 293.2178068554149490 ) ) ;
#6669=DIRECTION ( 'NONE',  ( 0.000000000000000000, -1.000000000000000000, 0.000000000000000000 ) ) ;
#6670=CARTESIAN_POINT ( 'NONE',  ( 107.5678551521628492, -47.81755451042874228, 188.6003871806729535 ) ) ;
#6672=EDGE_CURVE ( 'NONE', #70541, #52915, #56349, .T. ) ;
#6673=CARTESIAN_POINT ( 'NONE',  ( 112.1081655520365388, -43.62419673505787898, 227.5009912566479784 ) ) ;
#6674=EDGE_LOOP ( 'NONE', ( #84794, #57553, #83720, #34810 ) ) ;
#6678=CARTESIAN_POINT ( 'NONE',  ( 116.3435622888236196, -40.58882322890893590, 183.5124998200998334 ) ) ;
#6680=CARTESIAN_POINT ( 'NONE',  ( 98.34985890712087553, -31.65658481866827501, 75.90645861007901374 ) ) ;
#6681=CARTESIAN_POINT ( 'NONE',  ( 97.31592806723180900, -39.30618353892431571, 276.5310398549307251 ) ) ;
#6682=CARTESIAN_POINT ( 'NONE',  ( 177.8371591254545478, -47.82818131005477369, 129.9678068554150059 ) ) ;
#6684=CARTESIAN_POINT ( 'NONE',  ( 97.07201651732883363, -35.37898364459096001, 176.2190017941805422 ) ) ;
#6685=CARTESIAN_POINT ( 'NONE',  ( 115.1244435679684699, -31.12738977229718884, 279.3099109901971815 ) ) ;
#6687=ORIENTED_EDGE ( 'NONE', *, *, #41444, .F. ) ;
#6690=CARTESIAN_POINT ( 'NONE',  ( 99.39318122740648676, -32.72677799018995870, 88.74999513149600716 ) ) ;
#6692=EDGE_CURVE ( 'NONE', #86269, #87632, #55442, .T. ) ;
#6693=VECTOR ( 'NONE', #23245, 1000.000000000000000 ) ;
#6694=AXIS2_PLACEMENT_3D ( 'NONE', #30490, #23689, #51353 ) ;
#6696=DIRECTION ( 'NONE',  ( -0.9254794337955620787, -0.3787978585227822492, 0.000000000000000000 ) ) ;
#6697=DIRECTION ( 'NONE',  ( -1.000000000000000078E-15, 1.000000000000000000, 0.000000000000000000 ) ) ;
#6700=ORIENTED_EDGE ( 'NONE', *, *, #46702, .T. ) ;
#6701=CARTESIAN_POINT ( 'NONE',  ( 108.7432494476977922, -25.80391683235395917, 144.9432443235299672 ) ) ;
#6704=CARTESIAN_POINT ( 'NONE',  ( 99.03419491772403660, -31.85514013008181777, 122.3120594963729673 ) ) ;
#6707=AXIS2_PLACEMENT_3D ( 'NONE', #88018, #40743, #48434 ) ;
#6708=CARTESIAN_POINT ( 'NONE',  ( 118.0115981831179113, -38.42934884787886318, 64.69181575210097890 ) ) ;
#6709=CARTESIAN_POINT ( 'NONE',  ( 116.3212776292296127, -32.94146857471318413, 287.6356252759109680 ) ) ;
#6713=VERTEX_POINT ( 'NONE', #84091 ) ;
#6714=AXIS2_PLACEMENT_3D ( 'NONE', #45189, #10678, #34253 ) ;
#6715=ORIENTED_EDGE ( 'NONE', *, *, #74936, .F. ) ;
#6716=EDGE_CURVE ( 'NONE', #50271, #41960, #65521, .T. ) ;
#6719=EDGE_CURVE ( 'NONE', #88931, #55655, #49080, .T. ) ;
#6720=CARTESIAN_POINT ( 'NONE',  ( 115.1619974903381518, -42.21817061296157192, 273.3527681330542691 ) ) ;
#6721=CARTESIAN_POINT ( 'NONE',  ( 103.4608836344597194, -46.53438966646587005, 138.2956252759109645 ) ) ;
#6722=CARTESIAN_POINT ( 'NONE',  ( 107.0664832912739541, -23.22944715994095333, 311.6356252759109680 ) ) ;
#6723=CARTESIAN_POINT ( 'NONE',  ( 112.0638110394401679, -45.48956745532829871, 128.9896019377486027 ) ) ;
#6724=ADVANCED_FACE ( 'NONE', ( #7773 ), #54985, .F. ) ;
#6725=CARTESIAN_POINT ( 'NONE',  ( 102.9710815734590454, -46.31642646611675218, 88.25562527591095829 ) ) ;
#6731=AXIS2_PLACEMENT_3D ( 'NONE', #56747, #49922, #41316 ) ;
#6732=EDGE_LOOP ( 'NONE', ( #4607, #6799, #66363, #66183 ) ) ;
#6733=DIRECTION ( 'NONE',  ( -1.000000000000000078E-15, 0.000000000000000000, 1.000000000000000000 ) ) ;
#6734=CARTESIAN_POINT ( 'NONE',  ( 133.5842039024481096, -58.72944715994091780, 207.5838068554170377 ) ) ;
#6735=CARTESIAN_POINT ( 'NONE',  ( 108.0121126588926046, -24.94157235513505100, 265.0127681330535552 ) ) ;
#6736=LINE ( 'NONE', #81720, #17027 ) ;
#6739=CARTESIAN_POINT ( 'NONE',  ( 109.4546162266718454, -25.87086512622375878, 29.90419670448296685 ) ) ;
#6740=CARTESIAN_POINT ( 'NONE',  ( 97.19020072829189871, -38.39417980001610431, 101.4598920277657186 ) ) ;
#6741=CARTESIAN_POINT ( 'NONE',  ( 108.3168256696638281, -47.05733704442508980, 113.6727681330539639 ) ) ;
#6743=CARTESIAN_POINT ( 'NONE',  ( 107.9218747862861250, -47.19940893231376577, 177.6413395616249886 ) ) ;
#6745=EDGE_CURVE ( 'NONE', #48789, #57151, #42713, .T. ) ;
#6747=LINE ( 'NONE', #34894, #46849 ) ;
#6748=FACE_BOUND ( 'NONE', #68398, .T. ) ;
#6751=ORIENTED_EDGE ( 'NONE', *, *, #40651, .T. ) ;
#6753=CARTESIAN_POINT ( 'NONE',  ( 117.2811830599562057, -39.02712847638015603, 148.6499109901969859 ) ) ;
#6756=CARTESIAN_POINT ( 'NONE',  ( 97.03730526165486481, -41.43059529571826261, 207.6632443235299661 ) ) ;
#6757=VECTOR ( 'NONE', #78361, 1000.000000000000000 ) ;
#6760=CARTESIAN_POINT ( 'NONE',  ( 116.3114837287122754, -32.94280867712679850, 274.1356252759109680 ) ) ;
#6761=ORIENTED_EDGE ( 'NONE', *, *, #44679, .T. ) ;
#6762=AXIS2_PLACEMENT_3D ( 'NONE', #75247, #82970, #40708 ) ;
#6763=VECTOR ( 'NONE', #27033, 1000.000000000000000 ) ;
#6766=ORIENTED_EDGE ( 'NONE', *, *, #54500, .T. ) ;
#6767=VERTEX_POINT ( 'NONE', #49981 ) ;
#6768=DIRECTION ( 'NONE',  ( 1.000000000000000078E-15, -1.000000000000000000, 0.000000000000000000 ) ) ;
#6769=CARTESIAN_POINT ( 'NONE',  ( 97.91927484100293100, -41.73055353899491138, 217.7241967044829494 ) ) ;
#6770=CARTESIAN_POINT ( 'NONE',  ( 29.77381068363482441, -48.62134037875501491, 249.9678068554150059 ) ) ;
#6771=CARTESIAN_POINT ( 'NONE',  ( 136.5970450997423313, -17.65293374834612194, 2.807537076566525513 ) ) ;
#6774=DIRECTION ( 'NONE',  ( -8.673617379884035472E-16, -1.000000000000000000, 0.000000000000000000 ) ) ;
#6775=AXIS2_PLACEMENT_3D ( 'NONE', #50056, #56423, #43697 ) ;
#6777=EDGE_LOOP ( 'NONE', ( #35142, #56537, #570, #38893 ) ) ;
#6779=CARTESIAN_POINT ( 'NONE',  ( 194.0371591254584587, -46.82818131005407736, 180.4678068554150343 ) ) ;
#6780=CARTESIAN_POINT ( 'NONE',  ( 177.4809174648213741, -48.32844715993478957, 249.9678068554149775 ) ) ;
#6781=EDGE_CURVE ( 'NONE', #69697, #57874, #27780, .T. ) ;
#6782=CARTESIAN_POINT ( 'NONE',  ( 101.9853755998761500, -45.08682593082387058, 243.1413395616249886 ) ) ;
#6783=CARTESIAN_POINT ( 'NONE',  ( 172.5664832912729878, -27.57844715994070484, 78.92562527591199739 ) ) ;
#6784=CARTESIAN_POINT ( 'NONE',  ( 116.9446180447426826, -41.83184233209001235, 89.44705384733897802 ) ) ;
#6786=CARTESIAN_POINT ( 'NONE',  ( 102.0661958919803425, -27.97100149082080378, 21.48984596613240683 ) ) ;
#6788=DIRECTION ( 'NONE',  ( 0.000000000000000000, 1.000000000000000000, 0.000000000000000000 ) ) ;
#6789=EDGE_LOOP ( 'NONE', ( #2741, #76107 ) ) ;
#6790=ORIENTED_EDGE ( 'NONE', *, *, #14089, .F. ) ;
#6791=CARTESIAN_POINT ( 'NONE',  ( 48.16670390244701139, -28.27351298637280408, -5.074374724088000832 ) ) ;
#6792=CARTESIAN_POINT ( 'NONE',  ( 98.98570259493575918, -42.74373749968300729, 258.2672975916112819 ) ) ;
#6796=CARTESIAN_POINT ( 'NONE',  ( 108.4170684944699019, -26.73498250654907693, 139.9689921095843772 ) ) ;
#6797=DIRECTION ( 'NONE',  ( 0.000000000000000000, 0.000000000000000000, -1.000000000000000000 ) ) ;
#6798=DIRECTION ( 'NONE',  ( -0.7071067811865784369, 0.7071067811865165975, -7.071067811865791864E-16 ) ) ;
#6799=ORIENTED_EDGE ( 'NONE', *, *, #35830, .F. ) ;
#6801=CARTESIAN_POINT ( 'NONE',  ( 98.30747440715256857, -41.72872907108401108, 182.7402955621933813 ) ) ;
#6803=CARTESIAN_POINT ( 'NONE',  ( 103.4771249150381749, -25.43533399052049049, 55.32133956162594046 ) ) ;
#6805=CARTESIAN_POINT ( 'NONE',  ( 111.2703484347609333, -28.70728902343469002, 14.10289601855296837 ) ) ;
#6807=CARTESIAN_POINT ( 'NONE',  ( 112.0672218174811974, -45.48765836883565328, 127.9900062656194564 ) ) ;
#6808=CARTESIAN_POINT ( 'NONE',  ( 98.40655050692420502, -32.18313002855524729, 135.9413395616259947 ) ) ;
#6812=FACE_OUTER_BOUND ( 'NONE', #46378, .T. ) ;
#6815=CARTESIAN_POINT ( 'NONE',  ( 113.8273992703627044, -26.93653503804465288, 235.5956252759109759 ) ) ;
#6818=CIRCLE ( 'NONE', #18418, 2.030000000001872529 ) ;
#6819=VERTEX_POINT ( 'NONE', #38157 ) ;
#6820=CARTESIAN_POINT ( 'NONE',  ( 109.0806625061526205, -47.64460086702110431, 123.7337205140059666 ) ) ;
#6821=AXIS2_PLACEMENT_3D ( 'NONE', #87697, #18653, #45881 ) ;
#6828=CARTESIAN_POINT ( 'NONE',  ( 32.09598329127609873, -23.42844715994129956, 193.9678068554150911 ) ) ;
#6829=CARTESIAN_POINT ( 'NONE',  ( 25.56670390244722313, -42.82844715994178131, 137.2178068554150627 ) ) ;
#6830=FACE_OUTER_BOUND ( 'NONE', #78515, .T. ) ;
#6832=ADVANCED_FACE ( 'NONE', ( #50436 ), #37725, .T. ) ;
#6833=CARTESIAN_POINT ( 'NONE',  ( 100.4889591185686015, -31.84898980388015843, 178.6366617981629474 ) ) ;
#6834=CARTESIAN_POINT ( 'NONE',  ( 105.6290766085263044, -47.07696477925017575, 253.4670538473393719 ) ) ;
#6835=CARTESIAN_POINT ( 'NONE',  ( 97.81170508561586985, -40.51744524251693491, 57.63550115181184452 ) ) ;
#6836=ORIENTED_EDGE ( 'NONE', *, *, #53919, .F. ) ;
#6838=VECTOR ( 'NONE', #82006, 1000.000000000000000 ) ;
#6843=AXIS2_PLACEMENT_3D ( 'NONE', #81615, #19364, #12550 ) ;
#6844=CARTESIAN_POINT ( 'NONE',  ( 46.48091746482045750, -49.32844715994088602, 180.4678068554150911 ) ) ;
#6847=CARTESIAN_POINT ( 'NONE',  ( 97.53184222742581255, -39.74894927286113955, 16.57053032456689934 ) ) ;
#6848=CARTESIAN_POINT ( 'NONE',  ( 33.91903122894598965, -35.91149509761181235, -5.074374724088000832 ) ) ;
#6849=CARTESIAN_POINT ( 'NONE',  ( 62.56670390244828184, -48.82844715994019680, 300.4678068554150627 ) ) ;
#6850=CARTESIAN_POINT ( 'NONE',  ( 98.03781028509631312, -36.02536330594374192, 190.6990864947429998 ) ) ;
#6851=CARTESIAN_POINT ( 'NONE',  ( 96.87811797401508329, -32.32375813437732859, 61.01372051400599616 ) ) ;
#6852=CARTESIAN_POINT ( 'NONE',  ( 50.56670390244699576, -18.82844715994031048, -5.074374724088000832 ) ) ;
#6855=EDGE_CURVE ( 'NONE', #14017, #70942, #24872, .T. ) ;
#6856=DIRECTION ( 'NONE',  ( 0.7071067811873696929, 0.7071067811857253416, 7.071067811873690333E-16 ) ) ;
#6857=ORIENTED_EDGE ( 'NONE', *, *, #28591, .T. ) ;
#6858=LINE ( 'NONE', #62264, #22943 ) ;
#6859=ORIENTED_EDGE ( 'NONE', *, *, #84996, .F. ) ;
#6860=B_SPLINE_CURVE_WITH_KNOTS ( 'NONE', 3,
 ( #5014, #26790, #32713, #74502, #60407, #46770, #12280, #66786, #32259, #87247, #39972, #54022, #59954, #25454, #87687, #31816, #47224, #54473, #74951, #59512, #82237, #19991, #75406, #13180, #40863, #25012, #52676, #80435, #61748, #70378 ),
 .UNSPECIFIED., .F., .F.,
 ( 4, 2, 2, 2, 1, 2, 2, 2, 2, 2, 2, 2, 1, 2, 2, 4 ),
 ( 0.5000000000000000000, 0.5625000000000165423, 0.5937500000000232037, 0.6093750000000266454, 0.6171875000000283107, 0.6210937500000291989, 0.6250000000000299760, 0.6875000000000308642, 0.7187500000000315303, 0.7500000000000321965, 0.8125000000000320854, 0.8437500000000304201, 0.8593750000000295319, 0.8671875000000290878, 0.8750000000000286438, 1.000000000000000000 ),
 .UNSPECIFIED. ) ;
#6862=CARTESIAN_POINT ( 'NONE',  ( 168.0371591254543944, -48.62818131005519717, 249.9678068554149775 ) ) ;
#6867=CARTESIAN_POINT ( 'NONE',  ( 103.9507802182147600, -47.35902078718802954, 62.33753003781600199 ) ) ;
#6870=CARTESIAN_POINT ( 'NONE',  ( 107.0664832912739399, -36.72944715994096754, 296.0306255462182321 ) ) ;
#6872=ORIENTED_EDGE ( 'NONE', *, *, #15858, .T. ) ;
#6873=CARTESIAN_POINT ( 'NONE',  ( 100.2031981095150854, -29.33968530819532461, 121.6706578896535405 ) ) ;
#6875=CARTESIAN_POINT ( 'NONE',  ( 52.65249034007751305, -49.32844715994061602, 129.9678068554150911 ) ) ;
#6876=ORIENTED_EDGE ( 'NONE', *, *, #56333, .T. ) ;
#6877=CARTESIAN_POINT ( 'NONE',  ( 98.57234554589554421, -43.83823254894062416, 67.86895860924497015 ) ) ;
#6878=AXIS2_PLACEMENT_3D ( 'NONE', #9641, #71438, #63714 ) ;
#6879=LINE ( 'NONE', #20527, #43625 ) ;
#6880=DIRECTION ( 'NONE',  ( 1.000000000000000000, 8.843517682682131024E-16, 1.000000000000000078E-15 ) ) ;
#6882=AXIS2_PLACEMENT_3D ( 'NONE', #23760, #51428, #38698 ) ;
#6887=CARTESIAN_POINT ( 'NONE',  ( 118.1851208724671238, -36.91582462397654751, 149.8127681330539644 ) ) ;
#6889=ORIENTED_EDGE ( 'NONE', *, *, #17770, .F. ) ;
#6890=CARTESIAN_POINT ( 'NONE',  ( 97.24442698086048154, -40.26379795196656630, 262.6013395616254797 ) ) ;
#6891=CARTESIAN_POINT ( 'NONE',  ( 98.04096435976430257, -41.04069707603596129, 252.6812049413570946 ) ) ;
#6895=AXIS2_PLACEMENT_3D ( 'NONE', #44826, #66613, #12107 ) ;
#6897=DIRECTION ( 'NONE',  ( 0.000000000000000000, 0.000000000000000000, -1.000000000000000000 ) ) ;
#6899=AXIS2_PLACEMENT_3D ( 'NONE', #17138, #45262, #25273 ) ;
#6900=CARTESIAN_POINT ( 'NONE',  ( 98.80555182512723889, -41.96590078842033478, 186.7756252759109543 ) ) ;
#6901=VERTEX_POINT ( 'NONE', #78182 ) ;
#6902=ORIENTED_EDGE ( 'NONE', *, *, #6590, .T. ) ;
#6903=CARTESIAN_POINT ( 'NONE',  ( 111.6733053606431412, -27.77132819582071122, 166.1301547344679932 ) ) ;
#6904=LINE ( 'NONE', #29149, #19730 ) ;
#6905=ADVANCED_FACE ( 'NONE', ( #44061 ), #23654, .T. ) ;
#6906=CARTESIAN_POINT ( 'NONE',  ( 98.92341559625380398, -33.23365848574461268, 12.43586902018295426 ) ) ;
#6907=CARTESIAN_POINT ( 'NONE',  ( 79.68958420874191972, -33.97944715994105991, 1.625625275910942635 ) ) ;
#6909=EDGE_CURVE ( 'NONE', #14493, #24486, #1862, .T. ) ;
#6911=ADVANCED_FACE ( 'NONE', ( #30458 ), #58156, .T. ) ;
#6913=CARTESIAN_POINT ( 'NONE',  ( 107.0667039024479834, -36.72944715994100306, 239.5838068554170093 ) ) ;
#6914=CARTESIAN_POINT ( 'NONE',  ( 88.06670390244796920, -14.72944715994105991, 199.5838068554169809 ) ) ;
#6915=CARTESIAN_POINT ( 'NONE',  ( 104.4161250475293343, -26.02246701806295448, 240.2575300378159682 ) ) ;
#6916=CARTESIAN_POINT ( 'NONE',  ( 97.78518716477550754, -40.45211749721122629, 171.6302806827789311 ) ) ;
#6919=EDGE_CURVE ( 'NONE', #47694, #68380, #71313, .T. ) ;
#6923=CARTESIAN_POINT ( 'NONE',  ( 109.6438830164042031, -46.47987668453704657, 123.7798306129299846 ) ) ;
#6925=CIRCLE ( 'NONE', #38826, 4.749999999999976907 ) ;
#6927=FACE_OUTER_BOUND ( 'NONE', #37041, .T. ) ;
#6929=ORIENTED_EDGE ( 'NONE', *, *, #44609, .T. ) ;
#6930=CARTESIAN_POINT ( 'NONE',  ( 99.73159624296292236, -44.24858557630691536, 17.96133956162493206 ) ) ;
#6931=EDGE_CURVE ( 'NONE', #65097, #79518, #43615, .T. ) ;
#6932=CARTESIAN_POINT ( 'NONE',  ( 115.9069864544413662, -30.09434420101750973, 264.3508633711492735 ) ) ;
#6935=ADVANCED_FACE ( 'NONE', ( #50890 ), #78630, .F. ) ;
#6936=DIRECTION ( 'NONE',  ( 0.000000000000000000, 0.000000000000000000, -1.000000000000000000 ) ) ;
#6937=CARTESIAN_POINT ( 'NONE',  ( 116.9214244060436840, -38.68692813258547147, 168.6706793604847974 ) ) ;
#6938=ADVANCED_FACE ( 'NONE', ( #18945 ), #67991, .F. ) ;
#6939=CARTESIAN_POINT ( 'NONE',  ( 114.1581430127411352, -30.74577825543392606, 72.20237608387697037 ) ) ;
#6940=CARTESIAN_POINT ( 'NONE',  ( 111.4263534857568771, -47.77543206737910708, 168.8756252759109486 ) ) ;
#6946=ORIENTED_EDGE ( 'NONE', *, *, #32941, .T. ) ;
#6947=VECTOR ( 'NONE', #16726, 1000.000000000000000 ) ;
#6948=CIRCLE ( 'NONE', #48936, 3.299999999999999822 ) ;
#6951=ORIENTED_EDGE ( 'NONE', *, *, #37541, .F. ) ;
#6952=DIRECTION ( 'NONE',  ( 1.000000000000000000, 0.000000000000000000, 0.000000000000000000 ) ) ;
#6953=CARTESIAN_POINT ( 'NONE',  ( 106.7337219657603100, -28.19449539544314476, 84.52956268522000016 ) ) ;
#6954=CARTESIAN_POINT ( 'NONE',  ( 95.27000809083011745, -38.09955253919518015, 236.4184824187679510 ) ) ;
#6955=ADVANCED_FACE ( 'NONE', ( #75260, #89344 ), #88895, .F. ) ;
#6956=AXIS2_PLACEMENT_3D ( 'NONE', #76634, #2129, #42979 ) ;
#6957=CARTESIAN_POINT ( 'NONE',  ( 113.1426608820138426, -26.58408993604425419, 204.6470538473399756 ) ) ;
#6958=CARTESIAN_POINT ( 'NONE',  ( 99.08262072259969955, -44.34008189452608661, 32.92038718067297509 ) ) ;
#6959=ADVANCED_FACE ( 'NONE', ( #41604 ), #17614, .F. ) ;
#6960=DIRECTION ( 'NONE',  ( 1.000000000000000000, 0.000000000000000000, 0.000000000000000000 ) ) ;
#6961=CARTESIAN_POINT ( 'NONE',  ( 108.3313211724201182, -46.73510064337951064, 93.67712277074488725 ) ) ;
#6962=EDGE_CURVE ( 'NONE', #24929, #20886, #89795, .T. ) ;
#6963=VECTOR ( 'NONE', #89812, 999.9999999999998863 ) ;
#6964=ORIENTED_EDGE ( 'NONE', *, *, #67334, .T. ) ;
#6967=CIRCLE ( 'NONE', #17097, 1.000000000000000888 ) ;
#6968=VECTOR ( 'NONE', #15751, 1000.000000000000000 ) ;
#6969=CARTESIAN_POINT ( 'NONE',  ( 96.71010325458811963, -37.26253042779857338, 121.3794347997209684 ) ) ;
#6970=CARTESIAN_POINT ( 'NONE',  ( 117.4914506980151572, -37.69211045134998272, 78.75276813305399060 ) ) ;
#6971=CARTESIAN_POINT ( 'NONE',  ( 115.9975756407361018, -30.13790158448777845, 259.3203871806730945 ) ) ;
#6973=CARTESIAN_POINT ( 'NONE',  ( 115.4600223225059494, -29.53725764737424342, 229.4022919425779605 ) ) ;
#6974=CARTESIAN_POINT ( 'NONE',  ( 25.56670390244744340, -48.82844715994178841, 175.7178068554150627 ) ) ;
#6975=DIRECTION ( 'NONE',  ( 1.000000000000000000, 3.999999999999999995E-14, 1.000000000000000078E-15 ) ) ;
#6977=FACE_OUTER_BOUND ( 'NONE', #33388, .T. ) ;
#6978=LINE ( 'NONE', #43270, #45641 ) ;
#6979=DIRECTION ( 'NONE',  ( -1.000000000000000000, 1.816601132648505598E-15, 0.000000000000000000 ) ) ;
#6980=DIRECTION ( 'NONE',  ( 0.000000000000000000, -1.000000000000000000, 0.000000000000000000 ) ) ;
#6982=AXIS2_PLACEMENT_3D ( 'NONE', #74538, #19127, #39561 ) ;
#6983=DIRECTION ( 'NONE',  ( -1.000000000000000000, -4.299999999999999979E-14, -1.000000000000000078E-15 ) ) ;
#6988=CARTESIAN_POINT ( 'NONE',  ( 107.0667039024467186, -36.72944715994091069, 195.5838068554169809 ) ) ;
#6989=CARTESIAN_POINT ( 'NONE',  ( 99.36516439250377175, -29.66998179773359823, 275.7356252759109907 ) ) ;
#6990=CARTESIAN_POINT ( 'NONE',  ( 108.0069324954157537, -26.34569400419502827, 151.0041967044829505 ) ) ;
#6991=CARTESIAN_POINT ( 'NONE',  ( 100.8224507837568638, -45.17634439094529597, 253.0699109901969450 ) ) ;
#6996=CARTESIAN_POINT ( 'NONE',  ( 108.3333560997344733, -46.73487186194755338, 138.6772847610721726 ) ) ;
#6998=PLANE ( 'NONE',  #73185 ) ;
#6999=ORIENTED_EDGE ( 'NONE', *, *, #78443, .T. ) ;
#7002=CARTESIAN_POINT ( 'NONE',  ( 97.64684354035226477, -39.08338314719364348, 165.9438483995059528 ) ) ;
#7003=CARTESIAN_POINT ( 'NONE',  ( 98.30741342104360569, -41.72858007013866910, 186.7402835883439138 ) ) ;
#7004=ORIENTED_EDGE ( 'NONE', *, *, #65276, .T. ) ;
#7005=FACE_OUTER_BOUND ( 'NONE', #28073, .T. ) ;
#7006=CARTESIAN_POINT ( 'NONE',  ( 113.5515132932710713, -44.90922781482908732, 164.1099109901969655 ) ) ;
#7007=FACE_OUTER_BOUND ( 'NONE', #63430, .T. ) ;
#7008=LINE ( 'NONE', #33029, #79141 ) ;
#7009=LINE ( 'NONE', #12941, #6646 ) ;
#7011=DIRECTION ( 'NONE',  ( 0.000000000000000000, 0.000000000000000000, -1.000000000000000000 ) ) ;
#7012=CARTESIAN_POINT ( 'NONE',  ( 98.13101841594837538, -32.75189731695855500, 100.9927681330539713 ) ) ;
#7015=EDGE_LOOP ( 'NONE', ( #31162, #32205 ) ) ;
#7016=AXIS2_PLACEMENT_3D ( 'NONE', #14271, #41945, #88001 ) ;
#7017=AXIS2_PLACEMENT_3D ( 'NONE', #2647, #44845, #16715 ) ;
#7018=CARTESIAN_POINT ( 'NONE',  ( 41.56648329127499153, -36.32844715994070839, 254.1756252759120400 ) ) ;
#7019=CARTESIAN_POINT ( 'NONE',  ( 102.9544237342424395, -27.85507949283302764, 176.4213395616249898 ) ) ;
#7020=CARTESIAN_POINT ( 'NONE',  ( 101.9936210298387635, -45.44607158966083205, 37.15645861734014233 ) ) ;
#7021=DIRECTION ( 'NONE',  ( 1.000000000000000078E-15, -1.000000000000000083E-30, -1.000000000000000000 ) ) ;
#7022=EDGE_CURVE ( 'NONE', #64215, #2723, #84200, .T. ) ;
#7025=DIRECTION ( 'NONE',  ( -1.000000000000000078E-15, 0.000000000000000000, 1.000000000000000000 ) ) ;
#7027=EDGE_CURVE ( 'NONE', #10583, #42662, #50991, .T. ) ;
#7028=DIRECTION ( 'NONE',  ( 0.000000000000000000, 0.000000000000000000, -1.000000000000000000 ) ) ;
#7029=DIRECTION ( 'NONE',  ( 0.7071067811865434649, 0.7071067811865516806, 7.071067811865440820E-16 ) ) ;
#7030=CARTESIAN_POINT ( 'NONE',  ( 98.22092589535427010, -43.31882777834842813, 111.8480062282919647 ) ) ;
#7031=ORIENTED_EDGE ( 'NONE', *, *, #39109, .T. ) ;
#7032=ORIENTED_EDGE ( 'NONE', *, *, #15977, .F. ) ;
#7035=EDGE_CURVE ( 'NONE', #67326, #24182, #79999, .T. ) ;
#7036=ADVANCED_FACE ( 'NONE', ( #19393 ), #13475, .T. ) ;
#7038=CARTESIAN_POINT ( 'NONE',  ( 41.56648329127398966, -27.82844715994070484, 135.9256252759119832 ) ) ;
#7039=AXIS2_PLACEMENT_3D ( 'NONE', #89892, #40817, #28079 ) ;
#7041=CARTESIAN_POINT ( 'NONE',  ( 113.2509217664418202, -31.40192927973085801, 182.2109475124489677 ) ) ;
#7042=EDGE_CURVE ( 'NONE', #60711, #79108, #87248, .T. ) ;
#7043=CARTESIAN_POINT ( 'NONE',  ( 167.2371591254542693, -47.82818131005522844, 313.9678068554149490 ) ) ;
#7044=EDGE_CURVE ( 'NONE', #67515, #86125, #11833, .T. ) ;
#7045=CARTESIAN_POINT ( 'NONE',  ( 134.0664832912739826, -9.029447159941003775, 8.225625275910998013 ) ) ;
#7046=ORIENTED_EDGE ( 'NONE', *, *, #55799, .T. ) ;
#7048=ORIENTED_EDGE ( 'NONE', *, *, #86607, .F. ) ;
#7051=ORIENTED_EDGE ( 'NONE', *, *, #33199, .F. ) ;
#7053=CARTESIAN_POINT ( 'NONE',  ( 78.26014418490247238, -20.80290789369970739, 7.687431601936206782 ) ) ;
#7054=EDGE_CURVE ( 'NONE', #65246, #67223, #27862, .T. ) ;
#7055=CARTESIAN_POINT ( 'NONE',  ( 101.7595872045747285, -44.48272901101389465, 238.5425356868499591 ) ) ;
#7056=ORIENTED_EDGE ( 'NONE', *, *, #27552, .T. ) ;
#7057=CIRCLE ( 'NONE', #57820, 1.000000000000000888 ) ;
#7058=DIRECTION ( 'NONE',  ( 0.000000000000000000, 0.000000000000000000, 1.000000000000000000 ) ) ;
#7059=AXIS2_PLACEMENT_3D ( 'NONE', #19419, #34382, #33042 ) ;
#7060=EDGE_CURVE ( 'NONE', #82586, #50189, #36158, .T. ) ;
#7064=DIRECTION ( 'NONE',  ( -0.08544974978095701279, -0.9963424814100680926, -0.000000000000000000 ) ) ;
#7065=ORIENTED_EDGE ( 'NONE', *, *, #72271, .F. ) ;
#7066=VERTEX_POINT ( 'NONE', #70683 ) ;
#7067=CARTESIAN_POINT ( 'NONE',  ( 114.3096959184101280, -40.49343719410034481, 286.2623760838771432 ) ) ;
#7068=CARTESIAN_POINT ( 'NONE',  ( 97.81638875629413121, -31.87330516686267501, 135.9413395616259947 ) ) ;
#7069=CARTESIAN_POINT ( 'NONE',  ( 103.2134869792595708, -46.43093390711695889, 117.2756252759109543 ) ) ;
#7070=CARTESIAN_POINT ( 'NONE',  ( 99.34172024792457023, -34.41985901539234760, 249.5838068554171798 ) ) ;
#7071=DIRECTION ( 'NONE',  ( 0.7071067811874389708, -0.7071067811856560636, 0.000000000000000000 ) ) ;
#7072=CARTESIAN_POINT ( 'NONE',  ( 101.3491664457538945, -46.18916536780651683, 198.1318157521009482 ) ) ;
#7073=CARTESIAN_POINT ( 'NONE',  ( 163.0667039024470171, -32.29483332968611364, -5.074374724088000832 ) ) ;
#7074=CARTESIAN_POINT ( 'NONE',  ( 194.0371591254585155, -46.82818131005408446, 117.4678068554150627 ) ) ;
#7075=ORIENTED_EDGE ( 'NONE', *, *, #76850, .F. ) ;
#7077=ORIENTED_EDGE ( 'NONE', *, *, #61560, .F. ) ;
#7078=EDGE_CURVE ( 'NONE', #59914, #49287, #8459, .T. ) ;
#7080=VERTEX_POINT ( 'NONE', #35700 ) ;
#7081=DIRECTION ( 'NONE',  ( 4.299999999999999979E-14, -1.000000000000000000, 4.400000000000000367E-29 ) ) ;
#7082=EDGE_CURVE ( 'NONE', #69308, #85489, #23472, .T. ) ;
#7083=AXIS2_PLACEMENT_3D ( 'NONE', #59042, #64990, #45410 ) ;
#7085=VECTOR ( 'NONE', #22358, 1000.000000000000000 ) ;
#7086=CARTESIAN_POINT ( 'NONE',  ( 107.9456392385311005, -25.71100025151098478, 115.0251490854349612 ) ) ;
#7089=FACE_OUTER_BOUND ( 'NONE', #25418, .T. ) ;
#7090=PLANE ( 'NONE',  #72513 ) ;
#7091=CARTESIAN_POINT ( 'NONE',  ( 103.1008684890620799, -45.92814942240114107, 57.25235007397393616 ) ) ;
#7092=CARTESIAN_POINT ( 'NONE',  ( 98.91597900623165174, -29.29754952351882480, 226.7261014663869503 ) ) ;
#7099=FACE_BOUND ( 'NONE', #7499, .T. ) ;
#7100=AXIS2_PLACEMENT_3D ( 'NONE', #16306, #22231, #27350 ) ;
#7103=CARTESIAN_POINT ( 'NONE',  ( 105.8886092880350560, -47.16805723083484736, 282.4870538473393253 ) ) ;
#7106=CARTESIAN_POINT ( 'NONE',  ( 96.59657429157336139, -36.21044007025302136, 171.2870538473399620 ) ) ;
#7107=CARTESIAN_POINT ( 'NONE',  ( 95.25919473906076007, -35.71823372881362957, 32.25848241876794020 ) ) ;
#7108=CARTESIAN_POINT ( 'NONE',  ( 96.60651355459405920, -37.15606806638657389, 157.3584824187679487 ) ) ;
#7109=CARTESIAN_POINT ( 'NONE',  ( 34.67381068362099228, -26.00627455219321860, -5.074374724088000832 ) ) ;
#7111=CARTESIAN_POINT ( 'NONE',  ( 97.78479533213763375, -40.45114042110355967, 102.6299318713464714 ) ) ;
#7114=DIRECTION ( 'NONE',  ( -0.000000000000000000, 1.000000000000000000, 0.000000000000000000 ) ) ;
#7115=CARTESIAN_POINT ( 'NONE',  ( 63.56670390244739366, -47.82844715994014706, 180.4678068554151196 ) ) ;
#7117=EDGE_CURVE ( 'NONE', #43071, #5926, #74215, .T. ) ;
#7119=VERTEX_POINT ( 'NONE', #57489 ) ;
#7120=ORIENTED_EDGE ( 'NONE', *, *, #49047, .F. ) ;
#7121=VECTOR ( 'NONE', #81722, 1000.000000000000000 ) ;
#7122=ORIENTED_EDGE ( 'NONE', *, *, #85011, .T. ) ;
#7123=CARTESIAN_POINT ( 'NONE',  ( 107.3204973292724134, -25.70223992296343241, 71.04610146638795243 ) ) ;
#7124=CARTESIAN_POINT ( 'NONE',  ( 50.87649884952499946, -33.54226604284930602, 342.9256252759119548 ) ) ;
#7125=CYLINDRICAL_SURFACE ( 'NONE', #13762, 11.57110091390450179 ) ;
#7126=CARTESIAN_POINT ( 'NONE',  ( 108.3715344132687051, -47.75189438633907457, 158.6822919425779617 ) ) ;
#7128=CARTESIAN_POINT ( 'NONE',  ( 110.0852322082900372, -46.03269033891531592, 12.82705384733995402 ) ) ;
#7130=AXIS2_PLACEMENT_3D ( 'NONE', #2125, #319, #62987 ) ;
#7132=VERTEX_POINT ( 'NONE', #50670 ) ;
#7134=LINE ( 'NONE', #49792, #75369 ) ;
#7135=CARTESIAN_POINT ( 'NONE',  ( 25.56670390244744695, -48.82844715994178841, 173.2178068554150627 ) ) ;
#7136=DIRECTION ( 'NONE',  ( 0.9242245927363033076, 0.3818493186865918876, 0.000000000000000000 ) ) ;
#7138=ADVANCED_FACE ( 'NONE', ( #42060 ), #78411, .T. ) ;
#7139=DIRECTION ( 'NONE',  ( -2.999999999999999839E-15, 1.000000000000000000, -2.999999999999999900E-30 ) ) ;
#7142=EDGE_CURVE ( 'NONE', #29714, #47593, #30709, .T. ) ;
#7144=CARTESIAN_POINT ( 'NONE',  ( 97.12559377168363994, -39.79659400623925336, 21.56419670448195092 ) ) ;
#7145=DIRECTION ( 'NONE',  ( 1.000000000000000000, 2.999999999999999839E-15, 1.000000000000000078E-15 ) ) ;
#7147=CIRCLE ( 'NONE', #57903, 0.5000000000000079936 ) ;
#7148=ADVANCED_FACE ( 'NONE', ( #49322 ), #69786, .T. ) ;
#7149=DIRECTION ( 'NONE',  ( 1.000000000000000078E-15, -1.000000000000000083E-30, -1.000000000000000000 ) ) ;
#7150=DIRECTION ( 'NONE',  ( 0.000000000000000000, 0.000000000000000000, -1.000000000000000000 ) ) ;
#7151=CARTESIAN_POINT ( 'NONE',  ( 116.2870986197744969, -35.69205421237206366, 81.73380465530594563 ) ) ;
#7153=AXIS2_PLACEMENT_3D ( 'NONE', #80907, #18656, #17765 ) ;
#7154=EDGE_CURVE ( 'NONE', #38840, #14111, #13328, .T. ) ;
#7156=EDGE_CURVE ( 'NONE', #38464, #33505, #29290, .T. ) ;
#7157=CARTESIAN_POINT ( 'NONE',  ( 90.44969454456439450, -20.11243780205712639, 249.5838068554174924 ) ) ;
#7159=EDGE_LOOP ( 'NONE', ( #22491, #36896 ) ) ;
#7160=VECTOR ( 'NONE', #57308, 999.9999999999998863 ) ;
#7161=CARTESIAN_POINT ( 'NONE',  ( 79.32178306377458910, -34.08035908359609323, 8.141856907858651127 ) ) ;
#7162=VERTEX_POINT ( 'NONE', #17500 ) ;
#7163=CARTESIAN_POINT ( 'NONE',  ( 108.3661291232776023, -47.70624136733754028, 162.6822919425769669 ) ) ;
#7164=ORIENTED_EDGE ( 'NONE', *, *, #70515, .T. ) ;
#7167=CARTESIAN_POINT ( 'NONE',  ( 113.1640969444738971, -43.88191609279036243, 149.5825356868499512 ) ) ;
#7168=DIRECTION ( 'NONE',  ( -1.054009200593500181E-15, -1.000000000000000000, 0.000000000000000000 ) ) ;
#7170=CARTESIAN_POINT ( 'NONE',  ( 97.75304581901603740, -31.99688534799786765, 46.95276813305393659 ) ) ;
#7175=ORIENTED_EDGE ( 'NONE', *, *, #42821, .T. ) ;
#7179=CARTESIAN_POINT ( 'NONE',  ( 98.44183741489689510, -42.05700530801252768, 11.76800622829193799 ) ) ;
#7180=CARTESIAN_POINT ( 'NONE',  ( 114.5277216628477248, -29.41153075798395733, 145.4441967044819819 ) ) ;
#7182=CARTESIAN_POINT ( 'NONE',  ( 116.7941748454729378, -39.39121522621098137, 129.6145142487127373 ) ) ;
#7183=CARTESIAN_POINT ( 'NONE',  ( 108.9852221676114539, -46.97644323546262513, 78.72419670448194040 ) ) ;
#7184=CARTESIAN_POINT ( 'NONE',  ( 109.6430121533087174, -46.48008672894804505, 262.7814586111080644 ) ) ;
#7188=EDGE_CURVE ( 'NONE', #85115, #59657, #80062, .T. ) ;
#7193=CARTESIAN_POINT ( 'NONE',  ( 116.7701435943788653, -31.43623786049258584, 24.21181575210196257 ) ) ;
#7196=CARTESIAN_POINT ( 'NONE',  ( 194.0667039024482108, -40.32844715993407192, 180.4678068554150343 ) ) ;
#7197=CARTESIAN_POINT ( 'NONE',  ( 104.4155842956043614, -46.14412563975625403, 22.35848241876892217 ) ) ;
#7198=CARTESIAN_POINT ( 'NONE',  ( 97.01979814536845481, -36.11691246787002285, 101.2783118708028098 ) ) ;
#7199=CARTESIAN_POINT ( 'NONE',  ( 117.1424269838422987, -34.14023410701943817, 120.0270538473389479 ) ) ;
#7200=CYLINDRICAL_SURFACE ( 'NONE', #47982, 2.500000000000002220 ) ;
#7201=CARTESIAN_POINT ( 'NONE',  ( 114.8468557742592822, -29.67128889090990640, 209.4127681330539872 ) ) ;
#7204=CARTESIAN_POINT ( 'NONE',  ( 172.5664832912740110, 0.2215528400590013880, 256.8086252759120498 ) ) ;
#7207=CARTESIAN_POINT ( 'NONE',  ( 162.8913605087219878, -31.76306994223740432, -5.074374724088000832 ) ) ;
#7208=ORIENTED_EDGE ( 'NONE', *, *, #50630, .T. ) ;
#7209=CIRCLE ( 'NONE', #49195, 0.5000000000000004441 ) ;
#7211=CARTESIAN_POINT ( 'NONE',  ( 106.9746081534954669, -47.19836424831742505, 187.5699109901969734 ) ) ;
#7213=LINE ( 'NONE', #75358, #49456 ) ;
#7214=CARTESIAN_POINT ( 'NONE',  ( 106.8511646352646380, -47.80368950967726249, 223.5489586092439538 ) ) ;
#7216=LINE ( 'NONE', #34905, #72101 ) ;
#7217=CIRCLE ( 'NONE', #37689, 2.517500000000005844 ) ;
#7218=DIRECTION ( 'NONE',  ( 1.000000000000000000, 0.000000000000000000, 0.000000000000000000 ) ) ;
#7219=ORIENTED_EDGE ( 'NONE', *, *, #66210, .T. ) ;
#7220=AXIS2_PLACEMENT_3D ( 'NONE', #69280, #36558, #77890 ) ;
#7224=VECTOR ( 'NONE', #79020, 1000.000000000000000 ) ;
#7225=EDGE_LOOP ( 'NONE', ( #4998, #65786, #65384, #60754 ) ) ;
#7227=CARTESIAN_POINT ( 'NONE',  ( 118.0509465330791983, -35.49837129967784222, 229.9032443235299468 ) ) ;
#7231=CIRCLE ( 'NONE', #36209, 3.000000000000002665 ) ;
#7234=FACE_OUTER_BOUND ( 'NONE', #183, .T. ) ;
#7235=CARTESIAN_POINT ( 'NONE',  ( 97.08353706812128792, -39.80957011747380392, 21.56419670448195092 ) ) ;
#7236=ORIENTED_EDGE ( 'NONE', *, *, #33494, .T. ) ;
#7238=CARTESIAN_POINT ( 'NONE',  ( 25.56670390244722313, -42.82844715994178131, 137.2178068554150627 ) ) ;
#7239=CARTESIAN_POINT ( 'NONE',  ( 104.4910769649052895, -26.97849904278172417, 16.28477933405083178 ) ) ;
#7240=CARTESIAN_POINT ( 'NONE',  ( 114.1395267584829014, -29.97404255306821241, 230.4327681330529742 ) ) ;
#7241=EDGE_CURVE ( 'NONE', #65898, #53353, #87435, .T. ) ;
#7242=AXIS2_PLACEMENT_3D ( 'NONE', #69203, #47839, #68756 ) ;
#7243=DIRECTION ( 'NONE',  ( 0.000000000000000000, 0.000000000000000000, 1.000000000000000000 ) ) ;
#7244=CARTESIAN_POINT ( 'NONE',  ( 97.28369645613172167, -37.51102008256656717, 97.38991099019594344 ) ) ;
#7247=EDGE_CURVE ( 'NONE', #28751, #45771, #17057, .T. ) ;
#7250=DIRECTION ( 'NONE',  ( 1.000000000000000000, 0.000000000000000000, 0.000000000000000000 ) ) ;
#7252=ORIENTED_EDGE ( 'NONE', *, *, #22626, .T. ) ;
#7253=VERTEX_POINT ( 'NONE', #17934 ) ;
#7255=CARTESIAN_POINT ( 'NONE',  ( 97.87165577458247867, -34.79769342939158605, 257.6053928297065454 ) ) ;
#7256=FACE_OUTER_BOUND ( 'NONE', #74119, .T. ) ;
#7259=ADVANCED_FACE ( 'NONE', ( #59264 ), #58811, .T. ) ;
#7260=DIRECTION ( 'NONE',  ( -0.7071067811865462405, 0.000000000000000000, 0.7071067811865486830 ) ) ;
#7261=EDGE_LOOP ( 'NONE', ( #38067, #49841, #8229, #77872 ) ) ;
#7262=CIRCLE ( 'NONE', #29048, 11.57110091390434192 ) ;
#7264=DIRECTION ( 'NONE',  ( 0.000000000000000000, 0.000000000000000000, -1.000000000000000000 ) ) ;
#7266=CARTESIAN_POINT ( 'NONE',  ( 96.83338659586634378, -38.89961736000394410, 31.49276813305495892 ) ) ;
#7268=CARTESIAN_POINT ( 'NONE',  ( 114.5155466417691912, -41.88356374938643256, 12.77908649474396263 ) ) ;
#7270=CARTESIAN_POINT ( 'NONE',  ( 168.5667039024482960, -48.82844715993516616, 180.4678068554150059 ) ) ;
#7271=CARTESIAN_POINT ( 'NONE',  ( 98.33750497493203113, -41.21483588869663350, 196.7041967044829676 ) ) ;
#7273=DIRECTION ( 'NONE',  ( 0.000000000000000000, 0.000000000000000000, -1.000000000000000000 ) ) ;
#7274=CARTESIAN_POINT ( 'NONE',  ( 41.56648329127398966, -27.82844715994070484, 78.92562527591199739 ) ) ;
#7275=CARTESIAN_POINT ( 'NONE',  ( 172.5664832912729878, -27.82844715994070484, 15.92562527591200094 ) ) ;
#7276=CARTESIAN_POINT ( 'NONE',  ( 115.4949314580552624, -29.50734498268579387, 225.4022919425769658 ) ) ;
#7279=ORIENTED_EDGE ( 'NONE', *, *, #556, .F. ) ;
#7280=CARTESIAN_POINT ( 'NONE',  ( 136.5939002653012437, -37.81452881270037381, 7.047625865518532429 ) ) ;
#7282=CARTESIAN_POINT ( 'NONE',  ( 116.6381559899473217, -29.65878987416117241, 105.3327681330539463 ) ) ;
#7284=ORIENTED_EDGE ( 'NONE', *, *, #58792, .T. ) ;
#7287=AXIS2_PLACEMENT_3D ( 'NONE', #50048, #64597, #36451 ) ;
#7288=CARTESIAN_POINT ( 'NONE',  ( 179.1667039024475230, -28.27351298636771659, 237.4678068554150059 ) ) ;
#7289=DIRECTION ( 'NONE',  ( -4.237773401492740281E-14, 1.000000000000000000, 0.000000000000000000 ) ) ;
#7294=CARTESIAN_POINT ( 'NONE',  ( 113.2509217664418202, -31.40192927973085801, 182.2109475124489677 ) ) ;
#7295=CARTESIAN_POINT ( 'NONE',  ( 116.6018303087422225, -42.36526137987677743, 279.4137205140061724 ) ) ;
#7296=CARTESIAN_POINT ( 'NONE',  ( 97.86663541234594277, -40.64936128125661696, 57.64699884062476798 ) ) ;
#7300=FACE_OUTER_BOUND ( 'NONE', #45974, .T. ) ;
#7302=ORIENTED_EDGE ( 'NONE', *, *, #12341, .T. ) ;
#7304=CARTESIAN_POINT ( 'NONE',  ( 172.5664832912728457, -18.82844715994071194, 21.92562527591192989 ) ) ;
#7305=CYLINDRICAL_SURFACE ( 'NONE', #25410, 3.000000000000002665 ) ;
#7308=DIRECTION ( 'NONE',  ( 0.000000000000000000, -1.000000000000000000, 0.000000000000000000 ) ) ;
#7309=CIRCLE ( 'NONE', #36288, 2.030000000002079918 ) ;
#7310=CARTESIAN_POINT ( 'NONE',  ( 99.85230398470191915, -41.30238370604462261, 186.1981341137909567 ) ) ;
#7311=CARTESIAN_POINT ( 'NONE',  ( 98.55409819730274990, -43.85350384415066571, 71.86895860924397539 ) ) ;
#7314=ORIENTED_EDGE ( 'NONE', *, *, #77485, .F. ) ;
#7316=ORIENTED_EDGE ( 'NONE', *, *, #84660, .F. ) ;
#7318=ORIENTED_EDGE ( 'NONE', *, *, #75547, .T. ) ;
#7319=LINE ( 'NONE', #69992, #34879 ) ;
#7321=CARTESIAN_POINT ( 'NONE',  ( 113.1800950244601296, -44.75052191892536513, 274.0936886138787258 ) ) ;
#7322=CIRCLE ( 'NONE', #50814, 15.69999999999999041 ) ;
#7323=DIRECTION ( 'NONE',  ( -1.000000000000000000, 1.011922027653136551E-15, 0.000000000000000000 ) ) ;
#7324=ORIENTED_EDGE ( 'NONE', *, *, #52668, .F. ) ;
#7325=EDGE_CURVE ( 'NONE', #79308, #13477, #52422, .T. ) ;
#7326=CARTESIAN_POINT ( 'NONE',  ( 96.31560519187928548, -41.77450771427546528, 61.67562527591097421 ) ) ;
#7329=DIRECTION ( 'NONE',  ( 2.900000000000000265E-14, -2.000000000000000155E-15, 1.000000000000000000 ) ) ;
#7330=CARTESIAN_POINT ( 'NONE',  ( 134.0664832912739826, -15.97944715994100306, 1.625625275910997480 ) ) ;
#7331=ORIENTED_EDGE ( 'NONE', *, *, #72210, .F. ) ;
#7332=CIRCLE ( 'NONE', #85676, 2.749999999999974687 ) ;
#7333=DIRECTION ( 'NONE',  ( -0.8543009526837940237, -0.03605348183280988883, 0.5185267868599396923 ) ) ;
#7336=DIRECTION ( 'NONE',  ( 1.000000000000000000, 4.163336342344333240E-14, 0.000000000000000000 ) ) ;
#7338=CARTESIAN_POINT ( 'NONE',  ( 117.2433672581536968, -42.84935593481555571, 124.3956252759109731 ) ) ;
#7339=CARTESIAN_POINT ( 'NONE',  ( 91.12500358871285755, -35.36225116344564157, 247.7440089327910755 ) ) ;
#7340=CARTESIAN_POINT ( 'NONE',  ( 127.0664832912738262, -46.72944715994102438, 14.82207188531765318 ) ) ;
#7341=DIRECTION ( 'NONE',  ( -1.000000000000000000, 8.775353200852647323E-16, 0.000000000000000000 ) ) ;
#7342=CARTESIAN_POINT ( 'NONE',  ( 51.56670390244799762, -33.35206098992650681, -5.074374724088000832 ) ) ;
#7343=CARTESIAN_POINT ( 'NONE',  ( 98.15811136316406760, -31.42099212808723863, 126.9108633711489915 ) ) ;
#7344=AXIS2_PLACEMENT_3D ( 'NONE', #26384, #47254, #33200 ) ;
#7345=CARTESIAN_POINT ( 'NONE',  ( 31.56670390244671509, -32.29483332968584364, 193.9678068554150911 ) ) ;
#7347=CARTESIAN_POINT ( 'NONE',  ( 108.0121126588926046, -24.94157235513516468, 261.0127681330534415 ) ) ;
#7349=DIRECTION ( 'NONE',  ( -0.7071067811866279529, 0.7071067811864671926, -7.071067811866286874E-16 ) ) ;
#7350=CARTESIAN_POINT ( 'NONE',  ( 107.0664832912750057, -36.72944715993903486, 9.425625275910970657 ) ) ;
#7355=CARTESIAN_POINT ( 'NONE',  ( 99.57924082623969753, -30.38476633542323313, 215.7670538473399517 ) ) ;
#7357=ORIENTED_EDGE ( 'NONE', *, *, #76967, .F. ) ;
#7358=CARTESIAN_POINT ( 'NONE',  ( 109.0885512386393259, -27.55405797182273631, 176.3234880678019465 ) ) ;
#7360=CARTESIAN_POINT ( 'NONE',  ( 113.3415799102510277, -29.55617248177381740, 285.5032443235294863 ) ) ;
#7361=CARTESIAN_POINT ( 'NONE',  ( 63.06670390244799052, -40.32844715994017548, 249.9678068554150343 ) ) ;
#7363=CARTESIAN_POINT ( 'NONE',  ( 109.6423509097492683, -46.48025314540840469, 267.7815664546420180 ) ) ;
#7364=EDGE_CURVE ( 'NONE', #40724, #8960, #59535, .T. ) ;
#7366=CIRCLE ( 'NONE', #68257, 11.45913725231036118 ) ;
#7368=DIRECTION ( 'NONE',  ( 0.000000000000000000, 0.000000000000000000, -1.000000000000000000 ) ) ;
#7370=CARTESIAN_POINT ( 'NONE',  ( 118.7655994573051714, -38.45539276985795851, 223.7099109901969598 ) ) ;
#7371=DIRECTION ( 'NONE',  ( 0.000000000000000000, 1.000000000000000000, 0.000000000000000000 ) ) ;
#7373=ORIENTED_EDGE ( 'NONE', *, *, #87930, .F. ) ;
#7374=CARTESIAN_POINT ( 'NONE',  ( 107.0709637938113445, -25.26751228799909299, 321.4478161181093583 ) ) ;
#7375=CARTESIAN_POINT ( 'NONE',  ( 82.76600038373111090, -19.25405382162969303, 6.823682607504162334 ) ) ;
#7376=DIRECTION ( 'NONE',  ( 1.000000000000000000, 4.510281037539788691E-14, 0.000000000000000000 ) ) ;
#7377=CYLINDRICAL_SURFACE ( 'NONE', #36068, 2.749999999999974687 ) ;
#7380=CARTESIAN_POINT ( 'NONE',  ( 97.81168895331838087, -40.51742574516882200, 287.6356252759109680 ) ) ;
#7381=ORIENTED_EDGE ( 'NONE', *, *, #9709, .T. ) ;
#7383=CARTESIAN_POINT ( 'NONE',  ( 96.26778515314977369, -34.36995442310919202, 256.1432443235300980 ) ) ;
#7385=CARTESIAN_POINT ( 'NONE',  ( 77.72936414032395191, -38.17925173417307150, 7.255518600572461452 ) ) ;
#7388=CARTESIAN_POINT ( 'NONE',  ( 107.2657893863845260, -28.07721033202879113, 72.86428084578200526 ) ) ;
#7389=CARTESIAN_POINT ( 'NONE',  ( 108.0088980509730305, -26.32399177548269620, 151.0041967044829505 ) ) ;
#7392=ORIENTED_EDGE ( 'NONE', *, *, #82329, .F. ) ;
#7393=CARTESIAN_POINT ( 'NONE',  ( 142.8841478025725849, -84.11588139007200482, 542.9756252759101471 ) ) ;
#7394=ORIENTED_EDGE ( 'NONE', *, *, #21957, .T. ) ;
#7396=ORIENTED_EDGE ( 'NONE', *, *, #48538, .T. ) ;
#7397=LINE ( 'NONE', #41447, #47346 ) ;
#7399=ORIENTED_EDGE ( 'NONE', *, *, #80773, .T. ) ;
#7401=ADVANCED_FACE ( 'NONE', ( #45611 ), #66529, .T. ) ;
#7402=CARTESIAN_POINT ( 'NONE',  ( 109.2109342822782168, -45.52796977871753370, 87.17718173283900285 ) ) ;
#7403=CARTESIAN_POINT ( 'NONE',  ( 118.1050840190196567, -32.34957160481850025, 249.1270538473389706 ) ) ;
#7404=CARTESIAN_POINT ( 'NONE',  ( 109.6005296801413351, -26.60309369064632534, 199.8813395616249977 ) ) ;
#7405=CARTESIAN_POINT ( 'NONE',  ( 96.36089708107968477, -41.75325360632972149, 57.67562527591096710 ) ) ;
#7406=CARTESIAN_POINT ( 'NONE',  ( 95.60734603896359829, -36.72944715994100306, 305.0306255462182321 ) ) ;
#7408=CIRCLE ( 'NONE', #21952, 2.517500000000005844 ) ;
#7410=CARTESIAN_POINT ( 'NONE',  ( 116.3212776292278363, -32.94146857470881429, 179.1356252759109395 ) ) ;
#7412=DIRECTION ( 'NONE',  ( -0.1811243269278930978, 0.9834602067165288952, 0.000000000000000000 ) ) ;
#7413=CARTESIAN_POINT ( 'NONE',  ( 107.8912859324307334, -26.39220933555693094, 115.0251490854349612 ) ) ;
#7414=CARTESIAN_POINT ( 'NONE',  ( 98.68712911129445331, -43.00583860492766064, 66.83848241876793850 ) ) ;
#7415=CARTESIAN_POINT ( 'NONE',  ( 97.57529025620152652, -41.14803526195210992, 256.6727681330537507 ) ) ;
#7417=EDGE_CURVE ( 'NONE', #29419, #49604, #85668, .T. ) ;
#7418=CARTESIAN_POINT ( 'NONE',  ( 104.3243669996922307, -26.02151151870134171, 245.2880062282919482 ) ) ;
#7422=LINE ( 'NONE', #14697, #10002 ) ;
#7427=EDGE_CURVE ( 'NONE', #75208, #22872, #16610, .T. ) ;
#7428=AXIS2_PLACEMENT_3D ( 'NONE', #14154, #7341, #516 ) ;
#7430=LINE ( 'NONE', #15602, #66256 ) ;
#7431=EDGE_CURVE ( 'NONE', #3837, #27267, #34243, .T. ) ;
#7432=LINE ( 'NONE', #22870, #17287 ) ;
#7433=CARTESIAN_POINT ( 'NONE',  ( 105.7995184695716802, -26.72403496795282152, 260.1772919440113583 ) ) ;
#7435=ADVANCED_FACE ( 'NONE', ( #48298 ), #41055, .T. ) ;
#7436=FACE_OUTER_BOUND ( 'NONE', #36178, .T. ) ;
#7437=CARTESIAN_POINT ( 'NONE',  ( 111.1360948925329808, -27.10735667079447353, 244.7584824187679544 ) ) ;
#7438=CARTESIAN_POINT ( 'NONE',  ( 109.0722782120600840, -47.59916505968618594, 123.7337205140059666 ) ) ;
#7439=CARTESIAN_POINT ( 'NONE',  ( 105.1596118751612323, -47.03031267540156080, 8.429910990196965770 ) ) ;
#7441=AXIS2_PLACEMENT_3D ( 'NONE', #48341, #13855, #10169 ) ;
#7443=CARTESIAN_POINT ( 'NONE',  ( 81.91948822001464237, -34.69035895457181340, 7.660272404659449919 ) ) ;
#7444=CARTESIAN_POINT ( 'NONE',  ( 116.7951173353165188, -39.38786206668564915, 139.6147893462380409 ) ) ;
#7445=EDGE_CURVE ( 'NONE', #32962, #84043, #7366, .T. ) ;
#7448=VERTEX_POINT ( 'NONE', #41494 ) ;
#7451=CARTESIAN_POINT ( 'NONE',  ( 99.13191293290623207, -41.09468066504173578, 176.1371817328389966 ) ) ;
#7452=FACE_OUTER_BOUND ( 'NONE', #33256, .T. ) ;
#7454=CARTESIAN_POINT ( 'NONE',  ( 51.24204729617298426, -31.76306994223730840, 342.9256252759119548 ) ) ;
#7455=CARTESIAN_POINT ( 'NONE',  ( 118.8928063919343145, -36.92768728534039013, 149.8127681330539644 ) ) ;
#7456=DIRECTION ( 'NONE',  ( 0.7071067811566161820, 0.7071067812164789634, 0.000000000000000000 ) ) ;
#7457=CARTESIAN_POINT ( 'NONE',  ( 172.5664832912740110, 0.2215528400590013880, 76.80862527591200717 ) ) ;
#7459=CARTESIAN_POINT ( 'NONE',  ( 112.9729688188983658, -28.63767724599300735, 85.57429560595268470 ) ) ;
#7462=FACE_OUTER_BOUND ( 'NONE', #34948, .T. ) ;
#7463=CARTESIAN_POINT ( 'NONE',  ( 102.0418483691416469, -28.29933337693050532, 85.50419670448295051 ) ) ;
#7464=VERTEX_POINT ( 'NONE', #54216 ) ;
#7466=AXIS2_PLACEMENT_3D ( 'NONE', #4753, #60137, #67410 ) ;
#7467=ORIENTED_EDGE ( 'NONE', *, *, #48631, .T. ) ;
#7468=CARTESIAN_POINT ( 'NONE',  ( 102.0302726170450711, -29.40150668315268234, 46.98729759161196284 ) ) ;
#7470=CARTESIAN_POINT ( 'NONE',  ( 96.72778144249465981, -35.92320320382071230, 187.2765776568629406 ) ) ;
#7472=DIRECTION ( 'NONE',  ( 0.000000000000000000, 1.000000000000000000, 0.000000000000000000 ) ) ;
#7473=CARTESIAN_POINT ( 'NONE',  ( 131.0667039024480118, -61.87844715994100397, 225.9838068554150254 ) ) ;
#7476=EDGE_CURVE ( 'NONE', #74301, #28950, #103, .T. ) ;
#7478=DIRECTION ( 'NONE',  ( 0.000000000000000000, 0.000000000000000000, -1.000000000000000000 ) ) ;
#7480=CARTESIAN_POINT ( 'NONE',  ( 117.5589153096732105, -33.32758106675089493, 134.0880062282919880 ) ) ;
#7481=ORIENTED_EDGE ( 'NONE', *, *, #39232, .F. ) ;
#7482=ORIENTED_EDGE ( 'NONE', *, *, #50855, .F. ) ;
#7488=EDGE_CURVE ( 'NONE', #58627, #69807, #33804, .T. ) ;
#7489=CARTESIAN_POINT ( 'NONE',  ( 152.0368932755773130, -23.42844715993587812, 129.9678068554149775 ) ) ;
#7491=CARTESIAN_POINT ( 'NONE',  ( 97.93802767643609286, -38.39294625876189571, 199.2880903695909751 ) ) ;
#7492=LINE ( 'NONE', #27923, #62481 ) ;
#7495=EDGE_LOOP ( 'NONE', ( #4885, #24710 ) ) ;
#7497=AXIS2_PLACEMENT_3D ( 'NONE', #39813, #67535, #20737 ) ;
#7498=CARTESIAN_POINT ( 'NONE',  ( 20.56670390244833158, -48.82844715994187368, 249.9678068554150059 ) ) ;
#7499=EDGE_LOOP ( 'NONE', ( #88999, #5162 ) ) ;
#7502=CARTESIAN_POINT ( 'NONE',  ( 110.9273191204289191, -44.70580129652318391, 244.3672975916109635 ) ) ;
#7503=CARTESIAN_POINT ( 'NONE',  ( 118.5256205435843526, -36.72944715994100306, 293.2242906452868851 ) ) ;
#7505=VECTOR ( 'NONE', #9121, 1000.000000000000000 ) ;
#7506=DIRECTION ( 'NONE',  ( -1.000000000000000078E-15, 1.000000000000000083E-30, 1.000000000000000000 ) ) ;
#7508=ORIENTED_EDGE ( 'NONE', *, *, #20968, .T. ) ;
#7509=VERTEX_POINT ( 'NONE', #4761 ) ;
#7510=DIRECTION ( 'NONE',  ( 0.9963424814100663163, -0.08544974978097671925, 0.000000000000000000 ) ) ;
#7513=CARTESIAN_POINT ( 'NONE',  ( 99.62303294566419254, -42.26939103296757594, 259.6538046553056915 ) ) ;
#7514=CARTESIAN_POINT ( 'NONE',  ( 117.2437917682886592, -42.84961121563711828, 128.3956252759109873 ) ) ;
#7515=CARTESIAN_POINT ( 'NONE',  ( 113.9719413768824694, -28.12837331961970122, 119.5261014663869474 ) ) ;
#7517=SURFACE_STYLE_FILL_AREA ( #21608 ) ;
#7518=CARTESIAN_POINT ( 'NONE',  ( 107.2492351517315683, -24.88034519751278850, 226.0641967044829812 ) ) ;
#7519=FACE_OUTER_BOUND ( 'NONE', #57138, .T. ) ;
#7521=ORIENTED_EDGE ( 'NONE', *, *, #25382, .F. ) ;
#7522=CARTESIAN_POINT ( 'NONE',  ( 41.56648329127398966, -27.57844715994070484, 18.92562527591200094 ) ) ;
#7527=CIRCLE ( 'NONE', #58290, 0.5000000000000004441 ) ;
#7528=CARTESIAN_POINT ( 'NONE',  ( 103.2855693325404047, -27.47176340111613513, 136.3850188330253275 ) ) ;
#7530=ORIENTED_EDGE ( 'NONE', *, *, #64647, .T. ) ;
#7531=ADVANCED_FACE ( 'NONE', ( #54662 ), #75142, .T. ) ;
#7532=CARTESIAN_POINT ( 'NONE',  ( 114.0810491752689160, -44.48971597834975000, 133.1613395616249989 ) ) ;
#7533=DIRECTION ( 'NONE',  ( 0.000000000000000000, 0.000000000000000000, 1.000000000000000000 ) ) ;
#7535=DIRECTION ( 'NONE',  ( 1.000000000000000000, 4.163336342344333240E-14, 0.000000000000000000 ) ) ;
#7536=EDGE_CURVE ( 'NONE', #58062, #14741, #61498, .T. ) ;
#7538=CARTESIAN_POINT ( 'NONE',  ( 114.7059021729713919, -43.25973416145915706, 58.26301525237845169 ) ) ;
#7539=CARTESIAN_POINT ( 'NONE',  ( 110.8846227072671979, -27.01418920731900641, 265.7784824187680783 ) ) ;
#7542=ORIENTED_EDGE ( 'NONE', *, *, #47527, .T. ) ;
#7544=DIRECTION ( 'NONE',  ( -1.000000000000000000, 0.000000000000000000, 2.820351377559424413E-14 ) ) ;
#7549=EDGE_CURVE ( 'NONE', #89358, #54421, #88786, .T. ) ;
#7551=CARTESIAN_POINT ( 'NONE',  ( 96.87130625142565066, -34.19761792387945576, 276.1327681330536734 ) ) ;
#7554=LINE ( 'NONE', #83866, #58229 ) ;
#7555=CARTESIAN_POINT ( 'NONE',  ( 102.3026241189005532, -26.72939285866361914, 140.4422919425769578 ) ) ;
#7556=CARTESIAN_POINT ( 'NONE',  ( 109.6429888323185224, -46.83113546657025950, 43.77562527591094721 ) ) ;
#7557=CARTESIAN_POINT ( 'NONE',  ( 108.2828737166157964, -47.76209090725709672, 153.6518157521009584 ) ) ;
#7559=CARTESIAN_POINT ( 'NONE',  ( 97.81169951533574647, -40.51743117454552134, 102.6356342116286413 ) ) ;
#7561=DIRECTION ( 'NONE',  ( 0.7071067811861589947, -0.7071067811869361508, 0.000000000000000000 ) ) ;
#7562=DIRECTION ( 'NONE',  ( 0.000000000000000000, 1.000000000000000000, 0.000000000000000000 ) ) ;
#7563=DIRECTION ( 'NONE',  ( 0.000000000000000000, 1.000000000000000000, 0.000000000000000000 ) ) ;
#7565=ADVANCED_FACE ( 'NONE', ( #26543 ), #46502, .F. ) ;
#7566=CARTESIAN_POINT ( 'NONE',  ( 72.06648329127401098, -45.72944715994106701, 14.67562527591093513 ) ) ;
#7567=ADVANCED_FACE ( 'NONE', ( #60145 ), #87880, .F. ) ;
#7568=ORIENTED_EDGE ( 'NONE', *, *, #59083, .F. ) ;
#7569=EDGE_LOOP ( 'NONE', ( #81110, #73297 ) ) ;
#7571=CARTESIAN_POINT ( 'NONE',  ( 110.3472192523918238, -25.36789009815987228, 60.85276813305395649 ) ) ;
#7572=LINE ( 'NONE', #83888, #41115 ) ;
#7574=LINE ( 'NONE', #70695, #67441 ) ;
#7575=CARTESIAN_POINT ( 'NONE',  ( 116.8472425118689841, -43.50793233799721094, 159.3441967044829539 ) ) ;
#7577=CARTESIAN_POINT ( 'NONE',  ( 99.27767200979357654, -42.52643314540505060, 261.2581341137909590 ) ) ;
#7578=ORIENTED_EDGE ( 'NONE', *, *, #75886, .F. ) ;
#7579=VERTEX_POINT ( 'NONE', #178 ) ;
#7581=AXIS2_PLACEMENT_3D ( 'NONE', #23924, #52902, #52032 ) ;
#7582=ORIENTED_EDGE ( 'NONE', *, *, #69182, .T. ) ;
#7584=CARTESIAN_POINT ( 'NONE',  ( 162.5667039024476139, -32.29483332967974718, 313.9678068554149490 ) ) ;
#7585=CARTESIAN_POINT ( 'NONE',  ( 116.3183303039212291, -32.94226276200836878, 104.1356252759109680 ) ) ;
#7586=DIRECTION ( 'NONE',  ( 0.000000000000000000, 0.000000000000000000, -1.000000000000000000 ) ) ;
#7589=CARTESIAN_POINT ( 'NONE',  ( 156.5667039024483529, -42.82844715993568485, 134.7178068554149775 ) ) ;
#7590=CARTESIAN_POINT ( 'NONE',  ( 50.56670390244699576, -18.82844715994031048, -5.074374724088000832 ) ) ;
#7591=CARTESIAN_POINT ( 'NONE',  ( 101.6204011159889831, -47.22657592904994317, 17.19562527591095247 ) ) ;
#7592=CARTESIAN_POINT ( 'NONE',  ( 34.67381068360400320, -28.98061976758901892, -5.074374724088000832 ) ) ;
#7597=EDGE_CURVE ( 'NONE', #35491, #78335, #53754, .T. ) ;
#7598=DIRECTION ( 'NONE',  ( 0.000000000000000000, -1.000000000000000000, 0.000000000000000000 ) ) ;
#7599=CARTESIAN_POINT ( 'NONE',  ( 98.91570299145236334, -37.17047609451836365, 74.18809036959095238 ) ) ;
#7603=PLANE ( 'NONE',  #16947 ) ;
#7604=EDGE_LOOP ( 'NONE', ( #54535, #24412, #47241, #75658 ) ) ;
#7605=ORIENTED_EDGE ( 'NONE', *, *, #59367, .F. ) ;
#7606=CARTESIAN_POINT ( 'NONE',  ( 77.71552635664649245, -35.29868341350233862, 7.242354772874388225 ) ) ;
#7607=VERTEX_POINT ( 'NONE', #21988 ) ;
#7608=ORIENTED_EDGE ( 'NONE', *, *, #45954, .F. ) ;
#7609=LINE ( 'NONE', #6261, #43118 ) ;
#7610=CARTESIAN_POINT ( 'NONE',  ( 97.38361328163530573, -33.95226689236985607, 137.5358690201829575 ) ) ;
#7611=LINE ( 'NONE', #28039, #60528 ) ;
#7612=CARTESIAN_POINT ( 'NONE',  ( 98.18387371117843543, -43.34642931133835475, 107.8480062282919647 ) ) ;
#7613=CARTESIAN_POINT ( 'NONE',  ( 142.8841478025725849, -84.11588139007200482, 540.9756252759101471 ) ) ;
#7614=ORIENTED_EDGE ( 'NONE', *, *, #58904, .T. ) ;
#7615=CARTESIAN_POINT ( 'NONE',  ( 92.55667057654251551, -29.98664840991042269, 9.125625275910955736 ) ) ;
#7616=VERTEX_POINT ( 'NONE', #15615 ) ;
#7618=VECTOR ( 'NONE', #29464, 1000.000000000000000 ) ;
#7619=FACE_BOUND ( 'NONE', #67240, .T. ) ;
#7620=VERTEX_POINT ( 'NONE', #62843 ) ;
#7621=CARTESIAN_POINT ( 'NONE',  ( 100.6111884388666766, -28.52632756463403751, 15.60705384733995871 ) ) ;
#7622=CARTESIAN_POINT ( 'NONE',  ( 107.5668116379858787, -47.79447663526521239, 188.6003871806729535 ) ) ;
#7625=CARTESIAN_POINT ( 'NONE',  ( 96.02365317015762969, -37.20890873343472549, 112.3489586092449599 ) ) ;
#7627=EDGE_LOOP ( 'NONE', ( #78906, #19146, #10783, #85873 ) ) ;
#7628=LINE ( 'NONE', #36228, #6115 ) ;
#7629=LINE ( 'NONE', #57556, #37533 ) ;
#7630=EDGE_CURVE ( 'NONE', #10930, #17773, #11553, .T. ) ;
#7635=CARTESIAN_POINT ( 'NONE',  ( 99.14341341762981585, -43.50528616620496791, 31.88991099019594699 ) ) ;
#7638=DIRECTION ( 'NONE',  ( 0.000000000000000000, 0.000000000000000000, -1.000000000000000000 ) ) ;
#7639=CARTESIAN_POINT ( 'NONE',  ( 156.5667039024483245, -42.82844715993568485, 173.2178068554149775 ) ) ;
#7640=ADVANCED_FACE ( 'NONE', ( #57369 ), #49204, .F. ) ;
#7641=CARTESIAN_POINT ( 'NONE',  ( 98.46141696562543189, -39.55439615822902510, 286.0133722090292849 ) ) ;
#7642=CARTESIAN_POINT ( 'NONE',  ( 99.09540760583590213, -30.55081426086826113, 110.8023302363145461 ) ) ;
#7643=CARTESIAN_POINT ( 'NONE',  ( 113.3016265961369697, -28.35762455946455773, 100.5670538473389684 ) ) ;
#7645=CARTESIAN_POINT ( 'NONE',  ( 108.4336792877692517, -20.78796745737986740, 293.6356252759109680 ) ) ;
#7649=FACE_BOUND ( 'NONE', #22946, .T. ) ;
#7651=EDGE_LOOP ( 'NONE', ( #4839, #67483, #36780, #19790 ) ) ;
#7654=CARTESIAN_POINT ( 'NONE',  ( 117.8245512228195224, -33.99506276729055543, 169.0365776568629599 ) ) ;
#7655=VERTEX_POINT ( 'NONE', #620 ) ;
#7656=CARTESIAN_POINT ( 'NONE',  ( 162.7866693523289996, -36.02818131005891189, -5.074374724088000832 ) ) ;
#7657=CARTESIAN_POINT ( 'NONE',  ( 117.2182995153958132, -34.26411022451439692, 205.0156252759109634 ) ) ;
#7658=CARTESIAN_POINT ( 'NONE',  ( 96.14773132834588409, -38.72402830165600562, 47.48229194257797303 ) ) ;
#7659=DIRECTION ( 'NONE',  ( 4.012088370409549976E-14, -1.000000000000000000, 0.000000000000000000 ) ) ;
#7660=DIRECTION ( 'NONE',  ( 1.000000000000000078E-15, 0.000000000000000000, -1.000000000000000000 ) ) ;
#7661=CARTESIAN_POINT ( 'NONE',  ( 109.6430121383572072, -46.48008673305788108, 77.78145860988261973 ) ) ;
#7662=VERTEX_POINT ( 'NONE', #79187 ) ;
#7663=EDGE_CURVE ( 'NONE', #48540, #38670, #5886, .T. ) ;
#7666=ADVANCED_FACE ( 'NONE', ( #37386 ), #79627, .F. ) ;
#7667=ORIENTED_EDGE ( 'NONE', *, *, #29206, .F. ) ;
#7669=FACE_OUTER_BOUND ( 'NONE', #27591, .T. ) ;
#7670=CARTESIAN_POINT ( 'NONE',  ( 99.53941477645811631, -29.46552450412116997, 246.7156252759109520 ) ) ;
#7672=CARTESIAN_POINT ( 'NONE',  ( 50.88849390559378350, -32.11662333284569115, 117.4678068554150485 ) ) ;
#7673=EDGE_CURVE ( 'NONE', #37315, #18895, #19107, .T. ) ;
#7674=DIRECTION ( 'NONE',  ( -0.7071067811567173234, 0.7071067812163779331, 0.000000000000000000 ) ) ;
#7676=CARTESIAN_POINT ( 'NONE',  ( 31.46648329127298993, 12.92155284005730387, 361.9756252759109998 ) ) ;
#7677=CARTESIAN_POINT ( 'NONE',  ( 111.0547186471684995, -47.06334559972322751, 17.85753003781598380 ) ) ;
#7678=VERTEX_POINT ( 'NONE', #2425 ) ;
#7679=ORIENTED_EDGE ( 'NONE', *, *, #25926, .F. ) ;
#7680=LINE ( 'NONE', #8588, #52810 ) ;
#7682=CARTESIAN_POINT ( 'NONE',  ( 112.0813997088635432, -45.80630777137064058, 248.9661014663869878 ) ) ;
#7683=DIRECTION ( 'NONE',  ( 1.000000000000000078E-15, -1.000000000000000083E-30, -1.000000000000000000 ) ) ;
#7684=VECTOR ( 'NONE', #4774, 1000.000000000000000 ) ;
#7685=CARTESIAN_POINT ( 'NONE',  ( 104.3903674582245742, -25.93822912171390982, 86.26991099019598153 ) ) ;
#7686=CARTESIAN_POINT ( 'NONE',  ( 99.04393567086002292, -42.84106820361873247, 31.84416257778224946 ) ) ;
#7687=CARTESIAN_POINT ( 'NONE',  ( 103.2776430504499388, -27.47500554358347813, 21.38570024634822886 ) ) ;
#7690=B_SPLINE_CURVE_WITH_KNOTS ( 'NONE', 3,
 ( #45426, #15974, #2343, #73143, #10926, #43654, #19082, #11828, #54468, #60858, #67227, #4114, #53116, #74948, #26349, #33609, #61306, #5465, #89025, #59508, #26783, #46766, #88143, #45867, #18185, #25450, #19987 ),
 .UNSPECIFIED., .F., .F.,
 ( 4, 2, 2, 2, 2, 2, 2, 2, 2, 2, 1, 1, 1, 2, 4 ),
 ( 0.000000000000000000, 0.06251142263352413297, 0.1250228452670482659, 0.1875342679005723989, 0.2500456905340965319, 0.3125571131676206371, 0.3750685358011447978, 0.4375799584346689031, 0.4688356697514310945, 0.4844635254098123567, 0.4922774532390031266, 0.4961844171535987891, 0.4981378991108966203, 0.4991146400895454804, 0.5000913810681943961 ),
 .UNSPECIFIED. ) ;
#7691=ORIENTED_EDGE ( 'NONE', *, *, #66765, .F. ) ;
#7692=ORIENTED_EDGE ( 'NONE', *, *, #7597, .F. ) ;
#7693=EDGE_CURVE ( 'NONE', #67525, #4530, #4452, .T. ) ;
#7695=CARTESIAN_POINT ( 'NONE',  ( 114.6260888371869555, -31.15012018194425281, 255.7520594963732492 ) ) ;
#7697=CARTESIAN_POINT ( 'NONE',  ( 115.0372574805542740, -42.90846260123733913, 193.3022919391792698 ) ) ;
#7698=CARTESIAN_POINT ( 'NONE',  ( 25.56670390244797275, -65.37844715994100397, 173.2178068554149775 ) ) ;
#7703=CARTESIAN_POINT ( 'NONE',  ( 109.6412978090997967, -46.48051820152372215, 183.7818762376771247 ) ) ;
#7705=CARTESIAN_POINT ( 'NONE',  ( 112.8178475080015772, -27.29012000701139939, 49.62895860924498947 ) ) ;
#7706=ORIENTED_EDGE ( 'NONE', *, *, #13742, .T. ) ;
#7707=CARTESIAN_POINT ( 'NONE',  ( 98.56427472769081533, -33.61093641167653345, 20.45718173283900398 ) ) ;
#7708=CARTESIAN_POINT ( 'NONE',  ( 172.5664832912729878, -27.82844715994070484, 198.9256252759119832 ) ) ;
#7709=CARTESIAN_POINT ( 'NONE',  ( 108.5755967597531821, -27.06580334247533770, 189.9527681330539792 ) ) ;
#7710=ADVANCED_FACE ( 'NONE', ( #44179 ), #9674, .F. ) ;
#7712=DIRECTION ( 'NONE',  ( 1.000000000000000000, 4.163336342344333240E-14, 0.000000000000000000 ) ) ;
#7713=CARTESIAN_POINT ( 'NONE',  ( 142.8679068202682458, 10.65431904611001634, 396.9756252759102040 ) ) ;
#7715=CARTESIAN_POINT ( 'NONE',  ( 116.2568870038579547, -41.81614494787783798, 259.4241967044827106 ) ) ;
#7716=CARTESIAN_POINT ( 'NONE',  ( 99.36242816078741669, -43.15851294862928711, 116.8811511109068562 ) ) ;
#7717=ORIENTED_EDGE ( 'NONE', *, *, #78008, .F. ) ;
#7719=ADVANCED_FACE ( 'NONE', ( #52308 ), #16945, .T. ) ;
#7720=CARTESIAN_POINT ( 'NONE',  ( 154.4532655810166091, -72.54279768053238797, 396.9756252759102040 ) ) ;
#7721=VERTEX_POINT ( 'NONE', #72359 ) ;
#7722=CARTESIAN_POINT ( 'NONE',  ( 98.29982688861167617, -42.45122269429050021, 97.78705384733993355 ) ) ;
#7724=CIRCLE ( 'NONE', #26582, 2.030000000001311644 ) ;
#7725=ORIENTED_EDGE ( 'NONE', *, *, #42991, .F. ) ;
#7726=LINE ( 'NONE', #79353, #73386 ) ;
#7727=ORIENTED_EDGE ( 'NONE', *, *, #64673, .T. ) ;
#7729=AXIS2_PLACEMENT_3D ( 'NONE', #59864, #53026, #67142 ) ;
#7734=DIRECTION ( 'NONE',  ( 0.000000000000000000, 0.000000000000000000, 1.000000000000000000 ) ) ;
#7735=CARTESIAN_POINT ( 'NONE',  ( 109.9953477121747767, -26.70153551007575388, 255.8499109901966051 ) ) ;
#7740=ORIENTED_EDGE ( 'NONE', *, *, #23144, .T. ) ;
#7741=VERTEX_POINT ( 'NONE', #10126 ) ;
#7742=CARTESIAN_POINT ( 'NONE',  ( 82.61444500289061921, -19.76411817600001442, 2.828498113172249528 ) ) ;
#7743=AXIS2_PLACEMENT_3D ( 'NONE', #40152, #45176, #46957 ) ;
#7744=FACE_OUTER_BOUND ( 'NONE', #86214, .T. ) ;
#7745=CARTESIAN_POINT ( 'NONE',  ( 97.80400251452438454, -40.49860548021092654, 16.63400711711531699 ) ) ;
#7746=ADVANCED_FACE ( 'NONE', ( #31444 ), #45502, .T. ) ;
#7747=DIRECTION ( 'NONE',  ( 0.000000000000000000, 0.000000000000000000, 1.000000000000000000 ) ) ;
#7748=CARTESIAN_POINT ( 'NONE',  ( 34.67381068360400320, -28.98061976758901892, -5.074374724088000832 ) ) ;
#7749=EDGE_CURVE ( 'NONE', #44764, #75304, #38707, .T. ) ;
#7750=CARTESIAN_POINT ( 'NONE',  ( 102.3821975904229333, -44.47993990548584975, 201.5543245899819738 ) ) ;
#7752=CARTESIAN_POINT ( 'NONE',  ( 99.46959489307312197, -43.93319290153426238, 81.92991099019597812 ) ) ;
#7753=ORIENTED_EDGE ( 'NONE', *, *, #14720, .T. ) ;
#7754=CARTESIAN_POINT ( 'NONE',  ( 37.56670390244722313, -48.82844715994106366, 180.4678068554150911 ) ) ;
#7757=ADVANCED_FACE ( 'NONE', ( #60487 ), #6007, .F. ) ;
#7758=CARTESIAN_POINT ( 'NONE',  ( 34.27482367531500529, -30.08671355700301575, -5.074374724088000832 ) ) ;
#7759=ORIENTED_EDGE ( 'NONE', *, *, #54168, .F. ) ;
#7762=ORIENTED_EDGE ( 'NONE', *, *, #58424, .F. ) ;
#7764=DIRECTION ( 'NONE',  ( 1.000000000000000078E-15, -1.000000000000000000, 0.000000000000000000 ) ) ;
#7766=AXIS2_PLACEMENT_3D ( 'NONE', #81248, #18092, #80792 ) ;
#7768=ORIENTED_EDGE ( 'NONE', *, *, #73671, .T. ) ;
#7769=CARTESIAN_POINT ( 'NONE',  ( 103.5913855974186362, -46.58186107657011377, 57.30705384733997221 ) ) ;
#7771=CARTESIAN_POINT ( 'NONE',  ( 107.0667039024479834, -48.82844715994099971, 160.9178068554150229 ) ) ;
#7773=FACE_OUTER_BOUND ( 'NONE', #68488, .T. ) ;
#7774=CARTESIAN_POINT ( 'NONE',  ( 133.3151098752327925, -16.05633243510672159, 1.690787911849395364 ) ) ;
#7777=DIRECTION ( 'NONE',  ( 1.000000000000000078E-15, -1.000000000000000083E-30, -1.000000000000000000 ) ) ;
#7778=CARTESIAN_POINT ( 'NONE',  ( 116.3162492855249894, -32.94856389518969308, 154.1356252759109680 ) ) ;
#7780=CARTESIAN_POINT ( 'NONE',  ( 96.00057345886969529, -37.20991081664785582, 112.3489586092449599 ) ) ;
#7781=DIRECTION ( 'NONE',  ( -0.7071067811865462405, 0.000000000000000000, 0.7071067811865486830 ) ) ;
#7782=CARTESIAN_POINT ( 'NONE',  ( 172.5664832912729878, -18.82844715994071194, 138.9256252759119832 ) ) ;
#7785=EDGE_LOOP ( 'NONE', ( #7679, #59910, #42118, #48186 ) ) ;
#7786=TOROIDAL_SURFACE ( 'NONE', #13553, 11.75000000000000000, 2.125000000000000000 ) ;
#7788=CARTESIAN_POINT ( 'NONE',  ( 98.32242264099485851, -42.30440888850449710, 137.7661014663869992 ) ) ;
#7789=DIRECTION ( 'NONE',  ( 0.000000000000000000, 0.000000000000000000, -1.000000000000000000 ) ) ;
#7791=CARTESIAN_POINT ( 'NONE',  ( 96.55902551080276908, -40.08462249002850086, 277.5603871806729899 ) ) ;
#7795=CARTESIAN_POINT ( 'NONE',  ( 180.1667039024476082, -26.71338133338667120, 193.9678068554150059 ) ) ;
#7796=CARTESIAN_POINT ( 'NONE',  ( 31.78666935232975987, -36.02818131005922453, 313.9678068554150059 ) ) ;
#7797=CYLINDRICAL_SURFACE ( 'NONE', #61656, 9.999999999999998224 ) ;
#7798=CARTESIAN_POINT ( 'NONE',  ( 107.2322476904469966, -46.54200526979099095, 212.5899109901969837 ) ) ;
#7800=VERTEX_POINT ( 'NONE', #67768 ) ;
#7801=ADVANCED_FACE ( 'NONE', ( #4648 ), #33249, .T. ) ;
#7802=CARTESIAN_POINT ( 'NONE',  ( 108.0961452412413166, -46.06846630830715128, 154.0834880678019374 ) ) ;
#7804=CARTESIAN_POINT ( 'NONE',  ( 115.0635112019030686, -32.91162553226137533, 15.61301187732594364 ) ) ;
#7806=CARTESIAN_POINT ( 'NONE',  ( 59.67079009362632291, -0.9310397146383332379, 542.9756252759101471 ) ) ;
#7810=CIRCLE ( 'NONE', #541, 10.00000000000000888 ) ;
#7812=CARTESIAN_POINT ( 'NONE',  ( 31.56670390244700641, -19.82844715994111340, 342.9256252759119548 ) ) ;
#7813=CARTESIAN_POINT ( 'NONE',  ( 118.0279888096068390, -35.50094427011355691, 233.9032443235299752 ) ) ;
#7814=CARTESIAN_POINT ( 'NONE',  ( 123.0664832912757163, -36.72944715993921960, -5.074374724089014244 ) ) ;
#7815=ORIENTED_EDGE ( 'NONE', *, *, #81938, .T. ) ;
#7816=ORIENTED_EDGE ( 'NONE', *, *, #69676, .T. ) ;
#7819=CARTESIAN_POINT ( 'NONE',  ( 97.83871787020589750, -40.58289724771079676, 122.6407992083991587 ) ) ;
#7820=CARTESIAN_POINT ( 'NONE',  ( 151.0371591254575208, -24.42818131005592264, 193.9678068554149775 ) ) ;
#7821=CARTESIAN_POINT ( 'NONE',  ( 100.4186822966650539, -43.90371905523895890, 42.98133956162492098 ) ) ;
#7822=FACE_OUTER_BOUND ( 'NONE', #3521, .T. ) ;
#7826=CARTESIAN_POINT ( 'NONE',  ( 99.53925745938779812, -29.46537268684611632, 250.7156252759109520 ) ) ;
#7828=CARTESIAN_POINT ( 'NONE',  ( 77.37801896924342770, -37.30949827216422676, 6.839365140900691031 ) ) ;
#7829=DIRECTION ( 'NONE',  ( -0.04216478779797398074, 0.9991106698809455455, 0.000000000000000000 ) ) ;
#7831=CARTESIAN_POINT ( 'NONE',  ( 104.6321197217979488, -45.03455396584281800, 60.15570941721099274 ) ) ;
#7832=CARTESIAN_POINT ( 'NONE',  ( 107.6542194910912684, -47.14941140656445384, 148.6213395616249784 ) ) ;
#7833=ORIENTED_CLOSED_SHELL ( 'NONE', *, #2450, .F. );
#7838=ORIENTED_EDGE ( 'NONE', *, *, #34373, .F. ) ;
#7839=AXIS2_PLACEMENT_3D ( 'NONE', #67861, #26528, #35570 ) ;
#7841=VERTEX_POINT ( 'NONE', #80974 ) ;
#7844=AXIS2_PLACEMENT_3D ( 'NONE', #81164, #41904, #28748 ) ;
#7845=LINE ( 'NONE', #53388, #88137 ) ;
#7846=EDGE_CURVE ( 'NONE', #20236, #60890, #4519, .T. ) ;
#7847=CARTESIAN_POINT ( 'NONE',  ( 99.00375160886646597, -32.60573182744733600, 95.38480078045697041 ) ) ;
#7848=CARTESIAN_POINT ( 'NONE',  ( 100.1240125862563275, -44.53639691489608765, 266.9984824187678782 ) ) ;
#7849=CARTESIAN_POINT ( 'NONE',  ( 117.9098725419245000, -34.70837513311212064, 203.9851490854349549 ) ) ;
#7850=FACE_OUTER_BOUND ( 'NONE', #83657, .T. ) ;
#7851=CARTESIAN_POINT ( 'NONE',  ( 113.1758862902701850, -44.75366746424991504, 94.09372177059972842 ) ) ;
#7853=ORIENTED_EDGE ( 'NONE', *, *, #40241, .T. ) ;
#7857=CARTESIAN_POINT ( 'NONE',  ( 98.20106483660278229, -31.34956418181668880, 125.8803871806729546 ) ) ;
#7858=CARTESIAN_POINT ( 'NONE',  ( 110.8102856614596021, -46.50649220725635757, 62.86705384733992474 ) ) ;
#7859=CARTESIAN_POINT ( 'NONE',  ( 96.76538361991065074, -40.86468949728195099, 251.6422919425776001 ) ) ;
#7860=AXIS2_PLACEMENT_3D ( 'NONE', #83022, #42987, #83453 ) ;
#7861=VERTEX_POINT ( 'NONE', #26438 ) ;
#7862=CARTESIAN_POINT ( 'NONE',  ( 116.0552987087602048, -42.01037774571695849, 238.4041967044829562 ) ) ;
#7864=LINE ( 'NONE', #78277, #34134 ) ;
#7865=AXIS2_PLACEMENT_3D ( 'NONE', #14892, #89858, #33964 ) ;
#7868=DIRECTION ( 'NONE',  ( 0.000000000000000000, 0.000000000000000000, -1.000000000000000000 ) ) ;
#7872=DIRECTION ( 'NONE',  ( 0.000000000000000000, 0.000000000000000000, -1.000000000000000000 ) ) ;
#7874=CARTESIAN_POINT ( 'NONE',  ( 51.03742451361310373, -23.42844715994068849, 193.9678068554150911 ) ) ;
#7878=EDGE_CURVE ( 'NONE', #47474, #22206, #68226, .T. ) ;
#7879=CARTESIAN_POINT ( 'NONE',  ( 109.7248659022256732, -27.00080517415949188, 10.86479194411551852 ) ) ;
#7882=ORIENTED_EDGE ( 'NONE', *, *, #78459, .T. ) ;
#7883=DIRECTION ( 'NONE',  ( 1.000000000000000000, 3.999999999999999995E-14, 1.000000000000000078E-15 ) ) ;
#7884=CARTESIAN_POINT ( 'NONE',  ( 110.8247753047693749, -26.30972152642112150, 249.7889586092445882 ) ) ;
#7885=CARTESIAN_POINT ( 'NONE',  ( 98.45631125714150755, -42.66967193002393088, 122.8070538473389490 ) ) ;
#7886=CARTESIAN_POINT ( 'NONE',  ( 96.32186211137589282, -39.41937243639647903, 12.53372051400597442 ) ) ;
#7887=DIRECTION ( 'NONE',  ( 1.327617956749546798E-15, -0.7071067811865555663, -0.7071067811865394681 ) ) ;
#7888=DIRECTION ( 'NONE',  ( 1.000000000000000000, 4.299999999999999979E-14, 1.000000000000000078E-15 ) ) ;
#7893=ORIENTED_EDGE ( 'NONE', *, *, #57603, .F. ) ;
#7894=CARTESIAN_POINT ( 'NONE',  ( 100.1837753934783990, -31.62254652264567767, 180.2409912566479591 ) ) ;
#7898=CARTESIAN_POINT ( 'NONE',  ( 102.9221092647374149, -27.14930527916913050, 151.4013395616249511 ) ) ;
#7899=CARTESIAN_POINT ( 'NONE',  ( 116.3159136950847170, -32.94903743517052419, 150.1356252759109680 ) ) ;
#7900=CARTESIAN_POINT ( 'NONE',  ( 41.56670390244718050, -42.82844715994109208, 180.4678068554150911 ) ) ;
#7903=CARTESIAN_POINT ( 'NONE',  ( 107.0667039024479834, -36.72944715994100306, 239.5838068554170093 ) ) ;
#7905=CARTESIAN_POINT ( 'NONE',  ( 103.5129713284349720, -46.47169217660404428, 97.28610146638794731 ) ) ;
#7906=ORIENTED_EDGE ( 'NONE', *, *, #78989, .F. ) ;
#7907=ORIENTED_EDGE ( 'NONE', *, *, #35199, .F. ) ;
#7910=CARTESIAN_POINT ( 'NONE',  ( 97.81060075337646254, -38.34349919808700236, 42.88348806780201272 ) ) ;
#7912=CARTESIAN_POINT ( 'NONE',  ( 98.02110346605356028, -41.80092515478911963, 177.7451490854339795 ) ) ;
#7915=CARTESIAN_POINT ( 'NONE',  ( 163.0667039024468465, -32.29483332967940612, 193.9678068554149775 ) ) ;
#7916=CYLINDRICAL_SURFACE ( 'NONE', #48017, 2.500000000000002220 ) ;
#7919=CARTESIAN_POINT ( 'NONE',  ( 107.0664832912739541, -23.72944715994095688, 311.6343304127839815 ) ) ;
#7921=CARTESIAN_POINT ( 'NONE',  ( 113.9719413768824694, -28.12837331961970122, 119.5261014663869474 ) ) ;
#7923=VERTEX_POINT ( 'NONE', #6436 ) ;
#7927=CARTESIAN_POINT ( 'NONE',  ( 97.75843501427306137, -40.38501350233762821, 131.6242676007061903 ) ) ;
#7928=CARTESIAN_POINT ( 'NONE',  ( 62.03742497533751532, -23.42844715994041849, 249.9678068554150343 ) ) ;
#7929=CARTESIAN_POINT ( 'NONE',  ( 113.1326720373799617, -31.22635327163875374, 207.2309475124489495 ) ) ;
#7932=DIRECTION ( 'NONE',  ( 0.7071067811865466846, -0.7071067811865483499, 7.071067811865460542E-16 ) ) ;
#7933=VECTOR ( 'NONE', #18061, 1000.000000000000000 ) ;
#7935=LINE ( 'NONE', #71078, #28610 ) ;
#7939=CIRCLE ( 'NONE', #80504, 13.99999999999999822 ) ;
#7943=EDGE_LOOP ( 'NONE', ( #54308, #70249, #16013, #33847 ) ) ;
#7944=CARTESIAN_POINT ( 'NONE',  ( 78.24498361945106240, -20.78962918510159952, 7.677444906559778737 ) ) ;
#7945=CARTESIAN_POINT ( 'NONE',  ( 112.7895289397446561, -28.43984804668171051, 236.0272975916119549 ) ) ;
#7946=EDGE_CURVE ( 'NONE', #88413, #88172, #88235, .T. ) ;
#7947=CARTESIAN_POINT ( 'NONE',  ( 100.8874669139039355, -44.70022063263273537, 272.0522918462373241 ) ) ;
#7948=ORIENTED_EDGE ( 'NONE', *, *, #75934, .T. ) ;
#7949=CARTESIAN_POINT ( 'NONE',  ( 134.0664832912740110, -36.72944715994100306, -5.074374724089001809 ) ) ;
#7951=ORIENTED_EDGE ( 'NONE', *, *, #3074, .T. ) ;
#7952=EDGE_LOOP ( 'NONE', ( #65165, #34982, #21396 ) ) ;
#7954=ORIENTED_EDGE ( 'NONE', *, *, #72453, .T. ) ;
#7957=AXIS2_PLACEMENT_3D ( 'NONE', #75575, #53742, #61030 ) ;
#7958=CARTESIAN_POINT ( 'NONE',  ( 113.8227294809096435, -41.31015272151215356, 271.1709475124484925 ) ) ;
#7959=CARTESIAN_POINT ( 'NONE',  ( 102.6066768796756037, -46.86875521856975269, 132.2346728949579528 ) ) ;
#7960=CARTESIAN_POINT ( 'NONE',  ( 117.3497117099304745, -32.73958051198272301, 94.10895860924395606 ) ) ;
#7961=DIRECTION ( 'NONE',  ( -1.000000000000000000, -3.999999999999999995E-14, -1.000000000000000078E-15 ) ) ;
#7962=SURFACE_SIDE_STYLE ('',( #7517 ) ) ;
#7963=CARTESIAN_POINT ( 'NONE',  ( 112.4543492094282726, -45.69561878580546477, 234.0070538473389377 ) ) ;
#7964=PLANE ( 'NONE',  #39959 ) ;
#7965=EDGE_CURVE ( 'NONE', #80800, #50606, #32794, .T. ) ;
#7967=ORIENTED_EDGE ( 'NONE', *, *, #71001, .T. ) ;
#7968=CARTESIAN_POINT ( 'NONE',  ( 46.48091746482041486, -48.32844715994088602, 180.4678068554150911 ) ) ;
#7969=ORIENTED_EDGE ( 'NONE', *, *, #74224, .T. ) ;
#7970=ORIENTED_EDGE ( 'NONE', *, *, #78837, .T. ) ;
#7972=CIRCLE ( 'NONE', #84826, 3.000000000000002665 ) ;
#7973=CARTESIAN_POINT ( 'NONE',  ( 50.56670390244699576, -18.82844715994031048, 342.9256252759119548 ) ) ;
#7974=ORIENTED_EDGE ( 'NONE', *, *, #45300, .F. ) ;
#7975=CARTESIAN_POINT ( 'NONE',  ( 109.0723201335305816, -47.59939223872296310, 127.7337205140059382 ) ) ;
#7976=LINE ( 'NONE', #50645, #86287 ) ;
#7981=CARTESIAN_POINT ( 'NONE',  ( 107.8260946937819398, -46.73210543769128833, 57.63636942760201265 ) ) ;
#7982=CARTESIAN_POINT ( 'NONE',  ( 97.19046783542286505, -39.99946004141659017, 237.5813395616249579 ) ) ;
#7983=CARTESIAN_POINT ( 'NONE',  ( 106.6093434278972865, -26.33948225654953035, 321.1698005525342978 ) ) ;
#7984=DIRECTION ( 'NONE',  ( 0.7071067811578790607, 0.7071067812152160847, 0.000000000000000000 ) ) ;
#7985=CARTESIAN_POINT ( 'NONE',  ( 107.0664832912739541, -20.72944715994095333, 302.7856252759109452 ) ) ;
#7986=EDGE_CURVE ( 'NONE', #82149, #45331, #69119, .T. ) ;
#7987=FACE_OUTER_BOUND ( 'NONE', #48562, .T. ) ;
#7989=DIRECTION ( 'NONE',  ( 0.000000000000000000, -1.000000000000000000, 0.000000000000000000 ) ) ;
#7990=ADVANCED_FACE ( 'NONE', ( #14608 ), #56696, .F. ) ;
#7991=DIRECTION ( 'NONE',  ( -0.7071067811865453523, -0.7071067811865496822, -7.071067811865460542E-16 ) ) ;
#7992=CARTESIAN_POINT ( 'NONE',  ( 97.17500156396280886, -33.29969143728342829, 286.0613395616251751 ) ) ;
#7995=CARTESIAN_POINT ( 'NONE',  ( 117.2597117638302393, -39.02229875088008981, 148.6499109901969859 ) ) ;
#7996=CARTESIAN_POINT ( 'NONE',  ( 112.7416762643710229, -27.24439759747685486, 50.65943479972101215 ) ) ;
#7997=CARTESIAN_POINT ( 'NONE',  ( 96.00793635059680753, -35.77758691827158799, 182.2461014663869889 ) ) ;
#7999=CARTESIAN_POINT ( 'NONE',  ( 98.34985881564388421, -31.65658497315240183, 31.90645862423135881 ) ) ;
#8000=DIRECTION ( 'NONE',  ( 1.000000000000000000, 4.163336342344333240E-14, 0.000000000000000000 ) ) ;
#8001=DIRECTION ( 'NONE',  ( -1.000000000000000000, 0.000000000000000000, 0.000000000000000000 ) ) ;
#8002=DIRECTION ( 'NONE',  ( 1.387778780781444492E-15, 0.000000000000000000, -1.000000000000000000 ) ) ;
#8003=DIRECTION ( 'NONE',  ( -0.9999999853157766072, -0.0001713722456150811827, 0.000000000000000000 ) ) ;
#8006=CARTESIAN_POINT ( 'NONE',  ( 128.0667039024480118, -58.72944715994110254, 10.91780685541499807 ) ) ;
#8007=AXIS2_PLACEMENT_3D ( 'NONE', #52766, #74597, #81442 ) ;
#8008=VECTOR ( 'NONE', #50898, 1000.000000000000000 ) ;
#8012=ORIENTED_EDGE ( 'NONE', *, *, #6719, .T. ) ;
#8013=DIRECTION ( 'NONE',  ( -1.000000000000000000, 1.011922027653136551E-15, 0.000000000000000000 ) ) ;
#8015=CARTESIAN_POINT ( 'NONE',  ( 117.0705705820183482, -32.08379757587637471, 55.16038718067301261 ) ) ;
#8017=VECTOR ( 'NONE', #84742, 1000.000000000000000 ) ;
#8019=CARTESIAN_POINT ( 'NONE',  ( 115.0729613760110084, -29.04219751930509119, 185.4232443235299570 ) ) ;
#8020=CARTESIAN_POINT ( 'NONE',  ( 110.2835424219824034, -44.64187515646635518, 282.3067055423625789 ) ) ;
#8021=ORIENTED_EDGE ( 'NONE', *, *, #81289, .F. ) ;
#8023=ORIENTED_EDGE ( 'NONE', *, *, #39509, .F. ) ;
#8024=ORIENTED_EDGE ( 'NONE', *, *, #43855, .T. ) ;
#8025=CARTESIAN_POINT ( 'NONE',  ( 101.9936209452192344, -45.44607154117929326, 107.1564586096423000 ) ) ;
#8026=DIRECTION ( 'NONE',  ( 1.000000000000000000, 4.299999999999999979E-14, 1.000000000000000078E-15 ) ) ;
#8027=LINE ( 'NONE', #76624, #17270 ) ;
#8028=CARTESIAN_POINT ( 'NONE',  ( 107.0664832912739399, -36.72944715994095333, 290.1356252759106837 ) ) ;
#8032=FACE_OUTER_BOUND ( 'NONE', #67940, .T. ) ;
#8034=CARTESIAN_POINT ( 'NONE',  ( 117.3629797429381654, -38.21633193987523214, 28.71276813305395592 ) ) ;
#8035=CARTESIAN_POINT ( 'NONE',  ( 97.81252181392954981, -40.51708140501057187, 272.6353344860016819 ) ) ;
#8036=VERTEX_POINT ( 'NONE', #69565 ) ;
#8039=CARTESIAN_POINT ( 'NONE',  ( 105.2602129278706400, -44.68979347096200883, 70.21666179816293152 ) ) ;
#8040=CIRCLE ( 'NONE', #47177, 13.63963572536219715 ) ;
#8042=VECTOR ( 'NONE', #10892, 1000.000000000000114 ) ;
#8045=DIRECTION ( 'NONE',  ( 0.000000000000000000, -1.000000000000000000, 0.000000000000000000 ) ) ;
#8047=VERTEX_POINT ( 'NONE', #34585 ) ;
#8050=ORIENTED_EDGE ( 'NONE', *, *, #47623, .T. ) ;
#8051=ORIENTED_EDGE ( 'NONE', *, *, #88668, .T. ) ;
#8053=CARTESIAN_POINT ( 'NONE',  ( 109.1422557193553047, -45.34451810791325954, 129.1958690201829825 ) ) ;
#8056=CARTESIAN_POINT ( 'NONE',  ( 112.8137514937528891, -47.12132662887700008, 98.97848241876793907 ) ) ;
#8060=ORIENTED_EDGE ( 'NONE', *, *, #4332, .F. ) ;
#8061=VECTOR ( 'NONE', #37399, 1000.000000000000000 ) ;
#8062=VECTOR ( 'NONE', #60624, 999.9999999999998863 ) ;
#8063=EDGE_LOOP ( 'NONE', ( #15193, #69490, #36757, #22324 ) ) ;
#8065=EDGE_CURVE ( 'NONE', #24929, #40317, #75584, .T. ) ;
#8066=CYLINDRICAL_SURFACE ( 'NONE', #84733, 2.116999999999993776 ) ;
#8068=CARTESIAN_POINT ( 'NONE',  ( 111.2075918398242038, -27.22220237496667394, 284.7375300378162706 ) ) ;
#8069=CARTESIAN_POINT ( 'NONE',  ( 97.40507707138063154, -42.14631300639911160, 177.7451490854349743 ) ) ;
#8072=DIRECTION ( 'NONE',  ( -4.237773401492740281E-14, 1.000000000000000000, 0.000000000000000000 ) ) ;
#8073=CARTESIAN_POINT ( 'NONE',  ( 101.5008874824296896, -27.91431070382771651, 106.5241967044819944 ) ) ;
#8080=CARTESIAN_POINT ( 'NONE',  ( 194.5664832912739826, -18.82844715994099971, -5.074374724088000832 ) ) ;
#8081=VECTOR ( 'NONE', #29575, 1000.000000000000000 ) ;
#8082=EDGE_LOOP ( 'NONE', ( #47579, #58887, #32435, #23390 ) ) ;
#8084=DIRECTION ( 'NONE',  ( -0.7071067811875165754, -0.7071067811855784591, -7.071067811875158601E-16 ) ) ;
#8085=CARTESIAN_POINT ( 'NONE',  ( 111.0463177226254174, -47.04157800189014438, 17.85753003781598380 ) ) ;
#8090=CARTESIAN_POINT ( 'NONE',  ( 116.4719273984281784, -32.36179259691358823, 59.16038718067295576 ) ) ;
#8091=FACE_OUTER_BOUND ( 'NONE', #31997, .T. ) ;
#8092=CARTESIAN_POINT ( 'NONE',  ( 108.7397100058831256, -25.82697924850577920, 140.9432443235299672 ) ) ;
#8094=DIRECTION ( 'NONE',  ( 0.000000000000000000, 1.000000000000000000, 0.000000000000000000 ) ) ;
#8095=ORIENTED_EDGE ( 'NONE', *, *, #63519, .T. ) ;
#8098=FACE_OUTER_BOUND ( 'NONE', #53166, .T. ) ;
#8101=ORIENTED_EDGE ( 'NONE', *, *, #74307, .F. ) ;
#8102=EDGE_CURVE ( 'NONE', #34909, #55155, #68317, .T. ) ;
#8103=DIRECTION ( 'NONE',  ( 0.7071067811865525687, -0.7071067811865425767, 7.071067811865221912E-16 ) ) ;
#8104=CARTESIAN_POINT ( 'NONE',  ( 103.5274535807004384, -26.83869072616077744, 190.3499109901969746 ) ) ;
#8105=VERTEX_POINT ( 'NONE', #21421 ) ;
#8106=PLANE ( 'NONE',  #27690 ) ;
#8107=CARTESIAN_POINT ( 'NONE',  ( 97.38187162881654046, -40.64678755884852279, 202.6327681330539860 ) ) ;
#8108=CARTESIAN_POINT ( 'NONE',  ( 113.5330014162060195, -28.49676089798827405, 75.54705384733995288 ) ) ;
#8109=EDGE_CURVE ( 'NONE', #88572, #54506, #28209, .T. ) ;
#8112=CARTESIAN_POINT ( 'NONE',  ( 46.48091746482126041, -48.32844715994084339, 300.4678068554150059 ) ) ;
#8115=ORIENTED_EDGE ( 'NONE', *, *, #6394, .T. ) ;
#8117=ORIENTED_EDGE ( 'NONE', *, *, #62939, .T. ) ;
#8119=CARTESIAN_POINT ( 'NONE',  ( 116.6057436952887372, -40.93480069938575383, 249.4956252759109532 ) ) ;
#8123=DIRECTION ( 'NONE',  ( -0.9834602067153815907, -0.1811243269341220596, 0.000000000000000000 ) ) ;
#8124=PLANE ( 'NONE',  #73287 ) ;
#8125=CARTESIAN_POINT ( 'NONE',  ( 111.1376129892989013, -47.03096861136451423, 22.88800622829195675 ) ) ;
#8126=VERTEX_POINT ( 'NONE', #10469 ) ;
#8128=VERTEX_POINT ( 'NONE', #30468 ) ;
#8130=AXIS2_PLACEMENT_3D ( 'NONE', #84126, #21447, #42304 ) ;
#8133=CARTESIAN_POINT ( 'NONE',  ( 109.7263425203086484, -27.00119676199070895, 15.86761370455112896 ) ) ;
#8134=CARTESIAN_POINT ( 'NONE',  ( 96.93540839703301515, -34.51582869190843894, 252.1432443235293590 ) ) ;
#8135=DIRECTION ( 'NONE',  ( -0.9825752044165969590, -0.1858654558159821002, 0.000000000000000000 ) ) ;
#8137=CARTESIAN_POINT ( 'NONE',  ( 102.5967720069230893, -27.99243076246528261, 116.4527681330529703 ) ) ;
#8140=ORIENTED_EDGE ( 'NONE', *, *, #47737, .F. ) ;
#8141=CARTESIAN_POINT ( 'NONE',  ( 116.3214902495786873, -32.94210931476069248, 180.1356252759109680 ) ) ;
#8143=ORIENTED_EDGE ( 'NONE', *, *, #13308, .T. ) ;
#8144=AXIS2_PLACEMENT_3D ( 'NONE', #28016, #40301, #33489 ) ;
#8146=CARTESIAN_POINT ( 'NONE',  ( 101.2106992548341822, -44.07698544542078167, 268.4606309249448941 ) ) ;
#8148=CARTESIAN_POINT ( 'NONE',  ( 97.07206128885297858, -35.37854637286780957, 141.2189669822484461 ) ) ;
#8151=EDGE_CURVE ( 'NONE', #46099, #2137, #71805, .T. ) ;
#8152=CARTESIAN_POINT ( 'NONE',  ( 150.5667039024475571, -25.42844715993593852, 180.4678068554149775 ) ) ;
#8153=CARTESIAN_POINT ( 'NONE',  ( 61.56670390244639890, -23.42844715994043270, 129.9678068554150911 ) ) ;
#8156=EDGE_CURVE ( 'NONE', #85809, #32010, #72702, .T. ) ;
#8157=CARTESIAN_POINT ( 'NONE',  ( 83.06670390244801183, -42.21678055153920184, 231.5838068554169524 ) ) ;
#8159=CARTESIAN_POINT ( 'NONE',  ( 115.5739025235967716, -42.75529552070533867, 53.33562527591095659 ) ) ;
#8160=ORIENTED_EDGE ( 'NONE', *, *, #46691, .F. ) ;
#8161=CARTESIAN_POINT ( 'NONE',  ( 106.1481202089414637, -44.86820639808929201, 280.3052332267342877 ) ) ;
#8162=EDGE_CURVE ( 'NONE', #61548, #88283, #17290, .T. ) ;
#8163=CARTESIAN_POINT ( 'NONE',  ( 115.0383104642609311, -42.90711831593061731, 128.3024873213930448 ) ) ;
#8164=CARTESIAN_POINT ( 'NONE',  ( 116.4020974974656042, -33.81230083437810663, 174.0670538473399347 ) ) ;
#8165=DIRECTION ( 'NONE',  ( -0.7071067811869841124, 0.7071067811861110330, 0.000000000000000000 ) ) ;
#8166=CYLINDRICAL_SURFACE ( 'NONE', #6731, 11.45913725231036118 ) ;
#8169=CARTESIAN_POINT ( 'NONE',  ( 104.5778203770529586, -26.56076746289640411, 281.2670538473396959 ) ) ;
#8171=ADVANCED_FACE ( 'NONE', ( #2323 ), #38169, .F. ) ;
#8172=ORIENTED_EDGE ( 'NONE', *, *, #31445, .T. ) ;
#8173=CARTESIAN_POINT ( 'NONE',  ( 136.5307003794576133, -37.95069274174123564, 7.120636252910355957 ) ) ;
#8174=ORIENTED_EDGE ( 'NONE', *, *, #74635, .F. ) ;
#8175=CARTESIAN_POINT ( 'NONE',  ( 108.9928688995437653, -47.66043690685247469, 118.7032443235299723 ) ) ;
#8178=ORIENTED_EDGE ( 'NONE', *, *, #58478, .T. ) ;
#8180=ADVANCED_FACE ( 'NONE', ( #66306 ), #37735, .F. ) ;
#8181=DIRECTION ( 'NONE',  ( -0.9254794337955620787, -0.3787978585227822492, 0.000000000000000000 ) ) ;
#8184=FACE_OUTER_BOUND ( 'NONE', #30031, .T. ) ;
#8185=CARTESIAN_POINT ( 'NONE',  ( 80.06648329127399677, -18.72944715994105991, -5.074374724089057764 ) ) ;
#8186=CARTESIAN_POINT ( 'NONE',  ( 116.4744410436840383, -32.23804052137624865, 15.18133956162492915 ) ) ;
#8188=CARTESIAN_POINT ( 'NONE',  ( 51.56670390244899238, -32.29483332968450782, -5.074374724088000832 ) ) ;
#8191=VECTOR ( 'NONE', #30847, 1000.000000000000000 ) ;
#8192=PLANE ( 'NONE',  #14251 ) ;
#8193=VERTEX_POINT ( 'NONE', #24107 ) ;
#8194=EDGE_CURVE ( 'NONE', #77917, #85594, #65859, .T. ) ;
#8195=VERTEX_POINT ( 'NONE', #85896 ) ;
#8197=AXIS2_PLACEMENT_3D ( 'NONE', #83628, #62720, #15030 ) ;
#8198=CARTESIAN_POINT ( 'NONE',  ( 82.60909586547545302, -19.77717416134804651, 2.822018739140870203 ) ) ;
#8200=LINE ( 'NONE', #84964, #9221 ) ;
#8201=CARTESIAN_POINT ( 'NONE',  ( 188.5667039024479834, -62.87844715994099687, 173.2178068554149775 ) ) ;
#8202=CIRCLE ( 'NONE', #24150, 13.16666666666669627 ) ;
#8203=LINE ( 'NONE', #76340, #18711 ) ;
#8204=DIRECTION ( 'NONE',  ( 0.000000000000000000, 0.000000000000000000, -1.000000000000000000 ) ) ;
#8205=CARTESIAN_POINT ( 'NONE',  ( 111.2765704384832759, -44.16122339008717290, 212.4095626852199530 ) ) ;
#8206=DIRECTION ( 'NONE',  ( -4.237773401492740281E-14, 1.000000000000000000, 0.000000000000000000 ) ) ;
#8207=LINE ( 'NONE', #56781, #27702 ) ;
#8208=CARTESIAN_POINT ( 'NONE',  ( 95.98894329157613470, -41.07880401750329469, 96.62419670448197451 ) ) ;
#8209=ORIENTED_EDGE ( 'NONE', *, *, #23422, .T. ) ;
#8210=LINE ( 'NONE', #64071, #11815 ) ;
#8211=ORIENTED_EDGE ( 'NONE', *, *, #72869, .F. ) ;
#8213=VERTEX_POINT ( 'NONE', #23668 ) ;
#8214=B_SPLINE_CURVE_WITH_KNOTS ( 'NONE', 3,
 ( #4334, #19302, #12040, #46973, #25659, #81106, #17947, #18852, #19747, #47430, #74710, #61510, #59719, #46535, #74271, #52441, #39727, #5226 ),
 .UNSPECIFIED., .F., .F.,
 ( 4, 2, 2, 2, 2, 2, 2, 2, 4 ),
 ( 0.000000000000000000, 0.06249999998159491699, 0.1249999999631898340, 0.1874999999447847510, 0.2499999999263796679, 0.3124999999079746127, 0.3749999998895695019, 0.4374999998711643912, 0.4999999998527593359 ),
 .UNSPECIFIED. ) ;
#8215=CARTESIAN_POINT ( 'NONE',  ( 19.56670390244796920, -48.82844715994099971, 10.91780685541479734 ) ) ;
#8217=DIRECTION ( 'NONE',  ( 1.000000000000000000, 0.000000000000000000, 9.351236661543306751E-17 ) ) ;
#8218=EDGE_CURVE ( 'NONE', #6713, #29287, #3094, .T. ) ;
#8220=AXIS2_PLACEMENT_3D ( 'NONE', #28271, #88740, #14673 ) ;
#8221=CARTESIAN_POINT ( 'NONE',  ( 131.0667039024480118, -58.72944715994097464, 228.3338068554150198 ) ) ;
#8222=ORIENTED_EDGE ( 'NONE', *, *, #27745, .F. ) ;
#8223=CARTESIAN_POINT ( 'NONE',  ( 115.1840797895677611, -43.30599572718466561, 88.28419670448195689 ) ) ;
#8225=CARTESIAN_POINT ( 'NONE',  ( 104.4893447449655923, -26.97897155733640417, 165.2815092204904772 ) ) ;
#8226=LINE ( 'NONE', #15038, #42795 ) ;
#8227=CARTESIAN_POINT ( 'NONE',  ( 191.6375511031394865, 22.69262065192448574, 328.6381252759109088 ) ) ;
#8228=CARTESIAN_POINT ( 'NONE',  ( 115.0372574993704404, -42.90846257614333581, 143.3022919416527827 ) ) ;
#8229=ORIENTED_EDGE ( 'NONE', *, *, #9209, .T. ) ;
#8231=DIRECTION ( 'NONE',  ( 0.000000000000000000, 0.000000000000000000, -1.000000000000000000 ) ) ;
#8233=EDGE_CURVE ( 'NONE', #1069, #34489, #65457, .T. ) ;
#8234=CARTESIAN_POINT ( 'NONE',  ( 95.46382812221506242, -34.19949780945433560, 102.1556252759109640 ) ) ;
#8236=CARTESIAN_POINT ( 'NONE',  ( 127.0664832912740110, -46.72944715994101017, 14.67562527591099197 ) ) ;
#8239=EDGE_LOOP ( 'NONE', ( #55078, #23976, #21834, #58747 ) ) ;
#8240=DIRECTION ( 'NONE',  ( 0.000000000000000000, 0.000000000000000000, 1.000000000000000000 ) ) ;
#8241=CARTESIAN_POINT ( 'NONE',  ( 116.6093774848465472, -38.87601340171671893, 144.6499109901959628 ) ) ;
#8242=DIRECTION ( 'NONE',  ( 9.030537910253610117E-13, -1.000000000000000000, 9.040537910253610592E-28 ) ) ;
#8243=ORIENTED_EDGE ( 'NONE', *, *, #53674, .F. ) ;
#8244=CARTESIAN_POINT ( 'NONE',  ( 109.4546162266722575, -25.87086512622489920, 25.90419670448196143 ) ) ;
#8245=CARTESIAN_POINT ( 'NONE',  ( 194.0667039024473581, -24.92844715993408045, 249.9678068554149775 ) ) ;
#8247=CARTESIAN_POINT ( 'NONE',  ( 177.8371591254543205, -47.82818131005477369, 300.4678068554149490 ) ) ;
#8249=CARTESIAN_POINT ( 'NONE',  ( 165.3359832912740046, -36.32844715994100682, -5.074374724088000832 ) ) ;
#8250=DIRECTION ( 'NONE',  ( 0.000000000000000000, 0.000000000000000000, -1.000000000000000000 ) ) ;
#8251=CARTESIAN_POINT ( 'NONE',  ( 113.6884830475839152, -29.53135334845044468, 199.4841967044829687 ) ) ;
#8252=ORIENTED_EDGE ( 'NONE', *, *, #36016, .T. ) ;
#8253=VERTEX_POINT ( 'NONE', #4093 ) ;
#8254=CARTESIAN_POINT ( 'NONE',  ( 108.5815432132388878, -45.46059095889125246, 164.1444404487539828 ) ) ;
#8257=CIRCLE ( 'NONE', #19862, 1.000000000000000888 ) ;
#8258=CARTESIAN_POINT ( 'NONE',  ( 112.0124476237220676, -28.73397683645143275, 285.6356252759109680 ) ) ;
#8259=AXIS2_PLACEMENT_3D ( 'NONE', #22584, #44335, #29394 ) ;
#8260=CARTESIAN_POINT ( 'NONE',  ( 72.25757238336811383, -1.944390235229867425, 394.9756252759101471 ) ) ;
#8261=EDGE_CURVE ( 'NONE', #31858, #78258, #52210, .T. ) ;
#8262=EDGE_CURVE ( 'NONE', #73152, #70182, #26297, .T. ) ;
#8264=DIRECTION ( 'NONE',  ( 1.000000000000000000, 4.299999999999999979E-14, 1.000000000000000078E-15 ) ) ;
#8265=CARTESIAN_POINT ( 'NONE',  ( 113.2454986968446207, -28.75867294377915684, 105.5522919427003359 ) ) ;
#8268=CARTESIAN_POINT ( 'NONE',  ( 112.1942863616536386, -45.78120396183496155, 212.9870538473389558 ) ) ;
#8269=CARTESIAN_POINT ( 'NONE',  ( 97.53211619416173050, -39.74981511173461257, 171.5707515385688566 ) ) ;
#8272=EDGE_CURVE ( 'NONE', #36906, #67921, #9138, .T. ) ;
#8273=CARTESIAN_POINT ( 'NONE',  ( 117.0718954857576932, -35.46248235859899722, 88.92729194239142032 ) ) ;
#8275=LINE ( 'NONE', #43219, #12770 ) ;
#8276=CARTESIAN_POINT ( 'NONE',  ( 172.5664832912740110, -36.32844715994070839, 318.9256252759120116 ) ) ;
#8278=CARTESIAN_POINT ( 'NONE',  ( 101.5079035968564654, -28.64143341885332816, 46.55562527591094835 ) ) ;
#8280=CIRCLE ( 'NONE', #50269, 2.117000000000000881 ) ;
#8281=EDGE_CURVE ( 'NONE', #12059, #34909, #88687, .T. ) ;
#8282=ORIENTED_EDGE ( 'NONE', *, *, #18037, .T. ) ;
#8283=CARTESIAN_POINT ( 'NONE',  ( 101.3604548305157920, -27.95253318249931596, 21.53562527591096298 ) ) ;
#8285=CARTESIAN_POINT ( 'NONE',  ( 105.1109252617814604, -26.48919212138316581, 235.2270538473399313 ) ) ;
#8286=EDGE_LOOP ( 'NONE', ( #52225, #51606 ) ) ;
#8287=EDGE_CURVE ( 'NONE', #85160, #11890, #35352, .T. ) ;
#8288=LINE ( 'NONE', #76878, #33220 ) ;
#8290=CARTESIAN_POINT ( 'NONE',  ( 80.06648329127402519, -46.72944715994105991, 4.925625275910944012 ) ) ;
#8291=CARTESIAN_POINT ( 'NONE',  ( 115.1946057043837328, -37.48001498139237953, 76.57094751244896713 ) ) ;
#8292=CARTESIAN_POINT ( 'NONE',  ( 114.1394676070193839, -29.04113448922185370, 195.4841967044819739 ) ) ;
#8293=DIRECTION ( 'NONE',  ( 4.299999999999999979E-14, -1.000000000000000000, 4.400000000000000367E-29 ) ) ;
#8294=VERTEX_POINT ( 'NONE', #73578 ) ;
#8295=DIRECTION ( 'NONE',  ( 0.000000000000000000, 0.000000000000000000, -1.000000000000000000 ) ) ;
#8296=ORIENTED_EDGE ( 'NONE', *, *, #24380, .F. ) ;
#8297=AXIS2_PLACEMENT_3D ( 'NONE', #6313, #7660, #61268 ) ;
#8298=EDGE_LOOP ( 'NONE', ( #11752, #11986, #4469, #54961 ) ) ;
#8299=DIRECTION ( 'NONE',  ( -1.000000000000000000, -2.756263715554006823E-15, 0.000000000000000000 ) ) ;
#8300=ORIENTED_EDGE ( 'NONE', *, *, #41642, .F. ) ;
#8301=EDGE_LOOP ( 'NONE', ( #33096, #28179 ) ) ;
#8304=CARTESIAN_POINT ( 'NONE',  ( 101.5215670198552544, -44.69967496328137457, 86.51527697093396796 ) ) ;
#8305=B_SPLINE_CURVE_WITH_KNOTS ( 'NONE', 3,
 ( #73524, #79479, #66711, #24937, #52601, #11298, #38119, #59878, #65810, #45798, #86278, #59440, #18560, #25375, #17239, #24057, #46243, #39001, #24498, #3598, #3164, #53044, #80810, #17678, #45357, #31291, #31744, #86725, #79924, #9530 ),
 .UNSPECIFIED., .F., .F.,
 ( 4, 2, 2, 2, 2, 2, 2, 2, 2, 2, 1, 1, 1, 1, 1, 1, 2, 4 ),
 ( 0.000000000000000000, 0.06250181204942577284, 0.1250036240988515457, 0.1875054361482773324, 0.2500072481977030914, 0.3125090602471288226, 0.3750108722965546648, 0.4375126843459803960, 0.4687635903706935392, 0.4843890433830502218, 0.4922017698892287019, 0.4961081331423181084, 0.4980613147688628395, 0.4990379055821350662, 0.4995262009887708743, 0.4997703486920889726, 0.4998924225437479940, 0.5000144963954069599 ),
 .UNSPECIFIED. ) ;
#8306=CARTESIAN_POINT ( 'NONE',  ( 97.19579330311479737, -33.30690068839255957, 286.0613395616251751 ) ) ;
#8310=ORIENTED_EDGE ( 'NONE', *, *, #33389, .F. ) ;
#8311=DIRECTION ( 'NONE',  ( 0.000000000000000000, 0.000000000000000000, 1.000000000000000000 ) ) ;
#8313=DIRECTION ( 'NONE',  ( 0.000000000000000000, 0.000000000000000000, -1.000000000000000000 ) ) ;
#8314=ADVANCED_FACE ( 'NONE', ( #88122 ), #87664, .T. ) ;
#8316=CARTESIAN_POINT ( 'NONE',  ( 118.1720832024965802, -36.20253795304678590, 118.8641967044829784 ) ) ;
#8317=CARTESIAN_POINT ( 'NONE',  ( 102.5390659930443746, -27.28968240376552501, 95.43276813305395478 ) ) ;
#8318=CIRCLE ( 'NONE', #79406, 11.45913725231036118 ) ;
#8320=ORIENTED_EDGE ( 'NONE', *, *, #1802, .F. ) ;
#8322=CARTESIAN_POINT ( 'NONE',  ( 116.5268644012694637, -41.19342475044518181, 228.4756252759109714 ) ) ;
#8324=AXIS2_PLACEMENT_3D ( 'NONE', #43786, #85603, #63805 ) ;
#8326=CARTESIAN_POINT ( 'NONE',  ( 168.3595971214444376, -48.62134037892997895, 129.9678068554150059 ) ) ;
#8330=CARTESIAN_POINT ( 'NONE',  ( 132.2129280580803652, -38.76093376058476991, 7.655955902698878823 ) ) ;
#8332=DIRECTION ( 'NONE',  ( 1.000000000000000000, 4.237773401492740281E-14, 0.000000000000000000 ) ) ;
#8333=CYLINDRICAL_SURFACE ( 'NONE', #40485, 9.999999999999998224 ) ;
#8334=CONICAL_SURFACE ( 'NONE', #6895, 11.57110091390449469, 0.7853981633974471688 ) ;
#8335=DIRECTION ( 'NONE',  ( -4.237773401492740281E-14, 1.000000000000000000, 0.000000000000000000 ) ) ;
#8336=ORIENTED_EDGE ( 'NONE', *, *, #10117, .F. ) ;
#8338=CARTESIAN_POINT ( 'NONE',  ( 96.75420216176078725, -40.77324476150559462, 246.6118157521009664 ) ) ;
#8339=CARTESIAN_POINT ( 'NONE',  ( 98.00710227423795118, -30.39686567179408172, 156.8289586092439549 ) ) ;
#8340=CARTESIAN_POINT ( 'NONE',  ( 97.05449064767977063, -33.74661928051879300, 27.09562527591097236 ) ) ;
#8341=VECTOR ( 'NONE', #82456, 1000.000000000000000 ) ;
#8342=FACE_OUTER_BOUND ( 'NONE', #54952, .T. ) ;
#8343=CIRCLE ( 'NONE', #89585, 2.116999999999980009 ) ;
#8345=CARTESIAN_POINT ( 'NONE',  ( 81.50686229670706950, -34.38644903112238893, 7.895285856724627571 ) ) ;
#8346=CARTESIAN_POINT ( 'NONE',  ( 109.6429292107771687, -46.48010952738405166, 138.7814519316777648 ) ) ;
#8348=AXIS2_PLACEMENT_3D ( 'NONE', #21159, #22073, #56093 ) ;
#8350=ORIENTED_EDGE ( 'NONE', *, *, #49991, .T. ) ;
#8351=DIRECTION ( 'NONE',  ( -4.237773401492740281E-14, 1.000000000000000000, 0.000000000000000000 ) ) ;
#8353=CARTESIAN_POINT ( 'NONE',  ( 98.04376085404715013, -35.95281974173802553, 185.6686103042669629 ) ) ;
#8354=LINE ( 'NONE', #42398, #13778 ) ;
#8355=EDGE_LOOP ( 'NONE', ( #12936, #72521, #82908, #33431 ) ) ;
#8357=CARTESIAN_POINT ( 'NONE',  ( 96.76471471792635271, -35.27954033865441374, 177.2156252759109805 ) ) ;
#8358=CARTESIAN_POINT ( 'NONE',  ( 80.06648329127402519, -41.22944715994105280, -0.5743747240890559880 ) ) ;
#8359=DIRECTION ( 'NONE',  ( -1.000000000000000000, 0.000000000000000000, -0.000000000000000000 ) ) ;
#8360=CARTESIAN_POINT ( 'NONE',  ( 98.35372588324824505, -31.64965747931991302, 86.90591219145825619 ) ) ;
#8361=DIRECTION ( 'NONE',  ( 1.000000000000000078E-15, -1.000000000000000083E-30, -1.000000000000000000 ) ) ;
#8362=CYLINDRICAL_SURFACE ( 'NONE', #9199, 2.030000000001310312 ) ;
#8363=CARTESIAN_POINT ( 'NONE',  ( 109.6029845306728419, -46.78454271877410520, 92.78514908543594686 ) ) ;
#8368=CARTESIAN_POINT ( 'NONE',  ( 101.8615262650677522, -29.55750872133152640, 72.00729759161094989 ) ) ;
#8370=CARTESIAN_POINT ( 'NONE',  ( 103.1049807579881588, -45.67203811392940338, 173.2441967044819648 ) ) ;
#8373=DIRECTION ( 'NONE',  ( 0.000000000000000000, -1.000000000000000000, 0.000000000000000000 ) ) ;
#8376=CARTESIAN_POINT ( 'NONE',  ( 165.3359832912740046, -36.32844715994100682, -5.074374724088000832 ) ) ;
#8379=CARTESIAN_POINT ( 'NONE',  ( 118.8789388927533111, -36.16900092901214947, 118.8641967044819836 ) ) ;
#8380=ORIENTED_EDGE ( 'NONE', *, *, #25773, .F. ) ;
#8381=ADVANCED_FACE ( 'NONE', ( #39055, #59487 ), #66761, .T. ) ;
#8384=EDGE_CURVE ( 'NONE', #54125, #74866, #74480, .T. ) ;
#8387=VECTOR ( 'NONE', #78916, 1000.000000000000000 ) ;
#8388=CARTESIAN_POINT ( 'NONE',  ( 97.07198155714206678, -35.37918349729778100, 131.2190186775771679 ) ) ;
#8389=DIRECTION ( 'NONE',  ( 1.000000000000000078E-15, -1.000000000000000083E-30, -1.000000000000000000 ) ) ;
#8390=CARTESIAN_POINT ( 'NONE',  ( 99.90434330870786539, -40.64524553156628173, 219.5423760838769738 ) ) ;
#8395=VERTEX_POINT ( 'NONE', #81758 ) ;
#8396=ORIENTED_EDGE ( 'NONE', *, *, #38268, .F. ) ;
#8397=ORIENTED_EDGE ( 'NONE', *, *, #32033, .T. ) ;
#8402=ORIENTED_EDGE ( 'NONE', *, *, #63979, .F. ) ;
#8405=CARTESIAN_POINT ( 'NONE',  ( 115.7948931938460362, -35.19871557519451954, 240.3958690201829427 ) ) ;
#8406=VECTOR ( 'NONE', #26506, 1000.000000000000000 ) ;
#8408=VERTEX_POINT ( 'NONE', #39507 ) ;
#8409=VECTOR ( 'NONE', #72721, 1000.000000000000114 ) ;
#8410=AXIS2_PLACEMENT_3D ( 'NONE', #59783, #31189, #85751 ) ;
#8411=CARTESIAN_POINT ( 'NONE',  ( 104.1241784947088149, -44.29815144288988193, 9.635625275910944865 ) ) ;
#8412=CARTESIAN_POINT ( 'NONE',  ( 162.8913605087219878, -31.76306994223740432, -5.074374724088000832 ) ) ;
#8413=VERTEX_POINT ( 'NONE', #55784 ) ;
#8417=ORIENTED_EDGE ( 'NONE', *, *, #68253, .T. ) ;
#8418=VERTEX_POINT ( 'NONE', #7676 ) ;
#8419=CARTESIAN_POINT ( 'NONE',  ( 102.3843679657495329, -43.41581164733459985, 279.9080903695913776 ) ) ;
#8420=CARTESIAN_POINT ( 'NONE',  ( 108.9491902927665734, -26.41713524962505133, 164.9327681330529742 ) ) ;
#8421=CARTESIAN_POINT ( 'NONE',  ( 114.6914383512288254, -44.69963429152232237, 113.1718157521009687 ) ) ;
#8423=CARTESIAN_POINT ( 'NONE',  ( 111.1274376763295635, -27.12782558180003889, 240.7584824187679544 ) ) ;
#8424=DIRECTION ( 'NONE',  ( 4.299999999999999979E-14, -1.000000000000000000, 0.000000000000000000 ) ) ;
#8425=LINE ( 'NONE', #50178, #34946 ) ;
#8428=VERTEX_POINT ( 'NONE', #21767 ) ;
#8431=ADVANCED_FACE ( 'NONE', ( #83994 ), #48523, .T. ) ;
#8432=VECTOR ( 'NONE', #26540, 1000.000000000000000 ) ;
#8434=CARTESIAN_POINT ( 'NONE',  ( 96.02342237304465300, -37.20891875426686823, 116.3489586092439652 ) ) ;
#8435=CARTESIAN_POINT ( 'NONE',  ( 107.0664832912739968, 19.62155284005901024, 336.6506252759110112 ) ) ;
#8436=EDGE_CURVE ( 'NONE', #57610, #43708, #410, .T. ) ;
#8440=CARTESIAN_POINT ( 'NONE',  ( 112.5709320333848069, -45.13014110428505177, 58.03751997880807068 ) ) ;
#8441=CARTESIAN_POINT ( 'NONE',  ( 101.6619702986603073, -45.61876124157276280, 243.1413395616249886 ) ) ;
#8443=DIRECTION ( 'NONE',  ( 0.7071067811865483499, 0.7071067811865466846, 7.071067811865491110E-16 ) ) ;
#8444=CARTESIAN_POINT ( 'NONE',  ( 134.0664832912739826, -9.029447159941003775, 4.925625275910997303 ) ) ;
#8446=CARTESIAN_POINT ( 'NONE',  ( 97.06107110138425753, -37.99641199796607793, 257.4272919453096051 ) ) ;
#8448=CARTESIAN_POINT ( 'NONE',  ( 96.51917584821923413, -40.19201726479878545, 286.5908633711491120 ) ) ;
#8449=VERTEX_POINT ( 'NONE', #77172 ) ;
#8451=CARTESIAN_POINT ( 'NONE',  ( 105.3125257651413307, -48.47460025707392361, 147.4584824187679715 ) ) ;
#8452=CARTESIAN_POINT ( 'NONE',  ( 106.5180998683148488, -25.68982506017174927, 41.12800622829193742 ) ) ;
#8453=CARTESIAN_POINT ( 'NONE',  ( 117.4569897637122011, -35.45259360763351708, 189.9241967044829664 ) ) ;
#8456=CARTESIAN_POINT ( 'NONE',  ( 51.34673845256583036, -36.02818131005845004, 237.4678068554150059 ) ) ;
#8457=CYLINDRICAL_SURFACE ( 'NONE', #37623, 4.875000000000017764 ) ;
#8458=LINE ( 'NONE', #22993, #74725 ) ;
#8459=LINE ( 'NONE', #21191, #35036 ) ;
#8460=DIRECTION ( 'NONE',  ( -1.000000000000000078E-15, 1.000000000000000083E-30, 1.000000000000000000 ) ) ;
#8463=CIRCLE ( 'NONE', #7016, 3.299999999999997158 ) ;
#8467=ORIENTED_EDGE ( 'NONE', *, *, #38910, .F. ) ;
#8469=FACE_OUTER_BOUND ( 'NONE', #4265, .T. ) ;
#8471=CARTESIAN_POINT ( 'NONE',  ( 115.5559444348970857, -42.74257571503945741, 49.33562527591095659 ) ) ;
#8476=CARTESIAN_POINT ( 'NONE',  ( 97.91841856125127208, -30.44371649139010927, 161.8594347997199918 ) ) ;
#8479=CARTESIAN_POINT ( 'NONE',  ( 114.6457050300329996, -40.66804080626008044, 287.8667055423626380 ) ) ;
#8480=EDGE_LOOP ( 'NONE', ( #48865, #25062, #72959, #34194 ) ) ;
#8481=ORIENTED_EDGE ( 'NONE', *, *, #73481, .F. ) ;
#8483=ORIENTED_EDGE ( 'NONE', *, *, #71364, .F. ) ;
#8484=DIRECTION ( 'NONE',  ( 1.000000000000000078E-15, -1.000000000000000000, 0.000000000000000000 ) ) ;
#8485=CARTESIAN_POINT ( 'NONE',  ( 138.8167039024479834, -67.87844715994100397, 37.63480685541480852 ) ) ;
#8486=LINE ( 'NONE', #35270, #33207 ) ;
#8487=CARTESIAN_POINT ( 'NONE',  ( 80.06648329127402519, -46.72944715994105991, 8.225625275910942946 ) ) ;
#8491=DIRECTION ( 'NONE',  ( 0.000000000000000000, -1.000000000000000000, 0.000000000000000000 ) ) ;
#8493=CARTESIAN_POINT ( 'NONE',  ( 110.5478855402368197, -46.57039549162855963, 37.84705384733994293 ) ) ;
#8494=ADVANCED_FACE ( 'NONE', ( #7234 ), #28101, .T. ) ;
#8495=ORIENTED_EDGE ( 'NONE', *, *, #2004, .F. ) ;
#8496=CARTESIAN_POINT ( 'NONE',  ( 142.8821648370248170, -72.54478064608022692, 542.9756252759101471 ) ) ;
#8497=CIRCLE ( 'NONE', #20096, 2.999999999999933387 ) ;
#8499=CARTESIAN_POINT ( 'NONE',  ( 111.9587407205840890, -30.16069495786998544, 102.3852332267339591 ) ) ;
#8501=FACE_OUTER_BOUND ( 'NONE', #63614, .T. ) ;
#8503=VERTEX_POINT ( 'NONE', #70351 ) ;
#8508=VERTEX_POINT ( 'NONE', #34474 ) ;
#8509=EDGE_CURVE ( 'NONE', #593, #42450, #35367, .T. ) ;
#8510=CARTESIAN_POINT ( 'NONE',  ( 113.1089835609813719, -43.92423027677314451, 144.5520594963729764 ) ) ;
#8513=CARTESIAN_POINT ( 'NONE',  ( 111.0909104302412373, -25.55688089738240976, 95.80133956162495679 ) ) ;
#8514=CARTESIAN_POINT ( 'NONE',  ( 37.35959712133814747, -48.62134037883198090, 180.4678068554150911 ) ) ;
#8517=AXIS2_PLACEMENT_3D ( 'NONE', #30505, #24140, #1469 ) ;
#8518=ORIENTED_EDGE ( 'NONE', *, *, #89490, .F. ) ;
#8519=VERTEX_POINT ( 'NONE', #75820 ) ;
#8521=CARTESIAN_POINT ( 'NONE',  ( 98.70474251149389033, -42.99264563182325816, 66.83848241876793850 ) ) ;
#8522=VERTEX_POINT ( 'NONE', #63077 ) ;
#8523=CARTESIAN_POINT ( 'NONE',  ( 99.81116105471912192, -29.32005551970541291, 270.7051490854354938 ) ) ;
#8524=CARTESIAN_POINT ( 'NONE',  ( 97.74302678327005367, -41.52030872683848628, 192.7041967044819728 ) ) ;
#8525=LINE ( 'NONE', #77119, #69827 ) ;
#8526=CARTESIAN_POINT ( 'NONE',  ( 98.30746454995575334, -41.72870539506785548, 127.7397773158203620 ) ) ;
#8527=CARTESIAN_POINT ( 'NONE',  ( 103.4684036848089050, -46.51393990267121836, 138.2956252759109645 ) ) ;
#8528=CARTESIAN_POINT ( 'NONE',  ( 149.4409906032288973, -0.9156555935619370423, 394.9756252759100903 ) ) ;
#8529=ORIENTED_EDGE ( 'NONE', *, *, #31487, .T. ) ;
#8530=VECTOR ( 'NONE', #84911, 1000.000000000000000 ) ;
#8532=VERTEX_POINT ( 'NONE', #89457 ) ;
#8533=AXIS2_PLACEMENT_3D ( 'NONE', #28997, #15376, #56682 ) ;
#8534=CARTESIAN_POINT ( 'NONE',  ( 98.04140018452436323, -41.04160969738705944, 132.6816209718298012 ) ) ;
#8535=ORIENTED_EDGE ( 'NONE', *, *, #14089, .T. ) ;
#8536=ORIENTED_EDGE ( 'NONE', *, *, #7142, .T. ) ;
#8538=CARTESIAN_POINT ( 'NONE',  ( 51.42025729303981052, -33.70561438052008896, 193.9678068554150911 ) ) ;
#8539=CARTESIAN_POINT ( 'NONE',  ( 101.6088808140983417, -47.24878093606274376, 17.19562527591095247 ) ) ;
#8540=DIRECTION ( 'NONE',  ( 0.000000000000000000, 0.000000000000000000, 1.000000000000000000 ) ) ;
#8541=ADVANCED_FACE ( 'NONE', ( #48980 ), #8124, .F. ) ;
#8542=DIRECTION ( 'NONE',  ( 1.000000000000000000, 4.163336342344333240E-14, 0.000000000000000000 ) ) ;
#8543=CARTESIAN_POINT ( 'NONE',  ( 117.0608945237863736, -38.08045311857467397, 74.71895860942261436 ) ) ;
#8544=CARTESIAN_POINT ( 'NONE',  ( 114.5308976578478735, -43.10096916487051288, 63.26419670448296984 ) ) ;
#8545=LINE ( 'NONE', #84859, #23194 ) ;
#8546=CARTESIAN_POINT ( 'NONE',  ( 96.69266148864274157, -35.94780844399463149, 142.2670538473399517 ) ) ;
#8547=CARTESIAN_POINT ( 'NONE',  ( 116.3212776292294421, -32.94146857471278622, 70.13562527591093954 ) ) ;
#8548=CYLINDRICAL_SURFACE ( 'NONE', #58299, 2.116999999999980009 ) ;
#8549=EDGE_LOOP ( 'NONE', ( #2632, #34325 ) ) ;
#8551=CARTESIAN_POINT ( 'NONE',  ( 20.03715912545739997, -46.82818131006202123, 129.9678068554150627 ) ) ;
#8552=DIRECTION ( 'NONE',  ( -4.299999999999999979E-14, 1.000000000000000000, 0.000000000000000000 ) ) ;
#8553=DIRECTION ( 'NONE',  ( 0.000000000000000000, 0.000000000000000000, -1.000000000000000000 ) ) ;
#8554=ORIENTED_EDGE ( 'NONE', *, *, #43746, .F. ) ;
#8555=CARTESIAN_POINT ( 'NONE',  ( 36.23715912545339535, -47.82818131006131779, 180.4678068554150911 ) ) ;
#8556=CARTESIAN_POINT ( 'NONE',  ( 109.4554010020096513, -25.88943074854985227, 179.8918157521019339 ) ) ;
#8557=ORIENTED_EDGE ( 'NONE', *, *, #33517, .T. ) ;
#8558=CARTESIAN_POINT ( 'NONE',  ( 75.26949937496601706, -71.54137415153812185, 394.9756252759101471 ) ) ;
#8559=CARTESIAN_POINT ( 'NONE',  ( 116.8778831976698882, -40.31743973661899361, 214.5470538473389581 ) ) ;
#8560=CARTESIAN_POINT ( 'NONE',  ( 115.3013748915712711, -44.17149383341634206, 79.25372051400697160 ) ) ;
#8562=CARTESIAN_POINT ( 'NONE',  ( 112.1368176753006338, -28.01137494322663102, 190.6564328795896586 ) ) ;
#8564=CARTESIAN_POINT ( 'NONE',  ( 179.7974245136200011, -36.32844715994040996, -5.074374724088000832 ) ) ;
#8568=ORIENTED_EDGE ( 'NONE', *, *, #45907, .F. ) ;
#8569=EDGE_CURVE ( 'NONE', #74616, #52978, #27215, .T. ) ;
#8571=CARTESIAN_POINT ( 'NONE',  ( 172.5667039024478129, -36.32844715993500273, 300.4678068554149490 ) ) ;
#8572=CARTESIAN_POINT ( 'NONE',  ( 110.2558863881303779, -26.76706588525435748, 230.8299109901969643 ) ) ;
#8573=DIRECTION ( 'NONE',  ( 0.000000000000000000, 1.000000000000000000, 0.000000000000000000 ) ) ;
#8574=CARTESIAN_POINT ( 'NONE',  ( 136.8164832912739826, -18.72944715994099951, 3.101481641215532825 ) ) ;
#8575=EDGE_CURVE ( 'NONE', #42339, #84277, #84449, .T. ) ;
#8576=AXIS2_PLACEMENT_3D ( 'NONE', #76918, #14246, #158 ) ;
#8578=LINE ( 'NONE', #1763, #7618 ) ;
#8579=CARTESIAN_POINT ( 'NONE',  ( 165.9667039024459996, -28.27351298637401200, -5.074374724088000832 ) ) ;
#8580=CARTESIAN_POINT ( 'NONE',  ( 107.0664832912739968, -8.350947159940998787, 333.4006252759120343 ) ) ;
#8581=CARTESIAN_POINT ( 'NONE',  ( 97.78948648769619467, -29.31518076255846239, 45.78991099019697231 ) ) ;
#8582=VERTEX_POINT ( 'NONE', #54895 ) ;
#8583=ADVANCED_FACE ( 'NONE', ( #82660 ), #86408, .T. ) ;
#8587=ORIENTED_EDGE ( 'NONE', *, *, #9605, .T. ) ;
#8588=CARTESIAN_POINT ( 'NONE',  ( 194.0667039024482108, -40.32844715993407192, 180.4678068554150343 ) ) ;
#8589=CARTESIAN_POINT ( 'NONE',  ( 97.79625303259112457, -40.47954707014128672, 17.63206288286017553 ) ) ;
#8591=CARTESIAN_POINT ( 'NONE',  ( 117.9377692877171313, -39.05906590213764673, 254.6584824187675338 ) ) ;
#8592=DIRECTION ( 'NONE',  ( 0.000000000000000000, 0.000000000000000000, -1.000000000000000000 ) ) ;
#8593=VECTOR ( 'NONE', #32739, 1000.000000000000000 ) ;
#8594=CARTESIAN_POINT ( 'NONE',  ( 97.33998274022617636, -37.75834089694784979, 122.4099109901959679 ) ) ;
#8596=EDGE_CURVE ( 'NONE', #9390, #47902, #36732, .T. ) ;
#8598=ORIENTED_EDGE ( 'NONE', *, *, #30832, .F. ) ;
#8600=CARTESIAN_POINT ( 'NONE',  ( 78.94209639488894936, -34.21971364483395206, 1.822997995688476314 ) ) ;
#8601=AXIS2_PLACEMENT_3D ( 'NONE', #60134, #48288, #61044 ) ;
#8605=CARTESIAN_POINT ( 'NONE',  ( 103.0821812797523194, -45.97846664716049503, 283.6844404487542874 ) ) ;
#8607=CARTESIAN_POINT ( 'NONE',  ( 97.33784131715731291, -34.07106450827230049, 86.11479194080892796 ) ) ;
#8609=CARTESIAN_POINT ( 'NONE',  ( 107.0664832912739968, -36.72944715994100306, 287.6356252759109680 ) ) ;
#8610=ORIENTED_EDGE ( 'NONE', *, *, #3051, .T. ) ;
#8614=ORIENTED_EDGE ( 'NONE', *, *, #49441, .T. ) ;
#8615=CARTESIAN_POINT ( 'NONE',  ( 107.6031522308233974, -26.28253885536559764, 95.03562527591097364 ) ) ;
#8616=EDGE_LOOP ( 'NONE', ( #54076, #71189, #24363, #22148 ) ) ;
#8617=ADVANCED_FACE ( 'NONE', ( #64433 ), #10359, .T. ) ;
#8618=CARTESIAN_POINT ( 'NONE',  ( 109.7027494226597071, -44.85393009491053817, 12.24956268521998304 ) ) ;
#8621=CARTESIAN_POINT ( 'NONE',  ( 103.7602102885707183, -27.48919103108766748, 190.3499109901969746 ) ) ;
#8622=CARTESIAN_POINT ( 'NONE',  ( 49.16670390244654953, -26.71338133339277121, 117.4678068554150485 ) ) ;
#8623=DIRECTION ( 'NONE',  ( 1.000000000000000000, 4.299999999999999979E-14, 1.000000000000000078E-15 ) ) ;
#8626=CARTESIAN_POINT ( 'NONE',  ( 154.4532655810166091, -72.54279768053238797, 396.9756252759102040 ) ) ;
#8628=CARTESIAN_POINT ( 'NONE',  ( 101.0616705854173460, -45.30470917520826646, 278.0899109901965858 ) ) ;
#8630=ORIENTED_EDGE ( 'NONE', *, *, #36475, .F. ) ;
#8631=CARTESIAN_POINT ( 'NONE',  ( 136.8037680012515409, -37.00431460297851061, 6.768845952122538812 ) ) ;
#8633=CARTESIAN_POINT ( 'NONE',  ( 95.62763156918455820, -33.44862719079586810, 137.1041967044819501 ) ) ;
#8634=FACE_OUTER_BOUND ( 'NONE', #89382, .T. ) ;
#8636=ORIENTED_EDGE ( 'NONE', *, *, #61694, .T. ) ;
#8637=ORIENTED_EDGE ( 'NONE', *, *, #37486, .F. ) ;
#8638=DIRECTION ( 'NONE',  ( 0.000000000000000000, 0.000000000000000000, -1.000000000000000000 ) ) ;
#8639=CARTESIAN_POINT ( 'NONE',  ( 116.3153332067577850, -32.94059133099460723, 170.1356252759109680 ) ) ;
#8640=DIRECTION ( 'NONE',  ( 1.000000000000000078E-15, 0.000000000000000000, 1.000000000000000000 ) ) ;
#8641=PLANE ( 'NONE',  #77096 ) ;
#8642=CARTESIAN_POINT ( 'NONE',  ( 41.56670390244695312, -36.32844715994109208, 129.9678068554150911 ) ) ;
#8643=CARTESIAN_POINT ( 'NONE',  ( 115.6112259330891305, -28.51835778375803798, 35.43562527591098643 ) ) ;
#8644=CARTESIAN_POINT ( 'NONE',  ( 25.56670390244797275, -67.87844715994100397, 178.0928068554149775 ) ) ;
#8645=VERTEX_POINT ( 'NONE', #57607 ) ;
#8646=CARTESIAN_POINT ( 'NONE',  ( 127.0664832912740394, -54.72944906728950798, -4.824374724089008915 ) ) ;
#8648=LINE ( 'NONE', #49501, #50474 ) ;
#8649=ORIENTED_EDGE ( 'NONE', *, *, #29402, .F. ) ;
#8651=VECTOR ( 'NONE', #58400, 1000.000000000000000 ) ;
#8652=AXIS2_PLACEMENT_3D ( 'NONE', #25137, #32385, #39655 ) ;
#8653=CARTESIAN_POINT ( 'NONE',  ( 81.19087023417348803, -21.23918067504819263, 1.822998012174939397 ) ) ;
#8654=DIRECTION ( 'NONE',  ( -1.000000000000000000, -6.493183223601999383E-14, -1.000000000000000078E-15 ) ) ;
#8655=DIRECTION ( 'NONE',  ( 0.000000000000000000, 0.000000000000000000, -1.000000000000000000 ) ) ;
#8656=FACE_BOUND ( 'NONE', #65713, .T. ) ;
#8657=PLANE ( 'NONE',  #76596 ) ;
#8658=CARTESIAN_POINT ( 'NONE',  ( 104.4064053327731472, -46.06725273453308489, 216.7781341137909692 ) ) ;
#8659=CARTESIAN_POINT ( 'NONE',  ( 172.5664832912729878, -27.82844715994070484, 18.92562527591200094 ) ) ;
#8661=CARTESIAN_POINT ( 'NONE',  ( 101.6553708923145649, -27.03755641387271069, 105.4937205140069665 ) ) ;
#8663=DIRECTION ( 'NONE',  ( -0.7071067811892205457, 0.7071067811838745998, -7.071067811892213774E-16 ) ) ;
#8666=DIRECTION ( 'NONE',  ( 0.000000000000000000, 0.000000000000000000, -1.000000000000000000 ) ) ;
#8668=CARTESIAN_POINT ( 'NONE',  ( 41.56648329127398966, -27.82844715994070484, 138.9256252759119832 ) ) ;
#8669=ORIENTED_EDGE ( 'NONE', *, *, #42492, .F. ) ;
#8671=ORIENTED_EDGE ( 'NONE', *, *, #59216, .T. ) ;
#8672=DIRECTION ( 'NONE',  ( -1.000000000000000000, 0.000000000000000000, -1.000000000000000078E-15 ) ) ;
#8674=CARTESIAN_POINT ( 'NONE',  ( 115.0388443161213416, -42.90644873051409292, 274.3020457939018115 ) ) ;
#8675=DIRECTION ( 'NONE',  ( 0.000000000000000000, 1.000000000000000000, 0.000000000000000000 ) ) ;
#8677=CARTESIAN_POINT ( 'NONE',  ( 109.9170780819575839, -46.81718586395340509, 72.79562527591099297 ) ) ;
#8680=CARTESIAN_POINT ( 'NONE',  ( 97.80409201228124516, -40.49881500342829810, 166.6340252493254752 ) ) ;
#8681=CARTESIAN_POINT ( 'NONE',  ( 150.8167039024480118, -58.72944715994110254, 10.91780685541479734 ) ) ;
#8682=ADVANCED_FACE ( 'NONE', ( #30364 ), #44409, .F. ) ;
#8686=EDGE_CURVE ( 'NONE', #9382, #30460, #47147, .T. ) ;
#8688=DIRECTION ( 'NONE',  ( 0.000000000000000000, 0.000000000000000000, -1.000000000000000000 ) ) ;
#8689=CARTESIAN_POINT ( 'NONE',  ( 162.5667039024471308, -32.29483332967974718, 313.9678068554149490 ) ) ;
#8691=CARTESIAN_POINT ( 'NONE',  ( 98.44073678691454177, -30.83591204966533894, 116.8499109901969604 ) ) ;
#8693=B_SPLINE_CURVE_WITH_KNOTS ( 'NONE', 3,
 ( #67204, #5891, #88120, #66759, #25878, #53093, #33584, #18614, #4545, #6327, #74929, #53551, #46296, #53998, #32686, #47643, #81319, #60833 ),
 .UNSPECIFIED., .F., .F.,
 ( 4, 2, 2, 2, 2, 2, 2, 2, 4 ),
 ( 0.000000000000000000, 0.06249962285685504298, 0.1249992457137100860, 0.1874988685705651359, 0.2499984914274201719, 0.3124981142842752080, 0.3749977371411302718, 0.4374973599979852801, 0.4999969828548403439 ),
 .UNSPECIFIED. ) ;
#8694=CYLINDRICAL_SURFACE ( 'NONE', #8768, 10.00000000000000711 ) ;
#8695=DIRECTION ( 'NONE',  ( 1.000000000000000078E-15, -1.000000000000000000, 0.000000000000000000 ) ) ;
#8699=DIRECTION ( 'NONE',  ( -4.299999999999999979E-14, 1.000000000000000000, -4.400000000000000367E-29 ) ) ;
#8700=ADVANCED_FACE ( 'NONE', ( #85788 ), #43967, .F. ) ;
#8701=CARTESIAN_POINT ( 'NONE',  ( 113.2097911582632292, -29.11871762112829032, 160.5356252759109736 ) ) ;
#8703=ORIENTED_EDGE ( 'NONE', *, *, #57058, .F. ) ;
#8705=CARTESIAN_POINT ( 'NONE',  ( 115.3461623907573710, -31.52268719801068642, 30.27276813305296344 ) ) ;
#8706=LINE ( 'NONE', #10038, #19352 ) ;
#8707=LINE ( 'NONE', #52993, #51876 ) ;
#8710=EDGE_CURVE ( 'NONE', #13820, #24965, #17181, .T. ) ;
#8711=TOROIDAL_SURFACE ( 'NONE', #31890, 11.75000000000000000, 2.125000000000000000 ) ;
#8712=FACE_OUTER_BOUND ( 'NONE', #60714, .T. ) ;
#8713=CARTESIAN_POINT ( 'NONE',  ( 114.7458293810857128, -30.61868467657531312, 244.3613395616259822 ) ) ;
#8714=ORIENTED_EDGE ( 'NONE', *, *, #72286, .F. ) ;
#8715=ORIENTED_EDGE ( 'NONE', *, *, #48760, .T. ) ;
#8717=CARTESIAN_POINT ( 'NONE',  ( 99.08321105494920289, -40.57595765811257138, 168.1158690201829700 ) ) ;
#8718=VECTOR ( 'NONE', #36237, 1000.000000000000000 ) ;
#8720=CARTESIAN_POINT ( 'NONE',  ( 98.47292639957201743, -32.93111785796080682, 52.41491663922997901 ) ) ;
#8723=CIRCLE ( 'NONE', #59460, 13.63963572536219715 ) ;
#8724=DIRECTION ( 'NONE',  ( 1.067522139062650671E-15, 1.000000000000000000, 0.000000000000000000 ) ) ;
#8725=FACE_OUTER_BOUND ( 'NONE', #39998, .T. ) ;
#8727=CARTESIAN_POINT ( 'NONE',  ( 115.9412561796928429, -30.17946786548967353, 259.3203871806730945 ) ) ;
#8729=ORIENTED_EDGE ( 'NONE', *, *, #77481, .F. ) ;
#8730=ORIENTED_EDGE ( 'NONE', *, *, #38917, .T. ) ;
#8732=DIRECTION ( 'NONE',  ( -2.900000000000000265E-14, 2.000000000000000155E-15, -1.000000000000000000 ) ) ;
#8734=CIRCLE ( 'NONE', #50790, 4.750000000000004441 ) ;
#8735=DIRECTION ( 'NONE',  ( 0.000000000000000000, -1.000000000000000000, 0.000000000000000000 ) ) ;
#8737=ADVANCED_FACE ( 'NONE', ( #70192 ), #7964, .F. ) ;
#8738=CARTESIAN_POINT ( 'NONE',  ( 97.32756240345236165, -42.09278592124177010, 22.72705384733897205 ) ) ;
#8740=VERTEX_POINT ( 'NONE', #48371 ) ;
#8741=CARTESIAN_POINT ( 'NONE',  ( 103.9444121564427235, -47.38074615057520589, 58.33753003781600199 ) ) ;
#8742=FACE_OUTER_BOUND ( 'NONE', #64337, .T. ) ;
#8743=CARTESIAN_POINT ( 'NONE',  ( 100.8231516252168234, -45.85084492350206631, 242.1108633711489517 ) ) ;
#8744=VERTEX_POINT ( 'NONE', #62022 ) ;
#8745=VECTOR ( 'NONE', #82403, 1000.000000000000000 ) ;
#8747=CARTESIAN_POINT ( 'NONE',  ( 115.0382687573691527, -42.90718446363899830, 19.30286595434970209 ) ) ;
#8749=CARTESIAN_POINT ( 'NONE',  ( 112.4846873277006267, -29.98081840548436006, 117.3442808457819666 ) ) ;
#8750=CARTESIAN_POINT ( 'NONE',  ( 95.38360599640527937, -38.85844429501600672, 197.4699109901969791 ) ) ;
#8751=DIRECTION ( 'NONE',  ( 0.000000000000000000, 0.000000000000000000, -1.000000000000000000 ) ) ;
#8752=VERTEX_POINT ( 'NONE', #27953 ) ;
#8753=CYLINDRICAL_SURFACE ( 'NONE', #52313, 3.250000000000002665 ) ;
#8754=VECTOR ( 'NONE', #25014, 1000.000000000000000 ) ;
#8756=ORIENTED_EDGE ( 'NONE', *, *, #62994, .F. ) ;
#8757=EDGE_CURVE ( 'NONE', #36458, #75252, #56552, .T. ) ;
#8758=FACE_BOUND ( 'NONE', #60618, .T. ) ;
#8762=CARTESIAN_POINT ( 'NONE',  ( 109.7225942113134067, -27.00020313397157423, 24.86497719015990882 ) ) ;
#8763=CARTESIAN_POINT ( 'NONE',  ( 112.7360809596688966, -29.66769577629168353, 118.9486103042669782 ) ) ;
#8764=CARTESIAN_POINT ( 'NONE',  ( 118.6786315247609167, -39.21782601141705271, 258.6584824187679033 ) ) ;
#8768=AXIS2_PLACEMENT_3D ( 'NONE', #22314, #62287, #42281 ) ;
#8769=ORIENTED_EDGE ( 'NONE', *, *, #39109, .F. ) ;
#8770=CARTESIAN_POINT ( 'NONE',  ( 150.5667039024483529, -47.82844715993594775, 249.9678068554149490 ) ) ;
#8771=DIRECTION ( 'NONE',  ( -0.7071067812152160847, 0.7071067811578790607, 0.000000000000000000 ) ) ;
#8774=AXIS2_PLACEMENT_3D ( 'NONE', #17804, #38243, #3727 ) ;
#8775=CARTESIAN_POINT ( 'NONE',  ( 109.7815504499144339, -47.49240650911489325, 92.78514908543495210 ) ) ;
#8779=CARTESIAN_POINT ( 'NONE',  ( 96.88875151864165503, -30.65867585538550344, 280.8984824187682534 ) ) ;
#8782=CARTESIAN_POINT ( 'NONE',  ( 172.5667039024478129, -36.32844715993500273, 300.4678068554149490 ) ) ;
#8783=ADVANCED_FACE ( 'NONE', ( #7519 ), #48825, .T. ) ;
#8784=LINE ( 'NONE', #70554, #17265 ) ;
#8785=FACE_OUTER_BOUND ( 'NONE', #9630, .T. ) ;
#8786=CARTESIAN_POINT ( 'NONE',  ( 97.81170242524891023, -40.51743837274789684, 121.6354095930283137 ) ) ;
#8789=CARTESIAN_POINT ( 'NONE',  ( 131.9720459102087489, -38.52018918697933714, 7.480061334670521589 ) ) ;
#8790=AXIS2_PLACEMENT_3D ( 'NONE', #41784, #89066, #13654 ) ;
#8793=CARTESIAN_POINT ( 'NONE',  ( 46.48091746482047171, -48.32844715994088602, 129.9678068554150911 ) ) ;
#8794=DIRECTION ( 'NONE',  ( -1.000000000000000000, 1.122464679914735423E-15, 0.000000000000000000 ) ) ;
#8795=FACE_OUTER_BOUND ( 'NONE', #50182, .T. ) ;
#8797=ADVANCED_FACE ( 'NONE', ( #70650 ), #83379, .F. ) ;
#8799=CARTESIAN_POINT ( 'NONE',  ( 96.64195684025510502, -42.47035700268206426, 26.72705384733997747 ) ) ;
#8800=CARTESIAN_POINT ( 'NONE',  ( 101.7695353289030322, -45.70857994070590991, 158.1527681330539963 ) ) ;
#8801=CARTESIAN_POINT ( 'NONE',  ( 111.4245298313290107, -46.22390286880558818, 23.91848241876792969 ) ) ;
#8804=CARTESIAN_POINT ( 'NONE',  ( 82.79255470691698804, -36.36732994130517227, 6.785344856283535897 ) ) ;
#8805=CARTESIAN_POINT ( 'NONE',  ( 116.3212776292297406, -32.94146857471347545, 140.1356252759109680 ) ) ;
#8806=ADVANCED_FACE ( 'NONE', ( #62918 ), #250, .F. ) ;
#8807=VERTEX_POINT ( 'NONE', #29316 ) ;
#8811=AXIS2_PLACEMENT_3D ( 'NONE', #84031, #9508, #85831 ) ;
#8812=CARTESIAN_POINT ( 'NONE',  ( 99.60253261678104764, -31.60088882024776780, 165.2819436375999658 ) ) ;
#8816=CARTESIAN_POINT ( 'NONE',  ( 98.27975524859429868, -42.29919363830185119, 182.7756252759109543 ) ) ;
#8818=DIRECTION ( 'NONE',  ( 1.000000000000000078E-15, 1.000000000000000083E-30, -1.000000000000000000 ) ) ;
#8823=CARTESIAN_POINT ( 'NONE',  ( 110.8996159922621842, -45.96566293992800922, 97.88950923702800822 ) ) ;
#8824=CARTESIAN_POINT ( 'NONE',  ( 116.9564367646783722, -33.61053620760070260, 129.0575300378169743 ) ) ;
#8825=VERTEX_POINT ( 'NONE', #22501 ) ;
#8827=VERTEX_POINT ( 'NONE', #27507 ) ;
#8828=CARTESIAN_POINT ( 'NONE',  ( 106.6003420031022415, -27.34545878416701115, 41.55967854399195005 ) ) ;
#8829=DIRECTION ( 'NONE',  ( 1.000000000000000078E-15, 0.000000000000000000, -1.000000000000000000 ) ) ;
#8830=CARTESIAN_POINT ( 'NONE',  ( 116.8431970675091662, -40.18699730018602168, 174.5680062282909546 ) ) ;
#8831=LINE ( 'NONE', #22450, #63570 ) ;
#8833=CARTESIAN_POINT ( 'NONE',  ( 115.0889048001385646, -30.61763654108453281, 110.3441337246927674 ) ) ;
#8837=CARTESIAN_POINT ( 'NONE',  ( 117.5859182825552978, -33.41202194707543782, 129.0575300378159795 ) ) ;
#8839=ORIENTED_EDGE ( 'NONE', *, *, #79967, .F. ) ;
#8840=EDGE_LOOP ( 'NONE', ( #73351, #26546, #41726, #34278, #45152, #42465 ) ) ;
#8841=AXIS2_PLACEMENT_3D ( 'NONE', #68562, #18159, #45843 ) ;
#8845=CARTESIAN_POINT ( 'NONE',  ( 97.81168839172025287, -40.51739946886939947, 131.6358419732753475 ) ) ;
#8848=CARTESIAN_POINT ( 'NONE',  ( 99.55502339443899018, -39.99451353983162960, 229.4709475124479638 ) ) ;
#8851=CARTESIAN_POINT ( 'NONE',  ( 96.01388918828124019, -36.58377270012555726, 156.3280062282919687 ) ) ;
#8852=DIRECTION ( 'NONE',  ( 1.000000000000000000, 6.493183223601999383E-14, 9.351236661543306751E-17 ) ) ;
#8855=ORIENTED_EDGE ( 'NONE', *, *, #24492, .F. ) ;
#8858=ORIENTED_EDGE ( 'NONE', *, *, #75266, .F. ) ;
#8860=CARTESIAN_POINT ( 'NONE',  ( 162.9033555647771436, -33.89581943344378345, 342.9256252759109884 ) ) ;
#8861=CARTESIAN_POINT ( 'NONE',  ( 131.6146038193916468, -35.48272374590327871, 7.134497377245147653 ) ) ;
#8863=CARTESIAN_POINT ( 'NONE',  ( 101.8980524138101345, -43.06915566006364315, 9.850947512448971821 ) ) ;
#8865=ORIENTED_EDGE ( 'NONE', *, *, #87411, .T. ) ;
#8866=EDGE_CURVE ( 'NONE', #18132, #14582, #70387, .T. ) ;
#8867=CARTESIAN_POINT ( 'NONE',  ( 115.8629299651497035, -40.02386399094653058, 9.635625275910941312 ) ) ;
#8868=CARTESIAN_POINT ( 'NONE',  ( 172.5667039024480118, -36.32844715993499563, 180.4678068554150059 ) ) ;
#8869=EDGE_LOOP ( 'NONE', ( #26561, #21478, #18962, #3621 ) ) ;
#8870=ORIENTED_EDGE ( 'NONE', *, *, #6399, .F. ) ;
#8872=CARTESIAN_POINT ( 'NONE',  ( 99.08985776380760058, -42.79589758595945170, 111.8440019053259391 ) ) ;
#8873=EDGE_LOOP ( 'NONE', ( #44938, #65304 ) ) ;
#8876=CARTESIAN_POINT ( 'NONE',  ( 99.16797791762762415, -38.78938375721887155, 274.3480903695913184 ) ) ;
#8877=CARTESIAN_POINT ( 'NONE',  ( 117.8019377669635190, -34.00081044253764162, 169.0365776568629599 ) ) ;
#8879=CARTESIAN_POINT ( 'NONE',  ( 99.11802762103501152, -45.48540990049890809, 156.9899109901969609 ) ) ;
#8880=DIRECTION ( 'NONE',  ( 0.000000000000000000, 1.000000000000000000, 0.000000000000000000 ) ) ;
#8881=CARTESIAN_POINT ( 'NONE',  ( 104.1858290503737408, -26.67344577167302688, 221.2984824187679465 ) ) ;
#8882=CARTESIAN_POINT ( 'NONE',  ( 151.0371591254584871, -46.82818131005592477, 180.4678068554149775 ) ) ;
#8886=EDGE_LOOP ( 'NONE', ( #17390, #83813, #44144, #69741 ) ) ;
#8887=ORIENTED_EDGE ( 'NONE', *, *, #38171, .T. ) ;
#8888=CIRCLE ( 'NONE', #14650, 0.5000000000000004441 ) ;
#8889=VECTOR ( 'NONE', #48143, 1000.000000000000000 ) ;
#8890=CARTESIAN_POINT ( 'NONE',  ( 98.51514891278741004, -45.00612994150532842, 191.9384824187679612 ) ) ;
#8891=ORIENTED_EDGE ( 'NONE', *, *, #42690, .F. ) ;
#8892=CARTESIAN_POINT ( 'NONE',  ( 103.8073253818723316, -26.82667379764869153, 165.3299109901969643 ) ) ;
#8893=DIRECTION ( 'NONE',  ( 4.299999999999999979E-14, -1.000000000000000000, 4.400000000000000367E-29 ) ) ;
#8896=DIRECTION ( 'NONE',  ( 0.000000000000000000, 0.000000000000000000, 1.000000000000000000 ) ) ;
#8897=CARTESIAN_POINT ( 'NONE',  ( 97.86538016267786588, -40.64618032142375625, 56.64632583547473388 ) ) ;
#8898=CARTESIAN_POINT ( 'NONE',  ( 116.0363244534468237, -41.99923036749492411, 234.4041967044819899 ) ) ;
#8899=CARTESIAN_POINT ( 'NONE',  ( 51.06648329127400388, 19.62155284005901024, 333.4006252759110112 ) ) ;
#8900=EDGE_CURVE ( 'NONE', #462, #7080, #13848, .T. ) ;
#8901=PLANE ( 'NONE',  #67044 ) ;
#8902=CARTESIAN_POINT ( 'NONE',  ( 112.1356898331065537, -28.01072921633739554, 270.6563675837870164 ) ) ;
#8907=CYLINDRICAL_SURFACE ( 'NONE', #78190, 2.030000000001807248 ) ;
#8908=AXIS2_PLACEMENT_3D ( 'NONE', #35616, #70145, #89258 ) ;
#8909=CARTESIAN_POINT ( 'NONE',  ( 115.4825246836782640, -36.90214395232434441, 195.5838068554167535 ) ) ;
#8911=ADVANCED_FACE ( 'NONE', ( #78375 ), #10638, .T. ) ;
#8913=CARTESIAN_POINT ( 'NONE',  ( 103.8004457107024194, -26.80577029241926112, 165.3299109901969643 ) ) ;
#8914=CARTESIAN_POINT ( 'NONE',  ( 97.26643838138058129, -31.61739275409173544, 86.93181575210095957 ) ) ;
#8915=CARTESIAN_POINT ( 'NONE',  ( 98.50201126197670476, -30.70924794336980668, 201.8384824187679385 ) ) ;
#8916=CARTESIAN_POINT ( 'NONE',  ( 134.0664832912740110, -46.72944715994100306, -0.8743747240890020755 ) ) ;
#8917=CARTESIAN_POINT ( 'NONE',  ( 138.8167039024479834, -50.82844715994100682, 33.40080685541480676 ) ) ;
#8920=CARTESIAN_POINT ( 'NONE',  ( 97.31584371032013792, -39.30597597718078617, 71.53145860744848505 ) ) ;
#8922=ORIENTED_EDGE ( 'NONE', *, *, #49156, .T. ) ;
#8924=CARTESIAN_POINT ( 'NONE',  ( 97.81315821180474757, -40.51681016098617505, 66.63608906629065132 ) ) ;
#8927=ORIENTED_EDGE ( 'NONE', *, *, #21621, .T. ) ;
#8928=ADVANCED_FACE ( 'NONE', ( #10201 ), #51950, .F. ) ;
#8929=DIRECTION ( 'NONE',  ( 0.000000000000000000, 0.000000000000000000, -1.000000000000000000 ) ) ;
#8931=CARTESIAN_POINT ( 'NONE',  ( 106.0785370228625055, -48.51385081415330092, 108.5099109901969712 ) ) ;
#8933=AXIS2_PLACEMENT_3D ( 'NONE', #78393, #86976, #37923 ) ;
#8935=FACE_OUTER_BOUND ( 'NONE', #49948, .T. ) ;
#8936=CARTESIAN_POINT ( 'NONE',  ( 116.8435662018514307, -36.99793375417353758, 43.80419670448193159 ) ) ;
#8937=ORIENTED_EDGE ( 'NONE', *, *, #49035, .F. ) ;
#8939=ORIENTED_EDGE ( 'NONE', *, *, #89621, .F. ) ;
#8940=FACE_OUTER_BOUND ( 'NONE', #79633, .T. ) ;
#8941=DIRECTION ( 'NONE',  ( 0.7071067811571405404, 0.7071067812159546051, 0.000000000000000000 ) ) ;
#8942=CARTESIAN_POINT ( 'NONE',  ( 142.8696205427243626, 0.6543191929522288453, 540.9756252759101471 ) ) ;
#8944=DIRECTION ( 'NONE',  ( 0.000000000000000000, 0.000000000000000000, -1.000000000000000000 ) ) ;
#8945=CARTESIAN_POINT ( 'NONE',  ( 99.09592356364612442, -30.55014542244788700, 51.80351315582143457 ) ) ;
#8946=VECTOR ( 'NONE', #1653, 1000.000000000000000 ) ;
#8948=CARTESIAN_POINT ( 'NONE',  ( 100.4791399132688809, -44.80881982087489490, 12.03276813305398463 ) ) ;
#8949=EDGE_LOOP ( 'NONE', ( #85518, #2182, #67689, #32378, #40237 ) ) ;
#8951=CIRCLE ( 'NONE', #16208, 2.030000000000003801 ) ;
#8952=CYLINDRICAL_SURFACE ( 'NONE', #13358, 11.57110091390434903 ) ;
#8953=EDGE_CURVE ( 'NONE', #26697, #53561, #31522, .T. ) ;
#8954=CARTESIAN_POINT ( 'NONE',  ( 98.87701435734486211, -36.85308710711977653, 134.1566617981629577 ) ) ;
#8955=AXIS2_PLACEMENT_3D ( 'NONE', #65380, #36785, #29077 ) ;
#8956=EDGE_CURVE ( 'NONE', #64680, #13607, #78666, .T. ) ;
#8960=VERTEX_POINT ( 'NONE', #64721 ) ;
#8961=CARTESIAN_POINT ( 'NONE',  ( 164.9667039024459996, -28.27351298637401200, -5.074374724088000832 ) ) ;
#8963=VERTEX_POINT ( 'NONE', #85188 ) ;
#8964=VECTOR ( 'NONE', #60745, 1000.000000000000000 ) ;
#8965=CARTESIAN_POINT ( 'NONE',  ( 108.8812380984771835, -28.05563920549329993, 136.3444404487549662 ) ) ;
#8967=CARTESIAN_POINT ( 'NONE',  ( 98.07812720205548374, -31.40528397058157850, 81.90133956162493689 ) ) ;
#8968=VECTOR ( 'NONE', #63293, 1000.000000000000000 ) ;
#8969=CARTESIAN_POINT ( 'NONE',  ( 101.9936209174699258, -45.44607152528067928, 83.15645860711320836 ) ) ;
#8970=ORIENTED_EDGE ( 'NONE', *, *, #39952, .F. ) ;
#8972=ORIENTED_EDGE ( 'NONE', *, *, #28236, .T. ) ;
#8975=CARTESIAN_POINT ( 'NONE',  ( 100.1721853667017825, -41.09961673838238028, 184.5938046553059735 ) ) ;
#8976=CARTESIAN_POINT ( 'NONE',  ( 113.4288541212755348, -27.66216098611360152, 84.57753003781698453 ) ) ;
#8977=ORIENTED_EDGE ( 'NONE', *, *, #88960, .F. ) ;
#8978=CARTESIAN_POINT ( 'NONE',  ( 118.7081646409642133, -34.65111545711807395, 48.96705384733895983 ) ) ;
#8979=CARTESIAN_POINT ( 'NONE',  ( 96.59701100649584760, -36.21046171878319342, 167.2870538473399620 ) ) ;
#8982=CARTESIAN_POINT ( 'NONE',  ( 96.02786343543940006, -37.29764797185995207, 117.3794347997199594 ) ) ;
#8983=VECTOR ( 'NONE', #32322, 1000.000000000000000 ) ;
#8984=FACE_OUTER_BOUND ( 'NONE', #929, .T. ) ;
#8985=ORIENTED_EDGE ( 'NONE', *, *, #84507, .F. ) ;
#8987=ORIENTED_CLOSED_SHELL ( 'NONE', *, #31468, .F. );
#8990=ORIENTED_EDGE ( 'NONE', *, *, #60455, .F. ) ;
#8991=ORIENTED_EDGE ( 'NONE', *, *, #40768, .F. ) ;
#8993=DIRECTION ( 'NONE',  ( 0.000000000000000000, 1.000000000000000000, 0.000000000000000000 ) ) ;
#8994=CARTESIAN_POINT ( 'NONE',  ( 97.48652011608379553, -32.61680585812226241, 16.00419670448194154 ) ) ;
#8995=CARTESIAN_POINT ( 'NONE',  ( 116.3212776292267989, -32.94146857470629186, 109.1356252759109680 ) ) ;
#8997=CARTESIAN_POINT ( 'NONE',  ( 97.35451824726682446, -37.88753622196094994, 41.42133956162496844 ) ) ;
#8998=CARTESIAN_POINT ( 'NONE',  ( 104.4896289049376605, -26.97888955764241814, 110.2814849738620069 ) ) ;
#8999=CARTESIAN_POINT ( 'NONE',  ( 108.2752786314947286, -47.69320359391959840, 153.6518157521009584 ) ) ;
#9000=FACE_OUTER_BOUND ( 'NONE', #48637, .T. ) ;
#9001=EDGE_CURVE ( 'NONE', #30523, #73517, #78817, .T. ) ;
#9002=FACE_OUTER_BOUND ( 'NONE', #71931, .T. ) ;
#9004=LINE ( 'NONE', #30773, #56989 ) ;
#9010=CARTESIAN_POINT ( 'NONE',  ( 115.0114139542580318, -28.97761122332106964, 194.4537205140059370 ) ) ;
#9011=ORIENTED_EDGE ( 'NONE', *, *, #6692, .T. ) ;
#9012=EDGE_CURVE ( 'NONE', #27479, #49045, #30647, .T. ) ;
#9013=FACE_OUTER_BOUND ( 'NONE', #79748, .T. ) ;
#9014=CARTESIAN_POINT ( 'NONE',  ( 101.6393319275751992, -45.65599671332518028, 243.1413395616249886 ) ) ;
#9015=CARTESIAN_POINT ( 'NONE',  ( 117.3817195963474518, -32.63147225404833307, 95.13943479972097350 ) ) ;
#9016=LINE ( 'NONE', #29901, #60622 ) ;
#9025=ORIENTED_EDGE ( 'NONE', *, *, #59757, .F. ) ;
#9026=CARTESIAN_POINT ( 'NONE',  ( 168.3595971214449207, -48.62134037892947447, 129.9678068554150059 ) ) ;
#9027=CARTESIAN_POINT ( 'NONE',  ( 107.5100279102752552, -47.14509671329473406, 233.6099109901969655 ) ) ;
#9028=DIRECTION ( 'NONE',  ( 0.000000000000000000, 0.000000000000000000, 1.000000000000000000 ) ) ;
#9030=CARTESIAN_POINT ( 'NONE',  ( 194.0371591254585155, -46.82818131005407736, 129.9678068554150343 ) ) ;
#9032=CARTESIAN_POINT ( 'NONE',  ( 188.5667039024482960, -42.82844715993431350, 259.7178068554150059 ) ) ;
#9035=CARTESIAN_POINT ( 'NONE',  ( 114.1055592783800137, -46.29424852498188869, 33.08133956162495792 ) ) ;
#9038=ORIENTED_EDGE ( 'NONE', *, *, #6562, .F. ) ;
#9040=CARTESIAN_POINT ( 'NONE',  ( 100.5881272547050429, -39.38103216960048059, -2.364374724089013391 ) ) ;
#9042=CARTESIAN_POINT ( 'NONE',  ( 101.4562479827646371, -44.74122725731964323, 278.0899109901961879 ) ) ;
#9043=AXIS2_PLACEMENT_3D ( 'NONE', #44383, #9886, #24849 ) ;
#9045=CARTESIAN_POINT ( 'NONE',  ( 103.4440497394146092, -45.85039829771042719, 113.2756252759109827 ) ) ;
#9047=CARTESIAN_POINT ( 'NONE',  ( 116.7947425855253130, -39.38919346347031336, 28.61468008947841568 ) ) ;
#9048=ORIENTED_EDGE ( 'NONE', *, *, #61121, .T. ) ;
#9050=CARTESIAN_POINT ( 'NONE',  ( 77.59184326792608033, -35.51852171453446516, 2.740177351673668937 ) ) ;
#9051=ORIENTED_EDGE ( 'NONE', *, *, #24870, .T. ) ;
#9053=CARTESIAN_POINT ( 'NONE',  ( 101.9087497524793804, -29.77971984236790703, 33.41475703625796001 ) ) ;
#9054=LINE ( 'NONE', #16754, #40643 ) ;
#9056=DIRECTION ( 'NONE',  ( 0.000000000000000000, 0.000000000000000000, -1.000000000000000000 ) ) ;
#9057=DIRECTION ( 'NONE',  ( 1.000000000000000000, 0.000000000000000000, 0.000000000000000000 ) ) ;
#9058=ORIENTED_EDGE ( 'NONE', *, *, #7035, .F. ) ;
#9059=DIRECTION ( 'NONE',  ( 1.000000000000000078E-15, 0.000000000000000000, -1.000000000000000000 ) ) ;
#9060=CARTESIAN_POINT ( 'NONE',  ( 164.9667039024459996, -26.71338133339301635, 342.9256252759119548 ) ) ;
#9062=CARTESIAN_POINT ( 'NONE',  ( 109.9110735108787793, -46.79593677437021881, 72.79562527591099297 ) ) ;
#9064=CARTESIAN_POINT ( 'NONE',  ( 111.0503013157718044, -29.17396400730615369, 59.11241982807696616 ) ) ;
#9066=CARTESIAN_POINT ( 'NONE',  ( 98.96845470676149148, -30.25173782105007803, 195.7775300378159784 ) ) ;
#9068=CARTESIAN_POINT ( 'NONE',  ( 107.0664832912748068, -36.72944715993923381, 14.92562527591097066 ) ) ;
#9070=DIRECTION ( 'NONE',  ( 1.000000000000000078E-15, -1.000000000000000083E-30, -1.000000000000000000 ) ) ;
#9071=CARTESIAN_POINT ( 'NONE',  ( 114.4457317200277089, -27.39361268404408634, 270.5441967044823741 ) ) ;
#9072=ORIENTED_EDGE ( 'NONE', *, *, #20266, .T. ) ;
#9073=CIRCLE ( 'NONE', #53956, 0.9999999999991942001 ) ;
#9076=CARTESIAN_POINT ( 'NONE',  ( 117.0748215982922176, -30.29170057715430531, 140.2813395616249750 ) ) ;
#9077=ADVANCED_FACE ( 'NONE', ( #48312, #19743 ), #41070, .F. ) ;
#9078=CARTESIAN_POINT ( 'NONE',  ( 142.8832909413445122, -79.11588146349311046, 394.9756252759100903 ) ) ;
#9081=VERTEX_POINT ( 'NONE', #53784 ) ;
#9083=DIRECTION ( 'NONE',  ( 0.9999999853157766072, 0.0001713722456143218888, -0.000000000000000000 ) ) ;
#9084=DIRECTION ( 'NONE',  ( 0.000000000000000000, 0.000000000000000000, -1.000000000000000000 ) ) ;
#9085=DIRECTION ( 'NONE',  ( 1.000000000000000000, -5.337610695313248426E-16, 0.000000000000000000 ) ) ;
#9086=DIRECTION ( 'NONE',  ( 0.000000000000000000, 0.000000000000000000, -1.000000000000000000 ) ) ;
#9087=CARTESIAN_POINT ( 'NONE',  ( 118.2085198165198676, -40.76548936363617059, 19.54991099019698453 ) ) ;
#9088=EDGE_CURVE ( 'NONE', #23895, #63431, #34258, .T. ) ;
#9090=CARTESIAN_POINT ( 'NONE',  ( 83.73314995794051185, 12.92155284005802685, 336.5756252759109657 ) ) ;
#9092=CARTESIAN_POINT ( 'NONE',  ( 101.3372171518963398, -46.20893634704900421, 198.1318157521009482 ) ) ;
#9093=ADVANCED_FACE ( 'NONE', ( #75156 ), #38338, .T. ) ;
#9094=CARTESIAN_POINT ( 'NONE',  ( 115.0372571628051048, -42.90846324673419332, 43.30193824323413310 ) ) ;
#9098=DIRECTION ( 'NONE',  ( 0.000000000000000000, 1.000000000000000000, 0.000000000000000000 ) ) ;
#9099=DIRECTION ( 'NONE',  ( -6.493183223601999383E-14, 1.000000000000000000, -2.193183223602000424E-29 ) ) ;
#9103=FACE_OUTER_BOUND ( 'NONE', #16025, .T. ) ;
#9104=CARTESIAN_POINT ( 'NONE',  ( 98.55846751192062527, -35.97459669770627499, 230.6781341137909465 ) ) ;
#9105=VECTOR ( 'NONE', #58256, 1000.000000000000000 ) ;
#9107=CARTESIAN_POINT ( 'NONE',  ( 97.82856912889593559, -29.34641599088761765, 41.78991099019596334 ) ) ;
#9109=CARTESIAN_POINT ( 'NONE',  ( 111.0995558192250456, -25.53287967237518430, 99.80133956162498521 ) ) ;
#9110=VERTEX_POINT ( 'NONE', #12038 ) ;
#9111=CARTESIAN_POINT ( 'NONE',  ( 131.5555141844761522, -19.85480617632529743, 7.067502061084848464 ) ) ;
#9112=VERTEX_POINT ( 'NONE', #54226 ) ;
#9114=CARTESIAN_POINT ( 'NONE',  ( 103.9854521423141875, -27.20984610156289207, 276.3255691088649542 ) ) ;
#9115=EDGE_CURVE ( 'NONE', #16229, #54739, #7009, .T. ) ;
#9116=VERTEX_POINT ( 'NONE', #87894 ) ;
#9117=CARTESIAN_POINT ( 'NONE',  ( 41.56670390244689628, -36.32844715994109208, 180.4678068554150911 ) ) ;
#9118=EDGE_LOOP ( 'NONE', ( #16068, #24050, #85374, #45043 ) ) ;
#9121=DIRECTION ( 'NONE',  ( 0.9999999853157766072, 0.0001713722456133601202, -9.999999853157765648E-16 ) ) ;
#9122=ORIENTED_EDGE ( 'NONE', *, *, #84900, .T. ) ;
#9123=CARTESIAN_POINT ( 'NONE',  ( 116.9960073371140652, -33.48122977351050622, 89.07848241876791917 ) ) ;
#9124=CARTESIAN_POINT ( 'NONE',  ( 97.70660944625170430, -40.25144590732936933, 166.6128667725130299 ) ) ;
#9128=EDGE_CURVE ( 'NONE', #7579, #9112, #70461, .T. ) ;
#9129=CIRCLE ( 'NONE', #16390, 0.5000000000000004441 ) ;
#9130=CARTESIAN_POINT ( 'NONE',  ( 46.03715912545348488, -48.62818131006090283, 117.4678068554150485 ) ) ;
#9131=ADVANCED_FACE ( 'NONE', ( #13824 ), #12489, .T. ) ;
#9132=CARTESIAN_POINT ( 'NONE',  ( 184.5664832912729878, -71.37844715994266664, 361.9756252759109998 ) ) ;
#9133=EDGE_CURVE ( 'NONE', #87762, #45263, #82080, .T. ) ;
#9134=CARTESIAN_POINT ( 'NONE',  ( 131.0667039024480118, -61.87844715994100397, 207.5838068554149913 ) ) ;
#9135=EDGE_CURVE ( 'NONE', #47300, #27344, #25310, .T. ) ;
#9136=DIRECTION ( 'NONE',  ( 0.1858654558203329255, -0.9825752044157738396, 0.000000000000000000 ) ) ;
#9138=LINE ( 'NONE', #57256, #77084 ) ;
#9142=CARTESIAN_POINT ( 'NONE',  ( 113.2764755850017480, -45.03455287549797248, 184.0994347997199725 ) ) ;
#9144=ORIENTED_EDGE ( 'NONE', *, *, #74811, .F. ) ;
#9145=CARTESIAN_POINT ( 'NONE',  ( 111.8051046833288353, -27.50533224649500497, 15.71086337114796549 ) ) ;
#9146=DIRECTION ( 'NONE',  ( 0.000000000000000000, 0.000000000000000000, -1.000000000000000000 ) ) ;
#9148=CARTESIAN_POINT ( 'NONE',  ( 109.6408691443087804, -46.48062605549592519, 12.78166324958517919 ) ) ;
#9150=CARTESIAN_POINT ( 'NONE',  ( 106.3491918589965763, -46.48387837312656501, 222.5184824187689401 ) ) ;
#9151=ORIENTED_EDGE ( 'NONE', *, *, #22173, .T. ) ;
#9153=CARTESIAN_POINT ( 'NONE',  ( 115.6736222539786638, -40.49689781175994341, 204.9177737820879486 ) ) ;
#9155=CARTESIAN_POINT ( 'NONE',  ( 134.0664832912740110, 0.2215528400590013880, 2.408125275911999097 ) ) ;
#9156=CARTESIAN_POINT ( 'NONE',  ( 111.8905564713631549, -28.66688903671830246, 51.09110711541997318 ) ) ;
#9159=ADVANCED_FACE ( 'NONE', ( #18850 ), #60613, .F. ) ;
#9160=AXIS2_PLACEMENT_3D ( 'NONE', #16933, #38695, #24629 ) ;
#9163=VERTEX_POINT ( 'NONE', #35148 ) ;
#9164=DIRECTION ( 'NONE',  ( -0.7071067811865171526, -0.7071067811865779928, -7.071067811865164719E-16 ) ) ;
#9165=CARTESIAN_POINT ( 'NONE',  ( 97.70656171685999425, -40.25131786594292294, 37.61256612285666989 ) ) ;
#9166=CARTESIAN_POINT ( 'NONE',  ( 96.27200394136420414, -34.46162041542910970, 261.1737205140064475 ) ) ;
#9170=CARTESIAN_POINT ( 'NONE',  ( 100.8874678751566165, -44.70022136795945755, 82.05229194164871842 ) ) ;
#9171=CARTESIAN_POINT ( 'NONE',  ( 177.4809174648214309, -49.32844715993478957, 249.9678068554149775 ) ) ;
#9172=CARTESIAN_POINT ( 'NONE',  ( 41.56648329127381203, -27.82844715994070484, 201.9256252759119832 ) ) ;
#9174=CARTESIAN_POINT ( 'NONE',  ( 97.95204982468537480, -33.09064556074058316, 37.02419670448192335 ) ) ;
#9177=CARTESIAN_POINT ( 'NONE',  ( 99.03245663461365211, -44.38790092286875932, 32.92038718067297509 ) ) ;
#9178=EDGE_CURVE ( 'NONE', #21130, #70069, #22894, .T. ) ;
#9179=DIRECTION ( 'NONE',  ( -4.299999999999999979E-14, 1.000000000000000000, -4.400000000000000367E-29 ) ) ;
#9180=AXIS2_PLACEMENT_3D ( 'NONE', #75373, #18610, #46292 ) ;
#9181=CARTESIAN_POINT ( 'NONE',  ( 97.46629803964546568, -32.60812463323921406, 16.00419670448194154 ) ) ;
#9182=EDGE_CURVE ( 'NONE', #13694, #21258, #48768, .T. ) ;
#9184=EDGE_CURVE ( 'NONE', #78468, #61208, #22336, .T. ) ;
#9185=VECTOR ( 'NONE', #18966, 1000.000000000000000 ) ;
#9189=CARTESIAN_POINT ( 'NONE',  ( 98.90423600646026614, -36.64316113183544843, 109.1366617981629474 ) ) ;
#9190=CARTESIAN_POINT ( 'NONE',  ( 110.1438736645959580, -26.08919931346192911, 210.8403871806729626 ) ) ;
#9198=ADVANCED_FACE ( 'NONE', ( #84231 ), #21090, .T. ) ;
#9199=AXIS2_PLACEMENT_3D ( 'NONE', #196, #41510, #82443 ) ;
#9200=CARTESIAN_POINT ( 'NONE',  ( 107.0664832912739968, -8.350947159940998787, 333.4006252759120343 ) ) ;
#9201=ORIENTED_EDGE ( 'NONE', *, *, #34828, .T. ) ;
#9203=DIRECTION ( 'NONE',  ( -0.9825752044165969590, -0.1858654558159821002, 0.000000000000000000 ) ) ;
#9205=CARTESIAN_POINT ( 'NONE',  ( 104.9213734224019987, -26.94988814155465207, 41.24833046483934851 ) ) ;
#9206=CARTESIAN_POINT ( 'NONE',  ( 113.3268105416314171, -43.27322076882862945, 112.5943245899819516 ) ) ;
#9207=CARTESIAN_POINT ( 'NONE',  ( 109.2165397428488376, -48.40897078886088423, 277.7213395616254843 ) ) ;
#9208=DIRECTION ( 'NONE',  ( 1.000000000000000000, 4.299999999999999979E-14, 1.000000000000000078E-15 ) ) ;
#9209=EDGE_CURVE ( 'NONE', #54183, #78471, #29690, .T. ) ;
#9210=ORIENTED_EDGE ( 'NONE', *, *, #24168, .T. ) ;
#9211=VERTEX_POINT ( 'NONE', #3770 ) ;
#9212=CARTESIAN_POINT ( 'NONE',  ( 33.96670390244699433, -26.71338133339301635, -5.074374724088000832 ) ) ;
#9213=CARTESIAN_POINT ( 'NONE',  ( 97.81281252356875200, -40.52015776331121089, 277.6356251289804504 ) ) ;
#9215=CIRCLE ( 'NONE', #71606, 10.00000000000000888 ) ;
#9216=CARTESIAN_POINT ( 'NONE',  ( 102.3593652026347343, -47.65646955129418672, 287.2527681330535643 ) ) ;
#9219=CARTESIAN_POINT ( 'NONE',  ( 105.7763445623522500, -26.38427570067176831, 270.1756252759109884 ) ) ;
#9220=CARTESIAN_POINT ( 'NONE',  ( 107.0664832912739399, -36.72944715994095333, 302.7856252759109452 ) ) ;
#9221=VECTOR ( 'NONE', #43143, 1000.000000000000000 ) ;
#9222=CARTESIAN_POINT ( 'NONE',  ( 21.03715912545829880, -47.82818131006185780, 237.4678068554150059 ) ) ;
#9223=LINE ( 'NONE', #72343, #47705 ) ;
#9225=DIRECTION ( 'NONE',  ( 2.900000000000000265E-14, -2.000000000000000155E-15, 1.000000000000000000 ) ) ;
#9227=CARTESIAN_POINT ( 'NONE',  ( 131.4346950876521589, -37.52719034724653113, 6.916533740478220338 ) ) ;
#9228=CARTESIAN_POINT ( 'NONE',  ( 97.06107110476884259, -37.99641202601070233, 12.42729194741101750 ) ) ;
#9230=EDGE_CURVE ( 'NONE', #60102, #37281, #77727, .T. ) ;
#9231=CYLINDRICAL_SURFACE ( 'NONE', #73299, 9.999999999999998224 ) ;
#9233=CARTESIAN_POINT ( 'NONE',  ( 113.7702145813751571, -29.06794043779556347, 289.5032443235301116 ) ) ;
#9234=CARTESIAN_POINT ( 'NONE',  ( 106.9749963086187279, -47.15413504876184447, 183.5699109901969734 ) ) ;
#9235=CARTESIAN_POINT ( 'NONE',  ( 99.74686247383996829, -44.23293585951837059, 17.96133956162493206 ) ) ;
#9238=CARTESIAN_POINT ( 'NONE',  ( 82.19340217262779902, -34.98608769071991276, 7.448832051635564611 ) ) ;
#9239=CARTESIAN_POINT ( 'NONE',  ( 81.33214528239159335, -34.28157797492866621, 1.873071231920440560 ) ) ;
#9242=ORIENTED_EDGE ( 'NONE', *, *, #76000, .T. ) ;
#9243=DIRECTION ( 'NONE',  ( 4.012088370409549976E-14, -1.000000000000000000, 0.000000000000000000 ) ) ;
#9244=ORIENTED_EDGE ( 'NONE', *, *, #38935, .F. ) ;
#9245=CARTESIAN_POINT ( 'NONE',  ( 101.5072281473882612, -27.97539281467255279, 61.51467289495899138 ) ) ;
#9247=ORIENTED_EDGE ( 'NONE', *, *, #60667, .F. ) ;
#9249=CARTESIAN_POINT ( 'NONE',  ( 104.4077974134580415, -46.45800023490631503, 48.36476695192959596 ) ) ;
#9250=CARTESIAN_POINT ( 'NONE',  ( 96.69582475441080760, -35.54038568221479011, 202.2356252759109623 ) ) ;
#9251=DIRECTION ( 'NONE',  ( 0.7071067811865434649, 0.7071067811865516806, 7.071067811865440820E-16 ) ) ;
#9252=CARTESIAN_POINT ( 'NONE',  ( 100.8874001080617830, -44.70016547043675814, 147.0523531915934541 ) ) ;
#9253=CARTESIAN_POINT ( 'NONE',  ( 97.07208990303480789, -35.37826891733848811, 151.2194583338160783 ) ) ;
#9254=DIRECTION ( 'NONE',  ( 0.000000000000000000, 0.000000000000000000, 1.000000000000000000 ) ) ;
#9255=CARTESIAN_POINT ( 'NONE',  ( 112.0305244341996342, -48.74436686551289455, 289.6356252759107406 ) ) ;
#9256=CARTESIAN_POINT ( 'NONE',  ( 98.54768855250307524, -41.97703652509544980, 96.76583743525021930 ) ) ;
#9257=CARTESIAN_POINT ( 'NONE',  ( 105.0928733274061670, -25.78792777683064585, 125.2184824187689856 ) ) ;
#9258=ORIENTED_EDGE ( 'NONE', *, *, #69074, .T. ) ;
#9260=AXIS2_PLACEMENT_3D ( 'NONE', #51058, #78355, #84721 ) ;
#9261=CARTESIAN_POINT ( 'NONE',  ( 115.1135551441502258, -33.01825958633261848, 100.6015833058969378 ) ) ;
#9262=DIRECTION ( 'NONE',  ( 0.7071067810573865575, 0.7071067813157084769, 7.071067810573858582E-16 ) ) ;
#9263=CARTESIAN_POINT ( 'NONE',  ( 109.8674951572811267, -26.74480306206640989, 215.8708633711489711 ) ) ;
#9266=CARTESIAN_POINT ( 'NONE',  ( 109.7248605079479518, -27.00080355044804037, 110.8650604066596941 ) ) ;
#9268=CARTESIAN_POINT ( 'NONE',  ( 31.56670390244760327, -32.29483332968575837, 313.9678068554150059 ) ) ;
#9270=CARTESIAN_POINT ( 'NONE',  ( 105.3199149336540046, -48.42511963160334432, 147.4584824187679715 ) ) ;
#9272=ORIENTED_EDGE ( 'NONE', *, *, #78745, .F. ) ;
#9273=ORIENTED_EDGE ( 'NONE', *, *, #40956, .F. ) ;
#9274=PLANE ( 'NONE',  #48755 ) ;
#9276=CARTESIAN_POINT ( 'NONE',  ( 97.80412695053506411, -40.49890085506758908, 131.6340326293677663 ) ) ;
#9277=DIRECTION ( 'NONE',  ( 1.000000000000000000, -1.387778780781444413E-13, 0.000000000000000000 ) ) ;
#9278=CARTESIAN_POINT ( 'NONE',  ( 97.84965203270614609, -37.79993896977983070, 234.2366617981629702 ) ) ;
#9279=EDGE_CURVE ( 'NONE', #89264, #2491, #10578, .T. ) ;
#9280=VECTOR ( 'NONE', #18363, 1000.000000000000000 ) ;
#9281=CARTESIAN_POINT ( 'NONE',  ( 115.7831043715999613, -41.80231542608780870, 269.4064580736135781 ) ) ;
#9282=EDGE_CURVE ( 'NONE', #611, #50783, #45776, .T. ) ;
#9283=CARTESIAN_POINT ( 'NONE',  ( 114.3440588962603215, -29.21527388614784115, 174.4641967044819637 ) ) ;
#9284=EDGE_CURVE ( 'NONE', #5969, #27916, #52325, .T. ) ;
#9286=ORIENTED_EDGE ( 'NONE', *, *, #44441, .F. ) ;
#9287=ORIENTED_EDGE ( 'NONE', *, *, #4054, .T. ) ;
#9289=EDGE_CURVE ( 'NONE', #66368, #28588, #45086, .T. ) ;
#9294=CARTESIAN_POINT ( 'NONE',  ( 83.96770390244803650, -18.82844715994099971, 199.5838068554169524 ) ) ;
#9295=CARTESIAN_POINT ( 'NONE',  ( 116.4478251454372923, -36.21277458701120366, 270.3139642582781335 ) ) ;
#9297=CARTESIAN_POINT ( 'NONE',  ( 101.9936199353088995, -45.44607096256550705, 272.1564585177210915 ) ) ;
#9298=ORIENTED_EDGE ( 'NONE', *, *, #89274, .T. ) ;
#9299=CARTESIAN_POINT ( 'NONE',  ( 106.8296037779400081, -44.95279291948936873, 9.635625275910939536 ) ) ;
#9300=DIRECTION ( 'NONE',  ( -4.093947403305260305E-16, 1.000000000000000000, -6.162975822039159109E-32 ) ) ;
#9301=EDGE_LOOP ( 'NONE', ( #39882, #88682, #62816, #26599, #52697 ) ) ;
#9304=VECTOR ( 'NONE', #2364, 1000.000000000000000 ) ;
#9305=CARTESIAN_POINT ( 'NONE',  ( 116.3225472244029817, -32.94146556017791738, 114.1356252759109822 ) ) ;
#9306=VERTEX_POINT ( 'NONE', #59164 ) ;
#9307=ORIENTED_EDGE ( 'NONE', *, *, #60712, .T. ) ;
#9310=CARTESIAN_POINT ( 'NONE',  ( 114.0673224709094598, -30.00197523691782209, 38.85813411379096749 ) ) ;
#9311=CIRCLE ( 'NONE', #25309, 0.5000000000000197620 ) ;
#9312=CARTESIAN_POINT ( 'NONE',  ( 97.98778932149404852, -30.38336575973633913, 160.8289586092449497 ) ) ;
#9313=CARTESIAN_POINT ( 'NONE',  ( 102.3703197837810279, -46.01248081495484854, 127.2041967044829960 ) ) ;
#9314=CARTESIAN_POINT ( 'NONE',  ( 95.29510253380274776, -38.09663793710245017, 232.4184824187679794 ) ) ;
#9315=CARTESIAN_POINT ( 'NONE',  ( 105.7155902736374600, -46.72387562369726766, 98.47046800182013726 ) ) ;
#9316=CARTESIAN_POINT ( 'NONE',  ( 97.33769884349207757, -34.07164404254515944, 127.1148388564199934 ) ) ;
#9321=CARTESIAN_POINT ( 'NONE',  ( 116.8364808817232756, -40.58936182315601116, 193.5270538473389479 ) ) ;
#9322=EDGE_LOOP ( 'NONE', ( #33471, #65911, #68678, #88721 ) ) ;
#9323=CARTESIAN_POINT ( 'NONE',  ( 114.4629700169191580, -28.51537706926042404, 159.5051490854349652 ) ) ;
#9324=CARTESIAN_POINT ( 'NONE',  ( 97.81168895331838087, -40.51742574516882200, 287.6356252759109680 ) ) ;
#9325=CARTESIAN_POINT ( 'NONE',  ( 136.4140944162674032, -35.29397280665119752, 7.245803660799283286 ) ) ;
#9326=DIRECTION ( 'NONE',  ( 0.000000000000000000, 0.000000000000000000, -1.000000000000000000 ) ) ;
#9327=CARTESIAN_POINT ( 'NONE',  ( 97.98476046313764698, -40.12019249911318752, 277.6356252759110248 ) ) ;
#9328=CARTESIAN_POINT ( 'NONE',  ( 107.0664832912748068, -36.72944715993923381, -4.074374724089028454 ) ) ;
#9329=CARTESIAN_POINT ( 'NONE',  ( 96.78489722101822679, -35.14273565208915073, 262.2041967044821149 ) ) ;
#9331=DIRECTION ( 'NONE',  ( 0.0001713722456129695634, -0.9999999853157764962, 0.000000000000000000 ) ) ;
#9333=DIRECTION ( 'NONE',  ( 0.000000000000000000, -1.000000000000000000, 0.000000000000000000 ) ) ;
#9335=FACE_OUTER_BOUND ( 'NONE', #41361, .T. ) ;
#9336=CARTESIAN_POINT ( 'NONE',  ( 115.2812845904211798, -33.79598010883771053, 195.5838068554166966 ) ) ;
#9337=VERTEX_POINT ( 'NONE', #11020 ) ;
#9338=CARTESIAN_POINT ( 'NONE',  ( 127.0664832912739257, -54.72944906728947245, 14.82207188531768871 ) ) ;
#9339=CARTESIAN_POINT ( 'NONE',  ( 114.9947137121727820, -28.99390558034420451, 194.4537205140059370 ) ) ;
#9340=CARTESIAN_POINT ( 'NONE',  ( 110.7944688027788658, -46.46518603654068613, 58.86705384733998159 ) ) ;
#9341=CARTESIAN_POINT ( 'NONE',  ( 96.14593026560288536, -32.00158989507077223, 207.0013395616249738 ) ) ;
#9342=LINE ( 'NONE', #50213, #28595 ) ;
#9343=ADVANCED_FACE ( 'NONE', ( #25102 ), #37401, .T. ) ;
#9344=DIRECTION ( 'NONE',  ( -1.000000000000000000, 0.000000000000000000, 0.000000000000000000 ) ) ;
#9345=CARTESIAN_POINT ( 'NONE',  ( 165.6738106836199904, -26.00627455219321860, -5.074374724088000832 ) ) ;
#9348=CARTESIAN_POINT ( 'NONE',  ( 134.0664832912739826, -15.97944715994100306, 8.225625275910998013 ) ) ;
#9349=ORIENTED_EDGE ( 'NONE', *, *, #38715, .T. ) ;
#9351=CARTESIAN_POINT ( 'NONE',  ( 108.4199059663018829, -26.73533934207818774, 64.97014767438379579 ) ) ;
#9352=AXIS2_PLACEMENT_3D ( 'NONE', #32660, #10880, #11326 ) ;
#9353=ORIENTED_EDGE ( 'NONE', *, *, #60434, .T. ) ;
#9355=CARTESIAN_POINT ( 'NONE',  ( 104.6424027498074025, -44.91968313032340632, 106.7695626852199808 ) ) ;
#9357=ORIENTED_EDGE ( 'NONE', *, *, #84275, .F. ) ;
#9358=CARTESIAN_POINT ( 'NONE',  ( 99.07096106853141748, -43.38529345585680375, 112.8784824187679732 ) ) ;
#9361=EDGE_CURVE ( 'NONE', #81364, #3107, #18244, .T. ) ;
#9362=CARTESIAN_POINT ( 'NONE',  ( 116.3212776292303090, -32.94146857471486811, 175.1356252759109680 ) ) ;
#9363=CARTESIAN_POINT ( 'NONE',  ( 106.5519926023875712, -26.37212682281782250, 45.12800622829394115 ) ) ;
#9364=ORIENTED_EDGE ( 'NONE', *, *, #15451, .T. ) ;
#9366=ORIENTED_EDGE ( 'NONE', *, *, #9824, .F. ) ;
#9368=VECTOR ( 'NONE', #55946, 1000.000000000000000 ) ;
#9369=CONICAL_SURFACE ( 'NONE', #74646, 7.249999999999998224, 0.7853981633974772558 ) ;
#9370=CARTESIAN_POINT ( 'NONE',  ( 117.0608945236646861, -38.08045311976564307, 108.7189586093281264 ) ) ;
#9371=AXIS2_PLACEMENT_3D ( 'NONE', #31239, #73473, #30807 ) ;
#9372=LINE ( 'NONE', #73369, #4105 ) ;
#9373=CARTESIAN_POINT ( 'NONE',  ( 37.06648329127400388, 12.92155284005802685, 336.5756252759108520 ) ) ;
#9375=LINE ( 'NONE', #87015, #84251 ) ;
#9376=CARTESIAN_POINT ( 'NONE',  ( 98.35000982325539098, -31.65631374779490059, 51.90755703618102501 ) ) ;
#9379=VECTOR ( 'NONE', #33369, 1000.000000000000000 ) ;
#9381=CARTESIAN_POINT ( 'NONE',  ( 115.6551466294303623, -43.65033472170377138, 43.27467289495795200 ) ) ;
#9382=VERTEX_POINT ( 'NONE', #4216 ) ;
#9383=CARTESIAN_POINT ( 'NONE',  ( 104.4899551042411190, -26.97880742045457936, 270.2814585562571779 ) ) ;
#9385=CARTESIAN_POINT ( 'NONE',  ( 103.3362113047044772, -29.43782462767379116, 118.2709475124489842 ) ) ;
#9386=EDGE_CURVE ( 'NONE', #48508, #62608, #16959, .T. ) ;
#9388=EDGE_CURVE ( 'NONE', #57294, #52002, #52537, .T. ) ;
#9389=LINE ( 'NONE', #37099, #83734 ) ;
#9390=VERTEX_POINT ( 'NONE', #6451 ) ;
#9391=ORIENTED_EDGE ( 'NONE', *, *, #81886, .F. ) ;
#9392=DIRECTION ( 'NONE',  ( -1.000000000000000000, -3.999999999999999995E-14, -1.000000000000000078E-15 ) ) ;
#9395=ORIENTED_EDGE ( 'NONE', *, *, #84590, .F. ) ;
#9396=CARTESIAN_POINT ( 'NONE',  ( 109.4376220470258119, -28.19094731436911871, 171.2930118773249717 ) ) ;
#9397=EDGE_CURVE ( 'NONE', #29192, #19551, #80642, .T. ) ;
#9399=CARTESIAN_POINT ( 'NONE',  ( 108.6520215831686329, -25.77392822130451577, 145.9737205140069420 ) ) ;
#9400=CARTESIAN_POINT ( 'NONE',  ( 97.06107107668189826, -37.99641179327961993, 121.4272919290289963 ) ) ;
#9402=VERTEX_POINT ( 'NONE', #47316 ) ;
#9404=ORIENTED_EDGE ( 'NONE', *, *, #3631, .T. ) ;
#9405=EDGE_CURVE ( 'NONE', #68551, #42008, #3530, .T. ) ;
#9406=CARTESIAN_POINT ( 'NONE',  ( 111.8340120402796032, -28.76913304608537914, 202.4652332267339716 ) ) ;
#9407=CARTESIAN_POINT ( 'NONE',  ( 101.9496561033292039, -27.62096520655628851, 60.48419670448296159 ) ) ;
#9409=CARTESIAN_POINT ( 'NONE',  ( 99.08262072259961428, -44.34008189452615056, 36.92038718067297509 ) ) ;
#9410=CARTESIAN_POINT ( 'NONE',  ( 109.6111442688334563, -26.56067652042401406, 195.8813395616249977 ) ) ;
#9411=CARTESIAN_POINT ( 'NONE',  ( 57.56670390244816815, -48.82844715994039575, 295.7178068554150627 ) ) ;
#9413=CARTESIAN_POINT ( 'NONE',  ( 108.9848500582430404, -47.61493517985451973, 118.7032443235299723 ) ) ;
#9415=ORIENTED_EDGE ( 'NONE', *, *, #18030, .F. ) ;
#9416=LINE ( 'NONE', #16681, #52483 ) ;
#9418=CARTESIAN_POINT ( 'NONE',  ( 164.7812970173289955, -35.65087443492610930, 117.4678068554150485 ) ) ;
#9420=ORIENTED_EDGE ( 'NONE', *, *, #53914, .T. ) ;
#9421=AXIS2_PLACEMENT_3D ( 'NONE', #82252, #47240, #74967 ) ;
#9422=CARTESIAN_POINT ( 'NONE',  ( 107.0667039024467329, -36.72944715994091780, 196.2188068554169718 ) ) ;
#9425=CARTESIAN_POINT ( 'NONE',  ( 109.6678112925185076, -27.04287877648044613, 130.8675598213152966 ) ) ;
#9426=CARTESIAN_POINT ( 'NONE',  ( 115.2074362016368099, -44.20634311780637660, 78.22324432352995416 ) ) ;
#9428=AXIS2_PLACEMENT_3D ( 'NONE', #73175, #31844, #32283 ) ;
#9430=CARTESIAN_POINT ( 'NONE',  ( 113.1782937756739642, -44.75186858913631482, 74.09395860969014791 ) ) ;
#9431=CARTESIAN_POINT ( 'NONE',  ( 100.4186822966649828, -43.90371905523902996, 46.98133956162492098 ) ) ;
#9432=CARTESIAN_POINT ( 'NONE',  ( 107.0664832912739968, -36.72944715994100306, 287.6356252759109680 ) ) ;
#9433=CARTESIAN_POINT ( 'NONE',  ( 117.2886123466743129, -34.79635738071010564, 154.9756252759109714 ) ) ;
#9437=CARTESIAN_POINT ( 'NONE',  ( 120.0056275895821898, -31.38355669832866468, 293.1356252759106837 ) ) ;
#9438=CIRCLE ( 'NONE', #22551, 7.499999999999996447 ) ;
#9439=AXIS2_PLACEMENT_3D ( 'NONE', #1442, #14166, #70937 ) ;
#9441=FACE_OUTER_BOUND ( 'NONE', #38855, .T. ) ;
#9442=FACE_OUTER_BOUND ( 'NONE', #83982, .T. ) ;
#9443=CARTESIAN_POINT ( 'NONE',  ( 106.4811411369643679, -24.84306116243460139, 195.1156252759109861 ) ) ;
#9446=CARTESIAN_POINT ( 'NONE',  ( 97.14909927861904748, -40.01315743934404878, 237.5813395616249579 ) ) ;
#9447=CARTESIAN_POINT ( 'NONE',  ( 116.6381559899473217, -29.65878987416117241, 105.3327681330539463 ) ) ;
#9448=CARTESIAN_POINT ( 'NONE',  ( 97.31575293894259460, -39.30575261481694582, 252.5323662874646118 ) ) ;
#9449=ADVANCED_FACE ( 'NONE', ( #40518 ), #27339, .T. ) ;
#9450=CARTESIAN_POINT ( 'NONE',  ( 90.44969454456405344, -20.11243780205715481, 219.5838068554169809 ) ) ;
#9451=CIRCLE ( 'NONE', #15295, 5.599999999999994316 ) ;
#9453=ORIENTED_EDGE ( 'NONE', *, *, #7476, .F. ) ;
#9454=AXIS2_PLACEMENT_3D ( 'NONE', #76914, #14693, #84193 ) ;
#9456=VERTEX_POINT ( 'NONE', #19191 ) ;
#9458=LINE ( 'NONE', #84442, #67037 ) ;
#9459=CARTESIAN_POINT ( 'NONE',  ( 96.76336351750784104, -35.13941245127819002, 262.2041967044821149 ) ) ;
#9460=CARTESIAN_POINT ( 'NONE',  ( 84.32545390244801808, -42.97311385574013087, 231.5838068554169524 ) ) ;
#9462=FACE_OUTER_BOUND ( 'NONE', #33858, .T. ) ;
#9463=LINE ( 'NONE', #43518, #54382 ) ;
#9465=CARTESIAN_POINT ( 'NONE',  ( 98.89771913768545630, -40.63891803577419637, 216.1162293518859485 ) ) ;
#9466=ORIENTED_EDGE ( 'NONE', *, *, #1436, .F. ) ;
#9467=ORIENTED_EDGE ( 'NONE', *, *, #2845, .T. ) ;
#9468=B_SPLINE_CURVE_WITH_KNOTS ( 'NONE', 3,
 ( #50207, #49310, #77043, #28893, #24744, #58368, #51101, #17047, #57924, #37040, #78841, #30670, #65630, #2531, #43840, #9336, #44727, #71131, #72458, #52411, #8909, #64745, #72015, #17924, #3414, #64309, #23435, #71577, #30231, #16600, #31103, #85657, #17489, #86983, #44278, #9782, #37488, #51974, #58799, #80176, #65192, #86543, #24308, #2969, #36609, #2079, #86095, #79732, #10226, #23867, #45170, #66064, #29784, #57477, #51538, #79287, #85217, #78400, #37931, #72894, #10659, #22984, #38364, #3857, #31550, #59252, #50659, #16162, #87870, #59690, #18824, #61488, #26533, #19714, #40605, #25633, #53759, #82415, #45600, #19278, #6102, #33346 ),
 .UNSPECIFIED., .F., .F.,
 ( 4, 2, 2, 2, 2, 2, 2, 2, 2, 2, 2, 2, 2, 2, 2, 2, 2, 2, 2, 2, 2, 2, 2, 2, 2, 2, 2, 2, 2, 2, 2, 2, 2, 2, 2, 2, 2, 2, 2, 2, 4 ),
 ( 6.061704139448921493E-05, 0.0002290496303638520949, 0.0003974822193332150019, 0.0007343473972719562117, 0.001408077753149438848, 0.002755538464904434912, 0.004102999176659431410, 0.005450459888414427474, 0.006797920600169424406, 0.008145381311924420470, 0.009492842023679417401, 0.01084030273543441433, 0.01353522415894439952, 0.01623014558245438818, 0.01690387593833189359, 0.01757760629420940246, 0.01892506700596442368, 0.01959879736184192908, 0.02027252771771943796, 0.02161998842947449387, 0.02296744914122954978, 0.02431490985298460222, 0.02566237056473966507, 0.02700983127649471752, 0.02835729198824977343, 0.02970475270000482934, 0.03037848305588235903, 0.03105221341175988872, 0.03239967412351493076, 0.03374713483526996238, 0.03509459554702500095, 0.03644205625878003951, 0.03778951697053507808, 0.03913697768229010970, 0.04048443839404514827, 0.04183189910580018683, 0.04250562946167770612, 0.04284249463961645188, 0.04301092722858581435, 0.04309514352307049906, 0.04317935981755517683 ),
 .UNSPECIFIED. ) ;
#9469=AXIS2_PLACEMENT_3D ( 'NONE', #28860, #84291, #15233 ) ;
#9470=ORIENTED_EDGE ( 'NONE', *, *, #86312, .F. ) ;
#9471=ADVANCED_FACE ( 'NONE', ( #11479 ), #60501, .F. ) ;
#9472=CARTESIAN_POINT ( 'NONE',  ( 20.56670390244743984, -48.82844715994200158, 180.4678068554150911 ) ) ;
#9473=CIRCLE ( 'NONE', #89294, 2.750000000000002665 ) ;
#9474=CARTESIAN_POINT ( 'NONE',  ( 97.82528911858155141, -40.55050895928604149, 181.6384720198973071 ) ) ;
#9475=CARTESIAN_POINT ( 'NONE',  ( 112.3177584634462534, -44.98096486020153151, 259.0270538473389479 ) ) ;
#9476=CARTESIAN_POINT ( 'NONE',  ( 141.0664832912740394, -46.72944715994099596, -4.824374724088994704 ) ) ;
#9477=CARTESIAN_POINT ( 'NONE',  ( 118.1720832024964807, -36.20253795304678590, 114.8641967044819694 ) ) ;
#9478=DIRECTION ( 'NONE',  ( -1.000000000000000078E-15, 1.000000000000000083E-30, 1.000000000000000000 ) ) ;
#9479=ORIENTED_EDGE ( 'NONE', *, *, #13090, .F. ) ;
#9480=CARTESIAN_POINT ( 'NONE',  ( 77.31651910784952975, -36.55813574389581078, 3.101427645696278379 ) ) ;
#9481=VERTEX_POINT ( 'NONE', #67780 ) ;
#9483=CARTESIAN_POINT ( 'NONE',  ( 112.7530619618799932, -30.23101651580132199, 285.9349166392303800 ) ) ;
#9487=DIRECTION ( 'NONE',  ( 1.000000000000000000, 0.000000000000000000, 0.000000000000000000 ) ) ;
#9488=DIRECTION ( 'NONE',  ( 0.000000000000000000, 0.000000000000000000, -1.000000000000000000 ) ) ;
#9489=EDGE_CURVE ( 'NONE', #59170, #12768, #70923, .T. ) ;
#9490=DIRECTION ( 'NONE',  ( 1.000000000000000078E-15, -1.000000000000000083E-30, -1.000000000000000000 ) ) ;
#9491=AXIS2_PLACEMENT_3D ( 'NONE', #52307, #80072, #17826 ) ;
#9492=ORIENTED_EDGE ( 'NONE', *, *, #66796, .T. ) ;
#9493=CARTESIAN_POINT ( 'NONE',  ( 34.96670390244699433, -26.71338133339301635, 342.9256252759109884 ) ) ;
#9494=DIRECTION ( 'NONE',  ( 0.000000000000000000, 0.000000000000000000, -1.000000000000000000 ) ) ;
#9495=EDGE_CURVE ( 'NONE', #58352, #7509, #54563, .T. ) ;
#9497=ORIENTED_EDGE ( 'NONE', *, *, #34286, .F. ) ;
#9498=CARTESIAN_POINT ( 'NONE',  ( 96.07744114619573850, -37.92110155076959899, 81.40038718067299328 ) ) ;
#9499=ORIENTED_EDGE ( 'NONE', *, *, #86846, .T. ) ;
#9501=CARTESIAN_POINT ( 'NONE',  ( 107.1721053552439713, -28.18866407513752392, 34.48956268521896362 ) ) ;
#9503=CARTESIAN_POINT ( 'NONE',  ( 110.0265056719061363, -46.30983220778679055, 88.81405189569714764 ) ) ;
#9504=CARTESIAN_POINT ( 'NONE',  ( 109.3646161452266767, -45.83961241216247373, 89.21682140113502157 ) ) ;
#9505=CARTESIAN_POINT ( 'NONE',  ( 115.0363764831674303, -42.90958019793037437, 14.30217953636555706 ) ) ;
#9506=ADVANCED_FACE ( 'NONE', ( #75501 ), #53673, .T. ) ;
#9507=DIRECTION ( 'NONE',  ( 1.000000000000000078E-15, -1.000000000000000083E-30, -1.000000000000000000 ) ) ;
#9508=DIRECTION ( 'NONE',  ( -1.000000000000000078E-15, 1.000000000000000083E-30, 1.000000000000000000 ) ) ;
#9509=VECTOR ( 'NONE', #19516, 1000.000000000000000 ) ;
#9510=CARTESIAN_POINT ( 'NONE',  ( 111.4988423704183020, -26.55354146975621177, 280.7375300378156453 ) ) ;
#9511=CARTESIAN_POINT ( 'NONE',  ( 127.0664832912740394, -46.72944715994101017, -4.824374724089008915 ) ) ;
#9514=ORIENTED_EDGE ( 'NONE', *, *, #10852, .F. ) ;
#9515=CARTESIAN_POINT ( 'NONE',  ( 117.0647351476834643, -39.95015185843580952, 154.5784824187679476 ) ) ;
#9516=CARTESIAN_POINT ( 'NONE',  ( 80.06648329127399677, -21.47944715994105991, 1.625625275910943746 ) ) ;
#9517=ORIENTED_EDGE ( 'NONE', *, *, #61403, .T. ) ;
#9518=ORIENTED_EDGE ( 'NONE', *, *, #59603, .T. ) ;
#9519=ORIENTED_EDGE ( 'NONE', *, *, #88579, .F. ) ;
#9522=CARTESIAN_POINT ( 'NONE',  ( 61.67079006425787924, -0.9306969701460061639, 394.9756252759102040 ) ) ;
#9523=CARTESIAN_POINT ( 'NONE',  ( 99.06478422775786896, -31.10483629442210329, 205.8384824187689617 ) ) ;
#9527=DIRECTION ( 'NONE',  ( 1.000000000000000078E-15, -1.000000000000000083E-30, -1.000000000000000000 ) ) ;
#9528=AXIS2_PLACEMENT_3D ( 'NONE', #39764, #67476, #59756 ) ;
#9529=CARTESIAN_POINT ( 'NONE',  ( 112.1974349349366804, -26.93816038506360755, 10.68038718067299087 ) ) ;
#9530=CARTESIAN_POINT ( 'NONE',  ( 97.81170003938157720, -40.51743348276853851, 42.63567940883270069 ) ) ;
#9531=ORIENTED_EDGE ( 'NONE', *, *, #48509, .F. ) ;
#9532=CARTESIAN_POINT ( 'NONE',  ( 98.34947374717273760, -31.65727468815311596, 171.9064461681665534 ) ) ;
#9533=CARTESIAN_POINT ( 'NONE',  ( 108.3334406624257298, -46.73486044134102713, 42.67684850810000086 ) ) ;
#9536=VECTOR ( 'NONE', #67619, 1000.000000000000114 ) ;
#9539=CARTESIAN_POINT ( 'NONE',  ( 104.4161250475293343, -26.02246701806295448, 240.2575300378159682 ) ) ;
#9544=CARTESIAN_POINT ( 'NONE',  ( 115.5937312905896022, -36.23733611532740184, 228.2952769709339691 ) ) ;
#9546=CARTESIAN_POINT ( 'NONE',  ( 115.5933672690473912, -28.53551910654245205, 35.43562527591098643 ) ) ;
#9548=CARTESIAN_POINT ( 'NONE',  ( 108.0382549187111607, -25.67193643048636886, 109.9946728949589811 ) ) ;
#9549=ORIENTED_EDGE ( 'NONE', *, *, #33571, .F. ) ;
#9550=CARTESIAN_POINT ( 'NONE',  ( 131.3165200636276211, -18.90534128959012961, 6.749824347015441539 ) ) ;
#9553=DIRECTION ( 'NONE',  ( 0.000000000000000000, 1.000000000000000000, 0.000000000000000000 ) ) ;
#9555=LINE ( 'NONE', #29550, #81036 ) ;
#9556=EDGE_LOOP ( 'NONE', ( #48445, #70706, #84538, #29947 ) ) ;
#9557=CARTESIAN_POINT ( 'NONE',  ( 71.25416588882602298, -72.55705569728901594, 394.9756252759102040 ) ) ;
#9560=DIRECTION ( 'NONE',  ( 0.000000000000000000, 0.000000000000000000, -1.000000000000000000 ) ) ;
#9561=AXIS2_PLACEMENT_3D ( 'NONE', #41738, #6788, #28114 ) ;
#9562=ORIENTED_EDGE ( 'NONE', *, *, #33286, .T. ) ;
#9563=CARTESIAN_POINT ( 'NONE',  ( 112.5258771334048475, -27.82206915948941273, 94.63848241876793566 ) ) ;
#9564=VECTOR ( 'NONE', #48655, 1000.000000000000000 ) ;
#9565=VECTOR ( 'NONE', #4568, 1000.000000000000000 ) ;
#9567=AXIS2_PLACEMENT_3D ( 'NONE', #59620, #52779, #3346 ) ;
#9569=ADVANCED_FACE ( 'NONE', ( #76387 ), #42739, .F. ) ;
#9573=CYLINDRICAL_SURFACE ( 'NONE', #18486, 3.000000000000002665 ) ;
#9574=DIRECTION ( 'NONE',  ( 0.000000000000000000, 0.000000000000000000, 1.000000000000000000 ) ) ;
#9575=CARTESIAN_POINT ( 'NONE',  ( 142.0664832912740678, -45.72944715994100306, 14.82207188531769049 ) ) ;
#9576=CYLINDRICAL_SURFACE ( 'NONE', #56657, 2.999999999999999112 ) ;
#9578=CARTESIAN_POINT ( 'NONE',  ( 84.06648329127399677, -14.47844715994100007, 284.9256252759119548 ) ) ;
#9580=VECTOR ( 'NONE', #76819, 1000.000000000000000 ) ;
#9582=CARTESIAN_POINT ( 'NONE',  ( 97.26456095925938428, -36.24355304347524509, 167.2870538473389672 ) ) ;
#9583=DIRECTION ( 'NONE',  ( 0.000000000000000000, 0.000000000000000000, -1.000000000000000000 ) ) ;
#9585=CARTESIAN_POINT ( 'NONE',  ( 104.4155842969358332, -46.14412564300911157, 18.35848241876792031 ) ) ;
#9586=DIRECTION ( 'NONE',  ( 0.000000000000000000, -1.000000000000000000, 0.000000000000000000 ) ) ;
#9587=CARTESIAN_POINT ( 'NONE',  ( 97.81219525132515002, -40.51866273574350430, 51.63573126026001603 ) ) ;
#9588=CARTESIAN_POINT ( 'NONE',  ( 116.7940960725532733, -39.39149561008477463, 13.61514541225734298 ) ) ;
#9590=CARTESIAN_POINT ( 'NONE',  ( 98.35011216517960975, -31.65613066903540229, 30.90664309484206385 ) ) ;
#9591=CARTESIAN_POINT ( 'NONE',  ( 114.1395267584829867, -29.97404255306813781, 234.4327681330549638 ) ) ;
#9592=VERTEX_POINT ( 'NONE', #35945 ) ;
#9594=CARTESIAN_POINT ( 'NONE',  ( 114.9579445475069264, -42.99008164810605592, 194.7244404487539668 ) ) ;
#9595=CARTESIAN_POINT ( 'NONE',  ( 31.56670390244800828, -32.29483332968611364, -5.074374724088000832 ) ) ;
#9596=CARTESIAN_POINT ( 'NONE',  ( 99.16631175631914630, -32.71502711089942039, 47.38444044875394923 ) ) ;
#9598=CARTESIAN_POINT ( 'NONE',  ( 105.7995184934298152, -26.72403496524378141, 80.17729194211321442 ) ) ;
#9599=DIRECTION ( 'NONE',  ( -0.9254794337955620787, -0.3787978585227822492, 0.000000000000000000 ) ) ;
#9600=ORIENTED_EDGE ( 'NONE', *, *, #44551, .F. ) ;
#9602=CARTESIAN_POINT ( 'NONE',  ( 34.67381068362099228, -26.00627455219321860, 237.4678068554150059 ) ) ;
#9603=CARTESIAN_POINT ( 'NONE',  ( 111.1189502094635202, -27.14789314160929479, 244.7584824187679544 ) ) ;
#9605=EDGE_CURVE ( 'NONE', #14493, #20049, #84866, .T. ) ;
#9606=ORIENTED_EDGE ( 'NONE', *, *, #45425, .T. ) ;
#9607=CARTESIAN_POINT ( 'NONE',  ( 109.6430121231974653, -46.48008673722491579, 82.78145860864054839 ) ) ;
#9609=CYLINDRICAL_SURFACE ( 'NONE', #37467, 9.999999999999998224 ) ;
#9610=FACE_BOUND ( 'NONE', #21066, .T. ) ;
#9611=CARTESIAN_POINT ( 'NONE',  ( 111.8651074766111293, -28.16866562884743885, 30.66991099019594813 ) ) ;
#9616=CARTESIAN_POINT ( 'NONE',  ( 96.79082665085387305, -38.90864320302405588, 27.49276813305395706 ) ) ;
#9617=VECTOR ( 'NONE', #21788, 999.9999999999998863 ) ;
#9619=VECTOR ( 'NONE', #53121, 1000.000000000000114 ) ;
#9620=CARTESIAN_POINT ( 'NONE',  ( 96.88875151864165503, -30.65867585538550344, 280.8984824187682534 ) ) ;
#9623=CARTESIAN_POINT ( 'NONE',  ( 82.58883806303657593, -17.63381004753172121, 2.797770231024844456 ) ) ;
#9624=CARTESIAN_POINT ( 'NONE',  ( 99.08975689199405679, -42.79577111913272347, 17.84389778671033966 ) ) ;
#9625=EDGE_CURVE ( 'NONE', #30248, #45134, #32566, .T. ) ;
#9626=DIRECTION ( 'NONE',  ( 0.000000000000000000, 0.000000000000000000, -1.000000000000000000 ) ) ;
#9627=CARTESIAN_POINT ( 'NONE',  ( 111.9587407205840890, -30.16069495786998544, 102.3852332267339591 ) ) ;
#9628=CARTESIAN_POINT ( 'NONE',  ( 118.9020112566783354, -37.70028621367283961, 184.7613395616249647 ) ) ;
#9629=LINE ( 'NONE', #70978, #43507 ) ;
#9630=EDGE_LOOP ( 'NONE', ( #64937, #654, #60672, #82707 ) ) ;
#9632=FACE_OUTER_BOUND ( 'NONE', #22649, .T. ) ;
#9634=ORIENTED_EDGE ( 'NONE', *, *, #89028, .T. ) ;
#9635=FACE_BOUND ( 'NONE', #1819, .T. ) ;
#9640=AXIS2_PLACEMENT_3D ( 'NONE', #29360, #70238, #8929 ) ;
#9641=CARTESIAN_POINT ( 'NONE',  ( 34.27482367531452212, -30.08671355700332839, 313.9678068554150059 ) ) ;
#9642=CARTESIAN_POINT ( 'NONE',  ( 115.7614890496577402, -39.26115509793221747, 138.0114674471239766 ) ) ;
#9643=CARTESIAN_POINT ( 'NONE',  ( 115.9788024870550061, -30.15175701148841725, 259.3203871806730945 ) ) ;
#9644=CARTESIAN_POINT ( 'NONE',  ( 49.21213752016100784, -29.73316016639650883, 342.9256252759109884 ) ) ;
#9645=ORIENTED_EDGE ( 'NONE', *, *, #44960, .T. ) ;
#9646=CARTESIAN_POINT ( 'NONE',  ( 103.2780950051364925, -27.47482052217685222, 136.3856613811564671 ) ) ;
#9648=LINE ( 'NONE', #42803, #62367 ) ;
#9650=DIRECTION ( 'NONE',  ( 0.000000000000000000, 1.000000000000000000, 0.000000000000000000 ) ) ;
#9652=CARTESIAN_POINT ( 'NONE',  ( 105.8886092880350560, -47.16805723083484736, 282.4870538473393253 ) ) ;
#9653=VERTEX_POINT ( 'NONE', #49556 ) ;
#9654=CARTESIAN_POINT ( 'NONE',  ( 95.23113311243525914, -37.33357626913954164, 271.3670538473393776 ) ) ;
#9655=CARTESIAN_POINT ( 'NONE',  ( 100.3832715781272356, -28.67167693828054453, 36.62705384733894221 ) ) ;
#9656=DIRECTION ( 'NONE',  ( 5.512527431108029424E-15, -1.000000000000000000, 0.000000000000000000 ) ) ;
#9658=FACE_OUTER_BOUND ( 'NONE', #36723, .T. ) ;
#9659=EDGE_CURVE ( 'NONE', #29066, #2140, #84115, .T. ) ;
#9660=CYLINDRICAL_SURFACE ( 'NONE', #42332, 0.5000000000000073275 ) ;
#9661=CARTESIAN_POINT ( 'NONE',  ( 83.56670559755329464, -36.73837296219065252, 239.5838068554176914 ) ) ;
#9662=CARTESIAN_POINT ( 'NONE',  ( 131.6875538713384799, -38.11069332324941428, 7.213126773498808930 ) ) ;
#9663=CARTESIAN_POINT ( 'NONE',  ( 162.8595971212720031, -23.19206098994089160, 342.9256252759109884 ) ) ;
#9665=DIRECTION ( 'NONE',  ( 0.000000000000000000, 1.000000000000000000, 0.000000000000000000 ) ) ;
#9666=DIRECTION ( 'NONE',  ( 1.000000000000000000, 4.510281037539788691E-14, 0.000000000000000000 ) ) ;
#9667=CARTESIAN_POINT ( 'NONE',  ( 96.54134661961150243, -40.18473915001016650, 286.5908633711491120 ) ) ;
#9668=CARTESIAN_POINT ( 'NONE',  ( 100.0081584303796944, -27.21027357624165788, 181.5841967044829630 ) ) ;
#9669=CARTESIAN_POINT ( 'NONE',  ( 116.4070807376042609, -31.97209126034463011, 40.20133956162496958 ) ) ;
#9671=B_SPLINE_CURVE_WITH_KNOTS ( 'NONE', 3,
 ( #55481, #20106, #69146, #47783, #55032, #83679, #70494, #75518, #77305, #48225, #82346, #13731, #62766, #42754, #8265, #63222, #83234, #14182 ),
 .UNSPECIFIED., .F., .F.,
 ( 4, 2, 2, 2, 2, 2, 2, 2, 4 ),
 ( 0.4999999998527593359, 0.5624999998711643912, 0.6249999998895694464, 0.6874999999079746127, 0.7499999999263796679, 0.8124999999447847232, 0.8749999999631898895, 0.9374999999815949447, 1.000000000000000000 ),
 .UNSPECIFIED. ) ;
#9672=DIRECTION ( 'NONE',  ( 0.000000000000000000, 0.000000000000000000, -1.000000000000000000 ) ) ;
#9673=DIRECTION ( 'NONE',  ( 3.999999999999999995E-14, -1.000000000000000000, 4.100000000000000342E-29 ) ) ;
#9674=CYLINDRICAL_SURFACE ( 'NONE', #13147, 2.030000000002079918 ) ;
#9675=VECTOR ( 'NONE', #22869, 1000.000000000000000 ) ;
#9682=ORIENTED_EDGE ( 'NONE', *, *, #33810, .F. ) ;
#9683=CARTESIAN_POINT ( 'NONE',  ( 99.77418633167441442, -43.29726106931974527, 52.90991099019598209 ) ) ;
#9684=EDGE_CURVE ( 'NONE', #6056, #89556, #14622, .T. ) ;
#9687=CARTESIAN_POINT ( 'NONE',  ( 109.6425287038660343, -46.48020844107070815, 48.78141933728851853 ) ) ;
#9688=CARTESIAN_POINT ( 'NONE',  ( 116.3308458273175603, -44.07926308385594183, 194.2927681330539542 ) ) ;
#9689=DIRECTION ( 'NONE',  ( 4.299999999999999979E-14, -1.000000000000000000, 0.000000000000000000 ) ) ;
#9690=CARTESIAN_POINT ( 'NONE',  ( 97.92339371807813109, -40.78106740870623526, 146.6584159238782661 ) ) ;
#9692=DIRECTION ( 'NONE',  ( 1.000000000000000000, 6.831565154159360295E-14, 0.000000000000000000 ) ) ;
#9695=CARTESIAN_POINT ( 'NONE',  ( 50.56670390244699576, -22.48495420874030515, -5.074374724088000832 ) ) ;
#9696=CARTESIAN_POINT ( 'NONE',  ( 110.9332348646555175, -45.95165287104040885, 97.89240726581952856 ) ) ;
#9698=CARTESIAN_POINT ( 'NONE',  ( 103.4152017835535844, -27.65577212482025971, 130.3813395616259925 ) ) ;
#9699=EDGE_LOOP ( 'NONE', ( #9466, #4221, #32353, #21465 ) ) ;
#9700=ORIENTED_EDGE ( 'NONE', *, *, #72938, .T. ) ;
#9702=CARTESIAN_POINT ( 'NONE',  ( 109.3646161452266767, -45.83961241216247373, 89.21682140113502157 ) ) ;
#9706=CARTESIAN_POINT ( 'NONE',  ( 104.3638673426610950, -27.29495504168068365, 221.2984824187679465 ) ) ;
#9708=CARTESIAN_POINT ( 'NONE',  ( 116.3135889066590636, -32.94480564983713577, 259.1356252759109680 ) ) ;
#9709=EDGE_CURVE ( 'NONE', #36458, #49665, #671, .T. ) ;
#9710=DIRECTION ( 'NONE',  ( 0.000000000000000000, 0.000000000000000000, 1.000000000000000000 ) ) ;
#9711=DIRECTION ( 'NONE',  ( 1.000000000000000078E-15, -1.000000000000000083E-30, -1.000000000000000000 ) ) ;
#9715=ADVANCED_FACE ( 'NONE', ( #63206 ), #36411, .F. ) ;
#9716=CARTESIAN_POINT ( 'NONE',  ( 114.5119312840560184, -28.59475203354325501, 154.4746728949589851 ) ) ;
#9717=ORIENTED_EDGE ( 'NONE', *, *, #30070, .T. ) ;
#9718=EDGE_CURVE ( 'NONE', #20143, #71729, #50005, .T. ) ;
#9722=CARTESIAN_POINT ( 'NONE',  ( 100.8874678708047412, -44.70022136463035167, 78.05229194121726266 ) ) ;
#9723=CARTESIAN_POINT ( 'NONE',  ( 25.56670390244797275, -65.37844715994100397, 178.0928068554149775 ) ) ;
#9724=CARTESIAN_POINT ( 'NONE',  ( 106.9677948388671069, -45.38341651713141545, 230.3976141791149814 ) ) ;
#9725=AXIS2_PLACEMENT_3D ( 'NONE', #76917, #42367, #63735 ) ;
#9726=CARTESIAN_POINT ( 'NONE',  ( 131.0667039024480118, -67.87844715994100397, 237.1838068554150141 ) ) ;
#9727=CARTESIAN_POINT ( 'NONE',  ( 114.1248632939498719, -29.05700933358840032, 199.4841967044819739 ) ) ;
#9728=CARTESIAN_POINT ( 'NONE',  ( 134.0664832912740110, -46.72944715994100306, 4.925625275910997303 ) ) ;
#9729=ORIENTED_EDGE ( 'NONE', *, *, #68600, .T. ) ;
#9730=ORIENTED_EDGE ( 'NONE', *, *, #1049, .T. ) ;
#9731=ORIENTED_EDGE ( 'NONE', *, *, #37455, .F. ) ;
#9732=EDGE_CURVE ( 'NONE', #43936, #37298, #51427, .T. ) ;
#9733=CARTESIAN_POINT ( 'NONE',  ( 113.0895751218732244, -44.74357622511442401, 64.08993167605405006 ) ) ;
#9735=ADVANCED_FACE ( 'NONE', ( #16851 ), #71820, .T. ) ;
#9736=CARTESIAN_POINT ( 'NONE',  ( 133.8780722764369386, -33.97944715994099596, 8.225625275910998013 ) ) ;
#9737=EDGE_CURVE ( 'NONE', #79573, #32539, #63050, .T. ) ;
#9738=CARTESIAN_POINT ( 'NONE',  ( 99.80492824067951574, -39.70159478663597241, 9.453804655305930282 ) ) ;
#9739=FACE_OUTER_BOUND ( 'NONE', #2713, .T. ) ;
#9740=ORIENTED_EDGE ( 'NONE', *, *, #39321, .T. ) ;
#9744=CARTESIAN_POINT ( 'NONE',  ( 109.6203647746237948, -44.72533910755026909, 9.635625275910941312 ) ) ;
#9745=DIRECTION ( 'NONE',  ( 1.000000000000000000, -5.337610695313248426E-16, 0.000000000000000000 ) ) ;
#9746=ORIENTED_EDGE ( 'NONE', *, *, #45076, .F. ) ;
#9747=VERTEX_POINT ( 'NONE', #65873 ) ;
#9748=AXIS2_PLACEMENT_3D ( 'NONE', #85452, #38601, #10461 ) ;
#9750=CARTESIAN_POINT ( 'NONE',  ( 111.4545423736837648, -45.72122411965542454, 112.9377471918615328 ) ) ;
#9751=VECTOR ( 'NONE', #35635, 1000.000000000000000 ) ;
#9754=CARTESIAN_POINT ( 'NONE',  ( 115.0166753900997065, -32.39272993814809354, 23.63432458998199337 ) ) ;
#9755=CARTESIAN_POINT ( 'NONE',  ( 108.3688725116650602, -47.72941199507204146, 162.6822919425769669 ) ) ;
#9756=CARTESIAN_POINT ( 'NONE',  ( 96.69266148864264210, -35.94780844399461017, 146.2670538473399517 ) ) ;
#9757=DIRECTION ( 'NONE',  ( -0.7071067811864666375, -0.7071067811866283970, -7.071067811864971448E-16 ) ) ;
#9758=CARTESIAN_POINT ( 'NONE',  ( 116.9253062793529665, -41.72720563489927770, 244.4651490854349731 ) ) ;
#9760=CARTESIAN_POINT ( 'NONE',  ( 104.4884655257109642, -26.97921697585386980, 126.2815806043031444 ) ) ;
#9761=LINE ( 'NONE', #19253, #19259 ) ;
#9762=ORIENTED_EDGE ( 'NONE', *, *, #2556, .T. ) ;
#9765=AXIS2_PLACEMENT_3D ( 'NONE', #65283, #10317, #46145 ) ;
#9766=AXIS2_PLACEMENT_3D ( 'NONE', #67801, #75067, #40983 ) ;
#9767=CARTESIAN_POINT ( 'NONE',  ( 98.50147650033493107, -30.70887204493662281, 205.8384824187679669 ) ) ;
#9768=ORIENTED_EDGE ( 'NONE', *, *, #63647, .T. ) ;
#9769=CARTESIAN_POINT ( 'NONE',  ( 102.9133425085070712, -27.12904003091135152, 155.4013395616249795 ) ) ;
#9771=CARTESIAN_POINT ( 'NONE',  ( 136.1113402350696049, -34.88977106732826172, 7.516154048594613890 ) ) ;
#9775=CARTESIAN_POINT ( 'NONE',  ( 115.6373213143783545, -30.77082676042347487, 275.3099109901965562 ) ) ;
#9779=DIRECTION ( 'NONE',  ( -1.000000000000000000, 0.000000000000000000, 4.496403249731880833E-15 ) ) ;
#9780=CARTESIAN_POINT ( 'NONE',  ( 100.8874679095308409, -44.70022139425450547, 258.0522919450611994 ) ) ;
#9782=CARTESIAN_POINT ( 'NONE',  ( 108.9306573623864267, -44.50959214567147626, 195.5838068554169240 ) ) ;
#9783=ORIENTED_EDGE ( 'NONE', *, *, #51517, .F. ) ;
#9784=CARTESIAN_POINT ( 'NONE',  ( 134.4432975232482761, -21.47944369576867985, 8.225625303283965906 ) ) ;
#9785=CARTESIAN_POINT ( 'NONE',  ( 115.0566306311886819, -29.05787713660226856, 189.4232443235299570 ) ) ;
#9786=CARTESIAN_POINT ( 'NONE',  ( 96.33847535375279847, -41.76377544194641445, 57.67562527591096710 ) ) ;
#9787=CARTESIAN_POINT ( 'NONE',  ( 113.0470503471827044, -45.36488765107162635, 199.0584824187679374 ) ) ;
#9788=CARTESIAN_POINT ( 'NONE',  ( 141.8164832912740110, -45.62589376934770513, 14.92562527591100618 ) ) ;
#9790=DIRECTION ( 'NONE',  ( -3.360405532702990443E-14, 1.000000000000000000, 0.000000000000000000 ) ) ;
#9791=CARTESIAN_POINT ( 'NONE',  ( 114.1825262577302027, -43.80211088142657161, 39.20373200096445032 ) ) ;
#9793=DIRECTION ( 'NONE',  ( -0.9254794337955620787, -0.3787978585227822492, 0.000000000000000000 ) ) ;
#9796=DIRECTION ( 'NONE',  ( 0.000000000000000000, 0.000000000000000000, 1.000000000000000000 ) ) ;
#9797=EDGE_CURVE ( 'NONE', #44789, #53353, #72267, .T. ) ;
#9800=ORIENTED_EDGE ( 'NONE', *, *, #1826, .T. ) ;
#9801=CARTESIAN_POINT ( 'NONE',  ( 100.3264543382982907, -29.74069638407027938, 115.1095626852199558 ) ) ;
#9805=CARTESIAN_POINT ( 'NONE',  ( 113.4020503763144063, -27.70036014686462522, 80.57753003781597556 ) ) ;
#9806=DIRECTION ( 'NONE',  ( 1.000000000000000078E-15, -1.000000000000000083E-30, -1.000000000000000000 ) ) ;
#9809=ADVANCED_FACE ( 'NONE', ( #3225, #86344 ), #51785, .F. ) ;
#9810=CARTESIAN_POINT ( 'NONE',  ( 97.81169128372820865, -40.51741339292117772, 177.6357569005977268 ) ) ;
#9811=AXIS2_PLACEMENT_3D ( 'NONE', #49510, #34094, #27292 ) ;
#9812=CARTESIAN_POINT ( 'NONE',  ( 104.6499073705539331, -46.24122592705978718, 47.37848241876896083 ) ) ;
#9813=ORIENTED_EDGE ( 'NONE', *, *, #36190, .T. ) ;
#9815=VERTEX_POINT ( 'NONE', #24558 ) ;
#9819=DIRECTION ( 'NONE',  ( 4.299999999999999979E-14, -1.000000000000000000, 4.400000000000000367E-29 ) ) ;
#9820=LINE ( 'NONE', #52448, #56357 ) ;
#9822=CARTESIAN_POINT ( 'NONE',  ( 151.0371591254573502, -24.42818131005592974, 249.9678068554149490 ) ) ;
#9824=EDGE_CURVE ( 'NONE', #20049, #35637, #17740, .T. ) ;
#9825=CARTESIAN_POINT ( 'NONE',  ( 97.81193178031652735, -40.51732023384165160, 27.63604381180012837 ) ) ;
#9827=AXIS2_PLACEMENT_3D ( 'NONE', #10808, #4001, #87575 ) ;
#9829=CARTESIAN_POINT ( 'NONE',  ( 106.5192459994187715, -25.71289806663794408, 45.12800622829193742 ) ) ;
#9830=EDGE_CURVE ( 'NONE', #43807, #65403, #26495, .T. ) ;
#9832=CIRCLE ( 'NONE', #89580, 0.5000000000000104361 ) ;
#9835=CIRCLE ( 'NONE', #86728, 4.875000000000017764 ) ;
#9836=LINE ( 'NONE', #72934, #56846 ) ;
#9837=CARTESIAN_POINT ( 'NONE',  ( 101.2865843167392654, -43.98814532200950822, 119.8595189410199566 ) ) ;
#9838=ADVANCED_FACE ( 'NONE', ( #88581 ), #33151, .T. ) ;
#9839=CIRCLE ( 'NONE', #73623, 2.116999999999980009 ) ;
#9840=CARTESIAN_POINT ( 'NONE',  ( 41.56648329127399677, -9.303447159940999356, 318.9256252759120116 ) ) ;
#9841=DIRECTION ( 'NONE',  ( 0.7071067811868035902, 0.7071067811862914443, 7.071067811868340870E-16 ) ) ;
#9844=CARTESIAN_POINT ( 'NONE',  ( 97.82526847378206014, -40.55045903170837818, 136.6388370546689259 ) ) ;
#9845=ORIENTED_EDGE ( 'NONE', *, *, #78062, .T. ) ;
#9846=ORIENTED_EDGE ( 'NONE', *, *, #29676, .T. ) ;
#9847=EDGE_CURVE ( 'NONE', #42012, #48511, #74941, .T. ) ;
#9848=CARTESIAN_POINT ( 'NONE',  ( 98.83447963006204873, -41.25831470702095061, 173.1463452106589784 ) ) ;
#9850=EDGE_CURVE ( 'NONE', #17117, #5375, #19074, .T. ) ;
#9851=CARTESIAN_POINT ( 'NONE',  ( 117.6299819888065912, -33.39812594883869679, 125.0575300378149706 ) ) ;
#9852=DIRECTION ( 'NONE',  ( -1.000000000000000000, 0.000000000000000000, 4.496403249731880833E-15 ) ) ;
#9853=VECTOR ( 'NONE', #36339, 1000.000000000000000 ) ;
#9854=CARTESIAN_POINT ( 'NONE',  ( 77.31648329127401098, -36.72944715994107412, 6.749768910606400496 ) ) ;
#9855=ORIENTED_EDGE ( 'NONE', *, *, #47390, .F. ) ;
#9858=CARTESIAN_POINT ( 'NONE',  ( 98.92939184154955967, -35.79647825066581390, 204.0538046553059814 ) ) ;
#9859=CARTESIAN_POINT ( 'NONE',  ( 117.2885226371813872, -38.88728764921428649, 63.66133956162494911 ) ) ;
#9860=ORIENTED_EDGE ( 'NONE', *, *, #46396, .T. ) ;
#9861=CARTESIAN_POINT ( 'NONE',  ( 104.7405551043178491, -47.51155644559854352, 32.41943479972098174 ) ) ;
#9862=LINE ( 'NONE', #25714, #21989 ) ;
#9864=CARTESIAN_POINT ( 'NONE',  ( 96.01412018463531695, -36.58377574468403282, 152.3280062282919971 ) ) ;
#9865=CARTESIAN_POINT ( 'NONE',  ( 19.56670390244740076, -47.82844715994204421, 180.4678068554150911 ) ) ;
#9868=VECTOR ( 'NONE', #24949, 1000.000000000000000 ) ;
#9869=ORIENTED_EDGE ( 'NONE', *, *, #8233, .T. ) ;
#9870=FACE_OUTER_BOUND ( 'NONE', #6661, .T. ) ;
#9871=EDGE_LOOP ( 'NONE', ( #69340, #89239, #33946, #88363 ) ) ;
#9874=AXIS2_PLACEMENT_3D ( 'NONE', #65092, #71481, #77843 ) ;
#9876=CIRCLE ( 'NONE', #53400, 1.000000000000000888 ) ;
#9877=FACE_OUTER_BOUND ( 'NONE', #57266, .T. ) ;
#9878=CARTESIAN_POINT ( 'NONE',  ( 101.1416012009399026, -28.10844496237015733, 50.55562527591095545 ) ) ;
#9880=CARTESIAN_POINT ( 'NONE',  ( 107.0664832912739968, 12.92155284005902516, 333.4006252759110112 ) ) ;
#9881=CARTESIAN_POINT ( 'NONE',  ( 108.3334481027989540, -46.73485935290891291, 73.67729194320179431 ) ) ;
#9882=CARTESIAN_POINT ( 'NONE',  ( 97.35459460924916186, -38.14118110200430323, 66.44133956162595211 ) ) ;
#9884=CARTESIAN_POINT ( 'NONE',  ( 117.7782040715256926, -34.09831434418946827, 160.0061014663869798 ) ) ;
#9885=CARTESIAN_POINT ( 'NONE',  ( 97.33756857962994502, -34.07217399619458575, 61.11488175924079513 ) ) ;
#9886=DIRECTION ( 'NONE',  ( 4.194175870806139918E-14, -1.000000000000000000, 0.000000000000000000 ) ) ;
#9887=ORIENTED_EDGE ( 'NONE', *, *, #68087, .F. ) ;
#9891=PLANE ( 'NONE',  #79268 ) ;
#9893=PLANE ( 'NONE',  #66545 ) ;
#9894=CARTESIAN_POINT ( 'NONE',  ( 97.88046564956832185, -41.75177191353013484, 221.7241967044819546 ) ) ;
#9896=CARTESIAN_POINT ( 'NONE',  ( 113.2454386374689221, -28.75862319911502851, 144.5522981085485412 ) ) ;
#9897=CARTESIAN_POINT ( 'NONE',  ( 115.9252781128442535, -30.08061567962537453, 260.3508633711493871 ) ) ;
#9898=CARTESIAN_POINT ( 'NONE',  ( 113.3408031569382644, -28.30502284670691182, 100.5670538473389684 ) ) ;
#9902=ADVANCED_FACE ( 'NONE', ( #75393 ), #47209, .T. ) ;
#9904=DIRECTION ( 'NONE',  ( -0.7071067811865175967, -0.7071067811865774377, -7.071067811865480264E-16 ) ) ;
#9905=ORIENTED_EDGE ( 'NONE', *, *, #5669, .F. ) ;
#9907=ORIENTED_EDGE ( 'NONE', *, *, #11122, .T. ) ;
#9910=CIRCLE ( 'NONE', #21520, 2.029999999999997140 ) ;
#9911=EDGE_CURVE ( 'NONE', #71729, #20143, #19536, .T. ) ;
#9912=ORIENTED_EDGE ( 'NONE', *, *, #29499, .F. ) ;
#9914=CARTESIAN_POINT ( 'NONE',  ( 106.8364377494367403, -47.15199802307920152, 268.5584824187679374 ) ) ;
#9916=DIRECTION ( 'NONE',  ( 0.000000000000000000, 0.000000000000000000, 1.000000000000000000 ) ) ;
#9918=LINE ( 'NONE', #24439, #6206 ) ;
#9920=CARTESIAN_POINT ( 'NONE',  ( 156.5667039024483813, -48.82844715993569196, 257.2178068554149490 ) ) ;
#9921=AXIS2_PLACEMENT_3D ( 'NONE', #60878, #88164, #12746 ) ;
#9922=CARTESIAN_POINT ( 'NONE',  ( 107.2112434921279629, -45.29864470754334604, 212.0124198280769861 ) ) ;
#9925=ORIENTED_EDGE ( 'NONE', *, *, #46820, .F. ) ;
#9926=ORIENTED_EDGE ( 'NONE', *, *, #48509, .T. ) ;
#9928=FACE_OUTER_BOUND ( 'NONE', #51130, .T. ) ;
#9930=CARTESIAN_POINT ( 'NONE',  ( 97.18779024860596394, -39.88384922728100435, 277.5603871806723646 ) ) ;
#9932=CARTESIAN_POINT ( 'NONE',  ( 107.0664832912750057, -36.72944715993903486, 3.024967495036150922 ) ) ;
#9935=ORIENTED_EDGE ( 'NONE', *, *, #460, .T. ) ;
#9936=AXIS2_PLACEMENT_3D ( 'NONE', #40700, #74339, #6199 ) ;
#9937=FACE_OUTER_BOUND ( 'NONE', #49697, .T. ) ;
#9938=VERTEX_POINT ( 'NONE', #7589 ) ;
#9939=DIRECTION ( 'NONE',  ( 1.000000000000000000, 1.709087168450053081E-14, 0.000000000000000000 ) ) ;
#9940=CARTESIAN_POINT ( 'NONE',  ( 101.9647735066782843, -29.73848997801458083, 28.38428084578198352 ) ) ;
#9942=DIRECTION ( 'NONE',  ( 0.8571673007021091140, -8.250245410175212261E-16, 0.5150380749100597066 ) ) ;
#9945=ORIENTED_EDGE ( 'NONE', *, *, #73982, .F. ) ;
#9946=LINE ( 'NONE', #36309, #81322 ) ;
#9948=FACE_OUTER_BOUND ( 'NONE', #11664, .T. ) ;
#9949=VERTEX_POINT ( 'NONE', #35276 ) ;
#9950=CARTESIAN_POINT ( 'NONE',  ( 98.09668637883959263, -31.41627731406707724, 85.90133956162493689 ) ) ;
#9952=CARTESIAN_POINT ( 'NONE',  ( 109.1774539423994952, -45.00591588954721800, 47.19813411379097801 ) ) ;
#9954=DIRECTION ( 'NONE',  ( 0.000000000000000000, 0.000000000000000000, 1.000000000000000000 ) ) ;
#9955=CARTESIAN_POINT ( 'NONE',  ( 106.8749774919903359, -46.80089345537784595, 73.99301187732598351 ) ) ;
#9956=CARTESIAN_POINT ( 'NONE',  ( 108.3325648527817719, -46.73495960743948530, 13.67722169067239157 ) ) ;
#9957=DIRECTION ( 'NONE',  ( 1.000000000000000000, 4.163336342344333240E-14, 0.000000000000000000 ) ) ;
#9961=CARTESIAN_POINT ( 'NONE',  ( 112.1278237076712543, -26.87713336146359211, 15.71086337114896381 ) ) ;
#9962=LINE ( 'NONE', #58099, #30736 ) ;
#9963=ORIENTED_EDGE ( 'NONE', *, *, #20468, .F. ) ;
#9966=CARTESIAN_POINT ( 'NONE',  ( 117.3528398777633299, -34.78421141941176842, 154.9756252759109714 ) ) ;
#9971=CARTESIAN_POINT ( 'NONE',  ( 83.56670559755329464, -36.73837296219065252, 239.5838068554176914 ) ) ;
#9972=DIRECTION ( 'NONE',  ( 0.000000000000000000, 1.000000000000000000, 0.000000000000000000 ) ) ;
#9973=CARTESIAN_POINT ( 'NONE',  ( 101.7740290765682403, -45.64733444449330335, 207.1622919425779514 ) ) ;
#9977=CARTESIAN_POINT ( 'NONE',  ( 99.14357900773808296, -43.50514455292471894, 27.88991099019694175 ) ) ;
#9979=ORIENTED_EDGE ( 'NONE', *, *, #65322, .T. ) ;
#9980=CARTESIAN_POINT ( 'NONE',  ( 103.2773610487370632, -27.47512100226090581, 171.3857244979931522 ) ) ;
#9981=FACE_OUTER_BOUND ( 'NONE', #16758, .T. ) ;
#9982=ORIENTED_EDGE ( 'NONE', *, *, #32866, .T. ) ;
#9985=CARTESIAN_POINT ( 'NONE',  ( 107.0664832912739968, 25.62155284005901379, 327.8006252759110453 ) ) ;
#9986=CARTESIAN_POINT ( 'NONE',  ( 112.4430884738663821, -45.67687932769439385, 238.0070538473389377 ) ) ;
#9988=CARTESIAN_POINT ( 'NONE',  ( 107.0664832912750057, -36.72944715993903486, 9.425625275910970657 ) ) ;
#9989=FACE_OUTER_BOUND ( 'NONE', #58277, .T. ) ;
#9990=CARTESIAN_POINT ( 'NONE',  ( 100.3746636439974935, -30.62762610928201568, 230.1486103042669811 ) ) ;
#9992=CARTESIAN_POINT ( 'NONE',  ( 111.9186950350129877, -27.52701776748444473, 55.68991099019693536 ) ) ;
#9994=CARTESIAN_POINT ( 'NONE',  ( 109.5188487141873850, -46.90749067903785630, 132.7641967044819751 ) ) ;
#9995=EDGE_LOOP ( 'NONE', ( #17315, #57981, #23039, #45726 ) ) ;
#9996=LINE ( 'NONE', #3184, #32154 ) ;
#9997=ORIENTED_EDGE ( 'NONE', *, *, #87623, .F. ) ;
#9998=CARTESIAN_POINT ( 'NONE',  ( 51.23005224011598102, -33.89581943344511217, -5.074374724088000832 ) ) ;
#9999=CARTESIAN_POINT ( 'NONE',  ( 97.07207205126279348, -35.37844125359542602, 67.21895861358602531 ) ) ;
#10000=DIRECTION ( 'NONE',  ( -0.7071067811865483499, -7.937023868100978726E-16, -0.7071067811865466846 ) ) ;
#10002=VECTOR ( 'NONE', #27858, 1000.000000000000000 ) ;
#10003=CARTESIAN_POINT ( 'NONE',  ( 152.0371591254585724, -47.82818131005587503, 117.4678068554150485 ) ) ;
#10004=ORIENTED_EDGE ( 'NONE', *, *, #84548, .T. ) ;
#10005=DIRECTION ( 'NONE',  ( 0.000000000000000000, 0.000000000000000000, -1.000000000000000000 ) ) ;
#10007=VECTOR ( 'NONE', #74934, 1000.000000000000000 ) ;
#10008=CARTESIAN_POINT ( 'NONE',  ( 50.97905606903270836, -31.62489322948282222, 117.4678068554150485 ) ) ;
#10010=AXIS2_PLACEMENT_3D ( 'NONE', #8276, #56401, #27811 ) ;
#10011=CARTESIAN_POINT ( 'NONE',  ( 115.2246207261642894, -44.22212590188486558, 78.22324432352995416 ) ) ;
#10012=FILL_AREA_STYLE_COLOUR ( '', #21696 ) ;
#10013=DIRECTION ( 'NONE',  ( 0.000000000000000000, 0.000000000000000000, -1.000000000000000000 ) ) ;
#10014=DIRECTION ( 'NONE',  ( -4.237773401492740281E-14, 1.000000000000000000, 0.000000000000000000 ) ) ;
#10016=ORIENTED_EDGE ( 'NONE', *, *, #13908, .F. ) ;
#10018=AXIS2_PLACEMENT_3D ( 'NONE', #19116, #88179, #46796 ) ;
#10020=CYLINDRICAL_SURFACE ( 'NONE', #50447, 1.000000000000000888 ) ;
#10022=ADVANCED_FACE ( 'NONE', ( #84360 ), #77083, .T. ) ;
#10023=AXIS2_PLACEMENT_3D ( 'NONE', #3783, #65560, #3340 ) ;
#10024=LINE ( 'NONE', #43624, #79169 ) ;
#10025=ADVANCED_FACE ( 'NONE', ( #8032 ), #22572, .T. ) ;
#10026=CIRCLE ( 'NONE', #20135, 1.000000000002049694 ) ;
#10027=DIRECTION ( 'NONE',  ( 1.000000000000000078E-15, -1.000000000000000083E-30, -1.000000000000000000 ) ) ;
#10031=CARTESIAN_POINT ( 'NONE',  ( 134.0664832912740110, -46.72944715994100306, 4.925625275910997303 ) ) ;
#10032=CARTESIAN_POINT ( 'NONE',  ( 113.8091913586853821, -43.81457933525486936, 154.1813395616249807 ) ) ;
#10036=ORIENTED_EDGE ( 'NONE', *, *, #24204, .T. ) ;
#10037=CARTESIAN_POINT ( 'NONE',  ( 100.9974690995740190, -29.01719307973645812, 11.60705384733895507 ) ) ;
#10038=CARTESIAN_POINT ( 'NONE',  ( 141.8164832912740394, -36.72944715994099596, -5.074374724088994704 ) ) ;
#10039=DIRECTION ( 'NONE',  ( 0.000000000000000000, 1.000000000000000000, 0.000000000000000000 ) ) ;
#10042=DIRECTION ( 'NONE',  ( -0.9254794337955620787, -0.3787978585227822492, 0.000000000000000000 ) ) ;
#10045=VECTOR ( 'NONE', #49690, 1000.000000000000000 ) ;
#10046=CARTESIAN_POINT ( 'NONE',  ( 102.2713888833019240, -44.80927359098731699, 203.5939642582779641 ) ) ;
#10048=CARTESIAN_POINT ( 'NONE',  ( 100.2657625843003899, -43.21224928579215430, 33.35205949637398959 ) ) ;
#10050=CARTESIAN_POINT ( 'NONE',  ( 115.0889047246006669, -30.61763668096888580, 79.34395860915145704 ) ) ;
#10053=FACE_OUTER_BOUND ( 'NONE', #17360, .T. ) ;
#10054=LINE ( 'NONE', #10493, #35736 ) ;
#10055=VERTEX_POINT ( 'NONE', #64787 ) ;
#10056=CARTESIAN_POINT ( 'NONE',  ( 99.55514648348071205, -29.48070623161989801, 250.7156252759109520 ) ) ;
#10058=EDGE_LOOP ( 'NONE', ( #1921, #38732, #57507, #10281 ) ) ;
#10059=AXIS2_PLACEMENT_3D ( 'NONE', #2314, #24095, #30897 ) ;
#10060=CARTESIAN_POINT ( 'NONE',  ( 165.3359832912747436, -36.32844715993532958, 313.9678068554149490 ) ) ;
#10061=CARTESIAN_POINT ( 'NONE',  ( 164.9667039024474491, -28.27351298636832766, 313.9678068554149490 ) ) ;
#10062=CARTESIAN_POINT ( 'NONE',  ( 107.0664832912739968, -36.72944715994100306, 287.6356252759109680 ) ) ;
#10065=CARTESIAN_POINT ( 'NONE',  ( 103.2878376434171628, -26.96651641063459337, 211.3699109901969848 ) ) ;
#10066=VECTOR ( 'NONE', #82564, 1000.000000000000000 ) ;
#10069=ORIENTED_EDGE ( 'NONE', *, *, #11842, .F. ) ;
#10070=CARTESIAN_POINT ( 'NONE',  ( 114.8518103909616315, -43.72813715869710904, 34.24419670448197905 ) ) ;
#10073=CARTESIAN_POINT ( 'NONE',  ( 100.2471064434660093, -45.42859581790747825, 277.0594347997204636 ) ) ;
#10075=CIRCLE ( 'NONE', #11568, 1.000000000000000888 ) ;
#10076=FACE_OUTER_BOUND ( 'NONE', #82013, .T. ) ;
#10077=CARTESIAN_POINT ( 'NONE',  ( 117.0716111955790808, -35.46010980090269982, 19.92736465657518963 ) ) ;
#10079=DIRECTION ( 'NONE',  ( -0.9254794337955620787, -0.3787978585227822492, 0.000000000000000000 ) ) ;
#10080=CARTESIAN_POINT ( 'NONE',  ( 104.1008407059626251, -44.85999997644839254, 95.10428084578198593 ) ) ;
#10081=CARTESIAN_POINT ( 'NONE',  ( 113.0378785334839193, -46.05830800173890793, 214.0175300378159591 ) ) ;
#10083=ORIENTED_EDGE ( 'NONE', *, *, #27713, .T. ) ;
#10085=PLANE ( 'NONE',  #37456 ) ;
#10086=VERTEX_POINT ( 'NONE', #56155 ) ;
#10089=DIRECTION ( 'NONE',  ( -4.237773401492740281E-14, 1.000000000000000000, 0.000000000000000000 ) ) ;
#10091=ORIENTED_EDGE ( 'NONE', *, *, #8218, .T. ) ;
#10092=CARTESIAN_POINT ( 'NONE',  ( 107.0664832912739399, -36.72944715994095333, 312.1356252759112522 ) ) ;
#10094=CIRCLE ( 'NONE', #4325, 2.750000000000002665 ) ;
#10095=CARTESIAN_POINT ( 'NONE',  ( 98.49703967840136443, -36.85882374884989332, 135.7609912566479409 ) ) ;
#10096=CARTESIAN_POINT ( 'NONE',  ( 97.31040724827032307, -32.83447933365327742, 41.02419670448193045 ) ) ;
#10098=EDGE_LOOP ( 'NONE', ( #34355, #17990 ) ) ;
#10099=ORIENTED_CLOSED_SHELL ( 'NONE', *, #85136, .F. );
#10100=CARTESIAN_POINT ( 'NONE',  ( 103.2778847236115780, -27.47490660443877886, 136.3856794586381511 ) ) ;
#10102=DIRECTION ( 'NONE',  ( -0.7071067811875186848, -0.7071067811855763496, -7.071067811875180294E-16 ) ) ;
#10103=DIRECTION ( 'NONE',  ( 1.000000000000000000, 0.000000000000000000, 0.000000000000000000 ) ) ;
#10104=DIRECTION ( 'NONE',  ( 0.000000000000000000, 0.000000000000000000, -1.000000000000000000 ) ) ;
#10106=CARTESIAN_POINT ( 'NONE',  ( 96.49234500119369784, -40.10591448887350197, 281.5603871806727625 ) ) ;
#10107=ORIENTED_EDGE ( 'NONE', *, *, #37291, .T. ) ;
#10108=CARTESIAN_POINT ( 'NONE',  ( 118.1032226039154267, -36.12160442421116358, 273.8822919425776945 ) ) ;
#10109=CARTESIAN_POINT ( 'NONE',  ( 101.3604548305157920, -27.95253318249931596, 21.53562527591096298 ) ) ;
#10110=CARTESIAN_POINT ( 'NONE',  ( 116.7951252708672456, -39.38782979237640802, 119.6147919423895019 ) ) ;
#10113=DIRECTION ( 'NONE',  ( 2.900000000000000265E-14, -2.000000000000000155E-15, 1.000000000000000000 ) ) ;
#10114=DIRECTION ( 'NONE',  ( 0.000000000000000000, 1.000000000000000000, 0.000000000000000000 ) ) ;
#10115=VECTOR ( 'NONE', #55027, 1000.000000000000000 ) ;
#10116=DIRECTION ( 'NONE',  ( 2.900000000000000265E-14, -2.000000000000000155E-15, 1.000000000000000000 ) ) ;
#10117=EDGE_CURVE ( 'NONE', #74315, #83594, #743, .T. ) ;
#10118=CARTESIAN_POINT ( 'NONE',  ( 117.0718015256225328, -35.46170398102030674, 163.9272027694907194 ) ) ;
#10120=AXIS2_PLACEMENT_3D ( 'NONE', #44287, #17498, #17055 ) ;
#10121=CARTESIAN_POINT ( 'NONE',  ( 99.73113825573250324, -44.24905506706784308, 21.96133956162593748 ) ) ;
#10122=CARTESIAN_POINT ( 'NONE',  ( 113.6855667929701923, -45.58166236755234024, 184.0994347997199725 ) ) ;
#10123=CARTESIAN_POINT ( 'NONE',  ( 116.7650972879214919, -32.84690348374694224, 50.12991099019698282 ) ) ;
#10124=LINE ( 'NONE', #44177, #44982 ) ;
#10125=CARTESIAN_POINT ( 'NONE',  ( 117.0718954852358706, -35.46248235588101494, 48.92729194260762426 ) ) ;
#10126=CARTESIAN_POINT ( 'NONE',  ( 179.4595971212889935, -28.98061976758940617, -5.074374724088000832 ) ) ;
#10128=VECTOR ( 'NONE', #26483, 1000.000000000000000 ) ;
#10130=CARTESIAN_POINT ( 'NONE',  ( 97.33784133995732191, -34.07106442700378324, 187.1147919341439660 ) ) ;
#10131=ORIENTED_EDGE ( 'NONE', *, *, #87867, .T. ) ;
#10132=CARTESIAN_POINT ( 'NONE',  ( 106.9359508110862578, -26.91635713860572920, 56.08705384733897148 ) ) ;
#10135=ORIENTED_EDGE ( 'NONE', *, *, #83445, .F. ) ;
#10137=CARTESIAN_POINT ( 'NONE',  ( 110.6887065042382545, -47.98678726807230532, 203.8241967044819489 ) ) ;
#10138=CARTESIAN_POINT ( 'NONE',  ( 57.56670390244732260, -48.82844715994040286, 175.7178068554150911 ) ) ;
#10139=CARTESIAN_POINT ( 'NONE',  ( 101.9935279254791993, -45.44601432983314737, 147.1565244394456897 ) ) ;
#10142=CARTESIAN_POINT ( 'NONE',  ( 34.67381068362099228, -26.00627455219321860, 342.9256252759119548 ) ) ;
#10143=CARTESIAN_POINT ( 'NONE',  ( 99.09570906733897289, -30.55043176429327545, 46.80229194367134227 ) ) ;
#10144=LINE ( 'NONE', #2887, #50488 ) ;
#10145=CARTESIAN_POINT ( 'NONE',  ( 98.15093366565197641, -41.26152608243540243, 96.70072996894096207 ) ) ;
#10147=CARTESIAN_POINT ( 'NONE',  ( 116.4171719250473984, -30.71472603919669098, 144.2813395616259697 ) ) ;
#10148=VERTEX_POINT ( 'NONE', #57515 ) ;
#10149=VERTEX_POINT ( 'NONE', #43426 ) ;
#10150=CARTESIAN_POINT ( 'NONE',  ( 99.48689454471329441, -42.28159629070200509, 103.2492023535159831 ) ) ;
#10151=CARTESIAN_POINT ( 'NONE',  ( 25.56670390244797275, -58.35344715994099829, 293.2178068554150627 ) ) ;
#10152=CARTESIAN_POINT ( 'NONE',  ( 96.81359797424460112, -35.17473563989039320, 217.1946728949579608 ) ) ;
#10154=CARTESIAN_POINT ( 'NONE',  ( 138.8167039024479834, -57.40094715994099772, 88.43480685541499042 ) ) ;
#10161=CARTESIAN_POINT ( 'NONE',  ( 111.4081670832169237, -47.72935575799012753, 172.8756252759109771 ) ) ;
#10162=VERTEX_POINT ( 'NONE', #1228 ) ;
#10167=CARTESIAN_POINT ( 'NONE',  ( 113.1780517095743477, -44.75205797978776445, 104.0939343869516449 ) ) ;
#10169=DIRECTION ( 'NONE',  ( -0.9068632946707808618, 0.4214249218767877059, 0.000000000000000000 ) ) ;
#10172=CARTESIAN_POINT ( 'NONE',  ( 102.0509295376110117, -46.57948817496540528, 172.2137205140059564 ) ) ;
#10174=ORIENTED_EDGE ( 'NONE', *, *, #51929, .F. ) ;
#10175=EDGE_LOOP ( 'NONE', ( #8529, #47975, #81461, #54697 ) ) ;
#10176=ORIENTED_EDGE ( 'NONE', *, *, #57413, .T. ) ;
#10177=AXIS2_PLACEMENT_3D ( 'NONE', #7806, #63671, #49568 ) ;
#10178=CARTESIAN_POINT ( 'NONE',  ( 110.3946058071659024, -46.19501636738639405, 63.84634919539954012 ) ) ;
#10179=CARTESIAN_POINT ( 'NONE',  ( 72.26949937496598864, -71.54137415153812185, 361.9756252759101471 ) ) ;
#10180=CARTESIAN_POINT ( 'NONE',  ( 133.1188885517861991, -34.14703303315379657, 8.087249882926339950 ) ) ;
#10181=CARTESIAN_POINT ( 'NONE',  ( 115.8755296135227724, -35.76560983836216678, 275.3444404487542556 ) ) ;
#10182=VECTOR ( 'NONE', #42721, 1000.000000000000000 ) ;
#10184=EDGE_LOOP ( 'NONE', ( #70204, #48138, #57097, #54140 ) ) ;
#10185=CARTESIAN_POINT ( 'NONE',  ( 115.0891813775823920, -41.06744293826255188, 9.635625275910941312 ) ) ;
#10187=ORIENTED_EDGE ( 'NONE', *, *, #83020, .T. ) ;
#10189=EDGE_LOOP ( 'NONE', ( #46755, #38718, #10091, #69521 ) ) ;
#10191=CARTESIAN_POINT ( 'NONE',  ( 116.3347860427986120, -40.61045514847694449, 113.5106497359954290 ) ) ;
#10193=ORIENTED_EDGE ( 'NONE', *, *, #71546, .F. ) ;
#10194=CARTESIAN_POINT ( 'NONE',  ( 101.6694414210978294, -29.45726664942652917, 35.01908649474394508 ) ) ;
#10195=TOROIDAL_SURFACE ( 'NONE', #44992, 11.75000000000000000, 2.550000000000000266 ) ;
#10196=EDGE_CURVE ( 'NONE', #61676, #81923, #62136, .T. ) ;
#10197=CARTESIAN_POINT ( 'NONE',  ( 98.24258143063333648, -42.32275744278853580, 186.7756252759109543 ) ) ;
#10198=CARTESIAN_POINT ( 'NONE',  ( 117.0123300003821640, -30.33189756676010163, 144.2813395616249750 ) ) ;
#10200=CARTESIAN_POINT ( 'NONE',  ( 118.6539291974399219, -39.21253252500506647, 254.6584824187681022 ) ) ;
#10201=FACE_OUTER_BOUND ( 'NONE', #35231, .T. ) ;
#10203=EDGE_CURVE ( 'NONE', #27885, #59978, #27323, .T. ) ;
#10204=ORIENTED_EDGE ( 'NONE', *, *, #72427, .T. ) ;
#10205=ADVANCED_FACE ( 'NONE', ( #81119 ), #87019, .T. ) ;
#10206=ORIENTED_EDGE ( 'NONE', *, *, #63390, .F. ) ;
#10207=VECTOR ( 'NONE', #12229, 1000.000000000000000 ) ;
#10208=CARTESIAN_POINT ( 'NONE',  ( 113.0474237710022578, -45.36542684395109148, 203.0584824187679374 ) ) ;
#10209=ORIENTED_EDGE ( 'NONE', *, *, #58077, .T. ) ;
#10210=CARTESIAN_POINT ( 'NONE',  ( 98.66574799139598895, -30.49618532553466110, 180.8184824187679567 ) ) ;
#10211=DIRECTION ( 'NONE',  ( 1.000000000000000078E-15, 1.000000000000000083E-30, -1.000000000000000000 ) ) ;
#10212=EDGE_CURVE ( 'NONE', #26208, #6412, #32035, .T. ) ;
#10215=CYLINDRICAL_SURFACE ( 'NONE', #46205, 0.4999999999999994449 ) ;
#10216=DIRECTION ( 'NONE',  ( -1.000000000000000000, 9.251858538542979716E-16, 0.000000000000000000 ) ) ;
#10217=CARTESIAN_POINT ( 'NONE',  ( 117.4080659314678314, -35.59792815749688089, 274.9127681330538735 ) ) ;
#10218=CYLINDRICAL_SURFACE ( 'NONE', #1716, 11.45913725231036118 ) ;
#10219=DIRECTION ( 'NONE',  ( 0.000000000000000000, 0.000000000000000000, -1.000000000000000000 ) ) ;
#10220=AXIS2_PLACEMENT_3D ( 'NONE', #5939, #20009, #26806 ) ;
#10221=CARTESIAN_POINT ( 'NONE',  ( 149.4532656544376721, -72.54365454176046057, 361.9756252759100335 ) ) ;
#10222=DIRECTION ( 'NONE',  ( 0.000000000000000000, 0.000000000000000000, -1.000000000000000000 ) ) ;
#10224=EDGE_CURVE ( 'NONE', #19595, #26178, #10266, .T. ) ;
#10226=CARTESIAN_POINT ( 'NONE',  ( 101.4389981506307237, -42.56717821295191584, 195.5838068554170377 ) ) ;
#10228=CARTESIAN_POINT ( 'NONE',  ( 90.44969454456408187, -20.11243780205710507, 239.5838068554175209 ) ) ;
#10229=CARTESIAN_POINT ( 'NONE',  ( 108.1841437630847338, -47.11680481413669952, 202.6613395616249704 ) ) ;
#10230=CARTESIAN_POINT ( 'NONE',  ( 96.65662162753720565, -37.29271227441797265, 72.36991099019596163 ) ) ;
#10231=CARTESIAN_POINT ( 'NONE',  ( 100.6295653500825154, -44.98529764103543727, 228.0499109901969348 ) ) ;
#10233=LINE ( 'NONE', #37938, #1101 ) ;
#10234=AXIS2_PLACEMENT_3D ( 'NONE', #52574, #4911, #18988 ) ;
#10235=PLANE ( 'NONE',  #18870 ) ;
#10237=DIRECTION ( 'NONE',  ( 4.299999999999999979E-14, -1.000000000000000000, 0.000000000000000000 ) ) ;
#10238=CARTESIAN_POINT ( 'NONE',  ( 107.0667039024479834, -48.82844715994099971, 160.9178068554150229 ) ) ;
#10239=LINE ( 'NONE', #72906, #77620 ) ;
#10240=VERTEX_POINT ( 'NONE', #31146 ) ;
#10241=EDGE_LOOP ( 'NONE', ( #29274, #17213, #47247, #38005 ) ) ;
#10242=CARTESIAN_POINT ( 'NONE',  ( 108.2720842404240926, -28.27352272357859420, 104.3867055423629608 ) ) ;
#10245=ORIENTED_EDGE ( 'NONE', *, *, #6455, .T. ) ;
#10246=CARTESIAN_POINT ( 'NONE',  ( 116.9011659702703270, -33.23038410113878882, 110.0984824187679578 ) ) ;
#10247=FACE_OUTER_BOUND ( 'NONE', #22024, .T. ) ;
#10248=EDGE_CURVE ( 'NONE', #43365, #83807, #31587, .T. ) ;
#10250=AXIS2_PLACEMENT_3D ( 'NONE', #58593, #2321, #37277 ) ;
#10251=CARTESIAN_POINT ( 'NONE',  ( 77.71552635664387765, -17.29868341350664451, 7.242354772871751223 ) ) ;
#10252=CARTESIAN_POINT ( 'NONE',  ( 99.09570909151958062, -30.55043173361417175, 176.8022919406010374 ) ) ;
#10254=CARTESIAN_POINT ( 'NONE',  ( 107.1874307469290386, -26.94942635195914349, 35.06705384733993469 ) ) ;
#10255=VERTEX_POINT ( 'NONE', #59731 ) ;
#10256=ORIENTED_EDGE ( 'NONE', *, *, #69689, .F. ) ;
#10257=AXIS2_PLACEMENT_3D ( 'NONE', #35005, #496, #89544 ) ;
#10260=LINE ( 'NONE', #23466, #18631 ) ;
#10262=FACE_OUTER_BOUND ( 'NONE', #35085, .T. ) ;
#10264=CARTESIAN_POINT ( 'NONE',  ( 112.1400935167290100, -28.01325122303620319, 50.65751264254551955 ) ) ;
#10266=LINE ( 'NONE', #3008, #23011 ) ;
#10268=CARTESIAN_POINT ( 'NONE',  ( 97.79189512308828114, -32.01662636557816199, 50.95276813305294183 ) ) ;
#10269=ORIENTED_EDGE ( 'NONE', *, *, #47623, .F. ) ;
#10270=VERTEX_POINT ( 'NONE', #46093 ) ;
#10271=DIRECTION ( 'NONE',  ( 1.000000000000000078E-15, -1.000000000000000083E-30, -1.000000000000000000 ) ) ;
#10273=DIRECTION ( 'NONE',  ( -0.04216478779797398074, 0.9991106698809455455, 0.000000000000000000 ) ) ;
#10274=CARTESIAN_POINT ( 'NONE',  ( 98.42339386660059120, -37.17434067858062008, 119.1976141791149786 ) ) ;
#10275=CARTESIAN_POINT ( 'NONE',  ( 104.4870417173576556, -26.97960265801549795, 95.28170196733614716 ) ) ;
#10278=VERTEX_POINT ( 'NONE', #17960 ) ;
#10281=ORIENTED_EDGE ( 'NONE', *, *, #15477, .F. ) ;
#10284=CARTESIAN_POINT ( 'NONE',  ( 112.6324721509601545, -29.83393797428842831, 160.9672975916109579 ) ) ;
#10285=CARTESIAN_POINT ( 'NONE',  ( 172.5667039024478413, -36.32844715993500273, 249.9678068554149775 ) ) ;
#10287=CARTESIAN_POINT ( 'NONE',  ( 100.8735899011331014, -45.91031909761725416, 148.0918157521009562 ) ) ;
#10288=CARTESIAN_POINT ( 'NONE',  ( 113.2454987219876728, -28.75867296460453559, 119.5522919401142445 ) ) ;
#10292=EDGE_CURVE ( 'NONE', #64140, #37193, #87463, .T. ) ;
#10294=ORIENTED_EDGE ( 'NONE', *, *, #67526, .T. ) ;
#10295=ADVANCED_FACE ( 'NONE', ( #37966 ), #46548, .T. ) ;
#10296=CARTESIAN_POINT ( 'NONE',  ( 100.3991921706488171, -43.18259834960616672, 189.7566617981629804 ) ) ;
#10297=EDGE_CURVE ( 'NONE', #26172, #43699, #31462, .T. ) ;
#10298=CARTESIAN_POINT ( 'NONE',  ( 112.7719768816358936, -27.93537496831996592, 69.61848241876793963 ) ) ;
#10300=CARTESIAN_POINT ( 'NONE',  ( 115.5559444348971851, -42.74257571503951425, 53.33562527591095659 ) ) ;
#10301=CARTESIAN_POINT ( 'NONE',  ( 97.81085527707094229, -40.51777768585955641, 251.6359959587111064 ) ) ;
#10304=CARTESIAN_POINT ( 'NONE',  ( 98.28086921530724851, -31.05189054518432101, 141.8699109901969564 ) ) ;
#10306=ORIENTED_EDGE ( 'NONE', *, *, #15906, .T. ) ;
#10307=DIRECTION ( 'NONE',  ( 1.000000000000000078E-15, -1.000000000000000083E-30, -1.000000000000000000 ) ) ;
#10310=ADVANCED_FACE ( 'NONE', ( #66557 ), #87909, .F. ) ;
#10312=DIRECTION ( 'NONE',  ( -1.000000000000000078E-15, 1.000000000000000083E-30, 1.000000000000000000 ) ) ;
#10314=ORIENTED_EDGE ( 'NONE', *, *, #6781, .F. ) ;
#10315=AXIS2_PLACEMENT_3D ( 'NONE', #85327, #15379, #1746 ) ;
#10316=EDGE_CURVE ( 'NONE', #74086, #65069, #17086, .T. ) ;
#10317=DIRECTION ( 'NONE',  ( -4.237773401492740281E-14, 1.000000000000000000, 0.000000000000000000 ) ) ;
#10318=CARTESIAN_POINT ( 'NONE',  ( 97.81170212845945855, -40.51743756719207568, 176.6354241348688277 ) ) ;
#10319=CARTESIAN_POINT ( 'NONE',  ( 112.8178475080015772, -27.29012000701139939, 49.62895860924498947 ) ) ;
#10320=PLANE ( 'NONE',  #59071 ) ;
#10323=DIRECTION ( 'NONE',  ( -0.9254794337955620787, -0.3787978585227822492, 0.000000000000000000 ) ) ;
#10324=CARTESIAN_POINT ( 'NONE',  ( 116.7176835877704946, -38.50936494796418685, 88.68133956162593279 ) ) ;
#10326=CARTESIAN_POINT ( 'NONE',  ( 109.4403364888816981, -25.95778788316477304, 175.8918157521009391 ) ) ;
#10327=DIRECTION ( 'NONE',  ( 0.000000000000000000, 0.000000000000000000, 1.000000000000000000 ) ) ;
#10333=CARTESIAN_POINT ( 'NONE',  ( 108.4192877796676555, -26.73525438302016966, 134.9688338521367257 ) ) ;
#10334=CIRCLE ( 'NONE', #63965, 4.750000000000004441 ) ;
#10336=CARTESIAN_POINT ( 'NONE',  ( 162.7131505118679797, -31.94127993907790852, -5.074374724088000832 ) ) ;
#10337=CARTESIAN_POINT ( 'NONE',  ( 115.5532354207493171, -29.57487366316678745, 224.3718157521009573 ) ) ;
#10339=FACE_OUTER_BOUND ( 'NONE', #88951, .T. ) ;
#10340=CARTESIAN_POINT ( 'NONE',  ( 104.3186933571878399, -25.99935600364358024, 241.2880062282919482 ) ) ;
#10341=CARTESIAN_POINT ( 'NONE',  ( 114.1102230946791707, -44.52199131239810015, 129.1613395616249704 ) ) ;
#10343=CARTESIAN_POINT ( 'NONE',  ( 80.44329752325863581, -39.47944369577015067, 8.225625303283912615 ) ) ;
#10344=DIRECTION ( 'NONE',  ( 0.000000000000000000, 0.000000000000000000, -1.000000000000000000 ) ) ;
#10346=ORIENTED_EDGE ( 'NONE', *, *, #15764, .F. ) ;
#10347=ORIENTED_EDGE ( 'NONE', *, *, #80633, .T. ) ;
#10352=CARTESIAN_POINT ( 'NONE',  ( 117.4297252914212066, -35.59555830959087075, 274.9127681330538735 ) ) ;
#10355=EDGE_CURVE ( 'NONE', #82750, #78071, #72927, .T. ) ;
#10358=ADVANCED_FACE ( 'NONE', ( #3892 ), #68807, .T. ) ;
#10359=CYLINDRICAL_SURFACE ( 'NONE', #80574, 0.5000000000000104361 ) ;
#10360=VECTOR ( 'NONE', #31878, 1000.000000000000000 ) ;
#10361=CARTESIAN_POINT ( 'NONE',  ( 99.94932728663779642, -31.12955780999732980, 200.2305150661719892 ) ) ;
#10363=EDGE_LOOP ( 'NONE', ( #46261, #11269 ) ) ;
#10364=ORIENTED_EDGE ( 'NONE', *, *, #27657, .T. ) ;
#10365=AXIS2_PLACEMENT_3D ( 'NONE', #79811, #59330, #58439 ) ;
#10369=CARTESIAN_POINT ( 'NONE',  ( 115.9938408324894539, -42.00591253359444011, 279.4137205140056608 ) ) ;
#10372=CARTESIAN_POINT ( 'NONE',  ( 115.7824607000603123, -41.80340193948442362, 28.40635853151320589 ) ) ;
#10373=AXIS2_PLACEMENT_3D ( 'NONE', #76964, #41969, #35160 ) ;
#10375=CARTESIAN_POINT ( 'NONE',  ( 37.56670390244828184, -48.82844715994119866, 300.4678068554150059 ) ) ;
#10376=ORIENTED_EDGE ( 'NONE', *, *, #3237, .T. ) ;
#10377=CARTESIAN_POINT ( 'NONE',  ( 36.23715912545344509, -47.82818131006131779, 117.4678068554150485 ) ) ;
#10378=CARTESIAN_POINT ( 'NONE',  ( 115.7905465638341553, -39.88961339014866070, 21.36809036959191843 ) ) ;
#10379=VECTOR ( 'NONE', #76132, 1000.000000000000000 ) ;
#10380=CARTESIAN_POINT ( 'NONE',  ( 90.44969454456415292, -53.34645651782494724, 229.5838068554169809 ) ) ;
#10381=CARTESIAN_POINT ( 'NONE',  ( 97.95250717983367394, -32.49412669507730556, 0.4256252759109618311 ) ) ;
#10382=VECTOR ( 'NONE', #30205, 1000.000000000000114 ) ;
#10383=DIRECTION ( 'NONE',  ( 4.299999999999999979E-14, -1.000000000000000000, 4.400000000000000367E-29 ) ) ;
#10384=EDGE_LOOP ( 'NONE', ( #66042, #43587, #23502, #24758 ) ) ;
#10386=CARTESIAN_POINT ( 'NONE',  ( 168.0371591254545365, -48.62818131005519007, 193.9678068554149775 ) ) ;
#10387=VERTEX_POINT ( 'NONE', #6143 ) ;
#10388=CARTESIAN_POINT ( 'NONE',  ( 117.3714642245996629, -32.73114059124436892, 94.10895860924395606 ) ) ;
#10390=CARTESIAN_POINT ( 'NONE',  ( 114.9961339231967798, -33.55505389859023069, 53.55241982807695678 ) ) ;
#10392=CARTESIAN_POINT ( 'NONE',  ( 116.0020177893944435, -41.25514887265125452, 89.45255704496776161 ) ) ;
#10393=CARTESIAN_POINT ( 'NONE',  ( 97.73412737207827661, -37.81740788287748956, 82.86253568684892912 ) ) ;
#10398=CARTESIAN_POINT ( 'NONE',  ( 111.3320466151124322, -27.19308368994588676, 20.74133956162494030 ) ) ;
#10399=LINE ( 'NONE', #37666, #46665 ) ;
#10400=ORIENTED_EDGE ( 'NONE', *, *, #67614, .F. ) ;
#10401=CARTESIAN_POINT ( 'NONE',  ( 194.0371591254582881, -46.82818131005408446, 237.4678068554150059 ) ) ;
#10402=EDGE_LOOP ( 'NONE', ( #42548, #72070 ) ) ;
#10403=CARTESIAN_POINT ( 'NONE',  ( 78.42773927738237205, -20.94013506381011425, 2.060080721656760705 ) ) ;
#10404=ORIENTED_EDGE ( 'NONE', *, *, #12172, .T. ) ;
#10405=ORIENTED_EDGE ( 'NONE', *, *, #57344, .T. ) ;
#10406=EDGE_CURVE ( 'NONE', #82390, #19111, #26568, .T. ) ;
#10408=AXIS2_PLACEMENT_3D ( 'NONE', #36825, #70910, #72242 ) ;
#10409=FACE_OUTER_BOUND ( 'NONE', #86279, .T. ) ;
#10410=ADVANCED_FACE ( 'NONE', ( #6576 ), #88815, .T. ) ;
#10411=CARTESIAN_POINT ( 'NONE',  ( 101.7025241355416796, -45.60450926735023813, 202.1318157521019430 ) ) ;
#10412=CARTESIAN_POINT ( 'NONE',  ( 104.8368789347731536, -26.95710669931445125, 125.2537966132911436 ) ) ;
#10414=CARTESIAN_POINT ( 'NONE',  ( 96.33847535375279847, -41.76377544194641445, 57.67562527591096710 ) ) ;
#10415=LINE ( 'NONE', #51726, #33404 ) ;
#10416=ORIENTED_EDGE ( 'NONE', *, *, #81289, .T. ) ;
#10417=CARTESIAN_POINT ( 'NONE',  ( 103.3097373732736912, -27.46191326970934909, 171.3829422610906761 ) ) ;
#10418=ADVANCED_FACE ( 'NONE', ( #34726 ), #41085, .T. ) ;
#10419=LINE ( 'NONE', #3601, #62209 ) ;
#10420=ORIENTED_EDGE ( 'NONE', *, *, #63881, .T. ) ;
#10421=EDGE_CURVE ( 'NONE', #19365, #53353, #13396, .T. ) ;
#10422=AXIS2_PLACEMENT_3D ( 'NONE', #76560, #50175, #64719 ) ;
#10423=LINE ( 'NONE', #4946, #18434 ) ;
#10424=CARTESIAN_POINT ( 'NONE',  ( 188.5667039024479834, -67.87844715994100397, 257.2178068554150059 ) ) ;
#10425=CARTESIAN_POINT ( 'NONE',  ( 107.2488531970940073, -24.90511003128400347, 230.0641967044819580 ) ) ;
#10426=DIRECTION ( 'NONE',  ( 0.7071067811868693154, 0.7071067811862258301, -2.899137802863410076E-29 ) ) ;
#10427=FACE_BOUND ( 'NONE', #14936, .T. ) ;
#10428=CARTESIAN_POINT ( 'NONE',  ( 77.31648329127401098, -36.72944715994107412, 3.101481641215480867 ) ) ;
#10430=CARTESIAN_POINT ( 'NONE',  ( 101.8914336387190502, -44.16123909860101548, 236.5028960185529456 ) ) ;
#10431=CARTESIAN_POINT ( 'NONE',  ( 151.0371591254585155, -46.82818131005592477, 129.9678068554149775 ) ) ;
#10432=CARTESIAN_POINT ( 'NONE',  ( 107.3204973292724134, -25.70223992296343241, 71.04610146638795243 ) ) ;
#10434=CARTESIAN_POINT ( 'NONE',  ( 104.9539341177782177, -25.01766106605714768, 125.2184824187689856 ) ) ;
#10436=CARTESIAN_POINT ( 'NONE',  ( 132.9232751754135222, -21.23064218986711893, 8.021355262920867091 ) ) ;
#10437=VERTEX_POINT ( 'NONE', #83335 ) ;
#10438=DIRECTION ( 'NONE',  ( 1.000000000000000000, 4.299999999999999979E-14, 1.000000000000000078E-15 ) ) ;
#10439=CARTESIAN_POINT ( 'NONE',  ( 172.5664832912740110, 0.2215528400590013880, 196.8086252759119645 ) ) ;
#10442=CIRCLE ( 'NONE', #61197, 2.030000000000003801 ) ;
#10445=CARTESIAN_POINT ( 'NONE',  ( 114.0516219551475245, -28.93108169718528444, 114.4956252759109816 ) ) ;
#10446=ORIENTED_EDGE ( 'NONE', *, *, #22282, .F. ) ;
#10447=CARTESIAN_POINT ( 'NONE',  ( 168.0371591254543091, -48.62818131005519717, 313.9678068554149490 ) ) ;
#10448=LINE ( 'NONE', #15934, #86778 ) ;
#10451=ORIENTED_EDGE ( 'NONE', *, *, #48121, .T. ) ;
#10452=VECTOR ( 'NONE', #26713, 1000.000000000000000 ) ;
#10453=CARTESIAN_POINT ( 'NONE',  ( 97.91311022844104173, -31.62022761154550210, 110.9213395616259703 ) ) ;
#10458=VERTEX_POINT ( 'NONE', #67905 ) ;
#10459=AXIS2_PLACEMENT_3D ( 'NONE', #24077, #88089, #51299 ) ;
#10460=EDGE_LOOP ( 'NONE', ( #15861, #83793, #36202, #61115 ) ) ;
#10461=DIRECTION ( 'NONE',  ( 0.000000000000000000, 0.000000000000000000, -1.000000000000000000 ) ) ;
#10466=CARTESIAN_POINT ( 'NONE',  ( 116.9517947088517218, -38.63056867187965793, 249.6760957642232484 ) ) ;
#10469=CARTESIAN_POINT ( 'NONE',  ( 134.0664832912740110, 0.2215528400590013880, 7.443125275912000127 ) ) ;
#10471=CARTESIAN_POINT ( 'NONE',  ( 116.7951252848263692, -39.38782973560361000, 34.61479194698554096 ) ) ;
#10472=CARTESIAN_POINT ( 'NONE',  ( 96.28008679191522390, -39.42493101749851547, 162.5213395616249841 ) ) ;
#10473=DIRECTION ( 'NONE',  ( 0.7071067811987160612, 0.7071067811743789733, 0.000000000000000000 ) ) ;
#10474=ORIENTED_EDGE ( 'NONE', *, *, #62910, .T. ) ;
#10475=CARTESIAN_POINT ( 'NONE',  ( 106.5519926023875712, -26.37212682281792198, 41.12800622829093555 ) ) ;
#10476=CARTESIAN_POINT ( 'NONE',  ( 97.92339011489026745, -40.78105927379723283, 51.65841521686554927 ) ) ;
#10477=DIRECTION ( 'NONE',  ( 1.000000000000000078E-15, -1.000000000000000083E-30, -1.000000000000000000 ) ) ;
#10479=EDGE_CURVE ( 'NONE', #8418, #87481, #12689, .T. ) ;
#10480=CARTESIAN_POINT ( 'NONE',  ( 83.06670390244796920, -67.87844715994100397, 237.1838068554150141 ) ) ;
#10481=VERTEX_POINT ( 'NONE', #19314 ) ;
#10482=AXIS2_PLACEMENT_3D ( 'NONE', #20738, #41161, #13039 ) ;
#10483=ORIENTED_EDGE ( 'NONE', *, *, #38941, .F. ) ;
#10484=CARTESIAN_POINT ( 'NONE',  ( 106.5710281304903901, -26.66837221057895846, 191.5472975916109704 ) ) ;
#10485=CIRCLE ( 'NONE', #38053, 13.49999999999999822 ) ;
#10486=EDGE_CURVE ( 'NONE', #68920, #69055, #40211, .T. ) ;
#10487=LINE ( 'NONE', #38187, #86467 ) ;
#10490=CARTESIAN_POINT ( 'NONE',  ( 107.0664832912739399, -36.72944715994096754, 296.5517437918485939 ) ) ;
#10491=ORIENTED_EDGE ( 'NONE', *, *, #61889, .T. ) ;
#10493=CARTESIAN_POINT ( 'NONE',  ( 184.3595971212623112, -48.62134037874549364, 300.4678068554149490 ) ) ;
#10495=CARTESIAN_POINT ( 'NONE',  ( 116.9047011640240754, -41.71676023082953577, 248.4651490854349731 ) ) ;
#10497=ORIENTED_EDGE ( 'NONE', *, *, #85801, .F. ) ;
#10498=AXIS2_PLACEMENT_3D ( 'NONE', #13512, #41198, #68922 ) ;
#10499=DIRECTION ( 'NONE',  ( 1.000000000000000000, 4.163336342344333240E-14, 0.000000000000000000 ) ) ;
#10500=CARTESIAN_POINT ( 'NONE',  ( 63.03715912545732181, -24.89890238295017966, 300.4678068554150627 ) ) ;
#10501=CYLINDRICAL_SURFACE ( 'NONE', #65024, 2.117000000000007987 ) ;
#10502=DIRECTION ( 'NONE',  ( 1.000000000000000000, 0.000000000000000000, 0.000000000000000000 ) ) ;
#10503=CARTESIAN_POINT ( 'NONE',  ( 116.3890555338844450, -44.12544333927958462, 194.2927681330539542 ) ) ;
#10507=CARTESIAN_POINT ( 'NONE',  ( 112.2026027939200361, -27.56657145192123082, 30.66991099019694644 ) ) ;
#10509=CARTESIAN_POINT ( 'NONE',  ( 115.6954802162012044, -42.57986958318428350, 273.3527681330537575 ) ) ;
#10510=EDGE_CURVE ( 'NONE', #67090, #35473, #12053, .T. ) ;
#10511=EDGE_CURVE ( 'NONE', #20321, #73048, #39741, .T. ) ;
#10512=ORIENTED_EDGE ( 'NONE', *, *, #14902, .T. ) ;
#10513=EDGE_CURVE ( 'NONE', #54496, #72895, #57604, .T. ) ;
#10514=CARTESIAN_POINT ( 'NONE',  ( 80.81118397279384169, -16.08035908359608612, 1.709393751552206631 ) ) ;
#10515=CARTESIAN_POINT ( 'NONE',  ( 113.1794018818664398, -44.75104475741103016, 19.09459687979077458 ) ) ;
#10516=DIRECTION ( 'NONE',  ( 1.387778780781444492E-15, 0.000000000000000000, -1.000000000000000000 ) ) ;
#10517=CARTESIAN_POINT ( 'NONE',  ( 112.5126453671185942, -30.64922967528412556, 112.3138046553059723 ) ) ;
#10518=CARTESIAN_POINT ( 'NONE',  ( 100.6242249862060731, -26.75349815150567778, 216.5327681330539633 ) ) ;
#10521=EDGE_CURVE ( 'NONE', #31120, #29962, #19762, .T. ) ;
#10522=CARTESIAN_POINT ( 'NONE',  ( 136.6090958654756662, -37.77717416134755268, 2.822018739141234800 ) ) ;
#10523=B_SPLINE_CURVE_WITH_KNOTS ( 'NONE', 3,
 ( #22587, #49814, #56172, #37102, #9844, #64805, #30284, #57979, #22149, #36203, #57533, #23489, #63917, #1693, #37549, #84819, #64361, #71186, #14880, #77999, #51156, #42992, #70733, #56631, #77541, #42545, #15768, #78896, #1243 ),
 .UNSPECIFIED., .F., .F.,
 ( 4, 2, 1, 1, 1, 1, 1, 2, 2, 2, 2, 2, 2, 2, 2, 2, 4 ),
 ( 0.5000903094201638588, 0.5003344059487672135, 0.5005785024773704572, 0.5010666955345773887, 0.5020430816489914738, 0.5039958538778193109, 0.5079013983354746520, 0.5157124872507848901, 0.5313346650814048111, 0.5625790207426447642, 0.6250677320651241153, 0.6875564433876033554, 0.7500451547100827066, 0.8125338660325620577, 0.8750225773550412978, 0.9375112886775206489, 1.000000000000000000 ),
 .UNSPECIFIED. ) ;
#10525=ORIENTED_EDGE ( 'NONE', *, *, #76339, .F. ) ;
#10526=CARTESIAN_POINT ( 'NONE',  ( 172.5664832912740110, 0.2215528400590013880, 78.92562527591199739 ) ) ;
#10527=ORIENTED_EDGE ( 'NONE', *, *, #4425, .F. ) ;
#10529=CARTESIAN_POINT ( 'NONE',  ( 152.0371591254585724, -47.82818131005588214, 129.9678068554149775 ) ) ;
#10530=LINE ( 'NONE', #14340, #29767 ) ;
#10531=CARTESIAN_POINT ( 'NONE',  ( 106.4620492377333392, -26.72629803759836520, 41.12456998439165545 ) ) ;
#10532=EDGE_CURVE ( 'NONE', #45, #17090, #75173, .T. ) ;
#10533=CARTESIAN_POINT ( 'NONE',  ( 115.0376279413645761, -33.66073653188622927, 138.5409912566489652 ) ) ;
#10534=CARTESIAN_POINT ( 'NONE',  ( 109.6227372377152847, -25.10643708164309018, 29.90419670448196854 ) ) ;
#10535=ORIENTED_EDGE ( 'NONE', *, *, #5420, .F. ) ;
#10538=ORIENTED_EDGE ( 'NONE', *, *, #6118, .F. ) ;
#10539=DIRECTION ( 'NONE',  ( 0.000000000000000000, 0.000000000000000000, 1.000000000000000000 ) ) ;
#10541=CARTESIAN_POINT ( 'NONE',  ( 179.4595971212735890, -26.00627455218472406, 117.4678068554150627 ) ) ;
#10542=CARTESIAN_POINT ( 'NONE',  ( 71.24189083761808661, -0.9290567490904538817, 540.9756252759101471 ) ) ;
#10543=DIRECTION ( 'NONE',  ( -1.000000000000000000, -1.000000000000000078E-15, -1.000000000000000078E-15 ) ) ;
#10544=VECTOR ( 'NONE', #41772, 1000.000000000000000 ) ;
#10545=DIRECTION ( 'NONE',  ( 1.387778780781444492E-15, 0.000000000000000000, -1.000000000000000000 ) ) ;
#10547=CARTESIAN_POINT ( 'NONE',  ( 103.0904226585672916, -47.89329182393425555, 252.3041967044823366 ) ) ;
#10548=CARTESIAN_POINT ( 'NONE',  ( 110.5697598356958764, -46.63222799359486714, 33.84705384733993583 ) ) ;
#10549=DIRECTION ( 'NONE',  ( -0.7071067812162665778, -0.7071067811568285677, -7.071067812162659944E-16 ) ) ;
#10550=CARTESIAN_POINT ( 'NONE',  ( 107.0667039024479834, -36.72944715994100306, 239.5838068554170093 ) ) ;
#10553=CARTESIAN_POINT ( 'NONE',  ( 48.85858412957961860, -30.08671355700278127, 193.9678068554150911 ) ) ;
#10554=CARTESIAN_POINT ( 'NONE',  ( 115.0889047207443525, -30.61763667517494980, 10.34395860968370862 ) ) ;
#10556=FACE_OUTER_BOUND ( 'NONE', #80709, .T. ) ;
#10557=CARTESIAN_POINT ( 'NONE',  ( 105.8910851810002356, -47.14611527663348056, 282.4870538473393253 ) ) ;
#10558=CARTESIAN_POINT ( 'NONE',  ( 113.0221554258835823, -45.32894145911351558, 199.0584824187679374 ) ) ;
#10559=CARTESIAN_POINT ( 'NONE',  ( 100.9283148882350787, -46.89532829952024429, 48.14419670448194211 ) ) ;
#10561=CARTESIAN_POINT ( 'NONE',  ( 112.0659116242543263, -45.48839625953056043, 47.98979194274246396 ) ) ;
#10563=CARTESIAN_POINT ( 'NONE',  ( 151.0371591254582881, -46.82818131005593187, 249.9678068554149490 ) ) ;
#10564=VECTOR ( 'NONE', #39476, 1000.000000000000000 ) ;
#10565=EDGE_CURVE ( 'NONE', #64058, #22586, #70602, .T. ) ;
#10566=ORIENTED_EDGE ( 'NONE', *, *, #15989, .T. ) ;
#10569=VECTOR ( 'NONE', #5192, 999.9999999999998863 ) ;
#10570=CARTESIAN_POINT ( 'NONE',  ( 115.6651410650258214, -32.06827565682262815, 65.22133956162495849 ) ) ;
#10571=DIRECTION ( 'NONE',  ( -0.7071067811607679721, 0.7071067812123270624, 0.000000000000000000 ) ) ;
#10572=VERTEX_POINT ( 'NONE', #49688 ) ;
#10574=CARTESIAN_POINT ( 'NONE',  ( 106.9751875180390641, -47.13234726572959232, 183.5699109901969734 ) ) ;
#10576=DIRECTION ( 'NONE',  ( -2.900000000000000265E-14, 2.000000000000000155E-15, -1.000000000000000000 ) ) ;
#10577=DIRECTION ( 'NONE',  ( 1.000000000000000078E-15, -1.000000000000000083E-30, -1.000000000000000000 ) ) ;
#10578=LINE ( 'NONE', #24657, #18049 ) ;
#10579=DIRECTION ( 'NONE',  ( 1.000000000000000000, 4.237773401492740281E-14, 0.000000000000000000 ) ) ;
#10580=CARTESIAN_POINT ( 'NONE',  ( 112.2009934676607656, -45.31764602677214526, 98.00527226877483145 ) ) ;
#10581=CARTESIAN_POINT ( 'NONE',  ( 108.6395843534182291, -26.47938140272615470, 144.9432443235309904 ) ) ;
#10582=ORIENTED_EDGE ( 'NONE', *, *, #63743, .F. ) ;
#10583=VERTEX_POINT ( 'NONE', #50585 ) ;
#10584=CARTESIAN_POINT ( 'NONE',  ( 113.4424924140864590, -42.92691738999312889, 94.64444044875396855 ) ) ;
#10586=CARTESIAN_POINT ( 'NONE',  ( 32.15435173583699680, -31.62489322948790971, -5.074374724088000832 ) ) ;
#10587=CARTESIAN_POINT ( 'NONE',  ( 116.2779988688839552, -41.49250982992358416, 239.4346728949579699 ) ) ;
#10589=VECTOR ( 'NONE', #12468, 1000.000000000000000 ) ;
#10590=DIRECTION ( 'NONE',  ( -0.9068632946707805287, 0.4214249218767882610, -9.061988307341536250E-16 ) ) ;
#10595=CARTESIAN_POINT ( 'NONE',  ( 162.7131505118539962, -33.70561438052111214, -5.074374724088000832 ) ) ;
#10597=CARTESIAN_POINT ( 'NONE',  ( 98.18688568738947708, -31.30898482519904036, 170.8899109901960003 ) ) ;
#10598=ORIENTED_EDGE ( 'NONE', *, *, #6745, .F. ) ;
#10601=CARTESIAN_POINT ( 'NONE',  ( 112.1393456672597466, -28.01282279697495525, 150.6564586068802498 ) ) ;
#10602=DIRECTION ( 'NONE',  ( 0.000000000000000000, 0.000000000000000000, 1.000000000000000000 ) ) ;
#10605=CARTESIAN_POINT ( 'NONE',  ( 99.28842769779902255, -29.78762595464951346, 190.7470538473399415 ) ) ;
#10606=CARTESIAN_POINT ( 'NONE',  ( 179.1667039024460166, -26.71338133339251542, 193.9678068554150059 ) ) ;
#10608=EDGE_CURVE ( 'NONE', #87053, #12518, #59075, .T. ) ;
#10615=B_SPLINE_CURVE_WITH_KNOTS ( 'NONE', 3,
 ( #83811, #42440, #87822, #72414, #59202, #71969, #80569, #11519, #44681, #65585, #51489, #60086, #31057, #9733, #86050, #3808, #10178, #4704, #18322, #17876, #87377, #25585, #38319, #51926, #79685, #66464, #37886, #38761, #78793, #66923, #86492, #3368, #16550, #31950, #31494, #24257, #58751, #45121, #46003 ),
 .UNSPECIFIED., .F., .F.,
 ( 4, 2, 2, 2, 2, 2, 2, 2, 2, 2, 2, 2, 2, 2, 2, 1, 1, 1, 1, 1, 2, 4 ),
 ( 0.000000000000000000, 0.06249293107409987363, 0.1249858621481997473, 0.1874787932222996278, 0.2187252587593494224, 0.2499717242963992725, 0.2812181898334490948, 0.3124646553704988894, 0.3437111209075487395, 0.3749575864445985895, 0.4062040519816483841, 0.4374505175186981787, 0.4686969830557480843, 0.4843202158242727595, 0.4921318322085349584, 0.4960376404006660578, 0.4979905444967314687, 0.4989669965447642852, 0.4994552225687807767, 0.4996993355807888837, 0.4998213920867929372, 0.4999434485927969907 ),
 .UNSPECIFIED. ) ;
#10616=CARTESIAN_POINT ( 'NONE',  ( 133.3217830637655936, -34.08035908359602217, 8.141856907856576342 ) ) ;
#10617=CARTESIAN_POINT ( 'NONE',  ( 105.5764564592757466, -44.77785207962899250, 10.24809036959195652 ) ) ;
#10618=DIRECTION ( 'NONE',  ( 0.000000000000000000, 0.000000000000000000, 1.000000000000000000 ) ) ;
#10619=ORIENTED_EDGE ( 'NONE', *, *, #88693, .F. ) ;
#10622=CARTESIAN_POINT ( 'NONE',  ( 81.57739926165950806, -16.43204134599606903, 7.859568798195391004 ) ) ;
#10625=AXIS2_PLACEMENT_3D ( 'NONE', #69771, #76126, #42045 ) ;
#10628=ORIENTED_EDGE ( 'NONE', *, *, #87102, .F. ) ;
#10629=CARTESIAN_POINT ( 'NONE',  ( 97.07201853420036741, -35.37896439201897891, 157.2187929798531627 ) ) ;
#10632=CARTESIAN_POINT ( 'NONE',  ( 110.5540359372802328, -28.93245362646326768, 24.16384839950497110 ) ) ;
#10633=CARTESIAN_POINT ( 'NONE',  ( 110.0583800183467957, -26.06436417334086642, 219.8708633711489711 ) ) ;
#10634=CARTESIAN_POINT ( 'NONE',  ( 114.0662423116486082, -44.47333502991310183, 133.1613395616249989 ) ) ;
#10636=CARTESIAN_POINT ( 'NONE',  ( 80.06648329127399677, -8.350947159940998787, 308.6356252759119911 ) ) ;
#10637=CARTESIAN_POINT ( 'NONE',  ( 100.2472489666992743, -45.42841400796814355, 273.0594347997205773 ) ) ;
#10638=PLANE ( 'NONE',  #36927 ) ;
#10639=CARTESIAN_POINT ( 'NONE',  ( 41.56648329127398966, -18.82844715994071194, 75.92562527591206845 ) ) ;
#10641=ORIENTED_EDGE ( 'NONE', *, *, #51621, .F. ) ;
#10642=CARTESIAN_POINT ( 'NONE',  ( 117.2706010548463667, -41.09852764615815346, 213.5165776568629781 ) ) ;
#10643=ORIENTED_EDGE ( 'NONE', *, *, #68710, .T. ) ;
#10644=CARTESIAN_POINT ( 'NONE',  ( 108.6487477603288170, -25.79654920012707109, 149.9737205140059473 ) ) ;
#10646=VECTOR ( 'NONE', #59927, 1000.000000000000000 ) ;
#10647=FACE_OUTER_BOUND ( 'NONE', #70912, .T. ) ;
#10649=DIRECTION ( 'NONE',  ( 0.1858654558203195195, -0.9825752044157765042, 0.000000000000000000 ) ) ;
#10650=DIRECTION ( 'NONE',  ( 0.000000000000000000, -1.000000000000000000, 0.000000000000000000 ) ) ;
#10651=CARTESIAN_POINT ( 'NONE',  ( 101.9462946551393543, -46.59843102978671681, 13.19562527591094891 ) ) ;
#10652=FACE_OUTER_BOUND ( 'NONE', #84153, .T. ) ;
#10653=LINE ( 'NONE', #51532, #64148 ) ;
#10655=CIRCLE ( 'NONE', #36744, 4.874999999999990230 ) ;
#10656=CARTESIAN_POINT ( 'NONE',  ( 75.31670390244798341, -67.87844715994100397, 37.63480685541480852 ) ) ;
#10657=DIRECTION ( 'NONE',  ( -0.7071067811745735954, -0.7071067811985214391, 0.000000000000000000 ) ) ;
#10659=CARTESIAN_POINT ( 'NONE',  ( 98.61155387813832363, -36.65781496683363372, 195.5838068554172082 ) ) ;
#10662=CARTESIAN_POINT ( 'NONE',  ( 116.3700403630726612, -44.11035778917459993, 198.2927681330539542 ) ) ;
#10663=CARTESIAN_POINT ( 'NONE',  ( 100.2987399830848432, -46.45735886148204941, 83.09276813305294240 ) ) ;
#10664=CARTESIAN_POINT ( 'NONE',  ( 96.07947519314286922, -35.15364532898842498, 222.2251490854349640 ) ) ;
#10665=DIRECTION ( 'NONE',  ( -0.7071067811862239427, -0.7071067811868709807, 0.000000000000000000 ) ) ;
#10668=CARTESIAN_POINT ( 'NONE',  ( 116.4530457758195752, -40.23956994039711077, 39.54146743497934580 ) ) ;
#10669=EDGE_CURVE ( 'NONE', #16246, #61667, #35161, .T. ) ;
#10671=DIRECTION ( 'NONE',  ( 0.7071067811865459074, 0.7071067811865491270, 7.071067811865459556E-16 ) ) ;
#10673=CARTESIAN_POINT ( 'NONE',  ( 115.8272920594983049, -31.73323121823576898, 64.24007680160269729 ) ) ;
#10674=EDGE_CURVE ( 'NONE', #5130, #16097, #69220, .T. ) ;
#10675=ORIENTED_EDGE ( 'NONE', *, *, #32577, .F. ) ;
#10676=ORIENTED_EDGE ( 'NONE', *, *, #50721, .F. ) ;
#10677=CARTESIAN_POINT ( 'NONE',  ( 99.00375160886646597, -32.60573182744733600, 95.38480078045697041 ) ) ;
#10678=DIRECTION ( 'NONE',  ( -0.000000000000000000, -0.000000000000000000, 1.000000000000000000 ) ) ;
#10679=EDGE_LOOP ( 'NONE', ( #43599, #72030, #76312, #61680 ) ) ;
#10680=CARTESIAN_POINT ( 'NONE',  ( 110.1514708964275684, -46.66481413883387575, 93.81562527591097478 ) ) ;
#10681=DIRECTION ( 'NONE',  ( 0.000000000000000000, 0.000000000000000000, -1.000000000000000000 ) ) ;
#10682=CARTESIAN_POINT ( 'NONE',  ( 160.7738106836348209, -48.62134037874901082, 300.4678068554149490 ) ) ;
#10683=CARTESIAN_POINT ( 'NONE',  ( 51.27381068362099370, -23.19206098993950604, -5.074374724088000832 ) ) ;
#10684=CARTESIAN_POINT ( 'NONE',  ( 97.95204982468527533, -33.09064556074055474, 41.02419670448293232 ) ) ;
#10685=EDGE_LOOP ( 'NONE', ( #12209, #62229, #80700, #16228 ) ) ;
#10688=VECTOR ( 'NONE', #11101, 1000.000000000000000 ) ;
#10690=DIRECTION ( 'NONE',  ( 1.000000000000000078E-15, -1.000000000000000083E-30, -1.000000000000000000 ) ) ;
#10691=DIRECTION ( 'NONE',  ( 0.7071067811864676367, 0.7071067811866273978, 7.071067811864669709E-16 ) ) ;
#10692=CARTESIAN_POINT ( 'NONE',  ( 108.4174892559276913, -26.73503592823092845, 115.9689586089433391 ) ) ;
#10695=CARTESIAN_POINT ( 'NONE',  ( 32.56670390244700997, -22.48495420874110806, 342.9256252759119548 ) ) ;
#10696=CARTESIAN_POINT ( 'NONE',  ( 97.33789353722791304, -34.07085096390528633, 52.11557580465839123 ) ) ;
#10697=CARTESIAN_POINT ( 'NONE',  ( 107.0664832912739683, -24.97944715994095333, 307.1356252759109680 ) ) ;
#10700=CARTESIAN_POINT ( 'NONE',  ( 109.6376038899290677, -46.81002275840761939, 47.77562527591094721 ) ) ;
#10701=ORIENTED_EDGE ( 'NONE', *, *, #2789, .F. ) ;
#10703=ADVANCED_FACE ( 'NONE', ( #71506 ), #69706, .T. ) ;
#10705=CYLINDRICAL_SURFACE ( 'NONE', #86719, 5.500000000000000888 ) ;
#10707=CARTESIAN_POINT ( 'NONE',  ( 98.41263308787671349, -36.61538842024999241, 154.1461856076869594 ) ) ;
#10708=VECTOR ( 'NONE', #21796, 1000.000000000000000 ) ;
#10709=AXIS2_PLACEMENT_3D ( 'NONE', #6668, #34362, #89808 ) ;
#10711=AXIS2_PLACEMENT_3D ( 'NONE', #17144, #38458, #32093 ) ;
#10714=ORIENTED_EDGE ( 'NONE', *, *, #48793, .F. ) ;
#10715=FACE_OUTER_BOUND ( 'NONE', #84284, .T. ) ;
#10716=CIRCLE ( 'NONE', #25179, 0.4999999999999976685 ) ;
#10717=ORIENTED_EDGE ( 'NONE', *, *, #67518, .T. ) ;
#10718=ORIENTED_EDGE ( 'NONE', *, *, #75928, .F. ) ;
#10719=DIRECTION ( 'NONE',  ( -0.9254794337955620787, -0.3787978585227822492, 0.000000000000000000 ) ) ;
#10720=EDGE_CURVE ( 'NONE', #66156, #87997, #42418, .T. ) ;
#10721=CARTESIAN_POINT ( 'NONE',  ( 108.4337774161041921, -27.97394686652187090, 186.3844404487539634 ) ) ;
#10726=ORIENTED_EDGE ( 'NONE', *, *, #67301, .F. ) ;
#10728=ADVANCED_FACE ( 'NONE', ( #70146 ), #84245, .T. ) ;
#10729=CARTESIAN_POINT ( 'NONE',  ( 113.1326720373799617, -31.22635327163875374, 207.2309475124489495 ) ) ;
#10730=CARTESIAN_POINT ( 'NONE',  ( 101.6667450491003706, -27.05792876557581650, 105.4937205140069665 ) ) ;
#10731=CARTESIAN_POINT ( 'NONE',  ( 114.0759046727996093, -46.25395340493279406, 33.08133956162495792 ) ) ;
#10734=CARTESIAN_POINT ( 'NONE',  ( 73.06670390244801183, -50.82844715994100682, 310.9178068554150514 ) ) ;
#10735=CARTESIAN_POINT ( 'NONE',  ( 108.8488479242245290, -47.00104215551821341, 163.7127681330539701 ) ) ;
#10736=CYLINDRICAL_SURFACE ( 'NONE', #84268, 9.999999999999998224 ) ;
#10737=EDGE_CURVE ( 'NONE', #34489, #60854, #36534, .T. ) ;
#10740=ORIENTED_EDGE ( 'NONE', *, *, #67463, .T. ) ;
#10741=EDGE_CURVE ( 'NONE', #30195, #49111, #16529, .T. ) ;
#10742=ORIENTED_EDGE ( 'NONE', *, *, #36602, .F. ) ;
#10743=DIRECTION ( 'NONE',  ( 1.000000000000000000, 4.299999999999999979E-14, 1.000000000000000078E-15 ) ) ;
#10744=ORIENTED_EDGE ( 'NONE', *, *, #52344, .F. ) ;
#10747=ORIENTED_EDGE ( 'NONE', *, *, #2946, .T. ) ;
#10748=CARTESIAN_POINT ( 'NONE',  ( 115.5446080981639057, -31.35709777695358369, 130.2761217128978899 ) ) ;
#10749=CARTESIAN_POINT ( 'NONE',  ( 110.7945467183388502, -46.46538951521414873, 62.86705384733992474 ) ) ;
#10750=FACE_OUTER_BOUND ( 'NONE', #72031, .T. ) ;
#10752=DIRECTION ( 'NONE',  ( -0.08544974978095701279, -0.9963424814100680926, 0.000000000000000000 ) ) ;
#10753=DIRECTION ( 'NONE',  ( 1.000000000000000078E-15, -1.000000000000000083E-30, -1.000000000000000000 ) ) ;
#10754=CARTESIAN_POINT ( 'NONE',  ( 108.8666348730871221, -46.34312957481634498, 82.72419670448294937 ) ) ;
#10756=CARTESIAN_POINT ( 'NONE',  ( 106.9751875180390641, -47.13234726572959232, 183.5699109901969734 ) ) ;
#10757=DIRECTION ( 'NONE',  ( 0.000000000000000000, 1.000000000000000000, 0.000000000000000000 ) ) ;
#10758=DIRECTION ( 'NONE',  ( 1.042073847087816516E-15, 1.000000000000000000, 0.000000000000000000 ) ) ;
#10761=DIRECTION ( 'NONE',  ( 0.000000000000000000, 2.135044278125299371E-15, -1.000000000000000000 ) ) ;
#10763=FACE_OUTER_BOUND ( 'NONE', #52290, .T. ) ;
#10764=CARTESIAN_POINT ( 'NONE',  ( 117.2351557800294870, -41.18040025386632408, 208.4861014663869696 ) ) ;
#10765=EDGE_LOOP ( 'NONE', ( #51611, #37216, #50236, #79252 ) ) ;
#10766=CARTESIAN_POINT ( 'NONE',  ( 115.0888828095797010, -30.61760375934272105, 144.3439616953089342 ) ) ;
#10767=CARTESIAN_POINT ( 'NONE',  ( 113.8133276556114595, -26.95691720032833416, 235.5956252759109759 ) ) ;
#10768=CARTESIAN_POINT ( 'NONE',  ( 107.3350663223963153, -26.26422652666180468, 116.0556252759109555 ) ) ;
#10770=CARTESIAN_POINT ( 'NONE',  ( 82.50377070433003723, -38.00325133681918288, 7.150416387932702733 ) ) ;
#10774=VECTOR ( 'NONE', #27813, 1000.000000000000000 ) ;
#10776=AXIS2_PLACEMENT_3D ( 'NONE', #69, #27769, #83645 ) ;
#10780=ORIENTED_EDGE ( 'NONE', *, *, #27281, .F. ) ;
#10782=VECTOR ( 'NONE', #51887, 1000.000000000000000 ) ;
#10783=ORIENTED_EDGE ( 'NONE', *, *, #41535, .F. ) ;
#10784=CARTESIAN_POINT ( 'NONE',  ( 115.7831076666659413, -41.80230951636190895, 73.40645860869774708 ) ) ;
#10785=CARTESIAN_POINT ( 'NONE',  ( 113.7560087186648730, -29.08427257552855494, 285.5032443235299979 ) ) ;
#10786=B_SPLINE_CURVE_WITH_KNOTS ( 'NONE', 3,
 ( #53614, #52264, #81379, #40007, #67723, #32290, #66365, #5510, #38665, #33204, #73637, #10522, #18227, #51832, #79584, #38226, #59098, #80030, #73182, #65920, #3706, #31399, #24602, #10960, #4154, #31852, #25044, #45908, #49048, #61341 ),
 .UNSPECIFIED., .F., .F.,
 ( 4, 2, 2, 2, 1, 2, 2, 2, 2, 2, 2, 2, 1, 2, 2, 4 ),
 ( 0.5000000000000000000, 0.5625000000000072164, 0.5937500000000088818, 0.6093750000000097700, 0.6171875000000102141, 0.6210937500000091038, 0.6250000000000078826, 0.6875000000000095479, 0.7187500000000133227, 0.7500000000000170974, 0.8125000000000208722, 0.8437500000000262013, 0.8593750000000288658, 0.8671875000000301981, 0.8750000000000315303, 1.000000000000000000 ),
 .UNSPECIFIED. ) ;
#10789=DIRECTION ( 'NONE',  ( 0.000000000000000000, 0.000000000000000000, -1.000000000000000000 ) ) ;
#10791=CARTESIAN_POINT ( 'NONE',  ( 104.4064053327731472, -46.06725273453308489, 216.7781341137909692 ) ) ;
#10792=ORIENTED_EDGE ( 'NONE', *, *, #33079, .T. ) ;
#10793=ORIENTED_EDGE ( 'NONE', *, *, #3455, .F. ) ;
#10794=EDGE_LOOP ( 'NONE', ( #43035, #72771, #64959, #11516 ) ) ;
#10795=EDGE_CURVE ( 'NONE', #44803, #20780, #71945, .T. ) ;
#10796=CARTESIAN_POINT ( 'NONE',  ( 20.03715912545736089, -24.42818131006190541, 237.4678068554150059 ) ) ;
#10797=FACE_BOUND ( 'NONE', #84551, .T. ) ;
#10798=DIRECTION ( 'NONE',  ( 0.000000000000000000, -1.000000000000000000, 0.000000000000000000 ) ) ;
#10800=CARTESIAN_POINT ( 'NONE',  ( 100.8575770528253628, -43.09432028306430595, 18.39301187732595011 ) ) ;
#10802=EDGE_CURVE ( 'NONE', #67480, #12481, #45985, .T. ) ;
#10803=DIRECTION ( 'NONE',  ( 1.000000000000000078E-15, 1.000000000000000083E-30, -1.000000000000000000 ) ) ;
#10804=DIRECTION ( 'NONE',  ( 4.299999999999999979E-14, -1.000000000000000000, 4.400000000000000367E-29 ) ) ;
#10805=ADVANCED_FACE ( 'NONE', ( #11495 ), #39191, .F. ) ;
#10808=CARTESIAN_POINT ( 'NONE',  ( 179.8608231853560255, -35.55794170701751256, -5.074374724088000832 ) ) ;
#10811=CARTESIAN_POINT ( 'NONE',  ( 115.2261106523039444, -36.95351711827176899, 41.62237608387797394 ) ) ;
#10812=ADVANCED_FACE ( 'NONE', ( #26020 ), #39631, .T. ) ;
#10814=ADVANCED_FACE ( 'NONE', ( #12386 ), #20104, .T. ) ;
#10816=CIRCLE ( 'NONE', #67422, 2.117000000000000881 ) ;
#10818=FACE_OUTER_BOUND ( 'NONE', #85392, .T. ) ;
#10820=VERTEX_POINT ( 'NONE', #47780 ) ;
#10821=DIRECTION ( 'NONE',  ( 1.000000000000000000, 0.000000000000000000, 0.000000000000000000 ) ) ;
#10822=CARTESIAN_POINT ( 'NONE',  ( 19.56670390244643443, -25.42844715994203852, 180.4678068554150911 ) ) ;
#10824=ORIENTED_EDGE ( 'NONE', *, *, #40474, .T. ) ;
#10825=CARTESIAN_POINT ( 'NONE',  ( 107.3339538991774447, -26.30757161206916095, 120.0556252759109555 ) ) ;
#10826=ORIENTED_EDGE ( 'NONE', *, *, #2277, .F. ) ;
#10827=CARTESIAN_POINT ( 'NONE',  ( 111.2570682682515439, -29.25341213619239156, 34.09241982807698434 ) ) ;
#10829=LINE ( 'NONE', #22698, #73600 ) ;
#10830=CARTESIAN_POINT ( 'NONE',  ( 112.5403241924349942, -29.76056314593741803, 75.97872616303996551 ) ) ;
#10834=CARTESIAN_POINT ( 'NONE',  ( 115.9100415161514945, -31.16808610560197224, 30.27276813305396175 ) ) ;
#10837=CARTESIAN_POINT ( 'NONE',  ( 194.0667039024482108, -40.32844715993407192, 180.4678068554150343 ) ) ;
#10840=CARTESIAN_POINT ( 'NONE',  ( 77.31648329127399677, -18.72944715994106346, 3.101481641215480867 ) ) ;
#10841=AXIS2_PLACEMENT_3D ( 'NONE', #48641, #42722, #6880 ) ;
#10842=VECTOR ( 'NONE', #59597, 1000.000000000000000 ) ;
#10843=AXIS2_PLACEMENT_3D ( 'NONE', #66961, #30659, #59242 ) ;
#10844=ORIENTED_EDGE ( 'NONE', *, *, #85425, .F. ) ;
#10851=CARTESIAN_POINT ( 'NONE',  ( 100.2051353121704835, -29.75912871662441361, 225.6956252759109702 ) ) ;
#10852=EDGE_CURVE ( 'NONE', #27163, #4309, #40533, .T. ) ;
#10853=CARTESIAN_POINT ( 'NONE',  ( 116.0120085738102631, -32.18627031846445874, 124.2002723411735872 ) ) ;
#10855=CARTESIAN_POINT ( 'NONE',  ( 115.5737247207382552, -42.75516958203532880, 49.33562527591095659 ) ) ;
#10856=DIRECTION ( 'NONE',  ( 0.000000000000000000, 0.000000000000000000, 1.000000000000000000 ) ) ;
#10857=ADVANCED_FACE ( 'NONE', ( #47332 ), #75515, .F. ) ;
#10858=ORIENTED_EDGE ( 'NONE', *, *, #59471, .T. ) ;
#10859=CARTESIAN_POINT ( 'NONE',  ( 103.7225970069647474, -27.30339880462703661, 171.3477492379661555 ) ) ;
#10863=CARTESIAN_POINT ( 'NONE',  ( 61.56670390244634916, -23.42844715994043270, 180.4678068554151196 ) ) ;
#10864=DIRECTION ( 'NONE',  ( 0.000000000000000000, 0.000000000000000000, 1.000000000000000000 ) ) ;
#10865=CARTESIAN_POINT ( 'NONE',  ( 113.7851844261090264, -26.99768152489561501, 239.5956252759109759 ) ) ;
#10866=DIRECTION ( 'NONE',  ( 1.000000000000000078E-15, 1.000000000000000083E-30, -1.000000000000000000 ) ) ;
#10867=AXIS2_PLACEMENT_3D ( 'NONE', #78825, #31536, #37917 ) ;
#10869=CARTESIAN_POINT ( 'NONE',  ( 77.54412859703529648, -37.82508440162273189, 2.797770139040228976 ) ) ;
#10870=CARTESIAN_POINT ( 'NONE',  ( 101.4793796374089965, -43.85664460571122447, 276.4819436376007502 ) ) ;
#10871=LINE ( 'NONE', #73993, #34509 ) ;
#10872=CARTESIAN_POINT ( 'NONE',  ( 103.2867953297129873, -47.09177226061134292, 93.28610146638693834 ) ) ;
#10874=CARTESIAN_POINT ( 'NONE',  ( 106.0722674988897296, -48.58863484196640314, 112.5099109901969712 ) ) ;
#10875=ORIENTED_EDGE ( 'NONE', *, *, #26341, .T. ) ;
#10876=LINE ( 'NONE', #72225, #71287 ) ;
#10877=ORIENTED_EDGE ( 'NONE', *, *, #33199, .T. ) ;
#10880=DIRECTION ( 'NONE',  ( 1.000000000000000078E-15, 1.000000000000000083E-30, -1.000000000000000000 ) ) ;
#10882=DIRECTION ( 'NONE',  ( 0.000000000000000000, 0.000000000000000000, -1.000000000000000000 ) ) ;
#10883=CARTESIAN_POINT ( 'NONE',  ( 117.9212005353621322, -39.05065313503074975, 108.6708633711489824 ) ) ;
#10884=ORIENTED_EDGE ( 'NONE', *, *, #42633, .F. ) ;
#10885=CARTESIAN_POINT ( 'NONE',  ( 183.6524903400785433, -48.32844715993451956, 180.4678068554150343 ) ) ;
#10886=FACE_OUTER_BOUND ( 'NONE', #4161, .T. ) ;
#10888=DIRECTION ( 'NONE',  ( 1.000000000000000078E-15, -1.000000000000000083E-30, -1.000000000000000000 ) ) ;
#10889=ORIENTED_EDGE ( 'NONE', *, *, #32592, .T. ) ;
#10890=CARTESIAN_POINT ( 'NONE',  ( 96.00011186464382718, -37.20993085831212710, 116.3489586092439652 ) ) ;
#10891=SURFACE_STYLE_FILL_AREA ( #79060 ) ;
#10892=DIRECTION ( 'NONE',  ( -0.8660253910675250744, -0.0001484127182050486030, -0.5000000000000052180 ) ) ;
#10893=CARTESIAN_POINT ( 'NONE',  ( 177.8371591254543489, -47.82818131005477369, 249.9678068554149775 ) ) ;
#10894=ORIENTED_EDGE ( 'NONE', *, *, #29850, .F. ) ;
#10898=LINE ( 'NONE', #38603, #74808 ) ;
#10899=CYLINDRICAL_SURFACE ( 'NONE', #10250, 12.99999999999999822 ) ;
#10901=DIRECTION ( 'NONE',  ( 0.000000000000000000, 0.000000000000000000, -1.000000000000000000 ) ) ;
#10902=ORIENTED_EDGE ( 'NONE', *, *, #64830, .T. ) ;
#10903=AXIS2_PLACEMENT_3D ( 'NONE', #22212, #49887, #8123 ) ;
#10904=CIRCLE ( 'NONE', #57260, 7.799999999999994493 ) ;
#10905=AXIS2_PLACEMENT_3D ( 'NONE', #63698, #84607, #21470 ) ;
#10906=EDGE_CURVE ( 'NONE', #82312, #51989, #61860, .T. ) ;
#10907=CARTESIAN_POINT ( 'NONE',  ( 41.56670390244777735, -36.32844715994104234, 300.4678068554150059 ) ) ;
#10909=CARTESIAN_POINT ( 'NONE',  ( 103.7602102885707467, -27.48919103108776341, 186.3499109901959798 ) ) ;
#10910=FACE_BOUND ( 'NONE', #89150, .T. ) ;
#10911=ORIENTED_EDGE ( 'NONE', *, *, #51400, .T. ) ;
#10912=AXIS2_PLACEMENT_3D ( 'NONE', #3971, #79851, #10344 ) ;
#10914=CARTESIAN_POINT ( 'NONE',  ( 99.77418633167441442, -43.29726106931974527, 52.90991099019598209 ) ) ;
#10915=CARTESIAN_POINT ( 'NONE',  ( 100.8873880383125936, -44.70015583377661983, 52.05235198494534643 ) ) ;
#10918=DIRECTION ( 'NONE',  ( 1.907762142705490052E-15, 7.167082501179359715E-16, -1.000000000000000000 ) ) ;
#10921=FACE_OUTER_BOUND ( 'NONE', #82280, .T. ) ;
#10923=ORIENTED_EDGE ( 'NONE', *, *, #58584, .T. ) ;
#10924=CARTESIAN_POINT ( 'NONE',  ( 111.4343887032284783, -44.43980907907789657, 209.4187261630399632 ) ) ;
#10926=CARTESIAN_POINT ( 'NONE',  ( 116.7961848845175865, -39.38406792386692246, 54.61469027183413516 ) ) ;
#10928=CARTESIAN_POINT ( 'NONE',  ( 31.71315051185471390, -33.70561438052040160, 237.4678068554150059 ) ) ;
#10929=DIRECTION ( 'NONE',  ( 0.9963424814100679816, -0.08544974978095716545, 0.000000000000000000 ) ) ;
#10930=VERTEX_POINT ( 'NONE', #74167 ) ;
#10931=CARTESIAN_POINT ( 'NONE',  ( 114.0075790447422577, -33.88846322101949227, 9.125625275910969947 ) ) ;
#10932=CARTESIAN_POINT ( 'NONE',  ( 105.7925177523798368, -26.72498828120203740, 36.17735711206680094 ) ) ;
#10934=CARTESIAN_POINT ( 'NONE',  ( 117.5124197103495050, -37.28486668576427121, 18.78419670448294809 ) ) ;
#10938=CARTESIAN_POINT ( 'NONE',  ( 101.9936209311938740, -45.44607153314367309, 82.15645860836184511 ) ) ;
#10939=DIRECTION ( 'NONE',  ( -4.237773401492740281E-14, 1.000000000000000000, 0.000000000000000000 ) ) ;
#10940=PLANE ( 'NONE',  #59168 ) ;
#10941=DIRECTION ( 'NONE',  ( 1.000000000000000000, 4.163336342344333240E-14, 0.000000000000000000 ) ) ;
#10942=EDGE_CURVE ( 'NONE', #28049, #52806, #35961, .T. ) ;
#10943=CARTESIAN_POINT ( 'NONE',  ( 97.36167283409557172, -40.65495779399346077, 202.6327681330539860 ) ) ;
#10946=CARTESIAN_POINT ( 'NONE',  ( 101.1162363742629253, -27.35970543535582422, 61.51467289495899138 ) ) ;
#10947=CARTESIAN_POINT ( 'NONE',  ( 75.26949937496598864, -71.54137415153812185, 361.9756252759101471 ) ) ;
#10948=VECTOR ( 'NONE', #26981, 1000.000000000000000 ) ;
#10949=ORIENTED_EDGE ( 'NONE', *, *, #37347, .T. ) ;
#10950=ORIENTED_EDGE ( 'NONE', *, *, #36413, .T. ) ;
#10951=VERTEX_POINT ( 'NONE', #15533 ) ;
#10952=CARTESIAN_POINT ( 'NONE',  ( 82.27770840671846031, -17.08426318373788177, 2.472582314378777291 ) ) ;
#10953=DIRECTION ( 'NONE',  ( -0.7071067811865171526, -0.7071067811865779928, -7.071067811865164719E-16 ) ) ;
#10954=LINE ( 'NONE', #88624, #53774 ) ;
#10955=CARTESIAN_POINT ( 'NONE',  ( 103.6457284375485131, -44.67924975648479347, 135.0833284648299752 ) ) ;
#10956=CARTESIAN_POINT ( 'NONE',  ( 100.7369725318012570, -45.81913908486538389, 233.0803871806729717 ) ) ;
#10957=CARTESIAN_POINT ( 'NONE',  ( 134.0664832912739826, -15.97944715994100306, 1.625625275910997480 ) ) ;
#10958=ORIENTED_EDGE ( 'NONE', *, *, #84275, .T. ) ;
#10959=ADVANCED_FACE ( 'NONE', ( #70041 ), #42307, .F. ) ;
#10960=CARTESIAN_POINT ( 'NONE',  ( 135.3099588812963816, -39.18301917769485954, 1.868341932363548619 ) ) ;
#10961=ORIENTED_EDGE ( 'NONE', *, *, #79037, .F. ) ;
#10962=VERTEX_POINT ( 'NONE', #28702 ) ;
#10963=AXIS2_PLACEMENT_3D ( 'NONE', #7900, #15627, #2441 ) ;
#10964=PLANE ( 'NONE',  #48771 ) ;
#10968=DIRECTION ( 'NONE',  ( 0.0001713722455994998422, -0.9999999853157766072, 0.000000000000000000 ) ) ;
#10969=CARTESIAN_POINT ( 'NONE',  ( 80.06648329127402519, -46.72944715994105991, 8.225625275910942946 ) ) ;
#10970=AXIS2_PLACEMENT_3D ( 'NONE', #54499, #21823, #41331 ) ;
#10971=CARTESIAN_POINT ( 'NONE',  ( 104.4882254922823819, -26.97928299422803278, 25.28160027219495021 ) ) ;
#10972=CARTESIAN_POINT ( 'NONE',  ( 115.2241057928380599, -39.35723584706951783, 158.0009912566479500 ) ) ;
#10973=CARTESIAN_POINT ( 'NONE',  ( 100.5231322539815153, -27.76298515809465073, 30.56610146638794134 ) ) ;
#10976=VERTEX_POINT ( 'NONE', #35053 ) ;
#10977=AXIS2_PLACEMENT_3D ( 'NONE', #69240, #67434, #53331 ) ;
#10979=DIRECTION ( 'NONE',  ( 0.000000000000000000, 0.000000000000000000, -1.000000000000000000 ) ) ;
#10980=ORIENTED_EDGE ( 'NONE', *, *, #73804, .T. ) ;
#10981=CARTESIAN_POINT ( 'NONE',  ( 97.29212427557061460, -38.88438501596571939, 167.4992703951793089 ) ) ;
#10982=CARTESIAN_POINT ( 'NONE',  ( 188.5667039024479834, -67.87844715994100397, 132.3428068554150343 ) ) ;
#10983=CARTESIAN_POINT ( 'NONE',  ( 97.81362146037459127, -40.52214467932135022, 131.6360307733190211 ) ) ;
#10985=EDGE_CURVE ( 'NONE', #24816, #41305, #63510, .T. ) ;
#10987=ORIENTED_EDGE ( 'NONE', *, *, #22142, .T. ) ;
#10988=CARTESIAN_POINT ( 'NONE',  ( 95.23402374720009789, -35.71607800568281021, 36.25848241876794731 ) ) ;
#10989=CARTESIAN_POINT ( 'NONE',  ( 118.2550939253582811, -40.78236016348033388, 19.54991099019698453 ) ) ;
#10993=DIRECTION ( 'NONE',  ( 1.000000000000000078E-15, 1.000000000000000083E-30, -1.000000000000000000 ) ) ;
#10994=LINE ( 'NONE', #30557, #45249 ) ;
#10995=DIRECTION ( 'NONE',  ( 0.7071067811566161820, 0.7071067812164789634, 0.000000000000000000 ) ) ;
#10996=CARTESIAN_POINT ( 'NONE',  ( 132.9421938897440896, -39.23922437001930774, 8.028287874532662016 ) ) ;
#10997=CARTESIAN_POINT ( 'NONE',  ( 25.56670390244797275, -58.35344715994099829, 259.9678068554150059 ) ) ;
#10999=CARTESIAN_POINT ( 'NONE',  ( 100.4512773062034370, -27.81586575833916442, 35.59657765686397113 ) ) ;
#11000=CARTESIAN_POINT ( 'NONE',  ( 116.3502490628398647, -44.09465650233049416, 194.2927681330539542 ) ) ;
#11001=CARTESIAN_POINT ( 'NONE',  ( 115.6911227382933873, -43.67932486773085543, 39.27467289495895386 ) ) ;
#11004=CARTESIAN_POINT ( 'NONE',  ( 81.70522810117023482, -34.51875982968658718, 2.060081176875012243 ) ) ;
#11007=EDGE_CURVE ( 'NONE', #22788, #75220, #48961, .T. ) ;
#11008=CARTESIAN_POINT ( 'NONE',  ( 138.0667039024480403, -58.72944715994091069, 239.5838068554170377 ) ) ;
#11009=EDGE_LOOP ( 'NONE', ( #52588, #8554, #45030, #4244, #36247, #45912, #83324, #73113, #13509, #5033, #77672, #72489, #16612, #35301 ) ) ;
#11010=EDGE_CURVE ( 'NONE', #80032, #68275, #22344, .T. ) ;
#11011=CARTESIAN_POINT ( 'NONE',  ( 113.5587197313313936, -28.64306037466259625, 115.5261014663869474 ) ) ;
#11015=EDGE_CURVE ( 'NONE', #50715, #19682, #62005, .T. ) ;
#11016=CARTESIAN_POINT ( 'NONE',  ( 115.2346088729119629, -30.22974330756305505, 240.3613395616249875 ) ) ;
#11017=DIRECTION ( 'NONE',  ( 1.000000000000000078E-15, -1.000000000000000083E-30, -1.000000000000000000 ) ) ;
#11018=DIRECTION ( 'NONE',  ( 1.000000000000000000, 0.000000000000000000, 0.000000000000000000 ) ) ;
#11019=DIRECTION ( 'NONE',  ( 1.000000000000000078E-15, 1.000000000000000083E-30, -1.000000000000000000 ) ) ;
#11020=CARTESIAN_POINT ( 'NONE',  ( 51.06648329127400388, -18.82844715994099971, 330.8831252759119934 ) ) ;
#11021=DIRECTION ( 'NONE',  ( 0.000000000000000000, 0.000000000000000000, -1.000000000000000000 ) ) ;
#11025=CARTESIAN_POINT ( 'NONE',  ( 113.1634500054122583, -44.41975088505045477, 168.1099109901969939 ) ) ;
#11027=VERTEX_POINT ( 'NONE', #50019 ) ;
#11028=AXIS2_PLACEMENT_3D ( 'NONE', #26135, #4349, #25225 ) ;
#11029=CARTESIAN_POINT ( 'NONE',  ( 115.2337707449818680, -33.21411712777100433, 75.58158330589692753 ) ) ;
#11031=VECTOR ( 'NONE', #51852, 1000.000000000000000 ) ;
#11034=CARTESIAN_POINT ( 'NONE',  ( 117.9377692877171313, -39.05906590213764673, 254.6584824187675338 ) ) ;
#11035=DIRECTION ( 'NONE',  ( -4.237773401492740281E-14, 1.000000000000000000, 0.000000000000000000 ) ) ;
#11038=FACE_OUTER_BOUND ( 'NONE', #57099, .T. ) ;
#11039=ADVANCED_FACE ( 'NONE', ( #43207 ), #63220, .F. ) ;
#11044=CARTESIAN_POINT ( 'NONE',  ( 96.03721982003239077, -36.58408020053186505, 156.3280062282919687 ) ) ;
#11045=ORIENTED_EDGE ( 'NONE', *, *, #87356, .F. ) ;
#11046=ORIENTED_EDGE ( 'NONE', *, *, #42431, .T. ) ;
#11047=LINE ( 'NONE', #31935, #54636 ) ;
#11048=CARTESIAN_POINT ( 'NONE',  ( 105.7995185470425952, -26.72403495915586547, 151.1772919378495317 ) ) ;
#11052=CARTESIAN_POINT ( 'NONE',  ( 160.7738106836383167, -48.62134037874550785, 300.4678068554149490 ) ) ;
#11053=CIRCLE ( 'NONE', #38612, 3.299999999999997158 ) ;
#11054=CARTESIAN_POINT ( 'NONE',  ( 98.26116833961376074, -42.31097554054522902, 186.7756252759109543 ) ) ;
#11055=CARTESIAN_POINT ( 'NONE',  ( 135.5597725514587069, -39.04085022828070350, 7.869587501215970171 ) ) ;
#11056=ORIENTED_EDGE ( 'NONE', *, *, #9284, .T. ) ;
#11061=CARTESIAN_POINT ( 'NONE',  ( 97.81285236004582373, -40.52026819599429786, 166.6358693223811542 ) ) ;
#11062=CARTESIAN_POINT ( 'NONE',  ( 111.5696292435227122, -29.33873666780462486, 47.44713798863897836 ) ) ;
#11063=DIRECTION ( 'NONE',  ( 0.000000000000000000, 0.000000000000000000, -1.000000000000000000 ) ) ;
#11064=VERTEX_POINT ( 'NONE', #1896 ) ;
#11065=EDGE_CURVE ( 'NONE', #5327, #1305, #55578, .T. ) ;
#11068=ORIENTED_EDGE ( 'NONE', *, *, #5716, .T. ) ;
#11069=ORIENTED_EDGE ( 'NONE', *, *, #1302, .T. ) ;
#11072=ORIENTED_EDGE ( 'NONE', *, *, #31459, .T. ) ;
#11074=CARTESIAN_POINT ( 'NONE',  ( 116.0925701722734686, -37.46594287791281630, 38.19622935188693447 ) ) ;
#11075=CARTESIAN_POINT ( 'NONE',  ( 107.5668325082694139, -47.79493819276859057, 192.6003871806729535 ) ) ;
#11076=CARTESIAN_POINT ( 'NONE',  ( 95.59354794629800267, -39.59649474372138656, 166.5213395616259788 ) ) ;
#11077=DIRECTION ( 'NONE',  ( 0.7071067811866279529, -0.7071067811864671926, 7.071067811866286874E-16 ) ) ;
#11078=CARTESIAN_POINT ( 'NONE',  ( 100.1775528843425178, -45.37332466565996469, 268.0289586092443415 ) ) ;
#11079=LINE ( 'NONE', #38785, #66620 ) ;
#11081=ORIENTED_EDGE ( 'NONE', *, *, #20034, .F. ) ;
#11082=ORIENTED_EDGE ( 'NONE', *, *, #71720, .F. ) ;
#11083=AXIS2_PLACEMENT_3D ( 'NONE', #39442, #80347, #54378 ) ;
#11084=AXIS2_PLACEMENT_3D ( 'NONE', #17317, #77758, #37762 ) ;
#11085=ADVANCED_FACE ( 'NONE', ( #64567 ), #79997, .T. ) ;
#11088=CARTESIAN_POINT ( 'NONE',  ( 111.1446672340677111, -27.08708843538706645, 244.7584824187679544 ) ) ;
#11089=ORIENTED_EDGE ( 'NONE', *, *, #15170, .F. ) ;
#11091=CARTESIAN_POINT ( 'NONE',  ( 99.28842769779902255, -29.78762595464951346, 190.7470538473399415 ) ) ;
#11093=FACE_BOUND ( 'NONE', #47070, .T. ) ;
#11097=CARTESIAN_POINT ( 'NONE',  ( 51.06648329127330044, -0.7548456658612000547, 333.4006252759120343 ) ) ;
#11098=CARTESIAN_POINT ( 'NONE',  ( 118.3173389373706925, -33.08695204176930105, 280.0756252759109657 ) ) ;
#11100=CARTESIAN_POINT ( 'NONE',  ( 107.0664832912739399, -36.72944715994095333, 299.5571190294419921 ) ) ;
#11101=DIRECTION ( 'NONE',  ( 1.000000000000000078E-15, -1.000000000000000083E-30, -1.000000000000000000 ) ) ;
#11104=CARTESIAN_POINT ( 'NONE',  ( 152.0371591254583450, -47.82818131005588214, 249.9678068554149490 ) ) ;
#11107=CARTESIAN_POINT ( 'NONE',  ( 182.4202572930266228, -31.94127993907054730, 237.4678068554150059 ) ) ;
#11108=CARTESIAN_POINT ( 'NONE',  ( 113.6996774752161201, -45.60053368046675359, 188.0994347997199725 ) ) ;
#11109=CARTESIAN_POINT ( 'NONE',  ( 98.45872715028987443, -30.84820395253375125, 116.8499109901969604 ) ) ;
#11110=CARTESIAN_POINT ( 'NONE',  ( 116.0926836276447460, -42.03234139191665975, 234.4041967044819899 ) ) ;
#11111=DIRECTION ( 'NONE',  ( 1.000000000000000078E-15, -1.000000000000000083E-30, -1.000000000000000000 ) ) ;
#11112=CARTESIAN_POINT ( 'NONE',  ( 188.5667039024485518, -48.82844715993430640, 175.7178068554150343 ) ) ;
#11113=VECTOR ( 'NONE', #47364, 1000.000000000000114 ) ;
#11114=DIRECTION ( 'NONE',  ( 4.299999999999999979E-14, -1.000000000000000000, 0.000000000000000000 ) ) ;
#11115=CARTESIAN_POINT ( 'NONE',  ( 97.81748826816456699, -40.53157710480042653, 37.63655137377492110 ) ) ;
#11117=DIRECTION ( 'NONE',  ( 1.000000000000000000, 0.000000000000000000, 0.000000000000000000 ) ) ;
#11119=CLOSED_SHELL ( 'NONE', ( #60929, #9449, #21616, #44974 ) ) ;
#11120=VERTEX_POINT ( 'NONE', #30049 ) ;
#11122=EDGE_CURVE ( 'NONE', #48508, #49976, #57743, .T. ) ;
#11123=CARTESIAN_POINT ( 'NONE',  ( 99.76075522406560481, -42.08098971643298825, 106.2400388756959728 ) ) ;
#11124=LINE ( 'NONE', #58823, #86486 ) ;
#11125=ORIENTED_EDGE ( 'NONE', *, *, #73258, .F. ) ;
#11126=ADVANCED_FACE ( 'NONE', ( #38193 ), #45429, .F. ) ;
#11127=CARTESIAN_POINT ( 'NONE',  ( 108.7397100058831256, -25.82697924850577920, 140.9432443235299672 ) ) ;
#11129=EDGE_CURVE ( 'NONE', #1886, #21233, #9835, .T. ) ;
#11130=CARTESIAN_POINT ( 'NONE',  ( 79.69020591995840164, -15.99866847873249931, 8.209451181318300428 ) ) ;
#11132=EDGE_CURVE ( 'NONE', #81323, #86805, #47541, .T. ) ;
#11134=CARTESIAN_POINT ( 'NONE',  ( 98.20607846729126322, -32.50961293922092210, 75.97276813305397525 ) ) ;
#11135=ORIENTED_EDGE ( 'NONE', *, *, #64461, .T. ) ;
#11137=VECTOR ( 'NONE', #46277, 1000.000000000000114 ) ;
#11138=ORIENTED_EDGE ( 'NONE', *, *, #185, .T. ) ;
#11140=CARTESIAN_POINT ( 'NONE',  ( 98.75024281215311817, -42.92452016420547523, 107.8480062282919647 ) ) ;
#11142=FACE_OUTER_BOUND ( 'NONE', #31045, .T. ) ;
#11143=CARTESIAN_POINT ( 'NONE',  ( 116.3212776292294421, -32.94146857471278622, 70.13562527591093954 ) ) ;
#11144=EDGE_CURVE ( 'NONE', #1770, #41877, #44991, .T. ) ;
#11145=DIRECTION ( 'NONE',  ( 1.000000000000000078E-15, -1.000000000000000083E-30, -1.000000000000000000 ) ) ;
#11148=CARTESIAN_POINT ( 'NONE',  ( 112.8057071037347754, -27.31004523576145360, 49.62895860924498947 ) ) ;
#11149=EDGE_LOOP ( 'NONE', ( #60096, #84479 ) ) ;
#11155=CARTESIAN_POINT ( 'NONE',  ( 115.0870346033256055, -35.21269407640084381, 156.7938046553059905 ) ) ;
#11156=AXIS2_PLACEMENT_3D ( 'NONE', #54648, #60587, #13356 ) ;
#11158=VECTOR ( 'NONE', #9841, 1000.000000000000000 ) ;
#11160=ORIENTED_EDGE ( 'NONE', *, *, #24837, .F. ) ;
#11165=EDGE_LOOP ( 'NONE', ( #43808, #49860, #50879, #56493, #74952, #52267, #43683, #43081, #52460, #67556, #60658, #86519, #81909 ) ) ;
#11166=DIRECTION ( 'NONE',  ( 0.000000000000000000, 0.000000000000000000, -1.000000000000000000 ) ) ;
#11167=CARTESIAN_POINT ( 'NONE',  ( 111.9232213988593827, -44.14162454355680865, 174.4701547344689629 ) ) ;
#11168=DIRECTION ( 'NONE',  ( -0.7071067811855830110, -0.7071067811875120235, 0.000000000000000000 ) ) ;
#11170=CIRCLE ( 'NONE', #76482, 1.000000000000000888 ) ;
#11171=EDGE_CURVE ( 'NONE', #78707, #44910, #80434, .T. ) ;
#11172=CARTESIAN_POINT ( 'NONE',  ( 95.60734603896362671, -36.72944715994100306, 311.6356252759112522 ) ) ;
#11174=ORIENTED_EDGE ( 'NONE', *, *, #9495, .F. ) ;
#11176=AXIS2_PLACEMENT_3D ( 'NONE', #41131, #56560, #69756 ) ;
#11177=EDGE_LOOP ( 'NONE', ( #41145, #78809, #77255, #62677 ) ) ;
#11179=EDGE_CURVE ( 'NONE', #18758, #15646, #57670, .T. ) ;
#11180=CARTESIAN_POINT ( 'NONE',  ( 113.5820732635001491, -31.81245485458596889, 217.1595189410199396 ) ) ;
#11181=CARTESIAN_POINT ( 'NONE',  ( 108.3221154657901337, -47.10103102204929826, 117.6727681330539639 ) ) ;
#11182=CARTESIAN_POINT ( 'NONE',  ( 115.1902516771093445, -44.19056033372790893, 78.22324432352995416 ) ) ;
#11183=CARTESIAN_POINT ( 'NONE',  ( 34.33598329127499227, -36.32844715994100682, 342.9256252759119548 ) ) ;
#11184=PLANE ( 'NONE',  #10365 ) ;
#11186=CARTESIAN_POINT ( 'NONE',  ( 107.9182609186041333, -47.15517531916538019, 173.6413395616249886 ) ) ;
#11189=CARTESIAN_POINT ( 'NONE',  ( 173.8164832912729878, 12.92155284005802862, 355.9756252759109998 ) ) ;
#11190=VERTEX_POINT ( 'NONE', #18190 ) ;
#11191=ORIENTED_EDGE ( 'NONE', *, *, #59367, .T. ) ;
#11197=AXIS2_PLACEMENT_3D ( 'NONE', #8456, #29351, #50667 ) ;
#11198=CARTESIAN_POINT ( 'NONE',  ( 107.0664832912750057, -36.72944715993903486, 0.7256252759109708128 ) ) ;
#11200=ORIENTED_EDGE ( 'NONE', *, *, #1942, .F. ) ;
#11202=CARTESIAN_POINT ( 'NONE',  ( 117.9248307134361937, -41.47673871369620002, 58.49848241876792798 ) ) ;
#11203=DIRECTION ( 'NONE',  ( -1.000000000000000000, 0.000000000000000000, -1.424786214935630051E-15 ) ) ;
#11204=DIRECTION ( 'NONE',  ( 0.9963424814100678706, -0.08544974978095865037, 0.000000000000000000 ) ) ;
#11206=CARTESIAN_POINT ( 'NONE',  ( 116.8058161338298504, -37.62879752186918836, 78.75276813305399060 ) ) ;
#11208=CARTESIAN_POINT ( 'NONE',  ( 117.9257662994439499, -34.79559216868042171, 194.9546728949589749 ) ) ;
#11209=FACE_OUTER_BOUND ( 'NONE', #35306, .T. ) ;
#11210=FACE_OUTER_BOUND ( 'NONE', #27148, .T. ) ;
#11212=CARTESIAN_POINT ( 'NONE',  ( 184.3595971212630502, -48.62134037874749026, 180.4678068554150343 ) ) ;
#11216=CARTESIAN_POINT ( 'NONE',  ( 142.8682495647594521, 8.654319075478468903, 394.9756252759102040 ) ) ;
#11217=CARTESIAN_POINT ( 'NONE',  ( 110.1504846022309607, -26.06634163003500859, 214.8403871806729342 ) ) ;
#11218=ORIENTED_EDGE ( 'NONE', *, *, #66795, .F. ) ;
#11220=CARTESIAN_POINT ( 'NONE',  ( 110.2841144599940577, -46.64559811412390644, 8.827053847339950465 ) ) ;
#11221=CARTESIAN_POINT ( 'NONE',  ( 117.2057360052074415, -34.12396560160815540, 120.0270538473389479 ) ) ;
#11222=AXIS2_PLACEMENT_3D ( 'NONE', #59771, #3049, #60214 ) ;
#11223=CARTESIAN_POINT ( 'NONE',  ( 182.5667039024476139, -32.29483332967956954, 313.9678068554149490 ) ) ;
#11224=CARTESIAN_POINT ( 'NONE',  ( 81.91398979882924891, -38.77444411305296512, 7.664507283848216446 ) ) ;
#11226=LINE ( 'NONE', #46175, #40878 ) ;
#11227=ORIENTED_EDGE ( 'NONE', *, *, #74092, .T. ) ;
#11228=CIRCLE ( 'NONE', #64865, 5.599999999999994316 ) ;
#11231=EDGE_LOOP ( 'NONE', ( #18068, #22637 ) ) ;
#11234=DIRECTION ( 'NONE',  ( 0.000000000000000000, 1.000000000000000000, 0.000000000000000000 ) ) ;
#11235=CARTESIAN_POINT ( 'NONE',  ( 100.0240874364964299, -28.99487838171179632, 281.6641967044822650 ) ) ;
#11238=ADVANCED_FACE ( 'NONE', ( #85481 ), #72280, .F. ) ;
#11239=VECTOR ( 'NONE', #58018, 1000.000000000000000 ) ;
#11240=AXIS2_PLACEMENT_3D ( 'NONE', #68589, #75405, #26789 ) ;
#11242=CARTESIAN_POINT ( 'NONE',  ( 80.06648329127399677, -8.729447159940999512, 293.6356252759119911 ) ) ;
#11244=CARTESIAN_POINT ( 'NONE',  ( 110.0404421551223209, -45.97207645956791566, 207.2467055423619513 ) ) ;
#11249=CYLINDRICAL_SURFACE ( 'NONE', #48480, 2.750000000000002665 ) ;
#11250=CARTESIAN_POINT ( 'NONE',  ( 97.92338638096642001, -40.78105084111301437, 181.6584144844725870 ) ) ;
#11252=CARTESIAN_POINT ( 'NONE',  ( 107.5258121372104227, -46.79223613538503912, 39.04444044875393871 ) ) ;
#11254=EDGE_CURVE ( 'NONE', #37176, #19054, #18765, .T. ) ;
#11255=CARTESIAN_POINT ( 'NONE',  ( 57.56670390244829605, -48.82844715994039575, 290.7178068554150627 ) ) ;
#11256=EDGE_CURVE ( 'NONE', #2257, #59978, #67687, .T. ) ;
#11257=CARTESIAN_POINT ( 'NONE',  ( 96.02263050233423769, -38.01213896886783061, 236.4184824187689458 ) ) ;
#11258=DIRECTION ( 'NONE',  ( -0.9254794337955620787, -0.3787978585227822492, 0.000000000000000000 ) ) ;
#11259=ORIENTED_EDGE ( 'NONE', *, *, #68566, .T. ) ;
#11260=CARTESIAN_POINT ( 'NONE',  ( 116.3176178399231873, -32.93748434060082531, 55.13562527591098217 ) ) ;
#11261=VERTEX_POINT ( 'NONE', #39971 ) ;
#11262=CIRCLE ( 'NONE', #83779, 5.599999999999994316 ) ;
#11264=CARTESIAN_POINT ( 'NONE',  ( 98.96120113019971143, -37.69594967233602034, 39.23951894101995919 ) ) ;
#11265=AXIS2_PLACEMENT_3D ( 'NONE', #55404, #60897, #42236 ) ;
#11266=CARTESIAN_POINT ( 'NONE',  ( 135.9194882200600318, -16.69035895461892949, 7.660272404628020837 ) ) ;
#11268=DIRECTION ( 'NONE',  ( 1.000000000000000000, 4.163336342344333240E-14, 0.000000000000000000 ) ) ;
#11269=ORIENTED_EDGE ( 'NONE', *, *, #22738, .T. ) ;
#11272=ORIENTED_EDGE ( 'NONE', *, *, #449, .F. ) ;
#11273=CARTESIAN_POINT ( 'NONE',  ( 103.1745875910851851, -27.05783000869472588, 130.3813395616259925 ) ) ;
#11275=CARTESIAN_POINT ( 'NONE',  ( 102.1503607674210343, -29.12389592045764530, 69.96765792331494538 ) ) ;
#11276=CARTESIAN_POINT ( 'NONE',  ( 97.82210220655964861, -40.54279968662331157, 87.63734374981743258 ) ) ;
#11277=CARTESIAN_POINT ( 'NONE',  ( 102.5140397859015877, -29.09155558458053292, 81.93586902018296314 ) ) ;
#11278=DIRECTION ( 'NONE',  ( 1.424786214935630051E-15, -4.252453317207020267E-31, -1.000000000000000000 ) ) ;
#11279=DIRECTION ( 'NONE',  ( 1.000000000000000000, -3.885780586188044357E-13, 0.000000000000000000 ) ) ;
#11280=CARTESIAN_POINT ( 'NONE',  ( 99.12701999692106369, -43.51930588094383978, 27.88991099019694175 ) ) ;
#11282=ORIENTED_EDGE ( 'NONE', *, *, #7022, .T. ) ;
#11285=ORIENTED_EDGE ( 'NONE', *, *, #34914, .F. ) ;
#11288=VERTEX_POINT ( 'NONE', #82681 ) ;
#11290=ADVANCED_FACE ( 'NONE', ( #54471 ), #75846, .F. ) ;
#11292=CYLINDRICAL_SURFACE ( 'NONE', #31071, 0.5000000000000073275 ) ;
#11294=CARTESIAN_POINT ( 'NONE',  ( 116.5710038106515611, -34.42130396933979597, 209.0156252759109634 ) ) ;
#11295=CARTESIAN_POINT ( 'NONE',  ( 101.6182654208066367, -28.31338856567544582, 125.5326905051223321 ) ) ;
#11296=CARTESIAN_POINT ( 'NONE',  ( 116.8171228686476297, -34.15291832581976195, 190.0314586088004489 ) ) ;
#11297=CARTESIAN_POINT ( 'NONE',  ( 96.92707254288593788, -39.15325348941441064, 52.51276813305394597 ) ) ;
#11298=CARTESIAN_POINT ( 'NONE',  ( 115.7830219863385963, -41.80246318181204401, 44.40644472814330612 ) ) ;
#11299=ORIENTED_EDGE ( 'NONE', *, *, #69395, .F. ) ;
#11305=ORIENTED_EDGE ( 'NONE', *, *, #14771, .T. ) ;
#11307=CARTESIAN_POINT ( 'NONE',  ( 107.0664832912739257, -18.82844715994099971, 239.5838068554170093 ) ) ;
#11310=CARTESIAN_POINT ( 'NONE',  ( 96.29057984255072711, -34.37493501460198075, 256.1432443235300980 ) ) ;
#11314=CARTESIAN_POINT ( 'NONE',  ( 107.8428746604417654, -27.05123223485975714, 264.4352769709337849 ) ) ;
#11316=CARTESIAN_POINT ( 'NONE',  ( 113.4020503763144063, -27.70036014686462522, 80.57753003781597556 ) ) ;
#11318=CARTESIAN_POINT ( 'NONE',  ( 113.8721965385452677, -28.72731865945801744, 139.5156252759109634 ) ) ;
#11320=CARTESIAN_POINT ( 'NONE',  ( 132.2601441849021455, -20.80290789369900750, 7.687431601936014047 ) ) ;
#11323=EDGE_CURVE ( 'NONE', #37688, #30738, #82235, .T. ) ;
#11324=DIRECTION ( 'NONE',  ( 1.000000000000000000, 6.145690160522480771E-16, 0.000000000000000000 ) ) ;
#11325=CARTESIAN_POINT ( 'NONE',  ( 97.81168895331838087, -40.51742574516882200, 287.6356252759109680 ) ) ;
#11326=DIRECTION ( 'NONE',  ( 0.9068632946707805287, -0.4214249218767882610, 9.493511560072084562E-16 ) ) ;
#11329=EDGE_CURVE ( 'NONE', #68446, #27190, #80906, .T. ) ;
#11331=CARTESIAN_POINT ( 'NONE',  ( 107.3350830925955961, -26.26357308316309869, 120.0556252759109555 ) ) ;
#11335=CIRCLE ( 'NONE', #80994, 5.599999999999994316 ) ;
#11337=EDGE_CURVE ( 'NONE', #74946, #82764, #40488, .T. ) ;
#11338=LINE ( 'NONE', #38586, #84367 ) ;
#11339=VERTEX_POINT ( 'NONE', #54021 ) ;
#11340=CARTESIAN_POINT ( 'NONE',  ( 108.9889396673064397, -47.63814106062356757, 122.7032443235299723 ) ) ;
#11343=CARTESIAN_POINT ( 'NONE',  ( 52.65249034007825912, -48.32844715994060181, 300.4678068554150059 ) ) ;
#11344=CARTESIAN_POINT ( 'NONE',  ( 117.0718954858691774, -35.46248235918008618, 143.9272919423464714 ) ) ;
#11345=ORIENTED_EDGE ( 'NONE', *, *, #44966, .T. ) ;
#11346=EDGE_LOOP ( 'NONE', ( #18636, #11869, #11693, #26833 ) ) ;
#11347=CARTESIAN_POINT ( 'NONE',  ( 168.5667039024482960, -48.82844715993496720, 180.4678068554150059 ) ) ;
#11348=CARTESIAN_POINT ( 'NONE',  ( 48.45959712129000252, -28.98061976758940617, -5.074374724088000832 ) ) ;
#11349=LINE ( 'NONE', #39049, #10646 ) ;
#11350=EDGE_CURVE ( 'NONE', #34909, #12059, #31668, .T. ) ;
#11351=DIRECTION ( 'NONE',  ( -0.9254794337955620787, -0.3787978585227822492, 0.000000000000000000 ) ) ;
#11354=DIRECTION ( 'NONE',  ( 1.000000000000000000, 4.299999999999999979E-14, 1.000000000000000078E-15 ) ) ;
#11356=ORIENTED_EDGE ( 'NONE', *, *, #13761, .F. ) ;
#11357=FACE_OUTER_BOUND ( 'NONE', #4266, .T. ) ;
#11358=CARTESIAN_POINT ( 'NONE',  ( 117.2759483237919085, -34.91131378075003511, 194.9546728949579517 ) ) ;
#11362=AXIS2_PLACEMENT_3D ( 'NONE', #9171, #36870, #44107 ) ;
#11363=CARTESIAN_POINT ( 'NONE',  ( 117.3137205126583211, -38.32096045344800928, 64.69181575210097890 ) ) ;
#11364=CARTESIAN_POINT ( 'NONE',  ( 110.8543372361816779, -45.98429251226213665, 52.88561369035437565 ) ) ;
#11365=EDGE_CURVE ( 'NONE', #16163, #28852, #50462, .T. ) ;
#11366=CARTESIAN_POINT ( 'NONE',  ( 31.71315051185499811, -33.70561438052111214, -5.074374724088000832 ) ) ;
#11367=EDGE_CURVE ( 'NONE', #1618, #48508, #40602, .T. ) ;
#11368=VECTOR ( 'NONE', #17524, 1000.000000000000000 ) ;
#11369=FACE_BOUND ( 'NONE', #66700, .T. ) ;
#11370=ORIENTED_EDGE ( 'NONE', *, *, #18081, .F. ) ;
#11371=DIRECTION ( 'NONE',  ( 2.900000000000000265E-14, -2.000000000000000155E-15, 1.000000000000000000 ) ) ;
#11372=VECTOR ( 'NONE', #80214, 1000.000000000000000 ) ;
#11373=EDGE_CURVE ( 'NONE', #51366, #18171, #1342, .T. ) ;
#11374=VECTOR ( 'NONE', #85875, 1000.000000000000114 ) ;
#11375=ORIENTED_EDGE ( 'NONE', *, *, #69213, .T. ) ;
#11376=ORIENTED_EDGE ( 'NONE', *, *, #77592, .F. ) ;
#11378=CARTESIAN_POINT ( 'NONE',  ( 115.4467593082293178, -40.97768201889641659, 244.8968214011349573 ) ) ;
#11382=VECTOR ( 'NONE', #24833, 1000.000000000000000 ) ;
#11384=ORIENTED_EDGE ( 'NONE', *, *, #38621, .T. ) ;
#11388=CARTESIAN_POINT ( 'NONE',  ( 115.6373213143784398, -30.77082676042341802, 279.3099109901966131 ) ) ;
#11389=ORIENTED_EDGE ( 'NONE', *, *, #87650, .F. ) ;
#11390=ORIENTED_EDGE ( 'NONE', *, *, #43835, .T. ) ;
#11391=CARTESIAN_POINT ( 'NONE',  ( 97.79975852078015919, -37.20246216128834504, 269.1852332267342831 ) ) ;
#11392=CARTESIAN_POINT ( 'NONE',  ( 51.42025729302669390, -31.94127993907680718, 342.9256252759109884 ) ) ;
#11398=CARTESIAN_POINT ( 'NONE',  ( 97.88103918441719031, -41.75145834149261503, 217.7241967044829494 ) ) ;
#11400=ORIENTED_EDGE ( 'NONE', *, *, #47403, .T. ) ;
#11401=CARTESIAN_POINT ( 'NONE',  ( 117.0163018969640376, -33.47459087099611708, 85.07848241876791917 ) ) ;
#11402=CARTESIAN_POINT ( 'NONE',  ( 51.06648329127400388, 22.62155284005901024, 333.4006252759110112 ) ) ;
#11406=CARTESIAN_POINT ( 'NONE',  ( 78.92327517541032478, -39.23064218986550600, 8.021355262919639628 ) ) ;
#11407=CARTESIAN_POINT ( 'NONE',  ( 194.5667039024485803, -47.82844715993405060, 129.9678068554150343 ) ) ;
#11408=DIRECTION ( 'NONE',  ( 1.000000000000000078E-15, -1.000000000000000083E-30, -1.000000000000000000 ) ) ;
#11409=CARTESIAN_POINT ( 'NONE',  ( 115.3759468638744181, -39.14889752855258820, 136.4071379886389650 ) ) ;
#11410=CARTESIAN_POINT ( 'NONE',  ( 117.5124522703044931, -35.85713534702714611, 249.8927681330537780 ) ) ;
#11411=B_SPLINE_CURVE_WITH_KNOTS ( 'NONE', 3,
 ( #40102, #46005, #86937, #66466, #52798, #39216, #12873, #26044, #19229, #24699, #52365, #67818, #18776, #45555, #5609, #40559, #26484, #67358 ),
 .UNSPECIFIED., .F., .F.,
 ( 4, 2, 2, 2, 2, 2, 2, 2, 4 ),
 ( 0.000000000000000000, 0.06249899055469551601, 0.1249979811093910320, 0.1874969716640865480, 0.2499959622187820640, 0.3124949527734776078, 0.3749939433281730961, 0.4374929338828685843, 0.4999919244375641281 ),
 .UNSPECIFIED. ) ;
#11418=CIRCLE ( 'NONE', #60679, 37.00000000000000711 ) ;
#11420=DIRECTION ( 'NONE',  ( 0.7071067811989784069, -0.7071067811741166276, 6.612322855976402389E-17 ) ) ;
#11421=VERTEX_POINT ( 'NONE', #49459 ) ;
#11423=CARTESIAN_POINT ( 'NONE',  ( 109.6445583207592591, -46.47969343970833478, 168.7823647920304211 ) ) ;
#11425=ADVANCED_FACE ( 'NONE', ( #13616, #34497 ), #14523, .F. ) ;
#11427=CARTESIAN_POINT ( 'NONE',  ( 98.50657384982324061, -36.30512124771701821, 170.7095626852199359 ) ) ;
#11428=CARTESIAN_POINT ( 'NONE',  ( 116.5143565283028266, -32.21898467494469998, 19.18133956162493092 ) ) ;
#11430=ORIENTED_EDGE ( 'NONE', *, *, #55064, .F. ) ;
#11434=VERTEX_POINT ( 'NONE', #83565 ) ;
#11436=ADVANCED_FACE ( 'NONE', ( #41302 ), #84920, .F. ) ;
#11439=ORIENTED_EDGE ( 'NONE', *, *, #65361, .F. ) ;
#11440=CARTESIAN_POINT ( 'NONE',  ( 97.67427069871116885, -40.16553667892655710, 167.6058069957254872 ) ) ;
#11442=CARTESIAN_POINT ( 'NONE',  ( 115.7821352934020780, -41.80395130134588300, 33.40652350832453266 ) ) ;
#11443=CARTESIAN_POINT ( 'NONE',  ( 110.8537393078288602, -45.98453721465049426, 132.8855622535276098 ) ) ;
#11444=EDGE_CURVE ( 'NONE', #22928, #36736, #49910, .T. ) ;
#11445=DIRECTION ( 'NONE',  ( 1.000000000000000000, 4.163336342344333240E-14, 0.000000000000000000 ) ) ;
#11446=ORIENTED_EDGE ( 'NONE', *, *, #39337, .T. ) ;
#11447=CARTESIAN_POINT ( 'NONE',  ( 99.74655714901966519, -44.23324885335900802, 21.96133956162593748 ) ) ;
#11448=CARTESIAN_POINT ( 'NONE',  ( 116.7674666963954309, -31.33607907186020824, 25.24229194257798881 ) ) ;
#11453=LINE ( 'NONE', #81417, #17727 ) ;
#11455=CARTESIAN_POINT ( 'NONE',  ( 132.9232751754149149, -39.23064218986716867, 8.021355262921384011 ) ) ;
#11456=VECTOR ( 'NONE', #66605, 1000.000000000000000 ) ;
#11457=DIRECTION ( 'NONE',  ( 0.000000000000000000, 0.000000000000000000, -1.000000000000000000 ) ) ;
#11460=VERTEX_POINT ( 'NONE', #50360 ) ;
#11461=CARTESIAN_POINT ( 'NONE',  ( 112.2029234908279562, -27.56599932623266724, 34.66991099019695355 ) ) ;
#11462=CARTESIAN_POINT ( 'NONE',  ( 113.1000543987032785, -45.99065659369661319, 219.0480062282919960 ) ) ;
#11463=CARTESIAN_POINT ( 'NONE',  ( 115.5915050065794247, -42.76776344903117888, 49.33562527591095659 ) ) ;
#11467=AXIS2_PLACEMENT_3D ( 'NONE', #45749, #4453, #24895 ) ;
#11468=EDGE_CURVE ( 'NONE', #15026, #22617, #19726, .T. ) ;
#11469=ORIENTED_EDGE ( 'NONE', *, *, #19737, .F. ) ;
#11471=ORIENTED_EDGE ( 'NONE', *, *, #47558, .T. ) ;
#11472=CARTESIAN_POINT ( 'NONE',  ( 118.1720832024964807, -36.20253795304678590, 114.8641967044819694 ) ) ;
#11474=ORIENTED_EDGE ( 'NONE', *, *, #36868, .T. ) ;
#11475=CARTESIAN_POINT ( 'NONE',  ( 115.4997179687694171, -29.61999039777962039, 220.3718157521019521 ) ) ;
#11477=DIRECTION ( 'NONE',  ( -0.7071067811865476838, -0.7071067811865473507, 0.000000000000000000 ) ) ;
#11478=CARTESIAN_POINT ( 'NONE',  ( 142.8832909413445122, -79.11588146349312467, 543.8623766218582887 ) ) ;
#11479=FACE_OUTER_BOUND ( 'NONE', #13055, .T. ) ;
#11480=ADVANCED_FACE ( 'NONE', ( #22239 ), #62658, .T. ) ;
#11481=AXIS2_PLACEMENT_3D ( 'NONE', #60018, #87753, #80959 ) ;
#11482=CARTESIAN_POINT ( 'NONE',  ( 131.4004675426832875, -37.42701295172433618, 2.979899338979598689 ) ) ;
#11483=LINE ( 'NONE', #86895, #2233 ) ;
#11485=CARTESIAN_POINT ( 'NONE',  ( 113.7965574739370993, -44.62378898692907825, 153.1508633711499670 ) ) ;
#11487=ORIENTED_EDGE ( 'NONE', *, *, #58310, .F. ) ;
#11488=CARTESIAN_POINT ( 'NONE',  ( 112.9486100676287208, -29.40298074535265727, 115.9577737820869601 ) ) ;
#11491=CARTESIAN_POINT ( 'NONE',  ( 117.4208826025846690, -36.15918394849474282, 269.8822919425771829 ) ) ;
#11494=LINE ( 'NONE', #39189, #42317 ) ;
#11495=FACE_OUTER_BOUND ( 'NONE', #34002, .T. ) ;
#11496=AXIS2_PLACEMENT_3D ( 'NONE', #71858, #37330, #2818 ) ;
#11498=CARTESIAN_POINT ( 'NONE',  ( 107.0667039024479834, -36.72944715994099596, 239.5838068554170093 ) ) ;
#11499=LINE ( 'NONE', #67799, #41496 ) ;
#11500=AXIS2_PLACEMENT_3D ( 'NONE', #65617, #57119, #15815 ) ;
#11501=CARTESIAN_POINT ( 'NONE',  ( 113.6005200848514676, -45.61596423689133672, 183.0689586092439640 ) ) ;
#11502=VERTEX_POINT ( 'NONE', #10381 ) ;
#11505=CARTESIAN_POINT ( 'NONE',  ( 77.96925277059908410, -16.94806367528691027, 2.376725340793110597 ) ) ;
#11507=LINE ( 'NONE', #47344, #60597 ) ;
#11509=ADVANCED_FACE ( 'NONE', ( #64902 ), #4009, .F. ) ;
#11510=VERTEX_POINT ( 'NONE', #86243 ) ;
#11512=CARTESIAN_POINT ( 'NONE',  ( 117.4129020423329450, -35.18752443080737891, 218.9441967044829482 ) ) ;
#11516=ORIENTED_EDGE ( 'NONE', *, *, #33896, .T. ) ;
#11517=VECTOR ( 'NONE', #83173, 1000.000000000000000 ) ;
#11518=B_SPLINE_CURVE_WITH_KNOTS ( 'NONE', 3,
 ( #20807, #75776, #13543, #40344, #83056, #68957, #68063, #26711, #13108, #19015, #46699, #6281, #41227, #73978, #39455, #88957, #74430, #12204 ),
 .UNSPECIFIED., .F., .F.,
 ( 4, 2, 2, 2, 2, 2, 2, 2, 4 ),
 ( 0.4999390761915182280, 0.5624466916675784356, 0.6249543071436386432, 0.6874619226196989619, 0.7499695380957591695, 0.8124771535718193771, 0.8749847690478795847, 0.9374923845239397924, 1.000000000000000000 ),
 .UNSPECIFIED. ) ;
#11519=CARTESIAN_POINT ( 'NONE',  ( 116.4889884589737363, -40.12238724215244190, 64.55198567951927657 ) ) ;
#11520=DIRECTION ( 'NONE',  ( 0.000000000000000000, -1.000000000000000000, 0.000000000000000000 ) ) ;
#11521=CARTESIAN_POINT ( 'NONE',  ( 72.31648329127396835, -9.833000550534366724, 14.92562527591093691 ) ) ;
#11522=CARTESIAN_POINT ( 'NONE',  ( 106.4288663150950214, -28.56390168778064975, 22.95666179816197072 ) ) ;
#11523=CARTESIAN_POINT ( 'NONE',  ( 20.03715912545641231, -24.95799193693202156, 180.4678068554150911 ) ) ;
#11524=ORIENTED_EDGE ( 'NONE', *, *, #45663, .F. ) ;
#11526=CIRCLE ( 'NONE', #7130, 11.45913725231036118 ) ;
#11527=ADVANCED_FACE ( 'NONE', ( #10818 ), #24907, .F. ) ;
#11528=CARTESIAN_POINT ( 'NONE',  ( 80.80620050782613362, -16.05355276379784968, 8.162233076788782071 ) ) ;
#11529=EDGE_LOOP ( 'NONE', ( #80455, #62588, #45728, #66153 ) ) ;
#11530=ORIENTED_EDGE ( 'NONE', *, *, #79037, .T. ) ;
#11534=CARTESIAN_POINT ( 'NONE',  ( 51.06648329127400388, -0.2185775633790978945, 330.8831252759119934 ) ) ;
#11536=EDGE_CURVE ( 'NONE', #3245, #73802, #67915, .T. ) ;
#11537=CARTESIAN_POINT ( 'NONE',  ( 98.53752338633383090, -37.19093893883378144, 75.79241982807700140 ) ) ;
#11538=CARTESIAN_POINT ( 'NONE',  ( 117.9557474314311349, -34.69982462793587530, 203.9851490854349549 ) ) ;
#11540=EDGE_CURVE ( 'NONE', #45837, #29906, #58079, .T. ) ;
#11541=CARTESIAN_POINT ( 'NONE',  ( 117.4355769707883468, -40.49052663852281597, 173.5375300378159693 ) ) ;
#11542=CARTESIAN_POINT ( 'NONE',  ( 106.1835720340748139, -46.77890140548399955, 22.50653266953309384 ) ) ;
#11543=CARTESIAN_POINT ( 'NONE',  ( 100.8484424157226442, -45.14118303587278547, 253.0699109901968882 ) ) ;
#11547=AXIS2_PLACEMENT_3D ( 'NONE', #84991, #22762, #10013 ) ;
#11549=B_SPLINE_CURVE_WITH_KNOTS ( 'NONE', 3,
 ( #54268, #67031, #19782, #18885, #47909, #80676, #40208, #5257, #32951, #6164, #60649, #67928, #88390, #26150, #82032, #47467, #81586, #19338, #33854, #76087, #55609, #14775, #69730, #71086, #41998, #7944, #7053, #35642, #63813, #50157, #42443, #13864, #62455, #83363, #49260, #35185, #56066, #1135 ),
 .UNSPECIFIED., .F., .F.,
 ( 4, 2, 2, 1, 2, 2, 2, 2, 1, 1, 2, 2, 2, 1, 2, 2, 1, 2, 1, 2, 2, 4 ),
 ( 0.000000000000000000, 0.04166793602364190358, 0.05208492002955231182, 0.05729341203250756104, 0.05989765803398552912, 0.06250190403546351803, 0.08333587204728555575, 0.1041698400591075935, 0.1145868240650192021, 0.1197953160679756379, 0.1223995620694541958, 0.1250038080709327815, 0.1666717440945731377, 0.1770887281004829561, 0.1822972201034377959, 0.1875057121063926635, 0.2083396801182141878, 0.2291736481300356287, 0.2395906321359451141, 0.2447991241388997319, 0.2500076161418543497, 0.3333434881890883217 ),
 .UNSPECIFIED. ) ;
#11551=VECTOR ( 'NONE', #86493, 1000.000000000000000 ) ;
#11553=B_SPLINE_CURVE_WITH_KNOTS ( 'NONE', 3,
 ( #8805, #29675, #21074, #49654, #7444, #85110, #77381, #77837, #71027, #8346, #6996, #83307, #48750, #78296, #28316, #36043, #14267, #14716, #63757, #35584, #56009, #1537, #50101, #83760, #69226, #76485, #35132, #70116 ),
 .UNSPECIFIED., .F., .F.,
 ( 4, 2, 2, 2, 2, 2, 2, 2, 2, 2, 1, 1, 1, 1, 2, 4 ),
 ( 0.000000000000000000, 0.06250188926545433010, 0.1250037785309086602, 0.1875056677963629903, 0.2500075570618173204, 0.3125094463272716783, 0.3750113355927259806, 0.4375132248581803385, 0.4687641694909075452, 0.4843896418072711763, 0.4922023779654531306, 0.4961087460445438024, 0.4980619300840890551, 0.4990385221038616259, 0.4995268181137479391, 0.5000151141236341967 ),
 .UNSPECIFIED. ) ;
#11554=CARTESIAN_POINT ( 'NONE',  ( 97.81168895331838087, -40.51742574516882200, 287.6356252759109680 ) ) ;
#11555=CARTESIAN_POINT ( 'NONE',  ( 115.4954577264304731, -29.50689403799194110, 229.4022919425779605 ) ) ;
#11556=VERTEX_POINT ( 'NONE', #65346 ) ;
#11557=CARTESIAN_POINT ( 'NONE',  ( 106.9749943965245365, -47.15435292659226718, 187.5699109901969734 ) ) ;
#11558=CARTESIAN_POINT ( 'NONE',  ( 97.06110197059325628, -37.99657418247586804, 266.4273502531260078 ) ) ;
#11559=CARTESIAN_POINT ( 'NONE',  ( 49.16670390244701139, -26.71338133339240528, -5.074374724088000832 ) ) ;
#11562=CARTESIAN_POINT ( 'NONE',  ( 100.0247289185300588, -32.06647811954630356, 277.6356252759111953 ) ) ;
#11563=DIRECTION ( 'NONE',  ( 3.339108161477000479E-13, -1.000000000000000000, 4.100000000000000342E-29 ) ) ;
#11564=CARTESIAN_POINT ( 'NONE',  ( 97.83886487280460642, -40.58324923297708864, 172.6412926176714393 ) ) ;
#11566=EDGE_CURVE ( 'NONE', #65338, #81967, #85372, .T. ) ;
#11567=CARTESIAN_POINT ( 'NONE',  ( 128.5492039024480562, -58.72944715994093201, 231.5838068554170093 ) ) ;
#11568=AXIS2_PLACEMENT_3D ( 'NONE', #81481, #87381, #52368 ) ;
#11569=DIRECTION ( 'NONE',  ( 1.000000000000000078E-15, -1.000000000000000083E-30, -1.000000000000000000 ) ) ;
#11571=LINE ( 'NONE', #44725, #83672 ) ;
#11572=LINE ( 'NONE', #86982, #2827 ) ;
#11573=EDGE_CURVE ( 'NONE', #70290, #26617, #89647, .T. ) ;
#11577=CARTESIAN_POINT ( 'NONE',  ( 116.0742729640735007, -42.02152512393894312, 238.4041967044829562 ) ) ;
#11578=CARTESIAN_POINT ( 'NONE',  ( 98.84006766826026080, -28.19945879207355688, 111.6870538473389587 ) ) ;
#11579=CARTESIAN_POINT ( 'NONE',  ( 105.1027920011780452, -26.44660240447466037, 231.2270538473399597 ) ) ;
#11580=FACE_OUTER_BOUND ( 'NONE', #310, .T. ) ;
#11582=CARTESIAN_POINT ( 'NONE',  ( 184.5667039024486087, -48.82844715993447693, 129.9678068554150059 ) ) ;
#11584=CARTESIAN_POINT ( 'NONE',  ( 116.3216976867776964, -32.94060878512167534, 40.13562527591096796 ) ) ;
#11585=DIRECTION ( 'NONE',  ( 0.000000000000000000, 0.000000000000000000, -1.000000000000000000 ) ) ;
#11588=ORIENTED_EDGE ( 'NONE', *, *, #65287, .T. ) ;
#11589=VERTEX_POINT ( 'NONE', #58955 ) ;
#11590=CIRCLE ( 'NONE', #21706, 3.249999999999975131 ) ;
#11591=CARTESIAN_POINT ( 'NONE',  ( 99.46962827726154899, -41.65933777599243371, 146.2190864947439763 ) ) ;
#11592=CARTESIAN_POINT ( 'NONE',  ( 163.1543517358615247, -31.62489322947688919, 313.9678068554149490 ) ) ;
#11593=EDGE_LOOP ( 'NONE', ( #19158, #83622, #45477, #2774 ) ) ;
#11594=CARTESIAN_POINT ( 'NONE',  ( 117.7221270036566807, -41.68118999199129604, 4.925625275910981316 ) ) ;
#11595=CARTESIAN_POINT ( 'NONE',  ( 108.3168256696638281, -47.05733704442508980, 113.6727681330539639 ) ) ;
#11596=DIRECTION ( 'NONE',  ( -1.000000000000000000, -4.299999999999999979E-14, -1.000000000000000078E-15 ) ) ;
#11597=CARTESIAN_POINT ( 'NONE',  ( 77.67297288197553939, -17.37149612621849215, 7.198162082949088436 ) ) ;
#11598=CARTESIAN_POINT ( 'NONE',  ( 83.06670390244796920, -67.87844715994100397, 213.1838068554149856 ) ) ;
#11599=DIRECTION ( 'NONE',  ( -1.000000000000000078E-15, 1.000000000000000083E-30, 1.000000000000000000 ) ) ;
#11601=CARTESIAN_POINT ( 'NONE',  ( 96.86520444330096780, -38.59296402346417665, 51.48229194257797303 ) ) ;
#11602=EDGE_LOOP ( 'NONE', ( #32295, #56409 ) ) ;
#11604=EDGE_LOOP ( 'NONE', ( #29551, #82243, #78779, #43337 ) ) ;
#11607=CARTESIAN_POINT ( 'NONE',  ( 107.6167445103326230, -46.48501816386541208, 148.6213395616249784 ) ) ;
#11608=DIRECTION ( 'NONE',  ( 1.000000000000000000, 1.175184669633339961E-16, -2.900000000000000265E-14 ) ) ;
#11610=FACE_OUTER_BOUND ( 'NONE', #64712, .T. ) ;
#11611=DIRECTION ( 'NONE',  ( -1.000000000000000078E-15, 1.000000000000000000, 0.000000000000000000 ) ) ;
#11615=CARTESIAN_POINT ( 'NONE',  ( 98.66494773507966443, -43.87633619481174918, 76.89943479971999807 ) ) ;
#11618=AXIS2_PLACEMENT_3D ( 'NONE', #3422, #38822, #24317 ) ;
#11619=ADVANCED_FACE ( 'NONE', ( #45323 ), #64455, .T. ) ;
#11621=CARTESIAN_POINT ( 'NONE',  ( 45.77381068350503313, -48.62134037888107230, 300.4678068554150059 ) ) ;
#11623=CARTESIAN_POINT ( 'NONE',  ( 116.3457274436100164, -36.88499157630047165, 151.6309475124489552 ) ) ;
#11626=FACE_OUTER_BOUND ( 'NONE', #33127, .T. ) ;
#11627=ORIENTED_EDGE ( 'NONE', *, *, #68566, .F. ) ;
#11628=ORIENTED_EDGE ( 'NONE', *, *, #31977, .F. ) ;
#11630=ORIENTED_EDGE ( 'NONE', *, *, #3124, .T. ) ;
#11633=CARTESIAN_POINT ( 'NONE',  ( 97.82234778274722942, -32.72736474536957019, 207.4330118773259528 ) ) ;
#11635=VECTOR ( 'NONE', #44943, 1000.000000000000114 ) ;
#11638=ORIENTED_EDGE ( 'NONE', *, *, #70755, .T. ) ;
#11639=ORIENTED_EDGE ( 'NONE', *, *, #48627, .T. ) ;
#11642=EDGE_CURVE ( 'NONE', #55229, #61739, #78555, .T. ) ;
#11643=AXIS2_PLACEMENT_3D ( 'NONE', #63391, #84309, #28416 ) ;
#11644=CARTESIAN_POINT ( 'NONE',  ( 106.6756582537710187, -44.91051946355214852, 245.3566617981629463 ) ) ;
#11645=CARTESIAN_POINT ( 'NONE',  ( 96.76980119632513322, -38.49712976775982298, 91.46133956162493917 ) ) ;
#11646=ADVANCED_FACE ( 'NONE', ( #16311 ), #73042, .T. ) ;
#11647=CARTESIAN_POINT ( 'NONE',  ( 106.8416606513709866, -48.55305329746398257, 77.56133956162491927 ) ) ;
#11648=CARTESIAN_POINT ( 'NONE',  ( 112.8268282670517237, -28.64838596922752245, 249.5838068554169240 ) ) ;
#11650=CARTESIAN_POINT ( 'NONE',  ( 97.81169585860149596, -40.51742224678086046, 106.6356332503197137 ) ) ;
#11651=CARTESIAN_POINT ( 'NONE',  ( 114.4628154322623033, -28.51554874119783634, 155.5051490854349652 ) ) ;
#11653=ORIENTED_EDGE ( 'NONE', *, *, #37695, .F. ) ;
#11658=CARTESIAN_POINT ( 'NONE',  ( 97.81283413487385303, -40.52022386196461667, 132.6362477986331783 ) ) ;
#11662=CARTESIAN_POINT ( 'NONE',  ( 41.56648329127399677, -18.82844715994099971, 81.04262527591200183 ) ) ;
#11663=EDGE_CURVE ( 'NONE', #26420, #80043, #17646, .T. ) ;
#11664=EDGE_LOOP ( 'NONE', ( #23371, #83864 ) ) ;
#11665=CARTESIAN_POINT ( 'NONE',  ( 104.4875610206461971, -26.97946579336972306, 91.28165471780177143 ) ) ;
#11666=CARTESIAN_POINT ( 'NONE',  ( 96.08737379349030050, -38.00938547453511518, 86.43086337114897333 ) ) ;
#11669=CARTESIAN_POINT ( 'NONE',  ( 172.5664832912740110, -36.32844715994070839, 198.9256252759119832 ) ) ;
#11670=CARTESIAN_POINT ( 'NONE',  ( 103.2241971045484092, -45.72390501747114655, 92.25562527591097250 ) ) ;
#11672=CARTESIAN_POINT ( 'NONE',  ( 113.6717327907683597, -45.56316108038139845, 184.0994347997199725 ) ) ;
#11678=LINE ( 'NONE', #87978, #58726 ) ;
#11679=CARTESIAN_POINT ( 'NONE',  ( 115.0907168629284172, -30.61997542873368516, 134.3440372771844977 ) ) ;
#11680=VECTOR ( 'NONE', #48194, 1000.000000000000000 ) ;
#11681=CARTESIAN_POINT ( 'NONE',  ( 63.56670390244708813, -40.82844715994014706, 180.4678068554151196 ) ) ;
#11682=CARTESIAN_POINT ( 'NONE',  ( 117.5184129516626257, -36.12626193255995588, 228.8727681330539667 ) ) ;
#11683=VERTEX_POINT ( 'NONE', #5817 ) ;
#11684=CARTESIAN_POINT ( 'NONE',  ( 99.09551545717923204, -30.55067741387680158, 145.8023164730312828 ) ) ;
#11685=CARTESIAN_POINT ( 'NONE',  ( 116.6018303087422225, -42.36526137987677743, 279.4137205140061724 ) ) ;
#11686=CARTESIAN_POINT ( 'NONE',  ( 102.0609898346451274, -27.53498505803861107, 141.4727681330539895 ) ) ;
#11689=DIRECTION ( 'NONE',  ( -2.999999999999999839E-15, 1.000000000000000000, -2.999999999999999900E-30 ) ) ;
#11690=DIRECTION ( 'NONE',  ( 1.000000000000000000, 0.000000000000000000, 0.000000000000000000 ) ) ;
#11691=ORIENTED_EDGE ( 'NONE', *, *, #33403, .F. ) ;
#11693=ORIENTED_EDGE ( 'NONE', *, *, #68961, .T. ) ;
#11694=EDGE_LOOP ( 'NONE', ( #49271, #26950, #49740, #17613 ) ) ;
#11696=VERTEX_POINT ( 'NONE', #82133 ) ;
#11697=CARTESIAN_POINT ( 'NONE',  ( 134.0664832912739826, -9.029447159941003775, 4.925625275910997303 ) ) ;
#11698=CARTESIAN_POINT ( 'NONE',  ( 106.5192459994187715, -25.71289806663804711, 41.12800622829193742 ) ) ;
#11699=CARTESIAN_POINT ( 'NONE',  ( 50.97905606905892739, -31.62489322948754022, 342.9256252759109884 ) ) ;
#11701=DIRECTION ( 'NONE',  ( 0.000000000000000000, 1.000000000000000000, 0.000000000000000000 ) ) ;
#11704=CARTESIAN_POINT ( 'NONE',  ( 114.4310042120387862, -41.05610445278038156, 237.8267055423629586 ) ) ;
#11705=VERTEX_POINT ( 'NONE', #75297 ) ;
#11708=DIRECTION ( 'NONE',  ( 0.7071067811864693020, 0.7071067811866258435, -2.899137802865049595E-29 ) ) ;
#11709=CARTESIAN_POINT ( 'NONE',  ( 112.0660841691505993, -45.48830024005852124, 102.9895797908911277 ) ) ;
#11710=EDGE_CURVE ( 'NONE', #13679, #72194, #30186, .T. ) ;
#11713=CARTESIAN_POINT ( 'NONE',  ( 98.21984324360056462, -33.56503799257626497, 22.49682140113501561 ) ) ;
#11714=VECTOR ( 'NONE', #233, 1000.000000000000000 ) ;
#11717=CARTESIAN_POINT ( 'NONE',  ( 97.51798386322114709, -31.03399775848789233, 280.8984824187687082 ) ) ;
#11720=CARTESIAN_POINT ( 'NONE',  ( 106.6600009669583358, -26.71630602157825862, 56.10883478359531296 ) ) ;
#11721=VECTOR ( 'NONE', #12178, 1000.000000000000000 ) ;
#11722=DIRECTION ( 'NONE',  ( -1.000000000000000078E-15, 1.000000000000000083E-30, 1.000000000000000000 ) ) ;
#11723=CARTESIAN_POINT ( 'NONE',  ( 116.2008526694824582, -35.09873344310054932, 46.78523322673494533 ) ) ;
#11728=VERTEX_POINT ( 'NONE', #67126 ) ;
#11729=DIRECTION ( 'NONE',  ( 0.000000000000000000, 0.000000000000000000, -1.000000000000000000 ) ) ;
#11731=ORIENTED_EDGE ( 'NONE', *, *, #39589, .T. ) ;
#11732=CARTESIAN_POINT ( 'NONE',  ( 103.2053365856880873, -46.45145584090948176, 117.2756252759109543 ) ) ;
#11734=CARTESIAN_POINT ( 'NONE',  ( 113.7363519267670995, -42.85525508308114695, 77.64575316141092287 ) ) ;
#11736=CARTESIAN_POINT ( 'NONE',  ( 97.85179084974261343, -40.61417562505091894, 87.64349320109216990 ) ) ;
#11737=CARTESIAN_POINT ( 'NONE',  ( 103.8469135698534416, -45.55616208374542708, 93.71777378208700782 ) ) ;
#11740=CARTESIAN_POINT ( 'NONE',  ( 95.23451729606020422, -35.71612027476381002, 32.25848241876794020 ) ) ;
#11741=VECTOR ( 'NONE', #60816, 1000.000000000000000 ) ;
#11742=CARTESIAN_POINT ( 'NONE',  ( 99.09585084692569978, -30.55024265790509475, 181.8027529189448046 ) ) ;
#11743=ORIENTED_EDGE ( 'NONE', *, *, #62139, .T. ) ;
#11744=PLANE ( 'NONE',  #51670 ) ;
#11746=CARTESIAN_POINT ( 'NONE',  ( 77.40046754268347229, -19.42701295173674580, 2.979899338979277612 ) ) ;
#11747=ORIENTED_EDGE ( 'NONE', *, *, #16541, .T. ) ;
#11748=ORIENTED_EDGE ( 'NONE', *, *, #35730, .T. ) ;
#11749=ADVANCED_FACE ( 'NONE', ( #40761 ), #74849, .F. ) ;
#11750=VECTOR ( 'NONE', #15346, 1000.000000000000000 ) ;
#11751=CARTESIAN_POINT ( 'NONE',  ( 107.0667039024479834, -36.72944715994101017, 239.5838068554170093 ) ) ;
#11752=ORIENTED_EDGE ( 'NONE', *, *, #74295, .F. ) ;
#11753=CARTESIAN_POINT ( 'NONE',  ( 105.2318265017783716, -27.12228994480470945, 235.2270538473399313 ) ) ;
#11754=CARTESIAN_POINT ( 'NONE',  ( 99.37624259870420929, -30.29005673034905044, 125.7706194579988619 ) ) ;
#11756=EDGE_CURVE ( 'NONE', #58495, #26148, #82469, .T. ) ;
#11757=CARTESIAN_POINT ( 'NONE',  ( 101.1410050838726846, -27.39870825576502966, 61.51467289495899138 ) ) ;
#11758=VECTOR ( 'NONE', #53734, 1000.000000000000000 ) ;
#11759=CARTESIAN_POINT ( 'NONE',  ( 46.03715912545425937, -48.62818131006086020, 313.9678068554150059 ) ) ;
#11761=DIRECTION ( 'NONE',  ( 0.000000000000000000, 0.000000000000000000, 1.000000000000000000 ) ) ;
#11764=ORIENTED_EDGE ( 'NONE', *, *, #51117, .F. ) ;
#11767=CARTESIAN_POINT ( 'NONE',  ( 96.91023542590092177, -30.67149048741783091, 280.8984824187682534 ) ) ;
#11771=CARTESIAN_POINT ( 'NONE',  ( 100.7304913082922440, -30.25890808522221320, 270.1276579233149278 ) ) ;
#11772=PLANE ( 'NONE',  #63503 ) ;
#11773=CARTESIAN_POINT ( 'NONE',  ( 109.6783822832554591, -47.44587409406599221, 83.75467289495897205 ) ) ;
#11775=CARTESIAN_POINT ( 'NONE',  ( 103.4531379826000261, -46.55545292317445671, 142.2956252759109645 ) ) ;
#11777=DIRECTION ( 'NONE',  ( 0.000000000000000000, 0.000000000000000000, -1.000000000000000000 ) ) ;
#11778=EDGE_CURVE ( 'NONE', #64418, #14919, #19883, .T. ) ;
#11780=CARTESIAN_POINT ( 'NONE',  ( 83.56670390244801183, -36.72944715994108122, 218.8274735512160589 ) ) ;
#11781=VECTOR ( 'NONE', #53658, 1000.000000000000000 ) ;
#11782=LINE ( 'NONE', #11325, #74010 ) ;
#11783=EDGE_CURVE ( 'NONE', #40177, #77354, #15674, .T. ) ;
#11786=CARTESIAN_POINT ( 'NONE',  ( 41.56648329127398966, -27.82844715994070484, 138.9256252759119832 ) ) ;
#11787=CARTESIAN_POINT ( 'NONE',  ( 102.0606772939666627, -27.53441096011033906, 145.4727681330539610 ) ) ;
#11792=LINE ( 'NONE', #71898, #31486 ) ;
#11793=DIRECTION ( 'NONE',  ( -1.000000000000000000, -5.800000000000000483E-29, 2.900000000000000265E-14 ) ) ;
#11794=EDGE_LOOP ( 'NONE', ( #51067, #20486, #70340, #56437 ) ) ;
#11795=VECTOR ( 'NONE', #46695, 1000.000000000000000 ) ;
#11796=CARTESIAN_POINT ( 'NONE',  ( 95.75500511041516916, -40.34669435480882527, 131.5727681330539554 ) ) ;
#11798=CARTESIAN_POINT ( 'NONE',  ( 90.44969454456408187, -20.11243780205710507, 239.5838068554175209 ) ) ;
#11799=CARTESIAN_POINT ( 'NONE',  ( 46.32460016641721978, -48.34074026909785005, 300.4678068554150059 ) ) ;
#11801=ORIENTED_EDGE ( 'NONE', *, *, #67842, .F. ) ;
#11804=CARTESIAN_POINT ( 'NONE',  ( 111.0197563349041872, -27.48142275213628949, 249.7547965408143966 ) ) ;
#11805=CARTESIAN_POINT ( 'NONE',  ( 113.1782937260175288, -44.75186862798841503, 158.0939586047068985 ) ) ;
#11806=PLANE ( 'NONE',  #18316 ) ;
#11807=VECTOR ( 'NONE', #51578, 1000.000000000000000 ) ;
#11811=ORIENTED_EDGE ( 'NONE', *, *, #36868, .F. ) ;
#11812=DIRECTION ( 'NONE',  ( 1.000000000000000000, 0.000000000000000000, 0.000000000000000000 ) ) ;
#11814=CARTESIAN_POINT ( 'NONE',  ( 101.5632356570521324, -44.81509498605967678, 193.1013395616249682 ) ) ;
#11815=VECTOR ( 'NONE', #14581, 1000.000000000000000 ) ;
#11816=LINE ( 'NONE', #60391, #28366 ) ;
#11818=CARTESIAN_POINT ( 'NONE',  ( 113.9027609268605659, -43.72435554967452731, 69.19276813305297935 ) ) ;
#11819=CARTESIAN_POINT ( 'NONE',  ( 111.0144279432724232, -45.91752097597848348, 52.89941656328505815 ) ) ;
#11821=CIRCLE ( 'NONE', #39373, 16.00000000000000000 ) ;
#11822=CARTESIAN_POINT ( 'NONE',  ( 97.79819224205189698, -40.48430588183206424, 22.63277894479249142 ) ) ;
#11824=CARTESIAN_POINT ( 'NONE',  ( 107.0667039024479834, -36.72944715994101017, 239.5838068554170093 ) ) ;
#11825=VERTEX_POINT ( 'NONE', #54361 ) ;
#11826=EDGE_LOOP ( 'NONE', ( #89248, #73908, #7175, #37340 ) ) ;
#11827=CARTESIAN_POINT ( 'NONE',  ( 106.4165995140572250, -45.56720307917569102, 218.9501547344689527 ) ) ;
#11828=CARTESIAN_POINT ( 'NONE',  ( 113.1804603017864252, -44.75025694503620599, 54.09380354789409751 ) ) ;
#11830=DIRECTION ( 'NONE',  ( 1.000000000000000000, -5.337610695313248426E-16, 0.000000000000000000 ) ) ;
#11833=CIRCLE ( 'NONE', #62604, 11.57110091390434192 ) ;
#11834=VERTEX_POINT ( 'NONE', #81235 ) ;
#11836=LINE ( 'NONE', #31373, #82193 ) ;
#11838=CARTESIAN_POINT ( 'NONE',  ( 98.42358855985509081, -42.06826316073455274, 11.76800622829193799 ) ) ;
#11839=ORIENTED_EDGE ( 'NONE', *, *, #29925, .T. ) ;
#11841=CARTESIAN_POINT ( 'NONE',  ( 98.99928044157054785, -35.48447157832033128, 264.0223760838769635 ) ) ;
#11842=EDGE_CURVE ( 'NONE', #28950, #22788, #24423, .T. ) ;
#11843=EDGE_CURVE ( 'NONE', #733, #43944, #18525, .T. ) ;
#11844=CARTESIAN_POINT ( 'NONE',  ( 191.6377717143134589, -48.82844715994099971, 307.9888746672805269 ) ) ;
#11845=CARTESIAN_POINT ( 'NONE',  ( 111.8077268321493563, -46.78591733285071541, 137.9270538473399768 ) ) ;
#11849=AXIS2_PLACEMENT_3D ( 'NONE', #32217, #73112, #88108 ) ;
#11850=CARTESIAN_POINT ( 'NONE',  ( 103.8062037941931095, -48.17417041148343060, 213.3556252759109668 ) ) ;
#11852=EDGE_LOOP ( 'NONE', ( #9730, #83809 ) ) ;
#11854=CARTESIAN_POINT ( 'NONE',  ( 116.7149026195978792, -32.57661448200846621, 75.14991099019697174 ) ) ;
#11855=DIRECTION ( 'NONE',  ( 0.000000000000000000, 1.000000000000000000, 0.000000000000000000 ) ) ;
#11856=EDGE_CURVE ( 'NONE', #21233, #1886, #2646, .T. ) ;
#11858=VERTEX_POINT ( 'NONE', #12174 ) ;
#11861=CARTESIAN_POINT ( 'NONE',  ( 115.8239080364990059, -31.72738345397315385, 159.2397836617124085 ) ) ;
#11864=ADVANCED_FACE ( 'NONE', ( #14422 ), #27143, .T. ) ;
#11865=CARTESIAN_POINT ( 'NONE',  ( 115.0306645585770298, -38.52089976383655312, 146.4680903695919767 ) ) ;
#11866=CARTESIAN_POINT ( 'NONE',  ( 97.45308667932049218, -40.90817919144255654, 227.6527681330539679 ) ) ;
#11869=ORIENTED_EDGE ( 'NONE', *, *, #80273, .T. ) ;
#11872=ORIENTED_EDGE ( 'NONE', *, *, #2900, .F. ) ;
#11874=ORIENTED_EDGE ( 'NONE', *, *, #33000, .T. ) ;
#11876=DIRECTION ( 'NONE',  ( 0.000000000000000000, -1.000000000000000000, 0.000000000000000000 ) ) ;
#11877=ORIENTED_EDGE ( 'NONE', *, *, #84996, .T. ) ;
#11878=ORIENTED_EDGE ( 'NONE', *, *, #24199, .F. ) ;
#11879=CARTESIAN_POINT ( 'NONE',  ( 117.0290271953209498, -38.08751257484902908, 9.718958609244278790 ) ) ;
#11880=CARTESIAN_POINT ( 'NONE',  ( 57.56670390244816815, -42.82844715994040286, 295.7178068554150627 ) ) ;
#11882=CARTESIAN_POINT ( 'NONE',  ( 115.8611420101186269, -34.56920459637935750, 163.4286103042669822 ) ) ;
#11883=CARTESIAN_POINT ( 'NONE',  ( 97.44607596320715004, -32.59944340835617282, 16.00419670448194154 ) ) ;
#11884=CARTESIAN_POINT ( 'NONE',  ( 105.7978665782029282, -26.72425971154408941, 126.1774233227885276 ) ) ;
#11885=ADVANCED_FACE ( 'NONE', ( #36199 ), #62996, .T. ) ;
#11886=VERTEX_POINT ( 'NONE', #63913 ) ;
#11888=DIRECTION ( 'NONE',  ( 0.000000000000000000, 0.000000000000000000, 1.000000000000000000 ) ) ;
#11889=AXIS2_PLACEMENT_3D ( 'NONE', #160, #603, #28771 ) ;
#11890=VERTEX_POINT ( 'NONE', #70729 ) ;
#11893=ORIENTED_EDGE ( 'NONE', *, *, #52546, .F. ) ;
#11895=ADVANCED_FACE ( 'NONE', ( #8501 ), #41643, .F. ) ;
#11899=ORIENTED_EDGE ( 'NONE', *, *, #59314, .F. ) ;
#11900=CARTESIAN_POINT ( 'NONE',  ( 118.0989925035467252, -37.71898322177068508, 33.74324432352998571 ) ) ;
#11901=CARTESIAN_POINT ( 'NONE',  ( 117.3094150574360128, -38.89169797369248727, 59.66133956162595098 ) ) ;
#11904=DIRECTION ( 'NONE',  ( 0.000000000000000000, 0.000000000000000000, 1.000000000000000000 ) ) ;
#11905=LINE ( 'NONE', #53192, #69913 ) ;
#11910=CARTESIAN_POINT ( 'NONE',  ( 110.5699785786504918, -46.63284631861461804, 37.84705384733994293 ) ) ;
#11911=CARTESIAN_POINT ( 'NONE',  ( 95.40797249125856183, -38.85400393358575855, 197.4699109901969791 ) ) ;
#11912=CARTESIAN_POINT ( 'NONE',  ( 98.07812720205548374, -31.40528397058157850, 81.90133956162493689 ) ) ;
#11915=CARTESIAN_POINT ( 'NONE',  ( 134.0664832912740110, -8.350947159940998787, 308.6356252759119911 ) ) ;
#11917=CARTESIAN_POINT ( 'NONE',  ( 30.48091746481830100, -49.32844715994148288, 300.4678068554150059 ) ) ;
#11918=VERTEX_POINT ( 'NONE', #69378 ) ;
#11920=CARTESIAN_POINT ( 'NONE',  ( 102.0841886111852688, -27.63463957783716651, 96.46324432352997746 ) ) ;
#11923=CARTESIAN_POINT ( 'NONE',  ( 98.85650974919605005, -29.36329775763232774, 231.7565776568629587 ) ) ;
#11924=CARTESIAN_POINT ( 'NONE',  ( 117.0608242671911512, -38.08101263064929043, 254.7201668676480324 ) ) ;
#11926=CARTESIAN_POINT ( 'NONE',  ( 111.0139104026190182, -45.91774244734033061, 147.8993717799802994 ) ) ;
#11928=DIRECTION ( 'NONE',  ( -6.524622321627019585E-16, -3.741823817616790462E-31, -1.000000000000000000 ) ) ;
#11932=CARTESIAN_POINT ( 'NONE',  ( 117.1372161989437899, -34.25576096370539148, 164.0061014663879746 ) ) ;
#11933=ORIENTED_EDGE ( 'NONE', *, *, #78243, .T. ) ;
#11934=ORIENTED_EDGE ( 'NONE', *, *, #35199, .T. ) ;
#11935=AXIS2_PLACEMENT_3D ( 'NONE', #37166, #58052, #78963 ) ;
#11936=CARTESIAN_POINT ( 'NONE',  ( 99.74759560186635099, -41.77880479991928553, 123.2387261630399564 ) ) ;
#11937=CONICAL_SURFACE ( 'NONE', #61203, 1.624999999999987566, 1.029744258676650093 ) ;
#11938=DIRECTION ( 'NONE',  ( 4.194175870806139918E-14, -1.000000000000000000, 0.000000000000000000 ) ) ;
#11939=EDGE_CURVE ( 'NONE', #51458, #35086, #21688, .T. ) ;
#11940=CARTESIAN_POINT ( 'NONE',  ( 105.8561066403589308, -27.02385992090132305, 266.1756252759109884 ) ) ;
#11941=DIRECTION ( 'NONE',  ( 0.000000000000000000, -1.000000000000000000, 0.000000000000000000 ) ) ;
#11943=DIRECTION ( 'NONE',  ( 4.299999999999999979E-14, -1.000000000000000000, 0.000000000000000000 ) ) ;
#11947=EDGE_CURVE ( 'NONE', #30264, #2214, #84372, .T. ) ;
#11949=CARTESIAN_POINT ( 'NONE',  ( 97.81168895331838087, -40.51742574516882200, 287.6356252759109680 ) ) ;
#11951=CARTESIAN_POINT ( 'NONE',  ( 97.40233316251681117, -42.04621543282991780, 176.7146728949589658 ) ) ;
#11954=VERTEX_POINT ( 'NONE', #56168 ) ;
#11958=CARTESIAN_POINT ( 'NONE',  ( 80.81782300817755527, -21.40255221908232741, 8.160479982078024719 ) ) ;
#11959=LINE ( 'NONE', #67345, #66433 ) ;
#11960=CYLINDRICAL_SURFACE ( 'NONE', #58408, 2.117000000000000881 ) ;
#11961=ADVANCED_FACE ( 'NONE', ( #22143, #28027 ), #77537, .T. ) ;
#11962=CARTESIAN_POINT ( 'NONE',  ( 97.60805412390877223, -39.98290213189324049, 96.59010508770597880 ) ) ;
#11966=CARTESIAN_POINT ( 'NONE',  ( 96.13794759894150843, -35.07228238994858316, 221.1946728949589840 ) ) ;
#11967=DIRECTION ( 'NONE',  ( 0.7071067708032388044, 0.0001211784769831114530, 0.7071067811865423547 ) ) ;
#11968=ORIENTED_EDGE ( 'NONE', *, *, #24195, .T. ) ;
#11969=ORIENTED_EDGE ( 'NONE', *, *, #14623, .T. ) ;
#11970=VECTOR ( 'NONE', #72144, 1000.000000000000000 ) ;
#11972=CARTESIAN_POINT ( 'NONE',  ( 177.0371591254545933, -48.62818131005479927, 117.4678068554150485 ) ) ;
#11973=CARTESIAN_POINT ( 'NONE',  ( 101.9933085522700082, -45.44587970176321789, 167.1565046981921796 ) ) ;
#11974=EDGE_CURVE ( 'NONE', #49665, #21567, #65244, .T. ) ;
#11975=CARTESIAN_POINT ( 'NONE',  ( 101.8554017947406862, -30.44658510084856218, 38.44523322673398980 ) ) ;
#11976=CARTESIAN_POINT ( 'NONE',  ( 98.26250712568560175, -31.04002435091596368, 141.8699109901969564 ) ) ;
#11977=CARTESIAN_POINT ( 'NONE',  ( 118.5256205435843526, -36.72944715994100306, 293.2242906452868851 ) ) ;
#11978=EDGE_LOOP ( 'NONE', ( #56740, #68843, #7740, #72861 ) ) ;
#11979=CARTESIAN_POINT ( 'NONE',  ( 107.0664832912750057, -36.72944715993903486, 0.7256252759109708128 ) ) ;
#11983=AXIS2_PLACEMENT_3D ( 'NONE', #87924, #25690, #53368 ) ;
#11984=LINE ( 'NONE', #79699, #69156 ) ;
#11985=VERTEX_POINT ( 'NONE', #72515 ) ;
#11986=ORIENTED_EDGE ( 'NONE', *, *, #21379, .F. ) ;
#11988=CARTESIAN_POINT ( 'NONE',  ( 111.0503013157718044, -29.17396400730615369, 59.11241982807696616 ) ) ;
#11989=CARTESIAN_POINT ( 'NONE',  ( 117.4347420270075730, -35.18426962645584410, 218.9441967044829482 ) ) ;
#11990=CARTESIAN_POINT ( 'NONE',  ( 108.9412587213991088, -26.46057952311815953, 164.9327681330529742 ) ) ;
#11991=FACE_OUTER_BOUND ( 'NONE', #12760, .T. ) ;
#11992=CARTESIAN_POINT ( 'NONE',  ( 116.5819428025096585, -42.35350697836285860, 279.4137205140061724 ) ) ;
#11995=EDGE_LOOP ( 'NONE', ( #40838, #22846, #13113, #42994 ) ) ;
#11996=CIRCLE ( 'NONE', #83079, 0.2999999999999943823 ) ;
#11997=EDGE_CURVE ( 'NONE', #20780, #31941, #71624, .T. ) ;
#11998=VERTEX_POINT ( 'NONE', #46449 ) ;
#12000=AXIS2_PLACEMENT_3D ( 'NONE', #33769, #75106, #12895 ) ;
#12001=FACE_OUTER_BOUND ( 'NONE', #89138, .T. ) ;
#12002=CARTESIAN_POINT ( 'NONE',  ( 98.90817802506259682, -30.16829472858045591, 240.7870538473399620 ) ) ;
#12003=ORIENTED_EDGE ( 'NONE', *, *, #9830, .F. ) ;
#12004=CARTESIAN_POINT ( 'NONE',  ( 101.4252639664679094, -46.23501037223531540, 207.1622919425779514 ) ) ;
#12005=CYLINDRICAL_SURFACE ( 'NONE', #7957, 4.750000000000004441 ) ;
#12007=CYLINDRICAL_SURFACE ( 'NONE', #87054, 2.750000000000002665 ) ;
#12009=CARTESIAN_POINT ( 'NONE',  ( 109.2259222164322523, -28.99876954086582614, 277.6356252759110248 ) ) ;
#12011=DIRECTION ( 'NONE',  ( -0.1811243269278930978, 0.9834602067165288952, 0.000000000000000000 ) ) ;
#12013=CIRCLE ( 'NONE', #43891, 6.999999999999997335 ) ;
#12014=DIRECTION ( 'NONE',  ( -0.7071067812163264188, 0.7071067811567686157, -7.071067812163272297E-16 ) ) ;
#12015=DIRECTION ( 'NONE',  ( -0.0001211784769825758164, 0.7071067708032326982, 0.7071067811865484609 ) ) ;
#12017=CARTESIAN_POINT ( 'NONE',  ( 108.4174892589812487, -26.73503592869370493, 75.96895860870016293 ) ) ;
#12019=VERTEX_POINT ( 'NONE', #44333 ) ;
#12021=CARTESIAN_POINT ( 'NONE',  ( 116.5468340722667051, -41.20284764396129873, 228.4756252759109714 ) ) ;
#12022=CARTESIAN_POINT ( 'NONE',  ( 117.3387810265436144, -32.64853063025485369, 95.13943479972097350 ) ) ;
#12023=CARTESIAN_POINT ( 'NONE',  ( 113.2457357650714727, -45.17988020286173878, 224.0784824187679476 ) ) ;
#12027=CARTESIAN_POINT ( 'NONE',  ( 116.3212776292296127, -32.94146857471318413, 287.6356252759109680 ) ) ;
#12029=FACE_OUTER_BOUND ( 'NONE', #57904, .T. ) ;
#12030=ORIENTED_EDGE ( 'NONE', *, *, #53430, .T. ) ;
#12031=VERTEX_POINT ( 'NONE', #86144 ) ;
#12032=CARTESIAN_POINT ( 'NONE',  ( 108.4402549024021312, -27.77817906387560143, 144.3657531614099412 ) ) ;
#12036=CARTESIAN_POINT ( 'NONE',  ( 102.3703197837810848, -46.01248081495474906, 123.2041967044829818 ) ) ;
#12037=CARTESIAN_POINT ( 'NONE',  ( 105.7809510460201210, -24.27257308096163868, 321.6188579224977389 ) ) ;
#12038=CARTESIAN_POINT ( 'NONE',  ( 107.0664832912739968, -18.82844715994099971, 330.8831252759119934 ) ) ;
#12040=CARTESIAN_POINT ( 'NONE',  ( 117.0718954851608373, -35.46248235549226990, 109.9272919426389734 ) ) ;
#12041=CARTESIAN_POINT ( 'NONE',  ( 106.9359508110862720, -26.91635713860562973, 60.08705384733998045 ) ) ;
#12042=ORIENTED_EDGE ( 'NONE', *, *, #42488, .F. ) ;
#12043=ORIENTED_EDGE ( 'NONE', *, *, #2128, .T. ) ;
#12044=ORIENTED_EDGE ( 'NONE', *, *, #20064, .F. ) ;
#12045=CIRCLE ( 'NONE', #26494, 5.500000000000000888 ) ;
#12046=DIRECTION ( 'NONE',  ( -0.7071067811865175967, -0.7071067811865774377, -7.071067811865168663E-16 ) ) ;
#12047=CARTESIAN_POINT ( 'NONE',  ( 108.5509251780138129, -26.47246927008498929, 145.9737205140059473 ) ) ;
#12048=DIRECTION ( 'NONE',  ( 0.000000000000000000, -1.000000000000000000, 0.000000000000000000 ) ) ;
#12049=DIRECTION ( 'NONE',  ( 0.000000000000000000, 0.000000000000000000, 1.000000000000000000 ) ) ;
#12050=EDGE_CURVE ( 'NONE', #16560, #9081, #22583, .T. ) ;
#12053=LINE ( 'NONE', #12503, #6838 ) ;
#12054=EDGE_CURVE ( 'NONE', #68641, #88437, #34847, .T. ) ;
#12056=CARTESIAN_POINT ( 'NONE',  ( 98.30752360899535347, -41.72884965087872189, 177.7397897205293305 ) ) ;
#12057=CARTESIAN_POINT ( 'NONE',  ( 96.10063762778146668, -37.91858611869022866, 81.40038718067299328 ) ) ;
#12059=VERTEX_POINT ( 'NONE', #30280 ) ;
#12061=DIRECTION ( 'NONE',  ( 1.000000000000000078E-15, -1.000000000000000083E-30, -1.000000000000000000 ) ) ;
#12064=CARTESIAN_POINT ( 'NONE',  ( 112.6831787765100898, -43.31780159632685212, 150.9690427505439914 ) ) ;
#12065=ADVANCED_FACE ( 'NONE', ( #57973 ), #50712, .F. ) ;
#12066=VECTOR ( 'NONE', #21275, 1000.000000000000114 ) ;
#12067=CONICAL_SURFACE ( 'NONE', #19326, 17.00000000000090239, 0.7853981633974447263 ) ;
#12068=EDGE_CURVE ( 'NONE', #85068, #27190, #23036, .T. ) ;
#12069=VECTOR ( 'NONE', #62899, 1000.000000000000000 ) ;
#12070=FACE_OUTER_BOUND ( 'NONE', #40045, .T. ) ;
#12072=ORIENTED_EDGE ( 'NONE', *, *, #78047, .F. ) ;
#12077=ADVANCED_FACE ( 'NONE', ( #6927 ), #20569, .T. ) ;
#12078=CARTESIAN_POINT ( 'NONE',  ( 97.15642216441104040, -38.53537999780244405, 197.9015833058969633 ) ) ;
#12080=CARTESIAN_POINT ( 'NONE',  ( 61.56670390244634916, -23.42844715994043270, 180.4678068554151196 ) ) ;
#12081=LINE ( 'NONE', #67479, #16942 ) ;
#12083=ORIENTED_EDGE ( 'NONE', *, *, #16178, .F. ) ;
#12084=AXIS2_PLACEMENT_3D ( 'NONE', #85890, #58160, #58589 ) ;
#12085=ORIENTED_EDGE ( 'NONE', *, *, #68062, .T. ) ;
#12086=ORIENTED_EDGE ( 'NONE', *, *, #47690, .T. ) ;
#12087=CARTESIAN_POINT ( 'NONE',  ( 102.5467118750096631, -28.62589253813684209, 253.2995189410198691 ) ) ;
#12089=CARTESIAN_POINT ( 'NONE',  ( 101.7446525173404979, -27.01484174591878329, 100.4632443235299633 ) ) ;
#12090=CARTESIAN_POINT ( 'NONE',  ( 97.30890135812528285, -33.12136451854834007, 66.04419670448297097 ) ) ;
#12091=CARTESIAN_POINT ( 'NONE',  ( 109.3549997033752277, -28.03260486696533249, 249.5838068554168387 ) ) ;
#12092=CARTESIAN_POINT ( 'NONE',  ( 131.5565945955649170, -17.60518703965928466, 7.068229416970669199 ) ) ;
#12093=CARTESIAN_POINT ( 'NONE',  ( 51.03742451361726751, -23.42844715994066362, 237.4678068554150059 ) ) ;
#12094=CARTESIAN_POINT ( 'NONE',  ( 113.0221554258835823, -45.32894145911351558, 199.0584824187679374 ) ) ;
#12098=ORIENTED_EDGE ( 'NONE', *, *, #82021, .T. ) ;
#12100=CARTESIAN_POINT ( 'NONE',  ( 31.71315051185382572, -33.70561438052049397, 117.4678068554150485 ) ) ;
#12101=EDGE_CURVE ( 'NONE', #73956, #6135, #34628, .T. ) ;
#12102=ORIENTED_EDGE ( 'NONE', *, *, #54447, .T. ) ;
#12105=CARTESIAN_POINT ( 'NONE',  ( 116.8171228671177175, -34.15291832207935130, 179.0314586091353704 ) ) ;
#12106=CARTESIAN_POINT ( 'NONE',  ( 117.3536837868190332, -38.62665896660388398, 88.68133956162493803 ) ) ;
#12107=DIRECTION ( 'NONE',  ( 1.000000000000000000, 0.000000000000000000, 0.000000000000000000 ) ) ;
#12108=DIRECTION ( 'NONE',  ( 0.7071067811864671926, 0.7071067811866279529, 6.612322855854137577E-17 ) ) ;
#12109=CARTESIAN_POINT ( 'NONE',  ( 97.81170008160388818, -40.51743097690945916, 72.63551179937353197 ) ) ;
#12111=CARTESIAN_POINT ( 'NONE',  ( 97.81997189479284316, -40.53760914905940638, 56.63694704664123947 ) ) ;
#12112=CARTESIAN_POINT ( 'NONE',  ( 116.3308458273175603, -44.07926308385594183, 194.2927681330539542 ) ) ;
#12113=DIRECTION ( 'NONE',  ( -1.000000000000000000, 0.000000000000000000, 0.000000000000000000 ) ) ;
#12114=CARTESIAN_POINT ( 'NONE',  ( 37.06648329127298780, 12.92155284005730387, 358.9756252759109998 ) ) ;
#12116=FACE_OUTER_BOUND ( 'NONE', #72440, .T. ) ;
#12118=CARTESIAN_POINT ( 'NONE',  ( 97.06386167369745976, -37.34267883451605030, 136.3754845998514043 ) ) ;
#12119=CARTESIAN_POINT ( 'NONE',  ( 156.5667039024483813, -48.82844715993569196, 254.7178068554149490 ) ) ;
#12121=CARTESIAN_POINT ( 'NONE',  ( 103.9260401568723324, -26.74224119611745820, 250.3184824187677577 ) ) ;
#12124=CARTESIAN_POINT ( 'NONE',  ( 97.19620376612084556, -33.30704266974938577, 282.0613395616252888 ) ) ;
#12125=CARTESIAN_POINT ( 'NONE',  ( 116.9452694852055998, -40.19391870447465465, 129.5584824187679658 ) ) ;
#12126=FACE_OUTER_BOUND ( 'NONE', #72113, .T. ) ;
#12128=CARTESIAN_POINT ( 'NONE',  ( 182.2300522401149863, -33.89581943344511217, -5.074374724088000832 ) ) ;
#12129=CARTESIAN_POINT ( 'NONE',  ( 182.6664832912729821, 12.92155284005730387, 355.9756252759109998 ) ) ;
#12130=DIRECTION ( 'NONE',  ( 0.000000000000000000, 1.000000000000000000, 0.000000000000000000 ) ) ;
#12131=CARTESIAN_POINT ( 'NONE',  ( 63.03715912545825262, -46.82818131006018803, 237.4678068554150059 ) ) ;
#12133=VECTOR ( 'NONE', #57575, 1000.000000000000000 ) ;
#12136=AXIS2_PLACEMENT_3D ( 'NONE', #69080, #33212, #69529 ) ;
#12141=CARTESIAN_POINT ( 'NONE',  ( 102.7643194828038702, -25.71402177940534983, 16.37276813305293999 ) ) ;
#12142=DIRECTION ( 'NONE',  ( -0.9254794337955620787, -0.3787978585227822492, 0.000000000000000000 ) ) ;
#12143=DIRECTION ( 'NONE',  ( 0.000000000000000000, -1.000000000000000000, 0.000000000000000000 ) ) ;
#12146=LINE ( 'NONE', #5334, #71870 ) ;
#12147=CARTESIAN_POINT ( 'NONE',  ( 101.9719466847405158, -43.62131184885326007, 256.4924198280769474 ) ) ;
#12151=VECTOR ( 'NONE', #60867, 1000.000000000000000 ) ;
#12152=CARTESIAN_POINT ( 'NONE',  ( 107.0664832912730020, -27.87844715994269862, 361.9756252759109998 ) ) ;
#12154=CARTESIAN_POINT ( 'NONE',  ( 115.0687214047011366, -42.78184030945386951, 183.3110242557596905 ) ) ;
#12155=CARTESIAN_POINT ( 'NONE',  ( 141.0667039024479834, -50.82844715994100682, 10.91780685541499807 ) ) ;
#12157=EDGE_CURVE ( 'NONE', #46735, #52987, #76073, .T. ) ;
#12158=CARTESIAN_POINT ( 'NONE',  ( 116.8454820155364331, -34.32316206775963963, 10.45015473446897403 ) ) ;
#12159=EDGE_CURVE ( 'NONE', #65845, #39861, #31068, .T. ) ;
#12163=FACE_OUTER_BOUND ( 'NONE', #78167, .T. ) ;
#12164=CARTESIAN_POINT ( 'NONE',  ( 110.7503262618283344, -45.78994064700705735, 282.8841967044829744 ) ) ;
#12167=EDGE_CURVE ( 'NONE', #49816, #17557, #76416, .T. ) ;
#12168=DIRECTION ( 'NONE',  ( 0.000000000000000000, 1.000000000000000000, 0.000000000000000000 ) ) ;
#12170=FACE_OUTER_BOUND ( 'NONE', #45567, .T. ) ;
#12171=CARTESIAN_POINT ( 'NONE',  ( 110.8736562448416549, -29.50897902285196039, 57.50809036959092424 ) ) ;
#12172=EDGE_CURVE ( 'NONE', #11460, #68161, #81908, .T. ) ;
#12173=CARTESIAN_POINT ( 'NONE',  ( 136.7838203269376152, -18.30343833344100801, 6.798133076499780714 ) ) ;
#12174=CARTESIAN_POINT ( 'NONE',  ( 106.5656518807525117, -24.23945688555024702, 323.2548426863285727 ) ) ;
#12176=LINE ( 'NONE', #81679, #22796 ) ;
#12177=ORIENTED_EDGE ( 'NONE', *, *, #66313, .F. ) ;
#12178=DIRECTION ( 'NONE',  ( 1.000000000000000078E-15, -1.000000000000000083E-30, -1.000000000000000000 ) ) ;
#12181=CARTESIAN_POINT ( 'NONE',  ( 117.6081704542122282, -33.40500446796587397, 129.0575300378159795 ) ) ;
#12183=CARTESIAN_POINT ( 'NONE',  ( 109.2109342822782168, -45.52796977871753370, 87.17718173283900285 ) ) ;
#12185=CARTESIAN_POINT ( 'NONE',  ( 112.8380968919016425, -43.45378765227984275, 104.5730118773259534 ) ) ;
#12186=LINE ( 'NONE', #39870, #37338 ) ;
#12187=CYLINDRICAL_SURFACE ( 'NONE', #15032, 9.999999999999998224 ) ;
#12188=CARTESIAN_POINT ( 'NONE',  ( 106.8407189164991706, -48.60257990303799858, 73.56133956162497611 ) ) ;
#12189=CARTESIAN_POINT ( 'NONE',  ( 152.4409905591762708, -0.9151414768251351362, 542.9756252759101471 ) ) ;
#12191=CARTESIAN_POINT ( 'NONE',  ( 154.4439038579832300, -17.91479848270203945, 542.9756252759101471 ) ) ;
#12193=CARTESIAN_POINT ( 'NONE',  ( 123.6837132603318707, -20.11243780205705534, 218.8274735512161158 ) ) ;
#12194=VECTOR ( 'NONE', #28283, 1000.000000000000000 ) ;
#12195=VERTEX_POINT ( 'NONE', #88277 ) ;
#12198=ORIENTED_EDGE ( 'NONE', *, *, #41724, .T. ) ;
#12199=CARTESIAN_POINT ( 'NONE',  ( 117.4008144674645280, -32.62901037329574905, 249.1270538473399654 ) ) ;
#12200=CARTESIAN_POINT ( 'NONE',  ( 116.9247085916874909, -40.18670803819183845, 129.5584824187679658 ) ) ;
#12203=CARTESIAN_POINT ( 'NONE',  ( 116.5983126044778402, -29.68822244385183140, 105.3327681330539463 ) ) ;
#12204=CARTESIAN_POINT ( 'NONE',  ( 116.3244028009478797, -32.94573790848593120, 95.13562527591096796 ) ) ;
#12206=CARTESIAN_POINT ( 'NONE',  ( 151.0371591254572934, -24.42818131005592974, 300.4678068554149490 ) ) ;
#12207=CYLINDRICAL_SURFACE ( 'NONE', #86870, 16.00000000000000000 ) ;
#12208=ADVANCED_FACE ( 'NONE', ( #5136 ), #40991, .T. ) ;
#12209=ORIENTED_EDGE ( 'NONE', *, *, #39509, .T. ) ;
#12210=VECTOR ( 'NONE', #21464, 1000.000000000000000 ) ;
#12211=CARTESIAN_POINT ( 'NONE',  ( 83.73314995794051185, 12.92155284005802685, 334.6228282640713019 ) ) ;
#12212=CIRCLE ( 'NONE', #7865, 2.517499999999998739 ) ;
#12213=DIRECTION ( 'NONE',  ( 0.000000000000000000, 0.000000000000000000, -1.000000000000000000 ) ) ;
#12214=CARTESIAN_POINT ( 'NONE',  ( 115.6373213143784398, -30.77082676042341802, 279.3099109901966131 ) ) ;
#12216=VECTOR ( 'NONE', #35329, 1000.000000000000000 ) ;
#12217=DIRECTION ( 'NONE',  ( -0.000000000000000000, -0.000000000000000000, 1.000000000000000000 ) ) ;
#12218=CARTESIAN_POINT ( 'NONE',  ( 78.42773927736698170, -38.94013506380486689, 2.060080721665560777 ) ) ;
#12219=CARTESIAN_POINT ( 'NONE',  ( 109.4611421171680945, -28.53056059958231216, 259.2724198280769770 ) ) ;
#12220=CARTESIAN_POINT ( 'NONE',  ( 97.63926207416247394, -40.07016425843875140, 101.5979595511756628 ) ) ;
#12221=CARTESIAN_POINT ( 'NONE',  ( 107.8666756518570793, -26.35696637107995954, 66.01562527591097762 ) ) ;
#12222=DIRECTION ( 'NONE',  ( -4.237773401492740281E-14, 1.000000000000000000, 0.000000000000000000 ) ) ;
#12223=CARTESIAN_POINT ( 'NONE',  ( 117.5013794172148351, -40.51439451343497922, 173.5375300378159693 ) ) ;
#12224=ORIENTED_EDGE ( 'NONE', *, *, #89028, .F. ) ;
#12228=CIRCLE ( 'NONE', #15145, 14.00000000000000888 ) ;
#12229=DIRECTION ( 'NONE',  ( -0.7071067811865453523, -0.7071067811865496822, -7.071067811865460542E-16 ) ) ;
#12230=LINE ( 'NONE', #66278, #55723 ) ;
#12231=VERTEX_POINT ( 'NONE', #6477 ) ;
#12232=DIRECTION ( 'NONE',  ( 0.000000000000000000, 0.000000000000000000, 1.000000000000000000 ) ) ;
#12233=CARTESIAN_POINT ( 'NONE',  ( 117.0754465142714054, -30.29129860725820222, 144.2813395616249750 ) ) ;
#12234=EDGE_LOOP ( 'NONE', ( #65295, #76282, #6766, #32383 ) ) ;
#12235=CARTESIAN_POINT ( 'NONE',  ( 194.5664832912739826, -18.82844715994099971, 342.9256252759119548 ) ) ;
#12237=DIRECTION ( 'NONE',  ( -1.000000000000000000, -4.510281037539694659E-14, 0.000000000000000000 ) ) ;
#12238=CARTESIAN_POINT ( 'NONE',  ( 41.56670390244801894, -27.57844715994070484, 342.9256252759119548 ) ) ;
#12240=EDGE_CURVE ( 'NONE', #27718, #23732, #74622, .T. ) ;
#12241=DIRECTION ( 'NONE',  ( 1.000000000000000078E-15, -1.000000000000000083E-30, -1.000000000000000000 ) ) ;
#12242=CARTESIAN_POINT ( 'NONE',  ( 20.03715912545645850, -24.95799193693202156, 129.9678068554150627 ) ) ;
#12243=EDGE_LOOP ( 'NONE', ( #30978, #73389, #51941, #22929 ) ) ;
#12247=CARTESIAN_POINT ( 'NONE',  ( 115.0372574787901954, -42.90846260359005271, 158.3022919389477465 ) ) ;
#12248=DIRECTION ( 'NONE',  ( 1.907762142705490052E-15, 7.167082501179359715E-16, -1.000000000000000000 ) ) ;
#12250=CARTESIAN_POINT ( 'NONE',  ( 107.0664832912739968, -36.72944715994100306, 287.6356252759109680 ) ) ;
#12252=CIRCLE ( 'NONE', #16613, 1.000000000002049694 ) ;
#12253=ORIENTED_EDGE ( 'NONE', *, *, #82128, .T. ) ;
#12255=CARTESIAN_POINT ( 'NONE',  ( 63.56670390244828184, -47.82844715994016127, 249.9678068554150343 ) ) ;
#12256=CARTESIAN_POINT ( 'NONE',  ( 101.7025241355417364, -45.60450926735014576, 198.1318157521009482 ) ) ;
#12257=EDGE_CURVE ( 'NONE', #34233, #17736, #67809, .T. ) ;
#12259=ORIENTED_EDGE ( 'NONE', *, *, #71760, .T. ) ;
#12260=CARTESIAN_POINT ( 'NONE',  ( 118.0115280580377402, -34.77548253539075063, 44.96705384733895272 ) ) ;
#12262=CARTESIAN_POINT ( 'NONE',  ( 116.3183049785035195, -32.94379174720932468, 54.13562527591098217 ) ) ;
#12263=EDGE_CURVE ( 'NONE', #79263, #26148, #68270, .T. ) ;
#12266=EDGE_LOOP ( 'NONE', ( #62571, #70882, #85295, #36284 ) ) ;
#12268=ADVANCED_FACE ( 'NONE', ( #56404 ), #35977, .T. ) ;
#12270=ORIENTED_EDGE ( 'NONE', *, *, #35385, .F. ) ;
#12271=CARTESIAN_POINT ( 'NONE',  ( 113.4748355983601300, -30.60888351595189860, 230.8644404487539816 ) ) ;
#12272=AXIS2_PLACEMENT_3D ( 'NONE', #63888, #16188, #57947 ) ;
#12274=VECTOR ( 'NONE', #30568, 1000.000000000000000 ) ;
#12277=AXIS2_PLACEMENT_3D ( 'NONE', #47943, #41139, #34331 ) ;
#12279=EDGE_CURVE ( 'NONE', #28336, #84782, #29611, .T. ) ;
#12280=CARTESIAN_POINT ( 'NONE',  ( 82.67340060512941591, -37.60624470235564587, 2.902100967938844089 ) ) ;
#12281=AXIS2_PLACEMENT_3D ( 'NONE', #29659, #76015, #20613 ) ;
#12284=AXIS2_PLACEMENT_3D ( 'NONE', #2336, #51343, #10477 ) ;
#12285=CARTESIAN_POINT ( 'NONE',  ( 97.12568611773902205, -37.99775231544951737, 37.42709075889258941 ) ) ;
#12286=EDGE_CURVE ( 'NONE', #53177, #87561, #62776, .T. ) ;
#12287=ORIENTED_EDGE ( 'NONE', *, *, #45300, .T. ) ;
#12288=CARTESIAN_POINT ( 'NONE',  ( 110.9847977634196496, -46.36662828626499078, 282.8841967044824628 ) ) ;
#12289=EDGE_LOOP ( 'NONE', ( #11299, #81159 ) ) ;
#12290=ORIENTED_EDGE ( 'NONE', *, *, #20468, .T. ) ;
#12291=CARTESIAN_POINT ( 'NONE',  ( 111.4490224358278994, -43.61588866942526721, 260.8452332267341376 ) ) ;
#12293=CARTESIAN_POINT ( 'NONE',  ( 108.8290724220007348, -27.07506712556656936, 164.9327681330539690 ) ) ;
#12295=CARTESIAN_POINT ( 'NONE',  ( 20.03715912545730760, -24.42818131006189830, 300.4678068554150059 ) ) ;
#12296=CARTESIAN_POINT ( 'NONE',  ( 73.06670390244801183, -48.82844715994099971, 179.9178068554149661 ) ) ;
#12297=CARTESIAN_POINT ( 'NONE',  ( 96.73312529990856490, -40.78150971882554643, 242.6118157521009664 ) ) ;
#12298=CYLINDRICAL_SURFACE ( 'NONE', #63032, 5.599999999999994316 ) ;
#12299=ORIENTED_EDGE ( 'NONE', *, *, #83569, .F. ) ;
#12300=CARTESIAN_POINT ( 'NONE',  ( 109.7813809329710040, -47.49173451690833048, 88.78514908543493789 ) ) ;
#12301=CARTESIAN_POINT ( 'NONE',  ( 48.79742451362097455, -36.32844715994040996, 342.9256252759109884 ) ) ;
#12302=ORIENTED_EDGE ( 'NONE', *, *, #14734, .F. ) ;
#12303=AXIS2_PLACEMENT_3D ( 'NONE', #77815, #49180, #64185 ) ;
#12305=ORIENTED_EDGE ( 'NONE', *, *, #20066, .F. ) ;
#12306=CARTESIAN_POINT ( 'NONE',  ( 177.8371591254542921, -47.82818131005477369, 313.9678068554149490 ) ) ;
#12308=CARTESIAN_POINT ( 'NONE',  ( 98.30745628127105817, -41.72868722923796270, 151.7403413731134663 ) ) ;
#12309=CARTESIAN_POINT ( 'NONE',  ( 103.1635642379172850, -29.56027560196853088, 143.2909475124489518 ) ) ;
#12310=CARTESIAN_POINT ( 'NONE',  ( 116.9459113946819286, -41.73765103896904805, 244.4651490854349731 ) ) ;
#12312=EDGE_LOOP ( 'NONE', ( #52481, #68052, #68784 ) ) ;
#12313=CARTESIAN_POINT ( 'NONE',  ( 107.0664832912739541, -23.56278049327425350, 311.6356252759109680 ) ) ;
#12315=EDGE_CURVE ( 'NONE', #43956, #18807, #1471, .T. ) ;
#12316=EDGE_LOOP ( 'NONE', ( #88395, #50327, #75661, #33760 ) ) ;
#12319=CARTESIAN_POINT ( 'NONE',  ( 31.89136050872134476, -31.76306994223885383, 193.9678068554150911 ) ) ;
#12320=ORIENTED_EDGE ( 'NONE', *, *, #18118, .F. ) ;
#12321=ORIENTED_EDGE ( 'NONE', *, *, #11997, .T. ) ;
#12324=PLANE ( 'NONE',  #777 ) ;
#12326=PLANE ( 'NONE',  #43177 ) ;
#12327=CARTESIAN_POINT ( 'NONE',  ( 111.7477409549918690, -43.87381266066567775, 177.4609912566479579 ) ) ;
#12328=CARTESIAN_POINT ( 'NONE',  ( 101.9388778781502509, -27.60177885026046596, 60.48419670448296159 ) ) ;
#12330=ORIENTED_EDGE ( 'NONE', *, *, #72769, .T. ) ;
#12331=DIRECTION ( 'NONE',  ( 0.7071067811868666508, 0.7071067811862283836, 7.071067811868659373E-16 ) ) ;
#12333=FACE_OUTER_BOUND ( 'NONE', #80855, .T. ) ;
#12334=EDGE_LOOP ( 'NONE', ( #87606, #70527, #72973, #8282 ) ) ;
#12335=CARTESIAN_POINT ( 'NONE',  ( 107.0222341398176127, -26.64422208933962821, 166.0788337594356676 ) ) ;
#12337=CARTESIAN_POINT ( 'NONE',  ( 113.2919313540066071, -44.57100634757310331, 133.1104735366473903 ) ) ;
#12339=VECTOR ( 'NONE', #22785, 1000.000000000000000 ) ;
#12340=VERTEX_POINT ( 'NONE', #78235 ) ;
#12341=EDGE_CURVE ( 'NONE', #22595, #36659, #35067, .T. ) ;
#12342=CARTESIAN_POINT ( 'NONE',  ( 116.1397716810727303, -31.55208187140975795, 289.2384824187681716 ) ) ;
#12343=AXIS2_PLACEMENT_3D ( 'NONE', #30024, #44073, #16397 ) ;
#12344=CARTESIAN_POINT ( 'NONE',  ( 101.1162363742629253, -27.35970543535582422, 61.51467289495899138 ) ) ;
#12345=VECTOR ( 'NONE', #38394, 1000.000000000000000 ) ;
#12347=AXIS2_PLACEMENT_3D ( 'NONE', #6829, #34071, #34532 ) ;
#12348=CARTESIAN_POINT ( 'NONE',  ( 134.0664832912740110, -8.350947159940998787, 2.408125275911999097 ) ) ;
#12349=LINE ( 'NONE', #40038, #38466 ) ;
#12350=DIRECTION ( 'NONE',  ( 1.000000000000000078E-15, 1.000000000000000083E-30, -1.000000000000000000 ) ) ;
#12351=FACE_OUTER_BOUND ( 'NONE', #1558, .T. ) ;
#12356=CARTESIAN_POINT ( 'NONE',  ( 114.8522965031571630, -43.72857415363870359, 38.24419670448192221 ) ) ;
#12357=CARTESIAN_POINT ( 'NONE',  ( 113.4285887376619968, -27.66253919562607422, 80.57753003781597556 ) ) ;
#12365=CARTESIAN_POINT ( 'NONE',  ( 108.2420053567034017, -46.43931755893575541, 113.6727681330529691 ) ) ;
#12368=CARTESIAN_POINT ( 'NONE',  ( 112.4005920293389948, -46.38403708128146974, 248.9661014663869878 ) ) ;
#12370=FACE_BOUND ( 'NONE', #26881, .T. ) ;
#12371=DIRECTION ( 'NONE',  ( 1.000000000000000000, 0.000000000000000000, 0.000000000000000000 ) ) ;
#12372=ADVANCED_FACE ( 'NONE', ( #7822 ), #28719, .F. ) ;
#12373=DIRECTION ( 'NONE',  ( 0.000000000000000000, 1.000000000000000000, 0.000000000000000000 ) ) ;
#12374=CARTESIAN_POINT ( 'NONE',  ( 131.5359215223105309, -37.80596063775243465, 2.807537029280252838 ) ) ;
#12376=CARTESIAN_POINT ( 'NONE',  ( 99.36405074150913208, -30.70139697576582805, 155.7984824187689412 ) ) ;
#12380=CARTESIAN_POINT ( 'NONE',  ( 99.34829255622855726, -41.08350393070648465, 133.1672975916119697 ) ) ;
#12382=CARTESIAN_POINT ( 'NONE',  ( 115.4101910119109533, -30.57141770992062035, 255.3203871806724123 ) ) ;
#12383=CARTESIAN_POINT ( 'NONE',  ( 165.2748236753145932, -30.08671355699731720, 237.4678068554150059 ) ) ;
#12385=LINE ( 'NONE', #40078, #39151 ) ;
#12386=FACE_OUTER_BOUND ( 'NONE', #674, .T. ) ;
#12387=EDGE_CURVE ( 'NONE', #46735, #72562, #64139, .T. ) ;
#12389=DIRECTION ( 'NONE',  ( 1.000000000000000000, 0.000000000000000000, 9.462128050782575008E-16 ) ) ;
#12390=DIRECTION ( 'NONE',  ( -1.000000000000000078E-15, 1.000000000000000083E-30, 1.000000000000000000 ) ) ;
#12391=EDGE_CURVE ( 'NONE', #18839, #6555, #56855, .T. ) ;
#12392=CARTESIAN_POINT ( 'NONE',  ( 107.9164806882189396, -47.13338536194959971, 177.6413395616249886 ) ) ;
#12393=PLANE ( 'NONE',  #44562 ) ;
#12395=ORIENTED_EDGE ( 'NONE', *, *, #80768, .F. ) ;
#12396=CARTESIAN_POINT ( 'NONE',  ( 31.78666935232957869, -29.62846900982343001, 237.4678068554150059 ) ) ;
#12397=CARTESIAN_POINT ( 'NONE',  ( 82.59390026529925422, -19.81452881270899269, 7.047625865520877220 ) ) ;
#12400=CARTESIAN_POINT ( 'NONE',  ( 116.3212776292296127, -32.94146857471318413, 287.6356252759109680 ) ) ;
#12401=ORIENTED_EDGE ( 'NONE', *, *, #1084, .T. ) ;
#12405=AXIS2_PLACEMENT_3D ( 'NONE', #53458, #5350, #52562 ) ;
#12406=CARTESIAN_POINT ( 'NONE',  ( 113.1555140577670215, -26.56262906569767068, 204.6470538473399756 ) ) ;
#12407=DIRECTION ( 'NONE',  ( -1.000000000000000000, 0.000000000000000000, 0.000000000000000000 ) ) ;
#12408=ORIENTED_EDGE ( 'NONE', *, *, #19175, .F. ) ;
#12409=CONICAL_SURFACE ( 'NONE', #58821, 9.571100913904478702, 0.7853981633974539411 ) ;
#12413=CARTESIAN_POINT ( 'NONE',  ( 110.2473415405206083, -44.77823998140315354, 20.70618560768600247 ) ) ;
#12414=CARTESIAN_POINT ( 'NONE',  ( 95.65143945485090171, -33.45545561978638460, 137.1041967044819501 ) ) ;
#12415=VECTOR ( 'NONE', #88569, 1000.000000000000000 ) ;
#12417=ORIENTED_EDGE ( 'NONE', *, *, #84066, .F. ) ;
#12419=CARTESIAN_POINT ( 'NONE',  ( 172.5664832912729878, -27.82844715994070484, 14.17562527591199917 ) ) ;
#12420=CARTESIAN_POINT ( 'NONE',  ( 82.58878920443973470, -17.63370978841311754, 7.053538376721526504 ) ) ;
#12425=ORIENTED_EDGE ( 'NONE', *, *, #79443, .T. ) ;
#12427=EDGE_CURVE ( 'NONE', #65668, #62636, #70966, .T. ) ;
#12428=CARTESIAN_POINT ( 'NONE',  ( 115.2492312947614437, -32.84933048162275071, 63.61337220902895950 ) ) ;
#12429=CARTESIAN_POINT ( 'NONE',  ( 96.62214413241265731, -36.48016117738031738, 196.3070538473399438 ) ) ;
#12430=CARTESIAN_POINT ( 'NONE',  ( 114.9485010938853975, -29.93956786141545834, 184.3927681330539770 ) ) ;
#12431=CARTESIAN_POINT ( 'NONE',  ( 97.82822030858592655, -40.55762851625022591, 21.63876279231929445 ) ) ;
#12432=CARTESIAN_POINT ( 'NONE',  ( 97.12559377168382468, -39.79659400623918231, 17.56419670448195092 ) ) ;
#12437=ORIENTED_EDGE ( 'NONE', *, *, #60849, .T. ) ;
#12441=CARTESIAN_POINT ( 'NONE',  ( 103.8060002238608774, -48.17488501466909412, 217.3556252759109668 ) ) ;
#12444=CARTESIAN_POINT ( 'NONE',  ( 103.7231215738078163, -26.19374500585225363, 205.3089586092439731 ) ) ;
#12448=CARTESIAN_POINT ( 'NONE',  ( 109.6421639904622936, -46.48030490558162597, 23.78138826461756139 ) ) ;
#12449=CARTESIAN_POINT ( 'NONE',  ( 151.0371591254583450, -46.82818131005583240, 300.4678068554149490 ) ) ;
#12451=CARTESIAN_POINT ( 'NONE',  ( 98.10142885082893827, -36.98438604582442224, 277.6356252759110816 ) ) ;
#12452=DIRECTION ( 'NONE',  ( 0.000000000000000000, 0.000000000000000000, 1.000000000000000000 ) ) ;
#12453=CARTESIAN_POINT ( 'NONE',  ( 98.54766419607773287, -41.97700047869818718, 172.7658057784116750 ) ) ;
#12455=DIRECTION ( 'NONE',  ( -1.000000000000000078E-15, 1.000000000000000083E-30, 1.000000000000000000 ) ) ;
#12458=FACE_OUTER_BOUND ( 'NONE', #84785, .T. ) ;
#12465=CARTESIAN_POINT ( 'NONE',  ( 118.0640922190486890, -35.40731289736847032, 238.9337205140059552 ) ) ;
#12466=CARTESIAN_POINT ( 'NONE',  ( 112.8017646537355176, -47.09965271489118521, 98.97848241876793907 ) ) ;
#12467=CARTESIAN_POINT ( 'NONE',  ( 111.7585843298372197, -27.37117935058896379, 275.7070538473396937 ) ) ;
#12468=DIRECTION ( 'NONE',  ( -1.058811598242755461E-16, 0.5150380749100580413, -0.8571673007021100021 ) ) ;
#12471=DIRECTION ( 'NONE',  ( 0.000000000000000000, 0.000000000000000000, 1.000000000000000000 ) ) ;
#12472=DIRECTION ( 'NONE',  ( -0.1041461484700691442, 0.008931931031208454816, 0.9945218953682739560 ) ) ;
#12474=CARTESIAN_POINT ( 'NONE',  ( 132.8008218761707724, -21.17731672736086423, 1.873071027759226626 ) ) ;
#12475=AXIS2_PLACEMENT_3D ( 'NONE', #33834, #4794, #61525 ) ;
#12478=AXIS2_PLACEMENT_3D ( 'NONE', #47334, #73718, #32363 ) ;
#12481=VERTEX_POINT ( 'NONE', #80450 ) ;
#12482=CARTESIAN_POINT ( 'NONE',  ( 99.86829443779211601, -32.07773762820211516, 145.2924198280769872 ) ) ;
#12484=EDGE_LOOP ( 'NONE', ( #29628, #23889, #41178, #51518, #74712, #88733, #35280, #62937 ) ) ;
#12485=DIRECTION ( 'NONE',  ( 0.9068632946707808618, -0.4214249218767877059, 0.000000000000000000 ) ) ;
#12486=CARTESIAN_POINT ( 'NONE',  ( 97.76587557681025942, -42.65924729906315349, 137.7661014663869992 ) ) ;
#12487=CARTESIAN_POINT ( 'NONE',  ( 151.0371591254576060, -24.95799193692592155, 129.9678068554149775 ) ) ;
#12489=PLANE ( 'NONE',  #3724 ) ;
#12492=CIRCLE ( 'NONE', #85062, 13.44999999999999396 ) ;
#12493=CARTESIAN_POINT ( 'NONE',  ( 97.30000116515907393, -37.25789978020652882, 76.36991099019796536 ) ) ;
#12495=EDGE_LOOP ( 'NONE', ( #81947, #78584, #62352, #51503 ) ) ;
#12497=CARTESIAN_POINT ( 'NONE',  ( 22.49563609058251146, -48.82844715994099971, 307.9888746672805269 ) ) ;
#12498=CARTESIAN_POINT ( 'NONE',  ( 97.26456095925938428, -36.24355304347524509, 167.2870538473389672 ) ) ;
#12499=DIRECTION ( 'NONE',  ( -1.000000000000000000, 8.775353200852647323E-16, 0.000000000000000000 ) ) ;
#12500=AXIS2_PLACEMENT_3D ( 'NONE', #56130, #28913, #16619 ) ;
#12503=CARTESIAN_POINT ( 'NONE',  ( 49.56670390244799762, -50.82844715994100682, 310.9178068554150514 ) ) ;
#12505=DIRECTION ( 'NONE',  ( 0.000000000000000000, 0.000000000000000000, -1.000000000000000000 ) ) ;
#12506=DIRECTION ( 'NONE',  ( -1.000000000000000000, 0.000000000000000000, 0.000000000000000000 ) ) ;
#12507=EDGE_CURVE ( 'NONE', #44520, #38912, #45889, .T. ) ;
#12508=CARTESIAN_POINT ( 'NONE',  ( 103.3702027031294506, -47.12181610991865455, 102.3165776568629752 ) ) ;
#12512=DIRECTION ( 'NONE',  ( -0.9254794337955620787, -0.3787978585227822492, 0.000000000000000000 ) ) ;
#12515=CARTESIAN_POINT ( 'NONE',  ( 31.89136050872298966, -31.76306994223740432, -5.074374724088000832 ) ) ;
#12516=CARTESIAN_POINT ( 'NONE',  ( 114.6928066196564515, -42.01481596195104373, 161.1623760838769783 ) ) ;
#12517=CARTESIAN_POINT ( 'NONE',  ( 20.56670390244743984, -48.82844715994200158, 180.4678068554150911 ) ) ;
#12518=VERTEX_POINT ( 'NONE', #37323 ) ;
#12519=ORIENTED_EDGE ( 'NONE', *, *, #74224, .F. ) ;
#12520=CARTESIAN_POINT ( 'NONE',  ( 95.05156358570199870, -41.69348830286664764, 293.6369201390379544 ) ) ;
#12521=CARTESIAN_POINT ( 'NONE',  ( 136.2737402105998967, -20.37320971850501650, 2.471387388698214060 ) ) ;
#12524=CARTESIAN_POINT ( 'NONE',  ( 106.0361919388305409, -11.55049677724511881, 323.5352776872487652 ) ) ;
#12525=CARTESIAN_POINT ( 'NONE',  ( 114.2499829074921820, -30.67355260991839216, 220.8034880678019647 ) ) ;
#12526=CIRCLE ( 'NONE', #89373, 1.000000000000000888 ) ;
#12527=CARTESIAN_POINT ( 'NONE',  ( 41.56670390244804025, -42.82844715994103524, 300.4678068554150059 ) ) ;
#12530=ORIENTED_EDGE ( 'NONE', *, *, #72949, .F. ) ;
#12532=AXIS2_PLACEMENT_3D ( 'NONE', #6150, #89267, #69261 ) ;
#12534=VECTOR ( 'NONE', #30935, 1000.000000000000000 ) ;
#12535=VERTEX_POINT ( 'NONE', #79568 ) ;
#12536=ORIENTED_EDGE ( 'NONE', *, *, #70949, .T. ) ;
#12537=CARTESIAN_POINT ( 'NONE',  ( 115.1064843935641022, -35.31944421942311862, 241.7823760838769545 ) ) ;
#12538=CARTESIAN_POINT ( 'NONE',  ( 116.5534958752826213, -32.35418074550542400, 104.1699109901969535 ) ) ;
#12539=CARTESIAN_POINT ( 'NONE',  ( 100.9560042165379059, -28.30978499293925310, 75.57562527591093726 ) ) ;
#12540=CARTESIAN_POINT ( 'NONE',  ( 99.08163574056251832, -37.52321402124415783, 249.5838068554173503 ) ) ;
#12542=CARTESIAN_POINT ( 'NONE',  ( 131.3325395364354904, -18.38432368373458559, 6.774690158158469089 ) ) ;
#12544=CARTESIAN_POINT ( 'NONE',  ( 110.4988674196275014, -26.88560509280327082, 205.8099109901969541 ) ) ;
#12545=DIRECTION ( 'NONE',  ( 1.000000000000000078E-15, -1.000000000000000083E-30, -1.000000000000000000 ) ) ;
#12546=VERTEX_POINT ( 'NONE', #73622 ) ;
#12549=EDGE_LOOP ( 'NONE', ( #27039, #57655, #74008, #63057 ) ) ;
#12550=DIRECTION ( 'NONE',  ( -1.000000000000000000, 0.000000000000000000, 0.000000000000000000 ) ) ;
#12553=DIRECTION ( 'NONE',  ( 0.000000000000000000, -1.000000000000000000, 0.000000000000000000 ) ) ;
#12554=( BOUNDED_CURVE ( )  B_SPLINE_CURVE ( 3, ( #74126, #39591, #18709, #4637 ),
 .UNSPECIFIED., .F., .T. ) 
 B_SPLINE_CURVE_WITH_KNOTS ( ( 4, 4 ),
 ( 4.647722573419573955, 4.714015861847076216 ),
 .UNSPECIFIED. ) 
 CURVE ( )  GEOMETRIC_REPRESENTATION_ITEM ( )  RATIONAL_B_SPLINE_CURVE ( ( 1.000000000000000000, 0.9996338001896092340, 0.9996338001896092340, 1.000000000000000000 ) ) 
 REPRESENTATION_ITEM ( '' )  );
#12556=CARTESIAN_POINT ( 'NONE',  ( 96.64175856332744274, -36.61924367559645788, 111.3184824187679567 ) ) ;
#12558=ADVANCED_FACE ( 'NONE', ( #80014 ), #2167, .F. ) ;
#12559=CARTESIAN_POINT ( 'NONE',  ( 136.8164806451553659, -36.72944715939129168, 6.749772901088312516 ) ) ;
#12560=DIRECTION ( 'NONE',  ( 0.000000000000000000, -1.000000000000000000, 0.000000000000000000 ) ) ;
#12562=DIRECTION ( 'NONE',  ( 1.000000000000000000, 4.163336342344333240E-14, 0.000000000000000000 ) ) ;
#12563=CARTESIAN_POINT ( 'NONE',  ( 25.56670390244797275, -58.35344715994099829, 139.9678068554150059 ) ) ;
#12564=CARTESIAN_POINT ( 'NONE',  ( 106.9407056411434951, -47.75886249174716625, 228.5794347997199907 ) ) ;
#12567=EDGE_LOOP ( 'NONE', ( #64618, #38153, #83468, #53760 ) ) ;
#12571=DIRECTION ( 'NONE',  ( 0.000000000000000000, 1.000000000000000000, 0.000000000000000000 ) ) ;
#12573=CARTESIAN_POINT ( 'NONE',  ( 72.06648329127401098, -45.72944715994106701, 14.67562527591093513 ) ) ;
#12574=CARTESIAN_POINT ( 'NONE',  ( 112.5123584215844659, -46.40184746663635451, 257.9965776568634510 ) ) ;
#12575=ORIENTED_EDGE ( 'NONE', *, *, #26072, .F. ) ;
#12578=CARTESIAN_POINT ( 'NONE',  ( 105.0174007254451567, -25.84429900004466063, 276.2365776568634033 ) ) ;
#12579=CARTESIAN_POINT ( 'NONE',  ( 101.7473938980672870, -45.74611303501656323, 158.1527681330539963 ) ) ;
#12580=CARTESIAN_POINT ( 'NONE',  ( 151.5667039024534120, -48.82844715994099971, 300.4678068554149490 ) ) ;
#12582=CARTESIAN_POINT ( 'NONE',  ( 182.0667039024478981, -32.29483332967958376, 117.4678068554150627 ) ) ;
#12583=DIRECTION ( 'NONE',  ( 4.299999999999999979E-14, -1.000000000000000000, 4.400000000000000367E-29 ) ) ;
#12584=DIRECTION ( 'NONE',  ( 0.000000000000000000, 0.000000000000000000, -1.000000000000000000 ) ) ;
#12585=CARTESIAN_POINT ( 'NONE',  ( 63.06670390244711655, -40.32844715994016838, 129.9678068554150911 ) ) ;
#12588=EDGE_CURVE ( 'NONE', #43667, #38868, #54936, .T. ) ;
#12589=ORIENTED_EDGE ( 'NONE', *, *, #82675, .F. ) ;
#12592=LINE ( 'NONE', #6666, #4474 ) ;
#12593=CARTESIAN_POINT ( 'NONE',  ( 115.8731522275743089, -31.19128430790907913, 30.27276813305396175 ) ) ;
#12594=DIRECTION ( 'NONE',  ( 1.639958061481212836E-42, -4.100000000000000342E-29, -1.000000000000000000 ) ) ;
#12599=AXIS2_PLACEMENT_3D ( 'NONE', #12191, #5833, #87160 ) ;
#12600=CARTESIAN_POINT ( 'NONE',  ( 105.8912501276363543, -45.18964566429946217, 256.8895626852198006 ) ) ;
#12602=ADVANCED_FACE ( 'NONE', ( #75423 ), #12298, .F. ) ;
#12604=VERTEX_POINT ( 'NONE', #5489 ) ;
#12606=CARTESIAN_POINT ( 'NONE',  ( 45.76696975232822950, -48.62818131006091704, 129.9678068554150911 ) ) ;
#12609=CARTESIAN_POINT ( 'NONE',  ( 107.0664832912750057, -36.72944715993903486, 9.125625275910969947 ) ) ;
#12610=CARTESIAN_POINT ( 'NONE',  ( 63.03715912545737865, -24.89890238295017966, 249.9678068554150343 ) ) ;
#12611=CARTESIAN_POINT ( 'NONE',  ( 116.2961902049681697, -40.76469377450285947, 54.93015473446794061 ) ) ;
#12612=DIRECTION ( 'NONE',  ( 0.000000000000000000, 1.000000000000000000, 0.000000000000000000 ) ) ;
#12613=CARTESIAN_POINT ( 'NONE',  ( 97.81170212845945855, -40.51743756719207568, 176.6354241348688277 ) ) ;
#12614=CARTESIAN_POINT ( 'NONE',  ( 100.4593435015893164, -29.47291325643525184, 285.6641967044828334 ) ) ;
#12615=CARTESIAN_POINT ( 'NONE',  ( 97.81168895331838087, -40.51742574516882200, 287.6356252759109680 ) ) ;
#12616=ORIENTED_EDGE ( 'NONE', *, *, #40558, .T. ) ;
#12617=ADVANCED_FACE ( 'NONE', ( #48130 ), #27711, .T. ) ;
#12618=DIRECTION ( 'NONE',  ( 0.000000000000000000, 1.000000000000000000, 0.000000000000000000 ) ) ;
#12620=AXIS2_PLACEMENT_3D ( 'NONE', #932, #56315, #64503 ) ;
#12621=DIRECTION ( 'NONE',  ( -4.554376769437570034E-14, 1.000000000000000000, 0.000000000000000000 ) ) ;
#12622=CARTESIAN_POINT ( 'NONE',  ( 102.4269143325283835, -29.42360532460997291, 63.33285227435298026 ) ) ;
#12623=CARTESIAN_POINT ( 'NONE',  ( 134.8062005078452614, -16.05355276379774310, 8.162233076783889985 ) ) ;
#12624=DIRECTION ( 'NONE',  ( 4.194175870806139918E-14, -1.000000000000000000, 0.000000000000000000 ) ) ;
#12625=CARTESIAN_POINT ( 'NONE',  ( 168.0371591254545649, -48.62818131005509059, 180.4678068554150059 ) ) ;
#12626=ORIENTED_EDGE ( 'NONE', *, *, #30594, .F. ) ;
#12627=CARTESIAN_POINT ( 'NONE',  ( 77.58678459498918301, -35.53883969337057636, 7.103318745425301728 ) ) ;
#12628=ORIENTED_EDGE ( 'NONE', *, *, #85798, .T. ) ;
#12629=CARTESIAN_POINT ( 'NONE',  ( 99.68446536626322541, -46.00016974189506413, 122.0413395616249659 ) ) ;
#12631=CARTESIAN_POINT ( 'NONE',  ( 98.07131787375925569, -37.77809840677601017, 85.85337220902894728 ) ) ;
#12632=CARTESIAN_POINT ( 'NONE',  ( 179.7974245136200011, -36.32844715994040996, -5.074374724088000832 ) ) ;
#12633=CARTESIAN_POINT ( 'NONE',  ( 103.9179606659962616, -45.58175368509670733, 98.74824997256392578 ) ) ;
#12634=DIRECTION ( 'NONE',  ( -0.7071067811865794361, 0.7071067811865157093, -7.071067811865492096E-16 ) ) ;
#12635=LINE ( 'NONE', #60768, #45465 ) ;
#12636=VECTOR ( 'NONE', #11278, 1000.000000000000000 ) ;
#12637=CARTESIAN_POINT ( 'NONE',  ( 104.0364404988798270, -47.38327494250712135, 63.36800622829197494 ) ) ;
#12641=CARTESIAN_POINT ( 'NONE',  ( 97.81399847929220925, -40.51646572127298640, 256.6355814287313137 ) ) ;
#12643=CARTESIAN_POINT ( 'NONE',  ( 72.26648329127297643, -1.929447159941394263, 342.9256252759109884 ) ) ;
#12644=ORIENTED_EDGE ( 'NONE', *, *, #72510, .F. ) ;
#12647=EDGE_LOOP ( 'NONE', ( #29385, #6494, #23836, #88821 ) ) ;
#12648=CARTESIAN_POINT ( 'NONE',  ( 106.5981863181247462, -46.53222597210214673, 247.5384824187689787 ) ) ;
#12649=CARTESIAN_POINT ( 'NONE',  ( 108.2803420215754500, -47.73912846947793298, 153.6518157521009584 ) ) ;
#12651=DIRECTION ( 'NONE',  ( 0.9068632946707807507, -0.4214249218767881500, 9.028300618466658994E-16 ) ) ;
#12652=CARTESIAN_POINT ( 'NONE',  ( 117.1064219673475719, -39.53695830471063744, 94.60991099019693706 ) ) ;
#12653=EDGE_LOOP ( 'NONE', ( #8756, #14881, #65348, #49049 ) ) ;
#12654=LINE ( 'NONE', #4940, #13371 ) ;
#12657=CARTESIAN_POINT ( 'NONE',  ( 98.30754538652605845, -41.72890334347444252, 157.7395978512973613 ) ) ;
#12659=VERTEX_POINT ( 'NONE', #75865 ) ;
#12660=AXIS2_PLACEMENT_3D ( 'NONE', #88669, #55446, #46840 ) ;
#12663=DIRECTION ( 'NONE',  ( -0.8660253910675250744, -0.0001484127182099123339, -0.5000000000000052180 ) ) ;
#12664=CARTESIAN_POINT ( 'NONE',  ( 114.3996560367811810, -27.45190519937920470, 274.5441967044824878 ) ) ;
#12665=CARTESIAN_POINT ( 'NONE',  ( 46.03715912545427358, -48.62818131006086020, 300.4678068554150059 ) ) ;
#12666=EDGE_CURVE ( 'NONE', #56235, #83503, #29724, .T. ) ;
#12667=DIRECTION ( 'NONE',  ( 1.000000000000000000, 0.000000000000000000, 0.000000000000000000 ) ) ;
#12670=CARTESIAN_POINT ( 'NONE',  ( 108.8243102715920685, -46.27830423087877421, 277.1438483995053161 ) ) ;
#12671=CARTESIAN_POINT ( 'NONE',  ( 99.98384727107165304, -29.55937221596129305, 100.6969498110766210 ) ) ;
#12672=CARTESIAN_POINT ( 'NONE',  ( 98.35456548258461851, -42.41549619454038123, 97.78705384733993355 ) ) ;
#12673=DIRECTION ( 'NONE',  ( -0.9999999853157766072, -0.0001713722456134502174, 0.000000000000000000 ) ) ;
#12674=CARTESIAN_POINT ( 'NONE',  ( 97.34100429996045989, -42.07995573552675950, 176.7146728949589658 ) ) ;
#12675=VERTEX_POINT ( 'NONE', #60884 ) ;
#12676=CYLINDRICAL_SURFACE ( 'NONE', #36533, 1.000000000000000888 ) ;
#12678=DIRECTION ( 'NONE',  ( 0.000000000000000000, 0.000000000000000000, -1.000000000000000000 ) ) ;
#12680=LINE ( 'NONE', #74901, #10207 ) ;
#12681=CARTESIAN_POINT ( 'NONE',  ( 136.5461822395192826, -35.53884010536734905, 2.747932095377162209 ) ) ;
#12682=ORIENTED_EDGE ( 'NONE', *, *, #51796, .T. ) ;
#12683=VECTOR ( 'NONE', #85644, 1000.000000000000000 ) ;
#12684=CARTESIAN_POINT ( 'NONE',  ( 97.07216744069562253, -35.37760030334273864, 62.21925782715792508 ) ) ;
#12685=EDGE_CURVE ( 'NONE', #25045, #40273, #76759, .T. ) ;
#12686=CARTESIAN_POINT ( 'NONE',  ( 113.3579092357397542, -45.09751872455207433, 143.0899109901969553 ) ) ;
#12689=CIRCLE ( 'NONE', #27137, 5.600000000000000533 ) ;
#12690=B_SPLINE_CURVE_WITH_KNOTS ( 'NONE', 3,
 ( #83786, #28345, #15183, #1562, #7020, #13836, #63328, #29704, #15639, #21559, #56039, #14746, #29263, #56946, #20658, #1106, #84689, #28817 ),
 .UNSPECIFIED., .F., .F.,
 ( 4, 2, 2, 2, 2, 2, 2, 2, 4 ),
 ( 0.5000000020452582961, 0.5625000017896010229, 0.6250000015339437498, 0.6875000012782863656, 0.7500000010226290925, 0.8125000007669718194, 0.8750000005113145463, 0.9375000002556572731, 1.000000000000000000 ),
 .UNSPECIFIED. ) ;
#12691=DIRECTION ( 'NONE',  ( 1.000000000000000078E-15, 1.000000000000000083E-30, -1.000000000000000000 ) ) ;
#12696=CONICAL_SURFACE ( 'NONE', #6843, 9.571100913904325935, 0.7853981633974543852 ) ;
#12697=EDGE_CURVE ( 'NONE', #83795, #49158, #72654, .T. ) ;
#12700=ORIENTED_EDGE ( 'NONE', *, *, #64862, .F. ) ;
#12701=EDGE_CURVE ( 'NONE', #22201, #18085, #49995, .T. ) ;
#12703=CARTESIAN_POINT ( 'NONE',  ( 163.0667039024477276, -33.35206098992141222, 237.4678068554150059 ) ) ;
#12707=CARTESIAN_POINT ( 'NONE',  ( 182.4202572930269923, -31.94127993907680718, 117.4678068554150627 ) ) ;
#12710=CIRCLE ( 'NONE', #64900, 11.45913725231036118 ) ;
#12713=LINE ( 'NONE', #60389, #36127 ) ;
#12714=CARTESIAN_POINT ( 'NONE',  ( 96.12852455334832769, -38.72269610271986551, 197.4699109901959844 ) ) ;
#12715=LINE ( 'NONE', #25434, #41442 ) ;
#12717=CARTESIAN_POINT ( 'NONE',  ( 99.16769444712207360, -43.44866735504064081, 72.89943479971999807 ) ) ;
#12719=DIRECTION ( 'NONE',  ( -0.7071067811856560636, -0.7071067811874389708, 0.000000000000000000 ) ) ;
#12720=FACE_OUTER_BOUND ( 'NONE', #76447, .T. ) ;
#12721=ORIENTED_EDGE ( 'NONE', *, *, #82221, .F. ) ;
#12722=LINE ( 'NONE', #20872, #71933 ) ;
#12724=EDGE_LOOP ( 'NONE', ( #60446, #17744 ) ) ;
#12725=VERTEX_POINT ( 'NONE', #68903 ) ;
#12726=EDGE_CURVE ( 'NONE', #26573, #20221, #75717, .T. ) ;
#12727=CARTESIAN_POINT ( 'NONE',  ( 104.7356562592608498, -27.62759180600148667, 241.7196785439919609 ) ) ;
#12730=AXIS2_PLACEMENT_3D ( 'NONE', #62409, #56021, #76041 ) ;
#12732=DIRECTION ( 'NONE',  ( 1.000000000000000078E-15, -1.000000000000000083E-30, -1.000000000000000000 ) ) ;
#12733=CARTESIAN_POINT ( 'NONE',  ( 182.3467384525650061, -36.02818131005800950, 342.9256252759119548 ) ) ;
#12734=VERTEX_POINT ( 'NONE', #62074 ) ;
#12739=CARTESIAN_POINT ( 'NONE',  ( 111.1290374500119498, -47.00926920395730235, 22.88800622829195675 ) ) ;
#12741=CARTESIAN_POINT ( 'NONE',  ( 109.3549613941650875, -28.89410453886290142, 257.6680903695913685 ) ) ;
#12743=DIRECTION ( 'NONE',  ( 0.000000000000000000, -1.000000000000000000, 0.000000000000000000 ) ) ;
#12744=CARTESIAN_POINT ( 'NONE',  ( 107.9488082096507213, -26.98745991040259895, 155.0041967044829505 ) ) ;
#12745=CARTESIAN_POINT ( 'NONE',  ( 80.06648329127398256, -9.029447159941060619, 4.925625275910944012 ) ) ;
#12746=DIRECTION ( 'NONE',  ( -3.360405532702990443E-14, 1.000000000000000000, 0.000000000000000000 ) ) ;
#12748=CYLINDRICAL_SURFACE ( 'NONE', #81145, 0.5000000000000104361 ) ;
#12750=CARTESIAN_POINT ( 'NONE',  ( 136.8164832912739826, -18.72944715994099951, -5.074374724088999145 ) ) ;
#12751=CARTESIAN_POINT ( 'NONE',  ( 118.0968619800241299, -35.49322535880637020, 229.9032443235299468 ) ) ;
#12754=ORIENTED_EDGE ( 'NONE', *, *, #19837, .T. ) ;
#12755=ADVANCED_FACE ( 'NONE', ( #27562 ), #7125, .T. ) ;
#12756=CARTESIAN_POINT ( 'NONE',  ( 95.98963492482539550, -41.07853246264400582, 92.62419670448296927 ) ) ;
#12757=CARTESIAN_POINT ( 'NONE',  ( 119.0814029968458811, -31.76540601701525901, 289.6356252759107406 ) ) ;
#12758=VERTEX_POINT ( 'NONE', #26658 ) ;
#12760=EDGE_LOOP ( 'NONE', ( #59513, #85069, #54529, #76186 ) ) ;
#12762=DIRECTION ( 'NONE',  ( 1.000000000000000078E-15, 0.000000000000000000, -1.000000000000000000 ) ) ;
#12763=DIRECTION ( 'NONE',  ( -1.000000000000000078E-15, 1.000000000000000083E-30, 1.000000000000000000 ) ) ;
#12764=LINE ( 'NONE', #61777, #5512 ) ;
#12765=CARTESIAN_POINT ( 'NONE',  ( 108.5685384152640864, -45.25263643686804471, 120.5214237029249915 ) ) ;
#12766=CARTESIAN_POINT ( 'NONE',  ( 117.4513846513745960, -35.59318846168486772, 274.9127681330539872 ) ) ;
#12767=LINE ( 'NONE', #74535, #17458 ) ;
#12768=VERTEX_POINT ( 'NONE', #47084 ) ;
#12770=VECTOR ( 'NONE', #35972, 1000.000000000000000 ) ;
#12771=CARTESIAN_POINT ( 'NONE',  ( 172.5667039024480118, -36.32844715993499563, 180.4678068554150059 ) ) ;
#12772=ORIENTED_EDGE ( 'NONE', *, *, #52901, .F. ) ;
#12774=ORIENTED_EDGE ( 'NONE', *, *, #21146, .T. ) ;
#12775=PLANE ( 'NONE',  #44503 ) ;
#12777=ORIENTED_EDGE ( 'NONE', *, *, #1942, .T. ) ;
#12778=DIRECTION ( 'NONE',  ( 1.000000000000000000, 4.299999999999999979E-14, 1.000000000000000078E-15 ) ) ;
#12779=DIRECTION ( 'NONE',  ( -1.000000000000000078E-15, 1.000000000000000083E-30, 1.000000000000000000 ) ) ;
#12783=CARTESIAN_POINT ( 'NONE',  ( 100.3400348588553328, -31.46521817125301368, 155.2209912566479488 ) ) ;
#12784=CARTESIAN_POINT ( 'NONE',  ( 117.5318583147471401, -37.01683481156648980, 43.80419670448293346 ) ) ;
#12785=CARTESIAN_POINT ( 'NONE',  ( 25.56670390244797275, -67.87844715994100397, 257.2178068554150059 ) ) ;
#12786=ORIENTED_EDGE ( 'NONE', *, *, #51122, .F. ) ;
#12787=EDGE_CURVE ( 'NONE', #84106, #18961, #25357, .T. ) ;
#12788=DIRECTION ( 'NONE',  ( 0.000000000000000000, 0.000000000000000000, 1.000000000000000000 ) ) ;
#12789=EDGE_CURVE ( 'NONE', #77070, #72856, #19852, .T. ) ;
#12792=EDGE_CURVE ( 'NONE', #12340, #76826, #28211, .T. ) ;
#12794=DIRECTION ( 'NONE',  ( 1.000000000000000000, -3.418174336900117128E-15, 0.000000000000000000 ) ) ;
#12795=CIRCLE ( 'NONE', #75160, 10.00000000000000711 ) ;
#12799=AXIS2_PLACEMENT_3D ( 'NONE', #51006, #86002, #49208 ) ;
#12800=CARTESIAN_POINT ( 'NONE',  ( 141.8545562996767444, -1.932463243632623229, 361.9756252759100335 ) ) ;
#12801=ORIENTED_EDGE ( 'NONE', *, *, #8272, .T. ) ;
#12802=AXIS2_PLACEMENT_3D ( 'NONE', #86757, #66287, #78174 ) ;
#12803=CARTESIAN_POINT ( 'NONE',  ( 118.2322726120735155, -40.77409347166903331, 23.54991099019593292 ) ) ;
#12804=CARTESIAN_POINT ( 'NONE',  ( 103.4621965996249600, -25.38836122657986394, 51.32133956162493149 ) ) ;
#12808=CARTESIAN_POINT ( 'NONE',  ( 102.0670646858952040, -27.97049243879484237, 146.4902315787838347 ) ) ;
#12809=CARTESIAN_POINT ( 'NONE',  ( 131.5094688080979211, -17.71735499139275305, 2.839545688279645042 ) ) ;
#12811=EDGE_CURVE ( 'NONE', #36283, #73560, #50684, .T. ) ;
#12813=CARTESIAN_POINT ( 'NONE',  ( 25.56670390244797275, -62.87844715994099687, 137.2178068554150059 ) ) ;
#12818=CARTESIAN_POINT ( 'NONE',  ( 106.6048964044850607, -25.63891871564037928, 40.09753003781596448 ) ) ;
#12819=CARTESIAN_POINT ( 'NONE',  ( 95.32466046839788021, -34.95410283156319053, 67.20705384733894050 ) ) ;
#12820=VECTOR ( 'NONE', #20833, 1000.000000000000000 ) ;
#12821=CARTESIAN_POINT ( 'NONE',  ( 116.8163290874346529, -34.14984622352434940, 174.0307337802608743 ) ) ;
#12822=FACE_OUTER_BOUND ( 'NONE', #71197, .T. ) ;
#12826=CARTESIAN_POINT ( 'NONE',  ( 97.28626111821324685, -36.62605694204433604, 107.3184824187669619 ) ) ;
#12830=CARTESIAN_POINT ( 'NONE',  ( 112.4430884738663394, -45.67687932769430859, 234.0070538473389377 ) ) ;
#12831=CARTESIAN_POINT ( 'NONE',  ( 97.81310256251512669, -40.52087785597539948, 252.6358801373274048 ) ) ;
#12832=CARTESIAN_POINT ( 'NONE',  ( 116.9155271266333642, -38.71841217917236122, 148.6681463939105754 ) ) ;
#12833=CYLINDRICAL_SURFACE ( 'NONE', #66078, 4.874999999999990230 ) ;
#12834=DIRECTION ( 'NONE',  ( 1.000000000000000000, 6.145690160522439356E-16, 0.000000000000000000 ) ) ;
#12835=CARTESIAN_POINT ( 'NONE',  ( 75.31670390244798341, -67.87844715994100397, 86.31780685541500020 ) ) ;
#12837=CARTESIAN_POINT ( 'NONE',  ( 99.89458030379213938, -28.23347241844141919, 150.6356252759109680 ) ) ;
#12841=ADVANCED_FACE ( 'NONE', ( #62969 ), #43412, .F. ) ;
#12842=AXIS2_PLACEMENT_3D ( 'NONE', #88803, #54227, #61509 ) ;
#12843=CARTESIAN_POINT ( 'NONE',  ( 112.1755263188685205, -29.48886997617658423, 126.0187261630399718 ) ) ;
#12844=LINE ( 'NONE', #60058, #28343 ) ;
#12845=CARTESIAN_POINT ( 'NONE',  ( 117.4008144674644285, -32.62901037329578458, 245.1270538473389706 ) ) ;
#12847=CARTESIAN_POINT ( 'NONE',  ( 57.56670390244804736, -42.82844715994040286, 293.2178068554150627 ) ) ;
#12852=DIRECTION ( 'NONE',  ( 1.000000000000000078E-15, 0.000000000000000000, -1.000000000000000000 ) ) ;
#12853=CARTESIAN_POINT ( 'NONE',  ( 98.27975524859421341, -42.29919363830190804, 186.7756252759109543 ) ) ;
#12854=LINE ( 'NONE', #40540, #86675 ) ;
#12855=VERTEX_POINT ( 'NONE', #78425 ) ;
#12860=DIRECTION ( 'NONE',  ( -3.999999999999999995E-14, 1.000000000000000000, -4.100000000000000342E-29 ) ) ;
#12861=DIRECTION ( 'NONE',  ( 1.000000000000000078E-15, -1.000000000000000083E-30, -1.000000000000000000 ) ) ;
#12867=FACE_OUTER_BOUND ( 'NONE', #28910, .T. ) ;
#12868=CARTESIAN_POINT ( 'NONE',  ( 103.6385507868184277, -26.22095696399066966, 210.3394347997209763 ) ) ;
#12869=VERTEX_POINT ( 'NONE', #28450 ) ;
#12870=AXIS2_PLACEMENT_3D ( 'NONE', #15663, #71083, #43790 ) ;
#12873=CARTESIAN_POINT ( 'NONE',  ( 115.0365168329930867, -42.90940218011385809, 164.3021974415819670 ) ) ;
#12874=CARTESIAN_POINT ( 'NONE',  ( 113.7569007282865101, -30.30027569836345336, 37.25380465530597718 ) ) ;
#12876=CARTESIAN_POINT ( 'NONE',  ( 109.3632651814324817, -25.89385771158341853, 180.9222919425779708 ) ) ;
#12877=CARTESIAN_POINT ( 'NONE',  ( 162.7131505118679797, -31.94127993907790852, 193.9678068554150059 ) ) ;
#12880=CARTESIAN_POINT ( 'NONE',  ( 111.7624441058946871, -45.65476495282741354, 67.96418635338669390 ) ) ;
#12882=ORIENTED_EDGE ( 'NONE', *, *, #21949, .T. ) ;
#12883=DIRECTION ( 'NONE',  ( -0.7071067811869841124, 0.7071067811861110330, 0.000000000000000000 ) ) ;
#12885=ORIENTED_EDGE ( 'NONE', *, *, #5497, .F. ) ;
#12888=CARTESIAN_POINT ( 'NONE',  ( 112.3043975166656736, -44.90470753876829235, 67.45241982807698378 ) ) ;
#12889=CARTESIAN_POINT ( 'NONE',  ( 118.8150946519381250, -38.46269469016341702, 223.7099109901969598 ) ) ;
#12890=CARTESIAN_POINT ( 'NONE',  ( 96.07698540226623152, -35.78353028925530310, 186.2461014663869889 ) ) ;
#12891=CARTESIAN_POINT ( 'NONE',  ( 84.06648329127399677, -18.82844715994099971, 239.5838068554169809 ) ) ;
#12892=CARTESIAN_POINT ( 'NONE',  ( 110.2773916389477478, -46.62487827714361543, 8.827053847339950465 ) ) ;
#12893=CARTESIAN_POINT ( 'NONE',  ( 194.0371591254573502, -24.89890238294407965, 249.9678068554149775 ) ) ;
#12895=DIRECTION ( 'NONE',  ( -1.000000000000000000, -5.512527431108013646E-15, 0.000000000000000000 ) ) ;
#12897=VECTOR ( 'NONE', #46421, 1000.000000000000000 ) ;
#12899=CARTESIAN_POINT ( 'NONE',  ( 105.6259887305572676, -47.09919361126699044, 257.4670538473392298 ) ) ;
#12900=ORIENTED_EDGE ( 'NONE', *, *, #49047, .T. ) ;
#12901=CARTESIAN_POINT ( 'NONE',  ( 114.1248632939498719, -29.05700933358840032, 199.4841967044819739 ) ) ;
#12902=DIRECTION ( 'NONE',  ( 0.000000000000000000, -1.000000000000000000, 0.000000000000000000 ) ) ;
#12905=CARTESIAN_POINT ( 'NONE',  ( 112.5286436197554849, -45.20754988127118423, 29.03387687458365818 ) ) ;
#12906=CARTESIAN_POINT ( 'NONE',  ( 99.40665670852901314, -32.99082215312059674, 277.6356252759109680 ) ) ;
#12908=CARTESIAN_POINT ( 'NONE',  ( 97.86658801961326049, -40.64925014044468554, 172.6469892981851615 ) ) ;
#12910=DIRECTION ( 'NONE',  ( 9.860761315262647568E-31, -0.7071067811865480168, 0.7071067811865470176 ) ) ;
#12911=ADVANCED_FACE ( 'NONE', ( #22558 ), #48546, .T. ) ;
#12912=DIRECTION ( 'NONE',  ( -1.000000000000000078E-15, -1.000000000000000083E-30, 1.000000000000000000 ) ) ;
#12913=EDGE_CURVE ( 'NONE', #8428, #21819, #79008, .T. ) ;
#12914=DIRECTION ( 'NONE',  ( 0.000000000000000000, 0.000000000000000000, -1.000000000000000000 ) ) ;
#12915=DIRECTION ( 'NONE',  ( 1.000000000000000078E-15, -1.000000000000000000, 0.000000000000000000 ) ) ;
#12916=CARTESIAN_POINT ( 'NONE',  ( 107.0667039024479834, -36.72944715994099596, 239.5838068554170093 ) ) ;
#12917=ORIENTED_EDGE ( 'NONE', *, *, #76897, .T. ) ;
#12918=VECTOR ( 'NONE', #43721, 1000.000000000000000 ) ;
#12920=CARTESIAN_POINT ( 'NONE',  ( 106.9401735163927611, -47.80552439772274909, 232.5794347997199907 ) ) ;
#12921=CARTESIAN_POINT ( 'NONE',  ( 98.14961424977839499, -43.26117181588809757, 102.8175300378159847 ) ) ;
#12922=CARTESIAN_POINT ( 'NONE',  ( 114.4457317200277089, -27.39361268404408634, 270.5441967044823741 ) ) ;
#12923=CARTESIAN_POINT ( 'NONE',  ( 115.8254323940822843, -31.73001883404345236, 154.2397919421239010 ) ) ;
#12924=CARTESIAN_POINT ( 'NONE',  ( 167.6524903400753601, -48.32844715993521589, 249.9678068554149775 ) ) ;
#12925=CARTESIAN_POINT ( 'NONE',  ( 164.9190312289449878, -35.91149509761181235, -5.074374724088000832 ) ) ;
#12928=CARTESIAN_POINT ( 'NONE',  ( 131.4524275574070487, -19.60567372263979280, 2.908038864009617086 ) ) ;
#12932=ORIENTED_EDGE ( 'NONE', *, *, #8710, .F. ) ;
#12933=CARTESIAN_POINT ( 'NONE',  ( 108.8156685800011303, -28.36903548837926792, 139.3352769709339896 ) ) ;
#12934=CIRCLE ( 'NONE', #65186, 0.9999999999991942001 ) ;
#12936=ORIENTED_EDGE ( 'NONE', *, *, #52027, .F. ) ;
#12937=CARTESIAN_POINT ( 'NONE',  ( 72.25757238336811383, -1.944390235229867425, 394.9756252759101471 ) ) ;
#12938=CARTESIAN_POINT ( 'NONE',  ( 108.2741602056595269, -26.36093993100608657, 125.9841967044819597 ) ) ;
#12940=VECTOR ( 'NONE', #19423, 1000.000000000000000 ) ;
#12941=CARTESIAN_POINT ( 'NONE',  ( 49.21437657594998427, -35.91149509761070391, 342.9256252759119548 ) ) ;
#12942=DIRECTION ( 'NONE',  ( -0.7071067811865501263, 0.7071067811865449082, -7.071067811865501957E-16 ) ) ;
#12944=AXIS2_PLACEMENT_3D ( 'NONE', #38260, #16051, #86432 ) ;
#12945=CARTESIAN_POINT ( 'NONE',  ( 104.2296407737279509, -46.70397019442136610, 67.36800622829292706 ) ) ;
#12946=ORIENTED_EDGE ( 'NONE', *, *, #27353, .F. ) ;
#12948=ORIENTED_EDGE ( 'NONE', *, *, #31545, .T. ) ;
#12949=DIRECTION ( 'NONE',  ( 0.000000000000000000, 1.000000000000000000, 0.000000000000000000 ) ) ;
#12950=CARTESIAN_POINT ( 'NONE',  ( 98.51953950620418254, -30.85675296092865239, 161.8594347997199918 ) ) ;
#12951=FACE_OUTER_BOUND ( 'NONE', #39964, .T. ) ;
#12952=DIRECTION ( 'NONE',  ( 1.000000000000000078E-15, 0.000000000000000000, -1.000000000000000000 ) ) ;
#12954=ADVANCED_FACE ( 'NONE', ( #57503 ), #76614, .T. ) ;
#12955=VECTOR ( 'NONE', #46711, 1000.000000000000000 ) ;
#12958=CARTESIAN_POINT ( 'NONE',  ( 107.0664832912739968, -36.72944715994100306, 277.6356252759110248 ) ) ;
#12959=CARTESIAN_POINT ( 'NONE',  ( 97.56228874418788166, -32.49873190831181802, 100.9927681330539713 ) ) ;
#12960=ORIENTED_EDGE ( 'NONE', *, *, #1943, .F. ) ;
#12962=ORIENTED_EDGE ( 'NONE', *, *, #60322, .T. ) ;
#12965=CYLINDRICAL_SURFACE ( 'NONE', #39481, 2.030000000002079918 ) ;
#12966=CARTESIAN_POINT ( 'NONE',  ( 103.7603453811189667, -44.19263536178414142, 175.0623760838769840 ) ) ;
#12967=VECTOR ( 'NONE', #53800, 1000.000000000000000 ) ;
#12968=EDGE_CURVE ( 'NONE', #23436, #61346, #22113, .T. ) ;
#12969=B_SPLINE_CURVE_WITH_KNOTS ( 'NONE', 3,
 ( #9810, #31572, #66093, #64333, #43867, #36632, #10252, #71600, #65653, #72485, #78427, #72915, #87005, #59278, #58392, #37069, #16189, #9362 ),
 .UNSPECIFIED., .F., .F.,
 ( 4, 2, 2, 2, 2, 2, 2, 2, 4 ),
 ( 0.4999946744394294096, 0.5624953401345007542, 0.6249960058295720433, 0.6874966715246433324, 0.7499973372197146215, 0.8124980029147859106, 0.8749986686098573108, 0.9374993343049287109, 1.000000000000000000 ),
 .UNSPECIFIED. ) ;
#12970=CARTESIAN_POINT ( 'NONE',  ( 102.0676263548437248, -27.97016309701666614, 26.48917362245403240 ) ) ;
#12973=ORIENTED_EDGE ( 'NONE', *, *, #38401, .T. ) ;
#12975=CARTESIAN_POINT ( 'NONE',  ( 135.2096185787404181, -21.23068377182193345, 1.829869271364342076 ) ) ;
#12976=ORIENTED_EDGE ( 'NONE', *, *, #38644, .T. ) ;
#12978=CARTESIAN_POINT ( 'NONE',  ( 34.67381068362099228, -26.00627455219321860, -5.074374724088000832 ) ) ;
#12979=EDGE_CURVE ( 'NONE', #16028, #25661, #7574, .T. ) ;
#12980=CARTESIAN_POINT ( 'NONE',  ( 97.76609424928555825, -35.39554716186696481, 222.6568214011349767 ) ) ;
#12982=EDGE_CURVE ( 'NONE', #2549, #31941, #31188, .T. ) ;
#12985=VECTOR ( 'NONE', #64178, 1000.000000000000000 ) ;
#12989=VERTEX_POINT ( 'NONE', #77067 ) ;
#12990=ORIENTED_EDGE ( 'NONE', *, *, #25793, .F. ) ;
#12991=EDGE_CURVE ( 'NONE', #49825, #8449, #14846, .T. ) ;
#12992=CARTESIAN_POINT ( 'NONE',  ( 108.8441613132982155, -28.76266695291210951, 222.7195189410199703 ) ) ;
#12994=CARTESIAN_POINT ( 'NONE',  ( 109.2059698035850914, -26.50355049596284118, 139.9127681330539872 ) ) ;
#12995=CARTESIAN_POINT ( 'NONE',  ( 96.11054930851071276, -38.00668368623060189, 86.43086337114897333 ) ) ;
#12996=CARTESIAN_POINT ( 'NONE',  ( 101.8644741850226580, -30.26426668629352079, 249.5838068554171514 ) ) ;
#12998=CARTESIAN_POINT ( 'NONE',  ( 107.9469797351305118, -25.30413091219610422, 322.6728824914080747 ) ) ;
#12999=CARTESIAN_POINT ( 'NONE',  ( 101.9845378472182773, -45.87248622144053911, 183.1727681330539781 ) ) ;
#13001=CARTESIAN_POINT ( 'NONE',  ( 116.3265940946004378, -32.93621273019581253, 125.1356252759109680 ) ) ;
#13002=EDGE_LOOP ( 'NONE', ( #24227, #62900, #16556, #47310, #32080 ) ) ;
#13004=ORIENTED_EDGE ( 'NONE', *, *, #43647, .F. ) ;
#13005=ORIENTED_EDGE ( 'NONE', *, *, #85904, .F. ) ;
#13008=CARTESIAN_POINT ( 'NONE',  ( 87.06648329127403940, -46.72944715994105280, -4.824374724089049771 ) ) ;
#13009=CARTESIAN_POINT ( 'NONE',  ( 99.50153220775246155, -43.90290835836871253, 81.92991099019597812 ) ) ;
#13011=CYLINDRICAL_SURFACE ( 'NONE', #2901, 0.2499999999999941991 ) ;
#13012=CARTESIAN_POINT ( 'NONE',  ( 152.0371591254585724, -47.82818131005588214, 129.9678068554149775 ) ) ;
#13013=CARTESIAN_POINT ( 'NONE',  ( 97.81169461453751524, -40.51741999607308742, 142.6356648221729131 ) ) ;
#13015=CARTESIAN_POINT ( 'NONE',  ( 105.1150531980676561, -26.51080800785444680, 231.2270538473399597 ) ) ;
#13016=FACE_OUTER_BOUND ( 'NONE', #8873, .T. ) ;
#13018=EDGE_LOOP ( 'NONE', ( #68121, #68080, #77595, #20230 ) ) ;
#13019=AXIS2_PLACEMENT_3D ( 'NONE', #70313, #84412, #8542 ) ;
#13020=CARTESIAN_POINT ( 'NONE',  ( 107.0664832912739257, -52.42944715994095617, 311.3356252759109566 ) ) ;
#13021=EDGE_CURVE ( 'NONE', #7162, #31385, #36172, .T. ) ;
#13022=DIRECTION ( 'NONE',  ( 0.000000000000000000, 1.000000000000000000, 0.000000000000000000 ) ) ;
#13027=CARTESIAN_POINT ( 'NONE',  ( 104.3127904766024443, -25.97630531626002437, 245.2880062282919482 ) ) ;
#13030=CARTESIAN_POINT ( 'NONE',  ( 104.2409529242390391, -46.76432966167102023, 18.35848241876792031 ) ) ;
#13031=CARTESIAN_POINT ( 'NONE',  ( 95.52146136750830863, -39.61450893497475079, 162.5213395616259788 ) ) ;
#13034=CARTESIAN_POINT ( 'NONE',  ( 172.5664832912740110, -27.82844715994070484, 143.6756252759119832 ) ) ;
#13036=DIRECTION ( 'NONE',  ( -6.493183223601999383E-14, 1.000000000000000000, -6.593183223602000791E-29 ) ) ;
#13037=CARTESIAN_POINT ( 'NONE',  ( 107.0664832912739968, -36.72944715994100306, 287.6356252759109680 ) ) ;
#13038=CARTESIAN_POINT ( 'NONE',  ( 130.5667039024480118, -34.21194715994094082, 229.5838068554170093 ) ) ;
#13039=DIRECTION ( 'NONE',  ( -1.000000000000000078E-15, 1.000000000000000083E-30, 1.000000000000000000 ) ) ;
#13041=ORIENTED_EDGE ( 'NONE', *, *, #40952, .F. ) ;
#13043=CONICAL_SURFACE ( 'NONE', #47820, 13.31607168056649826, 0.1047197551196538678 ) ;
#13046=CARTESIAN_POINT ( 'NONE',  ( 117.4903696573863385, -37.28369426754698424, 14.78419670448294454 ) ) ;
#13048=AXIS2_PLACEMENT_3D ( 'NONE', #72468, #45178, #31558 ) ;
#13049=CARTESIAN_POINT ( 'NONE',  ( 19.56670390244739721, -25.42844715994192129, 249.9678068554150059 ) ) ;
#13051=CARTESIAN_POINT ( 'NONE',  ( 105.4642979808546670, -28.33962392264099250, 234.6495626852199621 ) ) ;
#13053=EDGE_LOOP ( 'NONE', ( #34545, #22263, #52889, #21784 ) ) ;
#13055=EDGE_LOOP ( 'NONE', ( #87640, #42209, #52577, #32292, #64777, #16734 ) ) ;
#13057=CARTESIAN_POINT ( 'NONE',  ( 104.4081941772929980, -46.45811691506909114, 102.3647646864374110 ) ) ;
#13058=DIRECTION ( 'NONE',  ( 1.000000000000000078E-15, 1.000000000000000083E-30, -1.000000000000000000 ) ) ;
#13059=DIRECTION ( 'NONE',  ( 1.067522139062650671E-15, 1.000000000000000000, 0.000000000000000000 ) ) ;
#13060=FACE_OUTER_BOUND ( 'NONE', #65277, .T. ) ;
#13061=AXIS2_PLACEMENT_3D ( 'NONE', #27828, #48250, #27380 ) ;
#13062=FACE_OUTER_BOUND ( 'NONE', #63818, .T. ) ;
#13063=CARTESIAN_POINT ( 'NONE',  ( 100.6033219294167793, -44.83909144599476804, 272.0289586092449667 ) ) ;
#13065=ORIENTED_EDGE ( 'NONE', *, *, #46185, .F. ) ;
#13066=LINE ( 'NONE', #74392, #78048 ) ;
#13067=CIRCLE ( 'NONE', #85640, 0.5000000000000004441 ) ;
#13068=CYLINDRICAL_SURFACE ( 'NONE', #61261, 13.44999999999999396 ) ;
#13069=CARTESIAN_POINT ( 'NONE',  ( 114.1581430127411352, -30.74577825543392606, 72.20237608387697037 ) ) ;
#13070=EDGE_CURVE ( 'NONE', #9306, #87803, #69443, .T. ) ;
#13072=EDGE_CURVE ( 'NONE', #65138, #31678, #72914, .T. ) ;
#13074=VECTOR ( 'NONE', #74780, 1000.000000000000000 ) ;
#13075=DIRECTION ( 'NONE',  ( -2.900000000000000265E-14, 2.000000000000000155E-15, -1.000000000000000000 ) ) ;
#13077=EDGE_CURVE ( 'NONE', #31310, #81967, #18390, .T. ) ;
#13080=CARTESIAN_POINT ( 'NONE',  ( 114.2535261088984981, -44.28147934099003180, 158.1813395616249807 ) ) ;
#13081=VERTEX_POINT ( 'NONE', #51126 ) ;
#13082=EDGE_CURVE ( 'NONE', #21703, #28403, #83467, .T. ) ;
#13084=CARTESIAN_POINT ( 'NONE',  ( 103.2343105203340201, -28.73928255177903068, 91.86444044875396742 ) ) ;
#13085=EDGE_CURVE ( 'NONE', #85412, #21246, #78866, .T. ) ;
#13086=DIRECTION ( 'NONE',  ( 0.7071067811865514585, -0.7071067811865435759, 7.071067811865522665E-16 ) ) ;
#13089=CARTESIAN_POINT ( 'NONE',  ( 101.9498695335308014, -27.62134513440381411, 56.48419670448296159 ) ) ;
#13090=EDGE_CURVE ( 'NONE', #85887, #48350, #59715, .T. ) ;
#13091=EDGE_CURVE ( 'NONE', #22706, #70290, #46076, .T. ) ;
#13095=( BOUNDED_CURVE ( )  B_SPLINE_CURVE ( 3, ( #72017, #66066, #9338, #59692 ),
 .UNSPECIFIED., .F., .T. ) 
 B_SPLINE_CURVE_WITH_KNOTS ( ( 4, 4 ),
 ( 1.570796326794220432, 3.141592653588994200 ),
 .UNSPECIFIED. ) 
 CURVE ( )  GEOMETRIC_REPRESENTATION_ITEM ( )  RATIONAL_B_SPLINE_CURVE ( ( 1.000000000000000000, 0.8047378541243939143, 0.8047378541243939143, 1.000000000000000000 ) ) 
 REPRESENTATION_ITEM ( '' )  );
#13096=ORIENTED_EDGE ( 'NONE', *, *, #40952, .T. ) ;
#13099=CIRCLE ( 'NONE', #46394, 0.5000000000000004441 ) ;
#13100=CARTESIAN_POINT ( 'NONE',  ( 138.8167039024479834, -50.82844715994100682, 35.51780685541480409 ) ) ;
#13102=CARTESIAN_POINT ( 'NONE',  ( 96.91794407517402021, -34.59732685048006573, 261.1737205140070159 ) ) ;
#13103=CARTESIAN_POINT ( 'NONE',  ( 96.62828407576300549, -37.15518013270143172, 157.3584824187679487 ) ) ;
#13104=CARTESIAN_POINT ( 'NONE',  ( 57.56670390244744340, -48.82844715994040286, 173.2178068554150911 ) ) ;
#13106=CARTESIAN_POINT ( 'NONE',  ( 97.54238320567634446, -32.48987111900922997, 96.99276813305395706 ) ) ;
#13108=CARTESIAN_POINT ( 'NONE',  ( 102.0691103994968643, -27.96929322877106117, 96.48882554008449119 ) ) ;
#13109=ORIENTED_EDGE ( 'NONE', *, *, #36764, .F. ) ;
#13110=LINE ( 'NONE', #88959, #10452 ) ;
#13112=FACE_OUTER_BOUND ( 'NONE', #30753, .T. ) ;
#13113=ORIENTED_EDGE ( 'NONE', *, *, #41255, .T. ) ;
#13114=AXIS2_PLACEMENT_3D ( 'NONE', #43159, #70901, #51310 ) ;
#13115=DIRECTION ( 'NONE',  ( 1.000000000000000000, 2.999999999999999839E-15, 1.000000000000000078E-15 ) ) ;
#13116=CARTESIAN_POINT ( 'NONE',  ( 41.56670390244783420, -36.32844715994104234, 249.9678068554150343 ) ) ;
#13117=CARTESIAN_POINT ( 'NONE',  ( 116.1206117333611871, -31.56300607074027909, 289.2384824187681716 ) ) ;
#13118=CARTESIAN_POINT ( 'NONE',  ( 41.56648329127398966, -18.82844715994071194, 318.9256252759120116 ) ) ;
#13121=CARTESIAN_POINT ( 'NONE',  ( 107.1874307469290386, -26.94942635195914349, 35.06705384733993469 ) ) ;
#13122=CARTESIAN_POINT ( 'NONE',  ( 116.0344360784154532, -32.23950325226218183, 99.19648518757557554 ) ) ;
#13123=CARTESIAN_POINT ( 'NONE',  ( 113.8422018911646774, -44.62364141802220985, 104.1413395616249744 ) ) ;
#13124=DIRECTION ( 'NONE',  ( 3.999999999999999995E-14, -1.000000000000000000, 4.100000000000000342E-29 ) ) ;
#13125=CARTESIAN_POINT ( 'NONE',  ( 117.8245512228195224, -33.99506276729055543, 169.0365776568629599 ) ) ;
#13128=CIRCLE ( 'NONE', #14615, 2.750000000000002665 ) ;
#13129=DIRECTION ( 'NONE',  ( 0.000000000000000000, 0.000000000000000000, 1.000000000000000000 ) ) ;
#13130=LINE ( 'NONE', #40814, #18888 ) ;
#13131=CARTESIAN_POINT ( 'NONE',  ( 136.4174407532110251, -35.29868422067971778, 2.608896314047598253 ) ) ;
#13132=ORIENTED_EDGE ( 'NONE', *, *, #87637, .F. ) ;
#13133=ADVANCED_FACE ( 'NONE', ( #79204 ), #65106, .F. ) ;
#13134=FACE_OUTER_BOUND ( 'NONE', #47120, .T. ) ;
#13135=CARTESIAN_POINT ( 'NONE',  ( 97.70685376065341643, -42.69687791250295561, 141.7661014663869707 ) ) ;
#13136=ORIENTED_EDGE ( 'NONE', *, *, #33389, .T. ) ;
#13138=EDGE_CURVE ( 'NONE', #88437, #26589, #80224, .T. ) ;
#13139=DIRECTION ( 'NONE',  ( 1.000000000000000000, 4.163336342344333240E-14, 0.000000000000000000 ) ) ;
#13140=CARTESIAN_POINT ( 'NONE',  ( 193.0371591254583450, -47.82818131005411999, 237.4678068554150059 ) ) ;
#13141=DIRECTION ( 'NONE',  ( 0.000000000000000000, 0.000000000000000000, -1.000000000000000000 ) ) ;
#13146=EDGE_LOOP ( 'NONE', ( #17835, #64598, #80995, #87025 ) ) ;
#13147=AXIS2_PLACEMENT_3D ( 'NONE', #65533, #51438, #85998 ) ;
#13148=EDGE_LOOP ( 'NONE', ( #12408, #89748, #39042, #38993 ) ) ;
#13151=CARTESIAN_POINT ( 'NONE',  ( 116.3214453605167478, -32.94026287388232532, 159.1356252759109680 ) ) ;
#13153=FACE_OUTER_BOUND ( 'NONE', #11604, .T. ) ;
#13157=ORIENTED_EDGE ( 'NONE', *, *, #57972, .T. ) ;
#13160=CARTESIAN_POINT ( 'NONE',  ( 97.78144721833434971, -39.80378292816723018, 237.5813395616249579 ) ) ;
#13161=DIRECTION ( 'NONE',  ( 0.000000000000000000, 0.000000000000000000, -1.000000000000000000 ) ) ;
#13162=CARTESIAN_POINT ( 'NONE',  ( 98.84777479348176144, -29.24180311599948467, 76.73848241876795839 ) ) ;
#13163=CARTESIAN_POINT ( 'NONE',  ( 114.5898276930936532, -43.34969010434090819, 53.25228543077692933 ) ) ;
#13165=CARTESIAN_POINT ( 'NONE',  ( 103.3333906439367098, -27.45234650783311636, 21.38091191696080529 ) ) ;
#13167=ORIENTED_EDGE ( 'NONE', *, *, #64796, .T. ) ;
#13171=ADVANCED_FACE ( 'NONE', ( #72813 ), #24224, .T. ) ;
#13172=CARTESIAN_POINT ( 'NONE',  ( 97.76609424928555825, -35.39554716186696481, 222.6568214011349767 ) ) ;
#13173=VECTOR ( 'NONE', #44842, 1000.000000000000114 ) ;
#13174=PLANE ( 'NONE',  #5265 ) ;
#13175=CARTESIAN_POINT ( 'NONE',  ( 97.33780952251225926, -34.07119382363175220, 141.1148024095264759 ) ) ;
#13178=CARTESIAN_POINT ( 'NONE',  ( 113.1782937241120806, -44.75186862947914079, 154.0939586045162173 ) ) ;
#13180=CARTESIAN_POINT ( 'NONE',  ( 81.30995888129169202, -39.18301917769736065, 1.868341932361629265 ) ) ;
#13181=ORIENTED_EDGE ( 'NONE', *, *, #19258, .T. ) ;
#13184=CARTESIAN_POINT ( 'NONE',  ( 99.04388270494561652, -42.84098838056963388, 182.8444536297417073 ) ) ;
#13185=ORIENTED_EDGE ( 'NONE', *, *, #10117, .T. ) ;
#13186=CARTESIAN_POINT ( 'NONE',  ( 103.9573432206533283, -47.33663036165624050, 62.33753003781600199 ) ) ;
#13187=ORIENTED_EDGE ( 'NONE', *, *, #30943, .T. ) ;
#13188=CARTESIAN_POINT ( 'NONE',  ( 110.0029149558365305, -28.58829895313488834, 247.6071379886389821 ) ) ;
#13189=EDGE_CURVE ( 'NONE', #20374, #15487, #55808, .T. ) ;
#13191=CARTESIAN_POINT ( 'NONE',  ( 116.6093774848466325, -38.87601340171674025, 148.6499109901969859 ) ) ;
#13193=PLANE ( 'NONE',  #24441 ) ;
#13196=CARTESIAN_POINT ( 'NONE',  ( 115.8919449742516861, -44.71207447090664999, 229.2413395616249545 ) ) ;
#13197=DIRECTION ( 'NONE',  ( 0.7071067811865671127, 0.7071067811865279218, 7.071067811865664660E-16 ) ) ;
#13198=EDGE_CURVE ( 'NONE', #31817, #394, #16687, .T. ) ;
#13199=ORIENTED_EDGE ( 'NONE', *, *, #37585, .T. ) ;
#13200=CARTESIAN_POINT ( 'NONE',  ( 103.1584010082818850, -27.01760528431355368, 126.3813395616259783 ) ) ;
#13206=DIRECTION ( 'NONE',  ( 0.000000000000000000, 1.000000000000000000, 0.000000000000000000 ) ) ;
#13207=LINE ( 'NONE', #40891, #35614 ) ;
#13208=DIRECTION ( 'NONE',  ( 1.000000000000000000, 4.299999999999999979E-14, 1.000000000000000078E-15 ) ) ;
#13211=CARTESIAN_POINT ( 'NONE',  ( 107.8028422452843387, -28.59910946728008341, 152.8223760838769749 ) ) ;
#13212=CARTESIAN_POINT ( 'NONE',  ( 108.0160737019250377, -24.89219542061752577, 261.0127681330534415 ) ) ;
#13213=EDGE_CURVE ( 'NONE', #84792, #28839, #11483, .T. ) ;
#13214=FACE_OUTER_BOUND ( 'NONE', #45863, .T. ) ;
#13216=FACE_OUTER_BOUND ( 'NONE', #32481, .T. ) ;
#13217=AXIS2_PLACEMENT_3D ( 'NONE', #45484, #18251, #11445 ) ;
#13218=ORIENTED_EDGE ( 'NONE', *, *, #8596, .F. ) ;
#13219=EDGE_LOOP ( 'NONE', ( #68624, #25882, #64166, #1591 ) ) ;
#13222=ORIENTED_EDGE ( 'NONE', *, *, #32541, .T. ) ;
#13224=CARTESIAN_POINT ( 'NONE',  ( 182.2420472961719895, -31.76306994223730840, -5.074374724088000832 ) ) ;
#13225=CARTESIAN_POINT ( 'NONE',  ( 97.75831510205337338, -40.38470820808293382, 16.62424145675636922 ) ) ;
#13227=DIRECTION ( 'NONE',  ( 1.000000000000000078E-15, 1.000000000000000083E-30, -1.000000000000000000 ) ) ;
#13228=CARTESIAN_POINT ( 'NONE',  ( 114.6950545185401609, -40.57145610743049247, 202.8781341137909635 ) ) ;
#13229=CARTESIAN_POINT ( 'NONE',  ( 96.67089207319645539, -38.24056507437282448, 66.44133956162495735 ) ) ;
#13231=ORIENTED_EDGE ( 'NONE', *, *, #24360, .T. ) ;
#13235=CARTESIAN_POINT ( 'NONE',  ( 87.06648329127402519, -54.72944906728955061, 14.67562527591094934 ) ) ;
#13240=CARTESIAN_POINT ( 'NONE',  ( 110.8543353071601558, -45.98429331485927918, 132.8856134878540729 ) ) ;
#13241=AXIS2_PLACEMENT_3D ( 'NONE', #69328, #25744, #54315 ) ;
#13243=ORIENTED_EDGE ( 'NONE', *, *, #20579, .F. ) ;
#13244=CARTESIAN_POINT ( 'NONE',  ( 115.7470646134707266, -43.61006842878475709, 48.30514908543492680 ) ) ;
#13245=DIRECTION ( 'NONE',  ( 0.000000000000000000, 0.000000000000000000, 1.000000000000000000 ) ) ;
#13247=DIRECTION ( 'NONE',  ( 0.7071067811865597852, -0.7071067811865354713, 0.000000000000000000 ) ) ;
#13248=CARTESIAN_POINT ( 'NONE',  ( 131.4836309258849667, -17.78502016655529161, 2.871594975603859456 ) ) ;
#13249=ORIENTED_EDGE ( 'NONE', *, *, #19436, .F. ) ;
#13250=AXIS2_PLACEMENT_3D ( 'NONE', #20705, #56088, #22502 ) ;
#13251=CARTESIAN_POINT ( 'NONE',  ( 179.7974245136200295, -36.32844715994041707, 342.9256252759109884 ) ) ;
#13252=CIRCLE ( 'NONE', #43646, 2.749999999999974687 ) ;
#13255=ORIENTED_EDGE ( 'NONE', *, *, #51396, .F. ) ;
#13257=CARTESIAN_POINT ( 'NONE',  ( 102.9625221110550513, -46.33646342331733337, 88.25562527591095829 ) ) ;
#13258=DIRECTION ( 'NONE',  ( 0.08544974978095688789, 0.9963424814100680926, 0.000000000000000000 ) ) ;
#13259=DIRECTION ( 'NONE',  ( 0.000000000000000000, 0.000000000000000000, -1.000000000000000000 ) ) ;
#13261=EDGE_CURVE ( 'NONE', #50282, #59961, #67782, .T. ) ;
#13264=CARTESIAN_POINT ( 'NONE',  ( 102.6819511611811180, -27.33185899950651887, 131.4118157521009778 ) ) ;
#13267=VECTOR ( 'NONE', #83638, 1000.000000000000114 ) ;
#13268=CARTESIAN_POINT ( 'NONE',  ( 111.4711666614668673, -26.61707918639095993, 280.7375300378156453 ) ) ;
#13269=DIRECTION ( 'NONE',  ( 0.000000000000000000, 0.000000000000000000, -1.000000000000000000 ) ) ;
#13271=DIRECTION ( 'NONE',  ( 0.9242245927363033076, 0.3818493186865917766, 0.000000000000000000 ) ) ;
#13272=CARTESIAN_POINT ( 'NONE',  ( 107.0664832912739968, -36.72944715994100306, 293.2242906452868851 ) ) ;
#13274=CARTESIAN_POINT ( 'NONE',  ( 75.31670390244798341, -67.87844715994100397, 35.51780685541480409 ) ) ;
#13275=CARTESIAN_POINT ( 'NONE',  ( 106.5196382177906855, -25.62481104856546565, 195.1156252759109861 ) ) ;
#13276=EDGE_LOOP ( 'NONE', ( #40660, #668, #69729, #15122 ) ) ;
#13277=VECTOR ( 'NONE', #20055, 1000.000000000000000 ) ;
#13279=CARTESIAN_POINT ( 'NONE',  ( 100.0737993132363783, -29.47871783549896918, 112.1187261630399661 ) ) ;
#13280=CIRCLE ( 'NONE', #48078, 2.500000000000002220 ) ;
#13281=DIRECTION ( 'NONE',  ( 1.000000000000000000, 0.000000000000000000, 0.000000000000000000 ) ) ;
#13282=CARTESIAN_POINT ( 'NONE',  ( 109.2301907924558009, -26.89130329018268739, 26.33586902018297948 ) ) ;
#13283=CARTESIAN_POINT ( 'NONE',  ( 172.5664832912740110, -9.303447159940999356, 141.0426252759120018 ) ) ;
#13284=CARTESIAN_POINT ( 'NONE',  ( 141.8664832912740223, -71.52944715994085811, 394.9756252759100903 ) ) ;
#13287=DIRECTION ( 'NONE',  ( 0.4999999926578935772, 8.568612280667725471E-05, -0.8660254037844357100 ) ) ;
#13288=DIRECTION ( 'NONE',  ( 1.000000000000000000, 4.163336342344333240E-14, 0.000000000000000000 ) ) ;
#13289=DIRECTION ( 'NONE',  ( 0.000000000000000000, 0.000000000000000000, -1.000000000000000000 ) ) ;
#13290=EDGE_CURVE ( 'NONE', #6003, #28799, #71869, .T. ) ;
#13291=DIRECTION ( 'NONE',  ( -2.900000000000000265E-14, 2.000000000000000155E-15, -1.000000000000000000 ) ) ;
#13292=CARTESIAN_POINT ( 'NONE',  ( 113.7851844261090264, -26.99768152489561501, 239.5956252759109759 ) ) ;
#13294=ORIENTED_EDGE ( 'NONE', *, *, #64465, .T. ) ;
#13295=ORIENTED_EDGE ( 'NONE', *, *, #64773, .T. ) ;
#13296=AXIS2_PLACEMENT_3D ( 'NONE', #13611, #68584, #66894 ) ;
#13299=DIRECTION ( 'NONE',  ( -1.000000000000000000, -3.999999999999999995E-14, -1.000000000000000078E-15 ) ) ;
#13300=CARTESIAN_POINT ( 'NONE',  ( 113.2462366615943381, -28.75923750785663557, 184.5526495355683494 ) ) ;
#13303=CARTESIAN_POINT ( 'NONE',  ( 31.85959712127300847, -23.19206098994090581, -5.074374724088000832 ) ) ;
#13306=CARTESIAN_POINT ( 'NONE',  ( 117.1924066864372520, -41.16168844948898453, 208.4861014663869696 ) ) ;
#13307=VERTEX_POINT ( 'NONE', #89583 ) ;
#13308=EDGE_CURVE ( 'NONE', #22291, #15780, #83665, .T. ) ;
#13309=VECTOR ( 'NONE', #56674, 1000.000000000000000 ) ;
#13310=LINE ( 'NONE', #46457, #62190 ) ;
#13311=CARTESIAN_POINT ( 'NONE',  ( 51.24204729617191845, -31.76306994223782709, 117.4678068554150485 ) ) ;
#13312=CARTESIAN_POINT ( 'NONE',  ( 117.0903339436451347, -37.63109343375219140, 168.7546943088809996 ) ) ;
#13313=CIRCLE ( 'NONE', #30693, 0.1500000000000008271 ) ;
#13314=CARTESIAN_POINT ( 'NONE',  ( 112.0375358597863027, -29.64498801284190321, 82.39570941720997155 ) ) ;
#13315=CARTESIAN_POINT ( 'NONE',  ( 103.8005819418147411, -26.80618422321597194, 161.3299109901969643 ) ) ;
#13319=CARTESIAN_POINT ( 'NONE',  ( 97.84153879744087590, -40.58974903926429789, 66.64233031300194909 ) ) ;
#13323=ORIENTED_EDGE ( 'NONE', *, *, #26929, .T. ) ;
#13325=CARTESIAN_POINT ( 'NONE',  ( 172.5664832912740110, -36.32844715994070839, 78.92562527591199739 ) ) ;
#13326=CARTESIAN_POINT ( 'NONE',  ( 100.1216203692562630, -42.54163687813885275, 71.29146744712500094 ) ) ;
#13327=CARTESIAN_POINT ( 'NONE',  ( 105.1067973254952790, -26.46757623491196298, 235.2270538473399313 ) ) ;
#13328=CIRCLE ( 'NONE', #64108, 2.999999999999947153 ) ;
#13329=CARTESIAN_POINT ( 'NONE',  ( 110.0457755916377778, -26.10929462018208369, 219.8708633711489711 ) ) ;
#13330=DIRECTION ( 'NONE',  ( 0.000000000000000000, 0.000000000000000000, -1.000000000000000000 ) ) ;
#13331=CARTESIAN_POINT ( 'NONE',  ( 102.3792474187797694, -47.61030217832540501, 283.2527681330539053 ) ) ;
#13332=DIRECTION ( 'NONE',  ( -4.237773401492740281E-14, 1.000000000000000000, 0.000000000000000000 ) ) ;
#13333=FACE_OUTER_BOUND ( 'NONE', #49159, .T. ) ;
#13334=CARTESIAN_POINT ( 'NONE',  ( 125.0664832912740110, -14.47844715994100007, 284.9256252759119548 ) ) ;
#13336=ORIENTED_EDGE ( 'NONE', *, *, #384, .F. ) ;
#13337=CIRCLE ( 'NONE', #42354, 2.116999999999993776 ) ;
#13339=CIRCLE ( 'NONE', #85857, 2.500000000000002220 ) ;
#13340=CARTESIAN_POINT ( 'NONE',  ( 117.3261810260836597, -38.23854875528750341, 73.72229194257801055 ) ) ;
#13341=CARTESIAN_POINT ( 'NONE',  ( 98.82309110046458045, -43.24084327085208912, 91.85848241876892928 ) ) ;
#13342=CARTESIAN_POINT ( 'NONE',  ( 110.9088526855213388, -26.95253601363527807, 269.7784824187680783 ) ) ;
#13344=CARTESIAN_POINT ( 'NONE',  ( 118.0409265538620787, -35.41009787725452185, 238.9337205140059552 ) ) ;
#13345=DIRECTION ( 'NONE',  ( -0.000000000000000000, -0.000000000000000000, 1.000000000000000000 ) ) ;
#13347=EDGE_CURVE ( 'NONE', #1145, #7741, #34109, .T. ) ;
#13349=DIRECTION ( 'NONE',  ( 1.000000000000000000, 4.299999999999999979E-14, 1.000000000000000078E-15 ) ) ;
#13350=CARTESIAN_POINT ( 'NONE',  ( 115.2577283620428545, -37.00732651667798478, 277.6356252759109680 ) ) ;
#13352=DIRECTION ( 'NONE',  ( 0.000000000000000000, -1.000000000000000000, 4.100000000000000342E-29 ) ) ;
#13354=LINE ( 'NONE', #7874, #89095 ) ;
#13355=LINE ( 'NONE', #6533, #87857 ) ;
#13356=DIRECTION ( 'NONE',  ( 0.000000000000000000, 0.000000000000000000, -1.000000000000000000 ) ) ;
#13357=CARTESIAN_POINT ( 'NONE',  ( 98.34985891999399144, -31.65658479692842064, 76.90645860808798773 ) ) ;
#13358=AXIS2_PLACEMENT_3D ( 'NONE', #36651, #64352, #57523 ) ;
#13359=CARTESIAN_POINT ( 'NONE',  ( 97.33784130179184046, -34.07106456304081377, 261.1147919453016470 ) ) ;
#13360=ORIENTED_EDGE ( 'NONE', *, *, #73947, .F. ) ;
#13362=CARTESIAN_POINT ( 'NONE',  ( 102.2269548454591046, -45.98824451103227062, 212.1927681330539599 ) ) ;
#13363=CARTESIAN_POINT ( 'NONE',  ( 98.28086921530724851, -31.05189054518432101, 141.8699109901969564 ) ) ;
#13364=CARTESIAN_POINT ( 'NONE',  ( 112.5120184049100089, -46.40124356417671692, 253.9965776568635647 ) ) ;
#13365=DIRECTION ( 'NONE',  ( 0.7071067811862239427, 0.7071067811868709807, 0.000000000000000000 ) ) ;
#13366=CARTESIAN_POINT ( 'NONE',  ( 192.5667039024474434, -23.42844715993413374, 180.4678068554150343 ) ) ;
#13367=CARTESIAN_POINT ( 'NONE',  ( 134.0664832912740110, -46.72944715994100306, 10.42562527591099553 ) ) ;
#13368=DIRECTION ( 'NONE',  ( 1.000000000000000078E-15, -1.000000000000000000, 0.000000000000000000 ) ) ;
#13369=VECTOR ( 'NONE', #68773, 1000.000000000000000 ) ;
#13371=VECTOR ( 'NONE', #75329, 1000.000000000000000 ) ;
#13372=ADVANCED_FACE ( 'NONE', ( #76839 ), #7797, .T. ) ;
#13376=CARTESIAN_POINT ( 'NONE',  ( 115.7815527111783069, -39.19119195442627301, 143.0419436376009799 ) ) ;
#13378=ORIENTED_EDGE ( 'NONE', *, *, #18812, .F. ) ;
#13379=CARTESIAN_POINT ( 'NONE',  ( 107.2792697713003776, -24.20934055526686279, 321.5865679059475610 ) ) ;
#13380=CARTESIAN_POINT ( 'NONE',  ( 108.9412587213990804, -26.46057952311826611, 160.9327681330539690 ) ) ;
#13381=LINE ( 'NONE', #61958, #80195 ) ;
#13385=DIRECTION ( 'NONE',  ( 0.000000000000000000, 1.000000000000000000, 1.541976423090495239E-15 ) ) ;
#13386=CARTESIAN_POINT ( 'NONE',  ( 116.3126599349421895, -33.43976754494798342, 114.0984824187689668 ) ) ;
#13387=ORIENTED_EDGE ( 'NONE', *, *, #44959, .T. ) ;
#13388=ORIENTED_EDGE ( 'NONE', *, *, #88668, .F. ) ;
#13390=CARTESIAN_POINT ( 'NONE',  ( 181.9790560690451855, -31.62489322948519543, 342.9256252759109884 ) ) ;
#13391=CARTESIAN_POINT ( 'NONE',  ( 118.1851208724671238, -36.91582462397654751, 149.8127681330539644 ) ) ;
#13393=CARTESIAN_POINT ( 'NONE',  ( 115.0894923806533967, -30.61840087513353836, 54.34358037573613842 ) ) ;
#13394=LINE ( 'NONE', #21561, #85805 ) ;
#13395=EDGE_CURVE ( 'NONE', #19112, #29616, #14169, .T. ) ;
#13396=LINE ( 'NONE', #82901, #85196 ) ;
#13397=VECTOR ( 'NONE', #69455, 1000.000000000000000 ) ;
#13398=CARTESIAN_POINT ( 'NONE',  ( 61.56670390244727287, -23.42844715994043980, 300.4678068554150627 ) ) ;
#13399=EDGE_CURVE ( 'NONE', #72149, #24293, #735, .T. ) ;
#13400=FACE_OUTER_BOUND ( 'NONE', #64661, .T. ) ;
#13401=CARTESIAN_POINT ( 'NONE',  ( 115.2499566122393588, -44.12502604085376134, 83.25372051400698581 ) ) ;
#13402=ORIENTED_EDGE ( 'NONE', *, *, #6584, .F. ) ;
#13404=VERTEX_POINT ( 'NONE', #21889 ) ;
#13405=ORIENTED_EDGE ( 'NONE', *, *, #72997, .T. ) ;
#13406=EDGE_CURVE ( 'NONE', #89397, #54515, #73269, .T. ) ;
#13407=CARTESIAN_POINT ( 'NONE',  ( 46.83715912545343940, -47.82818131006086304, 129.9678068554150911 ) ) ;
#13408=CARTESIAN_POINT ( 'NONE',  ( 62.03715912545748523, -47.82818131006020934, 193.9678068554150911 ) ) ;
#13411=CARTESIAN_POINT ( 'NONE',  ( 114.6839398542181101, -39.73893943580953447, 191.3452332267339671 ) ) ;
#13413=CARTESIAN_POINT ( 'NONE',  ( 62.03715912545744260, -47.82818131006020934, 129.9678068554150911 ) ) ;
#13415=ORIENTED_EDGE ( 'NONE', *, *, #34709, .F. ) ;
#13418=LINE ( 'NONE', #27042, #4718 ) ;
#13419=CARTESIAN_POINT ( 'NONE',  ( 107.0667039024479834, -48.82844715994099971, 160.9178068554150229 ) ) ;
#13421=VERTEX_POINT ( 'NONE', #51346 ) ;
#13423=CARTESIAN_POINT ( 'NONE',  ( 103.6867908865108916, -46.21882986916993730, 248.7358690201829745 ) ) ;
#13424=EDGE_LOOP ( 'NONE', ( #3513, #52034, #18567, #39323 ) ) ;
#13425=FACE_OUTER_BOUND ( 'NONE', #10685, .T. ) ;
#13427=VERTEX_POINT ( 'NONE', #37748 ) ;
#13428=ORIENTED_EDGE ( 'NONE', *, *, #65899, .F. ) ;
#13429=AXIS2_PLACEMENT_3D ( 'NONE', #40689, #69305, #21613 ) ;
#13432=ORIENTED_EDGE ( 'NONE', *, *, #87176, .F. ) ;
#13434=CARTESIAN_POINT ( 'NONE',  ( 100.6713832604498577, -30.89818480590637861, 228.5442808457819979 ) ) ;
#13435=CARTESIAN_POINT ( 'NONE',  ( 108.9889396673064397, -47.63814106062356757, 122.7032443235299723 ) ) ;
#13436=CARTESIAN_POINT ( 'NONE',  ( 98.16825066461156268, -43.24752039522714142, 106.8175300378159704 ) ) ;
#13437=CARTESIAN_POINT ( 'NONE',  ( 104.1307268678290683, -28.83426272247936240, 249.5838068554171798 ) ) ;
#13438=CARTESIAN_POINT ( 'NONE',  ( 133.0522658619983360, -16.17316201338587689, 8.065992442478552960 ) ) ;
#13439=CARTESIAN_POINT ( 'NONE',  ( 98.55127668717894096, -44.97116251829300637, 187.9384824187679612 ) ) ;
#13444=VERTEX_POINT ( 'NONE', #16853 ) ;
#13446=ORIENTED_EDGE ( 'NONE', *, *, #73220, .F. ) ;
#13447=EDGE_CURVE ( 'NONE', #2655, #82610, #6567, .T. ) ;
#13449=CARTESIAN_POINT ( 'NONE',  ( 117.3714642245996629, -32.73114059124436892, 94.10895860924395606 ) ) ;
#13453=FACE_OUTER_BOUND ( 'NONE', #60971, .T. ) ;
#13456=CARTESIAN_POINT ( 'NONE',  ( 106.8520627977276973, -47.75749532952657006, 223.5489586092439538 ) ) ;
#13457=CARTESIAN_POINT ( 'NONE',  ( 107.0664832912739399, -36.72944715994095333, 302.7856252759109452 ) ) ;
#13458=CARTESIAN_POINT ( 'NONE',  ( 48.16670390244701139, -26.71338133339251542, 237.4678068554150059 ) ) ;
#13460=DIRECTION ( 'NONE',  ( -2.900000000000000265E-14, 2.000000000000000155E-15, -1.000000000000000000 ) ) ;
#13465=CARTESIAN_POINT ( 'NONE',  ( 97.12779447186500192, -40.02021159927672755, 241.5813395616249863 ) ) ;
#13466=ORIENTED_EDGE ( 'NONE', *, *, #41999, .F. ) ;
#13468=CARTESIAN_POINT ( 'NONE',  ( 108.3221154657901337, -47.10103102204929826, 117.6727681330539639 ) ) ;
#13469=CARTESIAN_POINT ( 'NONE',  ( 101.1417250294410337, -28.10862513908322313, 46.55562527591094835 ) ) ;
#13470=CARTESIAN_POINT ( 'NONE',  ( 98.82232569344716921, -30.27743405825323464, 151.7984824187679465 ) ) ;
#13472=CARTESIAN_POINT ( 'NONE',  ( 100.9547954897877702, -28.70692885872499289, 101.5939034364447338 ) ) ;
#13474=DIRECTION ( 'NONE',  ( 1.000000000000000000, 4.299999999999999979E-14, 1.000000000000000078E-15 ) ) ;
#13475=PLANE ( 'NONE',  #20536 ) ;
#13476=CARTESIAN_POINT ( 'NONE',  ( 192.5667039024473013, -23.42844715993434335, 249.9678068554149775 ) ) ;
#13477=VERTEX_POINT ( 'NONE', #77745 ) ;
#13478=VECTOR ( 'NONE', #18663, 1000.000000000000000 ) ;
#13480=EDGE_CURVE ( 'NONE', #28839, #2851, #23248, .T. ) ;
#13481=ORIENTED_EDGE ( 'NONE', *, *, #61280, .F. ) ;
#13482=ORIENTED_EDGE ( 'NONE', *, *, #61178, .T. ) ;
#13485=CARTESIAN_POINT ( 'NONE',  ( 116.7068942081671423, -31.36975501082244477, 25.24229194257798881 ) ) ;
#13486=CARTESIAN_POINT ( 'NONE',  ( 96.41083957889333078, -31.77770432788677013, 4.925625275910959999 ) ) ;
#13487=CARTESIAN_POINT ( 'NONE',  ( 107.0664832912739968, 12.92155284005902516, 330.1506252759110680 ) ) ;
#13488=EDGE_CURVE ( 'NONE', #26370, #68689, #56824, .T. ) ;
#13489=CARTESIAN_POINT ( 'NONE',  ( 102.9499971297430250, -26.42158413985995580, 171.3908633711489813 ) ) ;
#13490=LINE ( 'NONE', #33922, #6963 ) ;
#13491=CARTESIAN_POINT ( 'NONE',  ( 101.9513324583280962, -44.20259256747556975, 241.5333722090289825 ) ) ;
#13493=ORIENTED_EDGE ( 'NONE', *, *, #19893, .T. ) ;
#13495=VECTOR ( 'NONE', #13129, 1000.000000000000000 ) ;
#13497=CARTESIAN_POINT ( 'NONE',  ( 115.7832426263078958, -41.80208187097057504, 103.4062359794634176 ) ) ;
#13502=DIRECTION ( 'NONE',  ( -1.000000000000000000, -8.843517682682131024E-16, -1.000000000000000078E-15 ) ) ;
#13503=CONICAL_SURFACE ( 'NONE', #7729, 1.571100913904388552, 1.047197551196592302 ) ;
#13504=CARTESIAN_POINT ( 'NONE',  ( 48.45959712127301344, -26.00627455219131789, 237.4678068554150059 ) ) ;
#13505=DIRECTION ( 'NONE',  ( 5.512527431108029424E-15, -1.000000000000000000, 0.000000000000000000 ) ) ;
#13506=CARTESIAN_POINT ( 'NONE',  ( 97.54182784580959265, -34.36413255816223966, 276.1327681330543555 ) ) ;
#13507=EDGE_CURVE ( 'NONE', #7448, #58550, #36772, .T. ) ;
#13508=LINE ( 'NONE', #27133, #86470 ) ;
#13509=ORIENTED_EDGE ( 'NONE', *, *, #41356, .F. ) ;
#13510=FACE_OUTER_BOUND ( 'NONE', #63363, .T. ) ;
#13511=B_SPLINE_CURVE_WITH_KNOTS ( 'NONE', 3,
 ( #19048, #67645, #5430, #33126, #54429, #60820, #82192, #22200, #7661, #36718, #77157, #78514, #2650, #16274, #48965, #77601, #42600, #63064 ),
 .UNSPECIFIED., .F., .F.,
 ( 4, 2, 2, 2, 2, 2, 2, 2, 4 ),
 ( 0.5000000002356785878, 0.5625000002062188198, 0.6250000001767589408, 0.6875000001472990618, 0.7500000001178392939, 0.8125000000883795259, 0.8750000000589196469, 0.9375000000294597680, 1.000000000000000000 ),
 .UNSPECIFIED. ) ;
#13512=CARTESIAN_POINT ( 'NONE',  ( 141.8664832912739939, -71.52944715994085811, 361.9756252759100335 ) ) ;
#13513=CARTESIAN_POINT ( 'NONE',  ( 98.47016933319702048, -37.73160053143655546, 84.24904275054394986 ) ) ;
#13514=AXIS2_PLACEMENT_3D ( 'NONE', #9132, #36829, #29565 ) ;
#13515=DIRECTION ( 'NONE',  ( -0.9999999853157766072, -0.0001713722456150811827, 0.000000000000000000 ) ) ;
#13516=CARTESIAN_POINT ( 'NONE',  ( 168.0371591254545649, -48.62818131005499112, 180.4678068554150059 ) ) ;
#13517=ORIENTED_EDGE ( 'NONE', *, *, #37307, .T. ) ;
#13518=ADVANCED_FACE ( 'NONE', ( #37293 ), #63662, .T. ) ;
#13519=CARTESIAN_POINT ( 'NONE',  ( 79.41328093383648934, -34.05633243510678909, 8.161687850944868927 ) ) ;
#13520=AXIS2_PLACEMENT_3D ( 'NONE', #69574, #42291, #13269 ) ;
#13521=ORIENTED_EDGE ( 'NONE', *, *, #35833, .F. ) ;
#13522=CARTESIAN_POINT ( 'NONE',  ( 97.83587340921722841, -31.88353427759474457, 135.9413395616259947 ) ) ;
#13523=ORIENTED_EDGE ( 'NONE', *, *, #72969, .F. ) ;
#13526=CARTESIAN_POINT ( 'NONE',  ( 105.2783438540041061, -26.81616000048136428, 121.6501547344689698 ) ) ;
#13527=PLANE ( 'NONE',  #57700 ) ;
#13529=CARTESIAN_POINT ( 'NONE',  ( 96.69317630666223806, -38.23732580652426094, 62.44133956162495025 ) ) ;
#13530=AXIS2_PLACEMENT_3D ( 'NONE', #32167, #59862, #11279 ) ;
#13531=CARTESIAN_POINT ( 'NONE',  ( 115.7831076651936257, -41.80230951900219338, 84.40645860845914683 ) ) ;
#13533=CARTESIAN_POINT ( 'NONE',  ( 188.5667039024480971, -42.82844715993431350, 293.2178068554150059 ) ) ;
#13534=ORIENTED_EDGE ( 'NONE', *, *, #29495, .F. ) ;
#13535=ORIENTED_EDGE ( 'NONE', *, *, #42767, .F. ) ;
#13538=CARTESIAN_POINT ( 'NONE',  ( 100.6687104586878547, -44.89077600197693130, 277.0594347997210889 ) ) ;
#13539=CARTESIAN_POINT ( 'NONE',  ( 108.9491117623569636, -26.41756539094687639, 160.9327681330539690 ) ) ;
#13540=DIRECTION ( 'NONE',  ( -0.9254794337955620787, -0.3787978585227822492, 0.000000000000000000 ) ) ;
#13541=CARTESIAN_POINT ( 'NONE',  ( 99.09570908213733276, -30.55043174551792262, 141.8022919418074821 ) ) ;
#13542=CARTESIAN_POINT ( 'NONE',  ( 115.2072660578295284, -44.20618685261739245, 74.22324432352993995 ) ) ;
#13543=CARTESIAN_POINT ( 'NONE',  ( 97.06098806315000616, -37.99597704668403253, 97.42732106492178445 ) ) ;
#13545=DIRECTION ( 'NONE',  ( -1.000000000000000078E-15, 1.000000000000000083E-30, 1.000000000000000000 ) ) ;
#13546=CARTESIAN_POINT ( 'NONE',  ( 100.8875641163020873, -44.70030114050455694, 158.0521118432647825 ) ) ;
#13548=AXIS2_PLACEMENT_3D ( 'NONE', #80722, #89326, #60245 ) ;
#13549=DIRECTION ( 'NONE',  ( 1.000000000000000078E-15, 0.000000000000000000, -1.000000000000000000 ) ) ;
#13550=DIRECTION ( 'NONE',  ( 1.000000000000000078E-15, -1.000000000000000083E-30, -1.000000000000000000 ) ) ;
#13551=CARTESIAN_POINT ( 'NONE',  ( 100.2624651760415304, -28.85963121439194623, 260.6441967044822263 ) ) ;
#13552=CYLINDRICAL_SURFACE ( 'NONE', #60568, 0.2499999999999941991 ) ;
#13553=AXIS2_PLACEMENT_3D ( 'NONE', #5518, #76336, #81387 ) ;
#13556=CARTESIAN_POINT ( 'NONE',  ( 116.1300133678986413, -31.69047823903573047, 29.24229194257799236 ) ) ;
#13557=CARTESIAN_POINT ( 'NONE',  ( 97.76673074818263842, -40.40594551311712479, 101.6265170135205409 ) ) ;
#13558=CARTESIAN_POINT ( 'NONE',  ( 116.8835868046512587, -40.17228670562622739, 129.5584824187679658 ) ) ;
#13559=CARTESIAN_POINT ( 'NONE',  ( 168.0371591254546217, -48.62818131005519007, 129.9678068554150059 ) ) ;
#13560=CARTESIAN_POINT ( 'NONE',  ( 99.38968898744698777, -27.63536841754259044, 150.6356252759109680 ) ) ;
#13562=ORIENTED_EDGE ( 'NONE', *, *, #2308, .T. ) ;
#13563=DIRECTION ( 'NONE',  ( -0.9254794337955620787, -0.3787978585227822492, 0.000000000000000000 ) ) ;
#13565=CARTESIAN_POINT ( 'NONE',  ( 135.7756147485175688, -34.57277681851078199, 2.101554741580191621 ) ) ;
#13567=CARTESIAN_POINT ( 'NONE',  ( 51.23005224011609471, -33.89581943344337134, 193.9678068554150911 ) ) ;
#13568=CARTESIAN_POINT ( 'NONE',  ( 98.24359417337518607, -31.02780217081950909, 145.8699109901969848 ) ) ;
#13569=ORIENTED_EDGE ( 'NONE', *, *, #51953, .T. ) ;
#13572=FACE_OUTER_BOUND ( 'NONE', #398, .T. ) ;
#13574=EDGE_LOOP ( 'NONE', ( #43306, #47920, #79196, #7578 ) ) ;
#13575=ADVANCED_FACE ( 'NONE', ( #22331, #50011, #15519, #43194, #8712 ), #36414, .F. ) ;
#13579=EDGE_LOOP ( 'NONE', ( #31062, #17886, #80557, #88713 ) ) ;
#13580=ADVANCED_FACE ( 'NONE', ( #17743, #10921 ), #73138, .T. ) ;
#13581=AXIS2_PLACEMENT_3D ( 'NONE', #8028, #55252, #7136 ) ;
#13583=DIRECTION ( 'NONE',  ( 1.000000000000000078E-15, 1.000000000000000083E-30, -1.000000000000000000 ) ) ;
#13584=CARTESIAN_POINT ( 'NONE',  ( 98.43498668633466764, -29.82501040932825020, 191.7775300378159784 ) ) ;
#13589=FACE_OUTER_BOUND ( 'NONE', #4339, .T. ) ;
#13591=DIRECTION ( 'NONE',  ( 0.000000000000000000, 0.000000000000000000, -1.000000000000000000 ) ) ;
#13592=ORIENTED_EDGE ( 'NONE', *, *, #88566, .T. ) ;
#13593=EDGE_CURVE ( 'NONE', #50094, #81819, #82060, .T. ) ;
#13596=EDGE_LOOP ( 'NONE', ( #82709, #84404 ) ) ;
#13597=CARTESIAN_POINT ( 'NONE',  ( 37.56670390244833158, -48.82844715994119866, 249.9678068554150343 ) ) ;
#13600=CARTESIAN_POINT ( 'NONE',  ( 111.3277751695582651, -45.53312973143654574, 243.9356252759109509 ) ) ;
#13601=LINE ( 'NONE', #76727, #42879 ) ;
#13602=CARTESIAN_POINT ( 'NONE',  ( 97.42673588038243793, -38.38435052442952866, 87.46133956162493917 ) ) ;
#13604=CARTESIAN_POINT ( 'NONE',  ( 110.9562181391215745, -45.94203628685212237, 52.89439067654506488 ) ) ;
#13606=CARTESIAN_POINT ( 'NONE',  ( 103.4003208981030753, -27.42560052542062721, 21.37517646364080903 ) ) ;
#13607=VERTEX_POINT ( 'NONE', #81338 ) ;
#13610=EDGE_LOOP ( 'NONE', ( #3963, #71787, #56089, #16214 ) ) ;
#13611=CARTESIAN_POINT ( 'NONE',  ( 180.1667039024475230, -28.27351298636767396, 237.4678068554150059 ) ) ;
#13612=CARTESIAN_POINT ( 'NONE',  ( 100.6682639674293114, -30.55490919580550013, 247.1472975916109647 ) ) ;
#13614=CARTESIAN_POINT ( 'NONE',  ( 100.8874677989195447, -44.70022130964055407, 192.0522919340818362 ) ) ;
#13615=DIRECTION ( 'NONE',  ( 0.000000000000000000, 1.000000000000000000, 0.000000000000000000 ) ) ;
#13616=FACE_BOUND ( 'NONE', #83998, .T. ) ;
#13618=ORIENTED_EDGE ( 'NONE', *, *, #89695, .T. ) ;
#13621=CARTESIAN_POINT ( 'NONE',  ( 112.0640919193708243, -45.48941087331174771, 183.9901923727738620 ) ) ;
#13622=ORIENTED_EDGE ( 'NONE', *, *, #75159, .F. ) ;
#13623=CARTESIAN_POINT ( 'NONE',  ( 96.17734138947662359, -38.62830894954290528, 46.45181575210094138 ) ) ;
#13625=EDGE_CURVE ( 'NONE', #40317, #1757, #39068, .T. ) ;
#13626=CARTESIAN_POINT ( 'NONE',  ( 105.1260075982565212, -28.80065313513137326, 283.0852332267343172 ) ) ;
#13629=CARTESIAN_POINT ( 'NONE',  ( 98.32242264099468798, -42.30440888850458947, 141.7661014663879655 ) ) ;
#13630=CARTESIAN_POINT ( 'NONE',  ( 107.0664832912739968, -8.729447159940999512, 6.425625275911999168 ) ) ;
#13631=DIRECTION ( 'NONE',  ( -1.175184669632759901E-16, 1.000000000000000000, 2.000000000000003705E-15 ) ) ;
#13632=CARTESIAN_POINT ( 'NONE',  ( 94.86917197795300183, -31.06128196069623471, 25.56312527591095574 ) ) ;
#13635=CARTESIAN_POINT ( 'NONE',  ( 114.6369858128092858, -29.49892357452570124, 230.4327681330539690 ) ) ;
#13638=CIRCLE ( 'NONE', #31007, 2.030000000000003801 ) ;
#13639=ORIENTED_EDGE ( 'NONE', *, *, #6931, .T. ) ;
#13640=CARTESIAN_POINT ( 'NONE',  ( 95.43962894333766656, -34.19422119854147013, 102.1556252759109640 ) ) ;
#13643=VECTOR ( 'NONE', #32988, 1000.000000000000000 ) ;
#13645=VERTEX_POINT ( 'NONE', #74493 ) ;
#13647=AXIS2_PLACEMENT_3D ( 'NONE', #86574, #43876, #71168 ) ;
#13648=FACE_OUTER_BOUND ( 'NONE', #9871, .T. ) ;
#13652=CARTESIAN_POINT ( 'NONE',  ( 103.6346955097220643, -29.32319583828803999, 178.2395189410199805 ) ) ;
#13653=CARTESIAN_POINT ( 'NONE',  ( 110.7407540106703010, -26.28028736477551419, 250.8194347997206819 ) ) ;
#13654=DIRECTION ( 'NONE',  ( -1.000000000000000000, -4.163336342344333240E-14, 0.000000000000000000 ) ) ;
#13655=ORIENTED_EDGE ( 'NONE', *, *, #63390, .T. ) ;
#13657=DIRECTION ( 'NONE',  ( -0.000000000000000000, 0.000000000000000000, -1.000000000000000000 ) ) ;
#13658=ORIENTED_EDGE ( 'NONE', *, *, #66431, .F. ) ;
#13660=DIRECTION ( 'NONE',  ( 1.000000000000000000, 4.163336342344333240E-14, 0.000000000000000000 ) ) ;
#13662=DIRECTION ( 'NONE',  ( 1.000000000000000078E-15, -1.000000000000000083E-30, -1.000000000000000000 ) ) ;
#13663=CARTESIAN_POINT ( 'NONE',  ( 102.0669959706335561, -27.97053095873570427, 15.48979716230626913 ) ) ;
#13664=DIRECTION ( 'NONE',  ( 1.000000000000000000, -5.337610695313248426E-16, 0.000000000000000000 ) ) ;
#13665=DIRECTION ( 'NONE',  ( -0.7071067811571960515, 0.7071067812158990940, 0.000000000000000000 ) ) ;
#13666=CARTESIAN_POINT ( 'NONE',  ( 107.5482541545970605, -45.77270802984816811, 197.0533722090289643 ) ) ;
#13667=CARTESIAN_POINT ( 'NONE',  ( 118.0484485056734769, -38.34478726580598362, 73.72229194257801055 ) ) ;
#13668=VERTEX_POINT ( 'NONE', #10480 ) ;
#13669=CARTESIAN_POINT ( 'NONE',  ( 182.4202572930265660, -31.94127993907054730, 313.9678068554149490 ) ) ;
#13670=ORIENTED_EDGE ( 'NONE', *, *, #82936, .F. ) ;
#13672=ORIENTED_EDGE ( 'NONE', *, *, #18764, .T. ) ;
#13674=ORIENTED_EDGE ( 'NONE', *, *, #43727, .T. ) ;
#13677=CARTESIAN_POINT ( 'NONE',  ( 194.0371591254575776, -24.89890238294407254, 129.9678068554150343 ) ) ;
#13679=VERTEX_POINT ( 'NONE', #38181 ) ;
#13680=CARTESIAN_POINT ( 'NONE',  ( 101.1290945223330198, -28.09024711436062915, 50.55562527591095545 ) ) ;
#13681=VECTOR ( 'NONE', #86406, 1000.000000000000000 ) ;
#13683=DIRECTION ( 'NONE',  ( -0.000000000000000000, 1.000000000000000000, 0.000000000000000000 ) ) ;
#13686=ADVANCED_FACE ( 'NONE', ( #73593 ), #4563, .F. ) ;
#13687=DIRECTION ( 'NONE',  ( 0.000000000000000000, 1.000000000000000000, 0.000000000000000000 ) ) ;
#13688=ORIENTED_EDGE ( 'NONE', *, *, #17723, .F. ) ;
#13690=DIRECTION ( 'NONE',  ( 0.000000000000000000, -1.000000000000000000, 0.000000000000000000 ) ) ;
#13694=VERTEX_POINT ( 'NONE', #34938 ) ;
#13695=CARTESIAN_POINT ( 'NONE',  ( 96.06465719955961902, -38.01203376208108153, 82.43086337114895912 ) ) ;
#13696=CARTESIAN_POINT ( 'NONE',  ( 20.03715912545736799, -24.42818131006189830, 237.4678068554150059 ) ) ;
#13697=PLANE ( 'NONE',  #10841 ) ;
#13700=AXIS2_PLACEMENT_3D ( 'NONE', #84146, #22360, #85497 ) ;
#13701=AXIS2_PLACEMENT_3D ( 'NONE', #11915, #39163, #48195 ) ;
#13702=AXIS2_PLACEMENT_3D ( 'NONE', #34416, #48034, #27162 ) ;
#13703=AXIS2_PLACEMENT_3D ( 'NONE', #22972, #57011, #22081 ) ;
#13705=EDGE_CURVE ( 'NONE', #85160, #36866, #12722, .T. ) ;
#13706=ORIENTED_EDGE ( 'NONE', *, *, #52741, .F. ) ;
#13707=CARTESIAN_POINT ( 'NONE',  ( 114.0519814166326995, -29.87813257090978070, 145.4441967044819819 ) ) ;
#13708=CARTESIAN_POINT ( 'NONE',  ( 25.56670390244820368, -42.82844715994167473, 259.7178068554150059 ) ) ;
#13709=VERTEX_POINT ( 'NONE', #75835 ) ;
#13712=CARTESIAN_POINT ( 'NONE',  ( 100.0388059118473052, -29.01104360887439526, 281.6641967044822650 ) ) ;
#13715=DIRECTION ( 'NONE',  ( 0.000000000000000000, 0.000000000000000000, 1.000000000000000000 ) ) ;
#13716=DIRECTION ( 'NONE',  ( 0.000000000000000000, 0.000000000000000000, -1.000000000000000000 ) ) ;
#13717=ADVANCED_FACE ( 'NONE', ( #69474 ), #48541, .F. ) ;
#13718=CARTESIAN_POINT ( 'NONE',  ( 138.8664832912740223, -71.52944715994085811, 394.9756252759100903 ) ) ;
#13720=CARTESIAN_POINT ( 'NONE',  ( 112.6571330189593141, -45.46348522128867131, 218.0175300378159591 ) ) ;
#13721=VERTEX_POINT ( 'NONE', #76734 ) ;
#13722=ORIENTED_EDGE ( 'NONE', *, *, #6307, .F. ) ;
#13723=ADVANCED_FACE ( 'NONE', ( #68127 ), #14515, .F. ) ;
#13724=CARTESIAN_POINT ( 'NONE',  ( 110.7647657470428157, -46.09926102310604534, 169.3072975916109613 ) ) ;
#13725=DIRECTION ( 'NONE',  ( -1.000000000000000000, 6.745093096447288888E-17, -9.693101022688619289E-16 ) ) ;
#13726=CARTESIAN_POINT ( 'NONE',  ( 100.3317924633492737, -42.48897995906190772, 28.32158330589695794 ) ) ;
#13727=CARTESIAN_POINT ( 'NONE',  ( 97.79819076598835181, -40.48430223427173757, 57.63277862058793488 ) ) ;
#13728=LINE ( 'NONE', #7361, #10115 ) ;
#13731=CARTESIAN_POINT ( 'NONE',  ( 108.4174892490654258, -26.73503592719089639, 105.9689586094897038 ) ) ;
#13733=CARTESIAN_POINT ( 'NONE',  ( 96.79426660377257008, -34.87310936442964504, 241.1841967044819626 ) ) ;
#13734=CARTESIAN_POINT ( 'NONE',  ( 105.8002857911943977, -26.72392027096438127, 170.1763073387932934 ) ) ;
#13741=LINE ( 'NONE', #54594, #65111 ) ;
#13742=EDGE_CURVE ( 'NONE', #50282, #62015, #26778, .T. ) ;
#13745=ORIENTED_EDGE ( 'NONE', *, *, #47930, .F. ) ;
#13748=CARTESIAN_POINT ( 'NONE',  ( 116.9255123305063222, -41.72731008894000837, 248.4651490854349731 ) ) ;
#13749=EDGE_LOOP ( 'NONE', ( #54289, #3885, #44677, #62248 ) ) ;
#13751=CARTESIAN_POINT ( 'NONE',  ( 107.0664832912739968, -36.72944715994100306, 287.6356252759109680 ) ) ;
#13752=CARTESIAN_POINT ( 'NONE',  ( 105.7149151130501536, -46.72377363291952435, 167.4689823453068698 ) ) ;
#13753=CARTESIAN_POINT ( 'NONE',  ( 99.12283442819817481, -33.29442637601800214, 58.83189989340093007 ) ) ;
#13754=CARTESIAN_POINT ( 'NONE',  ( 102.9047493514100893, -27.10917607469848178, 151.4013395616249511 ) ) ;
#13756=ORIENTED_EDGE ( 'NONE', *, *, #16033, .F. ) ;
#13757=EDGE_CURVE ( 'NONE', #58541, #20859, #70446, .T. ) ;
#13758=FACE_OUTER_BOUND ( 'NONE', #47870, .T. ) ;
#13759=ORIENTED_EDGE ( 'NONE', *, *, #80876, .T. ) ;
#13761=EDGE_CURVE ( 'NONE', #33523, #62846, #89312, .T. ) ;
#13762=AXIS2_PLACEMENT_3D ( 'NONE', #88458, #6231, #5332 ) ;
#13763=FACE_OUTER_BOUND ( 'NONE', #20797, .T. ) ;
#13765=EDGE_LOOP ( 'NONE', ( #5284, #70786 ) ) ;
#13766=ORIENTED_EDGE ( 'NONE', *, *, #3035, .F. ) ;
#13767=DIRECTION ( 'NONE',  ( 0.000000000000000000, -1.000000000000000000, 0.000000000000000000 ) ) ;
#13768=VECTOR ( 'NONE', #19117, 1000.000000000000000 ) ;
#13769=CARTESIAN_POINT ( 'NONE',  ( 99.26324148224303201, -33.25589724784042289, 100.4152769709339736 ) ) ;
#13771=CARTESIAN_POINT ( 'NONE',  ( 117.4964429983690337, -36.12752982774328103, 228.8727681330539667 ) ) ;
#13773=CARTESIAN_POINT ( 'NONE',  ( 98.56907362037662779, -44.95393718666142746, 191.9384824187679612 ) ) ;
#13774=CARTESIAN_POINT ( 'NONE',  ( 96.73644666290624627, -38.23103596604165233, 62.44133956162495025 ) ) ;
#13775=LINE ( 'NONE', #1039, #12194 ) ;
#13777=ORIENTED_EDGE ( 'NONE', *, *, #44758, .F. ) ;
#13778=VECTOR ( 'NONE', #69235, 1000.000000000000000 ) ;
#13779=CARTESIAN_POINT ( 'NONE',  ( 116.0091996907507905, -30.12340400999213941, 109.3327681330539605 ) ) ;
#13780=CARTESIAN_POINT ( 'NONE',  ( 107.3221093067165128, -25.63226107660779007, 75.04610146638695767 ) ) ;
#13781=CARTESIAN_POINT ( 'NONE',  ( 97.51966259852430596, -43.83486848311488160, 261.8356252759109566 ) ) ;
#13783=CARTESIAN_POINT ( 'NONE',  ( 98.03659727384791722, -44.40418782976336587, 226.8870538473399563 ) ) ;
#13784=CARTESIAN_POINT ( 'NONE',  ( 113.2454986814590683, -28.75867293103612710, 34.55229194428200401 ) ) ;
#13786=CARTESIAN_POINT ( 'NONE',  ( 113.1774878185915298, -44.75247536050181907, 24.09387774641090729 ) ) ;
#13787=DIRECTION ( 'NONE',  ( 1.000000000000000078E-15, -1.000000000000000083E-30, -1.000000000000000000 ) ) ;
#13788=AXIS2_PLACEMENT_3D ( 'NONE', #76460, #50081, #29652 ) ;
#13790=LINE ( 'NONE', #41474, #4217 ) ;
#13791=PLANE ( 'NONE',  #44166 ) ;
#13793=ADVANCED_FACE ( 'NONE', ( #62198 ), #74944, .T. ) ;
#13795=PLANE ( 'NONE',  #49907 ) ;
#13797=DIRECTION ( 'NONE',  ( -4.237773401492740281E-14, 1.000000000000000000, 0.000000000000000000 ) ) ;
#13798=CARTESIAN_POINT ( 'NONE',  ( 37.06648329127400388, 12.92155284005802685, 349.2756252759108406 ) ) ;
#13799=DIRECTION ( 'NONE',  ( -0.7071067812159675947, -0.7071067811571274397, -7.071067812159980775E-16 ) ) ;
#13800=CARTESIAN_POINT ( 'NONE',  ( 99.09570905812269359, -30.55043177598640369, 260.8022919448715697 ) ) ;
#13801=ORIENTED_EDGE ( 'NONE', *, *, #81440, .T. ) ;
#13804=CARTESIAN_POINT ( 'NONE',  ( 118.1265197682042327, -36.12032134488166690, 273.8822919425775808 ) ) ;
#13805=CARTESIAN_POINT ( 'NONE',  ( 102.3931144830280715, -26.71278082505766704, 131.4118157521009778 ) ) ;
#13806=CARTESIAN_POINT ( 'NONE',  ( 97.52025866034094292, -43.83442485161933178, 257.8356252759109566 ) ) ;
#13807=LINE ( 'NONE', #88339, #25791 ) ;
#13808=PLANE ( 'NONE',  #47828 ) ;
#13812=DIRECTION ( 'NONE',  ( 4.299999999999999979E-14, -1.000000000000000000, 4.400000000000000367E-29 ) ) ;
#13814=ORIENTED_EDGE ( 'NONE', *, *, #82838, .T. ) ;
#13815=CARTESIAN_POINT ( 'NONE',  ( 45.56670390244706681, -48.82844715994099971, 300.4678068554150059 ) ) ;
#13816=EDGE_LOOP ( 'NONE', ( #38162, #26585, #7727, #15936, #5199, #56535, #72831, #11748, #36994, #7467, #61449, #89653, #85354, #6857 ) ) ;
#13817=EDGE_CURVE ( 'NONE', #48257, #49936, #6344, .T. ) ;
#13818=CARTESIAN_POINT ( 'NONE',  ( 102.9027671602101037, -44.22047980607887752, 186.5952769709339805 ) ) ;
#13819=CARTESIAN_POINT ( 'NONE',  ( 151.0371591254573502, -24.42818131005592974, 249.9678068554149490 ) ) ;
#13820=VERTEX_POINT ( 'NONE', #84467 ) ;
#13821=DIRECTION ( 'NONE',  ( 1.000000000000000000, 4.237773401492740281E-14, 0.000000000000000000 ) ) ;
#13822=CARTESIAN_POINT ( 'NONE',  ( 96.67182511810091228, -37.15340426533111895, 157.3584824187679487 ) ) ;
#13824=FACE_OUTER_BOUND ( 'NONE', #65494, .T. ) ;
#13826=CARTESIAN_POINT ( 'NONE',  ( 53.56670390244833158, -48.82844715994055917, 249.9678068554150343 ) ) ;
#13827=CARTESIAN_POINT ( 'NONE',  ( 114.6661721138975025, -42.88640786233948887, 88.28419670448295165 ) ) ;
#13832=VECTOR ( 'NONE', #65103, 1000.000000000000000 ) ;
#13834=VECTOR ( 'NONE', #4225, 1000.000000000000000 ) ;
#13835=CARTESIAN_POINT ( 'NONE',  ( 104.7173522264389618, -47.59653351925012288, 178.4070538473389718 ) ) ;
#13836=CARTESIAN_POINT ( 'NONE',  ( 104.4081007499953984, -46.45808916365906782, 37.36479194982128149 ) ) ;
#13837=VECTOR ( 'NONE', #26235, 1000.000000000000000 ) ;
#13839=DIRECTION ( 'NONE',  ( 0.000000000000000000, 0.000000000000000000, -1.000000000000000000 ) ) ;
#13840=AXIS2_PLACEMENT_3D ( 'NONE', #82984, #48406, #76139 ) ;
#13844=CARTESIAN_POINT ( 'NONE',  ( 97.85535806214033983, -31.89376338832682123, 135.9413395616259947 ) ) ;
#13845=ORIENTED_EDGE ( 'NONE', *, *, #87637, .T. ) ;
#13847=EDGE_LOOP ( 'NONE', ( #23848, #42094, #39662, #70734 ) ) ;
#13848=CIRCLE ( 'NONE', #29812, 0.5000000000000004441 ) ;
#13849=DIRECTION ( 'NONE',  ( 1.000000000000000000, 2.999999999999999839E-15, 1.000000000000000078E-15 ) ) ;
#13851=CARTESIAN_POINT ( 'NONE',  ( 183.6524903400783160, -48.32844715993452667, 300.4678068554149490 ) ) ;
#13852=EDGE_CURVE ( 'NONE', #73470, #28852, #2227, .T. ) ;
#13853=CARTESIAN_POINT ( 'NONE',  ( 113.3093514795881589, -30.73549005055465955, 187.2414237029249477 ) ) ;
#13854=APPLICATION_CONTEXT ( 'automotive_design' ) ;
#13855=DIRECTION ( 'NONE',  ( 0.4214249218767882055, 0.9068632946707806397, 4.214249218767890910E-16 ) ) ;
#13858=ORIENTED_EDGE ( 'NONE', *, *, #41190, .T. ) ;
#13860=ORIENTED_EDGE ( 'NONE', *, *, #58196, .F. ) ;
#13862=ORIENTED_EDGE ( 'NONE', *, *, #57502, .T. ) ;
#13863=ORIENTED_EDGE ( 'NONE', *, *, #8956, .F. ) ;
#13864=CARTESIAN_POINT ( 'NONE',  ( 78.82227874343284668, -21.18254450372301534, 7.982620440116730443 ) ) ;
#13865=CARTESIAN_POINT ( 'NONE',  ( 111.8242684682981718, -44.20552626741085334, 259.4587261630397848 ) ) ;
#13866=ORIENTED_EDGE ( 'NONE', *, *, #18307, .T. ) ;
#13867=DIRECTION ( 'NONE',  ( 1.000000000000000000, 0.000000000000000000, 9.462128050782575008E-16 ) ) ;
#13873=LINE ( 'NONE', #41555, #53613 ) ;
#13874=AXIS2_PLACEMENT_3D ( 'NONE', #11798, #74469, #31782 ) ;
#13875=ORIENTED_EDGE ( 'NONE', *, *, #40200, .T. ) ;
#13877=B_SPLINE_CURVE_WITH_KNOTS ( 'NONE', 3,
 ( #51987, #10673, #24756, #43854, #65642, #85231, #9351, #30244, #79745, #44741, #51551, #17503, #31563, #51114, #36623, #72473, #2983, #79302, #17061, #3427, #45183, #38377, #66076, #59266, #17937, #45614, #8924 ),
 .UNSPECIFIED., .F., .F.,
 ( 4, 2, 2, 2, 2, 2, 2, 2, 2, 2, 1, 1, 1, 2, 4 ),
 ( 0.000000000000000000, 0.06251142862490606522, 0.1250228572498121304, 0.1875342858747182095, 0.2500457144996242609, 0.3125571431245303122, 0.3750685717494364191, 0.4375800003743421374, 0.4688357146867948577, 0.4844635718430209126, 0.4922775004211341066, 0.4961844647101908423, 0.4981379468547192380, 0.4991146879269833803, 0.5000914289992475226 ),
 .UNSPECIFIED. ) ;
#13878=CARTESIAN_POINT ( 'NONE',  ( 103.3964814340166498, -45.24903370896166876, 285.0709475124485266 ) ) ;
#13879=CARTESIAN_POINT ( 'NONE',  ( 98.44037697964694189, -30.83566621160791144, 120.8499109901969604 ) ) ;
#13880=CARTESIAN_POINT ( 'NONE',  ( 96.66103594285301881, -37.56076609107802255, 101.3899109901969524 ) ) ;
#13881=CARTESIAN_POINT ( 'NONE',  ( 109.8023483073639710, -28.09558655615849787, 249.5838068554169240 ) ) ;
#13882=CARTESIAN_POINT ( 'NONE',  ( 131.4004675426832023, -18.03188136815630216, 6.871351212842276901 ) ) ;
#13883=CARTESIAN_POINT ( 'NONE',  ( 108.1817661827909376, -47.09470796318245078, 198.6613395616249989 ) ) ;
#13887=DIRECTION ( 'NONE',  ( 0.000000000000000000, 0.000000000000000000, 1.000000000000000000 ) ) ;
#13890=DIRECTION ( 'NONE',  ( -0.1858654557293184517, 0.9825752044329902901, 0.000000000000000000 ) ) ;
#13891=AXIS2_PLACEMENT_3D ( 'NONE', #64005, #23136, #17962 ) ;
#13892=CARTESIAN_POINT ( 'NONE',  ( 103.3014603440054628, -27.46527934327819054, 136.3836531168635702 ) ) ;
#13893=VECTOR ( 'NONE', #84570, 1000.000000000000000 ) ;
#13894=CIRCLE ( 'NONE', #28411, 2.030000000001807248 ) ;
#13895=CARTESIAN_POINT ( 'NONE',  ( 108.7432494476977922, -25.80391683235395917, 144.9432443235299672 ) ) ;
#13897=AXIS2_PLACEMENT_3D ( 'NONE', #76632, #33937, #89828 ) ;
#13898=CARTESIAN_POINT ( 'NONE',  ( 97.81169182074827972, -40.51741433969252881, 77.63574375254798099 ) ) ;
#13902=CARTESIAN_POINT ( 'NONE',  ( 117.1759530674218865, -34.27439392744689428, 205.0156252759109634 ) ) ;
#13903=CARTESIAN_POINT ( 'NONE',  ( 165.9667039024459996, -28.27351298637401200, 193.9678068554150059 ) ) ;
#13906=EDGE_LOOP ( 'NONE', ( #29408, #62715 ) ) ;
#13908=EDGE_CURVE ( 'NONE', #26420, #28268, #63172, .T. ) ;
#13911=DIRECTION ( 'NONE',  ( 0.000000000000000000, 0.000000000000000000, -1.000000000000000000 ) ) ;
#13913=CARTESIAN_POINT ( 'NONE',  ( 109.2210686807619453, -48.43357285789136313, 277.7213395616254843 ) ) ;
#13915=ADVANCED_FACE ( 'NONE', ( #38852 ), #63548, .F. ) ;
#13917=CARTESIAN_POINT ( 'NONE',  ( 108.6520877210037952, -25.77347123183324484, 149.9737205140059473 ) ) ;
#13918=CARTESIAN_POINT ( 'NONE',  ( 115.5737247207382552, -42.75516958203532880, 49.33562527591095659 ) ) ;
#13919=CARTESIAN_POINT ( 'NONE',  ( 99.39016829297771949, -27.63593621212785933, 146.6356252759109395 ) ) ;
#13921=CARTESIAN_POINT ( 'NONE',  ( 97.81151828220572497, -40.51700876243793203, 102.6355898084469942 ) ) ;
#13922=VECTOR ( 'NONE', #47201, 1000.000000000000114 ) ;
#13923=CARTESIAN_POINT ( 'NONE',  ( 183.6524903400785718, -48.32844715993451956, 129.9678068554150059 ) ) ;
#13924=CARTESIAN_POINT ( 'NONE',  ( 107.0664832912739968, -36.72944715994100306, 9.635625275910941312 ) ) ;
#13925=CARTESIAN_POINT ( 'NONE',  ( 71.24189083761808661, -0.9290567490904538817, 396.9756252759102040 ) ) ;
#13929=VERTEX_POINT ( 'NONE', #50352 ) ;
#13930=ORIENTED_EDGE ( 'NONE', *, *, #41872, .T. ) ;
#13932=ORIENTED_EDGE ( 'NONE', *, *, #53641, .F. ) ;
#13934=CARTESIAN_POINT ( 'NONE',  ( 103.8480726019013645, -46.65951555449685628, 78.32705384733995402 ) ) ;
#13937=CARTESIAN_POINT ( 'NONE',  ( 109.3680554845995232, -25.87125837001184081, 180.9222919425779708 ) ) ;
#13939=CARTESIAN_POINT ( 'NONE',  ( 114.1362055435773613, -41.52268812998874381, 272.7752769709339304 ) ) ;
#13942=VERTEX_POINT ( 'NONE', #66110 ) ;
#13943=CARTESIAN_POINT ( 'NONE',  ( 116.3195061320206207, -32.94150711290046729, 139.1356252759109680 ) ) ;
#13944=CARTESIAN_POINT ( 'NONE',  ( 172.5664832912740110, 0.2215528400590013880, 138.9256252759119832 ) ) ;
#13945=CARTESIAN_POINT ( 'NONE',  ( 112.1405389099331984, -28.01350764861801323, 19.65586982525807613 ) ) ;
#13946=FACE_OUTER_BOUND ( 'NONE', #67810, .T. ) ;
#13947=CARTESIAN_POINT ( 'NONE',  ( 184.5667039024480118, -67.87844715994100397, 10.91780685541479734 ) ) ;
#13948=CARTESIAN_POINT ( 'NONE',  ( 188.5667039024479834, -48.82844715994099971, 173.2178068554149775 ) ) ;
#13950=CARTESIAN_POINT ( 'NONE',  ( 102.7643194828038276, -25.71402177940525746, 20.37276813305294354 ) ) ;
#13953=CARTESIAN_POINT ( 'NONE',  ( 95.64925804648841279, -35.75026674902539980, 300.2406250056037038 ) ) ;
#13956=EDGE_CURVE ( 'NONE', #57074, #75399, #80216, .T. ) ;
#13957=CARTESIAN_POINT ( 'NONE',  ( 100.4295600883690014, -42.28392062234677695, 69.68713798863895192 ) ) ;
#13959=VECTOR ( 'NONE', #68432, 1000.000000000000000 ) ;
#13960=CIRCLE ( 'NONE', #24209, 11.57110091390439699 ) ;
#13962=EDGE_CURVE ( 'NONE', #8744, #83042, #71714, .T. ) ;
#13966=ORIENTED_EDGE ( 'NONE', *, *, #52227, .T. ) ;
#13967=CARTESIAN_POINT ( 'NONE',  ( 80.06648329127399677, -33.97944715994105991, 8.225625275910942946 ) ) ;
#13968=VERTEX_POINT ( 'NONE', #84910 ) ;
#13969=CARTESIAN_POINT ( 'NONE',  ( 105.3162203493976676, -48.44985994433862686, 147.4584824187679715 ) ) ;
#13970=ORIENTED_EDGE ( 'NONE', *, *, #12286, .F. ) ;
#13972=CARTESIAN_POINT ( 'NONE',  ( 116.0270257299131487, -33.90363670229466919, 125.4892023535159638 ) ) ;
#13973=CARTESIAN_POINT ( 'NONE',  ( 98.36549455146187881, -40.29075363668734155, 11.63562527591094309 ) ) ;
#13975=CARTESIAN_POINT ( 'NONE',  ( 101.1293421793351968, -28.09060746778665418, 46.55562527591094835 ) ) ;
#13976=CARTESIAN_POINT ( 'NONE',  ( 95.05156358570199870, -41.69348830286664764, 292.6356252759106837 ) ) ;
#13977=EDGE_LOOP ( 'NONE', ( #47423, #8101, #68931, #35770 ) ) ;
#13981=VECTOR ( 'NONE', #89004, 1000.000000000000000 ) ;
#13982=ORIENTED_EDGE ( 'NONE', *, *, #84179, .F. ) ;
#13984=ORIENTED_EDGE ( 'NONE', *, *, #36236, .T. ) ;
#13985=CARTESIAN_POINT ( 'NONE',  ( 96.36668125800717633, -39.40815171121898430, 16.53372051400597798 ) ) ;
#13986=CARTESIAN_POINT ( 'NONE',  ( 102.6884963789050289, -46.90384819475383438, 133.2651490854349561 ) ) ;
#13988=CARTESIAN_POINT ( 'NONE',  ( 115.0889047246291454, -30.61763668101085045, 140.3439586091480464 ) ) ;
#13989=CARTESIAN_POINT ( 'NONE',  ( 97.26643838138058129, -31.61739275409173544, 86.93181575210095957 ) ) ;
#13992=FACE_OUTER_BOUND ( 'NONE', #7627, .T. ) ;
#13994=DIRECTION ( 'NONE',  ( 8.673617379884035472E-16, 1.000000000000000000, 0.000000000000000000 ) ) ;
#13998=CARTESIAN_POINT ( 'NONE',  ( 163.5667039024460223, -18.82844715994111340, -5.074374724088000832 ) ) ;
#13999=CARTESIAN_POINT ( 'NONE',  ( 97.35142178662984236, -32.85085377626895564, 41.02419670448193045 ) ) ;
#14001=FACE_OUTER_BOUND ( 'NONE', #38225, .T. ) ;
#14002=CARTESIAN_POINT ( 'NONE',  ( 116.3229784443844324, -32.93528945216412041, 94.13562527591096796 ) ) ;
#14003=CARTESIAN_POINT ( 'NONE',  ( 117.8597870418416562, -34.07357964055000821, 14.01848241876896317 ) ) ;
#14004=CARTESIAN_POINT ( 'NONE',  ( 97.81413224952068219, -40.51639846094042952, 101.6360726122380100 ) ) ;
#14005=CARTESIAN_POINT ( 'NONE',  ( 97.95167206076199307, -31.64175201202211341, 106.9213395616259703 ) ) ;
#14006=LINE ( 'NONE', #55315, #84345 ) ;
#14007=CARTESIAN_POINT ( 'NONE',  ( 101.9504156919933280, -46.58027128656367921, 167.1832443235299763 ) ) ;
#14008=LINE ( 'NONE', #75347, #78634 ) ;
#14012=FACE_OUTER_BOUND ( 'NONE', #7785, .T. ) ;
#14013=EDGE_CURVE ( 'NONE', #50621, #60674, #56259, .T. ) ;
#14015=CARTESIAN_POINT ( 'NONE',  ( 104.4919955313450686, -26.97824969402968875, 61.28156387838701136 ) ) ;
#14016=CARTESIAN_POINT ( 'NONE',  ( 97.38432216341050207, -42.15794967186695175, 181.7451490854349743 ) ) ;
#14017=VERTEX_POINT ( 'NONE', #36748 ) ;
#14019=CARTESIAN_POINT ( 'NONE',  ( 99.06932979199925171, -29.95266829982950441, 211.7670538473399517 ) ) ;
#14020=VECTOR ( 'NONE', #66581, 1000.000000000000000 ) ;
#14022=B_SPLINE_CURVE_WITH_KNOTS ( 'NONE', 3,
 ( #66429, #19193, #59605, #87782, #17842, #45520, #32806, #25544, #53220, #65980, #88694, #52326, #87342, #80091, #88248, #25103, #46862, #5112, #73242, #60965, #3772, #26451, #31460, #60052, #12374, #52765, #80990, #11482, #18737, #26005, #40064 ),
 .UNSPECIFIED., .F., .F.,
 ( 4, 2, 2, 1, 2, 2, 2, 2, 2, 2, 2, 1, 1, 2, 2, 2, 4 ),
 ( 0.000000000000000000, 0.1249999999999613920, 0.1874999999999421019, 0.2187499999999242273, 0.2343749999999238942, 0.2499999999999235611, 0.3749999999998904765, 0.4374999999998728795, 0.4999999999998552269, 0.6249999999998172573, 0.6874999999997966071, 0.7187499999997883915, 0.7343749999997789546, 0.7421874999997795097, 0.7499999999997800648, 0.8749999999998900879, 1.000000000000000000 ),
 .UNSPECIFIED. ) ;
#14026=ORIENTED_EDGE ( 'NONE', *, *, #54049, .T. ) ;
#14027=AXIS2_PLACEMENT_3D ( 'NONE', #46949, #32890, #74679 ) ;
#14033=ADVANCED_FACE ( 'NONE', ( #29937 ), #49451, .F. ) ;
#14034=ORIENTED_EDGE ( 'NONE', *, *, #6318, .T. ) ;
#14035=DIRECTION ( 'NONE',  ( 0.000000000000000000, 0.000000000000000000, -1.000000000000000000 ) ) ;
#14036=CARTESIAN_POINT ( 'NONE',  ( 109.9601702690906677, -48.22123515106449787, 238.7727681330539724 ) ) ;
#14038=EDGE_CURVE ( 'NONE', #59995, #24816, #24789, .T. ) ;
#14039=CARTESIAN_POINT ( 'NONE',  ( 134.4427611689604589, -15.99866847873243714, 1.641799428526213855 ) ) ;
#14040=CARTESIAN_POINT ( 'NONE',  ( 89.06648329127401098, -18.82844715994099971, 17.92562527591199739 ) ) ;
#14042=CARTESIAN_POINT ( 'NONE',  ( 31.56670390244700641, -22.48495420874110806, -5.074374724088000832 ) ) ;
#14044=CARTESIAN_POINT ( 'NONE',  ( 112.1280348295452001, -26.87672238358117127, 19.71086337114896736 ) ) ;
#14045=VERTEX_POINT ( 'NONE', #42630 ) ;
#14046=EDGE_LOOP ( 'NONE', ( #50918, #79053, #78945, #23507 ) ) ;
#14049=DIRECTION ( 'NONE',  ( 0.000000000000000000, 0.000000000000000000, 1.000000000000000000 ) ) ;
#14050=CARTESIAN_POINT ( 'NONE',  ( 99.34779341711927714, -29.80408710710938891, 231.7565776568629587 ) ) ;
#14051=DIRECTION ( 'NONE',  ( 0.9242245927363033076, 0.3818493186865917766, 0.000000000000000000 ) ) ;
#14052=CARTESIAN_POINT ( 'NONE',  ( 112.9545114599701492, -28.19305977888952697, 85.60800622829195561 ) ) ;
#14054=CARTESIAN_POINT ( 'NONE',  ( 97.53183037146393985, -39.74891120937812872, 22.57051295153732440 ) ) ;
#14058=EDGE_LOOP ( 'NONE', ( #70968, #6189, #41636, #19399 ) ) ;
#14060=CARTESIAN_POINT ( 'NONE',  ( 106.0694874169909809, -45.56507127853855366, 278.9187261630399917 ) ) ;
#14061=CARTESIAN_POINT ( 'NONE',  ( 97.81170999939396893, -40.51745679428447744, 191.6351607553995393 ) ) ;
#14062=CARTESIAN_POINT ( 'NONE',  ( 97.81315821180474757, -40.51681016098617505, 66.63608906629065132 ) ) ;
#14063=EDGE_CURVE ( 'NONE', #36866, #13081, #57339, .T. ) ;
#14064=CARTESIAN_POINT ( 'NONE',  ( 97.07207206230401653, -35.37844117569200364, 86.21895860738254669 ) ) ;
#14067=CARTESIAN_POINT ( 'NONE',  ( 80.06648329127399677, -8.350947159940998787, 4.925625275911999168 ) ) ;
#14068=CARTESIAN_POINT ( 'NONE',  ( 115.0356694214038242, -42.91047690283549798, 184.3026665754189821 ) ) ;
#14069=ORIENTED_EDGE ( 'NONE', *, *, #65061, .F. ) ;
#14070=CARTESIAN_POINT ( 'NONE',  ( 112.9632928630424402, -28.13208318394687524, 44.59848241876795782 ) ) ;
#14071=ORIENTED_EDGE ( 'NONE', *, *, #86810, .F. ) ;
#14072=CARTESIAN_POINT ( 'NONE',  ( 114.1709767417603132, -32.67596046159766132, 287.0566617981627360 ) ) ;
#14074=CARTESIAN_POINT ( 'NONE',  ( 97.26456095925928480, -36.24355304347522377, 171.2870538473399620 ) ) ;
#14075=LINE ( 'NONE', #63573, #43318 ) ;
#14076=AXIS2_PLACEMENT_3D ( 'NONE', #42055, #76597, #288 ) ;
#14081=CARTESIAN_POINT ( 'NONE',  ( 116.6456181429820447, -40.95237922671789477, 249.4956252759109532 ) ) ;
#14084=DIRECTION ( 'NONE',  ( 0.000000000000000000, 0.000000000000000000, 1.000000000000000000 ) ) ;
#14085=VECTOR ( 'NONE', #47746, 1000.000000000000000 ) ;
#14086=ORIENTED_EDGE ( 'NONE', *, *, #85955, .T. ) ;
#14087=CARTESIAN_POINT ( 'NONE',  ( 102.2824096876565108, -27.37794169069978523, 116.4527681330539650 ) ) ;
#14088=AXIS2_PLACEMENT_3D ( 'NONE', #28592, #55827, #77209 ) ;
#14089=EDGE_CURVE ( 'NONE', #19776, #89932, #70505, .T. ) ;
#14092=B_SPLINE_CURVE_WITH_KNOTS ( 'NONE', 3,
 ( #31741, #11296, #53498, #38999, #60329, #66708, #87169, #24935, #24496, #18558, #39453, #17676, #87609, #73976, #25829, #24055, #4495, #3161 ),
 .UNSPECIFIED., .F., .F.,
 ( 4, 2, 2, 2, 2, 2, 2, 2, 4 ),
 ( 0.000000000000000000, 0.06250000026632723804, 0.1250000005326544761, 0.1875000007989817141, 0.2500000010653089522, 0.3125000013316361902, 0.3750000015979634282, 0.4375000018642906663, 0.5000000021306179043 ),
 .UNSPECIFIED. ) ;
#14093=ORIENTED_EDGE ( 'NONE', *, *, #15043, .F. ) ;
#14097=CARTESIAN_POINT ( 'NONE',  ( 98.34986732099139317, -31.65657060954530522, 266.9064573084277754 ) ) ;
#14099=CYLINDRICAL_SURFACE ( 'NONE', #74161, 3.250000000000002665 ) ;
#14101=CARTESIAN_POINT ( 'NONE',  ( 100.8299159177638984, -43.59960581930123880, 154.8080903695919801 ) ) ;
#14102=CARTESIAN_POINT ( 'NONE',  ( 105.7736751693905148, -26.36287077168075754, 266.1756252759109884 ) ) ;
#14103=EDGE_CURVE ( 'NONE', #34773, #15887, #87936, .T. ) ;
#14104=CARTESIAN_POINT ( 'NONE',  ( 97.92328980544225203, -40.78083263938301428, 57.65839077251143863 ) ) ;
#14105=EDGE_LOOP ( 'NONE', ( #29053, #48716, #25942, #87535 ) ) ;
#14106=CARTESIAN_POINT ( 'NONE',  ( 177.0664832912730162, 12.92155284005730387, 361.9756252759109998 ) ) ;
#14109=CIRCLE ( 'NONE', #21306, 0.5000000000000104361 ) ;
#14110=CYLINDRICAL_SURFACE ( 'NONE', #17173, 2.517500000000005844 ) ;
#14111=VERTEX_POINT ( 'NONE', #88817 ) ;
#14112=ORIENTED_EDGE ( 'NONE', *, *, #84101, .F. ) ;
#14114=CARTESIAN_POINT ( 'NONE',  ( 123.6837132603318992, -50.04645651782490745, 239.5838068554164693 ) ) ;
#14115=LINE ( 'NONE', #54963, #20819 ) ;
#14117=EDGE_CURVE ( 'NONE', #63602, #58568, #76331, .T. ) ;
#14118=DIRECTION ( 'NONE',  ( -0.7071067811865475727, 0.7071067811865475727, 0.000000000000000000 ) ) ;
#14119=LINE ( 'NONE', #34550, #64915 ) ;
#14120=CARTESIAN_POINT ( 'NONE',  ( 100.1837753934783990, -31.62254652264567767, 180.2409912566479591 ) ) ;
#14121=CARTESIAN_POINT ( 'NONE',  ( 99.26081945853924537, -43.75962541195023903, 56.90991099019593236 ) ) ;
#14126=ADVANCED_FACE ( 'NONE', ( #68365 ), #6145, .F. ) ;
#14129=VERTEX_POINT ( 'NONE', #89261 ) ;
#14130=DIRECTION ( 'NONE',  ( 0.000000000000000000, 0.000000000000000000, 1.000000000000000000 ) ) ;
#14131=CARTESIAN_POINT ( 'NONE',  ( 193.0371591254584587, -47.82818131005411999, 237.4678068554150059 ) ) ;
#14133=VECTOR ( 'NONE', #64752, 1000.000000000000000 ) ;
#14134=DIRECTION ( 'NONE',  ( 0.7071067811739274456, -0.7071067811991676999, 0.000000000000000000 ) ) ;
#14135=VERTEX_POINT ( 'NONE', #40187 ) ;
#14136=CARTESIAN_POINT ( 'NONE',  ( 116.2511270133230283, -31.75062363771698770, 69.22133956162495849 ) ) ;
#14137=DIRECTION ( 'NONE',  ( 0.000000000000000000, 1.000000000000000000, 0.000000000000000000 ) ) ;
#14139=DIRECTION ( 'NONE',  ( 0.7071067811989784069, -0.7071067811741166276, 7.071067811989480323E-16 ) ) ;
#14140=DIRECTION ( 'NONE',  ( 1.000000000000000078E-15, -1.000000000000000083E-30, -1.000000000000000000 ) ) ;
#14141=ORIENTED_EDGE ( 'NONE', *, *, #19561, .T. ) ;
#14143=LINE ( 'NONE', #9130, #51793 ) ;
#14145=ADVANCED_FACE ( 'NONE', ( #13400 ), #87466, .T. ) ;
#14149=CARTESIAN_POINT ( 'NONE',  ( 96.67756931115832231, -37.82841265861588909, 122.4099109901969626 ) ) ;
#14153=CYLINDRICAL_SURFACE ( 'NONE', #42726, 1.000000000000000888 ) ;
#14154=CARTESIAN_POINT ( 'NONE',  ( 107.0664832912739541, -21.02944715994095759, 311.3356252759109566 ) ) ;
#14155=VECTOR ( 'NONE', #45401, 1000.000000000000000 ) ;
#14156=CIRCLE ( 'NONE', #64924, 3.000000000000002665 ) ;
#14159=CARTESIAN_POINT ( 'NONE',  ( 103.6907823165633289, -45.90921117331522083, 138.2956252759109645 ) ) ;
#14160=CARTESIAN_POINT ( 'NONE',  ( 97.81168895331838087, -40.51742574516882200, 287.6356252759109680 ) ) ;
#14162=CARTESIAN_POINT ( 'NONE',  ( 101.0991643652557599, -45.25116564454916102, 278.0899109901965858 ) ) ;
#14164=PLANE ( 'NONE',  #30127 ) ;
#14166=DIRECTION ( 'NONE',  ( 0.7071067811866279529, -0.7071067811864671926, 7.071067811866286874E-16 ) ) ;
#14167=AXIS2_PLACEMENT_3D ( 'NONE', #53054, #88079, #46253 ) ;
#14168=CARTESIAN_POINT ( 'NONE',  ( 46.83715912545430626, -47.82818131006082751, 237.4678068554150059 ) ) ;
#14169=LINE ( 'NONE', #20094, #52937 ) ;
#14170=AXIS2_PLACEMENT_3D ( 'NONE', #59953, #12732, #87686 ) ;
#14172=CARTESIAN_POINT ( 'NONE',  ( 100.4443968677459083, -27.79860430499261881, 185.5841967044829630 ) ) ;
#14175=CARTESIAN_POINT ( 'NONE',  ( 115.8726827828676704, -31.83848043880258061, 175.6615833058969827 ) ) ;
#14176=VECTOR ( 'NONE', #77287, 1000.000000000000000 ) ;
#14177=DIRECTION ( 'NONE',  ( -1.000000000000000000, -5.512527431108013646E-15, 0.000000000000000000 ) ) ;
#14178=CARTESIAN_POINT ( 'NONE',  ( 97.51798391995397708, -31.03399779358258215, 276.8984824187675713 ) ) ;
#14179=DIRECTION ( 'NONE',  ( 1.000000000000000078E-15, 1.000000000000000083E-30, -1.000000000000000000 ) ) ;
#14180=CARTESIAN_POINT ( 'NONE',  ( 113.1775979644639278, -44.75238856601268367, 268.0940785184301944 ) ) ;
#14182=CARTESIAN_POINT ( 'NONE',  ( 116.3212776292292716, -32.94146857471233147, 105.1356252759109680 ) ) ;
#14183=DIRECTION ( 'NONE',  ( 4.299999999999999979E-14, -1.000000000000000000, 4.400000000000000367E-29 ) ) ;
#14184=B_SPLINE_CURVE_WITH_KNOTS ( 'NONE', 3,
 ( #21054, #19704, #61926, #89657, #88321, #33779, #82850, #13786, #53744, #12448, #33335, #54193, #55534, #41472, #32880, #6091, #81513, #76462, #39690, #34669, #62375, #83288, #40135, #47388, #19266, #68309, #67393, #75120, #46940 ),
 .UNSPECIFIED., .F., .F.,
 ( 4, 2, 2, 2, 2, 2, 2, 2, 2, 2, 1, 1, 1, 1, 1, 2, 4 ),
 ( 0.000000000000000000, 0.06250185527508492211, 0.1250037105501698442, 0.1875055658252547663, 0.2500074211003396885, 0.3125092763754245828, 0.3750111316505095327, 0.4375129869255944826, 0.4687639145631368187, 0.4843893783819079868, 0.4922021102912934598, 0.4961084762459861408, 0.4980616592233322870, 0.4990382507120053046, 0.4995265464563418689, 0.4997706943285100678, 0.5000148422006782667 ),
 .UNSPECIFIED. ) ;
#14185=CARTESIAN_POINT ( 'NONE',  ( 100.6510976905701824, -26.79511100149714764, 220.5327681330539633 ) ) ;
#14186=ORIENTED_EDGE ( 'NONE', *, *, #23186, .T. ) ;
#14188=CARTESIAN_POINT ( 'NONE',  ( 41.56648329127499153, -32.07844715994070839, 74.17562527591199739 ) ) ;
#14190=DIRECTION ( 'NONE',  ( 0.000000000000000000, 0.000000000000000000, -1.000000000000000000 ) ) ;
#14193=AXIS2_PLACEMENT_3D ( 'NONE', #64934, #56764, #1825 ) ;
#14195=EDGE_LOOP ( 'NONE', ( #60445, #33314, #41552, #62789 ) ) ;
#14197=CARTESIAN_POINT ( 'NONE',  ( 106.2268934648462420, -47.75097955688366369, 267.5280062282920994 ) ) ;
#14198=EDGE_CURVE ( 'NONE', #19079, #33965, #28407, .T. ) ;
#14199=ORIENTED_EDGE ( 'NONE', *, *, #13488, .F. ) ;
#14201=CARTESIAN_POINT ( 'NONE',  ( 77.43469508765247156, -37.52719034724768932, 6.916533740478608472 ) ) ;
#14202=DIRECTION ( 'NONE',  ( 0.000000000000000000, 0.000000000000000000, -1.000000000000000000 ) ) ;
#14204=CARTESIAN_POINT ( 'NONE',  ( 105.2602129278706400, -44.68979347096200883, 70.21666179816293152 ) ) ;
#14205=CARTESIAN_POINT ( 'NONE',  ( 99.99340640592768636, -27.19037833420660277, 181.5841967044829630 ) ) ;
#14207=CARTESIAN_POINT ( 'NONE',  ( 36.65249034007535300, -49.32844715994124130, 249.9678068554150343 ) ) ;
#14211=LINE ( 'NONE', #62790, #36423 ) ;
#14212=ORIENTED_EDGE ( 'NONE', *, *, #85904, .T. ) ;
#14213=EDGE_LOOP ( 'NONE', ( #20466, #87746 ) ) ;
#14214=EDGE_CURVE ( 'NONE', #72016, #25675, #56954, .T. ) ;
#14216=AXIS2_PLACEMENT_3D ( 'NONE', #80490, #73658, #9650 ) ;
#14217=FACE_OUTER_BOUND ( 'NONE', #34020, .T. ) ;
#14218=ORIENTED_EDGE ( 'NONE', *, *, #47383, .F. ) ;
#14219=EDGE_LOOP ( 'NONE', ( #27452, #71069, #70419, #4770 ) ) ;
#14220=DIRECTION ( 'NONE',  ( 0.000000000000000000, 0.000000000000000000, -1.000000000000000000 ) ) ;
#14221=EDGE_CURVE ( 'NONE', #22206, #12340, #74844, .T. ) ;
#14222=CARTESIAN_POINT ( 'NONE',  ( 115.9223471279375843, -38.62321220144315248, 108.0933722090289564 ) ) ;
#14223=CARTESIAN_POINT ( 'NONE',  ( 98.01753632367962155, -44.42038823906860756, 226.8870538473399563 ) ) ;
#14225=CARTESIAN_POINT ( 'NONE',  ( 113.0129699484216133, -46.01939436189644539, 218.0175300378159591 ) ) ;
#14226=CARTESIAN_POINT ( 'NONE',  ( 97.37192905580968727, -32.85904099757684804, 37.02419670448292521 ) ) ;
#14229=EDGE_CURVE ( 'NONE', #60536, #75621, #15403, .T. ) ;
#14232=CARTESIAN_POINT ( 'NONE',  ( 181.8884939055940038, -32.11662333284530746, 342.9256252759119548 ) ) ;
#14233=VECTOR ( 'NONE', #35671, 1000.000000000000114 ) ;
#14236=EDGE_CURVE ( 'NONE', #228, #43691, #71996, .T. ) ;
#14237=CARTESIAN_POINT ( 'NONE',  ( 106.1376555893193228, -47.80867374849579221, 112.5099109901969712 ) ) ;
#14238=CARTESIAN_POINT ( 'NONE',  ( 107.8717536863088640, -26.29114242999935769, 70.01562527591099183 ) ) ;
#14239=CARTESIAN_POINT ( 'NONE',  ( 103.0736367338192139, -47.94042275923426644, 252.3041967044822798 ) ) ;
#14241=CARTESIAN_POINT ( 'NONE',  ( 106.3019233867144351, -47.12668134090281313, 222.5184824187679453 ) ) ;
#14242=DIRECTION ( 'NONE',  ( 0.04216478779797398074, -0.9991106698809455455, 0.000000000000000000 ) ) ;
#14246=DIRECTION ( 'NONE',  ( 0.7071067811865459074, 0.7071067811865491270, 7.071067811865459556E-16 ) ) ;
#14247=DIRECTION ( 'NONE',  ( 0.000000000000000000, 0.000000000000000000, -1.000000000000000000 ) ) ;
#14248=PLANE ( 'NONE',  #30750 ) ;
#14250=DIRECTION ( 'NONE',  ( 0.000000000000000000, -0.000000000000000000, 1.000000000000000000 ) ) ;
#14251=AXIS2_PLACEMENT_3D ( 'NONE', #29086, #56770, #23625 ) ;
#14252=DIRECTION ( 'NONE',  ( 0.000000000000000000, 0.000000000000000000, 1.000000000000000000 ) ) ;
#14253=CARTESIAN_POINT ( 'NONE',  ( 115.8196581495599986, -31.72004586281034477, 39.23976723453453275 ) ) ;
#14256=CARTESIAN_POINT ( 'NONE',  ( 61.56670390244730839, -23.42844715994043980, 249.9678068554150343 ) ) ;
#14257=ORIENTED_EDGE ( 'NONE', *, *, #41456, .T. ) ;
#14258=CARTESIAN_POINT ( 'NONE',  ( 150.5667039024476139, -25.42844715993593852, 129.9678068554149775 ) ) ;
#14259=CARTESIAN_POINT ( 'NONE',  ( 106.5662725644766908, -47.20027100765710060, 247.5384824187679556 ) ) ;
#14260=CARTESIAN_POINT ( 'NONE',  ( 105.3162569294398168, -48.44961499074708655, 143.4584824187689662 ) ) ;
#14261=CARTESIAN_POINT ( 'NONE',  ( 99.36487284946518628, -28.73678208742278173, 261.6746728949589169 ) ) ;
#14263=DIRECTION ( 'NONE',  ( 1.000000000000000000, -9.073094938289460781E-13, 0.000000000000000000 ) ) ;
#14264=AXIS2_PLACEMENT_3D ( 'NONE', #30946, #31829, #17325 ) ;
#14265=CARTESIAN_POINT ( 'NONE',  ( 88.17226027475719263, -58.72944715994110254, 249.5838068554174924 ) ) ;
#14266=CARTESIAN_POINT ( 'NONE',  ( 82.57621891718092400, -35.60488046388260841, 7.068409955837002379 ) ) ;
#14267=CARTESIAN_POINT ( 'NONE',  ( 99.08975728047121834, -42.79576521077569851, 137.8439474464609589 ) ) ;
#14270=ORIENTED_EDGE ( 'NONE', *, *, #63910, .F. ) ;
#14271=CARTESIAN_POINT ( 'NONE',  ( 83.56670559755329464, -36.73837296219065252, 239.5838068554176914 ) ) ;
#14272=ORIENTED_EDGE ( 'NONE', *, *, #81395, .F. ) ;
#14273=CARTESIAN_POINT ( 'NONE',  ( 115.2610577610831655, -39.13882072599808026, 183.0209912566479602 ) ) ;
#14274=CARTESIAN_POINT ( 'NONE',  ( 100.8864776678791344, -44.69940107073664848, 187.0527194606352168 ) ) ;
#14276=DIRECTION ( 'NONE',  ( -0.9254794337955620787, -0.3787978585227822492, 0.000000000000000000 ) ) ;
#14277=CARTESIAN_POINT ( 'NONE',  ( 112.4747680694540293, -26.21285726233897506, 165.6984824187679521 ) ) ;
#14279=DIRECTION ( 'NONE',  ( -1.000000000000000078E-15, 0.000000000000000000, 1.000000000000000000 ) ) ;
#14280=DIRECTION ( 'NONE',  ( -0.7071067812160263255, 0.7071067811570687089, -7.071067812160270681E-16 ) ) ;
#14284=CARTESIAN_POINT ( 'NONE',  ( 112.9545114599701918, -28.19305977888944525, 89.60800622829296458 ) ) ;
#14285=EDGE_LOOP ( 'NONE', ( #59879, #43495, #7838, #64131 ) ) ;
#14286=ORIENTED_EDGE ( 'NONE', *, *, #30524, .F. ) ;
#14288=EDGE_CURVE ( 'NONE', #67926, #30523, #31042, .T. ) ;
#14290=CARTESIAN_POINT ( 'NONE',  ( 98.75489364002905290, -33.65605228111792968, 62.47586902018298360 ) ) ;
#14292=CARTESIAN_POINT ( 'NONE',  ( 19.56670390244796920, -48.82844715994099971, 10.91780685541479734 ) ) ;
#14293=CARTESIAN_POINT ( 'NONE',  ( 114.4888877093245583, -29.48743791597858177, 190.4537205140059655 ) ) ;
#14295=CARTESIAN_POINT ( 'NONE',  ( 97.81443832832722762, -40.51607714565724905, 56.63519146330476417 ) ) ;
#14296=DIRECTION ( 'NONE',  ( 0.000000000000000000, 0.000000000000000000, -1.000000000000000000 ) ) ;
#14298=VECTOR ( 'NONE', #8165, 999.9999999999998863 ) ;
#14300=CARTESIAN_POINT ( 'NONE',  ( 71.24189083761808661, -0.9290567490904538817, 542.9756252759101471 ) ) ;
#14301=CARTESIAN_POINT ( 'NONE',  ( 112.1095002620001821, -47.42599740258513208, 137.9270538473389820 ) ) ;
#14303=ORIENTED_EDGE ( 'NONE', *, *, #33517, .F. ) ;
#14305=AXIS2_PLACEMENT_3D ( 'NONE', #46981, #81562, #74720 ) ;
#14308=LINE ( 'NONE', #7928, #46779 ) ;
#14309=CARTESIAN_POINT ( 'NONE',  ( 103.6346955097220643, -29.32319583828803999, 178.2395189410199805 ) ) ;
#14311=FACE_OUTER_BOUND ( 'NONE', #10241, .T. ) ;
#14315=VERTEX_POINT ( 'NONE', #15644 ) ;
#14316=ORIENTED_EDGE ( 'NONE', *, *, #24868, .T. ) ;
#14317=ORIENTED_EDGE ( 'NONE', *, *, #46579, .T. ) ;
#14318=VECTOR ( 'NONE', #69414, 1000.000000000000000 ) ;
#14322=VERTEX_POINT ( 'NONE', #86476 ) ;
#14324=CARTESIAN_POINT ( 'NONE',  ( 98.91186986371705814, -40.27407823153063759, 228.0844404487539805 ) ) ;
#14325=LINE ( 'NONE', #7503, #12069 ) ;
#14326=ORIENTED_EDGE ( 'NONE', *, *, #59416, .T. ) ;
#14328=CIRCLE ( 'NONE', #82559, 1.000000000000003775 ) ;
#14331=ORIENTED_EDGE ( 'NONE', *, *, #29872, .F. ) ;
#14333=CARTESIAN_POINT ( 'NONE',  ( 107.0664832912749915, -36.72944715993903486, 25.56312527591096995 ) ) ;
#14334=ORIENTED_EDGE ( 'NONE', *, *, #1089, .F. ) ;
#14336=EDGE_CURVE ( 'NONE', #69712, #32370, #37869, .T. ) ;
#14337=CARTESIAN_POINT ( 'NONE',  ( 99.66640463149437323, -40.17452507577532117, 254.4909475124484857 ) ) ;
#14338=CARTESIAN_POINT ( 'NONE',  ( 117.6304226258691727, -33.39798698885631012, 129.0575300378159795 ) ) ;
#14339=CARTESIAN_POINT ( 'NONE',  ( 103.3702027031294506, -47.12181610991865455, 102.3165776568629752 ) ) ;
#14340=CARTESIAN_POINT ( 'NONE',  ( 164.7830935719630361, -29.99615139349950965, -5.074374724088000832 ) ) ;
#14342=CARTESIAN_POINT ( 'NONE',  ( 96.77275252345162926, -34.86922145964237529, 237.1841967044819626 ) ) ;
#14344=DIRECTION ( 'NONE',  ( 2.900000000000000265E-14, -2.000000000000000155E-15, 1.000000000000000000 ) ) ;
#14345=ORIENTED_EDGE ( 'NONE', *, *, #49820, .T. ) ;
#14347=EDGE_LOOP ( 'NONE', ( #67237, #34461, #37117, #41499 ) ) ;
#14348=EDGE_CURVE ( 'NONE', #77176, #19859, #86034, .T. ) ;
#14349=VECTOR ( 'NONE', #36921, 1000.000000000000000 ) ;
#14350=ORIENTED_EDGE ( 'NONE', *, *, #74881, .F. ) ;
#14353=CARTESIAN_POINT ( 'NONE',  ( 98.34965401982358912, -31.65695195725486855, 136.9064172575153862 ) ) ;
#14356=CARTESIAN_POINT ( 'NONE',  ( 117.2223540064780991, -42.83671953415140621, 128.3956252759109873 ) ) ;
#14360=CARTESIAN_POINT ( 'NONE',  ( 34.67381068360400320, -28.98061976758901892, 237.4678068554150059 ) ) ;
#14361=DIRECTION ( 'NONE',  ( 0.000000000000000000, 0.000000000000000000, -1.000000000000000000 ) ) ;
#14362=CARTESIAN_POINT ( 'NONE',  ( 99.76842024043818924, -29.31547782932927859, 221.6956252759109702 ) ) ;
#14365=FACE_OUTER_BOUND ( 'NONE', #27570, .T. ) ;
#14366=ORIENTED_EDGE ( 'NONE', *, *, #11144, .T. ) ;
#14367=DIRECTION ( 'NONE',  ( -0.000000000000000000, -0.000000000000000000, -1.000000000000000000 ) ) ;
#14371=DIRECTION ( 'NONE',  ( 0.000000000000000000, 0.000000000000000000, -1.000000000000000000 ) ) ;
#14372=CARTESIAN_POINT ( 'NONE',  ( 106.2233489284451338, -47.79750968570053971, 267.5280062282920994 ) ) ;
#14373=ORIENTED_EDGE ( 'NONE', *, *, #58591, .F. ) ;
#14375=CARTESIAN_POINT ( 'NONE',  ( 114.5434305778746733, -28.56033675696621899, 154.4746728949589851 ) ) ;
#14376=CARTESIAN_POINT ( 'NONE',  ( 97.80922128671791427, -29.33095300656633597, 41.78991099019596334 ) ) ;
#14377=CARTESIAN_POINT ( 'NONE',  ( 98.63080892621665896, -30.47026088752560824, 176.8184824187679567 ) ) ;
#14379=AXIS2_PLACEMENT_3D ( 'NONE', #88435, #27535, #20291 ) ;
#14381=CARTESIAN_POINT ( 'NONE',  ( 97.53181802940885348, -39.74887296861906805, 102.5705099596000593 ) ) ;
#14382=DIRECTION ( 'NONE',  ( 1.000000000000000078E-15, -1.000000000000000083E-30, -1.000000000000000000 ) ) ;
#14383=CARTESIAN_POINT ( 'NONE',  ( 19.56670390244740076, -47.82844715994204421, 180.4678068554150911 ) ) ;
#14385=CARTESIAN_POINT ( 'NONE',  ( 130.0664832912740110, -18.82844715994099971, 226.9256252759120116 ) ) ;
#14386=EDGE_LOOP ( 'NONE', ( #71538, #47212, #12973, #39532 ) ) ;
#14390=VECTOR ( 'NONE', #35895, 1000.000000000000000 ) ;
#14392=CARTESIAN_POINT ( 'NONE',  ( 117.4257108620837329, -37.68603989742253191, 74.75276813305397638 ) ) ;
#14394=DIRECTION ( 'NONE',  ( 1.000000000000000000, 3.999999999999999995E-14, 1.000000000000000078E-15 ) ) ;
#14396=CARTESIAN_POINT ( 'NONE',  ( 96.57517526037739231, -36.20937929227457630, 167.2870538473399620 ) ) ;
#14397=CARTESIAN_POINT ( 'NONE',  ( 112.5471327968798221, -30.46552556802231138, 288.9257531614101708 ) ) ;
#14398=EDGE_LOOP ( 'NONE', ( #74465, #24288, #47089, #35873 ) ) ;
#14399=CIRCLE ( 'NONE', #89870, 2.500000000000002220 ) ;
#14400=ORIENTED_EDGE ( 'NONE', *, *, #38917, .F. ) ;
#14401=VERTEX_POINT ( 'NONE', #78330 ) ;
#14403=ORIENTED_EDGE ( 'NONE', *, *, #65601, .T. ) ;
#14405=DIRECTION ( 'NONE',  ( 0.000000000000000000, 0.000000000000000000, -1.000000000000000000 ) ) ;
#14406=CARTESIAN_POINT ( 'NONE',  ( 99.09555428360187079, -30.55063820098889593, 161.8023122570933765 ) ) ;
#14407=CARTESIAN_POINT ( 'NONE',  ( 97.33795622581291695, -34.07061224223205897, 21.11392868892265540 ) ) ;
#14410=CARTESIAN_POINT ( 'NONE',  ( 33.96670390244699433, -26.71338133339301635, -5.074374724088000832 ) ) ;
#14412=LINE ( 'NONE', #83443, #63726 ) ;
#14413=CARTESIAN_POINT ( 'NONE',  ( 99.16013801855501697, -43.49098322490566204, 31.88991099019594699 ) ) ;
#14415=ORIENTED_EDGE ( 'NONE', *, *, #59147, .F. ) ;
#14417=CARTESIAN_POINT ( 'NONE',  ( 107.0667039024479834, -58.72944715994110254, 160.9178068554150229 ) ) ;
#14418=CARTESIAN_POINT ( 'NONE',  ( 108.5688297718456852, -44.75270591617022831, 80.54237608387698799 ) ) ;
#14420=VECTOR ( 'NONE', #61321, 1000.000000000000000 ) ;
#14422=FACE_OUTER_BOUND ( 'NONE', #79861, .T. ) ;
#14424=CARTESIAN_POINT ( 'NONE',  ( 108.4174892506360663, -26.73503592742903834, 44.96895860936416511 ) ) ;
#14425=ORIENTED_EDGE ( 'NONE', *, *, #85804, .F. ) ;
#14428=DIRECTION ( 'NONE',  ( -1.000000000000000000, 1.011922027653136551E-15, 0.000000000000000000 ) ) ;
#14430=EDGE_LOOP ( 'NONE', ( #48414, #26964, #36417, #86479 ) ) ;
#14433=CARTESIAN_POINT ( 'NONE',  ( 112.0659116485927456, -45.48839624525916747, 68.98979194496561718 ) ) ;
#14434=CARTESIAN_POINT ( 'NONE',  ( 113.1755435565086998, -43.14875213554007161, 154.6130118773249649 ) ) ;
#14435=EDGE_CURVE ( 'NONE', #2385, #6056, #74611, .T. ) ;
#14436=DIRECTION ( 'NONE',  ( 1.000000000000000000, 3.999999999999999995E-14, 1.000000000000000078E-15 ) ) ;
#14437=CARTESIAN_POINT ( 'NONE',  ( 97.24595611328004452, -31.60670846949429347, 86.93181575210095957 ) ) ;
#14439=ORIENTED_EDGE ( 'NONE', *, *, #43696, .F. ) ;
#14442=VERTEX_POINT ( 'NONE', #4234 ) ;
#14443=EDGE_CURVE ( 'NONE', #85594, #40569, #67337, .T. ) ;
#14444=VECTOR ( 'NONE', #88423, 1000.000000000000000 ) ;
#14445=DIRECTION ( 'NONE',  ( 1.000000000000000000, 2.999999999999999839E-15, 1.000000000000000078E-15 ) ) ;
#14447=CARTESIAN_POINT ( 'NONE',  ( 97.81168895331671820, -40.51742574516950413, 11.63562527591094309 ) ) ;
#14448=CARTESIAN_POINT ( 'NONE',  ( 114.3591167413298280, -29.19972650290871030, 170.4641967044829585 ) ) ;
#14449=CARTESIAN_POINT ( 'NONE',  ( 136.8164832912740110, -36.72944715994100306, -5.074374724088999145 ) ) ;
#14451=CARTESIAN_POINT ( 'NONE',  ( 117.3638278218041364, -38.35646377537064211, 109.7013395616249767 ) ) ;
#14453=ORIENTED_EDGE ( 'NONE', *, *, #89292, .F. ) ;
#14454=CARTESIAN_POINT ( 'NONE',  ( 97.31323063254396288, -38.96129955496207486, 116.5061487331113881 ) ) ;
#14455=LINE ( 'NONE', #85301, #30272 ) ;
#14456=AXIS2_PLACEMENT_3D ( 'NONE', #31928, #89146, #26908 ) ;
#14457=EDGE_LOOP ( 'NONE', ( #17782, #82727, #21581, #73000, #19185 ) ) ;
#14460=CARTESIAN_POINT ( 'NONE',  ( 118.5710604172009965, -33.89858672578665733, 14.01848241876796308 ) ) ;
#14463=DIRECTION ( 'NONE',  ( 1.000000000000000000, 4.299999999999999979E-14, 1.000000000000000078E-15 ) ) ;
#14464=CARTESIAN_POINT ( 'NONE',  ( 117.3951115944451402, -37.65585020919953507, 33.74324432352998571 ) ) ;
#14465=CARTESIAN_POINT ( 'NONE',  ( 97.70673715082763522, -40.25178540000793959, 111.6128956075913550 ) ) ;
#14466=CARTESIAN_POINT ( 'NONE',  ( 106.0785370228625055, -48.51385081415330092, 108.5099109901969712 ) ) ;
#14468=DIRECTION ( 'NONE',  ( 0.000000000000000000, -1.000000000000000000, 0.000000000000000000 ) ) ;
#14469=VERTEX_POINT ( 'NONE', #47336 ) ;
#14472=DIRECTION ( 'NONE',  ( 1.000000000000000000, 0.000000000000000000, 0.000000000000000000 ) ) ;
#14477=CARTESIAN_POINT ( 'NONE',  ( 113.6422709061198049, -28.58293356745306824, 164.5356252759109736 ) ) ;
#14479=CARTESIAN_POINT ( 'NONE',  ( 131.0667039024480118, -42.97311385573999587, 231.5838068554170093 ) ) ;
#14480=CARTESIAN_POINT ( 'NONE',  ( 97.07541381888600540, -41.51105113164680915, 212.6937205140059461 ) ) ;
#14481=CARTESIAN_POINT ( 'NONE',  ( 116.2698991418618419, -31.74044761805202342, 65.22133956162595325 ) ) ;
#14483=EDGE_CURVE ( 'NONE', #9211, #834, #11499, .T. ) ;
#14486=DIRECTION ( 'NONE',  ( 0.000000000000000000, -1.000000000000000000, 0.000000000000000000 ) ) ;
#14489=EDGE_CURVE ( 'NONE', #71741, #83417, #87799, .T. ) ;
#14492=VECTOR ( 'NONE', #30414, 1000.000000000000000 ) ;
#14493=VERTEX_POINT ( 'NONE', #32366 ) ;
#14494=DIRECTION ( 'NONE',  ( -0.1858654557293184517, 0.9825752044329902901, 0.000000000000000000 ) ) ;
#14495=CARTESIAN_POINT ( 'NONE',  ( 103.0905057572046672, -47.89305850247227880, 248.3041967044829619 ) ) ;
#14498=AXIS2_PLACEMENT_3D ( 'NONE', #40674, #68396, #42011 ) ;
#14499=CYLINDRICAL_SURFACE ( 'NONE', #42420, 0.4999999999999932832 ) ;
#14501=CARTESIAN_POINT ( 'NONE',  ( 143.0664832912740110, -18.82844715994099971, 17.92562527591199739 ) ) ;
#14502=CARTESIAN_POINT ( 'NONE',  ( 112.8299879122683791, -27.27019477826133453, 49.62895860924498947 ) ) ;
#14503=ORIENTED_EDGE ( 'NONE', *, *, #57742, .F. ) ;
#14506=DIRECTION ( 'NONE',  ( 0.000000000000000000, 0.000000000000000000, 1.000000000000000000 ) ) ;
#14508=CARTESIAN_POINT ( 'NONE',  ( 117.3720538532506623, -35.57445771113446398, 229.9032443235289520 ) ) ;
#14509=AXIS2_PLACEMENT_3D ( 'NONE', #31984, #59678, #65177 ) ;
#14510=CYLINDRICAL_SURFACE ( 'NONE', #31275, 13.00000000000000355 ) ;
#14511=CARTESIAN_POINT ( 'NONE',  ( 109.9668656698224538, -46.07028316908876775, 93.81562527591097478 ) ) ;
#14513=CARTESIAN_POINT ( 'NONE',  ( 98.34954641256851460, -31.65714432329926709, 21.90643418995717795 ) ) ;
#14514=VERTEX_POINT ( 'NONE', #53239 ) ;
#14515=CYLINDRICAL_SURFACE ( 'NONE', #9561, 2.116999999999993776 ) ;
#14516=ORIENTED_EDGE ( 'NONE', *, *, #7054, .T. ) ;
#14518=VECTOR ( 'NONE', #4121, 1000.000000000000000 ) ;
#14520=CARTESIAN_POINT ( 'NONE',  ( 111.6760726031484978, -44.91652306731177902, 254.4282499725637479 ) ) ;
#14521=CARTESIAN_POINT ( 'NONE',  ( 107.0664832912739968, -36.72944715994100306, 9.635625275910941312 ) ) ;
#14522=CARTESIAN_POINT ( 'NONE',  ( 97.31585367440334267, -39.30600031747468392, 141.5314607004144705 ) ) ;
#14523=PLANE ( 'NONE',  #79542 ) ;
#14527=DIRECTION ( 'NONE',  ( 1.147230458779309805E-16, 3.204747427460360459E-31, 1.000000000000000000 ) ) ;
#14529=ORIENTED_EDGE ( 'NONE', *, *, #18781, .F. ) ;
#14530=CARTESIAN_POINT ( 'NONE',  ( 100.4790876285538275, -27.85333844968608830, 35.59657765686397113 ) ) ;
#14532=B_SPLINE_CURVE_WITH_KNOTS ( 'NONE', 3,
 ( #22210, #56701, #14039, #43063, #14945, #84445, #27665, #83099, #49884, #48518, #20852, #70802, #63986, #28098, #21762, #28548, #853, #83990, #36274, #49432, #77613, #41720, #29463, #55781, #6771, #15394, #50332, #42614, #42172, #69902, #8574 ),
 .UNSPECIFIED., .F., .F.,
 ( 4, 2, 2, 1, 2, 2, 2, 2, 2, 2, 2, 1, 1, 2, 2, 2, 4 ),
 ( 0.000000000000000000, 0.06250000000001065814, 0.09375000000001587619, 0.1093750000000143774, 0.1171875000000136280, 0.1250000000000128786, 0.1875000000000279499, 0.2187500000000324185, 0.2500000000000368594, 0.3125000000000400235, 0.3437500000000436873, 0.3593750000000451306, 0.3671875000000462963, 0.3710937500000464073, 0.3750000000000465183, 0.4375000000000232592, 0.5000000000000000000 ),
 .UNSPECIFIED. ) ;
#14533=EDGE_CURVE ( 'NONE', #53830, #89358, #16823, .T. ) ;
#14534=CARTESIAN_POINT ( 'NONE',  ( 114.7745679063646378, -33.04956858091291139, 18.60384839950496172 ) ) ;
#14536=CARTESIAN_POINT ( 'NONE',  ( 98.71823956546961654, -31.63334453281603587, 170.8899109901969950 ) ) ;
#14537=LINE ( 'NONE', #42216, #59271 ) ;
#14539=DIRECTION ( 'NONE',  ( 0.000000000000000000, 2.135044278125299371E-15, -1.000000000000000000 ) ) ;
#14540=DIRECTION ( 'NONE',  ( -0.7071067811865192621, -0.7071067811865758834, -7.071067811865185427E-16 ) ) ;
#14542=CARTESIAN_POINT ( 'NONE',  ( 100.5841487926172277, -28.49196697857695781, 11.60705384733995515 ) ) ;
#14546=CARTESIAN_POINT ( 'NONE',  ( 136.7635286919469593, -37.26660482608871661, 6.827192804310227459 ) ) ;
#14548=CARTESIAN_POINT ( 'NONE',  ( 96.65590158217011663, -37.83070472558634378, 122.4099109901969626 ) ) ;
#14551=DIRECTION ( 'NONE',  ( 1.054009200593500181E-15, 1.000000000000000000, 0.000000000000000000 ) ) ;
#14552=ORIENTED_EDGE ( 'NONE', *, *, #3874, .T. ) ;
#14554=EDGE_CURVE ( 'NONE', #7464, #63748, #77769, .T. ) ;
#14561=CARTESIAN_POINT ( 'NONE',  ( 126.0667039024479266, -14.72944715994094977, 239.5838068554170377 ) ) ;
#14562=CARTESIAN_POINT ( 'NONE',  ( 138.8664832912739939, -71.52944715994085811, 361.9756252759100335 ) ) ;
#14563=CARTESIAN_POINT ( 'NONE',  ( 115.4543170047500098, -34.59750657913997429, 166.8547570362579506 ) ) ;
#14564=CARTESIAN_POINT ( 'NONE',  ( 114.4303731589454998, -27.41304352248915777, 270.5441967044823741 ) ) ;
#14566=VERTEX_POINT ( 'NONE', #89147 ) ;
#14567=DIRECTION ( 'NONE',  ( -1.000000000000000078E-15, 1.000000000000000083E-30, 1.000000000000000000 ) ) ;
#14572=CARTESIAN_POINT ( 'NONE',  ( 82.81651833456541567, -18.90056224776904159, 3.101534470965027435 ) ) ;
#14573=PLANE ( 'NONE',  #89027 ) ;
#14574=CARTESIAN_POINT ( 'NONE',  ( 104.4898988706324445, -26.97882157938011360, 15.28146304136766354 ) ) ;
#14575=PLANE ( 'NONE',  #40498 ) ;
#14576=CARTESIAN_POINT ( 'NONE',  ( 125.0664851986225159, -56.72944715994083964, 14.82207188531762654 ) ) ;
#14578=CARTESIAN_POINT ( 'NONE',  ( 107.4755550402934148, -45.77628807984756065, 192.0228960185529559 ) ) ;
#14579=CARTESIAN_POINT ( 'NONE',  ( 110.1710482807090585, -46.72786414817543488, 97.81562527591097478 ) ) ;
#14580=ORIENTED_EDGE ( 'NONE', *, *, #39762, .T. ) ;
#14581=DIRECTION ( 'NONE',  ( 0.000000000000000000, -1.000000000000000000, 0.000000000000000000 ) ) ;
#14582=VERTEX_POINT ( 'NONE', #26909 ) ;
#14586=ORIENTED_EDGE ( 'NONE', *, *, #48016, .T. ) ;
#14588=CARTESIAN_POINT ( 'NONE',  ( 41.56648329127398966, -27.57844715994070484, 78.92562527591199739 ) ) ;
#14589=CARTESIAN_POINT ( 'NONE',  ( 73.06648329127399677, -8.729447159941065237, -4.824374724089063982 ) ) ;
#14593=CARTESIAN_POINT ( 'NONE',  ( 117.5098600993040066, -37.01623072280121107, 43.80419670448293346 ) ) ;
#14595=CYLINDRICAL_SURFACE ( 'NONE', #5086, 5.599999999999994316 ) ;
#14596=ADVANCED_FACE ( 'NONE', ( #38744 ), #80109, .T. ) ;
#14598=CARTESIAN_POINT ( 'NONE',  ( 128.2504969244201334, -12.91928723231331588, 361.9756252759100903 ) ) ;
#14601=CARTESIAN_POINT ( 'NONE',  ( 105.6559524084447617, -26.80454636418725656, 121.1869003628085579 ) ) ;
#14602=LINE ( 'NONE', #36388, #49809 ) ;
#14603=CARTESIAN_POINT ( 'NONE',  ( 90.44969454456422397, -23.41243780205712710, 249.5838068554174924 ) ) ;
#14604=VECTOR ( 'NONE', #73122, 1000.000000000000000 ) ;
#14605=CARTESIAN_POINT ( 'NONE',  ( 96.00479252368074867, -37.29883552165912874, 117.3794347997199594 ) ) ;
#14606=LINE ( 'NONE', #7339, #10182 ) ;
#14608=FACE_OUTER_BOUND ( 'NONE', #66225, .T. ) ;
#14611=ADVANCED_FACE ( 'NONE', ( #87359 ), #80547, .F. ) ;
#14612=B_SPLINE_CURVE_WITH_KNOTS ( 'NONE', 3,
 ( #16676, #38009, #80697, #39344, #44362, #44811 ),
 .UNSPECIFIED., .F., .F.,
 ( 4, 2, 4 ),
 ( 0.9103247092270834173, 0.9551623546135417087, 1.000000000000000000 ),
 .UNSPECIFIED. ) ;
#14614=CARTESIAN_POINT ( 'NONE',  ( 113.4935171807053536, -28.59114140144097860, 120.5565776568629559 ) ) ;
#14615=AXIS2_PLACEMENT_3D ( 'NONE', #50397, #78143, #15901 ) ;
#14618=CARTESIAN_POINT ( 'NONE',  ( 106.2286657330468245, -47.72771449247510844, 263.5280062282920994 ) ) ;
#14619=CARTESIAN_POINT ( 'NONE',  ( 97.81399931465544739, -40.51646775427786196, 252.6355816051047896 ) ) ;
#14622=LINE ( 'NONE', #50010, #39824 ) ;
#14623=EDGE_CURVE ( 'NONE', #80786, #28614, #21453, .T. ) ;
#14624=DIRECTION ( 'NONE',  ( -1.175184669632759901E-16, 1.000000000000000000, 2.000000000000003705E-15 ) ) ;
#14626=CARTESIAN_POINT ( 'NONE',  ( 99.07755742602699911, -44.46178485432853478, 191.9384824187689560 ) ) ;
#14628=EDGE_LOOP ( 'NONE', ( #34198, #63678, #83983, #8222 ) ) ;
#14629=CARTESIAN_POINT ( 'NONE',  ( 105.5787418010314695, -46.69191849206237066, 143.8901547344689789 ) ) ;
#14631=CARTESIAN_POINT ( 'NONE',  ( 97.82556271424805061, -33.52526948863204126, 282.0613395616247772 ) ) ;
#14633=EDGE_CURVE ( 'NONE', #85887, #77884, #69597, .T. ) ;
#14635=CARTESIAN_POINT ( 'NONE',  ( 116.8174800920801317, -34.15430197086818254, 269.0316147097951216 ) ) ;
#14636=DIRECTION ( 'NONE',  ( 0.000000000000000000, 0.000000000000000000, -1.000000000000000000 ) ) ;
#14638=CARTESIAN_POINT ( 'NONE',  ( 90.44969454456416713, -53.34645651782494724, 219.5838068554169809 ) ) ;
#14640=B_SPLINE_CURVE_WITH_KNOTS ( 'NONE', 3,
 ( #16224, #56297, #31614, #10288, #86601, #30291, #23050, #71635, #44799, #24373, #58864, #65689, #43901, #30733, #37993, #9400, #2595, #72953 ),
 .UNSPECIFIED., .F., .F.,
 ( 4, 2, 2, 2, 2, 2, 2, 2, 4 ),
 ( 0.000000000000000000, 0.06249999963049208268, 0.1249999992609841654, 0.1874999988914762550, 0.2499999985219683307, 0.3124999981524604342, 0.3749999977829525100, 0.4374999974134445857, 0.4999999970439366614 ),
 .UNSPECIFIED. ) ;
#14641=CARTESIAN_POINT ( 'NONE',  ( 96.70388795518319114, -35.81005419191407668, 231.2556252759109725 ) ) ;
#14642=CARTESIAN_POINT ( 'NONE',  ( 128.5492039024480277, -43.72944715994093912, 231.5838068554170093 ) ) ;
#14643=ORIENTED_EDGE ( 'NONE', *, *, #71655, .T. ) ;
#14644=EDGE_CURVE ( 'NONE', #60102, #45673, #35056, .T. ) ;
#14647=CARTESIAN_POINT ( 'NONE',  ( 82.77657790094413315, -19.19711456032067787, 6.808568500765782794 ) ) ;
#14648=FACE_OUTER_BOUND ( 'NONE', #39241, .T. ) ;
#14649=CARTESIAN_POINT ( 'NONE',  ( 21.03715912545738220, -47.82818131006197149, 193.9678068554150627 ) ) ;
#14650=AXIS2_PLACEMENT_3D ( 'NONE', #44599, #72336, #49628 ) ;
#14655=CARTESIAN_POINT ( 'NONE',  ( 96.77253738264830929, -34.86918258059447595, 241.1841967044819626 ) ) ;
#14656=ORIENTED_EDGE ( 'NONE', *, *, #5838, .T. ) ;
#14658=CYLINDRICAL_SURFACE ( 'NONE', #79663, 9.999999999999998224 ) ;
#14659=CARTESIAN_POINT ( 'NONE',  ( 97.81168895331838087, -40.51742574516882200, 287.6356252759109680 ) ) ;
#14660=EDGE_CURVE ( 'NONE', #60222, #11985, #84134, .T. ) ;
#14662=ADVANCED_FACE ( 'NONE', ( #27802 ), #543, .T. ) ;
#14663=CARTESIAN_POINT ( 'NONE',  ( 109.9854453146643039, -44.35239847312019634, 60.68523322673397047 ) ) ;
#14664=CARTESIAN_POINT ( 'NONE',  ( 112.7920458925406422, -45.46759294451666022, 174.0384824187679556 ) ) ;
#14667=VERTEX_POINT ( 'NONE', #48227 ) ;
#14668=EDGE_CURVE ( 'NONE', #2787, #9116, #70044, .T. ) ;
#14669=DIRECTION ( 'NONE',  ( 0.9242245927363031965, 0.3818493186865917766, 0.000000000000000000 ) ) ;
#14670=ORIENTED_EDGE ( 'NONE', *, *, #14902, .F. ) ;
#14673=DIRECTION ( 'NONE',  ( 1.000000000000000000, 4.299999999999999979E-14, 1.000000000000000078E-15 ) ) ;
#14676=CARTESIAN_POINT ( 'NONE',  ( 107.0664832912730020, -27.87844715994269862, 361.9756252759109998 ) ) ;
#14678=CARTESIAN_POINT ( 'NONE',  ( 115.4827349520354858, -33.38588942772360468, 98.56194363760096167 ) ) ;
#14679=CIRCLE ( 'NONE', #87165, 1.219499999999975159 ) ;
#14680=CARTESIAN_POINT ( 'NONE',  ( 118.3649377238561300, -33.07154184081399961, 284.0756252759109657 ) ) ;
#14681=CARTESIAN_POINT ( 'NONE',  ( 99.10268845779062019, -29.98093639561593449, 215.7670538473399517 ) ) ;
#14682=DIRECTION ( 'NONE',  ( -2.283216351027200160E-14, 0.000000000000000000, 1.000000000000000000 ) ) ;
#14684=VERTEX_POINT ( 'NONE', #55482 ) ;
#14688=CARTESIAN_POINT ( 'NONE',  ( 108.8662857618680562, -46.94215964495590043, 122.7032443235309671 ) ) ;
#14689=CARTESIAN_POINT ( 'NONE',  ( 106.9267615183890854, -26.22553017860169433, 60.08705384733897858 ) ) ;
#14690=CARTESIAN_POINT ( 'NONE',  ( 112.5123584215844659, -46.40184746663635451, 257.9965776568634510 ) ) ;
#14692=CARTESIAN_POINT ( 'NONE',  ( 106.5673262220758772, -47.17821497701651623, 247.5384824187679556 ) ) ;
#14693=DIRECTION ( 'NONE',  ( 1.000000000000000000, -1.000000000000000078E-15, 0.000000000000000000 ) ) ;
#14696=CARTESIAN_POINT ( 'NONE',  ( 99.18883298691498851, -42.92813836781478898, 27.85781585569052154 ) ) ;
#14697=CARTESIAN_POINT ( 'NONE',  ( 134.0664832912740110, -8.350947159940998787, 7.443125275912000127 ) ) ;
#14700=CARTESIAN_POINT ( 'NONE',  ( 51.42025729302500281, -31.94127993907734719, 117.4678068554150485 ) ) ;
#14702=AXIS2_PLACEMENT_3D ( 'NONE', #73124, #51330, #44518 ) ;
#14704=CARTESIAN_POINT ( 'NONE',  ( 104.4899544214444944, -26.97880759237127180, 11.28145861166093766 ) ) ;
#14705=DIRECTION ( 'NONE',  ( -0.7071067811865475727, 0.7071067811865475727, 0.000000000000000000 ) ) ;
#14706=CARTESIAN_POINT ( 'NONE',  ( 108.4174892377433252, -26.73503592547494634, 259.9689586103912688 ) ) ;
#14707=ORIENTED_EDGE ( 'NONE', *, *, #2548, .F. ) ;
#14709=CARTESIAN_POINT ( 'NONE',  ( 96.22633597390384352, -34.45202597047101278, 261.1737205140064475 ) ) ;
#14710=CARTESIAN_POINT ( 'NONE',  ( 103.4684036848089050, -46.51393990267121836, 138.2956252759109645 ) ) ;
#14711=CARTESIAN_POINT ( 'NONE',  ( 118.5948618896802742, -33.89272371608580414, 10.01848241876795953 ) ) ;
#14712=DIRECTION ( 'NONE',  ( 0.000000000000000000, 0.000000000000000000, 1.000000000000000000 ) ) ;
#14714=DIRECTION ( 'NONE',  ( 0.6544127834855474335, 0.2678505344604093508, 0.7071067811865271446 ) ) ;
#14715=CARTESIAN_POINT ( 'NONE',  ( 81.63820548406727085, -34.47341874818841490, 7.827313014938356517 ) ) ;
#14716=CARTESIAN_POINT ( 'NONE',  ( 98.54777178369499779, -41.97717499081849013, 137.7658220778284317 ) ) ;
#14717=VECTOR ( 'NONE', #35309, 1000.000000000000000 ) ;
#14718=EDGE_CURVE ( 'NONE', #770, #54421, #61864, .T. ) ;
#14719=ORIENTED_EDGE ( 'NONE', *, *, #53939, .F. ) ;
#14720=EDGE_CURVE ( 'NONE', #12518, #87053, #73469, .T. ) ;
#14723=CARTESIAN_POINT ( 'NONE',  ( 109.3519496323076083, -28.49945473430254950, 174.2838483995049899 ) ) ;
#14725=DIRECTION ( 'NONE',  ( 1.000000000000000000, 4.299999999999999979E-14, 1.000000000000000078E-15 ) ) ;
#14726=ORIENTED_EDGE ( 'NONE', *, *, #59704, .F. ) ;
#14728=CARTESIAN_POINT ( 'NONE',  ( 113.6008039948045649, -28.63430547549730676, 160.5356252759109736 ) ) ;
#14729=CARTESIAN_POINT ( 'NONE',  ( 172.5664832912740110, -18.82844715994099971, 18.92562527591200094 ) ) ;
#14731=CARTESIAN_POINT ( 'NONE',  ( 107.7705136438765550, -26.73286797099179424, 86.02129597068410760 ) ) ;
#14733=AXIS2_PLACEMENT_3D ( 'NONE', #46546, #68359, #59289 ) ;
#14734=EDGE_CURVE ( 'NONE', #88862, #46552, #42982, .T. ) ;
#14737=CARTESIAN_POINT ( 'NONE',  ( 106.6854394624702707, -26.95610377642487165, 85.10705384733996937 ) ) ;
#14740=CIRCLE ( 'NONE', #61138, 2.517500000000005844 ) ;
#14741=VERTEX_POINT ( 'NONE', #89599 ) ;
#14743=CARTESIAN_POINT ( 'NONE',  ( 115.7370193921850898, -38.55977017368898174, 60.09301187732596361 ) ) ;
#14744=DIRECTION ( 'NONE',  ( 0.7071067811868717579, 0.7071067811862232766, 7.071067811868711635E-16 ) ) ;
#14745=CARTESIAN_POINT ( 'NONE',  ( 116.7742277529939230, -35.53649587948896027, 189.9241967044819717 ) ) ;
#14746=CARTESIAN_POINT ( 'NONE',  ( 115.0372575324259401, -42.90846253205904759, 38.30229194598641129 ) ) ;
#14747=CARTESIAN_POINT ( 'NONE',  ( 172.5664832912740110, -36.32844715994070839, 143.6756252759119832 ) ) ;
#14749=DIRECTION ( 'NONE',  ( 0.000000000000000000, 0.000000000000000000, -1.000000000000000000 ) ) ;
#14752=DIRECTION ( 'NONE',  ( 1.000000000000000000, 3.999999999999999995E-14, 1.000000000000000078E-15 ) ) ;
#14755=CARTESIAN_POINT ( 'NONE',  ( 109.2504006710444315, -46.93703897017543625, 107.7441967044829880 ) ) ;
#14756=VERTEX_POINT ( 'NONE', #6914 ) ;
#14757=VERTEX_POINT ( 'NONE', #83236 ) ;
#14760=LINE ( 'NONE', #64241, #58936 ) ;
#14762=CARTESIAN_POINT ( 'NONE',  ( 108.4158484965001890, -26.73482408474558270, 129.9690911813341927 ) ) ;
#14763=CARTESIAN_POINT ( 'NONE',  ( 116.3212776292292716, -32.94146857471233147, 105.1356252759109680 ) ) ;
#14764=CARTESIAN_POINT ( 'NONE',  ( 114.3567987304369495, -40.40109894280344349, 201.2738046553059803 ) ) ;
#14765=CARTESIAN_POINT ( 'NONE',  ( 37.03715912545425937, -48.62818131006122258, 313.9678068554150059 ) ) ;
#14766=CARTESIAN_POINT ( 'NONE',  ( 109.7258523471263914, -27.00106681210123938, 25.86424884311490047 ) ) ;
#14767=VERTEX_POINT ( 'NONE', #9602 ) ;
#14768=ORIENTED_EDGE ( 'NONE', *, *, #39603, .T. ) ;
#14769=ORIENTED_EDGE ( 'NONE', *, *, #88491, .T. ) ;
#14770=VECTOR ( 'NONE', #48626, 1000.000000000000000 ) ;
#14771=EDGE_CURVE ( 'NONE', #65869, #69742, #47323, .T. ) ;
#14774=ORIENTED_EDGE ( 'NONE', *, *, #76149, .T. ) ;
#14775=CARTESIAN_POINT ( 'NONE',  ( 77.97204591021541376, -20.52018918698335170, 7.480061334675825790 ) ) ;
#14776=EDGE_CURVE ( 'NONE', #59253, #28372, #2426, .T. ) ;
#14777=ADVANCED_FACE ( 'NONE', ( #71400 ), #36428, .T. ) ;
#14778=CARTESIAN_POINT ( 'NONE',  ( 111.6760726031484978, -44.91652306731177902, 254.4282499725637479 ) ) ;
#14779=CARTESIAN_POINT ( 'NONE',  ( 105.7999286771159149, -26.72397919236279762, 181.1777144871696237 ) ) ;
#14780=ORIENTED_EDGE ( 'NONE', *, *, #30314, .F. ) ;
#14781=EDGE_CURVE ( 'NONE', #89690, #46099, #57748, .T. ) ;
#14782=AXIS2_PLACEMENT_3D ( 'NONE', #68098, #40383, #33568 ) ;
#14785=VERTEX_POINT ( 'NONE', #64571 ) ;
#14786=ORIENTED_EDGE ( 'NONE', *, *, #68942, .F. ) ;
#14787=CYLINDRICAL_SURFACE ( 'NONE', #69668, 2.030000000002086580 ) ;
#14788=EDGE_LOOP ( 'NONE', ( #22564, #68338, #81411, #43003 ) ) ;
#14790=CARTESIAN_POINT ( 'NONE',  ( 114.0298635175061008, -31.59016113260716097, 257.1385665600676589 ) ) ;
#14791=CARTESIAN_POINT ( 'NONE',  ( 98.26213988389305598, -31.03978702703054537, 145.8699109901969848 ) ) ;
#14792=CARTESIAN_POINT ( 'NONE',  ( 114.5517459224756749, -44.00510994954056088, 98.21276813305395592 ) ) ;
#14793=DIRECTION ( 'NONE',  ( 0.000000000000000000, 0.000000000000000000, 1.000000000000000000 ) ) ;
#14794=FILL_AREA_STYLE_COLOUR ( '', #80074 ) ;
#14795=CARTESIAN_POINT ( 'NONE',  ( 98.94264532560653436, -30.19601435972772308, 236.7870538473399336 ) ) ;
#14798=ORIENTED_EDGE ( 'NONE', *, *, #35421, .F. ) ;
#14799=LINE ( 'NONE', #7968, #58414 ) ;
#14800=ORIENTED_EDGE ( 'NONE', *, *, #71834, .T. ) ;
#14803=LINE ( 'NONE', #69309, #63452 ) ;
#14804=CARTESIAN_POINT ( 'NONE',  ( 110.1409620311622604, -27.17888879385625600, 135.8284909550441455 ) ) ;
#14807=CARTESIAN_POINT ( 'NONE',  ( 99.68446536626322541, -46.00016974189506413, 122.0413395616249659 ) ) ;
#14808=PLANE ( 'NONE',  #41700 ) ;
#14809=CARTESIAN_POINT ( 'NONE',  ( 135.7892066358211594, -34.57943358557326263, 7.744922197164725297 ) ) ;
#14812=DIRECTION ( 'NONE',  ( 0.000000000000000000, 1.000000000000000000, 0.000000000000000000 ) ) ;
#14813=CARTESIAN_POINT ( 'NONE',  ( 100.1532602078033278, -44.50350736857013345, 262.9984824187678782 ) ) ;
#14816=VECTOR ( 'NONE', #41246, 1000.000000000000000 ) ;
#14818=DIRECTION ( 'NONE',  ( 0.000000000000000000, -1.000000000000000000, 0.000000000000000000 ) ) ;
#14819=DIRECTION ( 'NONE',  ( -1.000000000000000078E-15, 0.000000000000000000, -1.000000000000000000 ) ) ;
#14820=CIRCLE ( 'NONE', #59714, 2.500000000000002220 ) ;
#14821=CARTESIAN_POINT ( 'NONE',  ( 144.8664832912739939, -71.52944715994085811, 361.9756252759100335 ) ) ;
#14822=CARTESIAN_POINT ( 'NONE',  ( 96.93601811142059432, -39.37148068186442629, 276.5299109901966403 ) ) ;
#14823=ORIENTED_EDGE ( 'NONE', *, *, #11065, .T. ) ;
#14824=VECTOR ( 'NONE', #43450, 1000.000000000000000 ) ;
#14826=CARTESIAN_POINT ( 'NONE',  ( 117.8019377669635190, -34.00081044253764162, 169.0365776568629599 ) ) ;
#14827=CARTESIAN_POINT ( 'NONE',  ( 100.9411170126626587, -46.87412574091977291, 48.14419670448194211 ) ) ;
#14828=CARTESIAN_POINT ( 'NONE',  ( 117.2345208925008109, -41.18012235578145663, 204.4861014663869696 ) ) ;
#14830=CARTESIAN_POINT ( 'NONE',  ( 30.48091746481826192, -48.32844715994148999, 300.4678068554150059 ) ) ;
#14831=CYLINDRICAL_SURFACE ( 'NONE', #39156, 1.000000000000000888 ) ;
#14832=DIRECTION ( 'NONE',  ( 1.000000000000000000, 4.163336342344333240E-14, 0.000000000000000000 ) ) ;
#14833=CARTESIAN_POINT ( 'NONE',  ( 109.7248659280113827, -27.00080518171892052, 69.86479194203108989 ) ) ;
#14835=ORIENTED_EDGE ( 'NONE', *, *, #17689, .F. ) ;
#14836=CARTESIAN_POINT ( 'NONE',  ( 40.31648329127299490, 12.92155284005730387, 355.9756252759109998 ) ) ;
#14837=EDGE_CURVE ( 'NONE', #18507, #28799, #65016, .T. ) ;
#14838=ORIENTED_EDGE ( 'NONE', *, *, #51929, .T. ) ;
#14840=ORIENTED_EDGE ( 'NONE', *, *, #16190, .T. ) ;
#14841=ADVANCED_FACE ( 'NONE', ( #37311 ), #57525, .F. ) ;
#14842=DIRECTION ( 'NONE',  ( 0.000000000000000000, 0.000000000000000000, -1.000000000000000000 ) ) ;
#14843=ORIENTED_EDGE ( 'NONE', *, *, #10985, .T. ) ;
#14844=CARTESIAN_POINT ( 'NONE',  ( 110.4495079430909357, -47.22796928374258130, 53.83657765686300678 ) ) ;
#14845=DIRECTION ( 'NONE',  ( 0.1858654558203195195, -0.9825752044157765042, 0.000000000000000000 ) ) ;
#14846=LINE ( 'NONE', #63424, #66006 ) ;
#14848=CARTESIAN_POINT ( 'NONE',  ( 98.63080892621665896, -30.47026088752560824, 176.8184824187679567 ) ) ;
#14849=AXIS2_PLACEMENT_3D ( 'NONE', #80734, #18484, #11690 ) ;
#14850=CARTESIAN_POINT ( 'NONE',  ( 98.20387719113243463, -34.86749027545791080, 260.5962293518865636 ) ) ;
#14852=ORIENTED_EDGE ( 'NONE', *, *, #40949, .T. ) ;
#14853=ORIENTED_EDGE ( 'NONE', *, *, #79427, .T. ) ;
#14854=ADVANCED_FACE ( 'NONE', ( #85032 ), #29600, .T. ) ;
#14855=AXIS2_PLACEMENT_3D ( 'NONE', #49366, #77102, #70273 ) ;
#14857=LINE ( 'NONE', #42968, #67444 ) ;
#14858=FACE_OUTER_BOUND ( 'NONE', #81382, .T. ) ;
#14860=CARTESIAN_POINT ( 'NONE',  ( 188.5667039024479834, -67.87844715994100397, 173.2178068554149775 ) ) ;
#14864=CARTESIAN_POINT ( 'NONE',  ( 32.25690895536984470, -33.54226604285049262, 117.4678068554150485 ) ) ;
#14865=FACE_OUTER_BOUND ( 'NONE', #38446, .T. ) ;
#14866=CARTESIAN_POINT ( 'NONE',  ( 118.0525141433398773, -37.71481444994964960, 33.74324432352998571 ) ) ;
#14867=DIRECTION ( 'NONE',  ( 0.000000000000000000, -1.000000000000000000, 0.000000000000000000 ) ) ;
#14868=AXIS2_PLACEMENT_3D ( 'NONE', #4904, #32593, #46207 ) ;
#14869=ADVANCED_FACE ( 'NONE', ( #58626 ), #85927, .F. ) ;
#14870=EDGE_LOOP ( 'NONE', ( #8174, #45344, #70957, #8858 ) ) ;
#14871=DIRECTION ( 'NONE',  ( 2.900000000000000265E-14, -2.000000000000000155E-15, 1.000000000000000000 ) ) ;
#14872=FACE_BOUND ( 'NONE', #49170, .T. ) ;
#14873=CARTESIAN_POINT ( 'NONE',  ( 115.1946057043837328, -37.48001498139237953, 76.57094751244896713 ) ) ;
#14876=CIRCLE ( 'NONE', #17775, 0.5000000000000004441 ) ;
#14877=FACE_OUTER_BOUND ( 'NONE', #14347, .T. ) ;
#14879=ORIENTED_EDGE ( 'NONE', *, *, #54997, .T. ) ;
#14880=CARTESIAN_POINT ( 'NONE',  ( 108.3336695260893094, -46.73483522987581296, 137.6750204624211733 ) ) ;
#14881=ORIENTED_EDGE ( 'NONE', *, *, #24337, .F. ) ;
#14883=CARTESIAN_POINT ( 'NONE',  ( 115.7125814391468737, -38.67428926243481158, 145.0815833058969702 ) ) ;
#14885=EDGE_CURVE ( 'NONE', #46008, #39822, #10054, .T. ) ;
#14886=CARTESIAN_POINT ( 'NONE',  ( 108.3220630915710530, -47.10059840840933987, 113.6727681330539639 ) ) ;
#14887=DIRECTION ( 'NONE',  ( 1.000000000000000078E-15, -1.000000000000000000, 0.000000000000000000 ) ) ;
#14888=ORIENTED_EDGE ( 'NONE', *, *, #85729, .T. ) ;
#14889=VERTEX_POINT ( 'NONE', #86362 ) ;
#14891=AXIS2_PLACEMENT_3D ( 'NONE', #78076, #43517, #36730 ) ;
#14892=CARTESIAN_POINT ( 'NONE',  ( 130.5667039024479834, -36.72944715994093912, 239.5838068554170377 ) ) ;
#14893=ORIENTED_EDGE ( 'NONE', *, *, #43004, .F. ) ;
#14894=CARTESIAN_POINT ( 'NONE',  ( 97.21286698537356585, -39.96429565625729907, 286.5908633711495668 ) ) ;
#14895=CARTESIAN_POINT ( 'NONE',  ( 113.5786777234211939, -44.94349119991360197, 164.1099109901969655 ) ) ;
#14896=CARTESIAN_POINT ( 'NONE',  ( 193.0371591254586008, -47.82818131005411999, 193.9678068554150343 ) ) ;
#14898=CARTESIAN_POINT ( 'NONE',  ( 97.83606632657298974, -31.88363555591887533, 131.9413395616259947 ) ) ;
#14901=CARTESIAN_POINT ( 'NONE',  ( 25.56670390244797275, -67.87844715994100397, 132.3428068554150343 ) ) ;
#14902=EDGE_CURVE ( 'NONE', #48061, #63918, #63302, .T. ) ;
#14903=ORIENTED_EDGE ( 'NONE', *, *, #72157, .T. ) ;
#14904=CARTESIAN_POINT ( 'NONE',  ( 20.03715912545826328, -46.82818131006190043, 237.4678068554150059 ) ) ;
#14905=ORIENTED_EDGE ( 'NONE', *, *, #23526, .F. ) ;
#14906=AXIS2_PLACEMENT_3D ( 'NONE', #66353, #46791, #11855 ) ;
#14907=EDGE_CURVE ( 'NONE', #78010, #5742, #35632, .T. ) ;
#14909=LINE ( 'NONE', #42572, #58047 ) ;
#14910=CARTESIAN_POINT ( 'NONE',  ( 115.6114045197296178, -28.51818617053012161, 39.43562527591099354 ) ) ;
#14913=LINE ( 'NONE', #77578, #49935 ) ;
#14914=CARTESIAN_POINT ( 'NONE',  ( 111.0600676157742726, -27.80113716294804505, 24.74133956162494030 ) ) ;
#14915=CYLINDRICAL_SURFACE ( 'NONE', #62309, 9.999999999999998224 ) ;
#14916=CARTESIAN_POINT ( 'NONE',  ( 105.3199149336540046, -48.42511963160323774, 143.4584824187689662 ) ) ;
#14918=LINE ( 'NONE', #78499, #49593 ) ;
#14919=VERTEX_POINT ( 'NONE', #25015 ) ;
#14920=LINE ( 'NONE', #83504, #12066 ) ;
#14925=CARTESIAN_POINT ( 'NONE',  ( 115.0734612967709722, -29.04171753102041365, 189.4232443235299570 ) ) ;
#14926=ORIENTED_EDGE ( 'NONE', *, *, #58792, .F. ) ;
#14927=DIRECTION ( 'NONE',  ( 0.000000000000000000, 0.000000000000000000, 1.000000000000000000 ) ) ;
#14928=CARTESIAN_POINT ( 'NONE',  ( 96.66048121734328902, -35.80620304765527351, 227.2556252759109725 ) ) ;
#14929=CARTESIAN_POINT ( 'NONE',  ( 101.1169593292293598, -28.07258979649007102, 46.55562527591094835 ) ) ;
#14930=CARTESIAN_POINT ( 'NONE',  ( 29.77381068363477112, -48.62134037875501491, 300.4678068554150059 ) ) ;
#14931=CARTESIAN_POINT ( 'NONE',  ( 95.60734603896362671, -36.72944715994100306, 293.2242906452868851 ) ) ;
#14932=DIRECTION ( 'NONE',  ( 2.775557561562888827E-14, -1.000000000000000000, 0.000000000000000000 ) ) ;
#14936=EDGE_LOOP ( 'NONE', ( #74851, #58832 ) ) ;
#14939=AXIS2_PLACEMENT_3D ( 'NONE', #1521, #22410, #50087 ) ;
#14940=EDGE_CURVE ( 'NONE', #31872, #39210, #11836, .T. ) ;
#14941=ORIENTED_EDGE ( 'NONE', *, *, #55507, .F. ) ;
#14943=CARTESIAN_POINT ( 'NONE',  ( 101.6506511131177461, -45.63737897744897509, 243.1413395616249886 ) ) ;
#14945=CARTESIAN_POINT ( 'NONE',  ( 134.8111839727964139, -16.08035908359601507, 1.709393751552864993 ) ) ;
#14947=DIRECTION ( 'NONE',  ( 0.000000000000000000, 1.000000000000000000, 0.000000000000000000 ) ) ;
#14949=CARTESIAN_POINT ( 'NONE',  ( 91.06648329127391150, -36.72944715993925513, -5.074374724089045330 ) ) ;
#14950=CARTESIAN_POINT ( 'NONE',  ( 104.2349294074198411, -46.78572220631293277, 22.35848241876792031 ) ) ;
#14952=ORIENTED_EDGE ( 'NONE', *, *, #55209, .T. ) ;
#14955=CARTESIAN_POINT ( 'NONE',  ( 97.78098940324528598, -40.44159231346958450, 17.62882595293030619 ) ) ;
#14956=CARTESIAN_POINT ( 'NONE',  ( 107.2379402074490855, -25.61267671046461558, 226.0641967044819580 ) ) ;
#14958=DIRECTION ( 'NONE',  ( 4.012088370409549976E-14, -1.000000000000000000, 0.000000000000000000 ) ) ;
#14959=CIRCLE ( 'NONE', #25057, 2.517500000000005844 ) ;
#14960=CARTESIAN_POINT ( 'NONE',  ( 116.5944731948637809, -42.45914096480943556, 124.3956252759109731 ) ) ;
#14962=CARTESIAN_POINT ( 'NONE',  ( 103.2794297788319966, -27.47427420437042755, 21.38554664520359694 ) ) ;
#14966=ORIENTED_EDGE ( 'NONE', *, *, #48849, .T. ) ;
#14968=CARTESIAN_POINT ( 'NONE',  ( 101.7809741706781921, -43.87965855000975068, 253.5015833058971850 ) ) ;
#14969=CARTESIAN_POINT ( 'NONE',  ( 105.7154772450396081, -46.72385838138438174, 192.4689586024476853 ) ) ;
#14970=CYLINDRICAL_SURFACE ( 'NONE', #81259, 4.874999999999990230 ) ;
#14973=ORIENTED_EDGE ( 'NONE', *, *, #22510, .T. ) ;
#14975=CARTESIAN_POINT ( 'NONE',  ( 105.7142056743471557, -46.72366556389629011, 183.4694020350319477 ) ) ;
#14976=ORIENTED_EDGE ( 'NONE', *, *, #8436, .T. ) ;
#14977=CARTESIAN_POINT ( 'NONE',  ( 118.7327907441706571, -34.64671908090114272, 48.96705384733895983 ) ) ;
#14978=VERTEX_POINT ( 'NONE', #17756 ) ;
#14979=CARTESIAN_POINT ( 'NONE',  ( 98.53948418117370522, -33.67937232826720617, 25.48765792331497693 ) ) ;
#14980=CARTESIAN_POINT ( 'NONE',  ( 71.06648329127399677, -8.729447159940999512, 284.9256252759119548 ) ) ;
#14981=CARTESIAN_POINT ( 'NONE',  ( 116.8150918559700813, -40.26546416881835455, 173.5375300378159693 ) ) ;
#14982=CARTESIAN_POINT ( 'NONE',  ( 41.56648329127499153, -36.32844715994070839, 258.9256252759120116 ) ) ;
#14983=CARTESIAN_POINT ( 'NONE',  ( 86.06670390244796920, -48.82844715994099971, 198.9178068554149945 ) ) ;
#14985=EDGE_CURVE ( 'NONE', #16276, #56405, #46326, .T. ) ;
#14987=CARTESIAN_POINT ( 'NONE',  ( 115.3579863298411254, -45.26537652146382840, 264.1899109901965517 ) ) ;
#14990=AXIS2_PLACEMENT_3D ( 'NONE', #72563, #78502, #16261 ) ;
#14992=ORIENTED_EDGE ( 'NONE', *, *, #24770, .F. ) ;
#14993=CARTESIAN_POINT ( 'NONE',  ( 99.65376319600918009, -46.03872712633670972, 118.0413395616259606 ) ) ;
#14994=DIRECTION ( 'NONE',  ( 1.000000000000000078E-15, 1.000000000000000083E-30, -1.000000000000000000 ) ) ;
#14996=ORIENTED_EDGE ( 'NONE', *, *, #16535, .T. ) ;
#14997=ORIENTED_EDGE ( 'NONE', *, *, #70535, .F. ) ;
#14998=CARTESIAN_POINT ( 'NONE',  ( 116.8171228694637733, -34.15291832781043979, 124.0314586086284692 ) ) ;
#14999=CARTESIAN_POINT ( 'NONE',  ( 113.2455016744213765, -28.75867540999941241, 265.5522916365027299 ) ) ;
#15000=DIRECTION ( 'NONE',  ( 3.340531404218880531E-13, -1.000000000000000000, 3.350531404218880242E-28 ) ) ;
#15001=CARTESIAN_POINT ( 'NONE',  ( 163.0959832912770082, -23.42844715993521021, 313.9678068554149490 ) ) ;
#15002=CARTESIAN_POINT ( 'NONE',  ( 41.56648329127398966, -18.82844715994071194, 138.9256252759119832 ) ) ;
#15003=CARTESIAN_POINT ( 'NONE',  ( 118.0831039394318083, -37.62836316206458065, 34.77372051400695341 ) ) ;
#15004=CARTESIAN_POINT ( 'NONE',  ( 131.0667039024480118, -43.72944715994093201, 231.5838068554170093 ) ) ;
#15005=ORIENTED_EDGE ( 'NONE', *, *, #88579, .T. ) ;
#15007=CARTESIAN_POINT ( 'NONE',  ( 101.9936095392775712, -45.44606507104835202, 42.15594039548825123 ) ) ;
#15008=ORIENTED_EDGE ( 'NONE', *, *, #56837, .F. ) ;
#15009=EDGE_LOOP ( 'NONE', ( #79896, #18947, #7004, #46323 ) ) ;
#15010=EDGE_CURVE ( 'NONE', #7509, #27470, #19090, .T. ) ;
#15011=CARTESIAN_POINT ( 'NONE',  ( 82.67340060512943012, -19.60624470235704564, 2.902100967938844533 ) ) ;
#15013=DIRECTION ( 'NONE',  ( 0.000000000000000000, 0.000000000000000000, 1.000000000000000000 ) ) ;
#15015=CYLINDRICAL_SURFACE ( 'NONE', #4253, 2.117000000000000881 ) ;
#15016=DIRECTION ( 'NONE',  ( 0.7071067811865671127, 0.7071067811865279218, 7.071067811865664660E-16 ) ) ;
#15017=CARTESIAN_POINT ( 'NONE',  ( 101.2834890806669677, -28.93024170975123255, 185.0067055423629938 ) ) ;
#15018=FACE_OUTER_BOUND ( 'NONE', #68595, .T. ) ;
#15020=CARTESIAN_POINT ( 'NONE',  ( 108.9933628702935238, -47.01991853554855538, 82.72419670448194040 ) ) ;
#15024=AXIS2_PLACEMENT_3D ( 'NONE', #22781, #85906, #23678 ) ;
#15025=CARTESIAN_POINT ( 'NONE',  ( 103.3136250034697099, -27.46033481550304600, 276.3826084592540724 ) ) ;
#15026=VERTEX_POINT ( 'NONE', #5019 ) ;
#15027=CARTESIAN_POINT ( 'NONE',  ( 105.7993347760366021, -26.72405582829313531, 50.17730648672989702 ) ) ;
#15028=ORIENTED_EDGE ( 'NONE', *, *, #41444, .T. ) ;
#15029=LINE ( 'NONE', #22754, #42134 ) ;
#15030=DIRECTION ( 'NONE',  ( 1.000000000000000000, 0.000000000000000000, 0.000000000000000000 ) ) ;
#15032=AXIS2_PLACEMENT_3D ( 'NONE', #88503, #26256, #53934 ) ;
#15035=CARTESIAN_POINT ( 'NONE',  ( 96.93519779220999055, -32.25144590123284161, 55.98324432352897162 ) ) ;
#15036=( LENGTH_UNIT ( ) NAMED_UNIT ( * ) SI_UNIT ( .MILLI., .METRE. ) );
#15037=CARTESIAN_POINT ( 'NONE',  ( 109.7241730775608062, -27.00061873284944269, 164.8648492007025652 ) ) ;
#15038=CARTESIAN_POINT ( 'NONE',  ( 131.0667039024480118, -58.35344715994099829, 234.8338068554150198 ) ) ;
#15039=CARTESIAN_POINT ( 'NONE',  ( 179.1667039024475230, -28.27351298636771659, 237.4678068554150059 ) ) ;
#15040=CARTESIAN_POINT ( 'NONE',  ( 98.30753417366616986, -41.72887546178495910, 141.7397919399187458 ) ) ;
#15041=ORIENTED_EDGE ( 'NONE', *, *, #66403, .F. ) ;
#15043=EDGE_CURVE ( 'NONE', #35953, #47474, #74520, .T. ) ;
#15044=CARTESIAN_POINT ( 'NONE',  ( 110.0236307522814911, -27.14727356840723971, 120.8367254748248598 ) ) ;
#15046=EDGE_CURVE ( 'NONE', #39094, #29668, #50752, .T. ) ;
#15048=CARTESIAN_POINT ( 'NONE',  ( 117.6299819888065912, -33.39812594883869679, 125.0575300378149706 ) ) ;
#15049=EDGE_CURVE ( 'NONE', #83484, #5931, #20842, .T. ) ;
#15051=FACE_OUTER_BOUND ( 'NONE', #71151, .T. ) ;
#15052=DIRECTION ( 'NONE',  ( -1.907762142705490052E-15, -7.167082501179359715E-16, 1.000000000000000000 ) ) ;
#15053=AXIS2_PLACEMENT_3D ( 'NONE', #4854, #61590, #54309 ) ;
#15054=ORIENTED_EDGE ( 'NONE', *, *, #61694, .F. ) ;
#15055=AXIS2_PLACEMENT_3D ( 'NONE', #70884, #9099, #8654 ) ;
#15057=CARTESIAN_POINT ( 'NONE',  ( 116.9310496459149391, -33.53114825773884178, 130.0880062282909648 ) ) ;
#15059=LINE ( 'NONE', #62294, #76161 ) ;
#15060=ORIENTED_EDGE ( 'NONE', *, *, #62433, .F. ) ;
#15061=CARTESIAN_POINT ( 'NONE',  ( 97.63514171170974976, -41.12017164899855715, 252.6727681330536655 ) ) ;
#15063=CARTESIAN_POINT ( 'NONE',  ( 172.5664832912740110, -36.32844715994070839, 83.67562527591201160 ) ) ;
#15068=CARTESIAN_POINT ( 'NONE',  ( 117.2759483237920080, -34.91131378075001379, 198.9546728949589749 ) ) ;
#15069=ORIENTED_EDGE ( 'NONE', *, *, #77282, .T. ) ;
#15071=CARTESIAN_POINT ( 'NONE',  ( 99.43677639672335999, -41.29559517668970869, 158.1872975916109567 ) ) ;
#15072=CIRCLE ( 'NONE', #22121, 0.5000000000000004441 ) ;
#15073=CARTESIAN_POINT ( 'NONE',  ( 163.0667039024470171, -33.35206098992711077, 342.9256252759119548 ) ) ;
#15074=CARTESIAN_POINT ( 'NONE',  ( 111.4279401658702682, -28.40658880358809668, 11.11205949637394852 ) ) ;
#15076=CARTESIAN_POINT ( 'NONE',  ( 162.5667039024470171, -32.29483332968611364, 117.4678068554150485 ) ) ;
#15077=CARTESIAN_POINT ( 'NONE',  ( 167.6524903400753885, -49.32844715993521589, 249.9678068554149775 ) ) ;
#15078=DIRECTION ( 'NONE',  ( 0.000000000000000000, 0.000000000000000000, -1.000000000000000000 ) ) ;
#15079=AXIS2_PLACEMENT_3D ( 'NONE', #26670, #13058, #88471 ) ;
#15080=DIRECTION ( 'NONE',  ( -0.9254794337955623007, -0.3787978585227819162, 0.000000000000000000 ) ) ;
#15082=CARTESIAN_POINT ( 'NONE',  ( 96.14807755961376756, -35.16348456217429685, 226.2251490854349640 ) ) ;
#15086=CARTESIAN_POINT ( 'NONE',  ( 112.0659116112372402, -45.48839626716342366, 87.98979194155364780 ) ) ;
#15088=LINE ( 'NONE', #69154, #40306 ) ;
#15090=EDGE_CURVE ( 'NONE', #17736, #33658, #62662, .T. ) ;
#15091=CARTESIAN_POINT ( 'NONE',  ( 110.3395589168170545, -45.98151452051992294, 33.84705384733993583 ) ) ;
#15092=DIRECTION ( 'NONE',  ( 0.000000000000000000, 0.000000000000000000, 1.000000000000000000 ) ) ;
#15093=VERTEX_POINT ( 'NONE', #27697 ) ;
#15094=CARTESIAN_POINT ( 'NONE',  ( 106.2487395568334421, -26.25713557174866253, 21.13848241876792144 ) ) ;
#15097=CARTESIAN_POINT ( 'NONE',  ( 115.2518872279481030, -30.21599423016839836, 244.3613395616249875 ) ) ;
#15098=ORIENTED_EDGE ( 'NONE', *, *, #1498, .T. ) ;
#15099=DIRECTION ( 'NONE',  ( 0.000000000000000000, -1.000000000000000000, 0.000000000000000000 ) ) ;
#15100=LINE ( 'NONE', #82814, #19600 ) ;
#15101=CARTESIAN_POINT ( 'NONE',  ( 108.3327516424870964, -46.73493878462306128, 167.6772798019345032 ) ) ;
#15102=CARTESIAN_POINT ( 'NONE',  ( 98.91570299145236334, -37.17047609451836365, 74.18809036959095238 ) ) ;
#15103=CARTESIAN_POINT ( 'NONE',  ( 116.3968524479345348, -41.42853965253563331, 199.4556252759109611 ) ) ;
#15105=ORIENTED_EDGE ( 'NONE', *, *, #47383, .T. ) ;
#15107=ORIENTED_EDGE ( 'NONE', *, *, #64811, .T. ) ;
#15108=ORIENTED_EDGE ( 'NONE', *, *, #53290, .T. ) ;
#15109=VECTOR ( 'NONE', #68316, 1000.000000000000000 ) ;
#15111=DIRECTION ( 'NONE',  ( 0.000000000000000000, 0.000000000000000000, 1.000000000000000000 ) ) ;
#15112=VERTEX_POINT ( 'NONE', #48116 ) ;
#15113=ORIENTED_EDGE ( 'NONE', *, *, #46264, .F. ) ;
#15114=FACE_OUTER_BOUND ( 'NONE', #75080, .T. ) ;
#15115=VECTOR ( 'NONE', #73196, 1000.000000000000000 ) ;
#15116=B_SPLINE_CURVE_WITH_KNOTS ( 'NONE', 3,
 ( #27754, #55436, #84540, #83187, #48615, #77709, #8674, #7321, #56338, #28648, #35453, #84085, #36373, #21856, #22298, #29553, #22755, #76355 ),
 .UNSPECIFIED., .F., .F.,
 ( 4, 2, 2, 2, 2, 2, 2, 2, 4 ),
 ( 0.000000000000000000, 0.06250903880341492080, 0.1250180776068298416, 0.1875271164102447763, 0.2500361552136596832, 0.3125451940170745901, 0.3750542328204895526, 0.4375632716239044595, 0.5000723104273193664 ),
 .UNSPECIFIED. ) ;
#15117=CARTESIAN_POINT ( 'NONE',  ( 97.80977108376971785, -40.51273747973604600, 42.63522248069732967 ) ) ;
#15118=CARTESIAN_POINT ( 'NONE',  ( 116.7149163912777396, -35.64392129247566032, 83.33813411379098568 ) ) ;
#15119=CARTESIAN_POINT ( 'NONE',  ( 96.54134661961150243, -40.18473915001016650, 286.5908633711491120 ) ) ;
#15120=DIRECTION ( 'NONE',  ( -1.000000000000000000, -4.554376769437570034E-14, 0.000000000000000000 ) ) ;
#15122=ORIENTED_EDGE ( 'NONE', *, *, #83763, .T. ) ;
#15124=VERTEX_POINT ( 'NONE', #55375 ) ;
#15126=DIRECTION ( 'NONE',  ( -4.237773401492740281E-14, 1.000000000000000000, 0.000000000000000000 ) ) ;
#15128=CARTESIAN_POINT ( 'NONE',  ( 114.2351621074132879, -44.22269940884951467, 113.1718157521019776 ) ) ;
#15129=CARTESIAN_POINT ( 'NONE',  ( 98.05881815954255387, -31.39384645160161469, 85.90133956162493689 ) ) ;
#15132=ORIENTED_EDGE ( 'NONE', *, *, #20117, .F. ) ;
#15134=CARTESIAN_POINT ( 'NONE',  ( 113.1001805014122255, -45.99085015462044623, 223.0480062282919675 ) ) ;
#15136=AXIS2_PLACEMENT_3D ( 'NONE', #10238, #31114, #3425 ) ;
#15139=DIRECTION ( 'NONE',  ( 1.000000000000000078E-15, -1.000000000000000083E-30, -1.000000000000000000 ) ) ;
#15141=PLANE ( 'NONE',  #12281 ) ;
#15142=DIRECTION ( 'NONE',  ( 1.000000000000000000, 0.000000000000000000, 0.000000000000000000 ) ) ;
#15143=DIRECTION ( 'NONE',  ( 0.000000000000000000, 0.000000000000000000, 1.000000000000000000 ) ) ;
#15145=AXIS2_PLACEMENT_3D ( 'NONE', #22974, #14361, #42039 ) ;
#15146=CARTESIAN_POINT ( 'NONE',  ( 182.3467384525650061, -36.02818131005800950, -5.074374724088000832 ) ) ;
#15148=ADVANCED_FACE ( 'NONE', ( #34048 ), #89486, .F. ) ;
#15150=DIRECTION ( 'NONE',  ( 0.000000000000000000, 0.000000000000000000, -1.000000000000000000 ) ) ;
#15151=ORIENTED_EDGE ( 'NONE', *, *, #67570, .F. ) ;
#15153=CARTESIAN_POINT ( 'NONE',  ( 96.49566810458604493, -31.31724962161759507, 245.9499109901969689 ) ) ;
#15154=CARTESIAN_POINT ( 'NONE',  ( 116.9041476981693677, -40.17949737190902937, 129.5584824187679658 ) ) ;
#15155=CARTESIAN_POINT ( 'NONE',  ( 118.3880299729056276, -33.06406546148816261, 280.0756252759109657 ) ) ;
#15156=FACE_OUTER_BOUND ( 'NONE', #54490, .T. ) ;
#15158=CARTESIAN_POINT ( 'NONE',  ( 82.77273044669095725, -36.23917853419808210, 6.814128304791553070 ) ) ;
#15159=CARTESIAN_POINT ( 'NONE',  ( 177.8371591254543205, -47.82818131005477369, 300.4678068554149490 ) ) ;
#15160=ORIENTED_EDGE ( 'NONE', *, *, #41027, .T. ) ;
#15163=CARTESIAN_POINT ( 'NONE',  ( 115.5545030166667146, -32.01519760825960503, 178.6524198280769724 ) ) ;
#15165=DIRECTION ( 'NONE',  ( 4.299999999999999979E-14, -1.000000000000000000, 4.400000000000000367E-29 ) ) ;
#15166=EDGE_LOOP ( 'NONE', ( #52501, #60148, #42608, #5339 ) ) ;
#15168=CARTESIAN_POINT ( 'NONE',  ( 117.4047238282098249, -30.98758422922437106, 175.2299109901969700 ) ) ;
#15169=CARTESIAN_POINT ( 'NONE',  ( 109.6407380183136837, -46.48065911288304619, 148.7819440279659489 ) ) ;
#15170=EDGE_CURVE ( 'NONE', #58498, #77150, #13638, .T. ) ;
#15172=CARTESIAN_POINT ( 'NONE',  ( 97.31540730480230650, -39.30489313201859858, 87.53094125324652452 ) ) ;
#15173=CYLINDRICAL_SURFACE ( 'NONE', #53377, 3.299999999999997158 ) ;
#15174=CYLINDRICAL_SURFACE ( 'NONE', #17868, 0.5000000000000172085 ) ;
#15175=CARTESIAN_POINT ( 'NONE',  ( 97.28626111821314737, -36.62605694204433604, 111.3184824187689657 ) ) ;
#15179=AXIS2_PLACEMENT_3D ( 'NONE', #66297, #4536, #32224 ) ;
#15180=CARTESIAN_POINT ( 'NONE',  ( 98.47292639957201743, -32.93111785796080682, 52.41491663922997901 ) ) ;
#15181=CARTESIAN_POINT ( 'NONE',  ( 125.0664851986225159, -56.72944715994101728, 14.92562527591098842 ) ) ;
#15182=CARTESIAN_POINT ( 'NONE',  ( 98.91665286848252947, -30.31703347128394910, 196.8080062282909637 ) ) ;
#15183=CARTESIAN_POINT ( 'NONE',  ( 99.04406193110015977, -42.84125773391240699, 36.84395861861840871 ) ) ;
#15184=CIRCLE ( 'NONE', #25279, 2.116999999999980009 ) ;
#15185=FACE_OUTER_BOUND ( 'NONE', #63484, .T. ) ;
#15186=CARTESIAN_POINT ( 'NONE',  ( 163.0664832912739826, 19.62155284005901024, 330.1506252759110680 ) ) ;
#15187=DIRECTION ( 'NONE',  ( 0.000000000000000000, 0.000000000000000000, -1.000000000000000000 ) ) ;
#15190=CARTESIAN_POINT ( 'NONE',  ( 101.5125196766230289, -27.93273449574867229, 110.5241967044819944 ) ) ;
#15193=ORIENTED_EDGE ( 'NONE', *, *, #72427, .F. ) ;
#15196=CARTESIAN_POINT ( 'NONE',  ( 97.31313350590980349, -38.96086997259878615, 131.5054597300594423 ) ) ;
#15197=DIRECTION ( 'NONE',  ( -1.000000000000000000, -4.299999999999999979E-14, -1.000000000000000078E-15 ) ) ;
#15198=CARTESIAN_POINT ( 'NONE',  ( 99.23015118009998048, -40.40270512654389279, 209.4814237029249568 ) ) ;
#15199=VECTOR ( 'NONE', #67704, 1000.000000000000000 ) ;
#15200=VECTOR ( 'NONE', #38607, 1000.000000000000000 ) ;
#15201=DIRECTION ( 'NONE',  ( -1.000000000000000078E-15, 1.000000000000000083E-30, 1.000000000000000000 ) ) ;
#15202=AXIS2_PLACEMENT_3D ( 'NONE', #59832, #87563, #52990 ) ;
#15203=VECTOR ( 'NONE', #42476, 1000.000000000000000 ) ;
#15204=EDGE_CURVE ( 'NONE', #2549, #18180, #84021, .T. ) ;
#15206=VERTEX_POINT ( 'NONE', #49465 ) ;
#15210=VECTOR ( 'NONE', #45416, 1000.000000000000000 ) ;
#15214=LINE ( 'NONE', #20682, #43436 ) ;
#15216=CARTESIAN_POINT ( 'NONE',  ( 114.5371455856629694, -43.48665885088448135, 229.6730118773259619 ) ) ;
#15219=FACE_OUTER_BOUND ( 'NONE', #88697, .T. ) ;
#15220=FACE_OUTER_BOUND ( 'NONE', #83704, .T. ) ;
#15222=VERTEX_POINT ( 'NONE', #68143 ) ;
#15223=EDGE_CURVE ( 'NONE', #82107, #62559, #55617, .T. ) ;
#15225=ORIENTED_EDGE ( 'NONE', *, *, #24887, .T. ) ;
#15226=EDGE_LOOP ( 'NONE', ( #86021, #2447, #48391, #73749, #61310, #59737 ) ) ;
#15227=VECTOR ( 'NONE', #51524, 1000.000000000000114 ) ;
#15228=EDGE_CURVE ( 'NONE', #37616, #85174, #89034, .T. ) ;
#15229=CARTESIAN_POINT ( 'NONE',  ( 98.82205551832399237, -39.36200594543229414, 279.3785665600675543 ) ) ;
#15230=ADVANCED_FACE ( 'NONE', ( #51251, #79447 ), #16315, .F. ) ;
#15231=CARTESIAN_POINT ( 'NONE',  ( 96.59657429157336139, -36.21044007025302136, 171.2870538473399620 ) ) ;
#15232=CARTESIAN_POINT ( 'NONE',  ( 103.2867953297129588, -47.09177226061144239, 97.28610146638693834 ) ) ;
#15233=DIRECTION ( 'NONE',  ( 1.000000000000000000, 3.999999999999999995E-14, 1.000000000000000078E-15 ) ) ;
#15234=CARTESIAN_POINT ( 'NONE',  ( 176.5667039024485518, -48.82844715993482509, 180.4678068554150059 ) ) ;
#15235=CARTESIAN_POINT ( 'NONE',  ( 97.16978355702093495, -40.00630874038032658, 237.5813395616249579 ) ) ;
#15237=CARTESIAN_POINT ( 'NONE',  ( 41.56670390244689628, -36.32844715994109208, 180.4678068554150911 ) ) ;
#15238=ORIENTED_EDGE ( 'NONE', *, *, #11663, .T. ) ;
#15239=CARTESIAN_POINT ( 'NONE',  ( 34.67381068362099228, -26.00627455219321860, 313.9678068554150059 ) ) ;
#15240=EDGE_CURVE ( 'NONE', #64922, #14514, #58520, .T. ) ;
#15241=ORIENTED_EDGE ( 'NONE', *, *, #87729, .T. ) ;
#15242=ADVANCED_FACE ( 'NONE', ( #29949 ), #42644, .F. ) ;
#15243=ORIENTED_EDGE ( 'NONE', *, *, #23777, .T. ) ;
#15245=ADVANCED_FACE ( 'NONE', ( #1347 ), #64020, .F. ) ;
#15248=CARTESIAN_POINT ( 'NONE',  ( 95.77883191840808763, -40.33907488607122360, 131.5727681330539554 ) ) ;
#15249=DIRECTION ( 'NONE',  ( 1.000000000000000078E-15, -1.000000000000000083E-30, -1.000000000000000000 ) ) ;
#15250=VECTOR ( 'NONE', #84760, 1000.000000000000000 ) ;
#15253=PLANE ( 'NONE',  #42728 ) ;
#15254=CARTESIAN_POINT ( 'NONE',  ( 94.06648329127393993, -36.72944715994093912, 315.6356252759111953 ) ) ;
#15255=FACE_OUTER_BOUND ( 'NONE', #22397, .T. ) ;
#15256=CARTESIAN_POINT ( 'NONE',  ( 118.0585799961420577, -32.36802338489823683, 245.1270538473389706 ) ) ;
#15258=DIRECTION ( 'NONE',  ( 0.000000000000000000, 0.000000000000000000, -1.000000000000000000 ) ) ;
#15260=DIRECTION ( 'NONE',  ( 1.000000000000000078E-15, 0.000000000000000000, -1.000000000000000000 ) ) ;
#15261=CARTESIAN_POINT ( 'NONE',  ( 100.9546727936483848, -28.70702574047548339, 256.5939586109827246 ) ) ;
#15262=EDGE_CURVE ( 'NONE', #9337, #44647, #2044, .T. ) ;
#15263=CARTESIAN_POINT ( 'NONE',  ( 167.6524903400753033, -48.32844715993521589, 300.4678068554149490 ) ) ;
#15264=CARTESIAN_POINT ( 'NONE',  ( 96.49234500119369784, -40.10591448887350197, 281.5603871806727625 ) ) ;
#15265=EDGE_LOOP ( 'NONE', ( #5874, #41309, #88595, #82572 ) ) ;
#15266=CARTESIAN_POINT ( 'NONE',  ( 86.06670390244796920, -48.82844715994099971, 250.9178068554150514 ) ) ;
#15267=CARTESIAN_POINT ( 'NONE',  ( 108.7467888895124162, -25.78085441620226348, 144.9432443235299672 ) ) ;
#15268=CARTESIAN_POINT ( 'NONE',  ( 118.0755232325510917, -37.71687819837586630, 29.74324432352998215 ) ) ;
#15269=CARTESIAN_POINT ( 'NONE',  ( 110.1502920506493552, -26.06700738780482141, 210.8403871806729626 ) ) ;
#15271=DIRECTION ( 'NONE',  ( -2.106816776397999944E-14, 1.000000000000000000, -2.206816776398000223E-29 ) ) ;
#15272=FACE_OUTER_BOUND ( 'NONE', #40276, .T. ) ;
#15274=CARTESIAN_POINT ( 'NONE',  ( 99.09570908588736415, -30.55043174076017820, 70.80229194132837733 ) ) ;
#15275=CARTESIAN_POINT ( 'NONE',  ( 116.3212776292296127, -32.94146857471318413, 287.6356252759109680 ) ) ;
#15277=CARTESIAN_POINT ( 'NONE',  ( 140.9629299006807059, -46.47944715994099596, -5.074374724088994704 ) ) ;
#15278=AXIS2_PLACEMENT_3D ( 'NONE', #76390, #528, #41403 ) ;
#15279=AXIS2_PLACEMENT_3D ( 'NONE', #79976, #17730, #64985 ) ;
#15280=VECTOR ( 'NONE', #45203, 1000.000000000000000 ) ;
#15282=ORIENTED_EDGE ( 'NONE', *, *, #66383, .T. ) ;
#15283=VECTOR ( 'NONE', #19839, 1000.000000000000000 ) ;
#15285=CYLINDRICAL_SURFACE ( 'NONE', #9640, 4.750000000000004441 ) ;
#15287=CARTESIAN_POINT ( 'NONE',  ( 96.94236579736397630, -32.35154040576534840, 57.01372051400599616 ) ) ;
#15288=LINE ( 'NONE', #63423, #19413 ) ;
#15289=ADVANCED_FACE ( 'NONE', ( #22693 ), #44440, .F. ) ;
#15290=ADVANCED_FACE ( 'NONE', ( #9948 ), #57633, .T. ) ;
#15293=CARTESIAN_POINT ( 'NONE',  ( 109.4552518484143206, -25.89010755186295754, 175.8918157521009391 ) ) ;
#15294=EDGE_CURVE ( 'NONE', #78195, #41311, #56737, .T. ) ;
#15295=AXIS2_PLACEMENT_3D ( 'NONE', #56368, #84109, #21881 ) ;
#15296=CARTESIAN_POINT ( 'NONE',  ( 110.8947914379136961, -29.09399076817903662, 279.1295626852197529 ) ) ;
#15297=ORIENTED_EDGE ( 'NONE', *, *, #72673, .T. ) ;
#15299=VERTEX_POINT ( 'NONE', #8157 ) ;
#15303=CARTESIAN_POINT ( 'NONE',  ( 102.0667490476481589, -27.97067744669410061, 161.4898198796698239 ) ) ;
#15304=CARTESIAN_POINT ( 'NONE',  ( 97.33784130791669043, -34.07106454120959427, 76.11479194351055355 ) ) ;
#15305=CONICAL_SURFACE ( 'NONE', #77670, 1.258750000000002922, 1.029744258676650093 ) ;
#15310=CARTESIAN_POINT ( 'NONE',  ( 109.6066175024219973, -25.17973177368032012, 29.90419670448196854 ) ) ;
#15312=ORIENTED_EDGE ( 'NONE', *, *, #44683, .T. ) ;
#15314=FACE_OUTER_BOUND ( 'NONE', #1490, .T. ) ;
#15315=CARTESIAN_POINT ( 'NONE',  ( 115.0083044075158654, -38.73198694842640322, 121.4480903695919807 ) ) ;
#15316=VECTOR ( 'NONE', #46812, 1000.000000000000000 ) ;
#15317=AXIS2_PLACEMENT_3D ( 'NONE', #38427, #44346, #912 ) ;
#15320=ORIENTED_EDGE ( 'NONE', *, *, #29409, .T. ) ;
#15321=VERTEX_POINT ( 'NONE', #70841 ) ;
#15325=CARTESIAN_POINT ( 'NONE',  ( 100.5685618138929271, -29.03188392736010570, 147.0672975916109806 ) ) ;
#15327=CARTESIAN_POINT ( 'NONE',  ( 103.3547197592076969, -47.16534756318074528, 98.31657765686297523 ) ) ;
#15328=DIRECTION ( 'NONE',  ( 0.000000000000000000, 0.000000000000000000, 1.000000000000000000 ) ) ;
#15329=AXIS2_PLACEMENT_3D ( 'NONE', #11824, #11371, #75397 ) ;
#15331=AXIS2_PLACEMENT_3D ( 'NONE', #62856, #14279, #84674 ) ;
#15334=ORIENTED_EDGE ( 'NONE', *, *, #80783, .F. ) ;
#15335=EDGE_LOOP ( 'NONE', ( #62864, #30950, #9122, #50751 ) ) ;
#15338=EDGE_CURVE ( 'NONE', #9815, #81510, #64419, .T. ) ;
#15339=CARTESIAN_POINT ( 'NONE',  ( 96.17000221327154463, -38.71995997157278424, 51.48229194257797303 ) ) ;
#15340=ORIENTED_EDGE ( 'NONE', *, *, #26915, .F. ) ;
#15341=CARTESIAN_POINT ( 'NONE',  ( 109.0793648114890715, -47.66380995969711876, 277.7213395616258822 ) ) ;
#15342=CARTESIAN_POINT ( 'NONE',  ( 116.8155376854491720, -40.58108761943747567, 189.5270538473389479 ) ) ;
#15343=CARTESIAN_POINT ( 'NONE',  ( 128.0667039024480118, -58.35344715994099829, 10.91780685541479734 ) ) ;
#15345=CARTESIAN_POINT ( 'NONE',  ( 97.74639642956380214, -42.67166664343270099, 137.7661014663869992 ) ) ;
#15346=DIRECTION ( 'NONE',  ( -0.0001713722456127401463, 0.9999999853157766072, 1.713722456137401502E-19 ) ) ;
#15349=ADVANCED_FACE ( 'NONE', ( #37652 ), #35353, .F. ) ;
#15350=EDGE_CURVE ( 'NONE', #52647, #77884, #35847, .T. ) ;
#15351=ORIENTED_EDGE ( 'NONE', *, *, #1230, .T. ) ;
#15352=CARTESIAN_POINT ( 'NONE',  ( 98.38043711079399145, -41.69530130865705786, 132.7403033756623074 ) ) ;
#15353=ORIENTED_EDGE ( 'NONE', *, *, #44445, .F. ) ;
#15354=VECTOR ( 'NONE', #57157, 1000.000000000000000 ) ;
#15355=ORIENTED_EDGE ( 'NONE', *, *, #11783, .F. ) ;
#15356=EDGE_CURVE ( 'NONE', #66809, #43116, #46934, .T. ) ;
#15357=DIRECTION ( 'NONE',  ( 0.000000000000000000, 1.000000000000000000, 0.000000000000000000 ) ) ;
#15358=CARTESIAN_POINT ( 'NONE',  ( 46.83715912545422100, -47.82818131006082751, 313.9678068554150059 ) ) ;
#15359=CARTESIAN_POINT ( 'NONE',  ( 117.4878618838608872, -37.01562663403593234, 43.80419670448293346 ) ) ;
#15361=AXIS2_PLACEMENT_3D ( 'NONE', #6001, #32787, #19608 ) ;
#15363=PLANE ( 'NONE',  #53559 ) ;
#15365=CARTESIAN_POINT ( 'NONE',  ( 116.8435662018514307, -36.99793375417353758, 43.80419670448193159 ) ) ;
#15366=PLANE ( 'NONE',  #44870 ) ;
#15367=CARTESIAN_POINT ( 'NONE',  ( 117.0123300003820646, -30.33189756676014426, 140.2813395616249750 ) ) ;
#15368=CARTESIAN_POINT ( 'NONE',  ( 97.06107109872726824, -37.99641197594983311, 72.42729194355847255 ) ) ;
#15369=CARTESIAN_POINT ( 'NONE',  ( 33.92127028473484529, -29.73316016639607184, 193.9678068554150911 ) ) ;
#15370=ORIENTED_EDGE ( 'NONE', *, *, #41530, .T. ) ;
#15375=EDGE_CURVE ( 'NONE', #87925, #64058, #32158, .T. ) ;
#15376=DIRECTION ( 'NONE',  ( 4.299999999999999979E-14, -1.000000000000000000, 4.400000000000000367E-29 ) ) ;
#15377=CARTESIAN_POINT ( 'NONE',  ( 103.0327258024342427, -26.38818591439425632, 170.3603871806729444 ) ) ;
#15379=DIRECTION ( 'NONE',  ( 1.000000000000000078E-15, 1.000000000000000083E-30, -1.000000000000000000 ) ) ;
#15380=CARTESIAN_POINT ( 'NONE',  ( 117.4960079497888472, -36.12755493457860467, 224.8727681330539667 ) ) ;
#15381=CARTESIAN_POINT ( 'NONE',  ( 107.6053842629478794, -26.23908965751013156, 91.03562527591097364 ) ) ;
#15382=CARTESIAN_POINT ( 'NONE',  ( 51.42025729302798709, -31.94127993907680718, -5.074374724088000832 ) ) ;
#15383=CARTESIAN_POINT ( 'NONE',  ( 115.0868436454567387, -30.61496486536007211, 190.3439483173824556 ) ) ;
#15384=EDGE_CURVE ( 'NONE', #733, #34697, #38090, .T. ) ;
#15387=AXIS2_PLACEMENT_3D ( 'NONE', #81045, #51943, #60103 ) ;
#15389=ORIENTED_EDGE ( 'NONE', *, *, #53251, .F. ) ;
#15390=EDGE_LOOP ( 'NONE', ( #59169, #61700, #18042, #8296, #4412 ) ) ;
#15391=DIRECTION ( 'NONE',  ( 1.000000000000000000, 4.299999999999999979E-14, 1.000000000000000078E-15 ) ) ;
#15392=CARTESIAN_POINT ( 'NONE',  ( 104.8412801004068058, -26.50840007386317509, 256.2470538473397141 ) ) ;
#15393=LINE ( 'NONE', #41719, #1123 ) ;
#15394=CARTESIAN_POINT ( 'NONE',  ( 136.6003823147689786, -17.66080131299353795, 2.811527311783424743 ) ) ;
#15395=ADVANCED_FACE ( 'NONE', ( #31715 ), #73497, .T. ) ;
#15396=CARTESIAN_POINT ( 'NONE',  ( 182.0374245136142406, -23.42844715993458848, 193.9678068554150059 ) ) ;
#15397=DIRECTION ( 'NONE',  ( 0.7071067811578790607, 0.7071067812152160847, 0.000000000000000000 ) ) ;
#15399=CIRCLE ( 'NONE', #77767, 3.000000000000002665 ) ;
#15401=CARTESIAN_POINT ( 'NONE',  ( 112.9757402841042904, -28.11393523324086985, 44.59848241876795782 ) ) ;
#15402=ORIENTED_EDGE ( 'NONE', *, *, #21318, .T. ) ;
#15403=CIRCLE ( 'NONE', #859, 0.5000000000000004441 ) ;
#15405=VECTOR ( 'NONE', #3662, 1000.000000000000000 ) ;
#15408=CIRCLE ( 'NONE', #51609, 3.250000000000002665 ) ;
#15409=LINE ( 'NONE', #1774, #59318 ) ;
#15410=CARTESIAN_POINT ( 'NONE',  ( 97.21282778982880757, -39.96427141005798234, 282.5908633711484867 ) ) ;
#15412=CARTESIAN_POINT ( 'NONE',  ( 113.4935171807053536, -28.59114140144097860, 120.5565776568629559 ) ) ;
#15414=CARTESIAN_POINT ( 'NONE',  ( 108.3327080255635622, -46.73494336040992181, 27.67723307863499826 ) ) ;
#15415=ORIENTED_EDGE ( 'NONE', *, *, #6131, .F. ) ;
#15416=DIRECTION ( 'NONE',  ( 0.7071067811865259234, -0.7071067811865692221, 2.899137802865049595E-29 ) ) ;
#15417=CARTESIAN_POINT ( 'NONE',  ( 78.35491772849390202, -34.56918551488853097, 2.099346190924665567 ) ) ;
#15418=ORIENTED_EDGE ( 'NONE', *, *, #17702, .F. ) ;
#15419=ORIENTED_EDGE ( 'NONE', *, *, #60662, .T. ) ;
#15420=AXIS2_PLACEMENT_3D ( 'NONE', #3835, #4734, #81508 ) ;
#15421=CARTESIAN_POINT ( 'NONE',  ( 97.95250717983367394, -32.49412669507731266, 9.425625275910961776 ) ) ;
#15422=CARTESIAN_POINT ( 'NONE',  ( 98.67113652751868358, -38.83122756767168227, 14.35189989340096517 ) ) ;
#15423=EDGE_CURVE ( 'NONE', #78070, #46083, #83224, .T. ) ;
#15425=CARTESIAN_POINT ( 'NONE',  ( 177.0664832912730162, 12.92155284005730387, 358.9756252759109998 ) ) ;
#15426=CARTESIAN_POINT ( 'NONE',  ( 135.3838309168194201, -60.54606547621062163, 361.9756252759100335 ) ) ;
#15429=FACE_OUTER_BOUND ( 'NONE', #75796, .T. ) ;
#15430=CARTESIAN_POINT ( 'NONE',  ( 21.03715912545744615, -47.82818131006197149, 129.9678068554150627 ) ) ;
#15432=CARTESIAN_POINT ( 'NONE',  ( 113.5062182464826748, -28.53085922249196216, 79.54705384733995288 ) ) ;
#15434=CARTESIAN_POINT ( 'NONE',  ( 110.7520593201813597, -44.56232478875543990, 285.7328522743533767 ) ) ;
#15436=CARTESIAN_POINT ( 'NONE',  ( 98.02110346605346081, -41.80092515478916937, 181.7451490854359974 ) ) ;
#15438=DIRECTION ( 'NONE',  ( 0.000000000000000000, 1.000000000000000000, 1.598363122120870523E-15 ) ) ;
#15439=CYLINDRICAL_SURFACE ( 'NONE', #62250, 9.999999999999998224 ) ;
#15442=CARTESIAN_POINT ( 'NONE',  ( 118.1536727146126395, -36.20817079386891635, 264.8518157521014587 ) ) ;
#15446=VERTEX_POINT ( 'NONE', #48012 ) ;
#15447=CARTESIAN_POINT ( 'NONE',  ( 96.56348986465089013, -36.88801538493378018, 132.3384824187679669 ) ) ;
#15449=ORIENTED_EDGE ( 'NONE', *, *, #29747, .F. ) ;
#15451=EDGE_CURVE ( 'NONE', #26947, #58383, #19411, .T. ) ;
#15452=EDGE_CURVE ( 'NONE', #58845, #37060, #36619, .T. ) ;
#15454=CARTESIAN_POINT ( 'NONE',  ( 142.8698897858160421, -0.9167816978817300289, 361.9756252759100335 ) ) ;
#15455=ADVANCED_FACE ( 'NONE', ( #28032 ), #83028, .F. ) ;
#15459=DIRECTION ( 'NONE',  ( 1.067522139062650671E-15, 1.000000000000000000, 0.000000000000000000 ) ) ;
#15460=CARTESIAN_POINT ( 'NONE',  ( 107.1953983157108041, -26.30515493630308654, 31.06705384733893283 ) ) ;
#15461=DIRECTION ( 'NONE',  ( -4.237773401492740281E-14, 1.000000000000000000, 0.000000000000000000 ) ) ;
#15466=PLANE ( 'NONE',  #53367 ) ;
#15467=EDGE_LOOP ( 'NONE', ( #60413, #81927, #77958, #1377 ) ) ;
#15468=VERTEX_POINT ( 'NONE', #75301 ) ;
#15469=ADVANCED_FACE ( 'NONE', ( #47117 ), #82137, .F. ) ;
#15471=CARTESIAN_POINT ( 'NONE',  ( 82.16371341590115662, -20.51083119283027045, 2.376725019074904743 ) ) ;
#15473=CARTESIAN_POINT ( 'NONE',  ( 172.5664832912740110, -18.82844715994099971, 321.0426252759119734 ) ) ;
#15475=FACE_OUTER_BOUND ( 'NONE', #44425, .T. ) ;
#15476=LINE ( 'NONE', #30434, #73656 ) ;
#15477=EDGE_CURVE ( 'NONE', #69462, #48907, #15072, .T. ) ;
#15478=CARTESIAN_POINT ( 'NONE',  ( 112.5827476457113079, -28.73936235024410024, 239.0181341137909783 ) ) ;
#15479=CARTESIAN_POINT ( 'NONE',  ( 151.0371591254582881, -46.82818131005593187, 237.4678068554150059 ) ) ;
#15481=CARTESIAN_POINT ( 'NONE',  ( 98.82309110046458045, -43.24084327085208912, 91.85848241876892928 ) ) ;
#15483=LINE ( 'NONE', #7754, #84339 ) ;
#15484=EDGE_LOOP ( 'NONE', ( #88387, #11627, #49828, #77762 ) ) ;
#15485=CARTESIAN_POINT ( 'NONE',  ( 176.7738106835696499, -48.62134037881071436, 129.9678068554150059 ) ) ;
#15486=CARTESIAN_POINT ( 'NONE',  ( 99.09397582248948311, -30.55267087576145357, 276.8024460130702664 ) ) ;
#15487=VERTEX_POINT ( 'NONE', #74852 ) ;
#15489=ORIENTED_EDGE ( 'NONE', *, *, #19957, .T. ) ;
#15490=DIRECTION ( 'NONE',  ( 0.000000000000000000, -1.000000000000000000, 0.000000000000000000 ) ) ;
#15494=ORIENTED_EDGE ( 'NONE', *, *, #76391, .F. ) ;
#15495=CARTESIAN_POINT ( 'NONE',  ( 96.76980119632513322, -38.49712976775982298, 91.46133956162493917 ) ) ;
#15496=CARTESIAN_POINT ( 'NONE',  ( 108.4167997317111372, -26.73494551780935069, 164.9690142253840577 ) ) ;
#15500=VERTEX_POINT ( 'NONE', #23041 ) ;
#15501=CARTESIAN_POINT ( 'NONE',  ( 112.1400524529204148, -28.07738699070645438, 120.6531484116016912 ) ) ;
#15503=CARTESIAN_POINT ( 'NONE',  ( 95.75547692839532488, -40.34654347423973775, 127.5727681330539554 ) ) ;
#15505=CARTESIAN_POINT ( 'NONE',  ( 30.48091746481745901, -49.32844715994156815, 180.4678068554150911 ) ) ;
#15509=ORIENTED_EDGE ( 'NONE', *, *, #22282, .T. ) ;
#15510=CARTESIAN_POINT ( 'NONE',  ( 107.0664832912739399, -36.72944715994095333, 315.1356252759112522 ) ) ;
#15511=CARTESIAN_POINT ( 'NONE',  ( 107.8656169629272341, -46.51081515578102454, 173.6413395616249886 ) ) ;
#15512=CARTESIAN_POINT ( 'NONE',  ( 106.5646857698207981, -25.28130207810567498, 321.1698005525342978 ) ) ;
#15513=ORIENTED_EDGE ( 'NONE', *, *, #67656, .F. ) ;
#15514=CARTESIAN_POINT ( 'NONE',  ( 95.98894198207693762, -35.78073158428682632, 32.25848241876694544 ) ) ;
#15519=FACE_BOUND ( 'NONE', #72991, .T. ) ;
#15520=AXIS2_PLACEMENT_3D ( 'NONE', #16123, #65594, #42897 ) ;
#15521=CARTESIAN_POINT ( 'NONE',  ( 97.40895461294492463, -34.98419235835273611, 241.1841967044829573 ) ) ;
#15523=EDGE_LOOP ( 'NONE', ( #66561, #7753, #50453, #34741 ) ) ;
#15524=CARTESIAN_POINT ( 'NONE',  ( 108.1711956065674229, -46.05983505851052229, 159.1139642582779459 ) ) ;
#15526=VECTOR ( 'NONE', #36031, 1000.000000000000000 ) ;
#15527=DIRECTION ( 'NONE',  ( -0.7071067812162686872, -0.7071067811568263473, 2.899137802742872063E-29 ) ) ;
#15529=CARTESIAN_POINT ( 'NONE',  ( 101.4092135025303776, -29.90862777007100703, 37.05872616303995670 ) ) ;
#15532=B_SPLINE_CURVE_WITH_KNOTS ( 'NONE', 3,
 ( #70256, #759, #15749, #22125, #28460, #83004, #14406, #36183, #15303, #49346, #83901, #21213, #28927, #77976, #29378, #41628, #21672, #27572 ),
 .UNSPECIFIED., .F., .F.,
 ( 4, 2, 2, 2, 2, 2, 2, 2, 4 ),
 ( 0.4999919244375641281, 0.5624929338828685843, 0.6249939433281730405, 0.6874949527734776078, 0.7499959622187820640, 0.8124969716640865203, 0.8749979811093910875, 0.9374989905546955438, 1.000000000000000000 ),
 .UNSPECIFIED. ) ;
#15533=CARTESIAN_POINT ( 'NONE',  ( 48.16670390244661348, -28.27351298637380950, 117.4678068554150485 ) ) ;
#15535=CARTESIAN_POINT ( 'NONE',  ( 73.06648329127402519, -46.47944715994106701, -5.074374724089063982 ) ) ;
#15537=CARTESIAN_POINT ( 'NONE',  ( 105.1131368864170241, -25.87365329830167937, 275.2061014663871674 ) ) ;
#15538=CARTESIAN_POINT ( 'NONE',  ( 97.79668209375444121, -40.48056570805522369, 171.6327272062056295 ) ) ;
#15541=CARTESIAN_POINT ( 'NONE',  ( 101.9936209214569516, -45.44607152756502444, 87.15645860747564200 ) ) ;
#15543=CYLINDRICAL_SURFACE ( 'NONE', #57757, 5.599999999999994316 ) ;
#15546=VECTOR ( 'NONE', #4503, 1000.000000000000000 ) ;
#15547=CARTESIAN_POINT ( 'NONE',  ( 98.38136461969652657, -29.78821554292439444, 41.78991099019696520 ) ) ;
#15551=DIRECTION ( 'NONE',  ( 1.000000000000000000, 4.194175870806139918E-14, 0.000000000000000000 ) ) ;
#15552=CARTESIAN_POINT ( 'NONE',  ( 32.06670390244676128, -33.35206098992750157, 193.9678068554150911 ) ) ;
#15553=CARTESIAN_POINT ( 'NONE',  ( 112.4894639655092305, -46.36118470102660183, 257.9965776568635647 ) ) ;
#15557=LINE ( 'NONE', #16003, #37564 ) ;
#15558=LINE ( 'NONE', #57309, #77643 ) ;
#15559=EDGE_CURVE ( 'NONE', #71324, #82436, #85713, .T. ) ;
#15560=CYLINDRICAL_SURFACE ( 'NONE', #66888, 3.299999999999999822 ) ;
#15561=CARTESIAN_POINT ( 'NONE',  ( 114.5297761857384415, -31.21626383854846765, 107.1509475124489654 ) ) ;
#15562=CARTESIAN_POINT ( 'NONE',  ( 106.4823958901525458, -24.86854109859944373, 191.1156252759109861 ) ) ;
#15563=DIRECTION ( 'NONE',  ( -1.000000000000000000, 9.376883653928684652E-16, 1.500301384628589584E-15 ) ) ;
#15565=EDGE_CURVE ( 'NONE', #61198, #58395, #2138, .T. ) ;
#15566=CARTESIAN_POINT ( 'NONE',  ( 41.56648329127399677, -9.303447159940999356, 78.92562527591199739 ) ) ;
#15567=EDGE_LOOP ( 'NONE', ( #45739, #14034, #26057 ) ) ;
#15568=VECTOR ( 'NONE', #15139, 1000.000000000000000 ) ;
#15570=EDGE_CURVE ( 'NONE', #32982, #48113, #10523, .T. ) ;
#15571=FACE_BOUND ( 'NONE', #35193, .T. ) ;
#15572=ORIENTED_EDGE ( 'NONE', *, *, #27601, .F. ) ;
#15573=EDGE_LOOP ( 'NONE', ( #83420, #65712, #19462, #50343, #53812 ) ) ;
#15575=CARTESIAN_POINT ( 'NONE',  ( 97.78479357905025893, -40.45113604636035376, 42.62993149403730797 ) ) ;
#15576=EDGE_CURVE ( 'NONE', #30851, #39116, #9073, .T. ) ;
#15577=CARTESIAN_POINT ( 'NONE',  ( 100.8685319560204050, -42.60665150962044123, 81.35241982807694683 ) ) ;
#15578=CARTESIAN_POINT ( 'NONE',  ( 97.20287302226383019, -40.27875065248429820, 266.6013395616254797 ) ) ;
#15581=ORIENTED_EDGE ( 'NONE', *, *, #19918, .F. ) ;
#15582=ORIENTED_EDGE ( 'NONE', *, *, #10942, .F. ) ;
#15587=CARTESIAN_POINT ( 'NONE',  ( 114.7398264468854592, -44.75021323582976862, 113.1718157521009687 ) ) ;
#15589=DIRECTION ( 'NONE',  ( 0.0001713722456127401463, -0.9999999853157766072, -1.713722456137401502E-19 ) ) ;
#15591=VECTOR ( 'NONE', #18537, 1000.000000000000000 ) ;
#15592=CARTESIAN_POINT ( 'NONE',  ( 105.0216316738932107, -25.86677467614671500, 280.2365776568631759 ) ) ;
#15593=CARTESIAN_POINT ( 'NONE',  ( 97.75353936551157119, -40.54122631656009190, 7.635625275910939536 ) ) ;
#15594=VECTOR ( 'NONE', #42436, 1000.000000000000000 ) ;
#15595=CARTESIAN_POINT ( 'NONE',  ( 97.87053931029933551, -40.65856329638635458, 27.64823128951286080 ) ) ;
#15598=DIRECTION ( 'NONE',  ( 0.000000000000000000, 1.000000000000000000, 0.000000000000000000 ) ) ;
#15599=CARTESIAN_POINT ( 'NONE',  ( 86.06670390244796920, -50.82844715994100682, 151.9178068554149945 ) ) ;
#15600=CARTESIAN_POINT ( 'NONE',  ( 132.6453213455613991, -39.08531275930689475, 7.905164235259871219 ) ) ;
#15602=CARTESIAN_POINT ( 'NONE',  ( 194.0667039024475287, -24.92844715993407334, 180.4678068554150343 ) ) ;
#15603=LINE ( 'NONE', #21064, #60832 ) ;
#15605=DIRECTION ( 'NONE',  ( 1.000000000000000078E-15, -1.000000000000000000, 0.000000000000000000 ) ) ;
#15606=ORIENTED_EDGE ( 'NONE', *, *, #28959, .F. ) ;
#15608=CARTESIAN_POINT ( 'NONE',  ( 97.59524074137092953, -41.13874739096760891, 256.6727681330537507 ) ) ;
#15609=CARTESIAN_POINT ( 'NONE',  ( 117.7791004155048853, -34.00661502546044801, 165.0365776568629315 ) ) ;
#15610=CARTESIAN_POINT ( 'NONE',  ( 97.17561725847181719, -33.29990440931864271, 282.0613395616252888 ) ) ;
#15613=CARTESIAN_POINT ( 'NONE',  ( 101.9936209440171240, -45.44607154049054998, 47.15645860952901813 ) ) ;
#15615=CARTESIAN_POINT ( 'NONE',  ( 165.9667039024474491, -26.71338133338714016, 237.4678068554150059 ) ) ;
#15616=TOROIDAL_SURFACE ( 'NONE', #73561, 15.84999999999999964, 0.1499999999999999944 ) ;
#15617=ADVANCED_FACE ( 'NONE', ( #21693 ), #84377, .T. ) ;
#15619=DIRECTION ( 'NONE',  ( 1.000000000000000000, 1.110223024625155531E-13, 0.000000000000000000 ) ) ;
#15621=CARTESIAN_POINT ( 'NONE',  ( 104.3962608544918993, -28.61612207615715775, 164.7524198280769667 ) ) ;
#15622=PLANE ( 'NONE',  #26877 ) ;
#15623=VERTEX_POINT ( 'NONE', #44790 ) ;
#15624=DIRECTION ( 'NONE',  ( 1.000000000000000000, 0.000000000000000000, 0.000000000000000000 ) ) ;
#15625=CARTESIAN_POINT ( 'NONE',  ( 107.5647246096319094, -47.74832088493814553, 188.6003871806729535 ) ) ;
#15627=DIRECTION ( 'NONE',  ( 4.299999999999999979E-14, -1.000000000000000000, 4.400000000000000367E-29 ) ) ;
#15628=CARTESIAN_POINT ( 'NONE',  ( 97.81373435033219721, -40.51654435448209313, 87.63515866765291662 ) ) ;
#15630=CARTESIAN_POINT ( 'NONE',  ( 110.8522644532615828, -45.98514059693295053, 97.88543543875454134 ) ) ;
#15631=CARTESIAN_POINT ( 'NONE',  ( 102.6513375509277495, -45.45698538002856282, 127.2041967044829960 ) ) ;
#15634=VECTOR ( 'NONE', #16169, 1000.000000000000000 ) ;
#15635=CARTESIAN_POINT ( 'NONE',  ( 109.8762032759827321, -45.69504804023497968, 49.23777378208799149 ) ) ;
#15638=CARTESIAN_POINT ( 'NONE',  ( 101.7025241355417364, -45.60450926735014576, 198.1318157521009482 ) ) ;
#15639=CARTESIAN_POINT ( 'NONE',  ( 109.6430121981732952, -46.48008671661597191, 37.78145861478355272 ) ) ;
#15640=CYLINDRICAL_SURFACE ( 'NONE', #37676, 2.750000000000002665 ) ;
#15641=CARTESIAN_POINT ( 'NONE',  ( 97.80791547859365664, -40.51903635482080546, 112.6360621818907077 ) ) ;
#15643=PLANE ( 'NONE',  #28921 ) ;
#15644=CARTESIAN_POINT ( 'NONE',  ( 131.3164832912739826, -18.72944715994100662, 3.101481641215524832 ) ) ;
#15645=CARTESIAN_POINT ( 'NONE',  ( 97.63679352021414104, -31.00714225716590278, 125.8803871806719599 ) ) ;
#15646=VERTEX_POINT ( 'NONE', #17977 ) ;
#15647=ORIENTED_EDGE ( 'NONE', *, *, #73537, .F. ) ;
#15648=EDGE_LOOP ( 'NONE', ( #3668, #11072, #80898, #25802 ) ) ;
#15650=AXIS2_PLACEMENT_3D ( 'NONE', #73864, #4830, #38438 ) ;
#15651=CARTESIAN_POINT ( 'NONE',  ( 97.33763304300855168, -34.07186372398516028, 131.1148582292631772 ) ) ;
#15652=CARTESIAN_POINT ( 'NONE',  ( 104.4075942973239393, -46.45795486759642046, 103.3647508459505246 ) ) ;
#15653=CARTESIAN_POINT ( 'NONE',  ( 104.8109701446277171, -28.85573464981227687, 223.1166617981629656 ) ) ;
#15655=AXIS2_PLACEMENT_3D ( 'NONE', #35143, #20644, #14276 ) ;
#15656=CARTESIAN_POINT ( 'NONE',  ( 21.03715912545823130, -47.82818131006186491, 313.9678068554150059 ) ) ;
#15657=CARTESIAN_POINT ( 'NONE',  ( 114.5123156819773698, -29.42664080734638787, 149.4441967044819819 ) ) ;
#15658=DIRECTION ( 'NONE',  ( 0.000000000000000000, 0.000000000000000000, -1.000000000000000000 ) ) ;
#15659=ORIENTED_EDGE ( 'NONE', *, *, #39941, .F. ) ;
#15661=ORIENTED_EDGE ( 'NONE', *, *, #8102, .F. ) ;
#15663=CARTESIAN_POINT ( 'NONE',  ( 123.6837132603319560, -53.34645651782485487, 218.8274735512161158 ) ) ;
#15666=DIRECTION ( 'NONE',  ( -0.7071067811865101582, -0.7071067811865849873, 0.000000000000000000 ) ) ;
#15667=ADVANCED_FACE ( 'NONE', ( #10715 ), #24803, .F. ) ;
#15668=CARTESIAN_POINT ( 'NONE',  ( 132.4277392773736040, -34.51875925606939433, 7.791169830160155740 ) ) ;
#15669=CARTESIAN_POINT ( 'NONE',  ( 98.49168440212470443, -38.96576165349271292, 272.9615833058970225 ) ) ;
#15674=CIRCLE ( 'NONE', #28753, 2.999999999999919176 ) ;
#15675=VECTOR ( 'NONE', #73653, 1000.000000000000000 ) ;
#15676=CARTESIAN_POINT ( 'NONE',  ( 115.9158992903809633, -39.94991172188729678, 9.635625275910943088 ) ) ;
#15678=ORIENTED_EDGE ( 'NONE', *, *, #77160, .T. ) ;
#15680=AXIS2_PLACEMENT_3D ( 'NONE', #54804, #47552, #76170 ) ;
#15681=CARTESIAN_POINT ( 'NONE',  ( 110.8545889635279309, -45.98418948027816811, 112.8856353431071398 ) ) ;
#15684=EDGE_CURVE ( 'NONE', #13968, #19262, #85918, .T. ) ;
#15685=CARTESIAN_POINT ( 'NONE',  ( 111.3125147634731462, -44.27080922411229835, 255.8147570362582712 ) ) ;
#15686=CARTESIAN_POINT ( 'NONE',  ( 101.9611696646907433, -46.55956485693801028, 167.1832443235299763 ) ) ;
#15687=CARTESIAN_POINT ( 'NONE',  ( 108.5866130067098538, -47.05677245125747277, 142.6927681330539883 ) ) ;
#15688=EDGE_CURVE ( 'NONE', #60205, #2787, #32054, .T. ) ;
#15689=CYLINDRICAL_SURFACE ( 'NONE', #10422, 1.000000000000000888 ) ;
#15690=CARTESIAN_POINT ( 'NONE',  ( 113.0254242409527308, -46.03885118181761982, 214.0175300378159591 ) ) ;
#15692=DIRECTION ( 'NONE',  ( 0.000000000000000000, 0.000000000000000000, -1.000000000000000000 ) ) ;
#15694=DIRECTION ( 'NONE',  ( 1.000000000000000000, 8.163404592831600092E-16, 1.020425574103949962E-15 ) ) ;
#15696=ORIENTED_EDGE ( 'NONE', *, *, #38610, .F. ) ;
#15697=AXIS2_PLACEMENT_3D ( 'NONE', #83304, #5205, #41491 ) ;
#15698=CARTESIAN_POINT ( 'NONE',  ( 101.1758151987629333, -45.38431258166273352, 197.1013395616249966 ) ) ;
#15699=ORIENTED_EDGE ( 'NONE', *, *, #54699, .F. ) ;
#15700=CARTESIAN_POINT ( 'NONE',  ( 102.6160711382646156, -46.84739750188308705, 132.2346728949579528 ) ) ;
#15701=FACE_OUTER_BOUND ( 'NONE', #66639, .T. ) ;
#15702=CARTESIAN_POINT ( 'NONE',  ( 136.3178028891369422, -35.14744377621116200, 7.339349742409597255 ) ) ;
#15704=CARTESIAN_POINT ( 'NONE',  ( 143.9834832912729894, -71.52944715994142655, 342.9256252759109884 ) ) ;
#15706=CARTESIAN_POINT ( 'NONE',  ( 97.57986484199628308, -43.79006170206856297, 257.8356252759109566 ) ) ;
#15710=DIRECTION ( 'NONE',  ( -0.7071067811865779928, 0.7071067811865171526, -7.071067811865476319E-16 ) ) ;
#15711=CARTESIAN_POINT ( 'NONE',  ( 109.7248659108412170, -27.00080517668511249, 255.8647919434466473 ) ) ;
#15712=DIRECTION ( 'NONE',  ( 1.000000000000000000, 4.237773401492740281E-14, 0.000000000000000000 ) ) ;
#15713=CARTESIAN_POINT ( 'NONE',  ( 99.34894212307516170, -29.65511154620466172, 275.7356252759109907 ) ) ;
#15714=ORIENTED_EDGE ( 'NONE', *, *, #23337, .F. ) ;
#15716=CARTESIAN_POINT ( 'NONE',  ( 114.5280328947845732, -29.41122550446140949, 149.4441967044819819 ) ) ;
#15717=CARTESIAN_POINT ( 'NONE',  ( 98.30635682897023742, -28.74854496012902771, 76.73848241876795839 ) ) ;
#15718=CARTESIAN_POINT ( 'NONE',  ( 116.4163124136858443, -41.43834035574819552, 199.4556252759109611 ) ) ;
#15720=LINE ( 'NONE', #14830, #17060 ) ;
#15721=CYLINDRICAL_SURFACE ( 'NONE', #26004, 3.000000000000002665 ) ;
#15723=CARTESIAN_POINT ( 'NONE',  ( 182.2420472961719895, -31.76306994223730840, -5.074374724088000832 ) ) ;
#15726=FACE_OUTER_BOUND ( 'NONE', #87837, .T. ) ;
#15727=AXIS2_PLACEMENT_3D ( 'NONE', #16062, #84664, #15619 ) ;
#15728=AXIS2_PLACEMENT_3D ( 'NONE', #37719, #65415, #64967 ) ;
#15730=ORIENTED_EDGE ( 'NONE', *, *, #61073, .T. ) ;
#15732=AXIS2_PLACEMENT_3D ( 'NONE', #58633, #51368, #79112 ) ;
#15733=DIRECTION ( 'NONE',  ( 0.000000000000000000, 0.000000000000000000, -1.000000000000000000 ) ) ;
#15735=CARTESIAN_POINT ( 'NONE',  ( 116.1047473792919504, -29.10330858331350612, 70.38419670448192278 ) ) ;
#15736=CARTESIAN_POINT ( 'NONE',  ( 31.56670390244800828, -32.29483332968611364, 117.4678068554150485 ) ) ;
#15737=VECTOR ( 'NONE', #23902, 1000.000000000000000 ) ;
#15740=AXIS2_PLACEMENT_3D ( 'NONE', #70714, #8491, #29382 ) ;
#15741=AXIS2_PLACEMENT_3D ( 'NONE', #84537, #16375, #72231 ) ;
#15742=CARTESIAN_POINT ( 'NONE',  ( 100.7700969181924506, -30.95782257301981488, 275.1581341137911068 ) ) ;
#15743=ORIENTED_EDGE ( 'NONE', *, *, #28252, .T. ) ;
#15744=EDGE_LOOP ( 'NONE', ( #2204, #44855, #5039, #49619 ) ) ;
#15745=EDGE_LOOP ( 'NONE', ( #39573, #6649, #40203, #1587, #1818 ) ) ;
#15747=CARTESIAN_POINT ( 'NONE',  ( 117.0718954852079605, -35.46248235573542473, 108.9272919426195614 ) ) ;
#15749=CARTESIAN_POINT ( 'NONE',  ( 97.06108334801497506, -37.99647572000111495, 162.4272970119406523 ) ) ;
#15750=CARTESIAN_POINT ( 'NONE',  ( 97.31578350476630135, -39.30578092224938302, 21.53098511257883274 ) ) ;
#15751=DIRECTION ( 'NONE',  ( 0.000000000000000000, 0.000000000000000000, 1.000000000000000000 ) ) ;
#15752=DIRECTION ( 'NONE',  ( -0.9963424814100679816, 0.08544974978095716545, 0.000000000000000000 ) ) ;
#15753=DIRECTION ( 'NONE',  ( 9.351236661543306751E-17, -3.725950533538267725E-29, -1.000000000000000000 ) ) ;
#15754=CARTESIAN_POINT ( 'NONE',  ( 64.68306507141299733, -72.55818180160879649, 394.9756252759101471 ) ) ;
#15755=CARTESIAN_POINT ( 'NONE',  ( 107.1951288810177090, -26.32694189238797833, 35.06705384733893283 ) ) ;
#15761=DIRECTION ( 'NONE',  ( 9.032638163712999905E-13, -1.000000000000000000, 4.100000000000000342E-29 ) ) ;
#15762=CARTESIAN_POINT ( 'NONE',  ( 99.91476266851738330, -32.73750773393640401, 108.7395189410199663 ) ) ;
#15764=EDGE_CURVE ( 'NONE', #1830, #57751, #46564, .T. ) ;
#15768=CARTESIAN_POINT ( 'NONE',  ( 117.0718258217757466, -35.46190141227904746, 138.9264153952272807 ) ) ;
#15769=EDGE_LOOP ( 'NONE', ( #70176, #75321 ) ) ;
#15772=CARTESIAN_POINT ( 'NONE',  ( 108.0951925567892431, -27.89746624773302841, 126.4158690201829813 ) ) ;
#15773=AXIS2_PLACEMENT_3D ( 'NONE', #15254, #29775, #2070 ) ;
#15774=PLANE ( 'NONE',  #46681 ) ;
#15775=CARTESIAN_POINT ( 'NONE',  ( 104.2081133107797228, -25.20330419090194951, 86.26991099019699050 ) ) ;
#15776=CARTESIAN_POINT ( 'NONE',  ( 114.6097843884836323, -43.32694117741820605, 18.25468785797279025 ) ) ;
#15777=AXIS2_PLACEMENT_3D ( 'NONE', #72705, #31351, #73582 ) ;
#15780=VERTEX_POINT ( 'NONE', #58858 ) ;
#15781=ORIENTED_EDGE ( 'NONE', *, *, #11179, .T. ) ;
#15782=EDGE_CURVE ( 'NONE', #29833, #32371, #40948, .T. ) ;
#15783=CARTESIAN_POINT ( 'NONE',  ( 108.9893125699443175, -46.99828796752551341, 82.72419670448194040 ) ) ;
#15785=CARTESIAN_POINT ( 'NONE',  ( 99.99555918775621421, -44.36035129061385618, 46.98133956162592284 ) ) ;
#15786=CARTESIAN_POINT ( 'NONE',  ( 96.02367466659750050, -35.86829477906547226, 187.2765776568629406 ) ) ;
#15787=EDGE_CURVE ( 'NONE', #223, #13942, #58421, .T. ) ;
#15789=CARTESIAN_POINT ( 'NONE',  ( 100.8868993066867432, -44.69975041575762020, 128.0522334713024293 ) ) ;
#15790=CARTESIAN_POINT ( 'NONE',  ( 107.3339483091110225, -26.30778942656879948, 116.0556252759109555 ) ) ;
#15791=CARTESIAN_POINT ( 'NONE',  ( 31.89136050872298966, -31.76306994223740432, 342.9256252759109884 ) ) ;
#15792=ADVANCED_FACE ( 'NONE', ( #45224 ), #24365, .F. ) ;
#15793=EDGE_LOOP ( 'NONE', ( #81798, #28043, #70438, #46268, #46084 ) ) ;
#15794=AXIS2_PLACEMENT_3D ( 'NONE', #86905, #79213, #72385 ) ;
#15796=EDGE_CURVE ( 'NONE', #73048, #25675, #52471, .T. ) ;
#15797=ORIENTED_EDGE ( 'NONE', *, *, #36475, .T. ) ;
#15798=VECTOR ( 'NONE', #60698, 1000.000000000000000 ) ;
#15799=CARTESIAN_POINT ( 'NONE',  ( 97.82514972460828062, -40.55017182310744062, 132.6388286205130385 ) ) ;
#15803=LINE ( 'NONE', #76679, #8718 ) ;
#15804=CARTESIAN_POINT ( 'NONE',  ( 116.7272869458707305, -31.35841744470506498, 29.24229194257799236 ) ) ;
#15806=CARTESIAN_POINT ( 'NONE',  ( 172.5664832912740110, -36.32844715994070839, 138.9256252759119832 ) ) ;
#15808=CARTESIAN_POINT ( 'NONE',  ( 99.77418633167435758, -43.29726106931981633, 56.90991099019693422 ) ) ;
#15809=DIRECTION ( 'NONE',  ( 0.000000000000000000, 0.000000000000000000, -1.000000000000000000 ) ) ;
#15810=CARTESIAN_POINT ( 'NONE',  ( 97.76587557681025942, -42.65924729906315349, 137.7661014663869992 ) ) ;
#15811=PLANE ( 'NONE',  #23393 ) ;
#15813=ORIENTED_EDGE ( 'NONE', *, *, #63632, .T. ) ;
#15815=DIRECTION ( 'NONE',  ( 1.000000000000000000, 4.163336342344333240E-14, 0.000000000000000000 ) ) ;
#15817=ORIENTED_EDGE ( 'NONE', *, *, #62008, .T. ) ;
#15818=DIRECTION ( 'NONE',  ( -1.000000000000000078E-15, -1.000000000000000083E-30, 1.000000000000000000 ) ) ;
#15819=CARTESIAN_POINT ( 'NONE',  ( 109.3681991936945508, -25.87058038976459429, 184.9222919425779708 ) ) ;
#15822=CARTESIAN_POINT ( 'NONE',  ( 116.0738972362454149, -42.02130438377608357, 234.4041967044819899 ) ) ;
#15823=CARTESIAN_POINT ( 'NONE',  ( 117.9015171282527916, -39.13767059441630636, 99.64038718067195077 ) ) ;
#15824=CARTESIAN_POINT ( 'NONE',  ( 91.12500358871285755, -35.36225116344564157, 302.4856252759109907 ) ) ;
#15825=CYLINDRICAL_SURFACE ( 'NONE', #56125, 9.999999999999998224 ) ;
#15826=CIRCLE ( 'NONE', #40438, 2.116999999999993776 ) ;
#15827=LINE ( 'NONE', #8564, #74290 ) ;
#15828=ORIENTED_EDGE ( 'NONE', *, *, #19246, .T. ) ;
#15829=ORIENTED_EDGE ( 'NONE', *, *, #71382, .T. ) ;
#15830=ORIENTED_EDGE ( 'NONE', *, *, #52196, .F. ) ;
#15833=CARTESIAN_POINT ( 'NONE',  ( 100.8232821092315845, -45.85065428865130599, 238.1108633711489517 ) ) ;
#15835=CARTESIAN_POINT ( 'NONE',  ( 107.3428450438784694, -25.27364292152175551, 322.4523926293242653 ) ) ;
#15836=VECTOR ( 'NONE', #60472, 1000.000000000000000 ) ;
#15837=DIRECTION ( 'NONE',  ( 1.000000000000000078E-15, 1.000000000000000083E-30, -1.000000000000000000 ) ) ;
#15840=CARTESIAN_POINT ( 'NONE',  ( 105.4174756516424054, -47.04580008967651850, 37.44991099019695469 ) ) ;
#15843=VECTOR ( 'NONE', #60284, 1000.000000000000000 ) ;
#15847=CARTESIAN_POINT ( 'NONE',  ( 116.3181387014812458, -32.94505625723229514, 15.13562527591094664 ) ) ;
#15848=EDGE_CURVE ( 'NONE', #46344, #21324, #68827, .T. ) ;
#15849=CARTESIAN_POINT ( 'NONE',  ( 116.8725690376871569, -36.55701438716827312, 284.8413395616245793 ) ) ;
#15850=DIRECTION ( 'NONE',  ( -0.7071067811869841124, 0.7071067811861110330, 0.000000000000000000 ) ) ;
#15851=AXIS2_PLACEMENT_3D ( 'NONE', #28159, #28616, #35875 ) ;
#15852=EDGE_CURVE ( 'NONE', #56233, #72479, #72858, .T. ) ;
#15853=CARTESIAN_POINT ( 'NONE',  ( 101.8448680821487642, -28.45912855063591351, 106.5241967044819944 ) ) ;
#15855=EDGE_CURVE ( 'NONE', #36904, #3733, #63242, .T. ) ;
#15858=EDGE_CURVE ( 'NONE', #42921, #18344, #10485, .T. ) ;
#15859=CARTESIAN_POINT ( 'NONE',  ( 78.02982435611764345, -34.87939921900456142, 2.327894594453169042 ) ) ;
#15861=ORIENTED_EDGE ( 'NONE', *, *, #40284, .T. ) ;
#15863=CARTESIAN_POINT ( 'NONE',  ( 98.91757684337089529, -33.81461462136097396, 23.88332846482899186 ) ) ;
#15864=ADVANCED_FACE ( 'NONE', ( #75646 ), #49590, .T. ) ;
#15865=DIRECTION ( 'NONE',  ( 2.900000000000000265E-14, -2.000000000000000155E-15, 1.000000000000000000 ) ) ;
#15866=EDGE_CURVE ( 'NONE', #88862, #32266, #13418, .T. ) ;
#15867=AXIS2_PLACEMENT_3D ( 'NONE', #5632, #25157, #46482 ) ;
#15870=LINE ( 'NONE', #51248, #69142 ) ;
#15871=ORIENTED_EDGE ( 'NONE', *, *, #23886, .T. ) ;
#15872=LINE ( 'NONE', #57178, #47937 ) ;
#15873=DIRECTION ( 'NONE',  ( 0.000000000000000000, 0.000000000000000000, -1.000000000000000000 ) ) ;
#15874=ORIENTED_EDGE ( 'NONE', *, *, #1230, .F. ) ;
#15875=CARTESIAN_POINT ( 'NONE',  ( 116.9750915152277884, -33.48807190773455034, 89.07848241876791917 ) ) ;
#15876=EDGE_LOOP ( 'NONE', ( #25160, #49711, #11893 ) ) ;
#15877=CARTESIAN_POINT ( 'NONE',  ( 100.5751258508236674, -42.28088033547287949, 31.31241982807697610 ) ) ;
#15879=FACE_OUTER_BOUND ( 'NONE', #43991, .T. ) ;
#15880=CARTESIAN_POINT ( 'NONE',  ( 96.59955023297820276, -32.98040794253977737, 176.0527681330549683 ) ) ;
#15883=DIRECTION ( 'NONE',  ( 0.000000000000000000, 0.000000000000000000, 1.000000000000000000 ) ) ;
#15885=AXIS2_PLACEMENT_3D ( 'NONE', #22573, #63442, #84807 ) ;
#15886=CARTESIAN_POINT ( 'NONE',  ( 102.3596500697202174, -47.65578173298946751, 283.2527681330539053 ) ) ;
#15887=VERTEX_POINT ( 'NONE', #5711 ) ;
#15890=CARTESIAN_POINT ( 'NONE',  ( 117.1680251128577908, -33.85633223813928794, 145.0470538473399529 ) ) ;
#15893=EDGE_LOOP ( 'NONE', ( #17638, #5431, #19091, #83818, #40563, #76163, #41694, #68287, #84775, #36747, #59765, #35654 ) ) ;
#15894=VERTEX_POINT ( 'NONE', #21924 ) ;
#15895=CARTESIAN_POINT ( 'NONE',  ( 101.9936208123286150, -45.44607146504151274, 122.1564585975432067 ) ) ;
#15898=CARTESIAN_POINT ( 'NONE',  ( 41.56648329127381203, -18.82844715994071194, 321.9256252759119548 ) ) ;
#15899=CARTESIAN_POINT ( 'NONE',  ( 142.8687636814962616, 5.654319119531167281, 361.9756252759100335 ) ) ;
#15900=CARTESIAN_POINT ( 'NONE',  ( 115.9451031845006099, -42.19318012571019949, 14.38705384733995984 ) ) ;
#15901=DIRECTION ( 'NONE',  ( 0.000000000000000000, 0.000000000000000000, -1.000000000000000000 ) ) ;
#15902=EDGE_CURVE ( 'NONE', #78335, #35491, #45291, .T. ) ;
#15903=ORIENTED_EDGE ( 'NONE', *, *, #79250, .F. ) ;
#15904=DIRECTION ( 'NONE',  ( -4.237773401492740281E-14, 1.000000000000000000, 0.000000000000000000 ) ) ;
#15906=EDGE_CURVE ( 'NONE', #25266, #11985, #6155, .T. ) ;
#15907=CARTESIAN_POINT ( 'NONE',  ( 117.0718948736623020, -35.46247637142937492, 43.92702797836822981 ) ) ;
#15908=VERTEX_POINT ( 'NONE', #20233 ) ;
#15909=ORIENTED_EDGE ( 'NONE', *, *, #7417, .F. ) ;
#15910=AXIS2_PLACEMENT_3D ( 'NONE', #29644, #49623, #1950 ) ;
#15912=DIRECTION ( 'NONE',  ( 1.000000000000000078E-15, 0.000000000000000000, -1.000000000000000000 ) ) ;
#15913=PLANE ( 'NONE',  #74500 ) ;
#15915=DIRECTION ( 'NONE',  ( -0.000000000000000000, 1.000000000000000000, 0.000000000000000000 ) ) ;
#15917=CARTESIAN_POINT ( 'NONE',  ( 109.5825779133427460, -28.02991049533996204, 214.2628960185529365 ) ) ;
#15918=LINE ( 'NONE', #44039, #70783 ) ;
#15919=CARTESIAN_POINT ( 'NONE',  ( 95.28387218206130171, -35.72034718286344912, 32.25848241876794020 ) ) ;
#15921=CARTESIAN_POINT ( 'NONE',  ( 96.04102276344947597, -38.01478905114413465, 86.43086337114897333 ) ) ;
#15923=CARTESIAN_POINT ( 'NONE',  ( 131.3164832912739826, -18.72944715994100662, 6.749768910606465333 ) ) ;
#15925=AXIS2_PLACEMENT_3D ( 'NONE', #16784, #44465, #9083 ) ;
#15926=DIRECTION ( 'NONE',  ( -0.000000000000000000, 1.000000000000000000, 0.000000000000000000 ) ) ;
#15928=DIRECTION ( 'NONE',  ( 1.000000000000000000, -6.745093096447288888E-17, 9.693101022688619289E-16 ) ) ;
#15929=EDGE_LOOP ( 'NONE', ( #86961, #51835, #66029, #6377 ) ) ;
#15930=DIRECTION ( 'NONE',  ( 0.9068632946707807507, -0.4214249218767880945, 8.673617379884035472E-16 ) ) ;
#15932=FACE_OUTER_BOUND ( 'NONE', #81469, .T. ) ;
#15933=CIRCLE ( 'NONE', #50724, 6.571100913904396990 ) ;
#15934=CARTESIAN_POINT ( 'NONE',  ( 152.0371591254585155, -47.82818131005588214, 180.4678068554149775 ) ) ;
#15935=LINE ( 'NONE', #29556, #53822 ) ;
#15936=ORIENTED_EDGE ( 'NONE', *, *, #59644, .T. ) ;
#15937=CARTESIAN_POINT ( 'NONE',  ( 97.20468889015201341, -31.68559423518837193, 95.96229194257799122 ) ) ;
#15939=CARTESIAN_POINT ( 'NONE',  ( 97.39138288182120107, -39.27886290962566562, 166.5314880106770659 ) ) ;
#15940=DIRECTION ( 'NONE',  ( 0.000000000000000000, 0.000000000000000000, 1.000000000000000000 ) ) ;
#15943=CIRCLE ( 'NONE', #60841, 2.117000000000000881 ) ;
#15945=CARTESIAN_POINT ( 'NONE',  ( 97.33784134059621351, -34.07106442472682772, 156.1147919339565817 ) ) ;
#15947=DIRECTION ( 'NONE',  ( 5.512527431108029424E-15, -1.000000000000000000, 0.000000000000000000 ) ) ;
#15949=CARTESIAN_POINT ( 'NONE',  ( 180.1667039024460166, -26.71338133339240528, -5.074374724088000832 ) ) ;
#15953=EDGE_CURVE ( 'NONE', #2317, #20780, #81582, .T. ) ;
#15954=LINE ( 'NONE', #77736, #70903 ) ;
#15956=CARTESIAN_POINT ( 'NONE',  ( 97.38117110781249153, -35.36630255995241612, 177.2156252759109805 ) ) ;
#15958=ORIENTED_EDGE ( 'NONE', *, *, #60966, .T. ) ;
#15959=AXIS2_PLACEMENT_3D ( 'NONE', #60061, #32820, #87352 ) ;
#15960=EDGE_CURVE ( 'NONE', #26855, #7253, #33405, .T. ) ;
#15961=CARTESIAN_POINT ( 'NONE',  ( 110.8778723966665751, -46.37372517157803742, 18.88800622829095488 ) ) ;
#15962=DIRECTION ( 'NONE',  ( 0.000000000000000000, 0.000000000000000000, 1.000000000000000000 ) ) ;
#15966=ADVANCED_FACE ( 'NONE', ( #47905 ), #33850, .T. ) ;
#15967=CARTESIAN_POINT ( 'NONE',  ( 100.9552578586416018, -28.70656802983730671, 30.59412679818443337 ) ) ;
#15968=CARTESIAN_POINT ( 'NONE',  ( 99.44473759953881142, -30.59981194223813361, 240.7870538473399620 ) ) ;
#15969=ORIENTED_EDGE ( 'NONE', *, *, #75883, .F. ) ;
#15970=ORIENTED_EDGE ( 'NONE', *, *, #71995, .F. ) ;
#15971=CARTESIAN_POINT ( 'NONE',  ( 97.15642216441104040, -38.53537999780244405, 197.9015833058969633 ) ) ;
#15972=CIRCLE ( 'NONE', #1451, 0.5000000000000004441 ) ;
#15974=CARTESIAN_POINT ( 'NONE',  ( 116.8159028922284648, -34.14818352781880151, 55.03137681045001273 ) ) ;
#15975=CARTESIAN_POINT ( 'NONE',  ( 101.8597501770084364, -45.35270844728685802, 48.57586902018196184 ) ) ;
#15977=EDGE_CURVE ( 'NONE', #23851, #1382, #39524, .T. ) ;
#15983=DIRECTION ( 'NONE',  ( 0.000000000000000000, 0.000000000000000000, 1.000000000000000000 ) ) ;
#15985=CARTESIAN_POINT ( 'NONE',  ( 115.2346088729120339, -30.22974330756297690, 244.3613395616249875 ) ) ;
#15987=VERTEX_POINT ( 'NONE', #88386 ) ;
#15988=ORIENTED_EDGE ( 'NONE', *, *, #36853, .F. ) ;
#15989=EDGE_CURVE ( 'NONE', #27698, #29421, #30510, .T. ) ;
#15990=CARTESIAN_POINT ( 'NONE',  ( 105.7154773210734220, -46.72385839103964855, 82.46895860850119675 ) ) ;
#15991=FACE_OUTER_BOUND ( 'NONE', #84926, .T. ) ;
#15993=DIRECTION ( 'NONE',  ( 1.000000000000000000, 6.145690160522439356E-16, 0.000000000000000000 ) ) ;
#15995=CARTESIAN_POINT ( 'NONE',  ( 110.1676348244934331, -46.62498374987613659, 48.80610146638597513 ) ) ;
#15996=CARTESIAN_POINT ( 'NONE',  ( 51.56670390244699576, -19.82844715994031048, -5.074374724088000832 ) ) ;
#15998=CARTESIAN_POINT ( 'NONE',  ( 118.1291538054787509, -37.63212066291781355, 34.77372051400695341 ) ) ;
#15999=PLANE ( 'NONE',  #77278 ) ;
#16000=CARTESIAN_POINT ( 'NONE',  ( 99.33304576907053729, -28.83178728225833609, 270.7051490854348685 ) ) ;
#16002=CIRCLE ( 'NONE', #30461, 10.00000000000000888 ) ;
#16003=CARTESIAN_POINT ( 'NONE',  ( 37.35959712141530531, -48.62134037890907479, 180.4678068554150911 ) ) ;
#16004=DIRECTION ( 'NONE',  ( 1.000000000000000000, 0.000000000000000000, 0.000000000000000000 ) ) ;
#16006=CARTESIAN_POINT ( 'NONE',  ( 110.2109830224615052, -27.99972479296931382, 97.61951894101994753 ) ) ;
#16007=CARTESIAN_POINT ( 'NONE',  ( 102.2271567091324158, -45.98785831331388607, 208.1927681330539599 ) ) ;
#16008=CARTESIAN_POINT ( 'NONE',  ( 107.0664832912739399, -36.72944715994095333, 302.6356252759109680 ) ) ;
#16009=EDGE_LOOP ( 'NONE', ( #36790, #50827, #20500, #17506 ) ) ;
#16010=EDGE_CURVE ( 'NONE', #73246, #61299, #27994, .T. ) ;
#16013=ORIENTED_EDGE ( 'NONE', *, *, #1081, .T. ) ;
#16014=ORIENTED_EDGE ( 'NONE', *, *, #24103, .F. ) ;
#16016=( BOUNDED_CURVE ( )  B_SPLINE_CURVE ( 3, ( #49072, #35007, #76806, #14589 ),
 .UNSPECIFIED., .F., .T. ) 
 B_SPLINE_CURVE_WITH_KNOTS ( ( 4, 4 ),
 ( 4.712388980378937831, 6.283185307174309564 ),
 .UNSPECIFIED. ) 
 CURVE ( )  GEOMETRIC_REPRESENTATION_ITEM ( )  RATIONAL_B_SPLINE_CURVE ( ( 1.000000000000000000, 0.8047378541230092441, 0.8047378541230092441, 1.000000000000000000 ) ) 
 REPRESENTATION_ITEM ( '' )  );
#16018=VERTEX_POINT ( 'NONE', #22819 ) ;
#16020=CARTESIAN_POINT ( 'NONE',  ( 97.81136857603131318, -40.51756142711754194, 161.6353372277744143 ) ) ;
#16021=CARTESIAN_POINT ( 'NONE',  ( 107.2856214976012552, -28.19082255356615008, 119.4781341137909578 ) ) ;
#16022=CARTESIAN_POINT ( 'NONE',  ( 100.2327115992702176, -45.44695862323239055, 277.0594347997204068 ) ) ;
#16023=AXIS2_PLACEMENT_3D ( 'NONE', #59509, #39526, #33162 ) ;
#16024=DIRECTION ( 'NONE',  ( 0.000000000000000000, 1.000000000000000000, 0.000000000000000000 ) ) ;
#16025=EDGE_LOOP ( 'NONE', ( #87482, #78346, #31251, #55620 ) ) ;
#16026=CIRCLE ( 'NONE', #65301, 16.00000000000000000 ) ;
#16027=EDGE_CURVE ( 'NONE', #29809, #16028, #43681, .T. ) ;
#16028=VERTEX_POINT ( 'NONE', #72301 ) ;
#16031=FACE_OUTER_BOUND ( 'NONE', #32850, .T. ) ;
#16033=EDGE_CURVE ( 'NONE', #73048, #56141, #24149, .T. ) ;
#16034=CARTESIAN_POINT ( 'NONE',  ( 98.16479183632776540, -43.36064410082828857, 111.8480062282919647 ) ) ;
#16035=CARTESIAN_POINT ( 'NONE',  ( 111.0096634661633885, -46.42778601040829045, 282.8841967044824628 ) ) ;
#16036=ORIENTED_EDGE ( 'NONE', *, *, #55495, .F. ) ;
#16037=UNCERTAINTY_MEASURE_WITH_UNIT (LENGTH_MEASURE( 1.000000000000000082E-05 ), #48823, 'distance_accuracy_value', 'NONE');
#16038=CARTESIAN_POINT ( 'NONE',  ( 96.24916995763402383, -34.45682319295006124, 261.1737205140064475 ) ) ;
#16042=CARTESIAN_POINT ( 'NONE',  ( 97.81193178031652735, -40.51732023384165160, 27.63604381180012837 ) ) ;
#16043=LINE ( 'NONE', #2408, #12918 ) ;
#16044=DIRECTION ( 'NONE',  ( 0.000000000000000000, 0.000000000000000000, 1.000000000000000000 ) ) ;
#16045=CARTESIAN_POINT ( 'NONE',  ( 106.6155744189988326, -25.27918481551454732, 323.5352776872487652 ) ) ;
#16046=FACE_OUTER_BOUND ( 'NONE', #42275, .T. ) ;
#16047=CARTESIAN_POINT ( 'NONE',  ( 20.03715912545737510, -24.95799193693189721, 249.9678068554150059 ) ) ;
#16050=CARTESIAN_POINT ( 'NONE',  ( 95.60734603896362671, -36.72944715994100306, 293.2242906452868851 ) ) ;
#16051=DIRECTION ( 'NONE',  ( -0.9988791501868375944, -0.04215501712985142424, 0.02152667770007998804 ) ) ;
#16052=DIRECTION ( 'NONE',  ( 0.000000000000000000, 0.000000000000000000, 1.000000000000000000 ) ) ;
#16054=CARTESIAN_POINT ( 'NONE',  ( 115.4801557161918311, -43.01927310766588874, 28.31562527591097123 ) ) ;
#16055=CARTESIAN_POINT ( 'NONE',  ( 113.6142049395107421, -45.63457611473454989, 179.0689586092439640 ) ) ;
#16056=CARTESIAN_POINT ( 'NONE',  ( 116.7902211891048694, -31.42528581690661582, 20.21181575210195902 ) ) ;
#16057=DIRECTION ( 'NONE',  ( 4.299999999999999979E-14, -1.000000000000000000, 4.400000000000000367E-29 ) ) ;
#16058=CARTESIAN_POINT ( 'NONE',  ( 82.81648064515525220, -36.72944715939136273, 6.749772901088423538 ) ) ;
#16060=EDGE_LOOP ( 'NONE', ( #25568, #20622, #17062, #21051 ) ) ;
#16062=CARTESIAN_POINT ( 'NONE',  ( 163.0667039024479550, -33.35206098992140511, 117.4678068554150485 ) ) ;
#16063=VERTEX_POINT ( 'NONE', #80018 ) ;
#16064=EDGE_CURVE ( 'NONE', #28268, #5970, #79121, .T. ) ;
#16065=CIRCLE ( 'NONE', #45015, 2.117000000000007987 ) ;
#16066=CARTESIAN_POINT ( 'NONE',  ( 113.0229309284916184, -28.24065945027253477, 80.57753003781498080 ) ) ;
#16068=ORIENTED_EDGE ( 'NONE', *, *, #53027, .T. ) ;
#16072=CARTESIAN_POINT ( 'NONE',  ( 97.78191787992085438, -41.50032452247405246, 192.7041967044819728 ) ) ;
#16074=CARTESIAN_POINT ( 'NONE',  ( 97.81847858979224952, -40.53397798444700584, 146.6370489193171238 ) ) ;
#16075=CARTESIAN_POINT ( 'NONE',  ( 105.8001069787651716, -26.72395502425483826, 150.1776541679874128 ) ) ;
#16076=CARTESIAN_POINT ( 'NONE',  ( 188.5667039024479834, -65.37844715994100397, 173.2178068554149775 ) ) ;
#16079=CARTESIAN_POINT ( 'NONE',  ( 105.7137601602295121, -46.72359881362813638, 97.46889204442247490 ) ) ;
#16080=CARTESIAN_POINT ( 'NONE',  ( 113.7357275853186991, -44.67049210939298831, 148.1203871806729353 ) ) ;
#16081=ORIENTED_EDGE ( 'NONE', *, *, #67460, .T. ) ;
#16082=AXIS2_PLACEMENT_3D ( 'NONE', #38973, #26246, #39862 ) ;
#16083=ORIENTED_EDGE ( 'NONE', *, *, #66274, .T. ) ;
#16084=CARTESIAN_POINT ( 'NONE',  ( 115.1688055144990415, -30.74420868983300537, 105.7644404487539589 ) ) ;
#16085=DIRECTION ( 'NONE',  ( 0.000000000000000000, 0.000000000000000000, -1.000000000000000000 ) ) ;
#16086=CARTESIAN_POINT ( 'NONE',  ( 113.3831382903590566, -27.58002901871528323, 235.5956252759109759 ) ) ;
#16089=CARTESIAN_POINT ( 'NONE',  ( 98.34985026692173449, -31.65659937734086071, 111.9069137705935901 ) ) ;
#16090=B_SPLINE_CURVE_WITH_KNOTS ( 'NONE', 3,
 ( #72126, #9448, #36715, #58472, #3087, #37607, #65308, #30782, #2195, #38047, #24424, #52088, #79848, #45285, #73005, #1749, #84876, #43499 ),
 .UNSPECIFIED., .F., .F.,
 ( 4, 2, 2, 2, 2, 2, 2, 2, 4 ),
 ( 0.5000305911332758591, 0.5625267672416163212, 0.6250229433499568943, 0.6875191194582974674, 0.7500152955666379295, 0.8125114716749783916, 0.8750076477833189648, 0.9375038238916595379, 1.000000000000000000 ),
 .UNSPECIFIED. ) ;
#16091=EDGE_CURVE ( 'NONE', #30574, #56233, #50946, .T. ) ;
#16095=CARTESIAN_POINT ( 'NONE',  ( 98.10941331148539746, -42.08998169807674117, 161.7556252759109725 ) ) ;
#16096=EDGE_LOOP ( 'NONE', ( #5525, #58037, #7164, #78025 ) ) ;
#16097=VERTEX_POINT ( 'NONE', #44115 ) ;
#16098=ORIENTED_EDGE ( 'NONE', *, *, #86305, .F. ) ;
#16100=CARTESIAN_POINT ( 'NONE',  ( 62.03715912545739286, -47.82818131006020934, 180.4678068554151196 ) ) ;
#16102=CARTESIAN_POINT ( 'NONE',  ( 112.1377149357240341, -28.01188520256706482, 129.6566085857481596 ) ) ;
#16103=CARTESIAN_POINT ( 'NONE',  ( 97.81528920454944398, -40.52621084845757338, 102.6363811929704895 ) ) ;
#16104=CARTESIAN_POINT ( 'NONE',  ( 100.6247221172615127, -30.94977259965520844, 233.5747570362579495 ) ) ;
#16105=LINE ( 'NONE', #30615, #63991 ) ;
#16106=CARTESIAN_POINT ( 'NONE',  ( 114.9780134700875180, -29.01019993736734293, 194.4537205140059370 ) ) ;
#16107=DIRECTION ( 'NONE',  ( 0.7071067811865178188, 0.7071067811865773267, 7.071067811865170636E-16 ) ) ;
#16109=ORIENTED_EDGE ( 'NONE', *, *, #64099, .F. ) ;
#16112=CARTESIAN_POINT ( 'NONE',  ( 25.56670390244797275, -62.87844715994099687, 298.0928068554150627 ) ) ;
#16113=ORIENTED_EDGE ( 'NONE', *, *, #44683, .F. ) ;
#16114=ORIENTED_EDGE ( 'NONE', *, *, #9605, .F. ) ;
#16116=CARTESIAN_POINT ( 'NONE',  ( 50.97905606905900555, -31.62489322948711035, -5.074374724088000832 ) ) ;
#16117=VECTOR ( 'NONE', #89775, 1000.000000000000000 ) ;
#16118=CARTESIAN_POINT ( 'NONE',  ( 98.41530666024773666, -31.56922914487509502, 277.3301547344686355 ) ) ;
#16119=CARTESIAN_POINT ( 'NONE',  ( 116.7951251982872662, -39.38783008756426085, 273.6147919184925854 ) ) ;
#16122=CARTESIAN_POINT ( 'NONE',  ( 109.1587844380377277, -44.82492231645672121, 9.635625275910939536 ) ) ;
#16123=CARTESIAN_POINT ( 'NONE',  ( 41.56648329127499153, -36.32844715994070839, 318.9256252759120116 ) ) ;
#16126=CARTESIAN_POINT ( 'NONE',  ( 117.0527731729269476, -35.95361413649180093, 113.8882183681226081 ) ) ;
#16131=CARTESIAN_POINT ( 'NONE',  ( 107.5092159716399181, -46.42865411040452273, 42.03527697093395687 ) ) ;
#16132=CARTESIAN_POINT ( 'NONE',  ( 113.6284486023480724, -28.60005753680112761, 164.5356252759109736 ) ) ;
#16134=CARTESIAN_POINT ( 'NONE',  ( 116.8835868046513582, -40.17228670562625581, 133.5584824187679658 ) ) ;
#16135=( NAMED_UNIT ( * ) PLANE_ANGLE_UNIT ( ) SI_UNIT ( $, .RADIAN. ) );
#16136=CARTESIAN_POINT ( 'NONE',  ( 116.0551108448461264, -42.01026737563550029, 234.4041967044819899 ) ) ;
#16139=VERTEX_POINT ( 'NONE', #58641 ) ;
#16142=ORIENTED_EDGE ( 'NONE', *, *, #82831, .T. ) ;
#16145=EDGE_CURVE ( 'NONE', #84879, #26178, #22378, .T. ) ;
#16146=CARTESIAN_POINT ( 'NONE',  ( 101.4014481618761181, -46.27514046166531614, 207.1622919425779514 ) ) ;
#16148=CARTESIAN_POINT ( 'NONE',  ( 101.7694246217487972, -45.70876760617753831, 162.1527681330539679 ) ) ;
#16149=CARTESIAN_POINT ( 'NONE',  ( 99.09686023256277565, -30.54889700294794963, 255.8022268357593703 ) ) ;
#16151=CARTESIAN_POINT ( 'NONE',  ( 41.56648329127399677, 0.2215528400590013880, 198.9256252759119832 ) ) ;
#16153=CARTESIAN_POINT ( 'NONE',  ( 104.9367214363761889, -46.52192551884516547, 57.40585424230521028 ) ) ;
#16154=CARTESIAN_POINT ( 'NONE',  ( 116.1995025514323316, -41.78438384397597360, 259.4241967044825969 ) ) ;
#16155=DIRECTION ( 'NONE',  ( -0.000000000000000000, -0.000000000000000000, 1.000000000000000000 ) ) ;
#16157=CARTESIAN_POINT ( 'NONE',  ( 104.4871749466126545, -26.97957198089209641, 271.2812583532387407 ) ) ;
#16159=CARTESIAN_POINT ( 'NONE',  ( 117.0718954847100122, -35.46248235314624253, 259.9272919428255477 ) ) ;
#16162=CARTESIAN_POINT ( 'NONE',  ( 99.49891107524048550, -31.87110612240238439, 195.5838068554173219 ) ) ;
#16163=VERTEX_POINT ( 'NONE', #38213 ) ;
#16164=DIRECTION ( 'NONE',  ( 0.000000000000000000, -1.000000000000000000, 0.000000000000000000 ) ) ;
#16165=CARTESIAN_POINT ( 'NONE',  ( 117.9717084303226500, -34.78741065070708061, 198.9546728949589749 ) ) ;
#16166=CARTESIAN_POINT ( 'NONE',  ( 98.72253030179433608, -42.97932203522270100, 62.83848241876793850 ) ) ;
#16167=CARTESIAN_POINT ( 'NONE',  ( 114.8463700017591407, -29.67172957150665979, 205.4127681330539872 ) ) ;
#16168=CARTESIAN_POINT ( 'NONE',  ( 21.03715912545744615, -47.82818131006197149, 129.9678068554150627 ) ) ;
#16169=DIRECTION ( 'NONE',  ( -1.000000000000000000, -4.299999999999999979E-14, -1.000000000000000078E-15 ) ) ;
#16170=DIRECTION ( 'NONE',  ( 9.172741847159597097E-17, 0.1045284632676476005, -0.9945218953682739560 ) ) ;
#16171=CARTESIAN_POINT ( 'NONE',  ( 41.56648329127398966, -27.82844715994070484, 258.9256252759120116 ) ) ;
#16172=DIRECTION ( 'NONE',  ( 1.000000000000000000, 4.012088370409549976E-14, 0.000000000000000000 ) ) ;
#16173=LINE ( 'NONE', #71143, #49622 ) ;
#16176=EDGE_LOOP ( 'NONE', ( #88158, #64869, #57427, #48957 ) ) ;
#16178=EDGE_CURVE ( 'NONE', #58180, #15623, #24588, .T. ) ;
#16179=AXIS2_PLACEMENT_3D ( 'NONE', #697, #21154, #36121 ) ;
#16180=CARTESIAN_POINT ( 'NONE',  ( 115.3767887321059789, -38.82490071601502990, 123.0524198280769639 ) ) ;
#16181=DIRECTION ( 'NONE',  ( 0.000000000000000000, 0.000000000000000000, -1.000000000000000000 ) ) ;
#16182=ORIENTED_EDGE ( 'NONE', *, *, #14940, .T. ) ;
#16183=ADVANCED_FACE ( 'NONE', ( #8742 ), #15999, .F. ) ;
#16184=CARTESIAN_POINT ( 'NONE',  ( 96.04673288144557830, -37.20790665022158805, 112.3489586092449599 ) ) ;
#16185=FACE_OUTER_BOUND ( 'NONE', #81981, .T. ) ;
#16188=DIRECTION ( 'NONE',  ( 0.000000000000000000, 0.000000000000000000, -1.000000000000000000 ) ) ;
#16189=CARTESIAN_POINT ( 'NONE',  ( 115.8254323925114875, -31.73001883020303637, 175.2397919424540760 ) ) ;
#16190=EDGE_CURVE ( 'NONE', #50856, #27885, #88617, .T. ) ;
#16191=CARTESIAN_POINT ( 'NONE',  ( 99.61812512063040970, -43.94476044465314857, 41.95086337115000674 ) ) ;
#16192=ORIENTED_EDGE ( 'NONE', *, *, #71259, .T. ) ;
#16193=ORIENTED_EDGE ( 'NONE', *, *, #44119, .T. ) ;
#16195=CARTESIAN_POINT ( 'NONE',  ( 41.56648329127398966, -27.82844715994070484, 134.1756252759119832 ) ) ;
#16197=CARTESIAN_POINT ( 'NONE',  ( 116.3191307872214821, -32.94748812527954840, 115.1356252759109822 ) ) ;
#16201=EDGE_CURVE ( 'NONE', #69025, #20236, #60888, .T. ) ;
#16203=AXIS2_PLACEMENT_3D ( 'NONE', #86319, #71360, #24096 ) ;
#16205=CARTESIAN_POINT ( 'NONE',  ( 98.60777729073571152, -43.80857954853296121, 71.86895860924397539 ) ) ;
#16206=EDGE_LOOP ( 'NONE', ( #71656, #89570, #47362, #27556 ) ) ;
#16207=LINE ( 'NONE', #57067, #19994 ) ;
#16208=AXIS2_PLACEMENT_3D ( 'NONE', #68205, #41366, #75911 ) ;
#16210=CARTESIAN_POINT ( 'NONE',  ( 103.4072989863811074, -28.88653346237834185, 133.2299951314959685 ) ) ;
#16211=VECTOR ( 'NONE', #18901, 1000.000000000000000 ) ;
#16213=CARTESIAN_POINT ( 'NONE',  ( 73.06648329127402519, -46.72944715994106701, -4.824374724089063982 ) ) ;
#16214=ORIENTED_EDGE ( 'NONE', *, *, #15764, .T. ) ;
#16215=ORIENTED_EDGE ( 'NONE', *, *, #87928, .T. ) ;
#16220=CARTESIAN_POINT ( 'NONE',  ( 112.7482059764288778, -43.52991081625548020, 189.5615833058969883 ) ) ;
#16222=CARTESIAN_POINT ( 'NONE',  ( 101.4892552882362793, -27.89588691190665060, 106.5241967044819944 ) ) ;
#16223=EDGE_CURVE ( 'NONE', #34951, #89277, #87267, .T. ) ;
#16224=CARTESIAN_POINT ( 'NONE',  ( 116.3183510266638336, -32.94967450325654568, 119.1356252759109537 ) ) ;
#16226=CARTESIAN_POINT ( 'NONE',  ( 115.0850347510768330, -42.76005057245251351, 18.31318323247893076 ) ) ;
#16227=ORIENTED_EDGE ( 'NONE', *, *, #17770, .T. ) ;
#16228=ORIENTED_EDGE ( 'NONE', *, *, #61121, .F. ) ;
#16229=VERTEX_POINT ( 'NONE', #12301 ) ;
#16230=EDGE_CURVE ( 'NONE', #22054, #28950, #67144, .T. ) ;
#16232=CARTESIAN_POINT ( 'NONE',  ( 102.0328030160422230, -28.93470572416599751, 218.3509475124479593 ) ) ;
#16233=CARTESIAN_POINT ( 'NONE',  ( 96.31560519187928548, -41.77450771427546528, 61.67562527591097421 ) ) ;
#16235=CARTESIAN_POINT ( 'NONE',  ( 106.5192459994187715, -25.71289806663794408, 45.12800622829193742 ) ) ;
#16236=CARTESIAN_POINT ( 'NONE',  ( 106.4823958901525458, -24.86854109859944373, 191.1156252759109861 ) ) ;
#16237=CARTESIAN_POINT ( 'NONE',  ( 83.06670390244796920, -61.87844715994100397, 207.5838068554149913 ) ) ;
#16239=CARTESIAN_POINT ( 'NONE',  ( 102.3604841619309411, -46.03192315517718214, 123.2041967044829818 ) ) ;
#16240=CIRCLE ( 'NONE', #33669, 11.45913725231036118 ) ;
#16241=CARTESIAN_POINT ( 'NONE',  ( 182.5667039024480118, -32.29483332968450782, -5.074374724088000832 ) ) ;
#16245=CARTESIAN_POINT ( 'NONE',  ( 115.0378464896363795, -42.90772034720064454, 134.3033616519834368 ) ) ;
#16246=VERTEX_POINT ( 'NONE', #5035 ) ;
#16249=ADVANCED_FACE ( 'NONE', ( #52694 ), #26373, .F. ) ;
#16251=CARTESIAN_POINT ( 'NONE',  ( 107.2322097935746541, -25.67722466037449536, 80.07657765686299456 ) ) ;
#16252=DIRECTION ( 'NONE',  ( 0.000000000000000000, 0.000000000000000000, -1.000000000000000000 ) ) ;
#16253=DIRECTION ( 'NONE',  ( -0.9068632946707806397, 0.4214249218767882055, -9.068632946707802473E-16 ) ) ;
#16254=CARTESIAN_POINT ( 'NONE',  ( 106.6155744189988326, -25.27918481551454732, 323.5352776872487652 ) ) ;
#16255=CARTESIAN_POINT ( 'NONE',  ( 95.98894198207682393, -35.78073158428679790, 36.25848241876794731 ) ) ;
#16256=CARTESIAN_POINT ( 'NONE',  ( 115.8254209475894072, -31.72999086795746848, 109.2397943467912995 ) ) ;
#16257=CARTESIAN_POINT ( 'NONE',  ( 113.8292797163801851, -28.77778007523028947, 135.5156252759109634 ) ) ;
#16258=DIRECTION ( 'NONE',  ( -7.723290606088049820E-15, 0.000000000000000000, 1.000000000000000000 ) ) ;
#16260=VERTEX_POINT ( 'NONE', #12757 ) ;
#16261=DIRECTION ( 'NONE',  ( 1.387778780781444492E-15, 0.000000000000000000, -1.000000000000000000 ) ) ;
#16263=EDGE_LOOP ( 'NONE', ( #11068, #18857 ) ) ;
#16264=ADVANCED_FACE ( 'NONE', ( #39548 ), #54492, .T. ) ;
#16266=CARTESIAN_POINT ( 'NONE',  ( 103.8060002238608774, -48.17488501466909412, 217.3556252759109668 ) ) ;
#16269=CARTESIAN_POINT ( 'NONE',  ( 112.5006845157638651, -46.38111348219169372, 253.9965776568635647 ) ) ;
#16270=CARTESIAN_POINT ( 'NONE',  ( 111.0993040117788979, -25.53357873718133320, 95.80133956162495679 ) ) ;
#16273=DIRECTION ( 'NONE',  ( 1.000000000000000078E-15, 0.000000000000000000, -1.000000000000000000 ) ) ;
#16274=CARTESIAN_POINT ( 'NONE',  ( 116.7951252721859987, -39.38782978701362936, 78.61479194282316030 ) ) ;
#16276=VERTEX_POINT ( 'NONE', #80453 ) ;
#16277=ORIENTED_EDGE ( 'NONE', *, *, #29983, .T. ) ;
#16278=ORIENTED_EDGE ( 'NONE', *, *, #11144, .F. ) ;
#16279=DIRECTION ( 'NONE',  ( -1.000000000000000078E-15, 1.000000000000000083E-30, 1.000000000000000000 ) ) ;
#16280=CARTESIAN_POINT ( 'NONE',  ( 114.4150145978633049, -27.43247436093422920, 270.5441967044823741 ) ) ;
#16281=CARTESIAN_POINT ( 'NONE',  ( 107.0664832912739968, -36.72944715994100306, 312.6356252759112522 ) ) ;
#16282=CARTESIAN_POINT ( 'NONE',  ( 131.5094688080979495, -35.71735499139286674, 2.839545688279668578 ) ) ;
#16283=EDGE_CURVE ( 'NONE', #73924, #6162, #6222, .T. ) ;
#16284=AXIS2_PLACEMENT_3D ( 'NONE', #83016, #56624, #84368 ) ;
#16285=CARTESIAN_POINT ( 'NONE',  ( 51.06648329127400388, 12.92155284005902516, 330.1506252759110680 ) ) ;
#16287=DIRECTION ( 'NONE',  ( 1.346944695195362088E-15, -1.000000000000000000, 3.469446951953620425E-31 ) ) ;
#16288=CARTESIAN_POINT ( 'NONE',  ( 108.9266419529017327, -28.39302457734394736, 224.3238483995049819 ) ) ;
#16289=EDGE_LOOP ( 'NONE', ( #47531, #68337, #26250, #18840 ) ) ;
#16291=ORIENTED_EDGE ( 'NONE', *, *, #29682, .F. ) ;
#16292=EDGE_LOOP ( 'NONE', ( #37617, #27209, #62572, #45790 ) ) ;
#16295=CARTESIAN_POINT ( 'NONE',  ( 97.83899935994767816, -40.58357122989591659, 181.6413209514236371 ) ) ;
#16296=CARTESIAN_POINT ( 'NONE',  ( 105.7207279102414077, -46.41719084699259668, 253.4670538473389740 ) ) ;
#16297=VECTOR ( 'NONE', #25287, 1000.000000000000114 ) ;
#16298=LINE ( 'NONE', #43976, #35697 ) ;
#16299=EDGE_CURVE ( 'NONE', #58534, #74550, #59529, .T. ) ;
#16300=CARTESIAN_POINT ( 'NONE',  ( 108.9483104351207174, -46.92736419409149562, 123.7337205140059666 ) ) ;
#16302=AXIS2_PLACEMENT_3D ( 'NONE', #5995, #11904, #54542 ) ;
#16303=CARTESIAN_POINT ( 'NONE',  ( 116.8175521666927779, -34.15458112805423951, 29.03132320540886724 ) ) ;
#16304=VERTEX_POINT ( 'NONE', #68163 ) ;
#16306=CARTESIAN_POINT ( 'NONE',  ( 71.24189083761808661, -0.9290567490904538817, 542.9756252759101471 ) ) ;
#16309=CARTESIAN_POINT ( 'NONE',  ( 98.13886466857337609, -39.66030079267085995, 283.0225356868493805 ) ) ;
#16310=CARTESIAN_POINT ( 'NONE',  ( 25.56670390244832802, -48.82844715994168183, 254.7178068554150059 ) ) ;
#16311=FACE_OUTER_BOUND ( 'NONE', #24153, .T. ) ;
#16312=CYLINDRICAL_SURFACE ( 'NONE', #70639, 9.999999999999998224 ) ;
#16315=PLANE ( 'NONE',  #45503 ) ;
#16316=VECTOR ( 'NONE', #43965, 1000.000000000000000 ) ;
#16317=ORIENTED_EDGE ( 'NONE', *, *, #66487, .T. ) ;
#16318=CARTESIAN_POINT ( 'NONE',  ( 96.65640405957751113, -37.29272404675901242, 76.36991099019697060 ) ) ;
#16320=CARTESIAN_POINT ( 'NONE',  ( 113.4185696802295809, -42.43971249784851096, 37.66670554236295487 ) ) ;
#16321=CARTESIAN_POINT ( 'NONE',  ( 116.9299238147201692, -38.64270279391814711, 89.67301604876226406 ) ) ;
#16322=CARTESIAN_POINT ( 'NONE',  ( 115.4889021248300196, -33.97424487988631370, 85.51015473446898341 ) ) ;
#16326=CARTESIAN_POINT ( 'NONE',  ( 95.18190931754610062, -37.33608887137841492, 267.3670538473396618 ) ) ;
#16327=DIRECTION ( 'NONE',  ( 0.000000000000000000, 0.000000000000000000, 1.000000000000000000 ) ) ;
#16330=DIRECTION ( 'NONE',  ( -0.000000000000000000, 1.000000000000000000, 0.000000000000000000 ) ) ;
#16332=CARTESIAN_POINT ( 'NONE',  ( 98.82232569344716921, -30.27743405825323464, 151.7984824187679465 ) ) ;
#16333=CARTESIAN_POINT ( 'NONE',  ( 172.5664832912740110, -32.07844715994070839, 318.9256252759120116 ) ) ;
#16334=EDGE_LOOP ( 'NONE', ( #27733, #63292, #3365, #1032, #78598, #40445, #653, #39430 ) ) ;
#16336=EDGE_CURVE ( 'NONE', #40569, #9390, #56037, .T. ) ;
#16337=ORIENTED_EDGE ( 'NONE', *, *, #88097, .F. ) ;
#16338=CARTESIAN_POINT ( 'NONE',  ( 107.0664832912739968, -36.72944715994100306, 287.6356252759109680 ) ) ;
#16340=CARTESIAN_POINT ( 'NONE',  ( 96.80143343076635176, -35.25719154489700458, 226.2251490854349640 ) ) ;
#16341=DIRECTION ( 'NONE',  ( 0.000000000000000000, 2.135044278125299371E-15, -1.000000000000000000 ) ) ;
#16344=CARTESIAN_POINT ( 'NONE',  ( 115.4446095375818970, -42.99269977972175383, 24.31562527591096767 ) ) ;
#16345=VECTOR ( 'NONE', #50143, 1000.000000000000000 ) ;
#16347=ORIENTED_EDGE ( 'NONE', *, *, #4171, .F. ) ;
#16348=CARTESIAN_POINT ( 'NONE',  ( 106.5738132885318379, -26.72017395369831405, 171.1156838945207710 ) ) ;
#16349=DIRECTION ( 'NONE',  ( 0.000000000000000000, 0.000000000000000000, 1.000000000000000000 ) ) ;
#16351=CIRCLE ( 'NONE', #39546, 0.5000000000000079936 ) ;
#16352=CARTESIAN_POINT ( 'NONE',  ( 82.64938057483486489, -19.67376371870454932, 2.871651383883025321 ) ) ;
#16353=EDGE_CURVE ( 'NONE', #27831, #18963, #64247, .T. ) ;
#16355=CARTESIAN_POINT ( 'NONE',  ( 97.63514171170966449, -41.12017164899860688, 256.6727681330537507 ) ) ;
#16356=CARTESIAN_POINT ( 'NONE',  ( 48.16670390244647137, -26.71338133339281029, 193.9678068554150911 ) ) ;
#16357=EDGE_CURVE ( 'NONE', #63459, #27672, #12045, .T. ) ;
#16358=DIRECTION ( 'NONE',  ( -0.000000000000000000, 1.000000000000000000, 0.000000000000000000 ) ) ;
#16359=CARTESIAN_POINT ( 'NONE',  ( 83.06670390244806867, -51.22944715994108122, 207.5838068554169809 ) ) ;
#16360=CARTESIAN_POINT ( 'NONE',  ( 109.4373255760682611, -46.14484595950412427, 242.1952769709339464 ) ) ;
#16362=DIRECTION ( 'NONE',  ( 1.000000000000000000, 1.000000000000000078E-15, 1.000000000000000078E-15 ) ) ;
#16363=CARTESIAN_POINT ( 'NONE',  ( 115.0059970501926330, -43.50650750775896825, 59.26419670448196086 ) ) ;
#16365=CARTESIAN_POINT ( 'NONE',  ( 116.5734795788845020, -32.34496456428597355, 104.1699109901969535 ) ) ;
#16366=ORIENTED_EDGE ( 'NONE', *, *, #45145, .F. ) ;
#16368=ORIENTED_EDGE ( 'NONE', *, *, #47014, .F. ) ;
#16369=ADVANCED_FACE ( 'NONE', ( #80915 ), #86043, .F. ) ;
#16370=DIRECTION ( 'NONE',  ( -0.9254794337955620787, -0.3787978585227822492, 0.000000000000000000 ) ) ;
#16372=VERTEX_POINT ( 'NONE', #25931 ) ;
#16375=DIRECTION ( 'NONE',  ( 1.000000000000000078E-15, -1.000000000000000000, 0.000000000000000000 ) ) ;
#16376=ORIENTED_EDGE ( 'NONE', *, *, #11373, .F. ) ;
#16380=CYLINDRICAL_SURFACE ( 'NONE', #74223, 10.00000000000000711 ) ;
#16381=EDGE_CURVE ( 'NONE', #39961, #33407, #70402, .T. ) ;
#16382=EDGE_LOOP ( 'NONE', ( #40606, #30699 ) ) ;
#16383=CARTESIAN_POINT ( 'NONE',  ( 118.8678016624199358, -35.40170448615204890, 83.91562527591095488 ) ) ;
#16385=EDGE_CURVE ( 'NONE', #11556, #24002, #63130, .T. ) ;
#16386=CARTESIAN_POINT ( 'NONE',  ( 84.32545390244804651, -42.97311385574013087, 207.5838068554169809 ) ) ;
#16390=AXIS2_PLACEMENT_3D ( 'NONE', #2883, #78757, #85570 ) ;
#16391=EDGE_CURVE ( 'NONE', #48080, #51651, #22175, .T. ) ;
#16394=EDGE_CURVE ( 'NONE', #30630, #20434, #49703, .T. ) ;
#16395=CARTESIAN_POINT ( 'NONE',  ( 32.24491389930098251, -32.11662333284611748, -5.074374724088000832 ) ) ;
#16396=LINE ( 'NONE', #22771, #14604 ) ;
#16397=DIRECTION ( 'NONE',  ( -0.9254794337955620787, -0.3787978585227822492, 0.000000000000000000 ) ) ;
#16398=CARTESIAN_POINT ( 'NONE',  ( 179.1667039024460166, -26.71338133339251542, -5.074374724088000832 ) ) ;
#16399=ORIENTED_EDGE ( 'NONE', *, *, #18606, .F. ) ;
#16400=FACE_OUTER_BOUND ( 'NONE', #10058, .T. ) ;
#16401=CARTESIAN_POINT ( 'NONE',  ( 114.5468542906242391, -29.54732804739400365, 185.4232443235299570 ) ) ;
#16402=CARTESIAN_POINT ( 'NONE',  ( 95.60734603896362671, -36.72944715994100306, 292.6356252759106837 ) ) ;
#16403=EDGE_LOOP ( 'NONE', ( #54477, #13493, #21274, #67542 ) ) ;
#16405=CARTESIAN_POINT ( 'NONE',  ( 97.69287098190334007, -33.93680905855630670, 27.09562527591097236 ) ) ;
#16406=LINE ( 'NONE', #65441, #48308 ) ;
#16407=CARTESIAN_POINT ( 'NONE',  ( 20.03715912545735378, -24.42818131006189830, 249.9678068554150059 ) ) ;
#16408=DIRECTION ( 'NONE',  ( 1.000000000000000000, 3.987088437185090195E-11, 0.000000000000000000 ) ) ;
#16410=CARTESIAN_POINT ( 'NONE',  ( 115.8262887155365632, -31.73150010602303439, 29.23988951266790082 ) ) ;
#16411=EDGE_CURVE ( 'NONE', #45509, #40177, #42664, .T. ) ;
#16412=CARTESIAN_POINT ( 'NONE',  ( 107.2379402074490429, -25.61267671046441308, 230.0641967044829812 ) ) ;
#16413=ORIENTED_EDGE ( 'NONE', *, *, #51953, .F. ) ;
#16415=CARTESIAN_POINT ( 'NONE',  ( 104.0709181822855243, -28.35754658334662182, 186.7815833058969872 ) ) ;
#16418=CARTESIAN_POINT ( 'NONE',  ( 105.6677623720644306, -45.47998190943052066, 33.88158330589596545 ) ) ;
#16420=CIRCLE ( 'NONE', #81721, 1.000000000000000888 ) ;
#16421=AXIS2_PLACEMENT_3D ( 'NONE', #39149, #87311, #32323 ) ;
#16422=CARTESIAN_POINT ( 'NONE',  ( 116.3212776292269552, -32.94146857470667555, 79.13562527591095375 ) ) ;
#16423=CARTESIAN_POINT ( 'NONE',  ( 131.0667039024480118, -58.35344715994099829, 207.5838068554149913 ) ) ;
#16426=CARTESIAN_POINT ( 'NONE',  ( 131.0667039024480403, -42.97311385573999587, 207.5838068554170377 ) ) ;
#16427=CARTESIAN_POINT ( 'NONE',  ( 117.3134009501235795, -34.93240959161192194, 243.9641967044819637 ) ) ;
#16429=ORIENTED_EDGE ( 'NONE', *, *, #43175, .T. ) ;
#16431=CARTESIAN_POINT ( 'NONE',  ( 149.4512091874903206, -60.54365471797113685, 394.9756252759100903 ) ) ;
#16432=DIRECTION ( 'NONE',  ( -0.9834602067153815907, -0.1811243269341220596, 0.000000000000000000 ) ) ;
#16433=CARTESIAN_POINT ( 'NONE',  ( 36.74138383868164226, -48.33240602328862678, 300.4678068554150059 ) ) ;
#16434=CARTESIAN_POINT ( 'NONE',  ( 113.6564618781686136, -45.68400828401183844, 29.08133956162495082 ) ) ;
#16436=ORIENTED_EDGE ( 'NONE', *, *, #28710, .T. ) ;
#16437=CARTESIAN_POINT ( 'NONE',  ( 105.9839165226978110, -26.31690525417204540, 46.15848241876796720 ) ) ;
#16438=CARTESIAN_POINT ( 'NONE',  ( 130.5667039024479834, -33.42944715994100591, 239.5838068554162987 ) ) ;
#16439=VECTOR ( 'NONE', #25190, 1000.000000000000000 ) ;
#16440=CARTESIAN_POINT ( 'NONE',  ( 112.2083724274664291, -26.91728527761779333, 14.68038718067299442 ) ) ;
#16441=ORIENTED_EDGE ( 'NONE', *, *, #49686, .T. ) ;
#16445=CARTESIAN_POINT ( 'NONE',  ( 75.31670390244798341, -67.87844715994100397, 86.31780685541500020 ) ) ;
#16446=CARTESIAN_POINT ( 'NONE',  ( 103.5365535965830475, -29.36946602085958702, 93.25094751244894553 ) ) ;
#16447=CARTESIAN_POINT ( 'NONE',  ( 117.9712535577395869, -34.78749165583555225, 194.9546728949589749 ) ) ;
#16448=FACE_OUTER_BOUND ( 'NONE', #45875, .T. ) ;
#16449=ORIENTED_EDGE ( 'NONE', *, *, #32258, .T. ) ;
#16451=EDGE_LOOP ( 'NONE', ( #47586, #22505, #29842, #439 ) ) ;
#16454=CARTESIAN_POINT ( 'NONE',  ( 134.0664832912740110, -41.22944715994101017, -0.5743747240890021422 ) ) ;
#16455=ORIENTED_EDGE ( 'NONE', *, *, #84615, .F. ) ;
#16456=EDGE_LOOP ( 'NONE', ( #5722, #86819, #87283, #17706 ) ) ;
#16458=EDGE_CURVE ( 'NONE', #53148, #35758, #40886, .T. ) ;
#16460=CARTESIAN_POINT ( 'NONE',  ( 97.31302290375664654, -38.96038935385655577, 42.50539279665081693 ) ) ;
#16461=CARTESIAN_POINT ( 'NONE',  ( 115.1266331755855958, -39.55612640683342107, 132.9809912566479397 ) ) ;
#16462=CARTESIAN_POINT ( 'NONE',  ( 101.2817000042767148, -26.35783695576231267, 255.4813395616251626 ) ) ;
#16465=ORIENTED_EDGE ( 'NONE', *, *, #8287, .T. ) ;
#16467=ADVANCED_FACE ( 'NONE', ( #84945 ), #64039, .F. ) ;
#16468=DIRECTION ( 'NONE',  ( 1.000000000000000078E-15, -1.000000000000000083E-30, -1.000000000000000000 ) ) ;
#16469=ORIENTED_EDGE ( 'NONE', *, *, #63270, .F. ) ;
#16470=DIRECTION ( 'NONE',  ( 0.000000000000000000, 1.000000000000000000, 0.000000000000000000 ) ) ;
#16471=LINE ( 'NONE', #45045, #11031 ) ;
#16472=CARTESIAN_POINT ( 'NONE',  ( 97.86672365782918348, -40.64956839743646100, 131.6470187837300330 ) ) ;
#16473=EDGE_CURVE ( 'NONE', #2012, #82307, #64479, .T. ) ;
#16475=CARTESIAN_POINT ( 'NONE',  ( 131.0667039024480971, -58.72944715994092491, 207.5838068554170377 ) ) ;
#16476=ORIENTED_EDGE ( 'NONE', *, *, #23576, .F. ) ;
#16477=CARTESIAN_POINT ( 'NONE',  ( 96.26778515314977369, -34.36995442310919202, 256.1432443235300980 ) ) ;
#16478=CARTESIAN_POINT ( 'NONE',  ( 96.61551125061282619, -32.99117460050268846, 22.06514908543494258 ) ) ;
#16480=AXIS2_PLACEMENT_3D ( 'NONE', #44032, #64504, #78153 ) ;
#16481=B_SPLINE_CURVE_WITH_KNOTS ( 'NONE', 3,
 ( #49402, #16256, #21270, #85314, #55752, #48943, #42581, #71669, #8998, #77581, #35331, #7642, #70316, #37143, #50761, #56671, #70773, #57113, #63043, #825, #50301, #14465, #83959, #76685, #78041, #84415, #42142, #71226, #21730, #77138 ),
 .UNSPECIFIED., .F., .F.,
 ( 4, 2, 2, 2, 2, 2, 2, 2, 2, 2, 1, 1, 1, 1, 1, 1, 2, 4 ),
 ( 0.000000000000000000, 0.06250190528924848277, 0.1250038105784969655, 0.1875057158677454483, 0.2500076211569939311, 0.3125095264462424138, 0.3750114317354908966, 0.4375133370247393794, 0.4687642896693638428, 0.4843897659916759912, 0.4922025041528320100, 0.4961088732334101858, 0.4980620577736992183, 0.4990386500438436235, 0.4995269461789159093, 0.4997710942464516637, 0.4998931682802195686, 0.5000152423139874180 ),
 .UNSPECIFIED. ) ;
#16482=CARTESIAN_POINT ( 'NONE',  ( 130.5667039024480118, -39.24694715994083793, 219.5838068554170093 ) ) ;
#16483=ADVANCED_FACE ( 'NONE', ( #8634 ), #1816, .T. ) ;
#16484=DIRECTION ( 'NONE',  ( -0.9963424814100680926, 0.08544974978095698503, 0.000000000000000000 ) ) ;
#16488=CARTESIAN_POINT ( 'NONE',  ( 131.4905132191207997, -37.69637952317774676, 6.988870342676155367 ) ) ;
#16489=LINE ( 'NONE', #44168, #80752 ) ;
#16490=CARTESIAN_POINT ( 'NONE',  ( 109.6433924709448888, -46.47999098159603903, 162.7813146523185424 ) ) ;
#16491=ADVANCED_FACE ( 'NONE', ( #22262 ), #44909, .F. ) ;
#16492=DIRECTION ( 'NONE',  ( 1.000000000000000000, 4.299999999999999979E-14, 1.000000000000000078E-15 ) ) ;
#16494=CARTESIAN_POINT ( 'NONE',  ( 97.06250871634010480, -39.81605817309107920, 21.56419670448195092 ) ) ;
#16495=CARTESIAN_POINT ( 'NONE',  ( 96.74313874428034410, -35.27650366090898615, 177.2156252759109805 ) ) ;
#16496=CARTESIAN_POINT ( 'NONE',  ( 101.5975885682485398, -47.27054607199826819, 13.19562527591094891 ) ) ;
#16497=CARTESIAN_POINT ( 'NONE',  ( 97.81167943543778165, -40.51737693692245301, 166.6360185166829808 ) ) ;
#16498=LINE ( 'NONE', #71913, #12274 ) ;
#16499=CARTESIAN_POINT ( 'NONE',  ( 82.73250004807572111, -36.03188439719672687, 2.979900720421668758 ) ) ;
#16501=CIRCLE ( 'NONE', #70180, 2.517500000000005844 ) ;
#16502=ORIENTED_EDGE ( 'NONE', *, *, #29490, .T. ) ;
#16504=VERTEX_POINT ( 'NONE', #9078 ) ;
#16505=CARTESIAN_POINT ( 'NONE',  ( 116.4365193811696457, -32.28633913640747011, 60.19086337114898555 ) ) ;
#16507=ORIENTED_EDGE ( 'NONE', *, *, #66609, .F. ) ;
#16508=AXIS2_PLACEMENT_3D ( 'NONE', #9822, #16637, #23905 ) ;
#16509=CARTESIAN_POINT ( 'NONE',  ( 116.8173832505959666, -34.15392672464852808, 50.03137649336521520 ) ) ;
#16510=CARTESIAN_POINT ( 'NONE',  ( 96.07698540226633099, -35.78353028925530310, 182.2461014663869889 ) ) ;
#16511=CARTESIAN_POINT ( 'NONE',  ( 184.5667039024480118, -67.87844715994100397, 20.91780685541479912 ) ) ;
#16512=CARTESIAN_POINT ( 'NONE',  ( 97.82529570206294522, -40.55052488149144096, 146.6384733909613090 ) ) ;
#16513=CARTESIAN_POINT ( 'NONE',  ( 126.0667039024479266, -14.72944715994094977, 239.5838068554170377 ) ) ;
#16516=CARTESIAN_POINT ( 'NONE',  ( 63.06670390244794078, -40.32844715994017548, 300.4678068554150627 ) ) ;
#16517=CARTESIAN_POINT ( 'NONE',  ( 116.9402674190077391, -38.58240887119603713, 98.67907853902740101 ) ) ;
#16519=CARTESIAN_POINT ( 'NONE',  ( 108.2018929880948832, -26.98138995270364759, 129.9841967044829687 ) ) ;
#16521=ORIENTED_EDGE ( 'NONE', *, *, #65904, .F. ) ;
#16523=CARTESIAN_POINT ( 'NONE',  ( 103.5852769812406535, -44.87864842379759978, 88.68729759161098514 ) ) ;
#16525=CARTESIAN_POINT ( 'NONE',  ( 99.57924082623978279, -30.38476633542330774, 211.7670538473389570 ) ) ;
#16526=DIRECTION ( 'NONE',  ( -4.237773401492740281E-14, 1.000000000000000000, 0.000000000000000000 ) ) ;
#16529=LINE ( 'NONE', #31039, #33027 ) ;
#16532=CARTESIAN_POINT ( 'NONE',  ( 108.8451227504523331, -46.97957433935484772, 167.7127681330539701 ) ) ;
#16534=ORIENTED_EDGE ( 'NONE', *, *, #78333, .T. ) ;
#16535=EDGE_CURVE ( 'NONE', #86596, #22588, #44460, .T. ) ;
#16537=CARTESIAN_POINT ( 'NONE',  ( 77.50946880809777895, -17.71735499139141723, 2.839545688279708546 ) ) ;
#16538=DIRECTION ( 'NONE',  ( 4.299999999999999979E-14, -1.000000000000000000, 4.400000000000000367E-29 ) ) ;
#16540=CARTESIAN_POINT ( 'NONE',  ( 112.3381529121750191, -29.09364788469061480, 237.4138046553059951 ) ) ;
#16541=EDGE_CURVE ( 'NONE', #4843, #47987, #48395, .T. ) ;
#16542=FACE_OUTER_BOUND ( 'NONE', #36307, .T. ) ;
#16543=( BOUNDED_CURVE ( )  B_SPLINE_CURVE ( 3, ( #62640, #414, #28106, #55789 ),
 .UNSPECIFIED., .F., .T. ) 
 B_SPLINE_CURVE_WITH_KNOTS ( ( 4, 4 ),
 ( 4.712388980381146730, 6.283185307176318624 ),
 .UNSPECIFIED. ) 
 CURVE ( )  GEOMETRIC_REPRESENTATION_ITEM ( )  RATIONAL_B_SPLINE_CURVE ( ( 1.000000000000000000, 0.8047378541235299387, 0.8047378541235299387, 1.000000000000000000 ) ) 
 REPRESENTATION_ITEM ( '' )  );
#16544=AXIS2_PLACEMENT_3D ( 'NONE', #74551, #25962, #5065 ) ;
#16545=CARTESIAN_POINT ( 'NONE',  ( 107.6545119506432258, -47.76725988480858121, 197.6308633711489620 ) ) ;
#16546=LINE ( 'NONE', #1127, #40199 ) ;
#16547=VERTEX_POINT ( 'NONE', #59869 ) ;
#16549=EDGE_LOOP ( 'NONE', ( #71824, #71644, #19254, #24499 ) ) ;
#16550=CARTESIAN_POINT ( 'NONE',  ( 97.85750890579558359, -40.62776002508964268, 62.64559988044219807 ) ) ;
#16551=EDGE_LOOP ( 'NONE', ( #56364, #60554 ) ) ;
#16553=CARTESIAN_POINT ( 'NONE',  ( 131.8552587341498281, -35.08426237659745084, 7.378668740724780406 ) ) ;
#16554=CARTESIAN_POINT ( 'NONE',  ( 98.13886466857337609, -39.66030079267085995, 283.0225356868493805 ) ) ;
#16555=CARTESIAN_POINT ( 'NONE',  ( 83.06670390244796920, -61.87844715994100397, 237.1838068554150141 ) ) ;
#16556=ORIENTED_EDGE ( 'NONE', *, *, #60221, .T. ) ;
#16557=CARTESIAN_POINT ( 'NONE',  ( 114.2248125149048263, -42.04901104171000270, 9.635625275910941312 ) ) ;
#16558=ADVANCED_FACE ( 'NONE', ( #79914 ), #32376, .F. ) ;
#16560=VERTEX_POINT ( 'NONE', #18550 ) ;
#16561=VERTEX_POINT ( 'NONE', #39878 ) ;
#16562=AXIS2_PLACEMENT_3D ( 'NONE', #329, #20778, #82581 ) ;
#16563=CARTESIAN_POINT ( 'NONE',  ( 111.2307140782278765, -45.82263013567369825, 112.9182118773837118 ) ) ;
#16568=EDGE_CURVE ( 'NONE', #79504, #63431, #35296, .T. ) ;
#16569=ADVANCED_FACE ( 'NONE', ( #26262 ), #32619, .F. ) ;
#16570=CARTESIAN_POINT ( 'NONE',  ( 98.90470121413369498, -39.24767091914073802, 20.98670554236298358 ) ) ;
#16572=CARTESIAN_POINT ( 'NONE',  ( 102.9583934913338652, -26.44260899983745006, 175.3908633711489813 ) ) ;
#16574=CARTESIAN_POINT ( 'NONE',  ( 108.6454077996538530, -25.81962716842089378, 149.9737205140059473 ) ) ;
#16575=CARTESIAN_POINT ( 'NONE',  ( 25.56670390244797275, -48.82844715994099971, 259.9678068554150059 ) ) ;
#16576=CARTESIAN_POINT ( 'NONE',  ( 106.1383564330493812, -47.74364531592736682, 258.4975300378158636 ) ) ;
#16577=CARTESIAN_POINT ( 'NONE',  ( 59.68306514483415270, -72.55903866283681225, 542.9756252759101471 ) ) ;
#16578=CARTESIAN_POINT ( 'NONE',  ( 108.4156033759623909, -26.73479662881522856, 125.9691087597593082 ) ) ;
#16580=VERTEX_POINT ( 'NONE', #34412 ) ;
#16583=EDGE_CURVE ( 'NONE', #72917, #31310, #89853, .T. ) ;
#16584=CARTESIAN_POINT ( 'NONE',  ( 101.9629764938643035, -45.91127772325894085, 187.1727681330539781 ) ) ;
#16586=CARTESIAN_POINT ( 'NONE',  ( 117.4575111195971857, -40.49848259682686802, 173.5375300378159693 ) ) ;
#16587=CARTESIAN_POINT ( 'NONE',  ( 104.4889533838567104, -26.97908276470762701, 265.2814877645184879 ) ) ;
#16590=CARTESIAN_POINT ( 'NONE',  ( 97.99254151483945918, -40.00862495256633622, 277.6356252759111385 ) ) ;
#16592=CARTESIAN_POINT ( 'NONE',  ( 98.07879728544668296, -32.87107120142745487, 12.00419670448193976 ) ) ;
#16593=DIRECTION ( 'NONE',  ( 0.000000000000000000, 1.000000000000000000, 0.000000000000000000 ) ) ;
#16594=LINE ( 'NONE', #44273, #88850 ) ;
#16595=EDGE_CURVE ( 'NONE', #8519, #7620, #43986, .T. ) ;
#16596=CARTESIAN_POINT ( 'NONE',  ( 179.4595971212889651, -28.98061976758942748, 342.9256252759109884 ) ) ;
#16598=LINE ( 'NONE', #49755, #32872 ) ;
#16599=DIRECTION ( 'NONE',  ( 2.127927463864879951E-15, 1.848892746611749922E-31, 1.000000000000000000 ) ) ;
#16600=CARTESIAN_POINT ( 'NONE',  ( 111.4101316090540479, -43.50011782763849055, 195.5838068554169809 ) ) ;
#16601=VERTEX_POINT ( 'NONE', #34863 ) ;
#16602=FACE_OUTER_BOUND ( 'NONE', #19699, .T. ) ;
#16603=CARTESIAN_POINT ( 'NONE',  ( 98.24258143063333648, -42.32275744278853580, 186.7756252759109543 ) ) ;
#16604=CARTESIAN_POINT ( 'NONE',  ( 106.8411897839350786, -48.57781660025092663, 73.56133956162497611 ) ) ;
#16605=CARTESIAN_POINT ( 'NONE',  ( 96.00064313654479520, -35.86649870909684523, 187.2765776568629406 ) ) ;
#16607=DIRECTION ( 'NONE',  ( 1.000000000000000078E-15, -1.000000000000000083E-30, -1.000000000000000000 ) ) ;
#16608=DIRECTION ( 'NONE',  ( -4.237773401492740281E-14, 1.000000000000000000, 0.000000000000000000 ) ) ;
#16610=LINE ( 'NONE', #72026, #30579 ) ;
#16611=CARTESIAN_POINT ( 'NONE',  ( 46.48091746482130304, -49.32844715994084339, 300.4678068554150059 ) ) ;
#16612=ORIENTED_EDGE ( 'NONE', *, *, #62941, .T. ) ;
#16613=AXIS2_PLACEMENT_3D ( 'NONE', #19605, #83195, #63181 ) ;
#16618=CARTESIAN_POINT ( 'NONE',  ( 108.8595479556035599, -45.11020018309576329, 107.1667055423619672 ) ) ;
#16619=DIRECTION ( 'NONE',  ( 0.7071067811865473507, 0.000000000000000000, -0.7071067811865476838 ) ) ;
#16620=ORIENTED_EDGE ( 'NONE', *, *, #78011, .F. ) ;
#16621=CARTESIAN_POINT ( 'NONE',  ( 113.3292761056178648, -27.64973082387879444, 85.60800622829195561 ) ) ;
#16622=CYLINDRICAL_SURFACE ( 'NONE', #68642, 2.517499999999998739 ) ;
#16623=CARTESIAN_POINT ( 'NONE',  ( 48.45959712129000252, -28.98061976758940617, -5.074374724088000832 ) ) ;
#16626=CARTESIAN_POINT ( 'NONE',  ( 109.4837483930865574, -46.20680252518646114, 47.77562527591094721 ) ) ;
#16627=ORIENTED_EDGE ( 'NONE', *, *, #35363, .T. ) ;
#16629=ORIENTED_EDGE ( 'NONE', *, *, #2128, .F. ) ;
#16630=VECTOR ( 'NONE', #6669, 1000.000000000000000 ) ;
#16631=AXIS2_PLACEMENT_3D ( 'NONE', #46404, #33697, #13259 ) ;
#16632=DIRECTION ( 'NONE',  ( -0.7071067812163244204, 0.7071067811567707251, -7.071067812163251589E-16 ) ) ;
#16633=VECTOR ( 'NONE', #11708, 1000.000000000000114 ) ;
#16635=CARTESIAN_POINT ( 'NONE',  ( 100.9546728166709215, -28.70702572326774416, 116.5939586087175286 ) ) ;
#16636=AXIS2_PLACEMENT_3D ( 'NONE', #18811, #27408, #69204 ) ;
#16637=DIRECTION ( 'NONE',  ( -0.7071067811866279529, 0.7071067811864671926, -7.071067811866286874E-16 ) ) ;
#16638=CARTESIAN_POINT ( 'NONE',  ( 30.48091746481746611, -48.32844715994156815, 129.9678068554150627 ) ) ;
#16641=DIRECTION ( 'NONE',  ( 1.000000000000000078E-15, -1.000000000000000083E-30, -1.000000000000000000 ) ) ;
#16642=AXIS2_PLACEMENT_3D ( 'NONE', #13272, #81439, #68683 ) ;
#16644=CARTESIAN_POINT ( 'NONE',  ( 96.36089708107958529, -41.75325360632975702, 61.67562527591097421 ) ) ;
#16648=CARTESIAN_POINT ( 'NONE',  ( 110.7682021097048306, -28.22102727396991284, 132.5680903695919710 ) ) ;
#16651=CARTESIAN_POINT ( 'NONE',  ( 36.74138383868164226, -48.33240602328862678, 300.4678068554150059 ) ) ;
#16652=FACE_OUTER_BOUND ( 'NONE', #39322, .T. ) ;
#16653=ORIENTED_EDGE ( 'NONE', *, *, #14489, .F. ) ;
#16654=VERTEX_POINT ( 'NONE', #61658 ) ;
#16655=DIRECTION ( 'NONE',  ( 0.000000000000000000, 0.000000000000000000, 1.000000000000000000 ) ) ;
#16656=ORIENTED_EDGE ( 'NONE', *, *, #74199, .T. ) ;
#16658=CARTESIAN_POINT ( 'NONE',  ( 98.29135092237498839, -35.49440443996801520, 177.6472975916109647 ) ) ;
#16660=CARTESIAN_POINT ( 'NONE',  ( 96.64920772548965999, -35.94453432339758336, 142.2670538473399517 ) ) ;
#16662=AXIS2_PLACEMENT_3D ( 'NONE', #44292, #2547, #65206 ) ;
#16663=CARTESIAN_POINT ( 'NONE',  ( 97.81170008160388818, -40.51743097690945916, 72.63551179937353197 ) ) ;
#16664=VERTEX_POINT ( 'NONE', #76200 ) ;
#16665=VECTOR ( 'NONE', #69323, 1000.000000000000000 ) ;
#16667=ORIENTED_EDGE ( 'NONE', *, *, #53549, .T. ) ;
#16669=CARTESIAN_POINT ( 'NONE',  ( 98.55143180905920985, -33.04300857791147195, 208.8195189410199646 ) ) ;
#16670=CARTESIAN_POINT ( 'NONE',  ( 115.2246207261642894, -44.22212590188486558, 78.22324432352995416 ) ) ;
#16673=CARTESIAN_POINT ( 'NONE',  ( 118.1852327621007532, -40.75705396371412803, 23.54991099019593292 ) ) ;
#16674=CARTESIAN_POINT ( 'NONE',  ( 117.0725227226916587, -35.46769152344445786, 253.9273137617209954 ) ) ;
#16675=DIRECTION ( 'NONE',  ( 1.000000000000000000, 8.673617379883546378E-16, 9.757819552368989676E-16 ) ) ;
#16676=CARTESIAN_POINT ( 'NONE',  ( 112.8675307907708287, -28.58609239232746546, 195.5838076129389833 ) ) ;
#16677=ADVANCED_FACE ( 'NONE', ( #54833 ), #41215, .F. ) ;
#16678=CARTESIAN_POINT ( 'NONE',  ( 108.7432144037193922, -25.80414517310806488, 140.9432443235299672 ) ) ;
#16679=LINE ( 'NONE', #16241, #26266 ) ;
#16680=ORIENTED_EDGE ( 'NONE', *, *, #6399, .T. ) ;
#16681=CARTESIAN_POINT ( 'NONE',  ( 64.68306507141299733, -72.55818180160879649, 394.9756252759101471 ) ) ;
#16682=EDGE_CURVE ( 'NONE', #70782, #11886, #38170, .T. ) ;
#16684=CARTESIAN_POINT ( 'NONE',  ( 107.0667039024479834, -36.72944715994099596, 239.5838068554170093 ) ) ;
#16685=VERTEX_POINT ( 'NONE', #7615 ) ;
#16687=CIRCLE ( 'NONE', #8007, 2.116999999999993776 ) ;
#16689=TOROIDAL_SURFACE ( 'NONE', #15279, 13.50000000000000000, 0.5000000000000000000 ) ;
#16691=CARTESIAN_POINT ( 'NONE',  ( 75.31670390244798341, -67.87844715994100397, 88.43480685541499042 ) ) ;
#16692=CARTESIAN_POINT ( 'NONE',  ( 112.7417948769132039, -27.24419935825454431, 54.65943479971996055 ) ) ;
#16695=DIRECTION ( 'NONE',  ( 0.000000000000000000, 0.000000000000000000, 1.000000000000000000 ) ) ;
#16696=CARTESIAN_POINT ( 'NONE',  ( 116.8171228663217533, -34.15291832013626561, 75.03145860928886179 ) ) ;
#16697=CARTESIAN_POINT ( 'NONE',  ( 107.5734549334945456, -47.83597508069291138, 42.61276813305398292 ) ) ;
#16698=DIRECTION ( 'NONE',  ( 0.000000000000000000, 0.000000000000000000, -1.000000000000000000 ) ) ;
#16699=CARTESIAN_POINT ( 'NONE',  ( 114.5119312840559473, -28.59475203354334027, 150.4746728949579619 ) ) ;
#16700=CARTESIAN_POINT ( 'NONE',  ( 63.03715912545646205, -24.89890238295017255, 129.9678068554150911 ) ) ;
#16704=PLANE ( 'NONE',  #43953 ) ;
#16705=AXIS2_PLACEMENT_3D ( 'NONE', #1194, #1652, #7561 ) ;
#16708=DIRECTION ( 'NONE',  ( -0.000000000000000000, 1.000000000000000000, 0.000000000000000000 ) ) ;
#16710=CARTESIAN_POINT ( 'NONE',  ( 98.39836552415940218, -29.79571670633027836, 195.7775300378159784 ) ) ;
#16713=CARTESIAN_POINT ( 'NONE',  ( 96.78746529907793672, -40.85582509469530521, 247.6422919425769749 ) ) ;
#16714=CARTESIAN_POINT ( 'NONE',  ( 98.82360578189442890, -43.24043672769812474, 87.85848241876792031 ) ) ;
#16715=DIRECTION ( 'NONE',  ( -1.000000000000000078E-15, 1.000000000000000083E-30, 1.000000000000000000 ) ) ;
#16716=CARTESIAN_POINT ( 'NONE',  ( 87.06648329127401098, -46.72944715994105280, 14.67562527591094934 ) ) ;
#16718=DIRECTION ( 'NONE',  ( 1.387778780781444492E-15, 0.000000000000000000, -1.000000000000000000 ) ) ;
#16719=EDGE_LOOP ( 'NONE', ( #76085, #35168, #71841, #32705, #70531, #45877 ) ) ;
#16720=CIRCLE ( 'NONE', #21123, 5.035202529042187791 ) ;
#16721=ORIENTED_EDGE ( 'NONE', *, *, #53914, .F. ) ;
#16722=EDGE_LOOP ( 'NONE', ( #69601, #8350 ) ) ;
#16723=ORIENTED_EDGE ( 'NONE', *, *, #33251, .T. ) ;
#16724=CARTESIAN_POINT ( 'NONE',  ( 126.0667039024479266, -14.72944715994094977, 239.5838068554170377 ) ) ;
#16725=CARTESIAN_POINT ( 'NONE',  ( 100.2472489666992743, -45.42841400796814355, 273.0594347997205773 ) ) ;
#16726=DIRECTION ( 'NONE',  ( -1.000000000000000078E-15, 1.000000000000000083E-30, 1.000000000000000000 ) ) ;
#16727=CARTESIAN_POINT ( 'NONE',  ( 33.92127028473601769, -29.73316016639540749, -5.074374724088000832 ) ) ;
#16728=DIRECTION ( 'NONE',  ( 0.9068632946707807507, -0.4214249218767880945, 9.080193194566099635E-16 ) ) ;
#16729=PLANE ( 'NONE',  #3653 ) ;
#16732=CARTESIAN_POINT ( 'NONE',  ( 103.1098180292659947, -44.29918505015107399, 211.6152769709339623 ) ) ;
#16734=ORIENTED_EDGE ( 'NONE', *, *, #5625, .F. ) ;
#16737=CARTESIAN_POINT ( 'NONE',  ( 142.8838050580815775, -82.11588141944041297, 542.9756252759101471 ) ) ;
#16738=VECTOR ( 'NONE', #73565, 999.9999999999998863 ) ;
#16740=EDGE_CURVE ( 'NONE', #13307, #17048, #75909, .T. ) ;
#16741=CARTESIAN_POINT ( 'NONE',  ( 115.1244435615320612, -31.12738976831575144, 275.3099109901961015 ) ) ;
#16743=LINE ( 'NONE', #8249, #37544 ) ;
#16744=CARTESIAN_POINT ( 'NONE',  ( 113.1774560752732839, -44.75249464381799669, 28.09387619456539653 ) ) ;
#16745=ORIENTED_EDGE ( 'NONE', *, *, #1368, .F. ) ;
#16747=ORIENTED_EDGE ( 'NONE', *, *, #40872, .F. ) ;
#16748=DIRECTION ( 'NONE',  ( -0.7071067811865779928, 0.7071067811865171526, -2.899137802864836037E-29 ) ) ;
#16749=CARTESIAN_POINT ( 'NONE',  ( 101.3472728536945198, -42.59232338312836674, 19.77951894102097796 ) ) ;
#16750=AXIS2_PLACEMENT_3D ( 'NONE', #49901, #22229, #77631 ) ;
#16751=EDGE_CURVE ( 'NONE', #37281, #78352, #25210, .T. ) ;
#16752=AXIS2_PLACEMENT_3D ( 'NONE', #17402, #4661, #11019 ) ;
#16753=VECTOR ( 'NONE', #2451, 1000.000000000000000 ) ;
#16754=CARTESIAN_POINT ( 'NONE',  ( 38.69148329127400388, 12.92155284005802685, 335.5992267699910485 ) ) ;
#16755=CIRCLE ( 'NONE', #12405, 2.517500000000005844 ) ;
#16756=DIRECTION ( 'NONE',  ( 1.000000000000000078E-15, 1.000000000000000083E-30, -1.000000000000000000 ) ) ;
#16757=DIRECTION ( 'NONE',  ( 0.000000000000000000, 0.000000000000000000, 1.000000000000000000 ) ) ;
#16758=EDGE_LOOP ( 'NONE', ( #61347, #88175, #56874, #54711 ) ) ;
#16759=LINE ( 'NONE', #35846, #43610 ) ;
#16762=CARTESIAN_POINT ( 'NONE',  ( 101.0660769631361688, -27.44644056990073366, 70.54514908543497143 ) ) ;
#16763=VERTEX_POINT ( 'NONE', #40631 ) ;
#16764=CARTESIAN_POINT ( 'NONE',  ( 106.9524907322914089, -28.15978509997144741, 59.50956268521995440 ) ) ;
#16765=AXIS2_PLACEMENT_3D ( 'NONE', #21153, #42911, #55631 ) ;
#16768=CARTESIAN_POINT ( 'NONE',  ( 113.8294273123088374, -42.50220367264088139, 59.69586902018298247 ) ) ;
#16772=CIRCLE ( 'NONE', #29876, 13.44999999999999396 ) ;
#16773=CARTESIAN_POINT ( 'NONE',  ( 104.6438654950096350, -47.53759819287119370, 23.38895860924494841 ) ) ;
#16775=VERTEX_POINT ( 'NONE', #32021 ) ;
#16776=DIRECTION ( 'NONE',  ( 0.000000000000000000, 1.000000000000000000, 0.000000000000000000 ) ) ;
#16777=EDGE_LOOP ( 'NONE', ( #49209, #1265, #63031, #32085 ) ) ;
#16778=CARTESIAN_POINT ( 'NONE',  ( 114.1102230946791707, -44.52199131239810015, 129.1613395616249704 ) ) ;
#16779=CARTESIAN_POINT ( 'NONE',  ( 79.32178306374994747, -21.37853523628605501, 1.709393643969079113 ) ) ;
#16784=CARTESIAN_POINT ( 'NONE',  ( 71.25614885437424562, -84.12815644128085069, 396.9756252759102040 ) ) ;
#16785=CARTESIAN_POINT ( 'NONE',  ( 111.8874393434638250, -45.23954810143646910, 212.9870538473399506 ) ) ;
#16786=CARTESIAN_POINT ( 'NONE',  ( 80.06648329127401098, -41.22944715994105280, 8.225625275910942946 ) ) ;
#16790=EDGE_CURVE ( 'NONE', #36098, #54865, #61074, .T. ) ;
#16791=CARTESIAN_POINT ( 'NONE',  ( 116.7270850375765576, -31.35852969783502786, 25.24229194257798881 ) ) ;
#16793=ORIENTED_EDGE ( 'NONE', *, *, #69893, .F. ) ;
#16794=CARTESIAN_POINT ( 'NONE',  ( 103.2823872499383668, -27.47306433781803037, 171.3852924192453884 ) ) ;
#16795=CARTESIAN_POINT ( 'NONE',  ( 63.06670390244641311, -24.92844715994017335, 180.4678068554151196 ) ) ;
#16797=CIRCLE ( 'NONE', #28385, 2.750000000000002665 ) ;
#16799=CARTESIAN_POINT ( 'NONE',  ( 99.04384646079246579, -42.84093120032608226, 112.8445491430621246 ) ) ;
#16800=CARTESIAN_POINT ( 'NONE',  ( 96.79426660377257008, -34.87310936442964504, 241.1841967044819626 ) ) ;
#16803=FACE_BOUND ( 'NONE', #83057, .T. ) ;
#16804=DIRECTION ( 'NONE',  ( -0.7071067811865476838, -0.7071067811865473507, 0.000000000000000000 ) ) ;
#16805=CARTESIAN_POINT ( 'NONE',  ( 108.9266419529017327, -28.39302457734394736, 224.3238483995049819 ) ) ;
#16806=LINE ( 'NONE', #66267, #85323 ) ;
#16807=CARTESIAN_POINT ( 'NONE',  ( 115.5559444348970857, -42.74257571503945741, 49.33562527591095659 ) ) ;
#16809=CARTESIAN_POINT ( 'NONE',  ( 117.2063690954211808, -34.12380291655402687, 124.0270538473399426 ) ) ;
#16810=ORIENTED_EDGE ( 'NONE', *, *, #89292, .T. ) ;
#16811=CARTESIAN_POINT ( 'NONE',  ( 132.9421938897428674, -21.23922437001909103, 8.028287874532244572 ) ) ;
#16812=EDGE_CURVE ( 'NONE', #61339, #30803, #33821, .T. ) ;
#16813=ORIENTED_EDGE ( 'NONE', *, *, #72500, .F. ) ;
#16814=CARTESIAN_POINT ( 'NONE',  ( 97.33784129700110554, -34.07106458011696759, 67.11479194670231152 ) ) ;
#16815=EDGE_CURVE ( 'NONE', #75367, #51539, #67207, .T. ) ;
#16816=CARTESIAN_POINT ( 'NONE',  ( 103.3429861031523842, -27.44848569022927975, 276.3800890687926994 ) ) ;
#16818=DIRECTION ( 'NONE',  ( 1.000000000000000078E-15, 1.000000000000000083E-30, -1.000000000000000000 ) ) ;
#16821=CARTESIAN_POINT ( 'NONE',  ( 164.9667039024459996, -28.27351298637401200, -5.074374724088000832 ) ) ;
#16823=CIRCLE ( 'NONE', #66132, 1.000000000000000888 ) ;
#16824=ORIENTED_EDGE ( 'NONE', *, *, #45758, .T. ) ;
#16825=CARTESIAN_POINT ( 'NONE',  ( 104.2079940790944477, -25.20282339889105927, 90.26991099019693365 ) ) ;
#16827=CIRCLE ( 'NONE', #3781, 0.5000000000000004441 ) ;
#16828=SURFACE_STYLE_USAGE ( .BOTH. , #59024 ) ;
#16829=DIRECTION ( 'NONE',  ( 6.524622321627019585E-16, 3.741823817616790462E-31, 1.000000000000000000 ) ) ;
#16833=B_SPLINE_CURVE_WITH_KNOTS ( 'NONE', 3,
 ( #62023, #89757, #69303, #251, #9316, #19145, #78818, #29762, #43814, #9760, #11884, #16578, #5063, #53172, #80941, #39572, #37463, #60458 ),
 .UNSPECIFIED., .F., .F.,
 ( 4, 2, 2, 2, 2, 2, 2, 2, 4 ),
 ( 0.4999874473045213263, 0.5624890163914562091, 0.6249905854783910364, 0.6874921545653258637, 0.7499937236522606909, 0.8124952927391955182, 0.8749968618261303455, 0.9374984309130651727, 1.000000000000000000 ),
 .UNSPECIFIED. ) ;
#16835=DIRECTION ( 'NONE',  ( 4.299999999999999979E-14, -1.000000000000000000, 4.400000000000000367E-29 ) ) ;
#16837=LINE ( 'NONE', #79975, #5908 ) ;
#16838=DIRECTION ( 'NONE',  ( 0.000000000000000000, 1.000000000000000000, 0.000000000000000000 ) ) ;
#16839=DIRECTION ( 'NONE',  ( -0.7071067811865516806, 0.7071067811865434649, -7.071067811865511818E-16 ) ) ;
#16840=AXIS2_PLACEMENT_3D ( 'NONE', #50348, #8592, #84460 ) ;
#16843=DIRECTION ( 'NONE',  ( 1.000000000000000000, -3.885780586188044357E-13, 0.000000000000000000 ) ) ;
#16845=CARTESIAN_POINT ( 'NONE',  ( 98.25516505653069999, -40.97492784622581041, 167.6841967044819626 ) ) ;
#16846=CARTESIAN_POINT ( 'NONE',  ( 51.06648329127330044, -0.7548456658612000547, 333.4006252759120343 ) ) ;
#16848=CARTESIAN_POINT ( 'NONE',  ( 111.8651074766111293, -28.16866562884743885, 30.66991099019594813 ) ) ;
#16849=DIRECTION ( 'NONE',  ( 0.7071067811864980568, 0.7071067811865969777, 0.000000000000000000 ) ) ;
#16850=CARTESIAN_POINT ( 'NONE',  ( 20.03715912545830236, -46.82818131006180096, 300.4678068554150059 ) ) ;
#16851=FACE_OUTER_BOUND ( 'NONE', #23170, .T. ) ;
#16852=ORIENTED_EDGE ( 'NONE', *, *, #44445, .T. ) ;
#16853=CARTESIAN_POINT ( 'NONE',  ( 136.8164832912739826, -18.72944715994099951, 3.101481641215532825 ) ) ;
#16855=CARTESIAN_POINT ( 'NONE',  ( 114.9950743857441608, -30.04541929558963886, 224.3718157521019521 ) ) ;
#16857=ORIENTED_EDGE ( 'NONE', *, *, #14483, .T. ) ;
#16858=CARTESIAN_POINT ( 'NONE',  ( 104.2245914675057321, -27.77399204033938318, 201.7406309249449521 ) ) ;
#16859=CARTESIAN_POINT ( 'NONE',  ( 75.31670390244798341, -67.87844715994100397, 84.20080685541500998 ) ) ;
#16860=EDGE_CURVE ( 'NONE', #78803, #48612, #88805, .T. ) ;
#16861=CARTESIAN_POINT ( 'NONE',  ( 104.8770057419572908, -45.34735396192071732, 43.81015473446897346 ) ) ;
#16864=EDGE_CURVE ( 'NONE', #137, #88945, #53334, .T. ) ;
#16865=DIRECTION ( 'NONE',  ( -1.000000000000000078E-15, 1.000000000000000083E-30, 1.000000000000000000 ) ) ;
#16869=ORIENTED_EDGE ( 'NONE', *, *, #42244, .T. ) ;
#16870=CARTESIAN_POINT ( 'NONE',  ( 99.34937008002594894, -28.84845824588779095, 270.7051490854348685 ) ) ;
#16872=ORIENTED_EDGE ( 'NONE', *, *, #56541, .T. ) ;
#16874=EDGE_CURVE ( 'NONE', #6482, #68461, #8214, .T. ) ;
#16877=CARTESIAN_POINT ( 'NONE',  ( 152.0368932755772562, -23.42844715993587812, 193.9678068554149775 ) ) ;
#16878=AXIS2_PLACEMENT_3D ( 'NONE', #59867, #46231, #18546 ) ;
#16879=EDGE_CURVE ( 'NONE', #42339, #83669, #48770, .T. ) ;
#16880=CARTESIAN_POINT ( 'NONE',  ( 115.8115096128641284, -32.27542772465451293, 40.20133956162496958 ) ) ;
#16885=CARTESIAN_POINT ( 'NONE',  ( 115.6469432611725665, -28.48403513818922761, 35.43562527591098643 ) ) ;
#16886=AXIS2_PLACEMENT_3D ( 'NONE', #67461, #18871, #89722 ) ;
#16887=DIRECTION ( 'NONE',  ( 1.000000000000000078E-15, 1.000000000000000083E-30, -1.000000000000000000 ) ) ;
#16890=CARTESIAN_POINT ( 'NONE',  ( 117.5190927476815119, -36.54584727635032237, 288.8413395616252615 ) ) ;
#16891=VERTEX_POINT ( 'NONE', #68794 ) ;
#16892=CARTESIAN_POINT ( 'NONE',  ( 78.76282073104860615, -39.15113447711711103, 7.957506268071020017 ) ) ;
#16894=CARTESIAN_POINT ( 'NONE',  ( 107.0664832912739968, -36.72944715994100306, 287.6356252759109680 ) ) ;
#16895=EDGE_CURVE ( 'NONE', #37024, #67223, #6561, .T. ) ;
#16896=CARTESIAN_POINT ( 'NONE',  ( 109.1833626410332130, -45.12109460632434121, 90.60332846482899072 ) ) ;
#16897=CARTESIAN_POINT ( 'NONE',  ( 103.6314581395739793, -26.19921411638948427, 206.3394347997209763 ) ) ;
#16900=EDGE_LOOP ( 'NONE', ( #86491, #65153, #66775, #32797 ) ) ;
#16901=AXIS2_PLACEMENT_3D ( 'NONE', #49610, #71871, #15111 ) ;
#16902=CARTESIAN_POINT ( 'NONE',  ( 51.23005224011772185, -33.89581943344268211, 237.4678068554150059 ) ) ;
#16904=ORIENTED_EDGE ( 'NONE', *, *, #41190, .F. ) ;
#16905=CARTESIAN_POINT ( 'NONE',  ( 165.9667039024478754, -28.27351298636806831, 313.9678068554149490 ) ) ;
#16907=ORIENTED_EDGE ( 'NONE', *, *, #36377, .F. ) ;
#16908=DIRECTION ( 'NONE',  ( 1.000000000000000078E-15, -1.000000000000000083E-30, -1.000000000000000000 ) ) ;
#16910=CARTESIAN_POINT ( 'NONE',  ( 103.2785244713985833, -27.47464473206936830, 41.38562443853131612 ) ) ;
#16911=CARTESIAN_POINT ( 'NONE',  ( 103.4202683135912650, -45.01906637089264507, 131.6571817328389784 ) ) ;
#16912=CARTESIAN_POINT ( 'NONE',  ( 106.6048964044850607, -25.63891871564037928, 40.09753003781596448 ) ) ;
#16913=ADVANCED_FACE ( 'NONE', ( #54680 ), #8362, .F. ) ;
#16916=ORIENTED_EDGE ( 'NONE', *, *, #48847, .F. ) ;
#16918=CARTESIAN_POINT ( 'NONE',  ( 116.0743685831884733, -32.33849391669360784, 135.1874756336685834 ) ) ;
#16919=EDGE_LOOP ( 'NONE', ( #51925, #4766, #8568 ) ) ;
#16921=EDGE_CURVE ( 'NONE', #88540, #20676, #69692, .T. ) ;
#16923=DIRECTION ( 'NONE',  ( -1.000000000000000000, 0.000000000000000000, 0.000000000000000000 ) ) ;
#16924=LINE ( 'NONE', #85977, #42176 ) ;
#16927=CARTESIAN_POINT ( 'NONE',  ( 115.3236443966936235, -45.23002221789283084, 268.1899109901965517 ) ) ;
#16928=CARTESIAN_POINT ( 'NONE',  ( 100.4516903307928573, -27.81642228345825885, 31.59657765686396758 ) ) ;
#16929=FACE_OUTER_BOUND ( 'NONE', #31119, .T. ) ;
#16930=CARTESIAN_POINT ( 'NONE',  ( 152.0368932755770288, -23.42844715993588522, 300.4678068554149490 ) ) ;
#16932=CARTESIAN_POINT ( 'NONE',  ( 105.6962374661776209, -25.35223018209148194, 323.2475121285344244 ) ) ;
#16933=CARTESIAN_POINT ( 'NONE',  ( 107.0664832912739399, -36.72944715994096754, 298.1356252759109680 ) ) ;
#16934=CARTESIAN_POINT ( 'NONE',  ( 132.1198940698338902, -38.67261125154126233, 7.590611884332613357 ) ) ;
#16935=CARTESIAN_POINT ( 'NONE',  ( 116.3212776292296127, -32.94146857471318413, 287.6356252759109680 ) ) ;
#16936=PLANE ( 'NONE',  #12944 ) ;
#16937=CARTESIAN_POINT ( 'NONE',  ( 138.0667039024479550, -26.72944715994091069, 239.5838068554170377 ) ) ;
#16938=DIRECTION ( 'NONE',  ( 1.000000000000000078E-15, -1.000000000000000000, 0.000000000000000000 ) ) ;
#16939=CARTESIAN_POINT ( 'NONE',  ( 97.75295786963341982, -40.54146432227403807, 11.63562527591094309 ) ) ;
#16940=CARTESIAN_POINT ( 'NONE',  ( 97.95649862111255857, -30.46988169760521359, 161.8594347997199918 ) ) ;
#16941=CARTESIAN_POINT ( 'NONE',  ( 110.8022603587792219, -46.48553390388831019, 58.86705384733998159 ) ) ;
#16942=VECTOR ( 'NONE', #32503, 1000.000000000000000 ) ;
#16943=DIRECTION ( 'NONE',  ( 1.000000000000000078E-15, 1.000000000000000083E-30, -1.000000000000000000 ) ) ;
#16945=PLANE ( 'NONE',  #49427 ) ;
#16947=AXIS2_PLACEMENT_3D ( 'NONE', #48903, #83454, #19884 ) ;
#16948=ORIENTED_EDGE ( 'NONE', *, *, #50705, .T. ) ;
#16949=DIRECTION ( 'NONE',  ( 1.000000000000000078E-15, -1.000000000000000083E-30, -1.000000000000000000 ) ) ;
#16951=CARTESIAN_POINT ( 'NONE',  ( 96.07333748454176714, -35.06730156692550793, 67.20705384733894050 ) ) ;
#16952=CARTESIAN_POINT ( 'NONE',  ( 116.8189785850517524, -34.16011448583248722, 189.0314799851472287 ) ) ;
#16954=DIRECTION ( 'NONE',  ( 1.327617956749545812E-15, -0.7071067811865480168, -0.7071067811865470176 ) ) ;
#16955=CARTESIAN_POINT ( 'NONE',  ( 114.9613132280021830, -29.02649429439055595, 190.4537205140059655 ) ) ;
#16957=CARTESIAN_POINT ( 'NONE',  ( 98.15100683351592181, -41.26167086457207489, 146.7007424152079409 ) ) ;
#16958=DIRECTION ( 'NONE',  ( 0.000000000000000000, 0.000000000000000000, -1.000000000000000000 ) ) ;
#16959=LINE ( 'NONE', #79643, #29870 ) ;
#16963=CARTESIAN_POINT ( 'NONE',  ( 109.0694692412632492, -27.15596902575777349, 139.9127681330539872 ) ) ;
#16966=CARTESIAN_POINT ( 'NONE',  ( 97.22447099779657265, -34.58340453033963513, 102.5872975916109482 ) ) ;
#16967=CARTESIAN_POINT ( 'NONE',  ( 72.31648329127401098, -45.62589376934781882, 14.92562527591093691 ) ) ;
#16969=CARTESIAN_POINT ( 'NONE',  ( 97.32398421004042177, -35.86507053846868587, 227.2556252759109725 ) ) ;
#16971=DIRECTION ( 'NONE',  ( -1.000000000000000078E-15, -1.000000000000000083E-30, 1.000000000000000000 ) ) ;
#16973=ADVANCED_FACE ( 'NONE', ( #7462 ), #15174, .T. ) ;
#16975=ADVANCED_FACE ( 'NONE', ( #48314 ), #35150, .T. ) ;
#16976=CYLINDRICAL_SURFACE ( 'NONE', #864, 4.750000000000000888 ) ;
#16977=FACE_OUTER_BOUND ( 'NONE', #30134, .T. ) ;
#16979=CARTESIAN_POINT ( 'NONE',  ( 102.0615167388204725, -46.55869598106830409, 172.2137205140059564 ) ) ;
#16981=ORIENTED_EDGE ( 'NONE', *, *, #9718, .F. ) ;
#16982=ADVANCED_FACE ( 'NONE', ( #22003 ), #83777, .T. ) ;
#16983=ADVANCED_FACE ( 'NONE', ( #34712 ), #70589, .F. ) ;
#16984=DIRECTION ( 'NONE',  ( -4.237773401492740281E-14, 1.000000000000000000, 0.000000000000000000 ) ) ;
#16985=CARTESIAN_POINT ( 'NONE',  ( 77.31648329127399677, -18.72944715994106346, 3.101481641215480867 ) ) ;
#16990=EDGE_CURVE ( 'NONE', #46739, #78957, #68650, .T. ) ;
#16991=LINE ( 'NONE', #58742, #40754 ) ;
#16992=EDGE_CURVE ( 'NONE', #44371, #44076, #20650, .T. ) ;
#16993=CARTESIAN_POINT ( 'NONE',  ( 100.0080109101350985, -27.21007462382121744, 185.5841967044829630 ) ) ;
#16994=DIRECTION ( 'NONE',  ( 0.000000000000000000, 0.000000000000000000, -1.000000000000000000 ) ) ;
#16995=ORIENTED_EDGE ( 'NONE', *, *, #30084, .T. ) ;
#16996=ORIENTED_EDGE ( 'NONE', *, *, #23217, .T. ) ;
#16997=ORIENTED_EDGE ( 'NONE', *, *, #62518, .T. ) ;
#16999=LINE ( 'NONE', #31058, #11551 ) ;
#17002=CARTESIAN_POINT ( 'NONE',  ( 113.3129409812876389, -28.82675956000495887, 270.9758690201826425 ) ) ;
#17003=CARTESIAN_POINT ( 'NONE',  ( 108.3334472470058785, -46.73485946926888346, 272.6772918751394172 ) ) ;
#17007=CARTESIAN_POINT ( 'NONE',  ( 115.0813998565176774, -41.07721658520456742, 9.635625275910943088 ) ) ;
#17008=DIRECTION ( 'NONE',  ( 4.299999999999999979E-14, -1.000000000000000000, 0.000000000000000000 ) ) ;
#17009=ORIENTED_EDGE ( 'NONE', *, *, #23364, .T. ) ;
#17011=AXIS2_PLACEMENT_3D ( 'NONE', #30998, #86431, #11457 ) ;
#17012=VECTOR ( 'NONE', #68789, 1000.000000000000000 ) ;
#17013=CARTESIAN_POINT ( 'NONE',  ( 100.8875017264671783, -44.70024944885620499, 112.0523634285323453 ) ) ;
#17014=CIRCLE ( 'NONE', #89568, 1.000000000002049694 ) ;
#17016=ORIENTED_EDGE ( 'NONE', *, *, #65216, .F. ) ;
#17017=CARTESIAN_POINT ( 'NONE',  ( 101.7664832247249365, -29.99442739451795958, 15.02956268521998773 ) ) ;
#17018=CARTESIAN_POINT ( 'NONE',  ( 98.14931896820920088, -31.28605259387051518, 170.8899109901960003 ) ) ;
#17019=CARTESIAN_POINT ( 'NONE',  ( 114.5119312840560184, -28.59475203354325501, 154.4746728949589851 ) ) ;
#17021=CARTESIAN_POINT ( 'NONE',  ( 115.0547525607699697, -30.03093676393617173, 265.3813395616251682 ) ) ;
#17026=ADVANCED_FACE ( 'NONE', ( #65792 ), #73058, .T. ) ;
#17027=VECTOR ( 'NONE', #6291, 1000.000000000000000 ) ;
#17031=CIRCLE ( 'NONE', #8410, 10.00000000000000711 ) ;
#17032=CARTESIAN_POINT ( 'NONE',  ( 117.9946794957619431, -34.78331989172042427, 198.9546728949589749 ) ) ;
#17034=CARTESIAN_POINT ( 'NONE',  ( 117.0233241640237338, -39.93681227152024604, 158.5784824187679476 ) ) ;
#17035=DIRECTION ( 'NONE',  ( 0.000000000000000000, -1.000000000000000000, 0.000000000000000000 ) ) ;
#17040=CARTESIAN_POINT ( 'NONE',  ( 100.8736165617014677, -44.32606212243579336, 8.032768133052980986 ) ) ;
#17041=DIRECTION ( 'NONE',  ( -9.073094938289460781E-13, -1.000000000000000000, 0.000000000000000000 ) ) ;
#17042=DIRECTION ( 'NONE',  ( 0.7071067811865453523, 0.7071067811865496822, 7.071067811865460542E-16 ) ) ;
#17045=DIRECTION ( 'NONE',  ( 1.000000000000000078E-15, -1.000000000000000083E-30, -1.000000000000000000 ) ) ;
#17046=FACE_OUTER_BOUND ( 'NONE', #82432, .T. ) ;
#17047=CARTESIAN_POINT ( 'NONE',  ( 113.1460701246578680, -29.40654960323831801, 195.5838068554210452 ) ) ;
#17048=VERTEX_POINT ( 'NONE', #72632 ) ;
#17049=CARTESIAN_POINT ( 'NONE',  ( 136.1031364520983686, -20.57950990141002379, 7.523361336352738959 ) ) ;
#17050=CARTESIAN_POINT ( 'NONE',  ( 104.5572623809163701, -48.33710955716689028, 182.4070538473399665 ) ) ;
#17051=CARTESIAN_POINT ( 'NONE',  ( 116.6747397658760832, -32.59390121112949856, 75.14991099019697174 ) ) ;
#17052=CARTESIAN_POINT ( 'NONE',  ( 113.8273992703627044, -26.93653503804465288, 235.5956252759109759 ) ) ;
#17053=LINE ( 'NONE', #58806, #88070 ) ;
#17054=DIRECTION ( 'NONE',  ( -4.237773401492740281E-14, 1.000000000000000000, 0.000000000000000000 ) ) ;
#17055=DIRECTION ( 'NONE',  ( 1.000000000000000000, 4.443626637970137948E-14, 0.000000000000000000 ) ) ;
#17056=CARTESIAN_POINT ( 'NONE',  ( 97.86387113231445767, -40.64285381717150614, 37.64614471822871167 ) ) ;
#17057=LINE ( 'NONE', #25194, #29102 ) ;
#17060=VECTOR ( 'NONE', #57485, 1000.000000000000000 ) ;
#17061=CARTESIAN_POINT ( 'NONE',  ( 97.39135791878592840, -39.27877462570257450, 66.53211423348820119 ) ) ;
#17062=ORIENTED_EDGE ( 'NONE', *, *, #29495, .T. ) ;
#17063=ORIENTED_EDGE ( 'NONE', *, *, #66949, .T. ) ;
#17064=CARTESIAN_POINT ( 'NONE',  ( 113.3421067344362996, -42.52364098839497331, 122.6552769709339827 ) ) ;
#17067=CARTESIAN_POINT ( 'NONE',  ( 104.1140010245780729, -46.70499295924809502, 103.3470538473389411 ) ) ;
#17069=CARTESIAN_POINT ( 'NONE',  ( 77.54412859703477068, -17.63380991825937016, 7.053480412781051534 ) ) ;
#17072=CARTESIAN_POINT ( 'NONE',  ( 110.8002668817294847, -46.40403677370081681, 17.85753003781598380 ) ) ;
#17078=PLANE ( 'NONE',  #54383 ) ;
#17079=CARTESIAN_POINT ( 'NONE',  ( 73.06670390244801183, -50.82844715994100682, 198.9178068554149945 ) ) ;
#17080=CARTESIAN_POINT ( 'NONE',  ( 99.09570908081879281, -30.55043174719083510, 116.8022919419756107 ) ) ;
#17083=ADVANCED_FACE ( 'NONE', ( #25351 ), #62865, .T. ) ;
#17086=LINE ( 'NONE', #17530, #35885 ) ;
#17087=EDGE_CURVE ( 'NONE', #82750, #52712, #24483, .T. ) ;
#17089=CARTESIAN_POINT ( 'NONE',  ( 116.7246412902989903, -32.86309880586077270, 54.12991099019698282 ) ) ;
#17090=VERTEX_POINT ( 'NONE', #46227 ) ;
#17092=AXIS2_PLACEMENT_3D ( 'NONE', #35899, #8206, #43148 ) ;
#17094=LINE ( 'NONE', #88822, #56013 ) ;
#17097=AXIS2_PLACEMENT_3D ( 'NONE', #40695, #88865, #34326 ) ;
#17099=CARTESIAN_POINT ( 'NONE',  ( 104.0433210460927000, -44.34148882339519560, 115.0938046553049503 ) ) ;
#17101=CARTESIAN_POINT ( 'NONE',  ( 97.12565827820864683, -37.99761304849175758, 96.42736898879877572 ) ) ;
#17102=EDGE_CURVE ( 'NONE', #84365, #88986, #68044, .T. ) ;
#17110=CARTESIAN_POINT ( 'NONE',  ( 113.8438844162330810, -30.22226962059244215, 185.8549166392299696 ) ) ;
#17112=VECTOR ( 'NONE', #36435, 1000.000000000000000 ) ;
#17113=CARTESIAN_POINT ( 'NONE',  ( 95.28708132950120557, -38.28245711228485959, 147.4299109901969871 ) ) ;
#17114=LINE ( 'NONE', #79801, #86443 ) ;
#17115=VECTOR ( 'NONE', #63141, 1000.000000000000000 ) ;
#17116=CARTESIAN_POINT ( 'NONE',  ( 104.4081006377808620, -46.45808913390618500, 83.36479194067089793 ) ) ;
#17117=VERTEX_POINT ( 'NONE', #68937 ) ;
#17118=EDGE_LOOP ( 'NONE', ( #46126, #80367 ) ) ;
#17119=ORIENTED_EDGE ( 'NONE', *, *, #81628, .F. ) ;
#17120=CARTESIAN_POINT ( 'NONE',  ( 114.9947780803761503, -40.19975936245594283, 206.3042808457819604 ) ) ;
#17121=CARTESIAN_POINT ( 'NONE',  ( 116.2511270133230283, -31.75062363771698770, 69.22133956162495849 ) ) ;
#17123=CARTESIAN_POINT ( 'NONE',  ( 117.3629797429381654, -38.21633193987523214, 28.71276813305395592 ) ) ;
#17126=CARTESIAN_POINT ( 'NONE',  ( 156.5667039024485518, -48.82844715993568485, 173.2178068554149775 ) ) ;
#17127=CARTESIAN_POINT ( 'NONE',  ( 108.2778103265350893, -47.71616603169876214, 153.6518157521009584 ) ) ;
#17129=EDGE_LOOP ( 'NONE', ( #79545, #85673, #55337, #5424 ) ) ;
#17130=CARTESIAN_POINT ( 'NONE',  ( 194.0667039024475287, -24.92844715993407334, 180.4678068554150343 ) ) ;
#17132=VERTEX_POINT ( 'NONE', #5370 ) ;
#17133=FACE_OUTER_BOUND ( 'NONE', #47625, .T. ) ;
#17135=ADVANCED_FACE ( 'NONE', ( #48023 ), #34407, .T. ) ;
#17138=CARTESIAN_POINT ( 'NONE',  ( 50.88849390559499142, -32.11662333284530746, -5.074374724088000832 ) ) ;
#17139=VECTOR ( 'NONE', #87096, 1000.000000000000000 ) ;
#17140=LINE ( 'NONE', #45264, #78363 ) ;
#17141=CARTESIAN_POINT ( 'NONE',  ( 109.9110735108787793, -46.79593677437021881, 72.79562527591099297 ) ) ;
#17142=LINE ( 'NONE', #72552, #66341 ) ;
#17144=CARTESIAN_POINT ( 'NONE',  ( 107.0664832912739968, -36.72944715994100306, 9.635625275910941312 ) ) ;
#17145=CARTESIAN_POINT ( 'NONE',  ( 115.8115096128642136, -32.27542772465447030, 44.20133956162592170 ) ) ;
#17146=DIRECTION ( 'NONE',  ( 0.000000000000000000, 0.000000000000000000, 1.000000000000000000 ) ) ;
#17147=CARTESIAN_POINT ( 'NONE',  ( 107.5647246096319094, -47.74832088493814553, 188.6003871806729535 ) ) ;
#17148=CARTESIAN_POINT ( 'NONE',  ( 97.81170051792484799, -40.51743816602341752, 61.63542871443850402 ) ) ;
#17150=EDGE_LOOP ( 'NONE', ( #58977, #52125, #61979, #28480 ) ) ;
#17151=CARTESIAN_POINT ( 'NONE',  ( 94.58945128933383728, -41.88441296220994303, 293.6356252759107974 ) ) ;
#17154=CARTESIAN_POINT ( 'NONE',  ( 156.5667039024483813, -48.82844715993569196, 254.7178068554149490 ) ) ;
#17156=FACE_OUTER_BOUND ( 'NONE', #24997, .T. ) ;
#17158=CARTESIAN_POINT ( 'NONE',  ( 101.3806489482690694, -45.56251468762313550, 222.1213395616249784 ) ) ;
#17161=CARTESIAN_POINT ( 'NONE',  ( 97.54012738755939438, -43.81963713510241121, 257.8356252759109566 ) ) ;
#17162=CARTESIAN_POINT ( 'NONE',  ( 109.0806625061526205, -47.64460086702110431, 123.7337205140059666 ) ) ;
#17165=CIRCLE ( 'NONE', #4110, 0.5000000000000004441 ) ;
#17168=CARTESIAN_POINT ( 'NONE',  ( 112.0652232319741586, -45.48878010129285343, 263.9899091037361814 ) ) ;
#17169=VERTEX_POINT ( 'NONE', #55279 ) ;
#17171=ORIENTED_EDGE ( 'NONE', *, *, #64251, .T. ) ;
#17173=AXIS2_PLACEMENT_3D ( 'NONE', #89070, #40461, #69524 ) ;
#17175=CARTESIAN_POINT ( 'NONE',  ( 98.30753417922522885, -41.72887547139915654, 71.73979194078179944 ) ) ;
#17176=CARTESIAN_POINT ( 'NONE',  ( 112.6636929512762180, -45.52454417301038347, 259.0270538473393458 ) ) ;
#17178=CARTESIAN_POINT ( 'NONE',  ( 131.4450127212694781, -35.89730640218696323, 2.921034946745736605 ) ) ;
#17181=LINE ( 'NONE', #44866, #74792 ) ;
#17182=CARTESIAN_POINT ( 'NONE',  ( 112.0098809771561577, -44.31729861111978153, 222.4705150661719983 ) ) ;
#17183=ORIENTED_EDGE ( 'NONE', *, *, #67633, .F. ) ;
#17184=AXIS2_PLACEMENT_3D ( 'NONE', #79759, #50685, #23893 ) ;
#17186=EDGE_LOOP ( 'NONE', ( #85674, #84190, #69258, #62878 ) ) ;
#17188=CARTESIAN_POINT ( 'NONE',  ( 101.9934930118830749, -45.44599331293795785, 182.1565212684371033 ) ) ;
#17190=CARTESIAN_POINT ( 'NONE',  ( 105.1480534186857483, -26.53835308478808130, 276.2365776568628917 ) ) ;
#17191=EDGE_CURVE ( 'NONE', #61623, #59070, #52710, .T. ) ;
#17192=DIRECTION ( 'NONE',  ( 1.000000000000000000, 4.163336342344333240E-14, 0.000000000000000000 ) ) ;
#17194=DIRECTION ( 'NONE',  ( 1.000000000000000078E-15, -1.000000000000000083E-30, -1.000000000000000000 ) ) ;
#17195=CARTESIAN_POINT ( 'NONE',  ( 101.9933023703032262, -45.44587501993174072, 27.15642918372197556 ) ) ;
#17197=AXIS2_PLACEMENT_3D ( 'NONE', #2628, #31651, #59351 ) ;
#17199=CARTESIAN_POINT ( 'NONE',  ( 112.7925898505289979, -28.47466936393675851, 55.59362532201837581 ) ) ;
#17200=ORIENTED_EDGE ( 'NONE', *, *, #58489, .F. ) ;
#17201=FACE_OUTER_BOUND ( 'NONE', #6372, .T. ) ;
#17202=CARTESIAN_POINT ( 'NONE',  ( 114.0183221777719638, -41.00747610084435024, 16.20523322673395228 ) ) ;
#17203=AXIS2_PLACEMENT_3D ( 'NONE', #87367, #45995, #25127 ) ;
#17206=DIRECTION ( 'NONE',  ( 1.000000000000000000, 4.299999999999999979E-14, 1.000000000000000078E-15 ) ) ;
#17207=EDGE_CURVE ( 'NONE', #16775, #82312, #12635, .T. ) ;
#17208=CARTESIAN_POINT ( 'NONE',  ( 125.8897075496517317, -55.55267141831851774, -5.074374724089010691 ) ) ;
#17209=ORIENTED_EDGE ( 'NONE', *, *, #42767, .T. ) ;
#17210=DIRECTION ( 'NONE',  ( 0.000000000000000000, 0.000000000000000000, -1.000000000000000000 ) ) ;
#17211=CIRCLE ( 'NONE', #67974, 11.45913725231036118 ) ;
#17212=DIRECTION ( 'NONE',  ( -0.7071067811866279529, 0.7071067811864671926, -7.071067811866286874E-16 ) ) ;
#17213=ORIENTED_EDGE ( 'NONE', *, *, #82058, .T. ) ;
#17214=CARTESIAN_POINT ( 'NONE',  ( 116.1238663722925253, -29.08717671455551468, 74.38419670448293175 ) ) ;
#17215=ORIENTED_EDGE ( 'NONE', *, *, #31943, .T. ) ;
#17216=CARTESIAN_POINT ( 'NONE',  ( 99.10695020771697727, -33.55172231072156563, 40.44670554236296312 ) ) ;
#17217=VECTOR ( 'NONE', #16526, 1000.000000000000000 ) ;
#17218=CARTESIAN_POINT ( 'NONE',  ( 37.03715912545434463, -48.62818131006122258, 237.4678068554150059 ) ) ;
#17219=CARTESIAN_POINT ( 'NONE',  ( 98.33263373320089329, -38.22883053613415427, 87.89301187732596077 ) ) ;
#17220=DIRECTION ( 'NONE',  ( 0.000000000000000000, 0.000000000000000000, 1.000000000000000000 ) ) ;
#17221=FACE_BOUND ( 'NONE', #82489, .T. ) ;
#17224=CARTESIAN_POINT ( 'NONE',  ( 97.05449064767977063, -33.74661928051879300, 27.09562527591097236 ) ) ;
#17225=CARTESIAN_POINT ( 'NONE',  ( 142.8824340801165249, -74.11588153691421610, 540.9756252759101471 ) ) ;
#17227=PLANE ( 'NONE',  #86520 ) ;
#17228=VERTEX_POINT ( 'NONE', #68498 ) ;
#17229=CARTESIAN_POINT ( 'NONE',  ( 78.22143491580683872, -20.77077206072207360, 2.188418444514117489 ) ) ;
#17232=AXIS2_PLACEMENT_3D ( 'NONE', #73081, #80817, #59882 ) ;
#17234=PLANE ( 'NONE',  #63766 ) ;
#17235=CARTESIAN_POINT ( 'NONE',  ( 101.0525363619397012, -44.44280425155412217, 232.0499109901969632 ) ) ;
#17236=CARTESIAN_POINT ( 'NONE',  ( 135.3838309168194201, -60.54606547621062163, 361.9756252759100335 ) ) ;
#17237=DIRECTION ( 'NONE',  ( 1.000000000000000000, 4.163336342344333240E-14, 0.000000000000000000 ) ) ;
#17238=CARTESIAN_POINT ( 'NONE',  ( 116.1236770753320542, -29.08733643602844054, 70.38419670448192278 ) ) ;
#17239=CARTESIAN_POINT ( 'NONE',  ( 100.8870673645827480, -44.69991497499172084, 43.05225246011283247 ) ) ;
#17240=ORIENTED_EDGE ( 'NONE', *, *, #32059, .T. ) ;
#17241=CARTESIAN_POINT ( 'NONE',  ( 97.31305002966453799, -38.96050384283260826, 172.5054018742519020 ) ) ;
#17243=EDGE_CURVE ( 'NONE', #73652, #54474, #77403, .T. ) ;
#17244=AXIS2_PLACEMENT_3D ( 'NONE', #18282, #66881, #24660 ) ;
#17245=ORIENTED_EDGE ( 'NONE', *, *, #12991, .T. ) ;
#17247=CARTESIAN_POINT ( 'NONE',  ( 25.56670390244797275, -48.82844715994099971, 134.4678068554150059 ) ) ;
#17248=CARTESIAN_POINT ( 'NONE',  ( 116.0363244534468805, -41.99923036749497385, 238.4041967044829562 ) ) ;
#17249=FACE_OUTER_BOUND ( 'NONE', #20584, .T. ) ;
#17252=DIRECTION ( 'NONE',  ( 0.000000000000000000, 1.000000000000000000, 0.000000000000000000 ) ) ;
#17253=CARTESIAN_POINT ( 'NONE',  ( 106.6575247680289777, -45.29010455595041407, 246.9609912566479579 ) ) ;
#17254=DIRECTION ( 'NONE',  ( 0.000000000000000000, 0.000000000000000000, 1.000000000000000000 ) ) ;
#17255=CARTESIAN_POINT ( 'NONE',  ( 110.1514708964275684, -46.66481413883387575, 93.81562527591097478 ) ) ;
#17257=CARTESIAN_POINT ( 'NONE',  ( 102.3405178495751215, -46.07139110582879482, 127.2041967044829960 ) ) ;
#17259=LINE ( 'NONE', #24516, #59640 ) ;
#17261=LINE ( 'NONE', #9998, #62759 ) ;
#17262=LINE ( 'NONE', #71342, #42097 ) ;
#17263=CARTESIAN_POINT ( 'NONE',  ( 130.0664832912740110, -14.47844715994100007, 17.92562527591199739 ) ) ;
#17264=ORIENTED_EDGE ( 'NONE', *, *, #42381, .F. ) ;
#17265=VECTOR ( 'NONE', #601, 1000.000000000000000 ) ;
#17267=EDGE_LOOP ( 'NONE', ( #42679, #16113, #33606, #18306 ) ) ;
#17270=VECTOR ( 'NONE', #57054, 1000.000000000000000 ) ;
#17271=CARTESIAN_POINT ( 'NONE',  ( 156.5667039024485803, -48.82844715993568485, 137.2178068554149775 ) ) ;
#17273=VECTOR ( 'NONE', #7, 1000.000000000000000 ) ;
#17274=ADVANCED_FACE ( 'NONE', ( #46683 ), #12187, .T. ) ;
#17275=CARTESIAN_POINT ( 'NONE',  ( 114.3686432469292527, -44.20104832357726110, 73.19276813305397411 ) ) ;
#17277=DIRECTION ( 'NONE',  ( 0.000000000000000000, 1.000000000000000000, 0.000000000000000000 ) ) ;
#17278=DIRECTION ( 'NONE',  ( 0.7071067811739274456, -0.7071067811991676999, 0.000000000000000000 ) ) ;
#17279=CARTESIAN_POINT ( 'NONE',  ( 72.26648329127297643, -1.929447159941394263, 361.9756252759109998 ) ) ;
#17282=ORIENTED_EDGE ( 'NONE', *, *, #15046, .F. ) ;
#17283=CYLINDRICAL_SURFACE ( 'NONE', #46015, 16.00000000000000000 ) ;
#17287=VECTOR ( 'NONE', #1066, 1000.000000000000000 ) ;
#17288=DIRECTION ( 'NONE',  ( 0.000000000000000000, 0.000000000000000000, -1.000000000000000000 ) ) ;
#17290=LINE ( 'NONE', #9578, #81434 ) ;
#17293=CARTESIAN_POINT ( 'NONE',  ( 113.1634500054121872, -44.41975088505036240, 164.1099109901959707 ) ) ;
#17294=EDGE_CURVE ( 'NONE', #16097, #3936, #48379, .T. ) ;
#17295=VECTOR ( 'NONE', #69420, 1000.000000000000000 ) ;
#17297=ORIENTED_EDGE ( 'NONE', *, *, #2460, .F. ) ;
#17298=CARTESIAN_POINT ( 'NONE',  ( 97.32756240345236165, -42.09278592124177010, 22.72705384733897205 ) ) ;
#17300=DIRECTION ( 'NONE',  ( -0.1858654557293118459, 0.9825752044329915114, 0.000000000000000000 ) ) ;
#17301=EDGE_CURVE ( 'NONE', #50227, #8645, #50158, .T. ) ;
#17302=CARTESIAN_POINT ( 'NONE',  ( 138.8167039024479834, -67.87844715994100397, 35.51780685541480409 ) ) ;
#17303=VERTEX_POINT ( 'NONE', #9294 ) ;
#17306=EDGE_LOOP ( 'NONE', ( #49870, #68354, #75192, #76379 ) ) ;
#17307=EDGE_LOOP ( 'NONE', ( #76641, #10717, #55680, #67993 ) ) ;
#17308=CIRCLE ( 'NONE', #53504, 2.116999999999993776 ) ;
#17309=CARTESIAN_POINT ( 'NONE',  ( 106.9887167903908392, -45.59072421142732168, 184.0015833058969577 ) ) ;
#17310=CARTESIAN_POINT ( 'NONE',  ( 51.34673845256598668, -29.62846900982231446, -5.074374724088000832 ) ) ;
#17312=DIRECTION ( 'NONE',  ( 0.000000000000000000, 1.000000000000000000, 0.000000000000000000 ) ) ;
#17313=EDGE_CURVE ( 'NONE', #23155, #66915, #51928, .T. ) ;
#17315=ORIENTED_EDGE ( 'NONE', *, *, #85399, .F. ) ;
#17317=CARTESIAN_POINT ( 'NONE',  ( 32.25690895537100289, -33.54226604285010893, -5.074374724088000832 ) ) ;
#17318=ADVANCED_FACE ( 'NONE', ( #77891 ), #51491, .T. ) ;
#17319=ORIENTED_EDGE ( 'NONE', *, *, #42991, .T. ) ;
#17320=CARTESIAN_POINT ( 'NONE',  ( 106.8369185487093063, -47.13021470646874178, 272.5584824187680510 ) ) ;
#17322=VERTEX_POINT ( 'NONE', #16116 ) ;
#17323=CARTESIAN_POINT ( 'NONE',  ( 98.30753418384445297, -41.72887547938789510, 81.73979194150940941 ) ) ;
#17324=DIRECTION ( 'NONE',  ( 0.000000000000000000, 0.000000000000000000, 1.000000000000000000 ) ) ;
#17325=DIRECTION ( 'NONE',  ( 1.000000000000000000, 0.000000000000000000, 0.000000000000000000 ) ) ;
#17326=CARTESIAN_POINT ( 'NONE',  ( 107.0664832912739968, -36.72944715994103149, 14.92562527591097066 ) ) ;
#17327=CARTESIAN_POINT ( 'NONE',  ( 114.8463700017591407, -29.67172957150665979, 205.4127681330539872 ) ) ;
#17329=DIRECTION ( 'NONE',  ( -1.000000000000000078E-15, 0.000000000000000000, 1.000000000000000000 ) ) ;
#17330=CIRCLE ( 'NONE', #59386, 3.299999999999997158 ) ;
#17331=ORIENTED_EDGE ( 'NONE', *, *, #27418, .T. ) ;
#17332=CARTESIAN_POINT ( 'NONE',  ( 100.4516903307928573, -27.81642228345825885, 31.59657765686396758 ) ) ;
#17333=CARTESIAN_POINT ( 'NONE',  ( 180.2121375201594731, -29.73316016638963433, 313.9678068554149490 ) ) ;
#17334=CARTESIAN_POINT ( 'NONE',  ( 98.40533970481327231, -42.07952101345657780, 11.76800622829193799 ) ) ;
#17336=VECTOR ( 'NONE', #79244, 1000.000000000000000 ) ;
#17337=CARTESIAN_POINT ( 'NONE',  ( 78.64532134553982701, -39.08531275929848903, 7.905164235249591442 ) ) ;
#17339=FACE_OUTER_BOUND ( 'NONE', #87785, .T. ) ;
#17340=CARTESIAN_POINT ( 'NONE',  ( 102.7086973628091187, -29.82731503872160417, 108.3423760838769851 ) ) ;
#17341=CARTESIAN_POINT ( 'NONE',  ( 103.0821958934680111, -47.91639064866039632, 248.3041967044829619 ) ) ;
#17343=ORIENTED_EDGE ( 'NONE', *, *, #84167, .T. ) ;
#17344=CARTESIAN_POINT ( 'NONE',  ( 172.5664832912729878, -27.82844715994070484, 198.9256252759119832 ) ) ;
#17345=ORIENTED_EDGE ( 'NONE', *, *, #87436, .F. ) ;
#17346=VERTEX_POINT ( 'NONE', #71972 ) ;
#17348=ORIENTED_EDGE ( 'NONE', *, *, #60344, .F. ) ;
#17349=EDGE_LOOP ( 'NONE', ( #43058, #27216, #83326, #34467 ) ) ;
#17350=CARTESIAN_POINT ( 'NONE',  ( 192.5667039024474434, -23.42844715993433624, 180.4678068554150343 ) ) ;
#17352=EDGE_CURVE ( 'NONE', #44183, #30803, #47204, .T. ) ;
#17353=CARTESIAN_POINT ( 'NONE',  ( 103.3178953596948162, -27.45860474605225221, 41.38224140060551548 ) ) ;
#17355=CARTESIAN_POINT ( 'NONE',  ( 100.5019087779429015, -42.19410572027086914, 116.3009912566479471 ) ) ;
#17356=CARTESIAN_POINT ( 'NONE',  ( 112.3495078575228376, -28.18909723048616911, 289.6356252759109680 ) ) ;
#17360=EDGE_LOOP ( 'NONE', ( #68460, #2038, #40057, #84735 ) ) ;
#17361=CARTESIAN_POINT ( 'NONE',  ( 97.03930911280052385, -36.38725636255255580, 167.2994274293335195 ) ) ;
#17363=CARTESIAN_POINT ( 'NONE',  ( 75.31670390244798341, -50.82844715994100682, 33.40080685541480676 ) ) ;
#17364=VECTOR ( 'NONE', #41416, 1000.000000000000000 ) ;
#17365=LINE ( 'NONE', #24186, #50940 ) ;
#17366=ORIENTED_EDGE ( 'NONE', *, *, #22416, .F. ) ;
#17368=CARTESIAN_POINT ( 'NONE',  ( 111.4804840314119758, -26.59568808167472653, 284.7375300378156453 ) ) ;
#17369=CARTESIAN_POINT ( 'NONE',  ( 99.11046098610404442, -43.53346720896296773, 27.88991099019694175 ) ) ;
#17370=LINE ( 'NONE', #72783, #88333 ) ;
#17372=LINE ( 'NONE', #17815, #75754 ) ;
#17374=CARTESIAN_POINT ( 'NONE',  ( 131.7676426598725072, -38.23887630717962338, 7.293197373621404189 ) ) ;
#17375=VECTOR ( 'NONE', #69143, 1000.000000000000000 ) ;
#17376=FACE_OUTER_BOUND ( 'NONE', #51550, .T. ) ;
#17380=EDGE_CURVE ( 'NONE', #7662, #61259, #64370, .T. ) ;
#17381=CARTESIAN_POINT ( 'NONE',  ( 106.2486884972880432, -26.25648168547507311, 25.13848241876792855 ) ) ;
#17382=CARTESIAN_POINT ( 'NONE',  ( 114.9778481211559154, -29.01036126763497336, 190.4537205140059655 ) ) ;
#17383=CARTESIAN_POINT ( 'NONE',  ( 100.3971814656068915, -28.68844771884695888, 36.62705384733894221 ) ) ;
#17384=DIRECTION ( 'NONE',  ( 0.000000000000000000, -1.000000000000000000, 0.000000000000000000 ) ) ;
#17385=CARTESIAN_POINT ( 'NONE',  ( 117.0608945236349143, -38.08045312005563687, 48.71895860930425926 ) ) ;
#17386=CARTESIAN_POINT ( 'NONE',  ( 80.44276116895382245, -33.99866847873249753, 1.641799428525402504 ) ) ;
#17388=AXIS2_PLACEMENT_3D ( 'NONE', #17877, #45553, #23821 ) ;
#17390=ORIENTED_EDGE ( 'NONE', *, *, #48267, .T. ) ;
#17391=DIRECTION ( 'NONE',  ( -1.000000000000000078E-15, 1.000000000000000000, 0.000000000000000000 ) ) ;
#17392=VERTEX_POINT ( 'NONE', #58753 ) ;
#17393=CARTESIAN_POINT ( 'NONE',  ( 114.7041265136727901, -43.74408836545391921, 74.22324432352993995 ) ) ;
#17396=ORIENTED_EDGE ( 'NONE', *, *, #37857, .T. ) ;
#17398=CARTESIAN_POINT ( 'NONE',  ( 102.2473430764597282, -45.94923854148469644, 208.1927681330539599 ) ) ;
#17399=CARTESIAN_POINT ( 'NONE',  ( 100.8864929060172528, -44.69947222835936884, 253.0533978726845419 ) ) ;
#17402=CARTESIAN_POINT ( 'NONE',  ( 128.5664832912740110, -41.22944715994101017, 4.925625275910991974 ) ) ;
#17404=DIRECTION ( 'NONE',  ( 0.7071067811864666375, 0.7071067811866283970, 7.071067811864971448E-16 ) ) ;
#17406=CARTESIAN_POINT ( 'NONE',  ( 109.6407163665292046, -46.48066509518846345, 97.78129702168313031 ) ) ;
#17407=AXIS2_PLACEMENT_3D ( 'NONE', #9971, #44912, #82041 ) ;
#17408=CARTESIAN_POINT ( 'NONE',  ( 113.5587197313314505, -28.64306037466250743, 119.5261014663879564 ) ) ;
#17410=ORIENTED_EDGE ( 'NONE', *, *, #66796, .F. ) ;
#17411=CARTESIAN_POINT ( 'NONE',  ( 109.2913206311583707, -45.85778897805103327, 84.18634521065892784 ) ) ;
#17413=CARTESIAN_POINT ( 'NONE',  ( 96.86352172870826394, -32.31225822881506815, 207.0013395616249738 ) ) ;
#17414=CARTESIAN_POINT ( 'NONE',  ( 51.42025729302664416, -31.94127993907661178, 237.4678068554150059 ) ) ;
#17415=CARTESIAN_POINT ( 'NONE',  ( 141.0664832912739826, -8.729447159940995959, 14.67562527591100441 ) ) ;
#17416=LINE ( 'NONE', #3342, #22070 ) ;
#17417=VECTOR ( 'NONE', #80607, 1000.000000000000000 ) ;
#17420=DIRECTION ( 'NONE',  ( -4.237773401492740281E-14, 1.000000000000000000, 0.000000000000000000 ) ) ;
#17421=CARTESIAN_POINT ( 'NONE',  ( 188.5667039024483529, -42.82844715993430640, 134.7178068554150059 ) ) ;
#17423=EDGE_CURVE ( 'NONE', #19595, #19378, #77550, .T. ) ;
#17424=CARTESIAN_POINT ( 'NONE',  ( 99.11802762103501152, -45.48540990049890809, 156.9899109901969609 ) ) ;
#17426=ORIENTED_EDGE ( 'NONE', *, *, #30752, .T. ) ;
#17430=EDGE_CURVE ( 'NONE', #74275, #17303, #19671, .T. ) ;
#17433=DIRECTION ( 'NONE',  ( 0.7071067811862279395, -0.7071067811868672059, 7.071067811862286363E-16 ) ) ;
#17434=CARTESIAN_POINT ( 'NONE',  ( 108.6750451637706618, -26.42898313331718541, 189.9527681330539792 ) ) ;
#17435=LINE ( 'NONE', #19223, #70568 ) ;
#17437=VERTEX_POINT ( 'NONE', #88728 ) ;
#17438=EDGE_LOOP ( 'NONE', ( #18891, #47908, #77129, #14345 ) ) ;
#17439=VECTOR ( 'NONE', #2236, 1000.000000000000000 ) ;
#17440=LINE ( 'NONE', #37439, #83937 ) ;
#17442=CARTESIAN_POINT ( 'NONE',  ( 132.3573525511357332, -34.57277629268848074, 7.749696248598098691 ) ) ;
#17443=CARTESIAN_POINT ( 'NONE',  ( 98.69396380956492010, -33.82637249272325164, 282.4930118773256709 ) ) ;
#17444=CIRCLE ( 'NONE', #24702, 4.750000000000004441 ) ;
#17445=LINE ( 'NONE', #72851, #5730 ) ;
#17446=ORIENTED_EDGE ( 'NONE', *, *, #83021, .F. ) ;
#17447=CARTESIAN_POINT ( 'NONE',  ( 104.9952014352892888, -44.61589190275481798, 9.635625275910941312 ) ) ;
#17448=CARTESIAN_POINT ( 'NONE',  ( 82.15318967143088003, -16.93816060012580138, 7.482180659745496065 ) ) ;
#17450=CIRCLE ( 'NONE', #30488, 0.5000000000000079936 ) ;
#17453=ORIENTED_EDGE ( 'NONE', *, *, #46897, .F. ) ;
#17454=ORIENTED_EDGE ( 'NONE', *, *, #12789, .F. ) ;
#17455=CARTESIAN_POINT ( 'NONE',  ( 115.0871287824179348, -30.61533435494355970, 155.3439420463051590 ) ) ;
#17456=EDGE_CURVE ( 'NONE', #65898, #76316, #67269, .T. ) ;
#17457=CARTESIAN_POINT ( 'NONE',  ( 106.3992821860680635, -28.18503700880033236, 24.56099125664901095 ) ) ;
#17458=VECTOR ( 'NONE', #40004, 1000.000000000000000 ) ;
#17459=CARTESIAN_POINT ( 'NONE',  ( 101.4133560641720067, -46.25507541695031222, 207.1622919425779514 ) ) ;
#17460=CARTESIAN_POINT ( 'NONE',  ( 117.6812658759005217, -39.72780374360938538, 143.6194347997209775 ) ) ;
#17461=DIRECTION ( 'NONE',  ( 0.000000000000000000, 0.000000000000000000, -1.000000000000000000 ) ) ;
#17462=CARTESIAN_POINT ( 'NONE',  ( 96.97881741550158097, -39.36031858868991407, 272.5299109901966972 ) ) ;
#17464=CARTESIAN_POINT ( 'NONE',  ( 164.7812970173241922, -35.65087443489296248, 313.9678068554149490 ) ) ;
#17465=ORIENTED_EDGE ( 'NONE', *, *, #68368, .F. ) ;
#17466=ORIENTED_EDGE ( 'NONE', *, *, #6672, .F. ) ;
#17467=VECTOR ( 'NONE', #58140, 1000.000000000000000 ) ;
#17468=CARTESIAN_POINT ( 'NONE',  ( 116.9264758816979537, -41.82782236628663242, 243.4346728949589647 ) ) ;
#17471=CARTESIAN_POINT ( 'NONE',  ( 97.38189020833135601, -42.05746220039552696, 176.7146728949589658 ) ) ;
#17472=CARTESIAN_POINT ( 'NONE',  ( 116.3216976867776964, -32.94060878512167534, 40.13562527591096796 ) ) ;
#17474=CARTESIAN_POINT ( 'NONE',  ( 46.83715912545343940, -47.82818131006086304, 129.9678068554150911 ) ) ;
#17478=DIRECTION ( 'NONE',  ( 0.000000000000000000, 1.000000000000000000, 0.000000000000000000 ) ) ;
#17479=CARTESIAN_POINT ( 'NONE',  ( 115.6772654923306902, -42.56752007954064965, 269.3527681330536439 ) ) ;
#17483=CARTESIAN_POINT ( 'NONE',  ( 25.56670390244722668, -42.82844715994178131, 134.7178068554150627 ) ) ;
#17484=EDGE_CURVE ( 'NONE', #51994, #29546, #11411, .T. ) ;
#17486=LINE ( 'NONE', #73330, #60424 ) ;
#17487=EDGE_CURVE ( 'NONE', #49481, #19751, #54146, .T. ) ;
#17488=CARTESIAN_POINT ( 'NONE',  ( 97.31584371105238063, -39.30597598001633486, 77.53145860767988040 ) ) ;
#17489=CARTESIAN_POINT ( 'NONE',  ( 110.2163081462844900, -44.10521182743453039, 195.5838068554167819 ) ) ;
#17491=EDGE_CURVE ( 'NONE', #66455, #50481, #27666, .T. ) ;
#17492=CARTESIAN_POINT ( 'NONE',  ( 136.6795104150337750, -19.60592655292144926, 6.943955837743826187 ) ) ;
#17493=CARTESIAN_POINT ( 'NONE',  ( 103.7160641590222809, -26.17150546779393494, 205.3089586092439731 ) ) ;
#17494=CARTESIAN_POINT ( 'NONE',  ( 104.7595845749942782, -46.89609389129499561, 68.39848241876794077 ) ) ;
#17495=CARTESIAN_POINT ( 'NONE',  ( 97.05457585776278506, -41.52102392564493272, 212.6937205140059461 ) ) ;
#17496=CARTESIAN_POINT ( 'NONE',  ( 33.92127028473601769, -29.73316016639540749, 237.4678068554150059 ) ) ;
#17498=DIRECTION ( 'NONE',  ( 1.000000000000000078E-15, -1.000000000000000083E-30, -1.000000000000000000 ) ) ;
#17499=CARTESIAN_POINT ( 'NONE',  ( 97.91933391361872907, -40.77183597370108004, 37.65731701089936223 ) ) ;
#17500=CARTESIAN_POINT ( 'NONE',  ( 84.06648329127399677, -18.72966777111500036, 239.5838068554169809 ) ) ;
#17501=LINE ( 'NONE', #38375, #26720 ) ;
#17503=CARTESIAN_POINT ( 'NONE',  ( 99.09629730216126120, -30.54963492062786656, 65.80361837691383187 ) ) ;
#17506=ORIENTED_EDGE ( 'NONE', *, *, #60447, .T. ) ;
#17507=CARTESIAN_POINT ( 'NONE',  ( 98.01892258562502036, -37.12227740767932715, 115.7714674471239675 ) ) ;
#17508=CYLINDRICAL_SURFACE ( 'NONE', #6714, 11.45913725231036118 ) ;
#17509=VERTEX_POINT ( 'NONE', #48694 ) ;
#17510=CARTESIAN_POINT ( 'NONE',  ( 96.81317962367450036, -38.48968277746985933, 87.46133956162493917 ) ) ;
#17511=EDGE_CURVE ( 'NONE', #33965, #19776, #77326, .T. ) ;
#17516=CARTESIAN_POINT ( 'NONE',  ( 77.53258422225751190, -17.66080143920404666, 7.039723185228972113 ) ) ;
#17517=FACE_OUTER_BOUND ( 'NONE', #35623, .T. ) ;
#17518=CARTESIAN_POINT ( 'NONE',  ( 111.8051047218221896, -27.50533234054179843, 19.71086337114996567 ) ) ;
#17520=ORIENTED_EDGE ( 'NONE', *, *, #11323, .T. ) ;
#17523=CARTESIAN_POINT ( 'NONE',  ( 76.06670390244799762, -26.72944715994109899, 199.5838068554169524 ) ) ;
#17524=DIRECTION ( 'NONE',  ( 0.000000000000000000, 0.000000000000000000, 1.000000000000000000 ) ) ;
#17525=DIRECTION ( 'NONE',  ( -0.9254794337955620787, -0.3787978585227822492, 0.000000000000000000 ) ) ;
#17526=LINE ( 'NONE', #45206, #26673 ) ;
#17527=LINE ( 'NONE', #17957, #73689 ) ;
#17530=CARTESIAN_POINT ( 'NONE',  ( 90.44969454456408187, -16.81243780205710436, 239.5838068554175209 ) ) ;
#17534=CARTESIAN_POINT ( 'NONE',  ( 96.94236579736387682, -32.35154040576531997, 61.01372051400599616 ) ) ;
#17536=ORIENTED_EDGE ( 'NONE', *, *, #52510, .T. ) ;
#17537=EDGE_CURVE ( 'NONE', #63665, #80398, #68335, .T. ) ;
#17539=CARTESIAN_POINT ( 'NONE',  ( 80.06648329127402519, -46.72944715994105991, 4.925625275910944012 ) ) ;
#17542=CARTESIAN_POINT ( 'NONE',  ( 111.3099657731024337, -28.47785412639777647, 167.5166617981629713 ) ) ;
#17543=AXIS2_PLACEMENT_3D ( 'NONE', #15566, #51386, #44580 ) ;
#17544=LINE ( 'NONE', #12517, #3976 ) ;
#17545=ORIENTED_EDGE ( 'NONE', *, *, #54603, .F. ) ;
#17550=DIRECTION ( 'NONE',  ( -0.9254794337955620787, -0.3787978585227822492, 0.000000000000000000 ) ) ;
#17551=VECTOR ( 'NONE', #72905, 999.9999999999998863 ) ;
#17552=CARTESIAN_POINT ( 'NONE',  ( 112.6928898907800090, -44.25407833457246909, 184.5311071154209799 ) ) ;
#17554=AXIS2_PLACEMENT_3D ( 'NONE', #80491, #72778, #10545 ) ;
#17555=DIRECTION ( 'NONE',  ( 0.000000000000000000, 0.000000000000000000, 1.000000000000000000 ) ) ;
#17556=CARTESIAN_POINT ( 'NONE',  ( 110.8778075460668617, -45.97466301617711792, 17.88763232902943301 ) ) ;
#17557=VERTEX_POINT ( 'NONE', #35525 ) ;
#17560=ORIENTED_EDGE ( 'NONE', *, *, #61272, .T. ) ;
#17561=CARTESIAN_POINT ( 'NONE',  ( 116.3142130228717264, -37.48801553205211690, 186.5795189410199555 ) ) ;
#17562=CARTESIAN_POINT ( 'NONE',  ( 96.61701384456422659, -37.56428313387978335, 101.3899109901969524 ) ) ;
#17563=CARTESIAN_POINT ( 'NONE',  ( 116.7246412902989903, -32.86309880586077270, 54.12991099019698282 ) ) ;
#17564=CARTESIAN_POINT ( 'NONE',  ( 115.0348970223676872, -42.91145613756582833, 253.3023792191510495 ) ) ;
#17567=CARTESIAN_POINT ( 'NONE',  ( 103.8073934974285066, -26.82688076304711444, 161.3299109901969643 ) ) ;
#17569=ORIENTED_EDGE ( 'NONE', *, *, #4425, .T. ) ;
#17570=CARTESIAN_POINT ( 'NONE',  ( 151.5667039024483245, -48.82844715993591223, 300.4678068554149490 ) ) ;
#17571=VERTEX_POINT ( 'NONE', #29621 ) ;
#17574=CARTESIAN_POINT ( 'NONE',  ( 97.81168895331838087, -40.51742574516882200, 287.6356252759109680 ) ) ;
#17579=ORIENTED_EDGE ( 'NONE', *, *, #20266, .F. ) ;
#17581=CARTESIAN_POINT ( 'NONE',  ( 104.7595363604009435, -46.89630637601933927, 72.39848241876795498 ) ) ;
#17585=DIRECTION ( 'NONE',  ( 0.000000000000000000, -1.000000000000000000, 0.000000000000000000 ) ) ;
#17586=EDGE_CURVE ( 'NONE', #49295, #26572, #77027, .T. ) ;
#17587=CARTESIAN_POINT ( 'NONE',  ( 102.0418483691416469, -28.29933337693050532, 85.50419670448295051 ) ) ;
#17589=CARTESIAN_POINT ( 'NONE',  ( 103.5497706991577189, -26.90106182813410740, 186.3499109901969746 ) ) ;
#17591=CARTESIAN_POINT ( 'NONE',  ( 107.0664832912739541, -36.72944715994095333, 305.7008218191032256 ) ) ;
#17593=VECTOR ( 'NONE', #49965, 1000.000000000000000 ) ;
#17594=DIRECTION ( 'NONE',  ( 0.000000000000000000, 0.000000000000000000, -1.000000000000000000 ) ) ;
#17595=ADVANCED_FACE ( 'NONE', ( #17339 ), #85949, .F. ) ;
#17596=CARTESIAN_POINT ( 'NONE',  ( 74.38348329127296665, -1.929447159941392931, 361.9756252759109998 ) ) ;
#17597=CARTESIAN_POINT ( 'NONE',  ( 97.81469011401388514, -40.51612824417846070, 136.6360017533206417 ) ) ;
#17600=FACE_OUTER_BOUND ( 'NONE', #42409, .T. ) ;
#17601=CARTESIAN_POINT ( 'NONE',  ( 108.1864980337677764, -47.13868502929719284, 202.6613395616249704 ) ) ;
#17602=ORIENTED_EDGE ( 'NONE', *, *, #32291, .F. ) ;
#17603=DIRECTION ( 'NONE',  ( 0.8571673007021091140, -8.250245410175212261E-16, 0.5150380749100597066 ) ) ;
#17604=CARTESIAN_POINT ( 'NONE',  ( 106.1364166314141499, -47.76666518589912869, 258.4975300378158636 ) ) ;
#17605=CARTESIAN_POINT ( 'NONE',  ( 113.3575164265628672, -45.09699625868619677, 139.0899109901969553 ) ) ;
#17606=PLANE ( 'NONE',  #7017 ) ;
#17607=CARTESIAN_POINT ( 'NONE',  ( 82.76352869194737139, -37.26660482608630076, 6.827192804309592411 ) ) ;
#17608=DIRECTION ( 'NONE',  ( -3.999999999999999995E-14, 1.000000000000000000, -4.100000000000000342E-29 ) ) ;
#17610=ORIENTED_EDGE ( 'NONE', *, *, #70053, .T. ) ;
#17612=ORIENTED_EDGE ( 'NONE', *, *, #86231, .T. ) ;
#17613=ORIENTED_EDGE ( 'NONE', *, *, #25792, .F. ) ;
#17614=CONICAL_SURFACE ( 'NONE', #68383, 5.800000000000000711, 0.7853981633974476129 ) ;
#17617=CARTESIAN_POINT ( 'NONE',  ( 118.3409026158823281, -33.07932318167559060, 280.0756252759109657 ) ) ;
#17618=DIRECTION ( 'NONE',  ( 1.000000000000000078E-15, -1.000000000000000083E-30, -1.000000000000000000 ) ) ;
#17619=DIRECTION ( 'NONE',  ( 1.000000000000000000, -5.337610695313248426E-16, 0.000000000000000000 ) ) ;
#17620=ADVANCED_FACE ( 'NONE', ( #1480 ), #15560, .F. ) ;
#17621=DIRECTION ( 'NONE',  ( 1.000000000000000000, 3.999999999999999995E-14, -4.193851878741028267E-47 ) ) ;
#17623=CIRCLE ( 'NONE', #58266, 16.00000000000000000 ) ;
#17624=CARTESIAN_POINT ( 'NONE',  ( 115.9822952273240304, -35.14169155943780964, 198.3771817328379825 ) ) ;
#17625=EDGE_LOOP ( 'NONE', ( #6405, #75395 ) ) ;
#17630=CARTESIAN_POINT ( 'NONE',  ( 116.3212776292296127, -32.94146857471318413, 287.6356252759109680 ) ) ;
#17631=CARTESIAN_POINT ( 'NONE',  ( 97.81555862303321192, -40.52686724714011746, 181.6364370671610118 ) ) ;
#17633=CARTESIAN_POINT ( 'NONE',  ( 111.4141554795631492, -28.97316737322958957, 31.10158330589696263 ) ) ;
#17635=DIRECTION ( 'NONE',  ( 0.000000000000000000, 0.000000000000000000, 1.000000000000000000 ) ) ;
#17636=CARTESIAN_POINT ( 'NONE',  ( 107.0664832912739968, -36.72944715994100306, 287.6356252759109680 ) ) ;
#17638=ORIENTED_EDGE ( 'NONE', *, *, #39096, .F. ) ;
#17641=ADVANCED_FACE ( 'NONE', ( #35986 ), #30518, .T. ) ;
#17643=CARTESIAN_POINT ( 'NONE',  ( 113.7275377883433549, -41.44750597731145092, 51.15380465530594734 ) ) ;
#17646=LINE ( 'NONE', #18077, #43195 ) ;
#17648=DIRECTION ( 'NONE',  ( 0.000000000000000000, 1.000000000000000000, 0.000000000000000000 ) ) ;
#17652=VERTEX_POINT ( 'NONE', #63699 ) ;
#17653=CARTESIAN_POINT ( 'NONE',  ( 98.33613682261365341, -42.42752411612296015, 101.7870538473399620 ) ) ;
#17654=ORIENTED_EDGE ( 'NONE', *, *, #1705, .F. ) ;
#17655=CARTESIAN_POINT ( 'NONE',  ( 107.5092159716399181, -46.42865411040452273, 42.03527697093395687 ) ) ;
#17656=VECTOR ( 'NONE', #27969, 1000.000000000000000 ) ;
#17657=CARTESIAN_POINT ( 'NONE',  ( 76.06670390244796920, -26.72944715994109899, 239.5838068554169809 ) ) ;
#17658=CARTESIAN_POINT ( 'NONE',  ( 99.90998525089342763, -42.81722683197487811, 73.33110711542096283 ) ) ;
#17661=PLANE ( 'NONE',  #21207 ) ;
#17663=CARTESIAN_POINT ( 'NONE',  ( 99.04917799727566319, -44.37196124675453746, 32.92038718067297509 ) ) ;
#17667=FACE_OUTER_BOUND ( 'NONE', #43199, .T. ) ;
#17668=ORIENTED_EDGE ( 'NONE', *, *, #57985, .F. ) ;
#17669=CARTESIAN_POINT ( 'NONE',  ( 77.96454488116506809, -20.51222316633940679, 2.376608873914837439 ) ) ;
#17670=ORIENTED_EDGE ( 'NONE', *, *, #47105, .T. ) ;
#17671=ORIENTED_EDGE ( 'NONE', *, *, #67570, .T. ) ;
#17673=ORIENTED_EDGE ( 'NONE', *, *, #51338, .T. ) ;
#17674=CARTESIAN_POINT ( 'NONE',  ( 116.7732407090126827, -35.28285290846962141, 218.9441967044829482 ) ) ;
#17675=DIRECTION ( 'NONE',  ( 6.745093096447288888E-17, 1.000000000000000000, 0.000000000000000000 ) ) ;
#17676=CARTESIAN_POINT ( 'NONE',  ( 105.7154772411971209, -46.72385838089639520, 188.4689586021422087 ) ) ;
#17677=CARTESIAN_POINT ( 'NONE',  ( 101.9605410436089699, -27.64034152677590583, 56.48419670448296159 ) ) ;
#17678=CARTESIAN_POINT ( 'NONE',  ( 97.83877808327316927, -40.58304141722473446, 42.64127468446370983 ) ) ;
#17680=CARTESIAN_POINT ( 'NONE',  ( 103.2774353142084038, -27.47509059510596074, 171.3857181134776226 ) ) ;
#17683=ORIENTED_EDGE ( 'NONE', *, *, #61112, .T. ) ;
#17685=DIRECTION ( 'NONE',  ( 5.512527431108029424E-15, -1.000000000000000000, 0.000000000000000000 ) ) ;
#17686=CARTESIAN_POINT ( 'NONE',  ( 109.6408376098527242, -46.48063368938936435, 113.7820702227787137 ) ) ;
#17687=CARTESIAN_POINT ( 'NONE',  ( 96.83034234600413015, -40.83861266248845823, 251.6422919425777138 ) ) ;
#17688=CARTESIAN_POINT ( 'NONE',  ( 177.4809174648213741, -49.32844715993478957, 300.4678068554149490 ) ) ;
#17689=EDGE_CURVE ( 'NONE', #27267, #2214, #78248, .T. ) ;
#17691=CARTESIAN_POINT ( 'NONE',  ( 77.53258422225754032, -37.79809288067778539, 2.811527366592890154 ) ) ;
#17692=EDGE_CURVE ( 'NONE', #80451, #19992, #29170, .T. ) ;
#17693=CARTESIAN_POINT ( 'NONE',  ( 110.8947914379136961, -29.09399076817903662, 279.1295626852197529 ) ) ;
#17695=CARTESIAN_POINT ( 'NONE',  ( 98.66494773507974969, -43.87633619481167102, 72.89943479972099283 ) ) ;
#17697=CARTESIAN_POINT ( 'NONE',  ( 116.9635770353169733, -33.20817898692279613, 114.0984824187679720 ) ) ;
#17702=EDGE_CURVE ( 'NONE', #60793, #45550, #57310, .T. ) ;
#17703=CARTESIAN_POINT ( 'NONE',  ( 172.5664832912729878, -27.82844715994070484, 138.9256252759119832 ) ) ;
#17705=DIRECTION ( 'NONE',  ( 0.000000000000000000, 1.000000000000000000, 0.000000000000000000 ) ) ;
#17706=ORIENTED_EDGE ( 'NONE', *, *, #20153, .F. ) ;
#17707=LINE ( 'NONE', #67183, #21574 ) ;
#17708=EDGE_CURVE ( 'NONE', #27001, #10481, #65482, .T. ) ;
#17709=CARTESIAN_POINT ( 'NONE',  ( 114.8040440383551157, -44.68828107661028781, 118.2022919425779719 ) ) ;
#17713=VECTOR ( 'NONE', #2418, 999.9999999999998863 ) ;
#17715=ORIENTED_EDGE ( 'NONE', *, *, #59116, .T. ) ;
#17718=CARTESIAN_POINT ( 'NONE',  ( 117.1850550582282580, -34.12927998004249730, 124.0270538473399426 ) ) ;
#17720=DIRECTION ( 'NONE',  ( 1.000000000000000000, 4.299999999999999979E-14, 1.000000000000000078E-15 ) ) ;
#17723=EDGE_CURVE ( 'NONE', #89397, #4393, #64594, .T. ) ;
#17724=ORIENTED_EDGE ( 'NONE', *, *, #59489, .T. ) ;
#17726=LINE ( 'NONE', #51325, #78826 ) ;
#17727=VECTOR ( 'NONE', #18707, 1000.000000000000114 ) ;
#17728=CARTESIAN_POINT ( 'NONE',  ( 107.0664832912739968, -36.72944715994100306, 287.6356252759109680 ) ) ;
#17729=CARTESIAN_POINT ( 'NONE',  ( 97.95250717983367394, -32.49412669507730556, 3.024967495036141596 ) ) ;
#17730=DIRECTION ( 'NONE',  ( 0.000000000000000000, 0.000000000000000000, -1.000000000000000000 ) ) ;
#17732=EDGE_LOOP ( 'NONE', ( #46371, #44226, #64199, #31171 ) ) ;
#17733=FACE_OUTER_BOUND ( 'NONE', #11346, .T. ) ;
#17734=CARTESIAN_POINT ( 'NONE',  ( 112.6571330189592430, -45.46348522128858605, 214.0175300378159591 ) ) ;
#17735=LINE ( 'NONE', #31800, #13922 ) ;
#17736=VERTEX_POINT ( 'NONE', #33196 ) ;
#17738=CARTESIAN_POINT ( 'NONE',  ( 97.54819157151555942, -32.61351373332772852, 57.01372051400599616 ) ) ;
#17739=CARTESIAN_POINT ( 'NONE',  ( 99.08981029112005956, -42.79583336390666659, 51.84399569144299136 ) ) ;
#17740=LINE ( 'NONE', #66317, #15210 ) ;
#17743=FACE_BOUND ( 'NONE', #37019, .T. ) ;
#17744=ORIENTED_EDGE ( 'NONE', *, *, #35761, .T. ) ;
#17745=VECTOR ( 'NONE', #732, 1000.000000000000000 ) ;
#17746=ORIENTED_EDGE ( 'NONE', *, *, #12991, .F. ) ;
#17747=ADVANCED_FACE ( 'NONE', ( #66359 ), #31845, .F. ) ;
#17748=CARTESIAN_POINT ( 'NONE',  ( 99.68253537205306714, -30.91964177047806217, 197.2396785439919711 ) ) ;
#17749=VECTOR ( 'NONE', #40204, 1000.000000000000000 ) ;
#17750=DIRECTION ( 'NONE',  ( 0.000000000000000000, 0.000000000000000000, 1.000000000000000000 ) ) ;
#17752=DIRECTION ( 'NONE',  ( -4.299999999999999979E-14, 1.000000000000000000, 0.000000000000000000 ) ) ;
#17754=ORIENTED_EDGE ( 'NONE', *, *, #67015, .F. ) ;
#17756=CARTESIAN_POINT ( 'NONE',  ( 31.56670390244800117, -33.35206098992711077, 342.9256252759109884 ) ) ;
#17757=ORIENTED_EDGE ( 'NONE', *, *, #49169, .F. ) ;
#17758=CARTESIAN_POINT ( 'NONE',  ( 113.7419942178973287, -29.10023054337252546, 289.5032443235301116 ) ) ;
#17762=CARTESIAN_POINT ( 'NONE',  ( 113.1782937666078510, -44.75186859622988322, 83.09395860877987161 ) ) ;
#17763=CARTESIAN_POINT ( 'NONE',  ( 124.9629318080292393, -56.47944715994101728, -5.074374724089012467 ) ) ;
#17764=CARTESIAN_POINT ( 'NONE',  ( 156.5667039024484666, -48.82844715993568485, 139.7178068554149775 ) ) ;
#17765=DIRECTION ( 'NONE',  ( 0.000000000000000000, 0.000000000000000000, -1.000000000000000000 ) ) ;
#17766=CARTESIAN_POINT ( 'NONE',  ( 101.4018018619443922, -46.27454447023805528, 203.1622919425779514 ) ) ;
#17768=ORIENTED_EDGE ( 'NONE', *, *, #11444, .T. ) ;
#17769=VECTOR ( 'NONE', #33875, 1000.000000000000000 ) ;
#17770=EDGE_CURVE ( 'NONE', #14401, #67672, #29639, .T. ) ;
#17771=CARTESIAN_POINT ( 'NONE',  ( 97.77052560236188583, -29.30002703792375485, 41.78991099019596334 ) ) ;
#17772=CARTESIAN_POINT ( 'NONE',  ( 194.5667039024479834, -67.87844715994100397, 310.9178068554150514 ) ) ;
#17773=VERTEX_POINT ( 'NONE', #87712 ) ;
#17774=ORIENTED_EDGE ( 'NONE', *, *, #42250, .T. ) ;
#17775=AXIS2_PLACEMENT_3D ( 'NONE', #56572, #715, #41586 ) ;
#17776=CARTESIAN_POINT ( 'NONE',  ( 82.16842210270853286, -16.94667169166570986, 2.376609173400793473 ) ) ;
#17777=DIRECTION ( 'NONE',  ( -4.237773401492740281E-14, 1.000000000000000000, 0.000000000000000000 ) ) ;
#17779=CARTESIAN_POINT ( 'NONE',  ( 98.14730025337767927, -34.17130281729839680, 138.9223760838769692 ) ) ;
#17780=CARTESIAN_POINT ( 'NONE',  ( 104.1798084317939725, -26.65242854998196265, 221.2984824187679465 ) ) ;
#17782=ORIENTED_EDGE ( 'NONE', *, *, #69912, .F. ) ;
#17785=ORIENTED_EDGE ( 'NONE', *, *, #27463, .T. ) ;
#17791=CARTESIAN_POINT ( 'NONE',  ( 162.7866693523280048, -29.62846900982320264, -5.074374724088000832 ) ) ;
#17793=CARTESIAN_POINT ( 'NONE',  ( 102.7266122873206768, -44.08618886718738139, 161.5752769709339702 ) ) ;
#17794=CARTESIAN_POINT ( 'NONE',  ( 113.7702145813751571, -29.06794043779556347, 289.5032443235301116 ) ) ;
#17796=CIRCLE ( 'NONE', #80125, 5.599999999999994316 ) ;
#17797=ADVANCED_FACE ( 'NONE', ( #87273 ), #81810, .T. ) ;
#17800=ORIENTED_EDGE ( 'NONE', *, *, #63562, .T. ) ;
#17801=CARTESIAN_POINT ( 'NONE',  ( 61.68306511546568061, -72.55869591834559174, 394.9756252759102040 ) ) ;
#17804=CARTESIAN_POINT ( 'NONE',  ( 163.0664832912739826, 12.92155284005902516, 333.4006252759110112 ) ) ;
#17805=CARTESIAN_POINT ( 'NONE',  ( 116.8177678418650771, -34.15541691211213760, 34.03146788054147720 ) ) ;
#17806=DIRECTION ( 'NONE',  ( 0.000000000000000000, 0.000000000000000000, -1.000000000000000000 ) ) ;
#17807=AXIS2_PLACEMENT_3D ( 'NONE', #43570, #29515, #71746 ) ;
#17810=CARTESIAN_POINT ( 'NONE',  ( 100.4651824673786393, -27.83460210401261747, 35.59657765686397113 ) ) ;
#17811=CARTESIAN_POINT ( 'NONE',  ( 111.4336192290781753, -46.24370506310440732, 23.91848241876792969 ) ) ;
#17813=LINE ( 'NONE', #3301, #60742 ) ;
#17815=CARTESIAN_POINT ( 'NONE',  ( 82.10814995794051185, 12.92155284005802685, 335.5992267699911054 ) ) ;
#17816=DIRECTION ( 'NONE',  ( 0.000000000000000000, 0.000000000000000000, -1.000000000000000000 ) ) ;
#17817=LINE ( 'NONE', #74127, #29571 ) ;
#17818=ADVANCED_FACE ( 'NONE', ( #80921 ), #4600, .F. ) ;
#17819=CARTESIAN_POINT ( 'NONE',  ( 107.0664832912739257, -50.72944715994096043, 315.1356252759112522 ) ) ;
#17822=CARTESIAN_POINT ( 'NONE',  ( 115.9827728363227664, -42.21636132903250171, 18.38705384733896153 ) ) ;
#17823=CARTESIAN_POINT ( 'NONE',  ( 117.7763469108053869, -31.65663365956905650, 210.1784824187679703 ) ) ;
#17824=CARTESIAN_POINT ( 'NONE',  ( 112.7535375185862705, -27.22457367525289129, 50.65943479972101215 ) ) ;
#17825=LINE ( 'NONE', #2423, #68219 ) ;
#17826=DIRECTION ( 'NONE',  ( 1.000000000000000000, 0.000000000000000000, 0.000000000000000000 ) ) ;
#17827=CARTESIAN_POINT ( 'NONE',  ( 80.06648329127401098, -33.97944715994105991, 1.625625275910943746 ) ) ;
#17831=ORIENTED_EDGE ( 'NONE', *, *, #18606, .T. ) ;
#17833=CARTESIAN_POINT ( 'NONE',  ( 117.3261810260835603, -38.23854875528750341, 69.72229194257801055 ) ) ;
#17834=CARTESIAN_POINT ( 'NONE',  ( 172.5664832912740110, -32.07844715994070839, 138.9256252759119832 ) ) ;
#17835=ORIENTED_EDGE ( 'NONE', *, *, #54579, .F. ) ;
#17837=CARTESIAN_POINT ( 'NONE',  ( 116.8642987764956160, -41.79567201640973195, 239.4346728949589647 ) ) ;
#17839=DIRECTION ( 'NONE',  ( -0.000000000000000000, 1.000000000000000000, 0.000000000000000000 ) ) ;
#17840=DIRECTION ( 'NONE',  ( 0.0001713722456127291687, -0.9999999853157766072, -1.713722456127291814E-19 ) ) ;
#17842=CARTESIAN_POINT ( 'NONE',  ( 133.3217830637533439, -39.37853523628599106, 1.709393643968337706 ) ) ;
#17843=DIRECTION ( 'NONE',  ( 0.7071067811989691920, 0.7071067811741258424, -2.899137802813799626E-29 ) ) ;
#17844=CARTESIAN_POINT ( 'NONE',  ( 99.59366209610195142, -44.96145431533982162, 156.9899109901969609 ) ) ;
#17845=ORIENTED_EDGE ( 'NONE', *, *, #79684, .F. ) ;
#17848=CARTESIAN_POINT ( 'NONE',  ( 116.0163176773587708, -41.35234337494321721, 89.87872616303998541 ) ) ;
#17849=CARTESIAN_POINT ( 'NONE',  ( 107.0664832912739968, -36.72944715994100306, 287.6356252759109680 ) ) ;
#17850=CARTESIAN_POINT ( 'NONE',  ( 118.0655259830058270, -38.35211242607483939, 219.7099109901959935 ) ) ;
#17851=CARTESIAN_POINT ( 'NONE',  ( 168.0371591254543375, -48.62818131005509770, 300.4678068554149490 ) ) ;
#17852=CIRCLE ( 'NONE', #58500, 0.5000000000000004441 ) ;
#17854=LINE ( 'NONE', #46433, #4603 ) ;
#17856=CARTESIAN_POINT ( 'NONE',  ( 194.5667039024483529, -47.82844715993405771, 249.9678068554149775 ) ) ;
#17860=DIRECTION ( 'NONE',  ( 0.000000000000000000, 0.000000000000000000, -1.000000000000000000 ) ) ;
#17861=CARTESIAN_POINT ( 'NONE',  ( 103.8142050530422438, -26.84757730287814326, 165.3299109901969643 ) ) ;
#17862=VERTEX_POINT ( 'NONE', #19118 ) ;
#17868=AXIS2_PLACEMENT_3D ( 'NONE', #75616, #28334, #70134 ) ;
#17869=EDGE_CURVE ( 'NONE', #83824, #7721, #32067, .T. ) ;
#17870=DIRECTION ( 'NONE',  ( 4.299999999999999979E-14, -1.000000000000000000, 0.000000000000000000 ) ) ;
#17871=CARTESIAN_POINT ( 'NONE',  ( 96.05373888820416539, -35.78152935435744553, 186.2461014663869889 ) ) ;
#17873=ORIENTED_EDGE ( 'NONE', *, *, #35940, .F. ) ;
#17874=ORIENTED_EDGE ( 'NONE', *, *, #80174, .F. ) ;
#17876=CARTESIAN_POINT ( 'NONE',  ( 106.2078554787763522, -46.73095241849994608, 63.50879164150141776 ) ) ;
#17877=CARTESIAN_POINT ( 'NONE',  ( 142.8698897858160706, -0.9167816978817300289, 396.9756252759102040 ) ) ;
#17879=CARTESIAN_POINT ( 'NONE',  ( 103.6908924260029607, -28.08645471411401928, 18.19094751244793073 ) ) ;
#17880=EDGE_CURVE ( 'NONE', #87303, #11589, #10954, .T. ) ;
#17881=LINE ( 'NONE', #38765, #69594 ) ;
#17882=ORIENTED_EDGE ( 'NONE', *, *, #4708, .T. ) ;
#17884=CARTESIAN_POINT ( 'NONE',  ( 182.5667039024469886, -33.35206098992650681, 117.4678068554150627 ) ) ;
#17886=ORIENTED_EDGE ( 'NONE', *, *, #32967, .T. ) ;
#17889=VERTEX_POINT ( 'NONE', #69964 ) ;
#17890=VERTEX_POINT ( 'NONE', #83598 ) ;
#17891=DIRECTION ( 'NONE',  ( 0.000000000000000000, 0.000000000000000000, 1.000000000000000000 ) ) ;
#17893=CARTESIAN_POINT ( 'NONE',  ( 113.4185696802295809, -42.43971249784851096, 37.66670554236295487 ) ) ;
#17894=CARTESIAN_POINT ( 'NONE',  ( 96.65194983638532733, -35.53535514585328059, 206.2356252759109623 ) ) ;
#17895=CARTESIAN_POINT ( 'NONE',  ( 97.69433714244404143, -41.24514667321086847, 171.6841967044819626 ) ) ;
#17896=CARTESIAN_POINT ( 'NONE',  ( 107.3864418959535527, -26.30668689864625875, 322.4523926293242653 ) ) ;
#17897=CARTESIAN_POINT ( 'NONE',  ( 110.8926193997603065, -26.99384161864454157, 265.7784824187680783 ) ) ;
#17899=ADVANCED_FACE ( 'NONE', ( #68172 ), #5953, .T. ) ;
#17901=ORIENTED_EDGE ( 'NONE', *, *, #70688, .F. ) ;
#17903=CARTESIAN_POINT ( 'NONE',  ( 97.81169822462854313, -40.51742973538109993, 111.6355314416972391 ) ) ;
#17904=CARTESIAN_POINT ( 'NONE',  ( 113.8278214188052999, -26.93592357317604424, 239.5956252759109759 ) ) ;
#17905=VERTEX_POINT ( 'NONE', #40892 ) ;
#17906=CARTESIAN_POINT ( 'NONE',  ( 107.6545119506432258, -47.76725988480858121, 197.6308633711489620 ) ) ;
#17908=AXIS2_PLACEMENT_3D ( 'NONE', #7124, #36170, #14845 ) ;
#17909=CARTESIAN_POINT ( 'NONE',  ( 138.0667039024479834, -26.72944715994091069, 199.5838068554170093 ) ) ;
#17910=CARTESIAN_POINT ( 'NONE',  ( 91.06648329127391150, -36.72944715993925513, -5.074374724089045330 ) ) ;
#17911=LINE ( 'NONE', #4741, #70311 ) ;
#17914=CARTESIAN_POINT ( 'NONE',  ( 116.2977993645975232, -41.52656014244012539, 284.4441967044824082 ) ) ;
#17916=DIRECTION ( 'NONE',  ( -4.299999999999999979E-14, 1.000000000000000000, 0.000000000000000000 ) ) ;
#17918=EDGE_CURVE ( 'NONE', #4456, #18085, #75438, .T. ) ;
#17919=VECTOR ( 'NONE', #28683, 1000.000000000000000 ) ;
#17924=CARTESIAN_POINT ( 'NONE',  ( 114.8707465414360058, -39.51320248554598180, 195.5838068554167251 ) ) ;
#17926=CARTESIAN_POINT ( 'NONE',  ( 134.8178230081367133, -21.40255221908221372, 8.160479982092603279 ) ) ;
#17927=CARTESIAN_POINT ( 'NONE',  ( 113.6281634912633223, -45.65356023013480780, 183.0689586092439640 ) ) ;
#17928=CARTESIAN_POINT ( 'NONE',  ( 97.54238320567634446, -32.48987111900922997, 96.99276813305395706 ) ) ;
#17929=CARTESIAN_POINT ( 'NONE',  ( 117.5177603787924170, -36.12629959281294134, 224.8727681330539667 ) ) ;
#17930=CARTESIAN_POINT ( 'NONE',  ( 163.0664832912739826, -0.7548456658610993575, 331.7756252759120343 ) ) ;
#17932=CARTESIAN_POINT ( 'NONE',  ( 156.5667039024485518, -48.82844715993568485, 170.7178068554149775 ) ) ;
#17933=CARTESIAN_POINT ( 'NONE',  ( 98.03457007761814168, -41.02703092026990817, 37.67959706312523593 ) ) ;
#17934=CARTESIAN_POINT ( 'NONE',  ( 150.5667039024482960, -47.82844715993594775, 300.4678068554149490 ) ) ;
#17937=CARTESIAN_POINT ( 'NONE',  ( 97.79642245614456897, -40.47996586491548499, 66.63287571918958463 ) ) ;
#17939=ORIENTED_EDGE ( 'NONE', *, *, #60959, .T. ) ;
#17940=CARTESIAN_POINT ( 'NONE',  ( 98.52552435659306695, -36.63915763587115038, 110.7409912566489680 ) ) ;
#17941=DIRECTION ( 'NONE',  ( 0.000000000000000000, 1.000000000000000000, 0.000000000000000000 ) ) ;
#17942=ORIENTED_EDGE ( 'NONE', *, *, #50924, .F. ) ;
#17943=CARTESIAN_POINT ( 'NONE',  ( 96.11054930851091171, -38.00668368623056637, 82.43086337114895912 ) ) ;
#17944=CARTESIAN_POINT ( 'NONE',  ( 105.8881231706732962, -26.36991942434103819, 322.4846826458744431 ) ) ;
#17947=CARTESIAN_POINT ( 'NONE',  ( 115.0372575083174524, -42.90846256421102822, 109.3022919428230182 ) ) ;
#17948=CARTESIAN_POINT ( 'NONE',  ( 117.4022237771662276, -37.57280582802028590, 38.77372051400595865 ) ) ;
#17949=ORIENTED_EDGE ( 'NONE', *, *, #5222, .F. ) ;
#17950=VERTEX_POINT ( 'NONE', #89516 ) ;
#17951=ORIENTED_EDGE ( 'NONE', *, *, #2813, .T. ) ;
#17952=VECTOR ( 'NONE', #23324, 1000.000000000000000 ) ;
#17954=CARTESIAN_POINT ( 'NONE',  ( 117.0231039428182385, -39.62849705588580917, 134.5889586092439743 ) ) ;
#17955=DIRECTION ( 'NONE',  ( -0.7071067811865187069, -0.7071067811865764385, -7.071067811865181482E-16 ) ) ;
#17957=CARTESIAN_POINT ( 'NONE',  ( 71.06648329127399677, -18.82844715994099971, 17.92562527591199739 ) ) ;
#17960=CARTESIAN_POINT ( 'NONE',  ( 188.5667039024485518, -48.82844715993430640, 170.7178068554150059 ) ) ;
#17962=DIRECTION ( 'NONE',  ( -1.000000000000000000, -2.756263715554006823E-15, 0.000000000000000000 ) ) ;
#17963=CARTESIAN_POINT ( 'NONE',  ( 96.73644666290614680, -38.23103596604165944, 66.44133956162495735 ) ) ;
#17965=EDGE_LOOP ( 'NONE', ( #29754, #51494, #5620, #89830 ) ) ;
#17967=FACE_OUTER_BOUND ( 'NONE', #86658, .T. ) ;
#17969=CARTESIAN_POINT ( 'NONE',  ( 112.1934831763302896, -30.37778608165438854, 162.3538046553059644 ) ) ;
#17970=EDGE_CURVE ( 'NONE', #5764, #34865, #24818, .T. ) ;
#17971=AXIS2_PLACEMENT_3D ( 'NONE', #20071, #6002, #68220 ) ;
#17974=ORIENTED_EDGE ( 'NONE', *, *, #61376, .T. ) ;
#17976=EDGE_CURVE ( 'NONE', #48576, #33376, #61334, .T. ) ;
#17977=CARTESIAN_POINT ( 'NONE',  ( 33.78129701733065815, -35.65087443492598140, 342.9256252759109884 ) ) ;
#17980=ORIENTED_EDGE ( 'NONE', *, *, #86116, .F. ) ;
#17982=ADVANCED_FACE ( 'NONE', ( #6830 ), #89061, .T. ) ;
#17983=CARTESIAN_POINT ( 'NONE',  ( 108.6634326348915351, -27.98234008310821608, 161.3644404487539816 ) ) ;
#17986=FACE_OUTER_BOUND ( 'NONE', #57390, .T. ) ;
#17987=EDGE_CURVE ( 'NONE', #21680, #79544, #82264, .T. ) ;
#17989=EDGE_LOOP ( 'NONE', ( #80834, #14852, #18785, #73172, #80311, #36282 ) ) ;
#17990=ORIENTED_EDGE ( 'NONE', *, *, #12666, .F. ) ;
#17994=CARTESIAN_POINT ( 'NONE',  ( 115.1682430951150735, -35.73384980259207566, 191.7423760838769908 ) ) ;
#17995=CARTESIAN_POINT ( 'NONE',  ( 108.5410937779726623, -26.38672566707733225, 104.9641967044819779 ) ) ;
#17996=CARTESIAN_POINT ( 'NONE',  ( 101.0787430638808928, -27.46603582566399027, 70.54514908543497143 ) ) ;
#17997=CARTESIAN_POINT ( 'NONE',  ( 99.04379977427080917, -42.84086283679705076, 251.8441986198212703 ) ) ;
#17999=CARTESIAN_POINT ( 'NONE',  ( 107.9025279714727787, -25.30072614498174488, 322.7599154420194623 ) ) ;
#18000=CARTESIAN_POINT ( 'NONE',  ( 95.91002759172351944, -32.73343517516348555, 172.0527681330539735 ) ) ;
#18003=ORIENTED_EDGE ( 'NONE', *, *, #34700, .T. ) ;
#18004=CARTESIAN_POINT ( 'NONE',  ( 49.21437657594998427, -35.91149509761070391, 313.9678068554150059 ) ) ;
#18005=ORIENTED_EDGE ( 'NONE', *, *, #21294, .F. ) ;
#18007=CARTESIAN_POINT ( 'NONE',  ( 192.5667039024472444, -23.42844715993434335, 300.4678068554149490 ) ) ;
#18008=VERTEX_POINT ( 'NONE', #918 ) ;
#18012=ORIENTED_EDGE ( 'NONE', *, *, #78784, .F. ) ;
#18014=CARTESIAN_POINT ( 'NONE',  ( 95.34890500915419409, -34.95776856631113105, 71.20705384733993526 ) ) ;
#18016=VECTOR ( 'NONE', #11888, 1000.000000000000000 ) ;
#18017=DIRECTION ( 'NONE',  ( 0.000000000000000000, 0.000000000000000000, 1.000000000000000000 ) ) ;
#18019=CARTESIAN_POINT ( 'NONE',  ( 102.8368274790082921, -27.91052165842129185, 95.43276813305395478 ) ) ;
#18021=CARTESIAN_POINT ( 'NONE',  ( 96.06973772670292533, -35.87188691900273341, 187.2765776568629406 ) ) ;
#18022=CARTESIAN_POINT ( 'NONE',  ( 105.7963566878966191, -26.72446537362054286, 60.17754341170855525 ) ) ;
#18023=CARTESIAN_POINT ( 'NONE',  ( 41.56648329127399677, -18.82844715994099971, 201.0426252759120018 ) ) ;
#18025=LINE ( 'NONE', #52954, #77426 ) ;
#18026=EDGE_CURVE ( 'NONE', #78421, #55155, #20475, .T. ) ;
#18027=CARTESIAN_POINT ( 'NONE',  ( 20.03715912545639100, -24.42818131006202265, 180.4678068554150911 ) ) ;
#18029=CARTESIAN_POINT ( 'NONE',  ( 48.85858412958099706, -30.08671355700241179, -5.074374724088000832 ) ) ;
#18030=EDGE_CURVE ( 'NONE', #71705, #81882, #75603, .T. ) ;
#18032=CARTESIAN_POINT ( 'NONE',  ( 116.5668037432639608, -41.21227053747742985, 228.4756252759109714 ) ) ;
#18034=CARTESIAN_POINT ( 'NONE',  ( 132.0248166246069843, 12.92155284005802685, 335.5992267699912190 ) ) ;
#18035=CARTESIAN_POINT ( 'NONE',  ( 114.4303731589454998, -27.41304352248915777, 270.5441967044823741 ) ) ;
#18036=CARTESIAN_POINT ( 'NONE',  ( 108.3246818025246654, -47.12222909040148267, 113.6727681330539639 ) ) ;
#18037=EDGE_CURVE ( 'NONE', #44520, #47420, #82875, .T. ) ;
#18038=DIRECTION ( 'NONE',  ( 1.000000000000000000, 4.163336342344333240E-14, 0.000000000000000000 ) ) ;
#18040=FACE_OUTER_BOUND ( 'NONE', #53598, .T. ) ;
#18041=CARTESIAN_POINT ( 'NONE',  ( 115.7825805894831888, -41.80319946571558631, 264.4065922469304724 ) ) ;
#18042=ORIENTED_EDGE ( 'NONE', *, *, #2308, .F. ) ;
#18044=CIRCLE ( 'NONE', #86265, 1.000000000000000888 ) ;
#18045=AXIS2_PLACEMENT_3D ( 'NONE', #48985, #78538, #863 ) ;
#18047=ORIENTED_EDGE ( 'NONE', *, *, #14013, .F. ) ;
#18049=VECTOR ( 'NONE', #23351, 1000.000000000000000 ) ;
#18052=CARTESIAN_POINT ( 'NONE',  ( 97.55999611477783162, -43.80484941858547643, 257.8356252759109566 ) ) ;
#18056=CARTESIAN_POINT ( 'NONE',  ( 108.4181602030399461, -26.73512120126024882, 149.9692933348216854 ) ) ;
#18057=CARTESIAN_POINT ( 'NONE',  ( 109.1470148533826432, -28.41539336262556503, 199.3038483995049717 ) ) ;
#18058=ORIENTED_EDGE ( 'NONE', *, *, #3137, .T. ) ;
#18060=VERTEX_POINT ( 'NONE', #14561 ) ;
#18061=DIRECTION ( 'NONE',  ( -0.7071067811987160612, -0.7071067811743789733, 0.000000000000000000 ) ) ;
#18062=CARTESIAN_POINT ( 'NONE',  ( 110.9568920020971348, -45.94175259203705508, 182.8944488436118831 ) ) ;
#18064=CARTESIAN_POINT ( 'NONE',  ( 109.2301907924558009, -26.89130329018268739, 26.33586902018297948 ) ) ;
#18066=DIRECTION ( 'NONE',  ( 0.7071067811862258301, -0.7071067811868692043, 7.071067811862265655E-16 ) ) ;
#18067=CARTESIAN_POINT ( 'NONE',  ( 179.1667039024477504, -28.27351298636770949, 117.4678068554150627 ) ) ;
#18068=ORIENTED_EDGE ( 'NONE', *, *, #9718, .T. ) ;
#18069=CARTESIAN_POINT ( 'NONE',  ( 115.1583939375015291, -30.74836612253984569, 55.33262535118461045 ) ) ;
#18072=CARTESIAN_POINT ( 'NONE',  ( 99.45988105884268293, -33.69262468827373169, 38.84237608387697094 ) ) ;
#18073=CONICAL_SURFACE ( 'NONE', #21007, 3.299999999999999822, 0.7853981633974602694 ) ;
#18074=CARTESIAN_POINT ( 'NONE',  ( 136.4578062354350152, -17.36823420010915342, 7.200493380636948437 ) ) ;
#18075=AXIS2_PLACEMENT_3D ( 'NONE', #88544, #67181, #53522 ) ;
#18076=ADVANCED_FACE ( 'NONE', ( #76320 ), #14099, .F. ) ;
#18077=CARTESIAN_POINT ( 'NONE',  ( 80.54920390244802775, -51.22944715994108833, 231.5838068554169524 ) ) ;
#18078=CARTESIAN_POINT ( 'NONE',  ( 108.3333593921743301, -46.73486949315721262, 193.6772316444348974 ) ) ;
#18081=EDGE_CURVE ( 'NONE', #9481, #36458, #51276, .T. ) ;
#18083=VERTEX_POINT ( 'NONE', #35877 ) ;
#18084=CARTESIAN_POINT ( 'NONE',  ( 98.45613130301506999, -42.66979608177781813, 126.8070538473389490 ) ) ;
#18085=VERTEX_POINT ( 'NONE', #79023 ) ;
#18086=CARTESIAN_POINT ( 'NONE',  ( 106.8818968526635160, -46.43699862984655624, 76.98384839950495007 ) ) ;
#18087=ADVANCED_FACE ( 'NONE', ( #8184 ), #72200, .F. ) ;
#18089=CARTESIAN_POINT ( 'NONE',  ( 107.2828545668587878, -27.33638008851531609, 71.47777378208797927 ) ) ;
#18091=DIRECTION ( 'NONE',  ( 0.000000000000000000, 0.000000000000000000, -1.000000000000000000 ) ) ;
#18092=DIRECTION ( 'NONE',  ( 0.000000000000000000, 0.000000000000000000, 1.000000000000000000 ) ) ;
#18093=CARTESIAN_POINT ( 'NONE',  ( 117.5340331363998985, -37.28601590683526723, 14.78419670448294454 ) ) ;
#18094=LINE ( 'NONE', #45783, #30933 ) ;
#18102=VECTOR ( 'NONE', #74717, 1000.000000000000000 ) ;
#18105=EDGE_CURVE ( 'NONE', #74932, #11705, #84512, .T. ) ;
#18106=CIRCLE ( 'NONE', #74654, 29.00000000000000000 ) ;
#18107=VECTOR ( 'NONE', #86787, 1000.000000000000000 ) ;
#18109=CARTESIAN_POINT ( 'NONE',  ( 115.8019334949658798, -41.12891815432281817, 203.4556252759109611 ) ) ;
#18110=CARTESIAN_POINT ( 'NONE',  ( 116.1804594027163375, -40.96476762480074996, 25.56312527591098060 ) ) ;
#18111=DIRECTION ( 'NONE',  ( 0.000000000000000000, 0.000000000000000000, 1.000000000000000000 ) ) ;
#18112=CARTESIAN_POINT ( 'NONE',  ( 115.6731346838618464, -43.66482979471727077, 39.27467289495895386 ) ) ;
#18113=EDGE_CURVE ( 'NONE', #88467, #20221, #59671, .T. ) ;
#18114=LINE ( 'NONE', #58118, #85696 ) ;
#18115=VERTEX_POINT ( 'NONE', #56763 ) ;
#18117=FACE_OUTER_BOUND ( 'NONE', #11794, .T. ) ;
#18118=EDGE_CURVE ( 'NONE', #80487, #51959, #22269, .T. ) ;
#18119=VERTEX_POINT ( 'NONE', #15898 ) ;
#18122=CARTESIAN_POINT ( 'NONE',  ( 114.5897159479186342, -29.54407062678533791, 234.4327681330539690 ) ) ;
#18123=DIRECTION ( 'NONE',  ( 1.000000000000000000, 4.163336342344333240E-14, 0.000000000000000000 ) ) ;
#18124=VECTOR ( 'NONE', #83847, 1000.000000000000000 ) ;
#18125=DIRECTION ( 'NONE',  ( 1.000000000000000000, 0.000000000000000000, 0.000000000000000000 ) ) ;
#18126=CARTESIAN_POINT ( 'NONE',  ( 79.69020591994934932, -39.46022584114963649, 1.641799370504630984 ) ) ;
#18127=CARTESIAN_POINT ( 'NONE',  ( 116.5602560931381220, -38.76387722282552062, 258.0809912566484741 ) ) ;
#18129=CARTESIAN_POINT ( 'NONE',  ( 101.0787430638809496, -27.46603582566407908, 66.54514908543495721 ) ) ;
#18131=CARTESIAN_POINT ( 'NONE',  ( 98.16479183632776540, -43.36064410082828857, 111.8480062282919647 ) ) ;
#18132=VERTEX_POINT ( 'NONE', #71758 ) ;
#18136=DIRECTION ( 'NONE',  ( -1.000000000000000078E-15, 1.000000000000000083E-30, 1.000000000000000000 ) ) ;
#18139=ADVANCED_FACE ( 'NONE', ( #21824, #85846 ), #8641, .T. ) ;
#18140=PLANE ( 'NONE',  #49093 ) ;
#18141=CARTESIAN_POINT ( 'NONE',  ( 112.5373769503831625, -27.80330641407773840, 94.63848241876793566 ) ) ;
#18143=CYLINDRICAL_SURFACE ( 'NONE', #71217, 4.875000000000017764 ) ;
#18144=ADVANCED_FACE ( 'NONE', ( #64047, #1824 ), #23183, .T. ) ;
#18145=FACE_OUTER_BOUND ( 'NONE', #36541, .T. ) ;
#18147=CARTESIAN_POINT ( 'NONE',  ( 123.6837132603318707, -21.37118780205705448, 218.8274735512161158 ) ) ;
#18149=CARTESIAN_POINT ( 'NONE',  ( 102.3504518276437523, -46.05175434220414132, 127.2041967044829960 ) ) ;
#18152=CARTESIAN_POINT ( 'NONE',  ( 107.0664832912730020, -36.72944715994189835, 342.9256252759109884 ) ) ;
#18153=CARTESIAN_POINT ( 'NONE',  ( 33.96670390244699433, -28.27351298637401200, -5.074374724088000832 ) ) ;
#18156=CARTESIAN_POINT ( 'NONE',  ( 62.03715912545749944, -47.82818131006020934, 180.4678068554151196 ) ) ;
#18159=DIRECTION ( 'NONE',  ( 0.7071067811865671127, 0.7071067811865279218, 7.071067811865664660E-16 ) ) ;
#18161=CARTESIAN_POINT ( 'NONE',  ( 97.80411235625082611, -40.49886499406813556, 181.6340295426134048 ) ) ;
#18162=ADVANCED_FACE ( 'NONE', ( #44020 ), #78139, .T. ) ;
#18163=VECTOR ( 'NONE', #85019, 1000.000000000000000 ) ;
#18164=ORIENTED_EDGE ( 'NONE', *, *, #86404, .F. ) ;
#18168=CARTESIAN_POINT ( 'NONE',  ( 113.1782938590851160, -44.75186852387405168, 34.09395861806017081 ) ) ;
#18169=CARTESIAN_POINT ( 'NONE',  ( 116.7742277529939230, -35.53649587948896027, 189.9241967044819717 ) ) ;
#18170=PLANE ( 'NONE',  #87831 ) ;
#18171=VERTEX_POINT ( 'NONE', #17236 ) ;
#18172=AXIS2_PLACEMENT_3D ( 'NONE', #20301, #47970, #62513 ) ;
#18173=CARTESIAN_POINT ( 'NONE',  ( 110.5640613610537883, -45.86347053068958246, 58.86705384733897972 ) ) ;
#18174=CARTESIAN_POINT ( 'NONE',  ( 97.81169138727440782, -40.51741131469341184, 51.63568823874075520 ) ) ;
#18175=DIRECTION ( 'NONE',  ( -0.7071067811874389708, 0.7071067811856560636, 0.000000000000000000 ) ) ;
#18176=AXIS2_PLACEMENT_3D ( 'NONE', #41567, #69302, #69750 ) ;
#18178=ORIENTED_EDGE ( 'NONE', *, *, #25773, .T. ) ;
#18180=VERTEX_POINT ( 'NONE', #79921 ) ;
#18183=EDGE_CURVE ( 'NONE', #4939, #38575, #81449, .T. ) ;
#18184=CARTESIAN_POINT ( 'NONE',  ( 107.4435086560219474, -45.58304137281263024, 234.0415833058969781 ) ) ;
#18185=CARTESIAN_POINT ( 'NONE',  ( 97.82697590662368725, -40.55461666880389515, 52.63840751606506529 ) ) ;
#18186=LINE ( 'NONE', #82234, #21794 ) ;
#18187=AXIS2_PLACEMENT_3D ( 'NONE', #12916, #4308, #89220 ) ;
#18189=EDGE_CURVE ( 'NONE', #23638, #9163, #52157, .T. ) ;
#18190=CARTESIAN_POINT ( 'NONE',  ( 25.56670390244797275, -62.87844715994099687, 139.9678068554150059 ) ) ;
#18192=VERTEX_POINT ( 'NONE', #24495 ) ;
#18194=ADVANCED_FACE ( 'NONE', ( #19012 ), #67607, .T. ) ;
#18195=CARTESIAN_POINT ( 'NONE',  ( 102.0622438148563873, -27.97331942483490508, 36.48982574705384252 ) ) ;
#18197=CARTESIAN_POINT ( 'NONE',  ( 111.7292870705843768, -27.42961193919077445, 279.7070538473396937 ) ) ;
#18200=CARTESIAN_POINT ( 'NONE',  ( 115.1064843935641022, -35.31944421942311862, 241.7823760838769545 ) ) ;
#18202=LINE ( 'NONE', #4582, #30045 ) ;
#18203=CARTESIAN_POINT ( 'NONE',  ( 162.7131505118679797, -31.94127993907790852, -5.074374724088000832 ) ) ;
#18205=CARTESIAN_POINT ( 'NONE',  ( 21.56670390244726576, -23.42844715994183957, 237.4678068554150059 ) ) ;
#18206=AXIS2_PLACEMENT_3D ( 'NONE', #32643, #73989, #87621 ) ;
#18207=CARTESIAN_POINT ( 'NONE',  ( 96.09249528944252461, -35.06539016137039511, 217.1946728949589840 ) ) ;
#18209=EDGE_CURVE ( 'NONE', #82784, #62066, #52456, .T. ) ;
#18210=ORIENTED_EDGE ( 'NONE', *, *, #52235, .F. ) ;
#18211=CARTESIAN_POINT ( 'NONE',  ( 97.18453276023305420, -31.67528530451021851, 91.96229194257693962 ) ) ;
#18212=CARTESIAN_POINT ( 'NONE',  ( 87.17003668186745813, -46.62589376934782592, 14.92562527591089783 ) ) ;
#18213=B_SPLINE_CURVE_WITH_KNOTS ( 'NONE', 3,
 ( #14763, #35629, #50599, #72406, #57415, #24246, #86041, #10167, #71073, #43332, #65577, #29721, #15652, #51916, #45111, #78340, #64244, #23810, #2470, #2018, #30165, #31049, #3359, #85151, #58314, #37877, #16103, #43781, #2912, #72838 ),
 .UNSPECIFIED., .F., .F.,
 ( 4, 2, 2, 2, 2, 2, 2, 2, 2, 2, 1, 1, 1, 1, 1, 1, 2, 4 ),
 ( 0.000000000000000000, 0.06250180076269364060, 0.1250036015253872812, 0.1875054022880809357, 0.2500072030507745624, 0.3125090038134681891, 0.3750108045761618714, 0.4375126053388554981, 0.4687635057202020894, 0.4843889559108754961, 0.4922016810062120884, 0.4961080435538803846, 0.4980612248277145326, 0.4990378154646316622, 0.4995261107830904490, 0.4997702584423199257, 0.4998923322719344697, 0.5000144061015490138 ),
 .UNSPECIFIED. ) ;
#18214=AXIS2_PLACEMENT_3D ( 'NONE', #15146, #14252, #83295 ) ;
#18215=EDGE_LOOP ( 'NONE', ( #22273, #7530, #4736, #87669, #68379, #59101, #5946, #59310, #88269, #5037, #15988, #19917, #34475, #22008, #87223, #39521, #1139, #45306, #72150, #17348, #10628, #52187, #40735, #9746, #2372, #49938 ) ) ;
#18217=ORIENTED_EDGE ( 'NONE', *, *, #51420, .F. ) ;
#18219=CARTESIAN_POINT ( 'NONE',  ( 82.51836309791794122, -17.48272428399696210, 2.716753546982734857 ) ) ;
#18220=CARTESIAN_POINT ( 'NONE',  ( 130.5667039024480118, -36.72944715994093912, 229.5838068554170093 ) ) ;
#18222=CARTESIAN_POINT ( 'NONE',  ( 108.7381085716129263, -28.73974155568626898, 137.7309475124479548 ) ) ;
#18223=CARTESIAN_POINT ( 'NONE',  ( 99.73785018541691727, -29.28442226721861275, 221.6956252759109702 ) ) ;
#18224=EDGE_CURVE ( 'NONE', #43116, #31632, #86721, .T. ) ;
#18226=VERTEX_POINT ( 'NONE', #54393 ) ;
#18227=CARTESIAN_POINT ( 'NONE',  ( 136.5411229421764006, -37.94037323192798539, 2.740176903235941097 ) ) ;
#18231=AXIS2_PLACEMENT_3D ( 'NONE', #33150, #54009, #40410 ) ;
#18233=VECTOR ( 'NONE', #39185, 1000.000000000000000 ) ;
#18234=VERTEX_POINT ( 'NONE', #61671 ) ;
#18238=DIRECTION ( 'NONE',  ( 0.000000000000000000, 1.000000000000000000, 0.000000000000000000 ) ) ;
#18239=CARTESIAN_POINT ( 'NONE',  ( 112.8906599442021275, -43.66427313951261624, 147.5428960185529661 ) ) ;
#18240=CARTESIAN_POINT ( 'NONE',  ( 111.0631195717115673, -47.08511319755631774, 17.85753003781598380 ) ) ;
#18244=CIRCLE ( 'NONE', #65893, 13.63963572536219715 ) ;
#18247=CARTESIAN_POINT ( 'NONE',  ( 97.22634975616455222, -34.77161965005227273, 167.1698970065834828 ) ) ;
#18250=CARTESIAN_POINT ( 'NONE',  ( 97.81168839172025287, -40.51739946886939947, 131.6358419732753475 ) ) ;
#18251=DIRECTION ( 'NONE',  ( 1.000000000000000078E-15, -1.000000000000000083E-30, -1.000000000000000000 ) ) ;
#18253=CARTESIAN_POINT ( 'NONE',  ( 116.3173282457959345, -41.53670860177669510, 288.4441967044823514 ) ) ;
#18254=CARTESIAN_POINT ( 'NONE',  ( 109.6225776363756950, -25.10716277166327615, 25.90419670448196143 ) ) ;
#18255=AXIS2_PLACEMENT_3D ( 'NONE', #16395, #71802, #44965 ) ;
#18259=CARTESIAN_POINT ( 'NONE',  ( 97.81399847929220925, -40.51646572127298640, 256.6355814287313137 ) ) ;
#18260=DIRECTION ( 'NONE',  ( 1.000000000000000078E-15, -1.000000000000000083E-30, -1.000000000000000000 ) ) ;
#18261=LINE ( 'NONE', #45940, #56144 ) ;
#18264=CARTESIAN_POINT ( 'NONE',  ( 112.9881877051661263, -28.09578728253486446, 44.59848241876795782 ) ) ;
#18265=CARTESIAN_POINT ( 'NONE',  ( 110.6962928707952756, -48.01036458606073865, 203.8241967044819489 ) ) ;
#18266=CARTESIAN_POINT ( 'NONE',  ( 101.0536616762676374, -27.42723333900414318, 66.54514908543495721 ) ) ;
#18267=DIRECTION ( 'NONE',  ( 1.000000000000000000, 4.299999999999999979E-14, 1.000000000000000078E-15 ) ) ;
#18268=DIRECTION ( 'NONE',  ( -0.7071067812164788524, 0.7071067811566160710, 0.000000000000000000 ) ) ;
#18270=EDGE_CURVE ( 'NONE', #88009, #71659, #20549, .T. ) ;
#18271=VERTEX_POINT ( 'NONE', #81706 ) ;
#18274=CARTESIAN_POINT ( 'NONE',  ( 113.5922197990810645, -29.44396856740777224, 110.4956252759109816 ) ) ;
#18275=CARTESIAN_POINT ( 'NONE',  ( 31.56670390244700641, -19.82844715994111340, -5.074374724088000832 ) ) ;
#18277=CARTESIAN_POINT ( 'NONE',  ( 96.54020141486705597, -31.34005042439575561, 241.9499109901969689 ) ) ;
#18278=LINE ( 'NONE', #53215, #4825 ) ;
#18279=CARTESIAN_POINT ( 'NONE',  ( 41.56648329127399677, -9.303447159940999356, 81.04262527591200183 ) ) ;
#18280=FACE_OUTER_BOUND ( 'NONE', #19384, .T. ) ;
#18282=CARTESIAN_POINT ( 'NONE',  ( 107.0664832912739968, -36.72944715994100306, 287.6356252759109680 ) ) ;
#18284=VECTOR ( 'NONE', #74628, 1000.000000000000000 ) ;
#18285=CARTESIAN_POINT ( 'NONE',  ( 117.1170091337237551, -34.17489915221370467, 169.0365776568639831 ) ) ;
#18287=VERTEX_POINT ( 'NONE', #47589 ) ;
#18288=CARTESIAN_POINT ( 'NONE',  ( 97.38361328163530573, -33.95226689236985607, 137.5358690201829575 ) ) ;
#18289=AXIS2_PLACEMENT_3D ( 'NONE', #42188, #76730, #69470 ) ;
#18290=DIRECTION ( 'NONE',  ( 0.000000000000000000, 0.000000000000000000, 1.000000000000000000 ) ) ;
#18292=CARTESIAN_POINT ( 'NONE',  ( 115.1619974903459251, -42.21817061296636808, 269.3527681330531891 ) ) ;
#18293=DIRECTION ( 'NONE',  ( 0.9999999853157766072, 0.0001713722456133601202, -9.999999853157765648E-16 ) ) ;
#18297=ADVANCED_FACE ( 'NONE', ( #60783 ), #19458, .T. ) ;
#18299=CARTESIAN_POINT ( 'NONE',  ( 138.8167039024479834, -67.87844715994100397, 84.20080685541500998 ) ) ;
#18300=DIRECTION ( 'NONE',  ( 1.000000000000000078E-15, 1.000000000000000083E-30, -1.000000000000000000 ) ) ;
#18301=EDGE_CURVE ( 'NONE', #64730, #54616, #13280, .T. ) ;
#18302=DIRECTION ( 'NONE',  ( -1.000000000000000000, 0.000000000000000000, 0.000000000000000000 ) ) ;
#18303=CARTESIAN_POINT ( 'NONE',  ( 103.5497706991576905, -26.90106182813401503, 190.3499109901969746 ) ) ;
#18304=EDGE_CURVE ( 'NONE', #29424, #28847, #88517, .T. ) ;
#18306=ORIENTED_EDGE ( 'NONE', *, *, #17301, .F. ) ;
#18307=EDGE_CURVE ( 'NONE', #58766, #41861, #34988, .T. ) ;
#18312=CIRCLE ( 'NONE', #44370, 2.750000000000002665 ) ;
#18313=EDGE_CURVE ( 'NONE', #54780, #43708, #51003, .T. ) ;
#18314=ORIENTED_EDGE ( 'NONE', *, *, #3814, .T. ) ;
#18315=CARTESIAN_POINT ( 'NONE',  ( 117.0723199711336946, -35.46600488634853576, 63.92701177807728641 ) ) ;
#18316=AXIS2_PLACEMENT_3D ( 'NONE', #39940, #39504, #24544 ) ;
#18317=CARTESIAN_POINT ( 'NONE',  ( 108.1817894924016770, -47.09492459897622751, 202.6613395616249704 ) ) ;
#18320=ORIENTED_EDGE ( 'NONE', *, *, #39272, .F. ) ;
#18321=EDGE_CURVE ( 'NONE', #63793, #49742, #1687, .T. ) ;
#18322=CARTESIAN_POINT ( 'NONE',  ( 107.9598221976452521, -46.72791177985842381, 63.64822525680465048 ) ) ;
#18323=LINE ( 'NONE', #11972, #63759 ) ;
#18324=DIRECTION ( 'NONE',  ( 1.000000000000000078E-15, -1.000000000000000083E-30, -1.000000000000000000 ) ) ;
#18325=CARTESIAN_POINT ( 'NONE',  ( 98.55283614654496205, -38.28467619158744384, 49.30047132197196191 ) ) ;
#18326=LINE ( 'NONE', #45557, #60826 ) ;
#18327=ORIENTED_EDGE ( 'NONE', *, *, #24868, .F. ) ;
#18329=CARTESIAN_POINT ( 'NONE',  ( 81.62727349186526737, -16.46583755400498106, 7.833212107638633626 ) ) ;
#18330=ORIENTED_EDGE ( 'NONE', *, *, #18764, .F. ) ;
#18333=ORIENTED_EDGE ( 'NONE', *, *, #32140, .F. ) ;
#18335=FACE_OUTER_BOUND ( 'NONE', #75633, .T. ) ;
#18336=CARTESIAN_POINT ( 'NONE',  ( 99.05520249114191245, -33.76709814885239780, 65.46670554236195017 ) ) ;
#18337=CARTESIAN_POINT ( 'NONE',  ( 97.03688691280343903, -41.43079139552996537, 211.6632443235299945 ) ) ;
#18338=CARTESIAN_POINT ( 'NONE',  ( 97.97553865104310944, -30.48296430071270535, 165.8594347997199634 ) ) ;
#18339=CARTESIAN_POINT ( 'NONE',  ( 102.2973125513888988, -45.62237811309391589, 22.18432667138703707 ) ) ;
#18340=CARTESIAN_POINT ( 'NONE',  ( 96.91437895093065436, -34.20831442473366479, 272.1327681330538439 ) ) ;
#18343=ORIENTED_EDGE ( 'NONE', *, *, #89695, .F. ) ;
#18344=VERTEX_POINT ( 'NONE', #6722 ) ;
#18345=VECTOR ( 'NONE', #60200, 1000.000000000000000 ) ;
#18346=AXIS2_PLACEMENT_3D ( 'NONE', #45988, #42755, #7368 ) ;
#18347=CARTESIAN_POINT ( 'NONE',  ( 193.0374249753377001, -23.42844715993431848, 129.9678068554150343 ) ) ;
#18349=CARTESIAN_POINT ( 'NONE',  ( 117.4565820116822010, -35.18101482210430930, 218.9441967044829482 ) ) ;
#18350=ORIENTED_EDGE ( 'NONE', *, *, #38708, .F. ) ;
#18352=CARTESIAN_POINT ( 'NONE',  ( 114.9780134700875180, -29.01019993736734293, 194.4537205140059370 ) ) ;
#18353=CARTESIAN_POINT ( 'NONE',  ( 98.34958594534221277, -31.65707425133572173, 265.9065036673953273 ) ) ;
#18355=EDGE_CURVE ( 'NONE', #81510, #21246, #76211, .T. ) ;
#18356=CARTESIAN_POINT ( 'NONE',  ( 152.4532656103850456, -72.54314042502360849, 394.9756252759102040 ) ) ;
#18358=CARTESIAN_POINT ( 'NONE',  ( 112.0046464180979200, -30.41912573431281075, 277.6356252759109680 ) ) ;
#18360=CARTESIAN_POINT ( 'NONE',  ( 100.9974690995740190, -29.01719307973645812, 11.60705384733895507 ) ) ;
#18361=CARTESIAN_POINT ( 'NONE',  ( 75.31670390244798341, -57.40094715994099772, 58.80080685541479824 ) ) ;
#18363=DIRECTION ( 'NONE',  ( -1.000000000000000078E-15, 1.000000000000000083E-30, 1.000000000000000000 ) ) ;
#18364=DIRECTION ( 'NONE',  ( -1.000000000000000078E-15, 0.000000000000000000, 1.000000000000000000 ) ) ;
#18369=FACE_OUTER_BOUND ( 'NONE', #53928, .T. ) ;
#18370=CARTESIAN_POINT ( 'NONE',  ( 118.0743634110212383, -35.49574686983337557, 233.9032443235299752 ) ) ;
#18371=CARTESIAN_POINT ( 'NONE',  ( 108.0341493669268260, -25.71865232712709215, 105.9946728949589811 ) ) ;
#18372=CARTESIAN_POINT ( 'NONE',  ( 100.7237713325202861, -45.83809708005067307, 233.0803871806729717 ) ) ;
#18373=DIRECTION ( 'NONE',  ( -0.7071067811865671127, -0.7071067811865279218, -7.071067811865664660E-16 ) ) ;
#18374=LINE ( 'NONE', #72901, #67808 ) ;
#18376=CARTESIAN_POINT ( 'NONE',  ( 91.12500358871285755, -35.36225116344564157, 293.9356252759109793 ) ) ;
#18377=CARTESIAN_POINT ( 'NONE',  ( 98.14055758736320456, -41.24087220378398655, 37.69858362254909423 ) ) ;
#18382=ORIENTED_EDGE ( 'NONE', *, *, #65874, .F. ) ;
#18384=CARTESIAN_POINT ( 'NONE',  ( 112.8135049847298461, -43.08742197748514968, 132.5838483995059676 ) ) ;
#18386=VERTEX_POINT ( 'NONE', #22606 ) ;
#18387=DIRECTION ( 'NONE',  ( -0.4214249218767883165, -0.9068632946707806397, -4.214249218767892389E-16 ) ) ;
#18388=CARTESIAN_POINT ( 'NONE',  ( 117.0123300003820646, -30.33189756676014426, 140.2813395616249750 ) ) ;
#18390=LINE ( 'NONE', #58391, #35534 ) ;
#18392=DIRECTION ( 'NONE',  ( -0.7071067811865765496, 0.7071067811865185959, -7.071067811865461528E-16 ) ) ;
#18393=CARTESIAN_POINT ( 'NONE',  ( 110.5640613610538168, -45.86347053068967483, 62.86705384733992474 ) ) ;
#18394=ORIENTED_EDGE ( 'NONE', *, *, #57568, .T. ) ;
#18396=VECTOR ( 'NONE', #83088, 1000.000000000000000 ) ;
#18399=CARTESIAN_POINT ( 'NONE',  ( 116.0678243078410787, -40.55558035091540603, 164.5070538473389661 ) ) ;
#18400=LINE ( 'NONE', #65660, #11368 ) ;
#18407=CARTESIAN_POINT ( 'NONE',  ( 99.51750086509213133, -43.88776608678593760, 81.92991099019597812 ) ) ;
#18409=EDGE_CURVE ( 'NONE', #39122, #8508, #78915, .T. ) ;
#18410=ORIENTED_EDGE ( 'NONE', *, *, #47826, .F. ) ;
#18411=EDGE_CURVE ( 'NONE', #78071, #82260, #8525, .T. ) ;
#18412=CARTESIAN_POINT ( 'NONE',  ( 20.03715912545730760, -24.42818131006189830, 300.4678068554150059 ) ) ;
#18413=AXIS2_PLACEMENT_3D ( 'NONE', #62056, #20298, #47967 ) ;
#18415=CIRCLE ( 'NONE', #69192, 3.249999999999975131 ) ;
#18417=CARTESIAN_POINT ( 'NONE',  ( 99.76898186052154927, -41.38212431049157658, 139.5842808457819615 ) ) ;
#18418=AXIS2_PLACEMENT_3D ( 'NONE', #31434, #58259, #2862 ) ;
#18420=VECTOR ( 'NONE', #4909, 1000.000000000000114 ) ;
#18421=DIRECTION ( 'NONE',  ( 0.000000000000000000, 0.000000000000000000, -1.000000000000000000 ) ) ;
#18424=EDGE_CURVE ( 'NONE', #24618, #85625, #50739, .T. ) ;
#18428=EDGE_LOOP ( 'NONE', ( #36816, #31576 ) ) ;
#18429=ADVANCED_FACE ( 'NONE', ( #35762, #36679 ), #51174, .F. ) ;
#18431=CARTESIAN_POINT ( 'NONE',  ( 115.6736222539786638, -40.49689781175994341, 204.9177737820879486 ) ) ;
#18432=FACE_OUTER_BOUND ( 'NONE', #51674, .T. ) ;
#18433=VECTOR ( 'NONE', #40642, 1000.000000000000000 ) ;
#18434=VECTOR ( 'NONE', #46249, 1000.000000000000000 ) ;
#18435=CARTESIAN_POINT ( 'NONE',  ( 19.56648329127400032, 25.62155284005901379, 323.8756252759109202 ) ) ;
#18436=CARTESIAN_POINT ( 'NONE',  ( 97.81483072311490901, -40.51614641965803543, 17.63529977666319937 ) ) ;
#18437=ORIENTED_EDGE ( 'NONE', *, *, #55100, .F. ) ;
#18438=ORIENTED_EDGE ( 'NONE', *, *, #15953, .T. ) ;
#18441=ORIENTED_EDGE ( 'NONE', *, *, #28406, .F. ) ;
#18442=CARTESIAN_POINT ( 'NONE',  ( 99.31750181266291122, -39.29518527230509051, 239.3995189410199487 ) ) ;
#18443=CARTESIAN_POINT ( 'NONE',  ( 97.52207955639441650, -32.48083311392049666, 100.9927681330539713 ) ) ;
#18444=CARTESIAN_POINT ( 'NONE',  ( 110.3472192523918380, -25.36789009815977636, 64.85276813305395649 ) ) ;
#18445=DIRECTION ( 'NONE',  ( 0.000000000000000000, 0.000000000000000000, 1.000000000000000000 ) ) ;
#18446=CYLINDRICAL_SURFACE ( 'NONE', #28668, 4.749999999999976907 ) ;
#18447=CARTESIAN_POINT ( 'NONE',  ( 116.6607991934174322, -40.80763178269008762, 164.5070538473399608 ) ) ;
#18449=EDGE_LOOP ( 'NONE', ( #77330, #13655, #36587, #26913 ) ) ;
#18451=ORIENTED_EDGE ( 'NONE', *, *, #2764, .F. ) ;
#18453=LINE ( 'NONE', #72545, #33166 ) ;
#18454=CARTESIAN_POINT ( 'NONE',  ( 48.86082318535700608, -35.55794170701751256, -5.074374724088000832 ) ) ;
#18456=AXIS2_PLACEMENT_3D ( 'NONE', #79740, #24750, #60142 ) ;
#18457=DIRECTION ( 'NONE',  ( -1.000000000000000000, 0.000000000000000000, 0.000000000000000000 ) ) ;
#18458=VERTEX_POINT ( 'NONE', #14896 ) ;
#18459=CARTESIAN_POINT ( 'NONE',  ( 116.3201542697790529, -32.94256427661516540, 65.13562527591099638 ) ) ;
#18460=CARTESIAN_POINT ( 'NONE',  ( 109.7701363090614990, -47.44715903388583200, 92.78514908543495210 ) ) ;
#18464=CARTESIAN_POINT ( 'NONE',  ( 138.8167039024479834, -57.40094715994099772, 58.80080685541479824 ) ) ;
#18465=CARTESIAN_POINT ( 'NONE',  ( 99.96923091713365750, -43.45941328387855407, 81.92991099019697288 ) ) ;
#18466=FACE_OUTER_BOUND ( 'NONE', #19659, .T. ) ;
#18467=CARTESIAN_POINT ( 'NONE',  ( 100.0229104548316883, -27.23016881827670943, 181.5841967044829630 ) ) ;
#18468=CARTESIAN_POINT ( 'NONE',  ( 108.4138796129811055, -26.73457821205273532, 59.96924600114584081 ) ) ;
#18470=ORIENTED_EDGE ( 'NONE', *, *, #65431, .T. ) ;
#18471=LINE ( 'NONE', #39370, #84635 ) ;
#18473=CARTESIAN_POINT ( 'NONE',  ( 31.56670390244800828, -33.35206098992711077, -5.074374724088000832 ) ) ;
#18475=CARTESIAN_POINT ( 'NONE',  ( 97.43243490695729747, -40.91715606259069204, 231.6527681330539679 ) ) ;
#18476=VERTEX_POINT ( 'NONE', #84836 ) ;
#18477=CARTESIAN_POINT ( 'NONE',  ( 172.5664832912740110, -32.07844715994070839, 254.1756252759120400 ) ) ;
#18478=CARTESIAN_POINT ( 'NONE',  ( 99.36548562555644537, -29.67027625815665104, 271.7356252759109907 ) ) ;
#18479=CARTESIAN_POINT ( 'NONE',  ( 108.5961642634028692, -47.12166094979025388, 138.6927681330539883 ) ) ;
#18480=VECTOR ( 'NONE', #45916, 1000.000000000000000 ) ;
#18482=CARTESIAN_POINT ( 'NONE',  ( 82.67951041503442866, -37.60592655292794007, 6.943955837742791459 ) ) ;
#18483=CARTESIAN_POINT ( 'NONE',  ( 76.06670390244799762, -26.72944715994109899, 199.5838068554169524 ) ) ;
#18484=DIRECTION ( 'NONE',  ( 0.000000000000000000, 0.000000000000000000, 1.000000000000000000 ) ) ;
#18486=AXIS2_PLACEMENT_3D ( 'NONE', #52205, #30902, #79519 ) ;
#18487=VECTOR ( 'NONE', #89845, 1000.000000000000000 ) ;
#18488=ADVANCED_FACE ( 'NONE', ( #50278, #49831 ), #56649, .F. ) ;
#18489=VECTOR ( 'NONE', #21124, 1000.000000000000000 ) ;
#18492=VERTEX_POINT ( 'NONE', #9411 ) ;
#18494=CARTESIAN_POINT ( 'NONE',  ( 112.9508454419805332, -28.15023113465295879, 40.59848241876795782 ) ) ;
#18497=ADVANCED_FACE ( 'NONE', ( #63933 ), #56189, .F. ) ;
#18499=EDGE_CURVE ( 'NONE', #79518, #4931, #64824, .T. ) ;
#18500=AXIS2_PLACEMENT_3D ( 'NONE', #15077, #71396, #49570 ) ;
#18501=CYLINDRICAL_SURFACE ( 'NONE', #19226, 37.00000000000000711 ) ;
#18504=CARTESIAN_POINT ( 'NONE',  ( 113.2432932581317289, -30.83002766685618923, 233.8552769709339429 ) ) ;
#18505=VERTEX_POINT ( 'NONE', #63023 ) ;
#18506=EDGE_LOOP ( 'NONE', ( #73529, #3805, #56889, #17980, #67408, #60986, #88347, #23072, #84249, #62651, #61028, #55724, #38617, #55939, #59556, #51472, #10404, #34878, #64833, #43406, #46098, #7046, #89817, #72942, #21283, #75753, #77220, #67640, #51155, #37548, #66227, #88587, #69410, #87281 ) ) ;
#18507=VERTEX_POINT ( 'NONE', #83942 ) ;
#18508=CARTESIAN_POINT ( 'NONE',  ( 80.06648329127399677, -18.72944715994105991, -5.074374724089057764 ) ) ;
#18511=DIRECTION ( 'NONE',  ( 0.000000000000000000, 0.000000000000000000, 1.000000000000000000 ) ) ;
#18512=CARTESIAN_POINT ( 'NONE',  ( 98.92341559625380398, -33.23365848574461268, 12.43586902018295426 ) ) ;
#18515=B_SPLINE_CURVE_WITH_KNOTS ( 'NONE', 3,
 ( #65146, #58330, #22488, #71093, #2039, #45128, #71977, #86057, #2930, #29302, #31064, #51936, #57885, #15676, #8867, #23827, #36564, #30188, #50162, #77897, #30632, #51496, #79246, #64266, #10185, #58760, #17007, #23397, #78360, #79694, #50618, #16557, #85619, #56984, #2489, #44692, #51064, #84727, #29748, #57433, #85171, #86498, #72420, #44240, #37894, #22944, #43349, #3374, #9744, #16122, #24266, #43800, #71536, #9299, #37002, #65593, #64709, #17447, #8411, #78801, #37448, #36105, #63819, #1597, #24706 ),
 .UNSPECIFIED., .F., .F.,
 ( 4, 1, 1, 1, 1, 1, 2, 2, 1, 1, 1, 1, 2, 2, 1, 1, 1, 1, 1, 1, 2, 2, 1, 1, 1, 1, 1, 2, 2, 1, 1, 1, 1, 1, 2, 2, 1, 2, 2, 1, 2, 2, 2, 2, 2, 4 ),
 ( 0.000000000000000000, 0.03124999999989700600, 0.04687499999984345161, 0.05468749999981731974, 0.05859374999980424686, 0.06054687499979771736, 0.06152343749979605203, 0.06249999999979438670, 0.09374999999972724596, 0.1093749999996942862, 0.1171874999996784794, 0.1210937499996705830, 0.1230468749996672245, 0.1249999999996638522, 0.1562499999996239120, 0.1718749999996045941, 0.1796874999995961286, 0.1835937499995913824, 0.1855468749995903555, 0.1865234374995903555, 0.1870117187495903555, 0.1874999999995903555, 0.2187499999995501099, 0.2343749999995297095, 0.2421874999995189126, 0.2460937499995125566, 0.2480468749995090594, 0.2490234374995082822, 0.2499999999995075051, 0.3124999999995169420, 0.3437499999995223265, 0.3593749999995249911, 0.3671874999995263233, 0.3710937499995269895, 0.3730468749995266009, 0.3749999999995262123, 0.4374999999995722311, 0.4687499999995950462, 0.4999999999996179723, 0.5624999999996637134, 0.5937499999996874722, 0.6249999999997112310, 0.6874999999997587485, 0.7499999999998061551, 0.8749999999999031886, 1.000000000000000000 ),
 .UNSPECIFIED. ) ;
#18516=CARTESIAN_POINT ( 'NONE',  ( 112.8396959964676682, -44.62460075896473910, 228.0784824187689708 ) ) ;
#18517=EDGE_CURVE ( 'NONE', #19610, #34249, #32132, .T. ) ;
#18519=EDGE_LOOP ( 'NONE', ( #66584, #87890 ) ) ;
#18520=CARTESIAN_POINT ( 'NONE',  ( 194.0371591254575776, -24.89890238294407254, 129.9678068554150343 ) ) ;
#18522=CARTESIAN_POINT ( 'NONE',  ( 106.9575452361726491, -28.53976946500068124, 57.90523322673496409 ) ) ;
#18523=AXIS2_PLACEMENT_3D ( 'NONE', #28619, #85409, #9086 ) ;
#18524=CARTESIAN_POINT ( 'NONE',  ( 97.81170999939396893, -40.51745679428447744, 191.6351607553995393 ) ) ;
#18525=LINE ( 'NONE', #59848, #47596 ) ;
#18526=DIRECTION ( 'NONE',  ( 1.000000000000000000, 4.163336342344333240E-14, 0.000000000000000000 ) ) ;
#18529=EDGE_CURVE ( 'NONE', #611, #32172, #43742, .T. ) ;
#18532=CARTESIAN_POINT ( 'NONE',  ( 106.0764471815382279, -48.53877882342441552, 112.5099109901969712 ) ) ;
#18533=ORIENTED_EDGE ( 'NONE', *, *, #79747, .T. ) ;
#18534=EDGE_CURVE ( 'NONE', #35180, #87084, #23942, .T. ) ;
#18535=CARTESIAN_POINT ( 'NONE',  ( 99.05520249114191245, -33.76709814885239780, 65.46670554236195017 ) ) ;
#18537=DIRECTION ( 'NONE',  ( -4.299999999999999979E-14, 1.000000000000000000, -4.100000000000000342E-29 ) ) ;
#18538=CARTESIAN_POINT ( 'NONE',  ( 108.3172770934737628, -27.95654607328577868, 101.3958690201829711 ) ) ;
#18540=ADVANCED_FACE ( 'NONE', ( #65269, #31178, #52925, #73412 ), #11184, .T. ) ;
#18543=CARTESIAN_POINT ( 'NONE',  ( 96.32186211137589282, -39.41937243639647903, 12.53372051400597442 ) ) ;
#18546=DIRECTION ( 'NONE',  ( 1.000000000000000000, 4.163336342344333240E-14, 0.000000000000000000 ) ) ;
#18547=CIRCLE ( 'NONE', #80953, 1.000000000000000888 ) ;
#18550=CARTESIAN_POINT ( 'NONE',  ( 90.44969454456403923, -17.59493780205715652, 239.5838068554169809 ) ) ;
#18553=CIRCLE ( 'NONE', #69346, 5.035202529042104302 ) ;
#18554=DIRECTION ( 'NONE',  ( 0.000000000000000000, 0.000000000000000000, 1.000000000000000000 ) ) ;
#18556=CARTESIAN_POINT ( 'NONE',  ( 104.9788083641148688, -27.14010996210884485, 260.2470538473402826 ) ) ;
#18557=CARTESIAN_POINT ( 'NONE',  ( 105.4983833033492715, -26.83149777197436592, 125.2004868081602353 ) ) ;
#18558=CARTESIAN_POINT ( 'NONE',  ( 109.6430120601289957, -46.48008675456071614, 188.7814586034739364 ) ) ;
#18559=CARTESIAN_POINT ( 'NONE',  ( 112.9631696212496905, -28.13226286662721165, 40.59848241876795782 ) ) ;
#18560=CARTESIAN_POINT ( 'NONE',  ( 104.4076862809217516, -46.45797926106136799, 43.36475834774724802 ) ) ;
#18561=ORIENTED_EDGE ( 'NONE', *, *, #57502, .F. ) ;
#18562=VECTOR ( 'NONE', #85864, 1000.000000000000000 ) ;
#18564=AXIS2_PLACEMENT_3D ( 'NONE', #39527, #32712, #77644 ) ;
#18565=AXIS2_PLACEMENT_3D ( 'NONE', #4624, #25061, #46824 ) ;
#18566=CARTESIAN_POINT ( 'NONE',  ( 177.0371591254543659, -48.62818131005480637, 249.9678068554149775 ) ) ;
#18567=ORIENTED_EDGE ( 'NONE', *, *, #81184, .T. ) ;
#18568=AXIS2_PLACEMENT_3D ( 'NONE', #70712, #36185, #8944 ) ;
#18571=CARTESIAN_POINT ( 'NONE',  ( 100.1919508713739049, -45.35525880799018239, 272.0289586092443415 ) ) ;
#18573=EDGE_CURVE ( 'NONE', #4156, #8582, #87059, .T. ) ;
#18574=DIRECTION ( 'NONE',  ( 3.999999999999999995E-14, -1.000000000000000000, 4.100000000000000342E-29 ) ) ;
#18575=CARTESIAN_POINT ( 'NONE',  ( 79.05226586199937344, -39.28573230649617187, 1.785258109343057731 ) ) ;
#18576=CARTESIAN_POINT ( 'NONE',  ( 100.8994401894200053, -30.77800351108903598, 250.1381341137912671 ) ) ;
#18577=DIRECTION ( 'NONE',  ( 0.000000000000000000, 0.000000000000000000, -1.000000000000000000 ) ) ;
#18578=CARTESIAN_POINT ( 'NONE',  ( 102.5676158828201778, -27.34920955258912301, 91.43276813305395478 ) ) ;
#18580=CARTESIAN_POINT ( 'NONE',  ( 97.70685376065341643, -42.69687791250295561, 141.7661014663869707 ) ) ;
#18581=ORIENTED_EDGE ( 'NONE', *, *, #6616, .F. ) ;
#18582=FACE_OUTER_BOUND ( 'NONE', #17989, .T. ) ;
#18583=EDGE_LOOP ( 'NONE', ( #68301, #16449, #47907 ) ) ;
#18584=CIRCLE ( 'NONE', #50542, 0.4999999999999982236 ) ;
#18585=CARTESIAN_POINT ( 'NONE',  ( 177.4809174648215730, -49.32844715993478246, 180.4678068554150059 ) ) ;
#18586=CARTESIAN_POINT ( 'NONE',  ( 127.0664832912740394, -46.72944715994101017, -5.074374724089008915 ) ) ;
#18587=CARTESIAN_POINT ( 'NONE',  ( 177.8371591254543205, -47.82818131005477369, 300.4678068554149490 ) ) ;
#18588=ORIENTED_EDGE ( 'NONE', *, *, #58998, .F. ) ;
#18589=CARTESIAN_POINT ( 'NONE',  ( 97.70663789874652139, -40.25152162066777350, 51.61287317870858260 ) ) ;
#18590=CARTESIAN_POINT ( 'NONE',  ( 107.6554820827327461, -47.17179587048914158, 152.6213395616249500 ) ) ;
#18591=ORIENTED_EDGE ( 'NONE', *, *, #51497, .F. ) ;
#18595=CYLINDRICAL_SURFACE ( 'NONE', #48866, 2.517499999999998739 ) ;
#18597=LINE ( 'NONE', #67189, #75719 ) ;
#18598=ORIENTED_EDGE ( 'NONE', *, *, #23271, .F. ) ;
#18599=CARTESIAN_POINT ( 'NONE',  ( 117.2310933634200012, -39.29246586887208537, 123.6299109901969615 ) ) ;
#18602=DIRECTION ( 'NONE',  ( 0.000000000000000000, 0.000000000000000000, 1.000000000000000000 ) ) ;
#18603=EDGE_CURVE ( 'NONE', #43538, #2385, #9862, .T. ) ;
#18604=CARTESIAN_POINT ( 'NONE',  ( 86.06670390244796920, -50.82844715994100682, 295.9178068554149945 ) ) ;
#18606=EDGE_CURVE ( 'NONE', #26947, #63793, #72738, .T. ) ;
#18608=FACE_OUTER_BOUND ( 'NONE', #20848, .T. ) ;
#18610=DIRECTION ( 'NONE',  ( 0.000000000000000000, 0.000000000000000000, -1.000000000000000000 ) ) ;
#18611=CARTESIAN_POINT ( 'NONE',  ( 184.5664832912729878, -81.37844715994266664, 342.9256252759109884 ) ) ;
#18612=ADVANCED_FACE ( 'NONE', ( #80253 ), #30747, .F. ) ;
#18614=CARTESIAN_POINT ( 'NONE',  ( 105.7992971826924986, -26.72406505859367698, 105.1773095432808987 ) ) ;
#18617=EDGE_CURVE ( 'NONE', #6412, #70634, #6031, .T. ) ;
#18619=ORIENTED_EDGE ( 'NONE', *, *, #9386, .F. ) ;
#18620=AXIS2_PLACEMENT_3D ( 'NONE', #19835, #88441, #61163 ) ;
#18621=CARTESIAN_POINT ( 'NONE',  ( 100.8874680621459987, -44.70022151100008756, 33.05229196020944471 ) ) ;
#18623=CARTESIAN_POINT ( 'NONE',  ( 97.31640351007386869, -35.61153895465465524, 202.2356252759109623 ) ) ;
#18624=FACE_BOUND ( 'NONE', #80207, .T. ) ;
#18625=EDGE_LOOP ( 'NONE', ( #22835, #86146 ) ) ;
#18627=CARTESIAN_POINT ( 'NONE',  ( 110.1676348244934331, -46.62498374987613659, 48.80610146638597513 ) ) ;
#18630=ADVANCED_FACE ( 'NONE', ( #44810 ), #86613, .F. ) ;
#18631=VECTOR ( 'NONE', #10691, 1000.000000000000000 ) ;
#18632=CARTESIAN_POINT ( 'NONE',  ( 107.0664832912739968, -0.2185775633790978945, 335.9181252759120184 ) ) ;
#18633=ORIENTED_EDGE ( 'NONE', *, *, #60357, .F. ) ;
#18635=CIRCLE ( 'NONE', #44691, 5.599999999999994316 ) ;
#18636=ORIENTED_EDGE ( 'NONE', *, *, #59029, .F. ) ;
#18637=ORIENTED_EDGE ( 'NONE', *, *, #89661, .F. ) ;
#18638=CARTESIAN_POINT ( 'NONE',  ( 97.06047953529140671, -37.89159766150721964, 232.8501547344689584 ) ) ;
#18639=CARTESIAN_POINT ( 'NONE',  ( 177.4809174648213173, -48.32844715993478957, 300.4678068554149490 ) ) ;
#18641=CARTESIAN_POINT ( 'NONE',  ( 101.9936208421809454, -45.44607148214490877, 153.1564586002609190 ) ) ;
#18642=VECTOR ( 'NONE', #84405, 1000.000000000000000 ) ;
#18643=CARTESIAN_POINT ( 'NONE',  ( 63.03715912545637678, -24.42818131006026761, 193.9678068554150911 ) ) ;
#18648=CARTESIAN_POINT ( 'NONE',  ( 97.07516343140007109, -33.75277822987297327, 31.09562527591097592 ) ) ;
#18649=ORIENTED_EDGE ( 'NONE', *, *, #85976, .F. ) ;
#18650=ORIENTED_EDGE ( 'NONE', *, *, #89495, .F. ) ;
#18651=CARTESIAN_POINT ( 'NONE',  ( 103.9533468823514823, -45.47040322110986210, 250.1223760838773273 ) ) ;
#18653=DIRECTION ( 'NONE',  ( 0.000000000000000000, 0.000000000000000000, -1.000000000000000000 ) ) ;
#18654=CARTESIAN_POINT ( 'NONE',  ( 71.25443513191777356, -74.12815658812309039, 540.9756252759101471 ) ) ;
#18656=DIRECTION ( 'NONE',  ( -4.237773401492740281E-14, 1.000000000000000000, 0.000000000000000000 ) ) ;
#18659=CARTESIAN_POINT ( 'NONE',  ( 117.8211145215647946, -31.63542911875440211, 210.1784824187679703 ) ) ;
#18662=CARTESIAN_POINT ( 'NONE',  ( 110.3678327243794541, -25.29650332976257943, 60.85276813305395649 ) ) ;
#18663=DIRECTION ( 'NONE',  ( -4.237773401492740281E-14, 1.000000000000000000, 0.000000000000000000 ) ) ;
#18665=ORIENTED_EDGE ( 'NONE', *, *, #80365, .F. ) ;
#18667=CARTESIAN_POINT ( 'NONE',  ( 36.74138383868084645, -48.33240602328870494, 129.9678068554150911 ) ) ;
#18668=DIRECTION ( 'NONE',  ( 0.1858654558203329255, -0.9825752044157738396, 0.000000000000000000 ) ) ;
#18670=CARTESIAN_POINT ( 'NONE',  ( 115.0182259351703777, -41.51125854152899564, 126.2138046553059638 ) ) ;
#18671=CARTESIAN_POINT ( 'NONE',  ( 103.9327720845255669, -26.76365000536165439, 246.3184824187679567 ) ) ;
#18672=FACE_OUTER_BOUND ( 'NONE', #73604, .T. ) ;
#18676=VERTEX_POINT ( 'NONE', #38437 ) ;
#18677=ORIENTED_EDGE ( 'NONE', *, *, #11566, .T. ) ;
#18679=VECTOR ( 'NONE', #21916, 1000.000000000000000 ) ;
#18682=ORIENTED_EDGE ( 'NONE', *, *, #1668, .F. ) ;
#18683=DIRECTION ( 'NONE',  ( 1.000000000000000078E-15, 1.000000000000000083E-30, -1.000000000000000000 ) ) ;
#18685=DIRECTION ( 'NONE',  ( -0.7071067812160284349, 0.7071067811570665995, -7.071067812160292375E-16 ) ) ;
#18686=CARTESIAN_POINT ( 'NONE',  ( 109.3519496323076083, -28.49945473430254950, 174.2838483995049899 ) ) ;
#18687=CARTESIAN_POINT ( 'NONE',  ( 112.2029234908279562, -27.56599932623266724, 34.66991099019695355 ) ) ;
#18688=CARTESIAN_POINT ( 'NONE',  ( 107.0664832912739968, -18.82844715994099971, 335.9181252759120184 ) ) ;
#18689=ORIENTED_EDGE ( 'NONE', *, *, #85215, .F. ) ;
#18696=CARTESIAN_POINT ( 'NONE',  ( 97.80987186915811549, -40.51298665854582737, 167.6355175185183839 ) ) ;
#18697=AXIS2_PLACEMENT_3D ( 'NONE', #31662, #73442, #38920 ) ;
#18699=CARTESIAN_POINT ( 'NONE',  ( 111.0490742293896318, -45.90261773848913407, 132.9024169551198895 ) ) ;
#18701=VERTEX_POINT ( 'NONE', #73863 ) ;
#18702=CARTESIAN_POINT ( 'NONE',  ( 116.1776873554136813, -43.03363693755514419, 13.35657765686298859 ) ) ;
#18703=CARTESIAN_POINT ( 'NONE',  ( 113.4862441490110427, -46.74931658189198913, 64.02991099019695298 ) ) ;
#18705=LINE ( 'NONE', #47739, #63681 ) ;
#18706=DIRECTION ( 'NONE',  ( 0.000000000000000000, 0.000000000000000000, -1.000000000000000000 ) ) ;
#18707=DIRECTION ( 'NONE',  ( 0.7071067811874264253, -0.7071067811856686092, 7.071067811874271132E-16 ) ) ;
#18709=CARTESIAN_POINT ( 'NONE',  ( 106.3488784333137289, -25.28999724522163461, 322.7624077768622328 ) ) ;
#18710=CARTESIAN_POINT ( 'NONE',  ( 41.56670390244695312, -36.32844715994109208, 129.9678068554150911 ) ) ;
#18711=VECTOR ( 'NONE', #7747, 1000.000000000000000 ) ;
#18712=ADVANCED_FACE ( 'NONE', ( #61566 ), #27504, .F. ) ;
#18715=ADVANCED_FACE ( 'NONE', ( #5277 ), #20702, .F. ) ;
#18716=ORIENTED_EDGE ( 'NONE', *, *, #53539, .T. ) ;
#18717=CARTESIAN_POINT ( 'NONE',  ( 105.9838489277333480, -26.31625509990853828, 50.15848241876796720 ) ) ;
#18718=CARTESIAN_POINT ( 'NONE',  ( 113.0254242409527308, -46.03885118181761982, 214.0175300378159591 ) ) ;
#18719=CARTESIAN_POINT ( 'NONE',  ( 117.4691034930615103, -37.69004686371126667, 74.75276813305397638 ) ) ;
#18720=CARTESIAN_POINT ( 'NONE',  ( 97.81944477327695608, -40.53632314921513569, 171.6375141567590674 ) ) ;
#18721=CARTESIAN_POINT ( 'NONE',  ( 135.3756687995053483, -12.91806617559082504, 361.9756252759100335 ) ) ;
#18722=CARTESIAN_POINT ( 'NONE',  ( 194.0371591254583166, -46.82818131005407736, 236.4678068554149775 ) ) ;
#18723=VECTOR ( 'NONE', #77982, 999.9999999999998863 ) ;
#18724=EDGE_CURVE ( 'NONE', #46977, #15780, #23066, .T. ) ;
#18727=EDGE_CURVE ( 'NONE', #79957, #32858, #69300, .T. ) ;
#18728=CARTESIAN_POINT ( 'NONE',  ( 114.2951562036312936, -44.16484043540973659, 114.2022919425769771 ) ) ;
#18730=EDGE_LOOP ( 'NONE', ( #10747, #11305, #25473, #63166 ) ) ;
#18731=CARTESIAN_POINT ( 'NONE',  ( 118.0279888096067396, -35.50094427011356402, 229.9032443235299468 ) ) ;
#18732=CARTESIAN_POINT ( 'NONE',  ( 117.0719613561143433, -35.46296010572103086, 254.9279646184726573 ) ) ;
#18733=DIRECTION ( 'NONE',  ( 2.900000000000000265E-14, -2.000000000000000155E-15, 1.000000000000000000 ) ) ;
#18735=DIRECTION ( 'NONE',  ( -4.299999999999999979E-14, 1.000000000000000000, -4.400000000000000367E-29 ) ) ;
#18737=CARTESIAN_POINT ( 'NONE',  ( 131.3325395364355472, -37.07457063614607762, 3.076560393663394510 ) ) ;
#18739=CARTESIAN_POINT ( 'NONE',  ( 97.29384000864233428, -37.12803473146956890, 161.3584824187679487 ) ) ;
#18741=VERTEX_POINT ( 'NONE', #19803 ) ;
#18742=VECTOR ( 'NONE', #27675, 999.9999999999998863 ) ;
#18743=CARTESIAN_POINT ( 'NONE',  ( 115.8195149170444296, -38.11245691049232676, 110.1330118773259699 ) ) ;
#18744=AXIS2_PLACEMENT_3D ( 'NONE', #33628, #6366, #68154 ) ;
#18745=CARTESIAN_POINT ( 'NONE',  ( 20.03715912545730760, -24.42818131006189830, 300.4678068554150059 ) ) ;
#18746=CARTESIAN_POINT ( 'NONE',  ( 114.8131502045275880, -44.70447909941016462, 264.1899109901960401 ) ) ;
#18751=CONICAL_SURFACE ( 'NONE', #78244, 1.258750000000002922, 1.029744258676650093 ) ;
#18753=DIRECTION ( 'NONE',  ( 0.000000000000000000, 0.000000000000000000, 1.000000000000000000 ) ) ;
#18754=CARTESIAN_POINT ( 'NONE',  ( 107.0664832912739968, -36.72944715994100306, 287.6356252759109680 ) ) ;
#18755=CARTESIAN_POINT ( 'NONE',  ( 97.44537786355540732, -42.12371753947140007, 181.7451490854349743 ) ) ;
#18757=ORIENTED_EDGE ( 'NONE', *, *, #36290, .F. ) ;
#18758=VERTEX_POINT ( 'NONE', #82499 ) ;
#18760=DIRECTION ( 'NONE',  ( 0.000000000000000000, 0.000000000000000000, 1.000000000000000000 ) ) ;
#18763=CARTESIAN_POINT ( 'NONE',  ( 20.56670390244828184, -48.82844715994187368, 300.4678068554150059 ) ) ;
#18764=EDGE_CURVE ( 'NONE', #30005, #85483, #35049, .T. ) ;
#18765=B_SPLINE_CURVE_WITH_KNOTS ( 'NONE', 3,
 ( #16422, #58192, #10050, #44097, #71832, #65455, #3239, #9598, #30934, #58621, #51799, #79550, #53575, #54918, #6353, #67230, #34042, #33165 ),
 .UNSPECIFIED., .F., .F.,
 ( 4, 2, 2, 2, 2, 2, 2, 2, 4 ),
 ( 0.000000000000000000, 0.06249999997213293024, 0.1249999999442658605, 0.1874999999163987907, 0.2499999998885317209, 0.3124999998606646789, 0.3749999998327975814, 0.4374999998049304839, 0.4999999997770634419 ),
 .UNSPECIFIED. ) ;
#18767=ORIENTED_EDGE ( 'NONE', *, *, #12263, .F. ) ;
#18769=CARTESIAN_POINT ( 'NONE',  ( 117.9328099866778246, -34.70409988052399086, 203.9851490854349549 ) ) ;
#18770=CYLINDRICAL_SURFACE ( 'NONE', #53274, 9.999999999999998224 ) ;
#18773=AXIS2_PLACEMENT_3D ( 'NONE', #5860, #41239, #48053 ) ;
#18774=CARTESIAN_POINT ( 'NONE',  ( 51.56670390244899238, -32.29483332968450782, 313.9678068554150059 ) ) ;
#18775=DIRECTION ( 'NONE',  ( -1.000000000000000000, -4.299999999999999979E-14, -9.351236661543306751E-17 ) ) ;
#18776=CARTESIAN_POINT ( 'NONE',  ( 104.4075988886342401, -46.45794203021185353, 163.3647505914425153 ) ) ;
#18777=CARTESIAN_POINT ( 'NONE',  ( 113.6264423535256043, -41.63348889605062908, 26.13380465530496011 ) ) ;
#18778=CARTESIAN_POINT ( 'NONE',  ( 97.55141575199942849, -31.05946519635597269, 126.9108633711489915 ) ) ;
#18781=EDGE_CURVE ( 'NONE', #42224, #69089, #46648, .T. ) ;
#18783=AXIS2_PLACEMENT_3D ( 'NONE', #47335, #4233, #75064 ) ;
#18784=CARTESIAN_POINT ( 'NONE',  ( 81.78920663581700978, -16.57943358557456293, 7.744922197166920874 ) ) ;
#18785=ORIENTED_EDGE ( 'NONE', *, *, #4992, .T. ) ;
#18787=EDGE_CURVE ( 'NONE', #18458, #41728, #2054, .T. ) ;
#18791=CARTESIAN_POINT ( 'NONE',  ( 98.34940958104215269, -31.65739082969130180, 156.9063178242618051 ) ) ;
#18792=CARTESIAN_POINT ( 'NONE',  ( 115.2801527212906336, -32.91522314707135166, 58.58289601855292972 ) ) ;
#18793=CARTESIAN_POINT ( 'NONE',  ( 97.74263787230347589, -41.52050856888216401, 196.7041967044819728 ) ) ;
#18794=CIRCLE ( 'NONE', #57961, 2.750000000000002665 ) ;
#18795=CARTESIAN_POINT ( 'NONE',  ( 109.4403364888817123, -25.95778788316468422, 179.8918157521019339 ) ) ;
#18796=CARTESIAN_POINT ( 'NONE',  ( 97.81477617152367543, -40.51601309134415629, 21.63528831556280707 ) ) ;
#18797=CARTESIAN_POINT ( 'NONE',  ( 112.1067112481348431, -26.91823048478340397, 15.71086337114896381 ) ) ;
#18798=FACE_OUTER_BOUND ( 'NONE', #81740, .T. ) ;
#18799=PLANE ( 'NONE',  #85999 ) ;
#18800=ORIENTED_EDGE ( 'NONE', *, *, #33116, .F. ) ;
#18803=CIRCLE ( 'NONE', #88465, 3.250000000000002665 ) ;
#18805=CARTESIAN_POINT ( 'NONE',  ( 62.03715912545840183, -47.82818131006021645, 237.4678068554150059 ) ) ;
#18806=CARTESIAN_POINT ( 'NONE',  ( 100.7233752965418034, -45.83866581990632483, 237.0803871806729717 ) ) ;
#18807=VERTEX_POINT ( 'NONE', #22957 ) ;
#18808=CARTESIAN_POINT ( 'NONE',  ( 117.2917222856570447, -34.52255020207628888, 183.9956252759109532 ) ) ;
#18809=DIRECTION ( 'NONE',  ( -1.000000000000000000, 0.000000000000000000, 0.000000000000000000 ) ) ;
#18810=DIRECTION ( 'NONE',  ( 1.000000000000000078E-15, 1.000000000000000083E-30, -1.000000000000000000 ) ) ;
#18811=CARTESIAN_POINT ( 'NONE',  ( 188.5667039024479834, -62.87844715994099687, 137.2178068554150059 ) ) ;
#18812=EDGE_CURVE ( 'NONE', #71344, #61557, #36118, .T. ) ;
#18813=CARTESIAN_POINT ( 'NONE',  ( 114.4830409211623419, -33.53596877257181319, 277.6356252759111385 ) ) ;
#18814=DIRECTION ( 'NONE',  ( 1.000000000000000078E-15, 1.000000000000000083E-30, -1.000000000000000000 ) ) ;
#18815=CARTESIAN_POINT ( 'NONE',  ( 162.7131505118679797, -31.94127993907790852, 342.9256252759119548 ) ) ;
#18820=EDGE_CURVE ( 'NONE', #60117, #29891, #64282, .T. ) ;
#18821=CARTESIAN_POINT ( 'NONE',  ( 161.4809174648183330, -48.32844715993547879, 300.4678068554149490 ) ) ;
#18822=CARTESIAN_POINT ( 'NONE',  ( 164.9667039024459996, -26.71338133339301635, -5.074374724088000832 ) ) ;
#18823=CARTESIAN_POINT ( 'NONE',  ( 83.06670390244808289, -58.72944715994108122, 207.5838068554169809 ) ) ;
#18824=CARTESIAN_POINT ( 'NONE',  ( 100.3694914525244712, -30.29371855352183118, 195.5838068554172651 ) ) ;
#18826=EDGE_CURVE ( 'NONE', #77606, #5064, #62916, .T. ) ;
#18828=CARTESIAN_POINT ( 'NONE',  ( 113.2331319966886412, -45.16264392691098806, 228.0784824187679760 ) ) ;
#18829=CARTESIAN_POINT ( 'NONE',  ( 108.9848500582430404, -47.61493517985451973, 118.7032443235299723 ) ) ;
#18830=CARTESIAN_POINT ( 'NONE',  ( 101.3810039469494200, -45.56196318943892010, 218.1213395616249784 ) ) ;
#18832=AXIS2_PLACEMENT_3D ( 'NONE', #57659, #70411, #84949 ) ;
#18833=LINE ( 'NONE', #11582, #88124 ) ;
#18834=CYLINDRICAL_SURFACE ( 'NONE', #71089, 0.5000000000000197620 ) ;
#18835=DIRECTION ( 'NONE',  ( -0.4999999926578924114, -8.568612279970206714E-05, -0.8660254037844363761 ) ) ;
#18837=CARTESIAN_POINT ( 'NONE',  ( 86.06670390244796920, -58.72944715994112386, 198.9178068554149945 ) ) ;
#18838=ADVANCED_FACE ( 'NONE', ( #77912 ), #68463, .T. ) ;
#18839=VERTEX_POINT ( 'NONE', #42020 ) ;
#18840=ORIENTED_EDGE ( 'NONE', *, *, #33959, .F. ) ;
#18841=BREP_WITH_VOIDS ( 'NONE', #86604, ( #7833, #81688, #8987, #10099, #67821, #23948, #66688, #35626, #89470, #65572, #72248, #25060, #50594 ) );
#18844=CARTESIAN_POINT ( 'NONE',  ( 100.3400348588553328, -31.46521817125301368, 155.2209912566479488 ) ) ;
#18846=ORIENTED_EDGE ( 'NONE', *, *, #11468, .F. ) ;
#18847=CARTESIAN_POINT ( 'NONE',  ( 102.0669781233241196, -27.97054301683326116, 90.48814389190501117 ) ) ;
#18848=CARTESIAN_POINT ( 'NONE',  ( 118.8789388927531974, -36.16900092901214947, 114.8641967044819694 ) ) ;
#18849=CARTESIAN_POINT ( 'NONE',  ( 71.25614885437424562, -84.12815644128087911, 396.9756252759102040 ) ) ;
#18850=FACE_OUTER_BOUND ( 'NONE', #36342, .T. ) ;
#18852=CARTESIAN_POINT ( 'NONE',  ( 113.1782937742881927, -44.75186859022056751, 109.0939586095510805 ) ) ;
#18853=CARTESIAN_POINT ( 'NONE',  ( 102.2761128416349123, -28.20209198692209185, 60.48419670448296159 ) ) ;
#18854=EDGE_LOOP ( 'NONE', ( #41657, #65091, #60815, #18164 ) ) ;
#18856=ORIENTED_EDGE ( 'NONE', *, *, #70728, .T. ) ;
#18857=ORIENTED_EDGE ( 'NONE', *, *, #17487, .T. ) ;
#18859=CARTESIAN_POINT ( 'NONE',  ( 108.2857792741417597, -47.02760743735399984, 158.6822919425769669 ) ) ;
#18860=DIRECTION ( 'NONE',  ( 0.000000000000000000, 1.000000000000000000, 0.000000000000000000 ) ) ;
#18863=CARTESIAN_POINT ( 'NONE',  ( 142.8821648370248170, -72.54478064608022692, 540.9756252759101471 ) ) ;
#18864=CIRCLE ( 'NONE', #69634, 0.5000000000000031086 ) ;
#18867=CARTESIAN_POINT ( 'NONE',  ( 106.8416606513709866, -48.55305329746398257, 77.56133956162491927 ) ) ;
#18869=ORIENTED_EDGE ( 'NONE', *, *, #61272, .F. ) ;
#18870=AXIS2_PLACEMENT_3D ( 'NONE', #52420, #73340, #9790 ) ;
#18871=DIRECTION ( 'NONE',  ( 1.000000000000000078E-15, -1.000000000000000083E-30, -1.000000000000000000 ) ) ;
#18873=CARTESIAN_POINT ( 'NONE',  ( 31.78666935232998725, -36.02818131005891189, -5.074374724088000832 ) ) ;
#18874=ADVANCED_FACE ( 'NONE', ( #28397 ), #15689, .F. ) ;
#18875=CARTESIAN_POINT ( 'NONE',  ( 114.8702562078425160, -31.70976148532177064, 142.0995189410209605 ) ) ;
#18877=DIRECTION ( 'NONE',  ( 0.000000000000000000, 0.000000000000000000, -1.000000000000000000 ) ) ;
#18884=CARTESIAN_POINT ( 'NONE',  ( 50.87649884952499946, -33.54226604284930602, -5.074374724088000832 ) ) ;
#18885=CARTESIAN_POINT ( 'NONE',  ( 77.37801896924341349, -19.30949827216399939, 6.839365140900691920 ) ) ;
#18886=CARTESIAN_POINT ( 'NONE',  ( 98.55918112442081735, -40.71722039560211925, 208.0949166392299787 ) ) ;
#18887=CARTESIAN_POINT ( 'NONE',  ( 127.0664832912740394, -46.47944715994101017, -5.074374724089008915 ) ) ;
#18888=VECTOR ( 'NONE', #68535, 1000.000000000000000 ) ;
#18891=ORIENTED_EDGE ( 'NONE', *, *, #27144, .F. ) ;
#18892=VERTEX_POINT ( 'NONE', #2503 ) ;
#18893=EDGE_CURVE ( 'NONE', #59306, #69327, #40884, .T. ) ;
#18894=ORIENTED_EDGE ( 'NONE', *, *, #20630, .T. ) ;
#18895=VERTEX_POINT ( 'NONE', #57896 ) ;
#18896=VECTOR ( 'NONE', #7506, 1000.000000000000000 ) ;
#18897=CARTESIAN_POINT ( 'NONE',  ( 99.00663190570655559, -35.27291570150341471, 239.0023760838769817 ) ) ;
#18898=CARTESIAN_POINT ( 'NONE',  ( 104.1015100224914960, -46.74719628246504044, 107.3470538473389411 ) ) ;
#18899=CARTESIAN_POINT ( 'NONE',  ( 101.9712125536870957, -27.65933791914790874, 60.48419670448296159 ) ) ;
#18900=CARTESIAN_POINT ( 'NONE',  ( 99.08156578439323425, -35.73259618917102642, 249.5838068554173503 ) ) ;
#18901=DIRECTION ( 'NONE',  ( 0.000000000000000000, 0.000000000000000000, -1.000000000000000000 ) ) ;
#18903=CARTESIAN_POINT ( 'NONE',  ( 96.05396905170981370, -35.78154916559406473, 182.2461014663869889 ) ) ;
#18905=ORIENTED_EDGE ( 'NONE', *, *, #46406, .T. ) ;
#18906=LINE ( 'NONE', #60218, #39492 ) ;
#18908=ORIENTED_EDGE ( 'NONE', *, *, #55362, .F. ) ;
#18909=FACE_OUTER_BOUND ( 'NONE', #54619, .T. ) ;
#18910=LINE ( 'NONE', #87959, #80775 ) ;
#18911=AXIS2_PLACEMENT_3D ( 'NONE', #41536, #43334, #64248 ) ;
#18912=ORIENTED_EDGE ( 'NONE', *, *, #81598, .F. ) ;
#18913=CARTESIAN_POINT ( 'NONE',  ( 75.31670390244798341, -50.82844715994100682, 63.03480685541479289 ) ) ;
#18914=( BOUNDED_CURVE ( )  B_SPLINE_CURVE ( 3, ( #46629, #53881, #67536, #5323 ),
 .UNSPECIFIED., .F., .T. ) 
 B_SPLINE_CURVE_WITH_KNOTS ( ( 4, 4 ),
 ( 8.874879220657207072E-12, 1.570796326806122467 ),
 .UNSPECIFIED. ) 
 CURVE ( )  GEOMETRIC_REPRESENTATION_ITEM ( )  RATIONAL_B_SPLINE_CURVE ( ( 1.000000000000000000, 0.8047378541238108252, 0.8047378541238108252, 1.000000000000000000 ) ) 
 REPRESENTATION_ITEM ( '' )  );
#18916=CARTESIAN_POINT ( 'NONE',  ( 101.7558625676976618, -27.03530485730228250, 100.4632443235299633 ) ) ;
#18917=FACE_OUTER_BOUND ( 'NONE', #79591, .T. ) ;
#18918=FACE_OUTER_BOUND ( 'NONE', #50933, .T. ) ;
#18919=CARTESIAN_POINT ( 'NONE',  ( 107.0664832912739968, -36.72944715994100306, 287.6356252759109680 ) ) ;
#18920=CARTESIAN_POINT ( 'NONE',  ( 62.56670390244752156, -48.82844715994099971, 249.9678068554150343 ) ) ;
#18921=CARTESIAN_POINT ( 'NONE',  ( 97.81371332943018615, -40.52236848741042508, 56.63563370667147012 ) ) ;
#18922=CARTESIAN_POINT ( 'NONE',  ( 115.0229693000240303, -29.09019634776603169, 185.4232443235299570 ) ) ;
#18924=EDGE_CURVE ( 'NONE', #27372, #17890, #13339, .T. ) ;
#18927=CARTESIAN_POINT ( 'NONE',  ( 51.42025729302798709, -31.94127993907680718, -5.074374724088000832 ) ) ;
#18928=VECTOR ( 'NONE', #42432, 1000.000000000000000 ) ;
#18929=ADVANCED_FACE ( 'NONE', ( #83833 ), #49282, .F. ) ;
#18931=ADVANCED_FACE ( 'NONE', ( #49733 ), #31520, .F. ) ;
#18932=CARTESIAN_POINT ( 'NONE',  ( 97.33774252606986011, -34.07133272141320646, 136.1149023111836129 ) ) ;
#18933=CIRCLE ( 'NONE', #30480, 10.00000000000002665 ) ;
#18935=CARTESIAN_POINT ( 'NONE',  ( 115.2864439380202271, -30.18849607537921997, 244.3613395616249875 ) ) ;
#18936=ORIENTED_EDGE ( 'NONE', *, *, #82128, .F. ) ;
#18938=DIRECTION ( 'NONE',  ( 1.000000000000000000, 4.163336342344333240E-14, 0.000000000000000000 ) ) ;
#18939=CARTESIAN_POINT ( 'NONE',  ( 116.1584918543541960, -31.54133664852386332, 285.2384824187680579 ) ) ;
#18940=CARTESIAN_POINT ( 'NONE',  ( 102.6793653923444651, -46.92506852294805952, 133.2651490854349561 ) ) ;
#18942=CARTESIAN_POINT ( 'NONE',  ( 81.30994157254338006, -39.18303583363594100, 7.982915248818332365 ) ) ;
#18945=FACE_OUTER_BOUND ( 'NONE', #81649, .T. ) ;
#18947=ORIENTED_EDGE ( 'NONE', *, *, #51517, .T. ) ;
#18948=VECTOR ( 'NONE', #34105, 1000.000000000000000 ) ;
#18950=VERTEX_POINT ( 'NONE', #54072 ) ;
#18951=EDGE_CURVE ( 'NONE', #87720, #72723, #5520, .T. ) ;
#18952=AXIS2_PLACEMENT_3D ( 'NONE', #15004, #84516, #1376 ) ;
#18953=ORIENTED_EDGE ( 'NONE', *, *, #32996, .T. ) ;
#18955=CARTESIAN_POINT ( 'NONE',  ( 118.7081646409640427, -34.65111545711814500, 44.96705384733895272 ) ) ;
#18957=DIRECTION ( 'NONE',  ( -5.551115123125777653E-14, -1.000000000000000000, 0.000000000000000000 ) ) ;
#18958=DIRECTION ( 'NONE',  ( -1.000000000000000000, 9.376883653928684652E-16, 1.500301384628589584E-15 ) ) ;
#18960=CARTESIAN_POINT ( 'NONE',  ( 100.8994401894200053, -30.77800351108903598, 250.1381341137912671 ) ) ;
#18961=VERTEX_POINT ( 'NONE', #23408 ) ;
#18962=ORIENTED_EDGE ( 'NONE', *, *, #20117, .T. ) ;
#18963=VERTEX_POINT ( 'NONE', #16575 ) ;
#18964=PLANE ( 'NONE',  #25361 ) ;
#18965=CARTESIAN_POINT ( 'NONE',  ( 112.4094413778908148, -45.19673273518448298, 183.0243865414169022 ) ) ;
#18966=DIRECTION ( 'NONE',  ( -4.237773401492740281E-14, 1.000000000000000000, 0.000000000000000000 ) ) ;
#18968=CARTESIAN_POINT ( 'NONE',  ( 100.3317924633492737, -42.48897995906190772, 28.32158330589695794 ) ) ;
#18969=CIRCLE ( 'NONE', #52256, 2.117000000000007987 ) ;
#18971=AXIS2_PLACEMENT_3D ( 'NONE', #72798, #57823, #78744 ) ;
#18973=CARTESIAN_POINT ( 'NONE',  ( 105.1480534446306621, -26.53835310083740850, 280.2365776568638580 ) ) ;
#18974=DIRECTION ( 'NONE',  ( 0.000000000000000000, 0.000000000000000000, 1.000000000000000000 ) ) ;
#18976=CARTESIAN_POINT ( 'NONE',  ( 111.1099401812523979, -27.53270267244794667, 55.74708093204620241 ) ) ;
#18978=DIRECTION ( 'NONE',  ( -0.7071067811578587436, 0.7071067812152364018, 0.000000000000000000 ) ) ;
#18980=CARTESIAN_POINT ( 'NONE',  ( 111.5100823108406587, -29.30278217496053017, 52.47761417911495130 ) ) ;
#18984=CARTESIAN_POINT ( 'NONE',  ( 188.5667039024479834, -62.87844715994099687, 257.2178068554150059 ) ) ;
#18988=DIRECTION ( 'NONE',  ( 0.0001713722456129695634, -0.9999999853157764962, 0.000000000000000000 ) ) ;
#18991=CARTESIAN_POINT ( 'NONE',  ( 117.8755673099929453, -39.04089478637848032, 108.6708633711489824 ) ) ;
#18993=CARTESIAN_POINT ( 'NONE',  ( 107.7234663162357151, -28.21331511381966806, 69.43813411379096578 ) ) ;
#18994=CIRCLE ( 'NONE', #47955, 0.5000000000000004441 ) ;
#18995=AXIS2_PLACEMENT_3D ( 'NONE', #20328, #69367, #35725 ) ;
#18996=CARTESIAN_POINT ( 'NONE',  ( 182.4202572930400095, -33.70561438051981185, -5.074374724088000832 ) ) ;
#18997=CARTESIAN_POINT ( 'NONE',  ( 98.20303647727408247, -37.43757155718014928, 97.82158330589696504 ) ) ;
#19000=CARTESIAN_POINT ( 'NONE',  ( 106.9270610292626742, -26.24804662171751346, 56.08705384733997334 ) ) ;
#19001=CARTESIAN_POINT ( 'NONE',  ( 184.5667039024485518, -48.82844715993447693, 180.4678068554150343 ) ) ;
#19002=CARTESIAN_POINT ( 'NONE',  ( 99.04403941723640514, -42.84122471778974983, 256.8438871033408191 ) ) ;
#19003=VERTEX_POINT ( 'NONE', #23843 ) ;
#19004=ADVANCED_FACE ( 'NONE', ( #72431 ), #81826, .T. ) ;
#19006=ORIENTED_EDGE ( 'NONE', *, *, #21294, .T. ) ;
#19007=ORIENTED_EDGE ( 'NONE', *, *, #11540, .T. ) ;
#19009=FACE_OUTER_BOUND ( 'NONE', #48921, .T. ) ;
#19010=ORIENTED_EDGE ( 'NONE', *, *, #7154, .F. ) ;
#19011=CARTESIAN_POINT ( 'NONE',  ( 115.6529839569025455, -41.48189714014875307, 263.4241967044829948 ) ) ;
#19012=FACE_OUTER_BOUND ( 'NONE', #39565, .T. ) ;
#19013=CARTESIAN_POINT ( 'NONE',  ( 107.8683515708180636, -26.33524229811608919, 66.01562527591097762 ) ) ;
#19014=AXIS2_PLACEMENT_3D ( 'NONE', #33989, #54413, #12673 ) ;
#19015=CARTESIAN_POINT ( 'NONE',  ( 104.4926606602381014, -26.97806419231898545, 96.28046078532923957 ) ) ;
#19017=DIRECTION ( 'NONE',  ( -1.000000000000000078E-15, 1.000000000000000083E-30, 1.000000000000000000 ) ) ;
#19019=EDGE_LOOP ( 'NONE', ( #59989, #42503, #34045, #7970 ) ) ;
#19021=CARTESIAN_POINT ( 'NONE',  ( 107.0664832912739399, -36.72944715994095333, 293.6356252759109680 ) ) ;
#19022=CARTESIAN_POINT ( 'NONE',  ( 95.25611604350963546, -37.33230102880722967, 271.3670538473393776 ) ) ;
#19023=DIRECTION ( 'NONE',  ( 0.000000000000000000, 0.000000000000000000, 1.000000000000000000 ) ) ;
#19024=DIRECTION ( 'NONE',  ( -1.000000000000000078E-15, 1.000000000000000083E-30, 1.000000000000000000 ) ) ;
#19025=CARTESIAN_POINT ( 'NONE',  ( 100.8881267872233707, -44.70076677403937282, 92.05261961146344163 ) ) ;
#19026=CARTESIAN_POINT ( 'NONE',  ( 105.2433400634091925, -28.35518594498741507, 259.6695626852197734 ) ) ;
#19027=CARTESIAN_POINT ( 'NONE',  ( 108.6549043256371618, -26.75500537441465099, 99.95237438151097820 ) ) ;
#19028=CARTESIAN_POINT ( 'NONE',  ( 96.81317962367450036, -38.48968277746985933, 87.46133956162493917 ) ) ;
#19029=CARTESIAN_POINT ( 'NONE',  ( 165.9667039024459996, -26.71338133339301635, -5.074374724088000832 ) ) ;
#19030=CARTESIAN_POINT ( 'NONE',  ( 117.3534821530742107, -34.78408995979881269, 158.9756252759109714 ) ) ;
#19035=VECTOR ( 'NONE', #46405, 1000.000000000000000 ) ;
#19037=CARTESIAN_POINT ( 'NONE',  ( 134.2548946453517260, -33.97944715994100306, 1.625625275910998147 ) ) ;
#19039=VERTEX_POINT ( 'NONE', #38340 ) ;
#19041=CARTESIAN_POINT ( 'NONE',  ( 102.3405178495751215, -46.07139110582879482, 127.2041967044829960 ) ) ;
#19044=LINE ( 'NONE', #4969, #43565 ) ;
#19047=CARTESIAN_POINT ( 'NONE',  ( 109.6430121245902853, -46.48008673684198300, 118.7814586087551447 ) ) ;
#19048=CARTESIAN_POINT ( 'NONE',  ( 97.81169962758427516, -40.51743340529665005, 76.63548575323150658 ) ) ;
#19050=AXIS2_PLACEMENT_3D ( 'NONE', #75773, #355, #40341 ) ;
#19052=LINE ( 'NONE', #45396, #8042 ) ;
#19054=VERTEX_POINT ( 'NONE', #61351 ) ;
#19055=EDGE_CURVE ( 'NONE', #26390, #29421, #67022, .T. ) ;
#19057=DIRECTION ( 'NONE',  ( 0.000000000000000000, 1.000000000000000000, 0.000000000000000000 ) ) ;
#19060=EDGE_CURVE ( 'NONE', #25721, #54206, #19579, .T. ) ;
#19064=DIRECTION ( 'NONE',  ( 0.000000000000000000, 0.000000000000000000, -1.000000000000000000 ) ) ;
#19065=CARTESIAN_POINT ( 'NONE',  ( 97.70662569943051778, -40.25148919734539277, 181.6128704218694168 ) ) ;
#19068=CARTESIAN_POINT ( 'NONE',  ( 109.4488926988246504, -27.20905326525217660, 195.8813395616249977 ) ) ;
#19071=EDGE_LOOP ( 'NONE', ( #33926, #89221, #42956, #86525 ) ) ;
#19072=CARTESIAN_POINT ( 'NONE',  ( 103.6990349130722677, -26.13358598113153164, 51.32133956162493149 ) ) ;
#19073=CARTESIAN_POINT ( 'NONE',  ( 112.4075703148740644, -45.19790706062806862, 53.02421102707163669 ) ) ;
#19074=LINE ( 'NONE', #81768, #44167 ) ;
#19075=VECTOR ( 'NONE', #37480, 1000.000000000000000 ) ;
#19076=DIRECTION ( 'NONE',  ( -0.000000000000000000, 1.000000000000000000, 0.000000000000000000 ) ) ;
#19079=VERTEX_POINT ( 'NONE', #44703 ) ;
#19080=ORIENTED_EDGE ( 'NONE', *, *, #65080, .T. ) ;
#19081=CARTESIAN_POINT ( 'NONE',  ( 100.1609931986295976, -31.17584605865120295, 237.2187261630399746 ) ) ;
#19082=CARTESIAN_POINT ( 'NONE',  ( 115.0392291604921127, -42.90596946611127294, 54.30216204422613657 ) ) ;
#19084=ADVANCED_FACE ( 'NONE', ( #51511 ), #79706, .T. ) ;
#19085=CARTESIAN_POINT ( 'NONE',  ( 25.56670390244797275, -65.37844715994100397, 142.0928068554150059 ) ) ;
#19086=CARTESIAN_POINT ( 'NONE',  ( 165.9667039024476196, -26.71338133338713305, 193.9678068554149775 ) ) ;
#19087=AXIS2_PLACEMENT_3D ( 'NONE', #2089, #29794, #22539 ) ;
#19088=EDGE_LOOP ( 'NONE', ( #1798, #60811, #79950, #16627, #39719, #71983, #40549, #60676, #10131 ) ) ;
#19090=LINE ( 'NONE', #40427, #12151 ) ;
#19091=ORIENTED_EDGE ( 'NONE', *, *, #67463, .F. ) ;
#19092=CARTESIAN_POINT ( 'NONE',  ( 109.2074818670226222, -48.35976665079991221, 277.7213395616254843 ) ) ;
#19093=VERTEX_POINT ( 'NONE', #5972 ) ;
#19095=CARTESIAN_POINT ( 'NONE',  ( 104.6179474607139213, -28.94263790944830106, 248.1366617981629474 ) ) ;
#19097=CARTESIAN_POINT ( 'NONE',  ( 113.2097911582632861, -29.11871762112820150, 164.5356252759109736 ) ) ;
#19099=CARTESIAN_POINT ( 'NONE',  ( 49.16670390244647137, -26.71338133339277121, 193.9678068554150911 ) ) ;
#19101=AXIS2_PLACEMENT_3D ( 'NONE', #64969, #85879, #51313 ) ;
#19102=B_SPLINE_CURVE_WITH_KNOTS ( 'NONE', 3,
 ( #3397, #52831, #87856, #51961, #31090, #86528, #59676, #66503, #16587, #79717, #87407, #52394, #18353, #46039, #80160, #11558, #24295, #2955 ),
 .UNSPECIFIED., .F., .F.,
 ( 4, 2, 2, 2, 2, 2, 2, 2, 4 ),
 ( 0.000000000000000000, 0.06249958877818252018, 0.1249991775563650404, 0.1874987663345475675, 0.2499983551127300807, 0.3124979438909126217, 0.3749975326690951349, 0.4374971214472776482, 0.4999967102254601614 ),
 .UNSPECIFIED. ) ;
#19103=CARTESIAN_POINT ( 'NONE',  ( 115.5527055449870772, -29.57532036350955806, 220.3718157521019521 ) ) ;
#19105=EDGE_LOOP ( 'NONE', ( #29358, #64834, #54730, #59920 ) ) ;
#19106=VECTOR ( 'NONE', #29759, 1000.000000000000000 ) ;
#19107=B_SPLINE_CURVE_WITH_KNOTS ( 'NONE', 3,
 ( #17827, #31006, #17386, #58700, #80073, #23336, #80514, #25085, #24208, #38267, #9239, #86440, #11004, #52749, #85558, #3315, #71914, #43740, #71477, #30126, #65089, #51002, #37836, #23770, #36937, #51875, #65963, #16499, #2872, #30570, #58269 ),
 .UNSPECIFIED., .F., .F.,
 ( 4, 2, 2, 1, 2, 2, 2, 2, 2, 2, 2, 1, 1, 2, 2, 2, 4 ),
 ( 0.000000000000000000, 0.06249999999999088229, 0.09374999999998391564, 0.1093749999999804184, 0.1171874999999810013, 0.1249999999999815842, 0.1874999999999718558, 0.2187499999999680811, 0.2499999999999643063, 0.3124999999999580891, 0.3437499999999560907, 0.3593749999999550915, 0.3671874999999563682, 0.3710937499999579225, 0.3749999999999594213, 0.4374999999999796829, 0.5000000000000000000 ),
 .UNSPECIFIED. ) ;
#19108=CARTESIAN_POINT ( 'NONE',  ( 96.04171114508396556, -38.01470880000633201, 82.43086337114895912 ) ) ;
#19111=VERTEX_POINT ( 'NONE', #37905 ) ;
#19112=VERTEX_POINT ( 'NONE', #74997 ) ;
#19113=ADVANCED_FACE ( 'NONE', ( #68189 ), #33214, .T. ) ;
#19114=ORIENTED_EDGE ( 'NONE', *, *, #26850, .T. ) ;
#19116=CARTESIAN_POINT ( 'NONE',  ( 29.56670390244797630, -48.82844715994099971, 300.9178068554150514 ) ) ;
#19117=DIRECTION ( 'NONE',  ( 1.000000000000000078E-15, -1.000000000000000083E-30, -1.000000000000000000 ) ) ;
#19118=CARTESIAN_POINT ( 'NONE',  ( 188.5667039024479834, -62.87844715994099687, 290.4678068554150627 ) ) ;
#19119=CARTESIAN_POINT ( 'NONE',  ( 108.0140583617620820, -28.59404368299928123, 127.8023760838769505 ) ) ;
#19120=CARTESIAN_POINT ( 'NONE',  ( 116.5464386332369600, -41.20266105201044127, 224.4756252759109714 ) ) ;
#19122=AXIS2_PLACEMENT_3D ( 'NONE', #4680, #32360, #60062 ) ;
#19124=EDGE_LOOP ( 'NONE', ( #34824, #36264 ) ) ;
#19126=EDGE_CURVE ( 'NONE', #17346, #30864, #45220, .T. ) ;
#19127=DIRECTION ( 'NONE',  ( 0.000000000000000000, 1.000000000000000000, 0.000000000000000000 ) ) ;
#19129=VECTOR ( 'NONE', #19057, 1000.000000000000000 ) ;
#19130=ORIENTED_EDGE ( 'NONE', *, *, #1498, .F. ) ;
#19131=ADVANCED_FACE ( 'NONE', ( #20495, #55865 ), #14575, .T. ) ;
#19135=ORIENTED_EDGE ( 'NONE', *, *, #45799, .T. ) ;
#19141=CARTESIAN_POINT ( 'NONE',  ( 99.37165735872611094, -40.43697808898449608, 171.1067055423629597 ) ) ;
#19143=CARTESIAN_POINT ( 'NONE',  ( 106.5157732221739195, -25.64298685704507363, 45.12800622829193742 ) ) ;
#19145=CARTESIAN_POINT ( 'NONE',  ( 98.34945445922909357, -31.65731027460955005, 126.9065242933907456 ) ) ;
#19146=ORIENTED_EDGE ( 'NONE', *, *, #78631, .T. ) ;
#19147=FACE_OUTER_BOUND ( 'NONE', #79873, .T. ) ;
#19151=CARTESIAN_POINT ( 'NONE',  ( 97.31587469922506273, -39.30605313450122651, 262.5315195711698379 ) ) ;
#19153=EDGE_LOOP ( 'NONE', ( #59815, #10726, #75228, #16436, #58537 ) ) ;
#19154=CARTESIAN_POINT ( 'NONE',  ( 105.0763451348094861, -26.90764585894701710, 166.2350905474758065 ) ) ;
#19157=DIRECTION ( 'NONE',  ( 0.000000000000000000, 0.000000000000000000, -1.000000000000000000 ) ) ;
#19158=ORIENTED_EDGE ( 'NONE', *, *, #39739, .F. ) ;
#19159=CARTESIAN_POINT ( 'NONE',  ( 111.1376129892989013, -47.03096861136451423, 22.88800622829195675 ) ) ;
#19160=CARTESIAN_POINT ( 'NONE',  ( 115.0558824863888390, -43.54908903376227158, 59.26419670448196086 ) ) ;
#19162=CARTESIAN_POINT ( 'NONE',  ( 151.0371591254585155, -46.82818131005592477, 117.4678068554150485 ) ) ;
#19164=CARTESIAN_POINT ( 'NONE',  ( 97.31584198560500454, -39.30596968595895646, 147.5320030024637674 ) ) ;
#19165=FACE_OUTER_BOUND ( 'NONE', #26560, .T. ) ;
#19167=CARTESIAN_POINT ( 'NONE',  ( 100.2650085812441461, -33.56876024586312468, 9.125625275910969947 ) ) ;
#19168=ADVANCED_FACE ( 'NONE', ( #34993 ), #15015, .F. ) ;
#19169=ADVANCED_FACE ( 'NONE', ( #82730 ), #69531, .T. ) ;
#19172=CARTESIAN_POINT ( 'NONE',  ( 104.7257947241298979, -47.57997989614905521, 32.41943479972098174 ) ) ;
#19173=CARTESIAN_POINT ( 'NONE',  ( 116.8574199659429098, -40.30995640862995799, 214.5470538473389581 ) ) ;
#19174=CARTESIAN_POINT ( 'NONE',  ( 112.5256494142567192, -27.82244069900259476, 90.63848241876793566 ) ) ;
#19175=EDGE_CURVE ( 'NONE', #70797, #79957, #8203, .T. ) ;
#19177=CARTESIAN_POINT ( 'NONE',  ( 98.38064376042838433, -41.69566365478069514, 171.7393974040084288 ) ) ;
#19178=CARTESIAN_POINT ( 'NONE',  ( 134.0664832912740110, -46.42944715994100591, 4.925625275910997303 ) ) ;
#19180=VECTOR ( 'NONE', #79344, 1000.000000000000000 ) ;
#19183=CARTESIAN_POINT ( 'NONE',  ( 113.4367438382843716, -44.15125393826585309, 104.1413395616249744 ) ) ;
#19185=ORIENTED_EDGE ( 'NONE', *, *, #71219, .F. ) ;
#19186=CARTESIAN_POINT ( 'NONE',  ( 118.0585799961420577, -32.36802338489823683, 245.1270538473389706 ) ) ;
#19187=LINE ( 'NONE', #74150, #57077 ) ;
#19191=CARTESIAN_POINT ( 'NONE',  ( 71.23990787207000608, 10.64204399490126463, 396.9756252759102040 ) ) ;
#19192=AXIS2_PLACEMENT_3D ( 'NONE', #34845, #35734, #7150 ) ;
#19193=CARTESIAN_POINT ( 'NONE',  ( 133.8780722764277868, -39.47944715994101728, 1.625625275910997258 ) ) ;
#19195=CARTESIAN_POINT ( 'NONE',  ( 96.03815445040686427, -38.18343476501375022, 151.4299109901969871 ) ) ;
#19197=ORIENTED_EDGE ( 'NONE', *, *, #18304, .T. ) ;
#19198=CARTESIAN_POINT ( 'NONE',  ( 115.6883067454668463, -38.90345035940969609, 120.0615833058969457 ) ) ;
#19201=CARTESIAN_POINT ( 'NONE',  ( 109.0793648129487678, -47.66380996059997699, 273.7213395616246885 ) ) ;
#19203=FACE_OUTER_BOUND ( 'NONE', #46220, .T. ) ;
#19207=CARTESIAN_POINT ( 'NONE',  ( 194.5664832912729878, -71.37844715994266664, 342.9256252759109884 ) ) ;
#19208=DIRECTION ( 'NONE',  ( -0.000000000000000000, -0.000000000000000000, 1.000000000000000000 ) ) ;
#19209=CARTESIAN_POINT ( 'NONE',  ( 118.8526415125689937, -37.69623653580512723, 188.7613395616259595 ) ) ;
#19210=CARTESIAN_POINT ( 'NONE',  ( 112.1406058298522197, -28.01353614044138496, 169.6558318805149668 ) ) ;
#19211=ORIENTED_EDGE ( 'NONE', *, *, #23257, .T. ) ;
#19214=LINE ( 'NONE', #5132, #33080 ) ;
#19215=LINE ( 'NONE', #54593, #30211 ) ;
#19220=EDGE_CURVE ( 'NONE', #77666, #40553, #56430, .T. ) ;
#19221=CARTESIAN_POINT ( 'NONE',  ( 116.3775870818408151, -41.41883695635522145, 203.4556252759109611 ) ) ;
#19222=EDGE_CURVE ( 'NONE', #11460, #82260, #483, .T. ) ;
#19223=CARTESIAN_POINT ( 'NONE',  ( 59.67079009362632291, -0.9310397146383332379, 540.9756252759101471 ) ) ;
#19224=ORIENTED_EDGE ( 'NONE', *, *, #73141, .T. ) ;
#19226=AXIS2_PLACEMENT_3D ( 'NONE', #47085, #40288, #18958 ) ;
#19227=LINE ( 'NONE', #46901, #2817 ) ;
#19228=DIRECTION ( 'NONE',  ( 0.000000000000000000, 0.000000000000000000, 1.000000000000000000 ) ) ;
#19229=CARTESIAN_POINT ( 'NONE',  ( 112.0650627701821094, -45.48886962380960597, 163.9897151582021593 ) ) ;
#19230=CARTESIAN_POINT ( 'NONE',  ( 115.6864120445923163, -37.50259225211298286, 31.56142370292397459 ) ) ;
#19231=CARTESIAN_POINT ( 'NONE',  ( 109.0764703591063522, -47.62188296335364157, 123.7337205140059666 ) ) ;
#19232=EDGE_CURVE ( 'NONE', #66717, #8294, #28634, .T. ) ;
#19233=DIRECTION ( 'NONE',  ( 0.000000000000000000, 0.000000000000000000, 1.000000000000000000 ) ) ;
#19234=VERTEX_POINT ( 'NONE', #84067 ) ;
#19235=EDGE_CURVE ( 'NONE', #64042, #72016, #6400, .T. ) ;
#19236=DIRECTION ( 'NONE',  ( -1.000000000000000078E-15, 0.000000000000000000, 1.000000000000000000 ) ) ;
#19239=ORIENTED_EDGE ( 'NONE', *, *, #22071, .T. ) ;
#19240=ADVANCED_FACE ( 'NONE', ( #61797 ), #89534, .F. ) ;
#19242=CARTESIAN_POINT ( 'NONE',  ( 172.5664832912740110, -18.82844715994099971, 16.80862527591200006 ) ) ;
#19244=VERTEX_POINT ( 'NONE', #6848 ) ;
#19245=DIRECTION ( 'NONE',  ( 0.000000000000000000, 1.000000000000000000, 2.000000000000000155E-15 ) ) ;
#19246=EDGE_CURVE ( 'NONE', #48350, #66137, #34549, .T. ) ;
#19247=CARTESIAN_POINT ( 'NONE',  ( 104.5891003629744631, -45.44008686965874944, 66.79051506617194889 ) ) ;
#19248=CARTESIAN_POINT ( 'NONE',  ( 98.51948014227190242, -30.72152729218522538, 205.8384824187679669 ) ) ;
#19249=CARTESIAN_POINT ( 'NONE',  ( 108.3633857348901586, -47.68307073960303910, 162.6822919425769669 ) ) ;
#19250=CARTESIAN_POINT ( 'NONE',  ( 115.3155962437203073, -42.52683630334157527, 23.33992995560114991 ) ) ;
#19251=CARTESIAN_POINT ( 'NONE',  ( 105.8935855965125938, -47.12395608077676457, 278.4870538473395527 ) ) ;
#19253=CARTESIAN_POINT ( 'NONE',  ( 194.0371591254575208, -24.89890238294407254, 180.4678068554150343 ) ) ;
#19254=ORIENTED_EDGE ( 'NONE', *, *, #52021, .F. ) ;
#19255=AXIS2_PLACEMENT_3D ( 'NONE', #13851, #6587, #70156 ) ;
#19257=ORIENTED_EDGE ( 'NONE', *, *, #3317, .F. ) ;
#19258=EDGE_CURVE ( 'NONE', #14322, #33917, #1343, .T. ) ;
#19259=VECTOR ( 'NONE', #87848, 1000.000000000000114 ) ;
#19261=CARTESIAN_POINT ( 'NONE',  ( 101.3806489482690694, -45.56251468762313550, 222.1213395616249784 ) ) ;
#19262=VERTEX_POINT ( 'NONE', #43591 ) ;
#19263=CARTESIAN_POINT ( 'NONE',  ( 102.2371489609593880, -45.96874152625851906, 212.1927681330539599 ) ) ;
#19264=DIRECTION ( 'NONE',  ( 0.000000000000000000, 0.000000000000000000, 1.000000000000000000 ) ) ;
#19265=DIRECTION ( 'NONE',  ( 0.000000000000000000, 0.000000000000000000, 1.000000000000000000 ) ) ;
#19266=CARTESIAN_POINT ( 'NONE',  ( 97.82515092478139707, -40.55017472135673984, 22.63844333753277738 ) ) ;
#19268=CARTESIAN_POINT ( 'NONE',  ( 101.9785357346435148, -30.23611602480990257, 277.6356252759111385 ) ) ;
#19271=CARTESIAN_POINT ( 'NONE',  ( 33.91903122894598965, -35.91149509761181235, 237.4678068554150059 ) ) ;
#19272=AXIS2_PLACEMENT_3D ( 'NONE', #56453, #21060, #48733 ) ;
#19273=PLANE ( 'NONE',  #54233 ) ;
#19274=LINE ( 'NONE', #18821, #778 ) ;
#19275=CARTESIAN_POINT ( 'NONE',  ( 115.0821792353001740, -30.60892512433434831, 39.34390919315809043 ) ) ;
#19278=CARTESIAN_POINT ( 'NONE',  ( 101.1531192966442347, -28.75920026314567934, 195.5838068554172082 ) ) ;
#19280=CARTESIAN_POINT ( 'NONE',  ( 136.7765779009448579, -19.19711456031681251, 6.808568500764772935 ) ) ;
#19281=CARTESIAN_POINT ( 'NONE',  ( 99.06899620534126427, -29.95238561887155981, 215.7670538473399517 ) ) ;
#19282=CARTESIAN_POINT ( 'NONE',  ( 104.9628592394672069, -25.06714115267218546, 121.2184824187679766 ) ) ;
#19283=CARTESIAN_POINT ( 'NONE',  ( 110.0014563237810137, -26.68062070874399438, 255.8499109901966051 ) ) ;
#19284=DIRECTION ( 'NONE',  ( -1.000000000000000078E-15, -1.000000000000000083E-30, 1.000000000000000000 ) ) ;
#19285=ADVANCED_FACE ( 'NONE', ( #64064, #15475 ), #43145, .F. ) ;
#19287=FACE_OUTER_BOUND ( 'NONE', #77885, .T. ) ;
#19288=DIRECTION ( 'NONE',  ( 0.000000000000000000, 2.135044278125299371E-15, -1.000000000000000000 ) ) ;
#19289=DIRECTION ( 'NONE',  ( 0.000000000000000000, 0.000000000000000000, 1.000000000000000000 ) ) ;
#19291=ORIENTED_EDGE ( 'NONE', *, *, #25713, .T. ) ;
#19292=ORIENTED_EDGE ( 'NONE', *, *, #34732, .F. ) ;
#19293=CARTESIAN_POINT ( 'NONE',  ( 100.0120368033278311, -41.59636475471172901, 126.2295626852199746 ) ) ;
#19295=ORIENTED_EDGE ( 'NONE', *, *, #64704, .T. ) ;
#19296=VECTOR ( 'NONE', #26553, 1000.000000000000000 ) ;
#19298=CARTESIAN_POINT ( 'NONE',  ( 97.63679352021421209, -31.00714225716596673, 121.8803871806729546 ) ) ;
#19299=FACE_OUTER_BOUND ( 'NONE', #56508, .T. ) ;
#19300=DIRECTION ( 'NONE',  ( -0.000000000000000000, -0.000000000000000000, 1.000000000000000000 ) ) ;
#19302=CARTESIAN_POINT ( 'NONE',  ( 116.8171228663878907, -34.15291832029765828, 110.0314586092749778 ) ) ;
#19303=CARTESIAN_POINT ( 'NONE',  ( 99.96923091713365750, -43.45941328387855407, 81.92991099019697288 ) ) ;
#19306=ORIENTED_EDGE ( 'NONE', *, *, #57290, .T. ) ;
#19307=VECTOR ( 'NONE', #77398, 1000.000000000000000 ) ;
#19308=ADVANCED_FACE ( 'NONE', ( #71771, #86289, #57222, #72660, #51291, #56777, #23199, #50866, #79038, #78604, #16803, #10427, #65394, #37247, #22283, #70886, #30433, #49958, #72217 ), #2733, .F. ) ;
#19309=CARTESIAN_POINT ( 'NONE',  ( 177.8371591254544910, -47.82818131005477369, 193.9678068554150059 ) ) ;
#19310=CARTESIAN_POINT ( 'NONE',  ( 116.4020974974655047, -33.81230083437814216, 170.0670538473389684 ) ) ;
#19311=CARTESIAN_POINT ( 'NONE',  ( 97.81169789812091153, -40.51742632959496859, 107.6355761348045519 ) ) ;
#19314=CARTESIAN_POINT ( 'NONE',  ( 31.89136050872298966, -31.76306994223740432, 237.4678068554150059 ) ) ;
#19315=CARTESIAN_POINT ( 'NONE',  ( 116.1804594027163660, -40.96476762480074996, 3.024967495036159804 ) ) ;
#19317=CARTESIAN_POINT ( 'NONE',  ( 117.0854383170106559, -39.53109055650223524, 98.60991099019594230 ) ) ;
#19318=ORIENTED_EDGE ( 'NONE', *, *, #66289, .T. ) ;
#19319=ORIENTED_EDGE ( 'NONE', *, *, #88046, .F. ) ;
#19320=CARTESIAN_POINT ( 'NONE',  ( 19.56648329127400032, -18.82844715994099971, 342.9256252759119548 ) ) ;
#19323=CARTESIAN_POINT ( 'NONE',  ( 106.0125404296577045, -27.51070622278902533, 157.9852332267339534 ) ) ;
#19325=AXIS2_PLACEMENT_3D ( 'NONE', #18585, #60353, #53065 ) ;
#19326=AXIS2_PLACEMENT_3D ( 'NONE', #48259, #54172, #33315 ) ;
#19327=ADVANCED_FACE ( 'NONE', ( #8656, #36799 ), #84967, .F. ) ;
#19329=VECTOR ( 'NONE', #24193, 1000.000000000000000 ) ;
#19332=ORIENTED_EDGE ( 'NONE', *, *, #52908, .F. ) ;
#19333=DIRECTION ( 'NONE',  ( 3.999999999999999995E-14, -1.000000000000000000, 4.100000000000000342E-29 ) ) ;
#19335=CARTESIAN_POINT ( 'NONE',  ( 136.6368519841215345, -19.70758306363340395, 2.855952960430312881 ) ) ;
#19336=ORIENTED_EDGE ( 'NONE', *, *, #84686, .T. ) ;
#19338=CARTESIAN_POINT ( 'NONE',  ( 77.74802179993506002, -20.20859666167768154, 7.273989459507554933 ) ) ;
#19339=CARTESIAN_POINT ( 'NONE',  ( 99.29109958770327182, -40.98052783126505005, 218.1558690201829620 ) ) ;
#19340=ADVANCED_FACE ( 'NONE', ( #44036 ), #2287, .F. ) ;
#19343=ORIENTED_EDGE ( 'NONE', *, *, #83635, .T. ) ;
#19344=EDGE_LOOP ( 'NONE', ( #57050, #83683, #27603, #62389 ) ) ;
#19347=TOROIDAL_SURFACE ( 'NONE', #12084, 11.75000000000000000, 2.125000000000000000 ) ;
#19351=CARTESIAN_POINT ( 'NONE',  ( 116.2459175369934172, -38.08366948007849118, 221.5280903695909842 ) ) ;
#19352=VECTOR ( 'NONE', #64554, 1000.000000000000000 ) ;
#19353=CARTESIAN_POINT ( 'NONE',  ( 96.06419827846988824, -38.01208726283962847, 86.43086337114897333 ) ) ;
#19354=CARTESIAN_POINT ( 'NONE',  ( 107.2318599658364207, -25.70055450771768690, 80.07657765686299456 ) ) ;
#19355=CARTESIAN_POINT ( 'NONE',  ( 113.1205385969929438, -43.14583419566791633, 249.5838068554168672 ) ) ;
#19357=DIRECTION ( 'NONE',  ( 1.000000000000000000, 1.806816776397999960E-14, 8.991631831580328678E-43 ) ) ;
#19358=CARTESIAN_POINT ( 'NONE',  ( 116.3773924821832111, -41.41873894932305689, 199.4556252759109611 ) ) ;
#19362=EDGE_LOOP ( 'NONE', ( #20520, #73083, #15418, #44545 ) ) ;
#19363=ORIENTED_EDGE ( 'NONE', *, *, #69578, .T. ) ;
#19364=DIRECTION ( 'NONE',  ( 0.000000000000000000, 0.000000000000000000, -1.000000000000000000 ) ) ;
#19365=VERTEX_POINT ( 'NONE', #39905 ) ;
#19366=AXIS2_PLACEMENT_3D ( 'NONE', #12643, #67599, #80799 ) ;
#19369=CARTESIAN_POINT ( 'NONE',  ( 113.8565348333340665, -44.64034031543166492, 108.1413395616249744 ) ) ;
#19370=CARTESIAN_POINT ( 'NONE',  ( 116.3186249068845939, -32.94868901192853627, 254.1356252759109395 ) ) ;
#19371=DIRECTION ( 'NONE',  ( -0.7071067811865336949, -0.7071067811865614505, 0.000000000000000000 ) ) ;
#19373=CARTESIAN_POINT ( 'NONE',  ( 115.0372575035121940, -42.90846257061950553, 144.3022919421925678 ) ) ;
#19374=DIRECTION ( 'NONE',  ( 0.000000000000000000, 0.000000000000000000, -1.000000000000000000 ) ) ;
#19375=CARTESIAN_POINT ( 'NONE',  ( 97.11708974113240345, -41.49110554365059045, 212.6937205140059461 ) ) ;
#19376=DIRECTION ( 'NONE',  ( -0.7071067811855830110, -0.7071067811875120235, 0.000000000000000000 ) ) ;
#19378=VERTEX_POINT ( 'NONE', #73990 ) ;
#19379=CARTESIAN_POINT ( 'NONE',  ( 106.5139905941028360, -24.40372801450956430, 320.5359728645732389 ) ) ;
#19380=LINE ( 'NONE', #82078, #36960 ) ;
#19381=DIRECTION ( 'NONE',  ( -4.237773401492740281E-14, 1.000000000000000000, 0.000000000000000000 ) ) ;
#19383=CARTESIAN_POINT ( 'NONE',  ( 110.8326918741827711, -26.28777313046090569, 249.7889586092445882 ) ) ;
#19384=EDGE_LOOP ( 'NONE', ( #34254, #11933 ) ) ;
#19385=CARTESIAN_POINT ( 'NONE',  ( 107.0664832912748068, -36.72944715993923381, -5.074374724089029343 ) ) ;
#19386=CARTESIAN_POINT ( 'NONE',  ( 118.3644662943939636, -33.07169432158188727, 280.0756252759109657 ) ) ;
#19387=CARTESIAN_POINT ( 'NONE',  ( 117.2805452986850412, -39.02698501918706597, 144.6499109901969859 ) ) ;
#19389=EDGE_CURVE ( 'NONE', #23550, #32370, #59892, .T. ) ;
#19390=CARTESIAN_POINT ( 'NONE',  ( 71.24162159452610865, 0.6420441417434794573, 540.9756252759101471 ) ) ;
#19391=CARTESIAN_POINT ( 'NONE',  ( 51.06648329127400388, -8.350947159940998787, 330.8831252759119934 ) ) ;
#19392=LINE ( 'NONE', #54773, #15283 ) ;
#19393=FACE_OUTER_BOUND ( 'NONE', #38199, .T. ) ;
#19394=CARTESIAN_POINT ( 'NONE',  ( 80.06648329127399677, -8.729447159940999512, 296.1531252759119752 ) ) ;
#19396=AXIS2_PLACEMENT_3D ( 'NONE', #4413, #32100, #27089 ) ;
#19398=ORIENTED_EDGE ( 'NONE', *, *, #89619, .T. ) ;
#19399=ORIENTED_EDGE ( 'NONE', *, *, #54686, .T. ) ;
#19400=DIRECTION ( 'NONE',  ( 0.000000000000000000, 0.000000000000000000, -1.000000000000000000 ) ) ;
#19401=CARTESIAN_POINT ( 'NONE',  ( 117.3629797429380659, -38.21633193987522503, 24.71276813305395237 ) ) ;
#19402=CARTESIAN_POINT ( 'NONE',  ( 77.31648329127399677, -18.72944715994106346, -5.074374724089059541 ) ) ;
#19403=CARTESIAN_POINT ( 'NONE',  ( 117.0707351141037833, -37.57509454027182016, 118.7609861400189715 ) ) ;
#19405=CARTESIAN_POINT ( 'NONE',  ( 107.0664832912739399, -36.72944715994095333, 315.6356252759111953 ) ) ;
#19406=CARTESIAN_POINT ( 'NONE',  ( 98.63267121701338169, -35.20533560836722131, 240.6067055423629597 ) ) ;
#19408=VERTEX_POINT ( 'NONE', #59450 ) ;
#19410=EDGE_CURVE ( 'NONE', #83042, #71543, #88531, .T. ) ;
#19411=CIRCLE ( 'NONE', #70177, 13.44999999999999396 ) ;
#19412=CARTESIAN_POINT ( 'NONE',  ( 51.06648329127400388, -8.350947159940998787, 333.4006252759120343 ) ) ;
#19413=VECTOR ( 'NONE', #42069, 1000.000000000000114 ) ;
#19414=CARTESIAN_POINT ( 'NONE',  ( 116.9901879630660630, -35.35324060233794796, 183.9360659761157990 ) ) ;
#19415=CARTESIAN_POINT ( 'NONE',  ( 29.56670390244797630, -67.87844715994100397, 20.91780685541479912 ) ) ;
#19416=DIRECTION ( 'NONE',  ( 3.999999999999999995E-14, -1.000000000000000000, 4.100000000000000342E-29 ) ) ;
#19417=CARTESIAN_POINT ( 'NONE',  ( 115.9456366428866119, -37.20155953748186306, 15.21586902018295895 ) ) ;
#19419=CARTESIAN_POINT ( 'NONE',  ( 107.0664832912739399, -36.72944715994095333, 315.6356252759111953 ) ) ;
#19420=CARTESIAN_POINT ( 'NONE',  ( 104.7413500955949672, -27.22895272701804359, 285.2670538473402075 ) ) ;
#19421=DIRECTION ( 'NONE',  ( -1.000000000000000078E-15, 1.000000000000000083E-30, 1.000000000000000000 ) ) ;
#19422=ORIENTED_EDGE ( 'NONE', *, *, #51301, .T. ) ;
#19423=DIRECTION ( 'NONE',  ( -1.000000000000000000, -4.299999999999999979E-14, -1.000000000000000078E-15 ) ) ;
#19424=CYLINDRICAL_SURFACE ( 'NONE', #1762, 0.5000000000000104361 ) ;
#19425=CARTESIAN_POINT ( 'NONE',  ( 100.8503319422675020, -42.75110701849109063, 39.76904275054393878 ) ) ;
#19426=CARTESIAN_POINT ( 'NONE',  ( 105.8259002483207922, -25.33766151058717142, 321.6188579224977389 ) ) ;
#19427=DIRECTION ( 'NONE',  ( 0.000000000000000000, -1.000000000000000000, 0.000000000000000000 ) ) ;
#19429=CARTESIAN_POINT ( 'NONE',  ( 129.8079539024480482, -42.97311385574000298, 207.5838068554170377 ) ) ;
#19431=CARTESIAN_POINT ( 'NONE',  ( 78.22143491581488206, -34.68812225914982861, 7.662832107313313657 ) ) ;
#19432=EDGE_CURVE ( 'NONE', #78028, #17169, #3608, .T. ) ;
#19433=ORIENTED_EDGE ( 'NONE', *, *, #60736, .F. ) ;
#19434=CARTESIAN_POINT ( 'NONE',  ( 113.3148160382734773, -28.33991531616941728, 104.5670538473399347 ) ) ;
#19435=ORIENTED_EDGE ( 'NONE', *, *, #15262, .F. ) ;
#19436=EDGE_CURVE ( 'NONE', #31238, #52939, #79683, .T. ) ;
#19437=CARTESIAN_POINT ( 'NONE',  ( 102.2116477823090293, -29.08462914334738869, 64.93718173283896533 ) ) ;
#19438=CARTESIAN_POINT ( 'NONE',  ( 98.22417599084440099, -41.40637017319168933, 87.71314181957467326 ) ) ;
#19439=CARTESIAN_POINT ( 'NONE',  ( 113.5614835896806625, -43.51851901557028413, 109.6034880678019618 ) ) ;
#19441=DIRECTION ( 'NONE',  ( 0.000000000000000000, 0.000000000000000000, -1.000000000000000000 ) ) ;
#19443=CARTESIAN_POINT ( 'NONE',  ( 115.0392540076567656, -43.53489519176116573, 59.26419670448196086 ) ) ;
#19445=AXIS2_PLACEMENT_3D ( 'NONE', #10553, #18260, #52740 ) ;
#19446=CARTESIAN_POINT ( 'NONE',  ( 116.7950397785617156, -39.38813467484644093, 258.6147150626158577 ) ) ;
#19447=ORIENTED_EDGE ( 'NONE', *, *, #11573, .F. ) ;
#19448=CARTESIAN_POINT ( 'NONE',  ( 77.67297288198761862, -20.08739819368273061, 2.653088468860025362 ) ) ;
#19450=VECTOR ( 'NONE', #16024, 1000.000000000000000 ) ;
#19451=ORIENTED_EDGE ( 'NONE', *, *, #45869, .T. ) ;
#19454=DIRECTION ( 'NONE',  ( -3.360405532702990443E-14, 1.000000000000000000, 0.000000000000000000 ) ) ;
#19455=ORIENTED_EDGE ( 'NONE', *, *, #81503, .T. ) ;
#19456=CARTESIAN_POINT ( 'NONE',  ( 107.9555263298577330, -25.64695713395843413, 265.0127681330543510 ) ) ;
#19457=CARTESIAN_POINT ( 'NONE',  ( 102.9047493514100893, -27.10917607469848178, 151.4013395616249511 ) ) ;
#19458=CYLINDRICAL_SURFACE ( 'NONE', #39401, 9.999999999999998224 ) ;
#19460=CARTESIAN_POINT ( 'NONE',  ( 117.4474071775726287, -37.68804338056689573, 74.75276813305397638 ) ) ;
#19461=DIRECTION ( 'NONE',  ( -0.000000000000000000, -0.000000000000000000, -1.000000000000000000 ) ) ;
#19462=ORIENTED_EDGE ( 'NONE', *, *, #57492, .F. ) ;
#19464=CARTESIAN_POINT ( 'NONE',  ( 116.8169405894235808, -34.15221262904118049, 160.0313671257249837 ) ) ;
#19465=ORIENTED_EDGE ( 'NONE', *, *, #28710, .F. ) ;
#19466=AXIS2_PLACEMENT_3D ( 'NONE', #13303, #61877, #48238 ) ;
#19468=VECTOR ( 'NONE', #12471, 1000.000000000000000 ) ;
#19469=AXIS2_PLACEMENT_3D ( 'NONE', #59265, #10671, #44290 ) ;
#19471=CARTESIAN_POINT ( 'NONE',  ( 118.0799254396265923, -36.12288750354066735, 273.8822919425776945 ) ) ;
#19473=AXIS2_PLACEMENT_3D ( 'NONE', #23085, #43479, #71224 ) ;
#19475=CARTESIAN_POINT ( 'NONE',  ( 116.8158949166094658, -34.14816870754088285, 94.03160469597915494 ) ) ;
#19476=CARTESIAN_POINT ( 'NONE',  ( 98.74870792914448714, -34.66384430100242753, 275.5552769709340737 ) ) ;
#19477=CARTESIAN_POINT ( 'NONE',  ( 116.3247715116346939, -32.94624160847306626, 99.13562527591096796 ) ) ;
#19478=CARTESIAN_POINT ( 'NONE',  ( 113.0643619202157453, -28.22920495858477352, 125.5870538473399591 ) ) ;
#19479=DIRECTION ( 'NONE',  ( 1.000000000000000000, 2.775557561562888827E-14, 0.000000000000000000 ) ) ;
#19480=CARTESIAN_POINT ( 'NONE',  ( 103.0327258024342427, -26.38818591439425632, 170.3603871806729444 ) ) ;
#19481=ORIENTED_EDGE ( 'NONE', *, *, #78573, .F. ) ;
#19484=PLANE ( 'NONE',  #78805 ) ;
#19486=CARTESIAN_POINT ( 'NONE',  ( 107.0664832912750057, -36.72944715993903486, 9.125625275910969947 ) ) ;
#19487=ORIENTED_EDGE ( 'NONE', *, *, #4153, .T. ) ;
#19488=CARTESIAN_POINT ( 'NONE',  ( 141.0664832912740110, -46.72944715994102438, 14.82207188531771358 ) ) ;
#19489=CARTESIAN_POINT ( 'NONE',  ( 116.9458863120112539, -40.19413502446316500, 133.5584824187679658 ) ) ;
#19490=ORIENTED_EDGE ( 'NONE', *, *, #7117, .T. ) ;
#19493=EDGE_CURVE ( 'NONE', #25402, #61470, #37595, .T. ) ;
#19494=CARTESIAN_POINT ( 'NONE',  ( 100.8874678769283264, -44.70022136931469703, 118.0522919418250893 ) ) ;
#19495=PLANE ( 'NONE',  #14782 ) ;
#19498=EDGE_CURVE ( 'NONE', #31238, #25043, #88081, .T. ) ;
#19500=ORIENTED_EDGE ( 'NONE', *, *, #80467, .T. ) ;
#19504=CARTESIAN_POINT ( 'NONE',  ( 101.9936208461673459, -45.44607148442891287, 157.1564586006232389 ) ) ;
#19505=CYLINDRICAL_SURFACE ( 'NONE', #71962, 9.999999999999998224 ) ;
#19509=CARTESIAN_POINT ( 'NONE',  ( 172.5667039024480118, -36.32844715993499563, 180.4678068554150059 ) ) ;
#19510=ORIENTED_EDGE ( 'NONE', *, *, #62831, .T. ) ;
#19511=EDGE_CURVE ( 'NONE', #23819, #29231, #52172, .T. ) ;
#19512=CARTESIAN_POINT ( 'NONE',  ( 188.5667039024479834, -62.87844715994099687, 137.2178068554150059 ) ) ;
#19514=CARTESIAN_POINT ( 'NONE',  ( 193.5667039024485803, -48.82844715993409324, 180.4678068554150343 ) ) ;
#19515=CARTESIAN_POINT ( 'NONE',  ( 114.4888877093245583, -29.48743791597858177, 190.4537205140059655 ) ) ;
#19516=DIRECTION ( 'NONE',  ( 0.000000000000000000, 0.000000000000000000, 1.000000000000000000 ) ) ;
#19518=CARTESIAN_POINT ( 'NONE',  ( 109.4837483930865289, -46.20680252518636166, 43.77562527591094721 ) ) ;
#19522=EDGE_LOOP ( 'NONE', ( #69663, #26815 ) ) ;
#19526=CARTESIAN_POINT ( 'NONE',  ( 99.39098736499681763, -43.25305561222647555, 223.3187261630399689 ) ) ;
#19532=CYLINDRICAL_SURFACE ( 'NONE', #21230, 9.999999999999998224 ) ;
#19533=AXIS2_PLACEMENT_3D ( 'NONE', #9328, #18814, #27410 ) ;
#19536=CIRCLE ( 'NONE', #41307, 2.117000000000000881 ) ;
#19539=CARTESIAN_POINT ( 'NONE',  ( 116.7701435943788653, -31.43623786049258584, 24.21181575210196257 ) ) ;
#19542=CARTESIAN_POINT ( 'NONE',  ( 110.6228153916969603, -44.07670705792993715, 245.7538046553059701 ) ) ;
#19544=CARTESIAN_POINT ( 'NONE',  ( 96.03815445040686427, -38.18343476501375022, 151.4299109901969871 ) ) ;
#19546=LINE ( 'NONE', #80905, #60653 ) ;
#19549=CARTESIAN_POINT ( 'NONE',  ( 116.9665165100108908, -41.74809644303882550, 244.4651490854349731 ) ) ;
#19551=VERTEX_POINT ( 'NONE', #73090 ) ;
#19552=CARTESIAN_POINT ( 'NONE',  ( 117.6393638915270827, -42.19070237429166070, 89.44705384733997278 ) ) ;
#19553=CARTESIAN_POINT ( 'NONE',  ( 172.5664832912740110, -32.07844715994070839, 74.17562527591199739 ) ) ;
#19556=ORIENTED_EDGE ( 'NONE', *, *, #81004, .F. ) ;
#19559=CARTESIAN_POINT ( 'NONE',  ( 115.0871287824145242, -30.61533435493911526, 159.3439420475139059 ) ) ;
#19560=CARTESIAN_POINT ( 'NONE',  ( 163.0664832912739826, -18.82844715994099971, 330.8831252759119934 ) ) ;
#19561=EDGE_CURVE ( 'NONE', #17346, #84744, #81118, .T. ) ;
#19563=LINE ( 'NONE', #40893, #76571 ) ;
#19564=CARTESIAN_POINT ( 'NONE',  ( 98.87701435734486211, -36.85308710711977653, 134.1566617981629577 ) ) ;
#19565=CARTESIAN_POINT ( 'NONE',  ( 111.8740745592753427, -46.04428811464656945, 268.9556252759110180 ) ) ;
#19567=VERTEX_POINT ( 'NONE', #73538 ) ;
#19573=CARTESIAN_POINT ( 'NONE',  ( 20.03715912545645850, -24.95799193693202156, 129.9678068554150627 ) ) ;
#19576=CARTESIAN_POINT ( 'NONE',  ( 136.8164832912740110, -36.72944715994100306, 3.101481641215515950 ) ) ;
#19577=AXIS2_PLACEMENT_3D ( 'NONE', #36143, #15710, #22980 ) ;
#19579=LINE ( 'NONE', #80146, #49565 ) ;
#19580=DIRECTION ( 'NONE',  ( 0.000000000000000000, -1.000000000000000000, 0.000000000000000000 ) ) ;
#19581=CARTESIAN_POINT ( 'NONE',  ( 108.1312808730283166, -45.72271566404705112, 162.1048007804579640 ) ) ;
#19582=CARTESIAN_POINT ( 'NONE',  ( 112.7657546104280044, -27.20415503536211688, 54.65943479971996055 ) ) ;
#19583=LINE ( 'NONE', #81831, #33527 ) ;
#19586=EDGE_LOOP ( 'NONE', ( #1771, #13482, #72548, #28674 ) ) ;
#19587=CARTESIAN_POINT ( 'NONE',  ( 97.06110197060442601, -37.99657418256868624, 262.4273502539846845 ) ) ;
#19588=ORIENTED_EDGE ( 'NONE', *, *, #88140, .F. ) ;
#19592=CARTESIAN_POINT ( 'NONE',  ( 110.9148046014321523, -45.95934737500046907, 132.8908183948595934 ) ) ;
#19593=LINE ( 'NONE', #33676, #232 ) ;
#19595=VERTEX_POINT ( 'NONE', #66723 ) ;
#19596=CARTESIAN_POINT ( 'NONE',  ( 100.0239399080498544, -28.99471651683304785, 285.6641967044823787 ) ) ;
#19598=CARTESIAN_POINT ( 'NONE',  ( 116.7853252867327996, -32.83880582269000570, 50.12991099019698282 ) ) ;
#19599=VECTOR ( 'NONE', #16632, 999.9999999999998863 ) ;
#19600=VECTOR ( 'NONE', #21015, 1000.000000000000000 ) ;
#19601=DIRECTION ( 'NONE',  ( 0.000000000000000000, -1.000000000000000000, 0.000000000000000000 ) ) ;
#19603=EDGE_CURVE ( 'NONE', #57294, #87995, #4507, .T. ) ;
#19604=CARTESIAN_POINT ( 'NONE',  ( 98.34986356287390663, -31.65657669940653207, 146.9069401482558419 ) ) ;
#19605=CARTESIAN_POINT ( 'NONE',  ( 49.16670390244701139, -26.71338133339240528, -5.074374724088000832 ) ) ;
#19606=VECTOR ( 'NONE', #80294, 1000.000000000000000 ) ;
#19608=DIRECTION ( 'NONE',  ( 0.9068632946707805287, -0.4214249218767880389, 9.068632946707802473E-16 ) ) ;
#19609=DIRECTION ( 'NONE',  ( -1.000000000000000000, -4.299999999999999979E-14, -1.000000000000000078E-15 ) ) ;
#19610=VERTEX_POINT ( 'NONE', #89878 ) ;
#19611=CARTESIAN_POINT ( 'NONE',  ( 100.9151287000745896, -46.91716693487881429, 52.14419670448194921 ) ) ;
#19612=CARTESIAN_POINT ( 'NONE',  ( 109.7757303681923418, -47.46933477669593771, 88.78514908543493789 ) ) ;
#19614=CARTESIAN_POINT ( 'NONE',  ( 34.96670390244699433, -26.71338133339301635, -5.074374724088000832 ) ) ;
#19616=AXIS2_PLACEMENT_3D ( 'NONE', #64214, #22887, #30133 ) ;
#19617=EDGE_CURVE ( 'NONE', #46374, #47812, #54989, .T. ) ;
#19620=ORIENTED_EDGE ( 'NONE', *, *, #24666, .F. ) ;
#19621=CARTESIAN_POINT ( 'NONE',  ( 115.9482186066388749, -32.63332544795709111, 100.1699109901959588 ) ) ;
#19623=ORIENTED_EDGE ( 'NONE', *, *, #58031, .F. ) ;
#19624=CARTESIAN_POINT ( 'NONE',  ( 98.91597900623165174, -29.29754952351882480, 226.7261014663869503 ) ) ;
#19625=CARTESIAN_POINT ( 'NONE',  ( 98.37992361594359636, -41.69440232629470700, 252.7399961474531835 ) ) ;
#19626=CARTESIAN_POINT ( 'NONE',  ( 116.9903668002740602, -35.35439823643719137, 148.9359728826448759 ) ) ;
#19628=CARTESIAN_POINT ( 'NONE',  ( 100.9546728272766956, -28.70702571534067005, 81.59395860767402553 ) ) ;
#19630=EDGE_CURVE ( 'NONE', #70136, #39283, #53493, .T. ) ;
#19631=CYLINDRICAL_SURFACE ( 'NONE', #17244, 9.999999999999998224 ) ;
#19633=CARTESIAN_POINT ( 'NONE',  ( 108.2029444874846007, -47.03713394308636708, 157.6518157521019532 ) ) ;
#19634=ORIENTED_EDGE ( 'NONE', *, *, #72155, .T. ) ;
#19636=AXIS2_PLACEMENT_3D ( 'NONE', #79593, #76559, #14793 ) ;
#19637=CARTESIAN_POINT ( 'NONE',  ( 99.14414808984345484, -41.78050036225572228, 138.1977737820869834 ) ) ;
#19639=CARTESIAN_POINT ( 'NONE',  ( 96.93540839703301515, -34.51582869190843894, 252.1432443235293590 ) ) ;
#19640=CARTESIAN_POINT ( 'NONE',  ( 180.1667039024474377, -26.71338133338667831, 237.4678068554150059 ) ) ;
#19641=AXIS2_PLACEMENT_3D ( 'NONE', #11343, #39040, #64814 ) ;
#19642=PLANE ( 'NONE',  #15959 ) ;
#19643=EDGE_CURVE ( 'NONE', #1830, #17950, #68801, .T. ) ;
#19644=DIRECTION ( 'NONE',  ( 0.000000000000000000, 0.000000000000000000, -1.000000000000000000 ) ) ;
#19647=DIRECTION ( 'NONE',  ( 1.000000000000000000, 4.163336342344333240E-14, 0.000000000000000000 ) ) ;
#19648=CARTESIAN_POINT ( 'NONE',  ( 109.6005296801413351, -26.60309369064632534, 199.8813395616249977 ) ) ;
#19650=ORIENTED_EDGE ( 'NONE', *, *, #70518, .T. ) ;
#19658=CARTESIAN_POINT ( 'NONE',  ( 143.0664832912740110, -18.82844715994099971, 93.42562527591199739 ) ) ;
#19659=EDGE_LOOP ( 'NONE', ( #47366, #44146, #56014, #57976, #87404 ) ) ;
#19660=AXIS2_PLACEMENT_3D ( 'NONE', #45518, #10577, #3769 ) ;
#19662=AXIS2_PLACEMENT_3D ( 'NONE', #67329, #25109, #88256 ) ;
#19664=CARTESIAN_POINT ( 'NONE',  ( 116.5268644012694637, -41.19342475044518181, 228.4756252759109714 ) ) ;
#19665=ORIENTED_EDGE ( 'NONE', *, *, #85297, .F. ) ;
#19666=VECTOR ( 'NONE', #58810, 1000.000000000000114 ) ;
#19668=LINE ( 'NONE', #27374, #69538 ) ;
#19671=LINE ( 'NONE', #25138, #3426 ) ;
#19673=CARTESIAN_POINT ( 'NONE',  ( 114.6306032519149198, -32.52409173292234357, 27.06047132197198124 ) ) ;
#19674=CARTESIAN_POINT ( 'NONE',  ( 108.9888594788934029, -47.63768604335348300, 118.7032443235299723 ) ) ;
#19675=VECTOR ( 'NONE', #5680, 1000.000000000000000 ) ;
#19676=CARTESIAN_POINT ( 'NONE',  ( 94.86917197795300183, -31.06128196069623471, 25.56312527591095574 ) ) ;
#19678=EDGE_CURVE ( 'NONE', #83074, #36562, #63040, .T. ) ;
#19679=VECTOR ( 'NONE', #7683, 1000.000000000000000 ) ;
#19680=CARTESIAN_POINT ( 'NONE',  ( 41.56648329127398966, -27.82844715994070484, 198.9256252759119832 ) ) ;
#19681=CARTESIAN_POINT ( 'NONE',  ( 101.7972116522101089, -45.32445798590094199, 67.13961389132575164 ) ) ;
#19682=VERTEX_POINT ( 'NONE', #54408 ) ;
#19683=EDGE_LOOP ( 'NONE', ( #27110, #64326, #44908, #45773 ) ) ;
#19684=LINE ( 'NONE', #41892, #11113 ) ;
#19685=ORIENTED_EDGE ( 'NONE', *, *, #83186, .T. ) ;
#19686=ORIENTED_EDGE ( 'NONE', *, *, #46876, .T. ) ;
#19688=AXIS2_PLACEMENT_3D ( 'NONE', #5550, #52743, #66405 ) ;
#19689=CARTESIAN_POINT ( 'NONE',  ( 102.8831062096190436, -29.28260300185988996, 59.90670554236199052 ) ) ;
#19690=CARTESIAN_POINT ( 'NONE',  ( 116.6260796636124155, -40.94376574832517690, 253.4956252759109532 ) ) ;
#19691=CARTESIAN_POINT ( 'NONE',  ( 114.2383551682310525, -44.26553795382362466, 158.1813395616249807 ) ) ;
#19692=CARTESIAN_POINT ( 'NONE',  ( 117.0881497372581634, -37.78494053717825096, 23.74254566645982933 ) ) ;
#19693=CARTESIAN_POINT ( 'NONE',  ( 116.1395517938576347, -31.55217135963209785, 285.2384824187680579 ) ) ;
#19695=CARTESIAN_POINT ( 'NONE',  ( 112.0634802680675222, -45.48975181846424931, 93.98957202063608918 ) ) ;
#19696=EDGE_LOOP ( 'NONE', ( #8160, #25756, #38094, #60392 ) ) ;
#19697=CARTESIAN_POINT ( 'NONE',  ( 83.56670390244801183, -36.72944715994108122, 218.0711402470150801 ) ) ;
#19698=CARTESIAN_POINT ( 'NONE',  ( 110.0016395821292292, -26.67999326470393839, 259.8499109901964630 ) ) ;
#19699=EDGE_LOOP ( 'NONE', ( #39221, #65552, #12962, #5741 ) ) ;
#19700=CARTESIAN_POINT ( 'NONE',  ( 114.8141470925876462, -29.70096138442027112, 209.4127681330539872 ) ) ;
#19703=FACE_OUTER_BOUND ( 'NONE', #22834, .T. ) ;
#19704=CARTESIAN_POINT ( 'NONE',  ( 116.8174769680534979, -34.15428111572317249, 25.03134733120764821 ) ) ;
#19705=DIRECTION ( 'NONE',  ( -0.7071067811865170416, -0.7071067811865778818, -7.071067811865162747E-16 ) ) ;
#19706=CARTESIAN_POINT ( 'NONE',  ( 113.4524916730000825, -42.42761561582053531, 277.6356252759110248 ) ) ;
#19708=DIRECTION ( 'NONE',  ( -0.7071067811865671127, -0.7071067811865279218, -7.071067811865664660E-16 ) ) ;
#19713=DIRECTION ( 'NONE',  ( 1.000000000000000000, 2.106816776397999944E-14, 9.351236661543306751E-17 ) ) ;
#19714=CARTESIAN_POINT ( 'NONE',  ( 101.0178098607260893, -29.23851721486679267, 195.5838068554161282 ) ) ;
#19715=ORIENTED_EDGE ( 'NONE', *, *, #72937, .F. ) ;
#19716=LINE ( 'NONE', #40607, #84386 ) ;
#19717=CARTESIAN_POINT ( 'NONE',  ( 96.66004714996478242, -35.80616453621266970, 231.2556252759109725 ) ) ;
#19718=CARTESIAN_POINT ( 'NONE',  ( 109.7700798034136511, -47.44693503648352362, 88.78514908543493789 ) ) ;
#19719=CARTESIAN_POINT ( 'NONE',  ( 118.1536727146126395, -36.20817079386891635, 264.8518157521014587 ) ) ;
#19720=CARTESIAN_POINT ( 'NONE',  ( 97.07207207514328218, -35.37844108510153518, 156.2189586001694579 ) ) ;
#19721=CARTESIAN_POINT ( 'NONE',  ( 182.0374245136142406, -23.42844715993458848, 193.9678068554150059 ) ) ;
#19723=CARTESIAN_POINT ( 'NONE',  ( 107.0664832912739399, -36.72944715994096754, 298.1356252759109680 ) ) ;
#19726=B_SPLINE_CURVE_WITH_KNOTS ( 'NONE', 3,
 ( #43092, #49004, #29489, #83125, #70836, #20884, #36305, #56732, #35389, #21791, #77199, #48552, #76293, #8607, #14064, #29045, #41748, #35843 ),
 .UNSPECIFIED., .F., .F.,
 ( 4, 2, 2, 2, 2, 2, 2, 2, 4 ),
 ( 0.000000000000000000, 0.06249999994414716376, 0.1249999998882943275, 0.1874999998324414774, 0.2499999997765886550, 0.3124999997207358327, 0.3749999996648829548, 0.4374999996090297993, 0.4999999995531766439 ),
 .UNSPECIFIED. ) ;
#19727=CARTESIAN_POINT ( 'NONE',  ( 131.5867845949916557, -19.92005462651755110, 2.747931806393766774 ) ) ;
#19728=AXIS2_PLACEMENT_3D ( 'NONE', #12958, #40645, #12506 ) ;
#19730=VECTOR ( 'NONE', #13725, 1000.000000000000000 ) ;
#19732=AXIS2_PLACEMENT_3D ( 'NONE', #89597, #26907, #13288 ) ;
#19733=ORIENTED_EDGE ( 'NONE', *, *, #71655, .F. ) ;
#19734=ADVANCED_FACE ( 'NONE', ( #14001 ), #822, .T. ) ;
#19736=CARTESIAN_POINT ( 'NONE',  ( 108.0580239150950774, -28.21657753114420331, 129.4067055423629711 ) ) ;
#19737=EDGE_CURVE ( 'NONE', #84886, #2655, #56205, .T. ) ;
#19740=CARTESIAN_POINT ( 'NONE',  ( 116.3191775144681515, -32.94222376661483764, 89.13562527591095375 ) ) ;
#19741=CARTESIAN_POINT ( 'NONE',  ( 108.9808406375926779, -47.59218431635552093, 118.7032443235299723 ) ) ;
#19743=FACE_OUTER_BOUND ( 'NONE', #66476, .T. ) ;
#19745=ADVANCED_FACE ( 'NONE', ( #47606 ), #68073, .F. ) ;
#19747=CARTESIAN_POINT ( 'NONE',  ( 112.0659116261392541, -45.48839625842523304, 108.9897919429150761 ) ) ;
#19748=AXIS2_PLACEMENT_3D ( 'NONE', #58335, #2495, #86062 ) ;
#19749=CARTESIAN_POINT ( 'NONE',  ( 116.4365193811697310, -32.28633913640743458, 64.19086337114998742 ) ) ;
#19751=VERTEX_POINT ( 'NONE', #68970 ) ;
#19752=EDGE_CURVE ( 'NONE', #18741, #28403, #49232, .T. ) ;
#19753=VERTEX_POINT ( 'NONE', #43028 ) ;
#19756=CARTESIAN_POINT ( 'NONE',  ( 112.9441315310008918, -44.54716313336194844, 139.0899109901959605 ) ) ;
#19757=DIRECTION ( 'NONE',  ( -4.237773401492740281E-14, 1.000000000000000000, 0.000000000000000000 ) ) ;
#19759=LINE ( 'NONE', #68358, #66838 ) ;
#19762=LINE ( 'NONE', #47440, #8341 ) ;
#19764=CARTESIAN_POINT ( 'NONE',  ( 112.0655926785064906, -45.48857413222889079, 178.9897630915276352 ) ) ;
#19765=CARTESIAN_POINT ( 'NONE',  ( 116.5135284680788175, -32.37261310794432490, 104.1699109901969535 ) ) ;
#19768=ADVANCED_FACE ( 'NONE', ( #50758 ), #2175, .T. ) ;
#19770=FACE_OUTER_BOUND ( 'NONE', #5476, .T. ) ;
#19771=CYLINDRICAL_SURFACE ( 'NONE', #86784, 2.117000000000000881 ) ;
#19772=CARTESIAN_POINT ( 'NONE',  ( 172.5664832912729878, -27.57844715994070484, 81.92562527591199739 ) ) ;
#19773=CARTESIAN_POINT ( 'NONE',  ( 98.92939184154955967, -35.79647825066581390, 204.0538046553059814 ) ) ;
#19774=CARTESIAN_POINT ( 'NONE',  ( 113.2464514564345706, -28.75940189997899310, 25.55195518195452564 ) ) ;
#19775=ORIENTED_EDGE ( 'NONE', *, *, #78663, .F. ) ;
#19776=VERTEX_POINT ( 'NONE', #30765 ) ;
#19779=CARTESIAN_POINT ( 'NONE',  ( 136.7495928495827400, -19.33856210725350167, 3.004220725469440634 ) ) ;
#19780=EDGE_LOOP ( 'NONE', ( #76760, #49996, #27041, #45898 ) ) ;
#19781=ORIENTED_EDGE ( 'NONE', *, *, #3499, .T. ) ;
#19782=CARTESIAN_POINT ( 'NONE',  ( 77.33333279747650124, -19.08363404521308482, 6.775960187534255219 ) ) ;
#19783=ADVANCED_FACE ( 'NONE', ( #77577 ), #29884, .F. ) ;
#19784=CARTESIAN_POINT ( 'NONE',  ( 108.0145050256332979, -45.54020952213421936, 199.0930118773259778 ) ) ;
#19786=VECTOR ( 'NONE', #87818, 1000.000000000000000 ) ;
#19790=ORIENTED_EDGE ( 'NONE', *, *, #32577, .T. ) ;
#19791=EDGE_LOOP ( 'NONE', ( #50703, #21020, #23262, #77874 ) ) ;
#19793=AXIS2_PLACEMENT_3D ( 'NONE', #4799, #32483, #60183 ) ;
#19794=PLANE ( 'NONE',  #14498 ) ;
#19797=ORIENTED_EDGE ( 'NONE', *, *, #18424, .F. ) ;
#19798=CARTESIAN_POINT ( 'NONE',  ( 110.0029149558365305, -28.58829895313488834, 247.6071379886389821 ) ) ;
#19799=CARTESIAN_POINT ( 'NONE',  ( 97.72652769937234041, -42.68433437468970482, 141.7661014663869707 ) ) ;
#19800=CARTESIAN_POINT ( 'NONE',  ( 96.97787942770413849, -32.27031107066116533, 55.98324432352897162 ) ) ;
#19801=CARTESIAN_POINT ( 'NONE',  ( 104.2046607136328191, -44.36613767402425879, 249.5838068554171230 ) ) ;
#19803=CARTESIAN_POINT ( 'NONE',  ( 33.78309357195659146, -29.99615139352317428, 117.4678068554150485 ) ) ;
#19804=CARTESIAN_POINT ( 'NONE',  ( 97.81138037892189629, -40.51667183916828918, 42.63556083456600732 ) ) ;
#19805=CARTESIAN_POINT ( 'NONE',  ( 117.2915085808104436, -34.52259632565112213, 179.9956252759109532 ) ) ;
#19807=VERTEX_POINT ( 'NONE', #8995 ) ;
#19809=ORIENTED_EDGE ( 'NONE', *, *, #63859, .F. ) ;
#19813=ORIENTED_EDGE ( 'NONE', *, *, #73659, .F. ) ;
#19814=CARTESIAN_POINT ( 'NONE',  ( 150.5667039024473297, -25.42844715993594562, 300.4678068554149490 ) ) ;
#19815=CARTESIAN_POINT ( 'NONE',  ( 102.0652380361773339, -27.97156370417384608, 91.48995787984884487 ) ) ;
#19816=CARTESIAN_POINT ( 'NONE',  ( 113.4154522487949919, -27.68126056648907252, 84.57753003781698453 ) ) ;
#19819=FACE_OUTER_BOUND ( 'NONE', #80935, .T. ) ;
#19820=CARTESIAN_POINT ( 'NONE',  ( 115.7831076679527058, -41.80230951405372508, 144.4064586089073714 ) ) ;
#19822=CARTESIAN_POINT ( 'NONE',  ( 117.1710321396410421, -41.15233254730026147, 204.4861014663869696 ) ) ;
#19825=ORIENTED_EDGE ( 'NONE', *, *, #52535, .T. ) ;
#19827=CARTESIAN_POINT ( 'NONE',  ( 37.56670390244828184, -48.82844715994119866, 300.4678068554150059 ) ) ;
#19828=CARTESIAN_POINT ( 'NONE',  ( 97.81171235735017433, -40.51746255502365557, 257.6350867217079212 ) ) ;
#19830=CARTESIAN_POINT ( 'NONE',  ( 110.0016395821292292, -26.67999326470393839, 259.8499109901964630 ) ) ;
#19832=CARTESIAN_POINT ( 'NONE',  ( 112.5227400616102500, -28.31493319190477109, 194.6183074944887039 ) ) ;
#19833=CARTESIAN_POINT ( 'NONE',  ( 115.7133342524696360, -42.59197454220085177, 269.3527681330536439 ) ) ;
#19834=CARTESIAN_POINT ( 'NONE',  ( 114.2698949211017663, -45.17901133753223064, 149.1508633711489722 ) ) ;
#19835=CARTESIAN_POINT ( 'NONE',  ( 107.0664832912739399, -36.72944715994095333, 293.9356252759109793 ) ) ;
#19836=CARTESIAN_POINT ( 'NONE',  ( 99.09577730710090293, -30.55033931252097545, 101.8022151059804656 ) ) ;
#19837=EDGE_CURVE ( 'NONE', #1672, #58534, #41971, .T. ) ;
#19839=DIRECTION ( 'NONE',  ( 4.012088370409549976E-14, -1.000000000000000000, 0.000000000000000000 ) ) ;
#19843=ADVANCED_FACE ( 'NONE', ( #85311, #43928 ), #15363, .T. ) ;
#19846=ORIENTED_EDGE ( 'NONE', *, *, #30209, .F. ) ;
#19848=EDGE_LOOP ( 'NONE', ( #1244, #80048, #472, #59054 ) ) ;
#19850=CARTESIAN_POINT ( 'NONE',  ( 116.3681181406586518, -31.99193570193499525, 40.20133956162496958 ) ) ;
#19852=LINE ( 'NONE', #13049, #23898 ) ;
#19853=ADVANCED_FACE ( 'NONE', ( #65288 ), #78930, .F. ) ;
#19854=DIRECTION ( 'NONE',  ( 0.000000000000000000, 1.000000000000000000, 0.000000000000000000 ) ) ;
#19855=VECTOR ( 'NONE', #28957, 1000.000000000000000 ) ;
#19856=CARTESIAN_POINT ( 'NONE',  ( 116.0662231142348162, -35.72080775710429634, 233.3257531614099776 ) ) ;
#19859=VERTEX_POINT ( 'NONE', #1277 ) ;
#19860=ADVANCED_FACE ( 'NONE', ( #44377 ), #43458, .F. ) ;
#19861=AXIS2_PLACEMENT_3D ( 'NONE', #50657, #78398, #14819 ) ;
#19862=AXIS2_PLACEMENT_3D ( 'NONE', #2804, #72730, #10499 ) ;
#19864=VECTOR ( 'NONE', #36306, 1000.000000000000000 ) ;
#19865=B_SPLINE_CURVE_WITH_KNOTS ( 'NONE', 3,
 ( #72572, #79396, #10766, #9896, #32108, #85771, #59802, #3083, #32549, #73900, #24859, #11684, #23541, #51204, #52965, #46169, #37604, #45282, #44391, #78947, #58910, #73445, #24420, #39377, #38043, #3514, #72122, #73001, #80289 ),
 .UNSPECIFIED., .F., .F.,
 ( 4, 2, 2, 2, 2, 2, 2, 2, 2, 2, 1, 1, 1, 1, 1, 2, 4 ),
 ( 0.000000000000000000, 0.06250189640743901431, 0.1250037928148780286, 0.1875056892223170568, 0.2500075856297560573, 0.3125094820371950854, 0.3750113784446341136, 0.4375132748520730863, 0.4687642230557926837, 0.4843896971576525656, 0.4922024342085823956, 0.4961088027340472273, 0.4980619869967797819, 0.4990385791281458094, 0.4995268751938287122, 0.4997710232266699970, 0.5000151712595112263 ),
 .UNSPECIFIED. ) ;
#19866=CARTESIAN_POINT ( 'NONE',  ( 100.8875041660994043, -44.70025221268588211, 102.0524332644927057 ) ) ;
#19867=CARTESIAN_POINT ( 'NONE',  ( 20.03715912545735023, -46.82818131006202123, 180.4678068554150911 ) ) ;
#19868=CARTESIAN_POINT ( 'NONE',  ( 100.9529263511984141, -28.70839242354088583, 275.5937037153142910 ) ) ;
#19871=CARTESIAN_POINT ( 'NONE',  ( 107.0664832912739257, -50.22944715994096043, 311.6356252759109680 ) ) ;
#19872=CARTESIAN_POINT ( 'NONE',  ( 96.93540839703290146, -34.51582869190840341, 256.1432443235307232 ) ) ;
#19874=EDGE_CURVE ( 'NONE', #34264, #65898, #23227, .T. ) ;
#19875=EDGE_LOOP ( 'NONE', ( #86948, #58834, #44181, #2147 ) ) ;
#19878=VECTOR ( 'NONE', #41791, 1000.000000000000000 ) ;
#19879=FACE_OUTER_BOUND ( 'NONE', #2657, .T. ) ;
#19880=CARTESIAN_POINT ( 'NONE',  ( 100.2308834438963174, -41.19087078291441628, 99.60523322673398638 ) ) ;
#19881=CIRCLE ( 'NONE', #27078, 1.571100913904333041 ) ;
#19882=CARTESIAN_POINT ( 'NONE',  ( 115.8243402359382657, -31.72812547371020031, 129.2399646760175074 ) ) ;
#19883=LINE ( 'NONE', #4462, #76616 ) ;
#19884=DIRECTION ( 'NONE',  ( -1.000000000000000078E-15, 1.000000000000000083E-30, 1.000000000000000000 ) ) ;
#19886=CARTESIAN_POINT ( 'NONE',  ( 107.0664832912739541, -23.22944715994095688, 315.1356252759112522 ) ) ;
#19888=CARTESIAN_POINT ( 'NONE',  ( 113.6146262985763258, -28.61718150614917633, 164.5356252759109736 ) ) ;
#19891=CARTESIAN_POINT ( 'NONE',  ( 112.3776303481765950, -29.59825886299321951, 100.9987261630399757 ) ) ;
#19893=EDGE_CURVE ( 'NONE', #22477, #47420, #50298, .T. ) ;
#19895=CARTESIAN_POINT ( 'NONE',  ( 98.70509129169590778, -42.99238438483101987, 62.83848241876793850 ) ) ;
#19897=CARTESIAN_POINT ( 'NONE',  ( 112.0657206150906120, -45.48850286296052303, 257.9896703071129878 ) ) ;
#19898=EDGE_LOOP ( 'NONE', ( #77055, #38976, #70055, #88686, #2996 ) ) ;
#19901=B_SPLINE_CURVE_WITH_KNOTS ( 'NONE', 3,
 ( #88082, #31304, #81279, #19025, #89879, #48054, #75789, #75341, #34886, #55750, #33985, #76228, #372, #42140, #40359, #55311, #19475, #14002 ),
 .UNSPECIFIED., .F., .F.,
 ( 4, 2, 2, 2, 2, 2, 2, 2, 4 ),
 ( 0.4999390785766987810, 0.5624466937546114265, 0.6249543089325240164, 0.6874619241104367173, 0.7499695392883494183, 0.8124771544662620082, 0.8749847696441745981, 0.9374923848220872991, 1.000000000000000000 ),
 .UNSPECIFIED. ) ;
#19902=EDGE_LOOP ( 'NONE', ( #47170, #20652 ) ) ;
#19905=CARTESIAN_POINT ( 'NONE',  ( 104.1325824198641499, -27.39908484284267587, 250.3184824187684683 ) ) ;
#19906=CARTESIAN_POINT ( 'NONE',  ( 95.65143945485090171, -33.45545561978638460, 137.1041967044819501 ) ) ;
#19907=CARTESIAN_POINT ( 'NONE',  ( 123.6837132603321692, -20.11243780205712639, 249.5838068554165261 ) ) ;
#19908=CARTESIAN_POINT ( 'NONE',  ( 97.33784131423797703, -34.07106451867782226, 142.1147919416630430 ) ) ;
#19909=CARTESIAN_POINT ( 'NONE',  ( 113.3423928682155406, -27.63071431045342763, 85.60800622829195561 ) ) ;
#19910=DIRECTION ( 'NONE',  ( -0.7071067811865753283, 0.7071067811865197061, -7.071067811865760309E-16 ) ) ;
#19911=VERTEX_POINT ( 'NONE', #71223 ) ;
#19913=EDGE_CURVE ( 'NONE', #24486, #35637, #10094, .T. ) ;
#19915=AXIS2_PLACEMENT_3D ( 'NONE', #66773, #47211, #4560 ) ;
#19916=CARTESIAN_POINT ( 'NONE',  ( 113.1786488514148061, -44.75160319904480843, 159.0938251498227771 ) ) ;
#19917=ORIENTED_EDGE ( 'NONE', *, *, #81304, .F. ) ;
#19918=EDGE_CURVE ( 'NONE', #63276, #74286, #66614, .T. ) ;
#19919=CIRCLE ( 'NONE', #47456, 2.750000000000002665 ) ;
#19921=CIRCLE ( 'NONE', #44540, 4.750000000000004441 ) ;
#19923=CARTESIAN_POINT ( 'NONE',  ( 111.7292870705843768, -27.42961193919077445, 279.7070538473396937 ) ) ;
#19924=DIRECTION ( 'NONE',  ( 0.000000000000000000, 0.000000000000000000, 1.000000000000000000 ) ) ;
#19926=DIRECTION ( 'NONE',  ( 0.000000000000000000, -1.000000000000000000, 0.000000000000000000 ) ) ;
#19928=CARTESIAN_POINT ( 'NONE',  ( 116.8666057829012033, -37.25052826422871277, 18.78419670448294809 ) ) ;
#19929=CARTESIAN_POINT ( 'NONE',  ( 97.11097791331823714, -37.83202729851629442, 101.4149069316836602 ) ) ;
#19930=CARTESIAN_POINT ( 'NONE',  ( 103.1828028919049984, -27.07824557232550688, 126.3813395616259783 ) ) ;
#19932=CARTESIAN_POINT ( 'NONE',  ( 96.60586043895887087, -37.15609470439714102, 161.3584824187679487 ) ) ;
#19936=DIRECTION ( 'NONE',  ( 0.000000000000000000, -1.000000000000000000, 0.000000000000000000 ) ) ;
#19939=EDGE_LOOP ( 'NONE', ( #9731, #401, #30128, #14218 ) ) ;
#19941=CARTESIAN_POINT ( 'NONE',  ( 115.8271982374479592, -31.73307718988874271, 60.23988603985338841 ) ) ;
#19942=CARTESIAN_POINT ( 'NONE',  ( 117.3534821530742107, -34.78408995979881269, 158.9756252759109714 ) ) ;
#19944=DIRECTION ( 'NONE',  ( -4.237773401492740281E-14, 1.000000000000000000, 0.000000000000000000 ) ) ;
#19945=AXIS2_PLACEMENT_3D ( 'NONE', #29267, #23365, #36075 ) ;
#19946=DIRECTION ( 'NONE',  ( 0.9068632946707805287, -0.4214249218767882055, 9.081056412856297650E-16 ) ) ;
#19956=ORIENTED_EDGE ( 'NONE', *, *, #38532, .F. ) ;
#19957=EDGE_CURVE ( 'NONE', #88399, #5757, #60685, .T. ) ;
#19961=CARTESIAN_POINT ( 'NONE',  ( 108.3334480150830501, -46.73485936483547931, 157.6772919362252310 ) ) ;
#19962=CARTESIAN_POINT ( 'NONE',  ( 63.56670390244739366, -47.82844715994014706, 180.4678068554151196 ) ) ;
#19963=EDGE_CURVE ( 'NONE', #18192, #64715, #44827, .T. ) ;
#19965=DIRECTION ( 'NONE',  ( -0.9254794337955620787, -0.3787978585227822492, 0.000000000000000000 ) ) ;
#19966=CARTESIAN_POINT ( 'NONE',  ( 98.34971108053937883, -31.65683447307292298, 180.9064812817925372 ) ) ;
#19967=AXIS2_PLACEMENT_3D ( 'NONE', #63463, #48022, #7168 ) ;
#19968=VERTEX_POINT ( 'NONE', #52508 ) ;
#19969=CIRCLE ( 'NONE', #11197, 2.029999999999997140 ) ;
#19970=ORIENTED_EDGE ( 'NONE', *, *, #76468, .T. ) ;
#19971=DIRECTION ( 'NONE',  ( 4.299999999999999979E-14, -1.000000000000000000, 0.000000000000000000 ) ) ;
#19972=CARTESIAN_POINT ( 'NONE',  ( 97.44287158780967673, -40.59272077381804422, 247.6422919425769749 ) ) ;
#19976=CARTESIAN_POINT ( 'NONE',  ( 113.0229309284916184, -28.24065945027253477, 80.57753003781498080 ) ) ;
#19977=CARTESIAN_POINT ( 'NONE',  ( 116.7486982854288726, -34.15480232083102408, 54.03335171816377169 ) ) ;
#19979=CARTESIAN_POINT ( 'NONE',  ( 100.9539600449370766, -28.70758302638736836, 21.59398670790487884 ) ) ;
#19980=ORIENTED_EDGE ( 'NONE', *, *, #78936, .T. ) ;
#19981=DIRECTION ( 'NONE',  ( -4.299999999999999979E-14, 1.000000000000000000, -4.400000000000000367E-29 ) ) ;
#19985=CARTESIAN_POINT ( 'NONE',  ( 100.0731593717985106, -30.45489967868845227, 232.1882499725639661 ) ) ;
#19986=VECTOR ( 'NONE', #48517, 1000.000000000000000 ) ;
#19987=CARTESIAN_POINT ( 'NONE',  ( 97.81452210549078075, -40.51628237377364883, 52.63520911028864901 ) ) ;
#19988=CIRCLE ( 'NONE', #12730, 2.117000000000000881 ) ;
#19990=CARTESIAN_POINT ( 'NONE',  ( 112.0659115654917599, -45.48839629398710827, 153.9897919373767081 ) ) ;
#19991=CARTESIAN_POINT ( 'NONE',  ( 81.48476992305924682, -39.08750326150863685, 1.944748881527252893 ) ) ;
#19992=VERTEX_POINT ( 'NONE', #67507 ) ;
#19994=VECTOR ( 'NONE', #14871, 1000.000000000000000 ) ;
#19997=CARTESIAN_POINT ( 'NONE',  ( 96.33825113647944249, -41.76388066030261115, 61.67562527591097421 ) ) ;
#19998=VERTEX_POINT ( 'NONE', #52946 ) ;
#19999=CARTESIAN_POINT ( 'NONE',  ( 114.5355946289170390, -40.02218186577253789, 251.3138046553057734 ) ) ;
#20000=VECTOR ( 'NONE', #74658, 999.9999999999998863 ) ;
#20001=CARTESIAN_POINT ( 'NONE',  ( 62.03715912545755629, -47.82818131006020934, 117.4678068554150485 ) ) ;
#20002=CARTESIAN_POINT ( 'NONE',  ( 98.54774150848822956, -41.53511815344526070, 136.7356252759109623 ) ) ;
#20003=LINE ( 'NONE', #18203, #41878 ) ;
#20004=CARTESIAN_POINT ( 'NONE',  ( 41.56648329127398966, -27.82844715994070484, 198.9256252759119832 ) ) ;
#20008=EDGE_CURVE ( 'NONE', #42564, #48576, #39361, .T. ) ;
#20009=DIRECTION ( 'NONE',  ( 0.000000000000000000, -1.000000000000000000, 0.000000000000000000 ) ) ;
#20010=CARTESIAN_POINT ( 'NONE',  ( 103.9262362324350590, -26.74286475366834281, 246.3184824187679567 ) ) ;
#20012=CIRCLE ( 'NONE', #82394, 5.500000000000000888 ) ;
#20014=CARTESIAN_POINT ( 'NONE',  ( 103.8278507311454177, -46.72190801433284690, 78.32705384733995402 ) ) ;
#20015=DIRECTION ( 'NONE',  ( 1.907762142705490052E-15, 7.167082501179359715E-16, -1.000000000000000000 ) ) ;
#20017=ORIENTED_EDGE ( 'NONE', *, *, #52036, .F. ) ;
#20020=DIRECTION ( 'NONE',  ( 0.000000000000000000, 0.000000000000000000, -1.000000000000000000 ) ) ;
#20021=FACE_OUTER_BOUND ( 'NONE', #63811, .T. ) ;
#20024=CARTESIAN_POINT ( 'NONE',  ( 114.8977050226898484, -39.03198754188770891, 181.4166617981629486 ) ) ;
#20025=CARTESIAN_POINT ( 'NONE',  ( 118.1305967499472160, -36.20925573564677791, 264.8518157521014587 ) ) ;
#20026=CARTESIAN_POINT ( 'NONE',  ( 48.79742451362098166, -36.32844715994040996, 313.9678068554150059 ) ) ;
#20030=CARTESIAN_POINT ( 'NONE',  ( 21.03689327557705369, -23.42844715994186089, 313.9678068554150059 ) ) ;
#20032=VECTOR ( 'NONE', #13365, 1000.000000000000000 ) ;
#20033=ORIENTED_EDGE ( 'NONE', *, *, #63740, .F. ) ;
#20034=EDGE_CURVE ( 'NONE', #35135, #23413, #38026, .T. ) ;
#20035=DIRECTION ( 'NONE',  ( -1.000000000000000078E-15, 1.000000000000000083E-30, 1.000000000000000000 ) ) ;
#20037=ORIENTED_EDGE ( 'NONE', *, *, #24983, .F. ) ;
#20040=CARTESIAN_POINT ( 'NONE',  ( 90.44969454456416713, -52.08770651782494809, 218.8274735512160589 ) ) ;
#20042=CARTESIAN_POINT ( 'NONE',  ( 104.1791519563360993, -28.66003454886012136, 189.7724198280769770 ) ) ;
#20043=CARTESIAN_POINT ( 'NONE',  ( 110.3680388590993573, -25.29578946207851331, 64.85276813305395649 ) ) ;
#20048=CARTESIAN_POINT ( 'NONE',  ( 105.7984081882107006, -26.72418595413192577, 261.1773184477624454 ) ) ;
#20049=VERTEX_POINT ( 'NONE', #31648 ) ;
#20053=DIRECTION ( 'NONE',  ( 1.000000000000000000, -5.337610695313248426E-16, 0.000000000000000000 ) ) ;
#20054=VECTOR ( 'NONE', #52981, 1000.000000000000000 ) ;
#20055=DIRECTION ( 'NONE',  ( -0.7071067811865165975, -0.7071067811865784369, -7.071067811865158803E-16 ) ) ;
#20057=AXIS2_PLACEMENT_3D ( 'NONE', #60817, #46276, #88105 ) ;
#20058=CARTESIAN_POINT ( 'NONE',  ( 106.6058666599951152, -25.66223100340348040, 40.09753003781596448 ) ) ;
#20061=CARTESIAN_POINT ( 'NONE',  ( 107.0664832912739399, -36.72944715994095333, 302.6356252759109680 ) ) ;
#20064=EDGE_CURVE ( 'NONE', #7066, #57830, #20285, .T. ) ;
#20066=EDGE_CURVE ( 'NONE', #76506, #16372, #50731, .T. ) ;
#20067=DIRECTION ( 'NONE',  ( 0.000000000000000000, 1.000000000000000000, 0.000000000000000000 ) ) ;
#20068=ADVANCED_FACE ( 'NONE', ( #18918 ), #53405, .F. ) ;
#20069=CIRCLE ( 'NONE', #50524, 2.124999999999998224 ) ;
#20071=CARTESIAN_POINT ( 'NONE',  ( 25.56670390244797275, -65.37844715994100397, 257.2178068554150059 ) ) ;
#20072=ORIENTED_EDGE ( 'NONE', *, *, #18424, .T. ) ;
#20073=CARTESIAN_POINT ( 'NONE',  ( 116.6948211927369812, -32.58525784656897883, 75.14991099019697174 ) ) ;
#20075=VECTOR ( 'NONE', #56270, 1000.000000000000000 ) ;
#20078=FACE_OUTER_BOUND ( 'NONE', #30967, .T. ) ;
#20081=ORIENTED_EDGE ( 'NONE', *, *, #18529, .F. ) ;
#20082=CARTESIAN_POINT ( 'NONE',  ( 103.2241971045484519, -45.72390501747104707, 88.25562527591095829 ) ) ;
#20083=EDGE_CURVE ( 'NONE', #66137, #71741, #45700, .T. ) ;
#20084=CIRCLE ( 'NONE', #57744, 3.000000000000002665 ) ;
#20086=VERTEX_POINT ( 'NONE', #51637 ) ;
#20087=CARTESIAN_POINT ( 'NONE',  ( 105.0259480979001552, -25.88970440745778134, 276.2365776568634033 ) ) ;
#20088=DIRECTION ( 'NONE',  ( 0.000000000000000000, 0.000000000000000000, -1.000000000000000000 ) ) ;
#20089=DIRECTION ( 'NONE',  ( 1.000000000000000078E-15, -1.000000000000000083E-30, -1.000000000000000000 ) ) ;
#20090=EDGE_CURVE ( 'NONE', #29287, #6713, #15943, .T. ) ;
#20091=FACE_OUTER_BOUND ( 'NONE', #427, .T. ) ;
#20094=CARTESIAN_POINT ( 'NONE',  ( 177.0371591254545933, -48.62818131005479927, 129.9678068554150059 ) ) ;
#20095=CARTESIAN_POINT ( 'NONE',  ( 99.76930146980365066, -30.21680002102808515, 190.7470538473399415 ) ) ;
#20096=AXIS2_PLACEMENT_3D ( 'NONE', #83580, #63119, #7273 ) ;
#20097=VERTEX_POINT ( 'NONE', #72984 ) ;
#20099=CARTESIAN_POINT ( 'NONE',  ( 112.8895349442155265, -29.35594087158844445, 120.9882499725639633 ) ) ;
#20100=DIRECTION ( 'NONE',  ( -4.012088370409549976E-14, 1.000000000000000000, 0.000000000000000000 ) ) ;
#20101=CARTESIAN_POINT ( 'NONE',  ( 100.6696166679599713, -29.33055989933774299, 256.6441967044817147 ) ) ;
#20102=CARTESIAN_POINT ( 'NONE',  ( 182.0374245136174522, -23.42844715993458848, 117.4678068554150627 ) ) ;
#20103=FACE_OUTER_BOUND ( 'NONE', #5516, .T. ) ;
#20104=CYLINDRICAL_SURFACE ( 'NONE', #56225, 9.999999999999998224 ) ;
#20106=CARTESIAN_POINT ( 'NONE',  ( 97.31584371825169910, -39.30597600789160140, 107.5314586099498229 ) ) ;
#20107=DIRECTION ( 'NONE',  ( 0.000000000000000000, 0.000000000000000000, 1.000000000000000000 ) ) ;
#20108=CARTESIAN_POINT ( 'NONE',  ( 96.06973772670281164, -35.87188691900273341, 191.2765776568629690 ) ) ;
#20109=FACE_BOUND ( 'NONE', #18625, .T. ) ;
#20111=VERTEX_POINT ( 'NONE', #59348 ) ;
#20114=CARTESIAN_POINT ( 'NONE',  ( 77.52387074034942316, -17.68172011937453192, 2.822018711114674172 ) ) ;
#20115=CARTESIAN_POINT ( 'NONE',  ( 117.0612157011691750, -38.07822042050563027, 124.7180529556605109 ) ) ;
#20117=EDGE_CURVE ( 'NONE', #86172, #49620, #11590, .T. ) ;
#20118=AXIS2_PLACEMENT_3D ( 'NONE', #10907, #79979, #52656 ) ;
#20121=ORIENTED_EDGE ( 'NONE', *, *, #46752, .F. ) ;
#20124=CARTESIAN_POINT ( 'NONE',  ( 98.89873792621239090, -29.28182854020744230, 230.7261014663869503 ) ) ;
#20126=AXIS2_PLACEMENT_3D ( 'NONE', #21343, #28594, #36318 ) ;
#20128=CARTESIAN_POINT ( 'NONE',  ( 177.8371591254542921, -47.82818131005477369, 313.9678068554149490 ) ) ;
#20129=CARTESIAN_POINT ( 'NONE',  ( 110.8799455303576593, -45.97378286453075447, 167.8878162705527188 ) ) ;
#20130=CARTESIAN_POINT ( 'NONE',  ( 99.15069935661746570, -33.23069170325895527, 53.80142370292495713 ) ) ;
#20132=CARTESIAN_POINT ( 'NONE',  ( 97.36185206511996171, -42.06848625969246314, 172.7146728949589942 ) ) ;
#20134=ORIENTED_EDGE ( 'NONE', *, *, #69676, .F. ) ;
#20135=AXIS2_PLACEMENT_3D ( 'NONE', #55215, #33898, #48396 ) ;
#20136=DIRECTION ( 'NONE',  ( -0.000000000000000000, -0.000000000000000000, -1.000000000000000000 ) ) ;
#20137=CARTESIAN_POINT ( 'NONE',  ( 97.87203513630441876, -40.66183252246401025, 66.64857268046317529 ) ) ;
#20138=ORIENTED_EDGE ( 'NONE', *, *, #16541, .F. ) ;
#20139=ORIENTED_EDGE ( 'NONE', *, *, #11129, .F. ) ;
#20141=CARTESIAN_POINT ( 'NONE',  ( 107.0664832912739968, -18.82844715994099971, 168.9256252759119832 ) ) ;
#20142=ORIENTED_EDGE ( 'NONE', *, *, #36386, .T. ) ;
#20143=VERTEX_POINT ( 'NONE', #76577 ) ;
#20144=FACE_OUTER_BOUND ( 'NONE', #64502, .T. ) ;
#20145=CIRCLE ( 'NONE', #28840, 5.599999999999994316 ) ;
#20146=CARTESIAN_POINT ( 'NONE',  ( 109.8440526342893975, -45.34906309516006928, 57.25908649474392575 ) ) ;
#20147=CARTESIAN_POINT ( 'NONE',  ( 116.5468340722667051, -41.20284764396129873, 228.4756252759109714 ) ) ;
#20148=CARTESIAN_POINT ( 'NONE',  ( 118.7655994573051714, -38.45539276985795851, 223.7099109901969598 ) ) ;
#20150=CARTESIAN_POINT ( 'NONE',  ( 109.6066175024219831, -25.17973177368044801, 25.90419670448196143 ) ) ;
#20152=CARTESIAN_POINT ( 'NONE',  ( 97.81169266289590780, -40.51741659614882707, 92.63571255866972365 ) ) ;
#20153=EDGE_CURVE ( 'NONE', #81352, #88467, #41580, .T. ) ;
#20154=ORIENTED_EDGE ( 'NONE', *, *, #76976, .F. ) ;
#20157=CARTESIAN_POINT ( 'NONE',  ( 112.4472966703649348, -46.45872411559678028, 102.9784824187679817 ) ) ;
#20158=CARTESIAN_POINT ( 'NONE',  ( 98.61163144626758026, -43.92169047526947168, 76.89943479971999807 ) ) ;
#20159=CARTESIAN_POINT ( 'NONE',  ( 96.20350199017366322, -34.44722874799195722, 261.1737205140063338 ) ) ;
#20161=CARTESIAN_POINT ( 'NONE',  ( 100.7500417190893245, -45.80037066963202363, 237.0803871806729717 ) ) ;
#20162=CARTESIAN_POINT ( 'NONE',  ( 105.7995184340200581, -26.72403497198984113, 35.17729194683857941 ) ) ;
#20163=CARTESIAN_POINT ( 'NONE',  ( 75.25757238336811383, -1.944390235229870978, 394.9756252759101471 ) ) ;
#20164=EDGE_CURVE ( 'NONE', #21258, #6226, #63788, .T. ) ;
#20165=DIRECTION ( 'NONE',  ( 0.9963424814100680926, -0.08544974978095698503, 0.000000000000000000 ) ) ;
#20166=CARTESIAN_POINT ( 'NONE',  ( 51.34673845256460112, -29.62846900982267329, 193.9678068554150911 ) ) ;
#20167=CARTESIAN_POINT ( 'NONE',  ( 114.3906737664497371, -40.90796621566182267, 277.6356252759109111 ) ) ;
#20169=CARTESIAN_POINT ( 'NONE',  ( 98.15085007322062438, -41.26136264609154125, 172.7007008575214400 ) ) ;
#20170=DIRECTION ( 'NONE',  ( 0.0001713722456127401463, -0.9999999853157766072, -1.713722456137401502E-19 ) ) ;
#20172=CARTESIAN_POINT ( 'NONE',  ( 87.06648329127403940, -46.72944715994105280, -5.074374724089050659 ) ) ;
#20173=DIRECTION ( 'NONE',  ( 0.000000000000000000, -1.000000000000000000, 0.000000000000000000 ) ) ;
#20175=FACE_OUTER_BOUND ( 'NONE', #49723, .T. ) ;
#20176=LINE ( 'NONE', #56460, #50083 ) ;
#20179=CARTESIAN_POINT ( 'NONE',  ( 78.13314995793999174, 12.92155284005730387, 355.9756252759109998 ) ) ;
#20180=CARTESIAN_POINT ( 'NONE',  ( 115.5353962700893788, -29.58991257470437120, 224.3718157521009573 ) ) ;
#20181=CARTESIAN_POINT ( 'NONE',  ( 112.1200623320449097, -47.44840020502576294, 133.9270538473399768 ) ) ;
#20182=CARTESIAN_POINT ( 'NONE',  ( 116.5760347145385367, -42.45360038892302157, 274.3832443235299365 ) ) ;
#20183=CARTESIAN_POINT ( 'NONE',  ( 115.0889047303822110, -30.61763668965400598, 154.3439586083368624 ) ) ;
#20184=DIRECTION ( 'NONE',  ( 0.7071067811865165975, 0.7071067811865784369, 7.071067811865158803E-16 ) ) ;
#20185=DIRECTION ( 'NONE',  ( 0.000000000000000000, 0.000000000000000000, 1.000000000000000000 ) ) ;
#20186=CARTESIAN_POINT ( 'NONE',  ( 89.06648138392549185, -56.72944715994095333, -4.970821333495735850 ) ) ;
#20187=CARTESIAN_POINT ( 'NONE',  ( 107.0664832912739968, -36.72944715994100306, 292.6356252759106837 ) ) ;
#20190=VECTOR ( 'NONE', #27046, 1000.000000000000000 ) ;
#20191=ORIENTED_EDGE ( 'NONE', *, *, #31926, .F. ) ;
#20192=VERTEX_POINT ( 'NONE', #13898 ) ;
#20193=CARTESIAN_POINT ( 'NONE',  ( 99.50386058399449496, -32.75919911893461034, 135.3638483995049739 ) ) ;
#20194=EDGE_CURVE ( 'NONE', #4612, #68436, #76118, .T. ) ;
#20197=ORIENTED_EDGE ( 'NONE', *, *, #73394, .F. ) ;
#20199=CARTESIAN_POINT ( 'NONE',  ( 104.5678333644584228, -48.28820816006142991, 178.4070538473399665 ) ) ;
#20200=CARTESIAN_POINT ( 'NONE',  ( 70.14948329127297200, -71.52944715994141234, 361.9756252759109998 ) ) ;
#20201=EDGE_CURVE ( 'NONE', #40235, #24929, #83394, .T. ) ;
#20205=CARTESIAN_POINT ( 'NONE',  ( 45.77381068350418758, -48.62134037888111493, 180.4678068554150911 ) ) ;
#20207=CARTESIAN_POINT ( 'NONE',  ( 113.9027609268606369, -43.72435554967460547, 73.19276813305496887 ) ) ;
#20208=ORIENTED_EDGE ( 'NONE', *, *, #62208, .F. ) ;
#20209=ORIENTED_EDGE ( 'NONE', *, *, #50469, .T. ) ;
#20211=DIRECTION ( 'NONE',  ( -6.524622321627019585E-16, -4.013151879589939944E-16, -1.000000000000000000 ) ) ;
#20212=CARTESIAN_POINT ( 'NONE',  ( 116.5042510202518571, -34.04512512578506289, 145.0470538473389581 ) ) ;
#20214=CARTESIAN_POINT ( 'NONE',  ( 116.3183049785035195, -32.94379174720932468, 54.13562527591098217 ) ) ;
#20215=FACE_OUTER_BOUND ( 'NONE', #71868, .T. ) ;
#20220=CARTESIAN_POINT ( 'NONE',  ( 113.4020503763144632, -27.70036014686454351, 84.57753003781698453 ) ) ;
#20221=VERTEX_POINT ( 'NONE', #26184 ) ;
#20223=ORIENTED_EDGE ( 'NONE', *, *, #49169, .T. ) ;
#20226=CARTESIAN_POINT ( 'NONE',  ( 162.7131505118539962, -33.70561438052090608, 117.4678068554150627 ) ) ;
#20227=CARTESIAN_POINT ( 'NONE',  ( 109.0547627366692041, -28.78404389176943212, 197.6995189410199600 ) ) ;
#20230=ORIENTED_EDGE ( 'NONE', *, *, #37098, .F. ) ;
#20231=ORIENTED_EDGE ( 'NONE', *, *, #56043, .T. ) ;
#20232=EDGE_LOOP ( 'NONE', ( #79898, #61902 ) ) ;
#20233=CARTESIAN_POINT ( 'NONE',  ( 143.0664832912740110, -8.729447159940999512, 284.9256252759119548 ) ) ;
#20234=CARTESIAN_POINT ( 'NONE',  ( 135.2499137886320284, -21.21189172703428483, 1.845048092482432400 ) ) ;
#20236=VERTEX_POINT ( 'NONE', #53852 ) ;
#20238=CARTESIAN_POINT ( 'NONE',  ( 115.9133815579708937, -36.21888896485111076, 225.3044404487539794 ) ) ;
#20239=AXIS2_PLACEMENT_3D ( 'NONE', #7771, #13683, #41373 ) ;
#20245=VECTOR ( 'NONE', #79686, 1000.000000000000000 ) ;
#20246=ORIENTED_EDGE ( 'NONE', *, *, #32952, .T. ) ;
#20247=ADVANCED_FACE ( 'NONE', ( #81621 ), #13011, .T. ) ;
#20248=DIRECTION ( 'NONE',  ( 0.9825752044328148749, 0.1858654557302456822, 0.000000000000000000 ) ) ;
#20250=ORIENTED_EDGE ( 'NONE', *, *, #75210, .T. ) ;
#20251=EDGE_CURVE ( 'NONE', #44627, #3441, #68421, .T. ) ;
#20252=CARTESIAN_POINT ( 'NONE',  ( 107.2095755159442376, -27.45176125347251173, 227.8823760838769488 ) ) ;
#20253=AXIS2_PLACEMENT_3D ( 'NONE', #24262, #39220, #4260 ) ;
#20255=CARTESIAN_POINT ( 'NONE',  ( 113.3446846601215441, -45.07992904040708737, 143.0899109901969553 ) ) ;
#20256=CARTESIAN_POINT ( 'NONE',  ( 104.2200364793041274, -25.25138339198301907, 90.26991099019693365 ) ) ;
#20257=CARTESIAN_POINT ( 'NONE',  ( 102.9521648518240085, -29.48031188516382528, 249.5838068554170661 ) ) ;
#20258=DIRECTION ( 'NONE',  ( 0.000000000000000000, 0.000000000000000000, -1.000000000000000000 ) ) ;
#20260=CARTESIAN_POINT ( 'NONE',  ( 117.1971262914088499, -34.26925207598063849, 205.0156252759109634 ) ) ;
#20263=CARTESIAN_POINT ( 'NONE',  ( 116.3212776292296127, -32.94146857471318413, 287.6356252759109680 ) ) ;
#20265=ORIENTED_EDGE ( 'NONE', *, *, #51821, .F. ) ;
#20266=EDGE_CURVE ( 'NONE', #28847, #44183, #56485, .T. ) ;
#20269=EDGE_LOOP ( 'NONE', ( #26210, #64600, #59087, #87899 ) ) ;
#20272=CARTESIAN_POINT ( 'NONE',  ( 152.0371591254583450, -47.82818131005588214, 237.4678068554150059 ) ) ;
#20273=AXIS2_PLACEMENT_3D ( 'NONE', #74591, #87779, #11018 ) ;
#20274=CARTESIAN_POINT ( 'NONE',  ( 100.2985985360463843, -46.45756217656626319, 87.09276813305393716 ) ) ;
#20276=ADVANCED_FACE ( 'NONE', ( #709 ), #70208, .T. ) ;
#20278=LINE ( 'NONE', #76119, #84801 ) ;
#20280=CARTESIAN_POINT ( 'NONE',  ( 80.06648329127402519, -36.72944715994107412, -5.074374724089057764 ) ) ;
#20281=CARTESIAN_POINT ( 'NONE',  ( 117.3910620576582318, -35.19077923515893502, 214.9441967044829767 ) ) ;
#20282=CARTESIAN_POINT ( 'NONE',  ( 37.03715912545425937, -48.62818131006122258, 313.9678068554150059 ) ) ;
#20284=ORIENTED_EDGE ( 'NONE', *, *, #4986, .F. ) ;
#20285=CIRCLE ( 'NONE', #37648, 2.124999999999994227 ) ;
#20290=EDGE_CURVE ( 'NONE', #89556, #58657, #16002, .T. ) ;
#20291=DIRECTION ( 'NONE',  ( 8.673617379884035472E-16, 1.000000000000000000, 0.000000000000000000 ) ) ;
#20292=CARTESIAN_POINT ( 'NONE',  ( 98.90817802506259682, -30.16829472858045591, 240.7870538473399620 ) ) ;
#20293=ORIENTED_EDGE ( 'NONE', *, *, #8281, .T. ) ;
#20295=CARTESIAN_POINT ( 'NONE',  ( 113.8578909311569305, -28.74413913138208088, 139.5156252759109634 ) ) ;
#20296=CARTESIAN_POINT ( 'NONE',  ( 118.7325469213664633, -34.64676260937859098, 44.96705384733895272 ) ) ;
#20297=CARTESIAN_POINT ( 'NONE',  ( 108.8562982717690062, -47.04397778784520057, 163.7127681330539701 ) ) ;
#20298=DIRECTION ( 'NONE',  ( 0.000000000000000000, 0.000000000000000000, -1.000000000000000000 ) ) ;
#20299=CARTESIAN_POINT ( 'NONE',  ( 97.80977320450685397, -40.51274266863887874, 102.6352229270316627 ) ) ;
#20301=CARTESIAN_POINT ( 'NONE',  ( 172.5664832912729878, -27.57844715994070484, 198.9256252759119832 ) ) ;
#20303=LINE ( 'NONE', #88896, #56702 ) ;
#20304=ORIENTED_EDGE ( 'NONE', *, *, #47223, .T. ) ;
#20305=EDGE_LOOP ( 'NONE', ( #9869, #66279, #85436, #87470 ) ) ;
#20306=ORIENTED_EDGE ( 'NONE', *, *, #22653, .T. ) ;
#20307=AXIS2_PLACEMENT_3D ( 'NONE', #86027, #65992, #57850 ) ;
#20309=ORIENTED_EDGE ( 'NONE', *, *, #63000, .F. ) ;
#20311=CARTESIAN_POINT ( 'NONE',  ( 97.09625384711495144, -33.75906160244647936, 27.09562527591097236 ) ) ;
#20314=EDGE_CURVE ( 'NONE', #69306, #36268, #43825, .T. ) ;
#20315=VECTOR ( 'NONE', #32443, 1000.000000000000000 ) ;
#20316=CARTESIAN_POINT ( 'NONE',  ( 116.6941949105806060, -33.85593710834429260, 119.0581585122466635 ) ) ;
#20319=CARTESIAN_POINT ( 'NONE',  ( 111.4459538621439805, -44.65616828817710626, 252.3886103042673028 ) ) ;
#20320=ORIENTED_EDGE ( 'NONE', *, *, #5379, .F. ) ;
#20321=VERTEX_POINT ( 'NONE', #64734 ) ;
#20322=AXIS2_PLACEMENT_3D ( 'NONE', #13116, #13550, #32641 ) ;
#20323=EDGE_LOOP ( 'NONE', ( #56591, #7381, #48830, #14786 ) ) ;
#20324=CARTESIAN_POINT ( 'NONE',  ( 46.48091746482135278, -49.32844715994084339, 249.9678068554150343 ) ) ;
#20327=CARTESIAN_POINT ( 'NONE',  ( 97.81252181335722184, -40.51708140359354360, 276.6353344664656220 ) ) ;
#20328=CARTESIAN_POINT ( 'NONE',  ( 37.06648329127298780, 12.92155284005730387, 355.9756252759109998 ) ) ;
#20329=PLANE ( 'NONE',  #57486 ) ;
#20332=CARTESIAN_POINT ( 'NONE',  ( 112.1541913332956710, -45.76570811864968391, 257.9965776568639626 ) ) ;
#20335=DIRECTION ( 'NONE',  ( 0.000000000000000000, 0.000000000000000000, 1.000000000000000000 ) ) ;
#20337=CARTESIAN_POINT ( 'NONE',  ( 34.96670390244699433, -28.27351298637401200, -5.074374724088000832 ) ) ;
#20338=CARTESIAN_POINT ( 'NONE',  ( 115.6288848908637732, -37.98889302744424867, 71.54047132197199232 ) ) ;
#20341=LINE ( 'NONE', #41644, #47387 ) ;
#20344=ORIENTED_EDGE ( 'NONE', *, *, #67949, .F. ) ;
#20345=CARTESIAN_POINT ( 'NONE',  ( 101.9719236373881444, -46.53885842731235556, 167.1832443235299763 ) ) ;
#20348=CARTESIAN_POINT ( 'NONE',  ( 99.74964917879287896, -31.73022550229359595, 117.2815833058969446 ) ) ;
#20349=CARTESIAN_POINT ( 'NONE',  ( 130.3998166246059895, 12.92155284005730387, 361.9756252759109998 ) ) ;
#20350=DIRECTION ( 'NONE',  ( 0.000000000000000000, 0.000000000000000000, 1.000000000000000000 ) ) ;
#20351=CARTESIAN_POINT ( 'NONE',  ( 110.3788355960759162, -47.29890920647816444, 48.80610146638797175 ) ) ;
#20352=CARTESIAN_POINT ( 'NONE',  ( 116.7951252697354363, -39.38782979697960940, 84.61479194201683640 ) ) ;
#20359=VECTOR ( 'NONE', #39419, 1000.000000000000000 ) ;
#20360=ADVANCED_FACE ( 'NONE', ( #52833 ), #58356, .T. ) ;
#20362=ORIENTED_EDGE ( 'NONE', *, *, #56626, .F. ) ;
#20363=CARTESIAN_POINT ( 'NONE',  ( 114.1395267584829867, -29.97404255306813781, 234.4327681330549638 ) ) ;
#20364=CARTESIAN_POINT ( 'NONE',  ( 118.9423443782970082, -36.92851767163586629, 149.8127681330539644 ) ) ;
#20365=CARTESIAN_POINT ( 'NONE',  ( 94.58945128933383728, -41.88441296220994303, 290.1356252759106837 ) ) ;
#20366=CARTESIAN_POINT ( 'NONE',  ( 115.0354244594187065, -42.91078753811923718, 129.3020580932306416 ) ) ;
#20367=CARTESIAN_POINT ( 'NONE',  ( 116.6747397658760832, -32.59390121112949856, 75.14991099019697174 ) ) ;
#20368=DIRECTION ( 'NONE',  ( -1.000000000000000078E-15, -1.000000000000000083E-30, 1.000000000000000000 ) ) ;
#20372=EDGE_CURVE ( 'NONE', #76842, #15468, #44716, .T. ) ;
#20373=CARTESIAN_POINT ( 'NONE',  ( 107.0664832912750057, -36.72944715993903486, 9.125625275910969947 ) ) ;
#20374=VERTEX_POINT ( 'NONE', #86083 ) ;
#20378=CARTESIAN_POINT ( 'NONE',  ( 86.06670390244796920, -58.72944715994110254, 250.9178068554150514 ) ) ;
#20379=CARTESIAN_POINT ( 'NONE',  ( 112.6519946835718855, -45.50616226388166297, 263.0270538473394595 ) ) ;
#20381=EDGE_CURVE ( 'NONE', #88157, #67349, #23854, .T. ) ;
#20382=B_SPLINE_CURVE_WITH_KNOTS ( 'NONE', 3,
 ( #18174, #9587, #31357, #78655, #57727, #64998, #52221, #65872, #10476, #79986, #87232, #37290, #3224, #17739, #73134, #10915, #2782, #38619, #66315, #4103, #59497, #52661, #80419, #45857, #73588, #11364, #2334, #30034, #61733, #26337, #82222, #20427, #13604, #11819, #74489, #26774, #74038, #19073, #40847, #53563, #13163, #88132, #54458, #68123, #25438, #67216, #4557, #66771, #19977, #81767, #12262 ),
 .UNSPECIFIED., .F., .F.,
 ( 4, 2, 1, 1, 1, 1, 1, 1, 2, 2, 2, 2, 2, 2, 2, 1, 1, 1, 1, 1, 1, 1, 2, 2, 2, 2, 2, 2, 2, 2, 2, 4 ),
 ( 0.5000150356002270868, 0.5001371022419210943, 0.5002591688836151018, 0.5005033021670026727, 0.5009915687337783696, 0.5019681018673299855, 0.5039211681344335503, 0.5078273006686406799, 0.5156395657370546060, 0.5312640958738821251, 0.5625131561475371633, 0.6250112766948475729, 0.6875093972421580935, 0.7500075177894686140, 0.7500685511103151182, 0.7501295844311617333, 0.7502516510728743926, 0.7504957843562853892, 0.7509840509230981676, 0.7519605840567150645, 0.7539136503239830533, 0.7578197828585190310, 0.7656320479275997570, 0.7812565780657612091, 0.8125056383420810047, 0.8437546986184008002, 0.8750037588947205958, 0.9062528191710403913, 0.9375018794473601869, 0.9687509397236802045, 0.9843754698618401022, 1.000000000000000000 ),
 .UNSPECIFIED. ) ;
#20384=CARTESIAN_POINT ( 'NONE',  ( 165.9667039024459996, -28.27351298637401200, -5.074374724088000832 ) ) ;
#20385=CARTESIAN_POINT ( 'NONE',  ( 100.2135729635196242, -43.75450166755856429, 21.96133956162593748 ) ) ;
#20386=CARTESIAN_POINT ( 'NONE',  ( 112.6101834458390556, -28.37539859851495905, 99.61086039997772446 ) ) ;
#20387=CARTESIAN_POINT ( 'NONE',  ( 98.85726102317303798, -28.21728661942041683, 111.6870538473389587 ) ) ;
#20388=DIRECTION ( 'NONE',  ( 0.000000000000000000, 0.000000000000000000, 1.000000000000000000 ) ) ;
#20389=CARTESIAN_POINT ( 'NONE',  ( 113.6422709061198049, -28.58293356745306824, 164.5356252759109736 ) ) ;
#20391=VERTEX_POINT ( 'NONE', #18356 ) ;
#20392=CIRCLE ( 'NONE', #39234, 3.250000000000002665 ) ;
#20394=CARTESIAN_POINT ( 'NONE',  ( 80.06648329127398256, -8.729447159941058132, 8.525625275910952539 ) ) ;
#20396=VERTEX_POINT ( 'NONE', #65618 ) ;
#20398=CARTESIAN_POINT ( 'NONE',  ( 165.6738106836199904, -26.00627455219321860, 193.9678068554150059 ) ) ;
#20399=CARTESIAN_POINT ( 'NONE',  ( 102.3732866125132688, -26.67028275327534814, 135.4118157521009493 ) ) ;
#20400=EDGE_LOOP ( 'NONE', ( #81403, #77497 ) ) ;
#20403=DIRECTION ( 'NONE',  ( 0.000000000000000000, 1.000000000000000000, 0.000000000000000000 ) ) ;
#20404=EDGE_CURVE ( 'NONE', #81215, #3837, #46041, .T. ) ;
#20407=ORIENTED_EDGE ( 'NONE', *, *, #48351, .F. ) ;
#20408=EDGE_LOOP ( 'NONE', ( #29922, #47811 ) ) ;
#20409=VECTOR ( 'NONE', #26995, 1000.000000000000000 ) ;
#20410=VERTEX_POINT ( 'NONE', #52396 ) ;
#20413=PLANE ( 'NONE',  #54131 ) ;
#20414=EDGE_CURVE ( 'NONE', #59817, #65595, #79276, .T. ) ;
#20421=ORIENTED_EDGE ( 'NONE', *, *, #65032, .F. ) ;
#20422=CARTESIAN_POINT ( 'NONE',  ( 172.5664832912728457, -27.82844715994070484, 321.9256252759120116 ) ) ;
#20423=DIRECTION ( 'NONE',  ( 1.067522139062650671E-15, 1.000000000000000000, 0.000000000000000000 ) ) ;
#20424=CARTESIAN_POINT ( 'NONE',  ( 101.1405520526760284, -45.23956608920054379, 233.0803871806719769 ) ) ;
#20426=CARTESIAN_POINT ( 'NONE',  ( 109.5220866130624700, -46.80460460589462457, 83.75467289495797729 ) ) ;
#20427=CARTESIAN_POINT ( 'NONE',  ( 110.8969065101373701, -45.96677993874423152, 52.88927660374830708 ) ) ;
#20429=CARTESIAN_POINT ( 'NONE',  ( 110.1781312709696863, -27.19109411000012244, 20.82538979885751473 ) ) ;
#20430=CIRCLE ( 'NONE', #27682, 3.250000000000002665 ) ;
#20432=EDGE_CURVE ( 'NONE', #50014, #57432, #7309, .T. ) ;
#20434=VERTEX_POINT ( 'NONE', #31092 ) ;
#20435=ORIENTED_EDGE ( 'NONE', *, *, #48849, .F. ) ;
#20437=CARTESIAN_POINT ( 'NONE',  ( 115.8755296135227724, -35.76560983836216678, 275.3444404487542556 ) ) ;
#20439=CARTESIAN_POINT ( 'NONE',  ( 117.0608945213714946, -38.08045314215456045, 193.7189586075451473 ) ) ;
#20440=CARTESIAN_POINT ( 'NONE',  ( 109.7244294343027633, -27.00068945919879582, 139.8648275368623501 ) ) ;
#20441=CARTESIAN_POINT ( 'NONE',  ( 99.04406177815982915, -42.84125753558077321, 152.8439585988425051 ) ) ;
#20442=CIRCLE ( 'NONE', #56677, 1.000000000000000888 ) ;
#20443=CYLINDRICAL_SURFACE ( 'NONE', #69082, 10.00000000000002665 ) ;
#20444=VERTEX_POINT ( 'NONE', #25171 ) ;
#20446=DIRECTION ( 'NONE',  ( 0.000000000000000000, 0.000000000000000000, 1.000000000000000000 ) ) ;
#20447=ORIENTED_EDGE ( 'NONE', *, *, #21605, .T. ) ;
#20448=CARTESIAN_POINT ( 'NONE',  ( 105.9884003220067399, -26.36003215364494423, 50.15848241876796720 ) ) ;
#20449=ORIENTED_EDGE ( 'NONE', *, *, #71148, .T. ) ;
#20450=CARTESIAN_POINT ( 'NONE',  ( 115.8942015304759252, -33.87145029861233070, 281.8938046553057575 ) ) ;
#20453=CARTESIAN_POINT ( 'NONE',  ( 99.89458030379213938, -28.23347241844141919, 150.6356252759109680 ) ) ;
#20454=FACE_BOUND ( 'NONE', #58985, .T. ) ;
#20455=DIRECTION ( 'NONE',  ( -1.000000000000000000, -4.299999999999999979E-14, -1.000000000000000078E-15 ) ) ;
#20459=CARTESIAN_POINT ( 'NONE',  ( 96.63877784842330243, -35.80427747552585060, 227.2556252759109725 ) ) ;
#20461=ORIENTED_EDGE ( 'NONE', *, *, #80248, .F. ) ;
#20462=ORIENTED_EDGE ( 'NONE', *, *, #22981, .F. ) ;
#20463=CARTESIAN_POINT ( 'NONE',  ( 96.59840162804212582, -36.61878533396502888, 107.3184824187679567 ) ) ;
#20464=DIRECTION ( 'NONE',  ( 0.000000000000000000, 0.000000000000000000, -1.000000000000000000 ) ) ;
#20465=VERTEX_POINT ( 'NONE', #81064 ) ;
#20466=ORIENTED_EDGE ( 'NONE', *, *, #17380, .T. ) ;
#20468=EDGE_CURVE ( 'NONE', #38670, #20086, #24297, .T. ) ;
#20472=ADVANCED_FACE ( 'NONE', ( #72880 ), #32420, .F. ) ;
#20474=DIRECTION ( 'NONE',  ( -0.8660253910675250744, -0.0001484127182077903334, 0.5000000000000052180 ) ) ;
#20475=LINE ( 'NONE', #48587, #8889 ) ;
#20477=CARTESIAN_POINT ( 'NONE',  ( 115.1781387256201725, -32.22423048609648788, 177.0480903695909660 ) ) ;
#20478=CARTESIAN_POINT ( 'NONE',  ( 111.7488185767529245, -27.39065688012293265, 275.7070538473396937 ) ) ;
#20479=CARTESIAN_POINT ( 'NONE',  ( 98.04142522629925338, -41.04166024399867041, 57.68117463785360144 ) ) ;
#20482=ADVANCED_FACE ( 'NONE', ( #10647 ), #12007, .F. ) ;
#20484=AXIS2_PLACEMENT_3D ( 'NONE', #5599, #40550, #88280 ) ;
#20486=ORIENTED_EDGE ( 'NONE', *, *, #33276, .T. ) ;
#20488=AXIS2_PLACEMENT_3D ( 'NONE', #41332, #69061, #83158 ) ;
#20489=CARTESIAN_POINT ( 'NONE',  ( 177.3246001664172695, -48.34074026909179622, 300.4678068554149490 ) ) ;
#20492=DIRECTION ( 'NONE',  ( -1.000000000000000000, -2.756263715554006823E-15, 0.000000000000000000 ) ) ;
#20493=CARTESIAN_POINT ( 'NONE',  ( 97.31303930280388670, -38.96046111533910050, 16.50542592143737508 ) ) ;
#20494=B_SPLINE_CURVE_WITH_KNOTS ( 'NONE', 3,
 ( #41818, #21410, #34573, #34119, #69106, #75918, #28659, #13248, #60, #12809, #49081, #42274, #75477, #6426, #82306, #959, #61822, #33686, #82756, #35462, #506, #28199, #41376, #70002, #35015, #83640, #20519, #7774, #48185, #7330 ),
 .UNSPECIFIED., .F., .F.,
 ( 4, 2, 2, 2, 1, 2, 2, 2, 2, 2, 2, 2, 1, 2, 2, 4 ),
 ( 0.000000000000000000, 0.1250000000000000555, 0.1875000000000011935, 0.2187500000000017764, 0.2343750000000021094, 0.2421874999999987510, 0.2499999999999953926, 0.3750000000000031641, 0.4375000000000122125, 0.5000000000000212053, 0.6250000000000273115, 0.6875000000000297540, 0.7187500000000239808, 0.7343750000000210942, 0.7500000000000182077, 1.000000000000000000 ),
 .UNSPECIFIED. ) ;
#20495=FACE_BOUND ( 'NONE', #12724, .T. ) ;
#20496=CARTESIAN_POINT ( 'NONE',  ( 31.71315051186898870, -31.94127993907790852, -5.074374724088000832 ) ) ;
#20497=EDGE_CURVE ( 'NONE', #39861, #65845, #46367, .T. ) ;
#20498=CARTESIAN_POINT ( 'NONE',  ( 106.9915265980828849, -45.27055441931952373, 186.9924198280769758 ) ) ;
#20499=CARTESIAN_POINT ( 'NONE',  ( 106.9267615183890854, -26.22553017860169433, 60.08705384733897858 ) ) ;
#20500=ORIENTED_EDGE ( 'NONE', *, *, #12968, .F. ) ;
#20501=LINE ( 'NONE', #6852, #87227 ) ;
#20502=ORIENTED_EDGE ( 'NONE', *, *, #54800, .F. ) ;
#20504=ORIENTED_EDGE ( 'NONE', *, *, #32140, .T. ) ;
#20506=CARTESIAN_POINT ( 'NONE',  ( 97.33774478693185017, -34.07145668260515237, 262.1148423024291105 ) ) ;
#20507=ORIENTED_EDGE ( 'NONE', *, *, #77383, .T. ) ;
#20508=CARTESIAN_POINT ( 'NONE',  ( 115.9865316739811476, -32.12318019333122265, 165.2061833773214801 ) ) ;
#20509=DIRECTION ( 'NONE',  ( -0.7071067811865336949, -0.7071067811865614505, 0.000000000000000000 ) ) ;
#20510=CARTESIAN_POINT ( 'NONE',  ( 37.06648329127400388, 12.92155284005802685, 349.2756252759108406 ) ) ;
#20511=CIRCLE ( 'NONE', #26328, 5.599999999999994316 ) ;
#20513=ORIENTED_EDGE ( 'NONE', *, *, #63338, .T. ) ;
#20514=CARTESIAN_POINT ( 'NONE',  ( 96.69266203715996255, -37.96645829736812061, 41.42133956162496844 ) ) ;
#20516=CARTESIAN_POINT ( 'NONE',  ( 112.1386878447022042, -28.01244317163742892, 164.6565191118704661 ) ) ;
#20519=CARTESIAN_POINT ( 'NONE',  ( 132.9420963948872725, -16.21971364483387035, 1.822997995689119133 ) ) ;
#20520=ORIENTED_EDGE ( 'NONE', *, *, #16223, .T. ) ;
#20526=CARTESIAN_POINT ( 'NONE',  ( 107.3215613407866584, -25.65604926530302166, 71.04610146638795243 ) ) ;
#20527=CARTESIAN_POINT ( 'NONE',  ( 33.91903122894598965, -35.91149509761181235, -5.074374724088000832 ) ) ;
#20529=EDGE_CURVE ( 'NONE', #45331, #53161, #76877, .T. ) ;
#20533=CARTESIAN_POINT ( 'NONE',  ( 100.1408543393099393, -45.42701269980175738, 118.0413395616249659 ) ) ;
#20534=FACE_OUTER_BOUND ( 'NONE', #59547, .T. ) ;
#20535=VERTEX_POINT ( 'NONE', #75577 ) ;
#20536=AXIS2_PLACEMENT_3D ( 'NONE', #41160, #6659, #34353 ) ;
#20537=CARTESIAN_POINT ( 'NONE',  ( 96.78489722101822679, -35.14273565208915073, 262.2041967044821149 ) ) ;
#20541=CARTESIAN_POINT ( 'NONE',  ( 108.4174892634158027, -26.73503592936582152, 80.96895860834700898 ) ) ;
#20543=DIRECTION ( 'NONE',  ( 1.000000000000000078E-15, 1.000000000000000083E-30, -1.000000000000000000 ) ) ;
#20544=CARTESIAN_POINT ( 'NONE',  ( 103.5361331145922890, -27.60804031003065262, 215.3699109901969848 ) ) ;
#20546=VECTOR ( 'NONE', #40928, 1000.000000000000000 ) ;
#20548=CARTESIAN_POINT ( 'NONE',  ( 100.0878889097611335, -31.26788461136058217, 152.2301547344689538 ) ) ;
#20549=CIRCLE ( 'NONE', #27794, 3.300000000000000711 ) ;
#20551=LINE ( 'NONE', #993, #25494 ) ;
#20552=CARTESIAN_POINT ( 'NONE',  ( 110.7503267229639476, -45.78994093226354778, 278.8841967044818375 ) ) ;
#20553=CARTESIAN_POINT ( 'NONE',  ( 97.81170508561586985, -40.51744524251693491, 57.63550115181184452 ) ) ;
#20557=DIRECTION ( 'NONE',  ( 0.7071067811865279218, -0.7071067811865670016, 2.899137802865041747E-29 ) ) ;
#20559=CARTESIAN_POINT ( 'NONE',  ( 101.4165038149807003, -45.50681337102575696, 222.1213395616249784 ) ) ;
#20560=CARTESIAN_POINT ( 'NONE',  ( 113.2467642917647623, -28.75963215629028369, 169.5517896119323780 ) ) ;
#20562=VERTEX_POINT ( 'NONE', #26974 ) ;
#20564=CARTESIAN_POINT ( 'NONE',  ( 97.81168895331838087, -40.51742574516882200, 287.6356252759109680 ) ) ;
#20565=CARTESIAN_POINT ( 'NONE',  ( 81.44716491658451218, -21.11090284774729042, 7.925007058935930715 ) ) ;
#20566=LINE ( 'NONE', #40090, #85351 ) ;
#20568=AXIS2_PLACEMENT_3D ( 'NONE', #43733, #87658, #32682 ) ;
#20569=PLANE ( 'NONE',  #19466 ) ;
#20570=ORIENTED_EDGE ( 'NONE', *, *, #16091, .T. ) ;
#20571=CARTESIAN_POINT ( 'NONE',  ( 102.7372881883638058, -25.64480981559214712, 16.37276813305293999 ) ) ;
#20572=CARTESIAN_POINT ( 'NONE',  ( 101.2938852305094173, -26.37968400006201719, 255.4813395616251626 ) ) ;
#20573=EDGE_CURVE ( 'NONE', #89037, #47853, #5187, .T. ) ;
#20575=AXIS2_PLACEMENT_3D ( 'NONE', #48946, #76688, #42145 ) ;
#20576=EDGE_CURVE ( 'NONE', #58675, #1366, #61031, .T. ) ;
#20579=EDGE_CURVE ( 'NONE', #54148, #83421, #88761, .T. ) ;
#20580=CARTESIAN_POINT ( 'NONE',  ( 110.8543953957528032, -45.98426871307141539, 167.8856186728536386 ) ) ;
#20581=CARTESIAN_POINT ( 'NONE',  ( 98.66659878002396056, -40.67125783036974696, 59.49380465530595785 ) ) ;
#20582=CARTESIAN_POINT ( 'NONE',  ( 114.3591167413298280, -29.19972650290871030, 170.4641967044829585 ) ) ;
#20584=EDGE_LOOP ( 'NONE', ( #80849, #54973, #56212, #68716 ) ) ;
#20589=CARTESIAN_POINT ( 'NONE',  ( 172.5664832912729878, -18.82844715994071194, 75.92562527591206845 ) ) ;
#20590=ORIENTED_EDGE ( 'NONE', *, *, #70758, .T. ) ;
#20594=CARTESIAN_POINT ( 'NONE',  ( 97.58007606596183336, -34.66094392094686327, 105.5781341137909664 ) ) ;
#20595=CARTESIAN_POINT ( 'NONE',  ( 109.3417050147583041, -26.53289234591626311, 224.9013395616249511 ) ) ;
#20596=CARTESIAN_POINT ( 'NONE',  ( 117.7539631054257967, -31.66723592997632863, 214.1784824187679419 ) ) ;
#20597=CARTESIAN_POINT ( 'NONE',  ( 101.3960830062750631, -28.00733582429768376, 21.53562527591096298 ) ) ;
#20598=CARTESIAN_POINT ( 'NONE',  ( 97.81262911421374895, -40.51702269960655656, 122.6351715870756323 ) ) ;
#20599=DIRECTION ( 'NONE',  ( 0.000000000000000000, 0.000000000000000000, 1.000000000000000000 ) ) ;
#20603=CARTESIAN_POINT ( 'NONE',  ( 116.5944731948638804, -42.45914096480947819, 128.3956252759109873 ) ) ;
#20604=CARTESIAN_POINT ( 'NONE',  ( 95.29943635023701631, -34.95028898632038050, 71.20705384733993526 ) ) ;
#20605=CARTESIAN_POINT ( 'NONE',  ( 112.4344423749254531, -46.44530527459760805, 252.9661014663871015 ) ) ;
#20606=ORIENTED_EDGE ( 'NONE', *, *, #22071, .F. ) ;
#20607=CARTESIAN_POINT ( 'NONE',  ( 112.4544618167839332, -45.69580618038663999, 238.0070538473389377 ) ) ;
#20609=DIRECTION ( 'NONE',  ( 1.000000000000000000, 1.261617073437676668E-15, 9.462128050782575008E-16 ) ) ;
#20611=DIRECTION ( 'NONE',  ( -0.7071067811865774377, 0.7071067811865175967, -7.071067811865782003E-16 ) ) ;
#20612=CARTESIAN_POINT ( 'NONE',  ( 108.6893337760746334, -46.06423824197239725, 277.6356252759110248 ) ) ;
#20613=DIRECTION ( 'NONE',  ( -1.000000000000000078E-15, 1.000000000000000083E-30, 1.000000000000000000 ) ) ;
#20614=DIRECTION ( 'NONE',  ( 1.000000000000000000, 3.999999999999999995E-14, 1.000000000000000078E-15 ) ) ;
#20616=CYLINDRICAL_SURFACE ( 'NONE', #20879, 13.44999999999999396 ) ;
#20617=DIRECTION ( 'NONE',  ( 0.000000000000000000, 1.000000000000000000, 0.000000000000000000 ) ) ;
#20619=CARTESIAN_POINT ( 'NONE',  ( 104.4899544611976836, -26.97880758236209786, 76.28145860849610926 ) ) ;
#20622=ORIENTED_EDGE ( 'NONE', *, *, #31360, .T. ) ;
#20623=CARTESIAN_POINT ( 'NONE',  ( 177.8371591254543489, -47.82818131005477369, 249.9678068554149775 ) ) ;
#20624=CARTESIAN_POINT ( 'NONE',  ( 100.1628669375702714, -45.39175184048325917, 272.0289586092442278 ) ) ;
#20625=CARTESIAN_POINT ( 'NONE',  ( 97.98655846647217516, -41.85169789442448263, 132.7356252759109623 ) ) ;
#20626=CARTESIAN_POINT ( 'NONE',  ( 101.0616705854173460, -45.30470917520826646, 278.0899109901965858 ) ) ;
#20627=CARTESIAN_POINT ( 'NONE',  ( 116.3212776292296127, -32.94146857471318413, 287.6356252759109680 ) ) ;
#20629=LINE ( 'NONE', #13367, #3719 ) ;
#20630=EDGE_CURVE ( 'NONE', #10962, #88157, #54640, .T. ) ;
#20631=DIRECTION ( 'NONE',  ( 0.000000000000000000, 0.000000000000000000, 1.000000000000000000 ) ) ;
#20635=EDGE_CURVE ( 'NONE', #66334, #51011, #14184, .T. ) ;
#20638=ORIENTED_EDGE ( 'NONE', *, *, #30260, .T. ) ;
#20641=CARTESIAN_POINT ( 'NONE',  ( 115.2191710476659665, -34.18193581181276386, 173.4895626852199371 ) ) ;
#20644=DIRECTION ( 'NONE',  ( 0.000000000000000000, 0.000000000000000000, -1.000000000000000000 ) ) ;
#20645=CARTESIAN_POINT ( 'NONE',  ( 97.97553865104319470, -30.48296430071277641, 161.8594347997199918 ) ) ;
#20647=VECTOR ( 'NONE', #7329, 1000.000000000000000 ) ;
#20649=LINE ( 'NONE', #69691, #1238 ) ;
#20650=LINE ( 'NONE', #13826, #29487 ) ;
#20651=CARTESIAN_POINT ( 'NONE',  ( 116.7274023843879718, -38.25590632018516857, 113.7013395616259857 ) ) ;
#20652=ORIENTED_EDGE ( 'NONE', *, *, #76718, .F. ) ;
#20653=ORIENTED_EDGE ( 'NONE', *, *, #20771, .T. ) ;
#20657=CARTESIAN_POINT ( 'NONE',  ( 108.1128363339379490, -46.45408497333508535, 198.6613395616249989 ) ) ;
#20658=CARTESIAN_POINT ( 'NONE',  ( 117.0608945257504985, -38.08045309939960532, 38.71895861094868252 ) ) ;
#20659=CARTESIAN_POINT ( 'NONE',  ( 102.0675651188745832, -27.97020183595695997, 55.48833508751222610 ) ) ;
#20661=VECTOR ( 'NONE', #38493, 1000.000000000000000 ) ;
#20662=LINE ( 'NONE', #48327, #62290 ) ;
#20664=CARTESIAN_POINT ( 'NONE',  ( 116.8835868046513582, -40.17228670562625581, 133.5584824187679658 ) ) ;
#20665=EDGE_LOOP ( 'NONE', ( #56738, #20209, #27388, #88489 ) ) ;
#20666=EDGE_LOOP ( 'NONE', ( #46450, #58883, #75676, #16507 ) ) ;
#20667=ORIENTED_EDGE ( 'NONE', *, *, #69334, .F. ) ;
#20668=EDGE_CURVE ( 'NONE', #8418, #79915, #71008, .T. ) ;
#20669=CARTESIAN_POINT ( 'NONE',  ( 151.0371591254575208, -24.42818131005592264, 180.4678068554149775 ) ) ;
#20670=DIRECTION ( 'NONE',  ( 1.000000000000000078E-15, -1.000000000000000083E-30, -1.000000000000000000 ) ) ;
#20672=CARTESIAN_POINT ( 'NONE',  ( 115.0725392204758890, -35.00151292932243052, 181.8138046553059723 ) ) ;
#20673=VECTOR ( 'NONE', #72945, 1000.000000000000000 ) ;
#20674=DIRECTION ( 'NONE',  ( 1.000000000000000000, 4.163336342344333240E-14, 0.000000000000000000 ) ) ;
#20675=CARTESIAN_POINT ( 'NONE',  ( 105.8003522596126516, -26.72392167762159332, 26.17665498994805517 ) ) ;
#20676=VERTEX_POINT ( 'NONE', #22859 ) ;
#20677=EDGE_LOOP ( 'NONE', ( #10525, #65682, #33607, #50844, #38276 ) ) ;
#20678=ORIENTED_EDGE ( 'NONE', *, *, #39495, .F. ) ;
#20680=ORIENTED_EDGE ( 'NONE', *, *, #8509, .F. ) ;
#20681=VERTEX_POINT ( 'NONE', #76916 ) ;
#20682=CARTESIAN_POINT ( 'NONE',  ( 71.25614885437424562, -84.12815644128085069, 540.9756252759101471 ) ) ;
#20683=EDGE_CURVE ( 'NONE', #37688, #76536, #65334, .T. ) ;
#20685=CARTESIAN_POINT ( 'NONE',  ( 101.2707639275114815, -30.02587231748817231, 257.0758690201828927 ) ) ;
#20687=DIRECTION ( 'NONE',  ( -9.073094938289460781E-13, -1.000000000000000000, 0.000000000000000000 ) ) ;
#20691=AXIS2_PLACEMENT_3D ( 'NONE', #7522, #56555, #1161 ) ;
#20694=ORIENTED_EDGE ( 'NONE', *, *, #21002, .T. ) ;
#20695=AXIS2_PLACEMENT_3D ( 'NONE', #72451, #58793, #9331 ) ;
#20696=EDGE_CURVE ( 'NONE', #89471, #36163, #16065, .T. ) ;
#20697=CARTESIAN_POINT ( 'NONE',  ( 99.11752347482735104, -34.75543446931638414, 273.9509475124486357 ) ) ;
#20698=CARTESIAN_POINT ( 'NONE',  ( 111.8042541167996546, -25.83965636698058432, 134.7499109901969518 ) ) ;
#20699=CARTESIAN_POINT ( 'NONE',  ( 99.07096106853131801, -43.38529345585687480, 116.8784824187679732 ) ) ;
#20700=CARTESIAN_POINT ( 'NONE',  ( 99.03962527909632740, -36.84879970159397544, 249.5838068554172082 ) ) ;
#20702=PLANE ( 'NONE',  #77159 ) ;
#20703=CARTESIAN_POINT ( 'NONE',  ( 113.1553867986010857, -26.56284154956258092, 200.6470538473399756 ) ) ;
#20705=CARTESIAN_POINT ( 'NONE',  ( 34.27258461953899626, -35.55794170701810941, -5.074374724088000832 ) ) ;
#20708=EDGE_LOOP ( 'NONE', ( #1692, #14141, #18665, #58748 ) ) ;
#20709=VERTEX_POINT ( 'NONE', #7275 ) ;
#20710=FACE_OUTER_BOUND ( 'NONE', #32965, .T. ) ;
#20712=CARTESIAN_POINT ( 'NONE',  ( 117.0333688383452397, -30.31836458025946968, 144.2813395616249750 ) ) ;
#20715=CARTESIAN_POINT ( 'NONE',  ( 128.0667039024480118, -48.82844715994099971, 250.9178068554150514 ) ) ;
#20717=CARTESIAN_POINT ( 'NONE',  ( 97.81443832832722762, -40.51607714565724905, 56.63519146330476417 ) ) ;
#20718=CARTESIAN_POINT ( 'NONE',  ( 103.3114313307234085, -27.02747569519259230, 211.3699109901969848 ) ) ;
#20720=DIRECTION ( 'NONE',  ( -6.831565154159360295E-14, 1.000000000000000000, 0.000000000000000000 ) ) ;
#20721=ORIENTED_EDGE ( 'NONE', *, *, #23450, .T. ) ;
#20724=CYLINDRICAL_SURFACE ( 'NONE', #708, 0.5000000000000079936 ) ;
#20725=DIRECTION ( 'NONE',  ( 0.7071067811865475727, -0.7071067811865475727, 0.000000000000000000 ) ) ;
#20727=DIRECTION ( 'NONE',  ( 0.000000000000000000, -1.000000000000000000, 0.000000000000000000 ) ) ;
#20729=CARTESIAN_POINT ( 'NONE',  ( 116.0324533029107670, -32.23654553487196495, 194.1959605532332489 ) ) ;
#20730=CARTESIAN_POINT ( 'NONE',  ( 95.99055855653007541, -36.58346519971924948, 156.3280062282919687 ) ) ;
#20731=CARTESIAN_POINT ( 'NONE',  ( 115.8915968718629017, -31.17968520675552924, 30.27276813305396175 ) ) ;
#20732=CARTESIAN_POINT ( 'NONE',  ( 112.8039874620816789, -45.48581773443041953, 174.0384824187679556 ) ) ;
#20733=FACE_OUTER_BOUND ( 'NONE', #76723, .T. ) ;
#20734=CARTESIAN_POINT ( 'NONE',  ( 105.7996235970844907, -26.72402767612700103, 101.1773280814526430 ) ) ;
#20735=CARTESIAN_POINT ( 'NONE',  ( 181.9694315774339941, -34.03355364505720360, -5.074374724088000832 ) ) ;
#20736=DIRECTION ( 'NONE',  ( 0.000000000000000000, 0.000000000000000000, -1.000000000000000000 ) ) ;
#20737=DIRECTION ( 'NONE',  ( 1.000000000000000000, -4.163336342344339393E-15, -2.775557561562892929E-14 ) ) ;
#20738=CARTESIAN_POINT ( 'NONE',  ( 37.03715912545427358, -48.62818131006122258, 300.4678068554150059 ) ) ;
#20739=ORIENTED_EDGE ( 'NONE', *, *, #4382, .F. ) ;
#20740=VECTOR ( 'NONE', #70970, 1000.000000000000000 ) ;
#20741=EDGE_CURVE ( 'NONE', #78070, #54444, #88612, .T. ) ;
#20742=ORIENTED_EDGE ( 'NONE', *, *, #31144, .F. ) ;
#20744=EDGE_LOOP ( 'NONE', ( #66354, #89764, #22353, #39640 ) ) ;
#20745=CARTESIAN_POINT ( 'NONE',  ( 130.5667039024482960, -33.42944715994102722, 249.5838068554162987 ) ) ;
#20746=CARTESIAN_POINT ( 'NONE',  ( 114.3378803067696197, -44.16957155219873243, 69.19276813305397411 ) ) ;
#20747=CARTESIAN_POINT ( 'NONE',  ( 151.0371591254572934, -24.42818131005592974, 300.4678068554149490 ) ) ;
#20749=CARTESIAN_POINT ( 'NONE',  ( 103.5276745422693523, -26.83930826182397311, 186.3499109901969746 ) ) ;
#20751=CARTESIAN_POINT ( 'NONE',  ( 98.80150335516665905, -38.88496061976939444, 275.9524198280767564 ) ) ;
#20752=ORIENTED_EDGE ( 'NONE', *, *, #77998, .T. ) ;
#20755=VECTOR ( 'NONE', #77586, 999.9999999999998863 ) ;
#20756=ADVANCED_FACE ( 'NONE', ( #62674 ), #89499, .F. ) ;
#20757=DIRECTION ( 'NONE',  ( 1.000000000000000000, 4.163336342344333240E-14, 0.000000000000000000 ) ) ;
#20759=TOROIDAL_SURFACE ( 'NONE', #55533, 13.50000000000000000, 0.5000000000000000000 ) ;
#20761=CARTESIAN_POINT ( 'NONE',  ( 108.4139696804844846, -26.73458958342868996, 274.9688129555700584 ) ) ;
#20762=FACE_OUTER_BOUND ( 'NONE', #78808, .T. ) ;
#20763=VECTOR ( 'NONE', #81712, 1000.000000000000000 ) ;
#20767=CARTESIAN_POINT ( 'NONE',  ( 100.6687104586878547, -44.89077600197693130, 277.0594347997210889 ) ) ;
#20768=DIRECTION ( 'NONE',  ( 1.000000000000000078E-15, 0.000000000000000000, -1.000000000000000000 ) ) ;
#20769=EDGE_CURVE ( 'NONE', #25006, #78471, #31991, .T. ) ;
#20770=ORIENTED_EDGE ( 'NONE', *, *, #39825, .T. ) ;
#20771=EDGE_CURVE ( 'NONE', #8503, #35967, #54036, .T. ) ;
#20772=DIRECTION ( 'NONE',  ( -1.000000000000000078E-15, 1.000000000000000083E-30, 1.000000000000000000 ) ) ;
#20773=CARTESIAN_POINT ( 'NONE',  ( 49.16670390244701139, -28.27351298637340093, -5.074374724088000832 ) ) ;
#20774=CARTESIAN_POINT ( 'NONE',  ( 114.5896176151078976, -33.49137084947443554, 76.96809036959095351 ) ) ;
#20778=DIRECTION ( 'NONE',  ( 4.299999999999999979E-14, -1.000000000000000000, 4.400000000000000367E-29 ) ) ;
#20779=CYLINDRICAL_SURFACE ( 'NONE', #28539, 3.249999999999975131 ) ;
#20780=VERTEX_POINT ( 'NONE', #50835 ) ;
#20783=VECTOR ( 'NONE', #30582, 1000.000000000000000 ) ;
#20785=CARTESIAN_POINT ( 'NONE',  ( 113.3314600845033482, -45.06233935626208620, 143.0899109901969553 ) ) ;
#20786=ORIENTED_EDGE ( 'NONE', *, *, #46720, .F. ) ;
#20788=CARTESIAN_POINT ( 'NONE',  ( 97.81169160209351787, -40.51741184665055329, 67.63577596198375375 ) ) ;
#20789=CARTESIAN_POINT ( 'NONE',  ( 97.07454461617307118, -38.04679588918885713, 147.8615833058969713 ) ) ;
#20790=CARTESIAN_POINT ( 'NONE',  ( 97.81168895331838087, -40.51742574516882200, 11.63562527591094309 ) ) ;
#20792=CARTESIAN_POINT ( 'NONE',  ( 115.2242804385497976, -44.22181337150698255, 74.22324432352993995 ) ) ;
#20797=EDGE_LOOP ( 'NONE', ( #50639, #7122 ) ) ;
#20799=FACE_OUTER_BOUND ( 'NONE', #80113, .T. ) ;
#20800=VERTEX_POINT ( 'NONE', #69948 ) ;
#20801=CARTESIAN_POINT ( 'NONE',  ( 117.4251315444616353, -36.24242395571270237, 268.8518157521021408 ) ) ;
#20802=CARTESIAN_POINT ( 'NONE',  ( 95.99102054923815786, -36.58347128883620059, 152.3280062282919971 ) ) ;
#20805=CARTESIAN_POINT ( 'NONE',  ( 113.2454986999111100, -28.75867294631898829, 140.5522919423851249 ) ) ;
#20806=CARTESIAN_POINT ( 'NONE',  ( 98.14961424977839499, -43.26117181588809757, 102.8175300378159847 ) ) ;
#20807=CARTESIAN_POINT ( 'NONE',  ( 97.81413651554109379, -40.51640884438177181, 97.63607350422876152 ) ) ;
#20809=EDGE_LOOP ( 'NONE', ( #44462, #30470, #44697, #64404 ) ) ;
#20811=EDGE_CURVE ( 'NONE', #65595, #22170, #29060, .T. ) ;
#20812=CARTESIAN_POINT ( 'NONE',  ( 21.03715912545745326, -47.82818131006196438, 117.4678068554150485 ) ) ;
#20815=DIRECTION ( 'NONE',  ( 0.7071067810573886669, 0.7071067813157063675, 7.071067810573880276E-16 ) ) ;
#20816=DIRECTION ( 'NONE',  ( 1.000000000000000000, 6.145690160522480771E-16, 0.000000000000000000 ) ) ;
#20817=CARTESIAN_POINT ( 'NONE',  ( 118.0833341887621373, -37.62838194956883342, 38.77372051400595865 ) ) ;
#20819=VECTOR ( 'NONE', #89532, 1000.000000000000000 ) ;
#20821=DIRECTION ( 'NONE',  ( 0.7071067811865460184, 0.000000000000000000, 0.7071067811865487940 ) ) ;
#20822=CARTESIAN_POINT ( 'NONE',  ( 111.8803212371932148, -27.54331830560560590, 14.68038718067299442 ) ) ;
#20823=FACE_OUTER_BOUND ( 'NONE', #84354, .T. ) ;
#20824=CARTESIAN_POINT ( 'NONE',  ( 114.7100688122352494, -43.78666090992606996, 119.2327681330539804 ) ) ;
#20826=CARTESIAN_POINT ( 'NONE',  ( 102.8958089960464690, -27.08850953439599962, 155.4013395616249795 ) ) ;
#20827=LINE ( 'NONE', #54864, #14816 ) ;
#20830=CARTESIAN_POINT ( 'NONE',  ( 194.0667039024473297, -24.92844715993408045, 300.4678068554149490 ) ) ;
#20831=CARTESIAN_POINT ( 'NONE',  ( 135.9115321082789194, -34.68812259377269669, 2.188418746640047541 ) ) ;
#20833=DIRECTION ( 'NONE',  ( -1.000000000000000078E-15, 1.000000000000000083E-30, 1.000000000000000000 ) ) ;
#20834=CARTESIAN_POINT ( 'NONE',  ( 113.5926674049485854, -44.96113684323219672, 168.1099109901969939 ) ) ;
#20836=FACE_OUTER_BOUND ( 'NONE', #84614, .T. ) ;
#20837=CARTESIAN_POINT ( 'NONE',  ( 97.45308667932049218, -40.90817919144255654, 227.6527681330539679 ) ) ;
#20840=DIRECTION ( 'NONE',  ( 0.000000000000000000, 0.000000000000000000, 1.000000000000000000 ) ) ;
#20842=CIRCLE ( 'NONE', #48359, 5.799999999999998934 ) ;
#20845=EDGE_LOOP ( 'NONE', ( #31904, #81782, #17974, #63107 ) ) ;
#20848=EDGE_LOOP ( 'NONE', ( #69792, #38632, #55869, #14926 ) ) ;
#20850=CARTESIAN_POINT ( 'NONE',  ( 115.8552077933167794, -44.67884570232850194, 229.2413395616249545 ) ) ;
#20851=DIRECTION ( 'NONE',  ( -0.7071067812160258814, 0.7071067811570692641, -2.899137802744100161E-29 ) ) ;
#20852=CARTESIAN_POINT ( 'NONE',  ( 135.3321452824298774, -16.28157797494703374, 1.873071231934059444 ) ) ;
#20854=PLANE ( 'NONE',  #45633 ) ;
#20855=DIRECTION ( 'NONE',  ( -0.9254794337955620787, -0.3787978585227822492, 0.000000000000000000 ) ) ;
#20856=CARTESIAN_POINT ( 'NONE',  ( 100.5368863760760973, -27.78183265877541430, 30.56610146638794134 ) ) ;
#20859=VERTEX_POINT ( 'NONE', #63579 ) ;
#20860=EDGE_CURVE ( 'NONE', #22586, #29395, #35403, .T. ) ;
#20861=FACE_OUTER_BOUND ( 'NONE', #25933, .T. ) ;
#20864=CARTESIAN_POINT ( 'NONE',  ( 98.06605190618653012, -40.64173669134672906, 227.6527681330529731 ) ) ;
#20865=CARTESIAN_POINT ( 'NONE',  ( 130.3998166246070127, 12.92155284005802685, 334.6228282640714156 ) ) ;
#20867=CARTESIAN_POINT ( 'NONE',  ( 98.65123886609836745, -31.74476095556103061, 81.90133956162493689 ) ) ;
#20868=CARTESIAN_POINT ( 'NONE',  ( 172.5664832912729878, -27.82844715994070484, 314.1756252759120116 ) ) ;
#20869=CARTESIAN_POINT ( 'NONE',  ( 103.2775828556913211, -27.47503018801354457, 21.38570542117368234 ) ) ;
#20870=EDGE_CURVE ( 'NONE', #36562, #20391, #22704, .T. ) ;
#20871=VERTEX_POINT ( 'NONE', #28600 ) ;
#20872=CARTESIAN_POINT ( 'NONE',  ( 116.3212776292296127, -32.94146857471318413, 287.6356252759109680 ) ) ;
#20875=VERTEX_POINT ( 'NONE', #71738 ) ;
#20877=CARTESIAN_POINT ( 'NONE',  ( 116.9161372654479578, -38.84013935494854763, 255.0901547344684559 ) ) ;
#20878=EDGE_CURVE ( 'NONE', #60824, #30264, #46500, .T. ) ;
#20879=AXIS2_PLACEMENT_3D ( 'NONE', #48285, #27863, #48734 ) ;
#20880=DIRECTION ( 'NONE',  ( 0.000000000000000000, 0.000000000000000000, 1.000000000000000000 ) ) ;
#20881=CARTESIAN_POINT ( 'NONE',  ( 193.5667039024416454, -48.82844715994099971, 180.4678068554150343 ) ) ;
#20883=ADVANCED_FACE ( 'NONE', ( #43109 ), #70393, .F. ) ;
#20884=CARTESIAN_POINT ( 'NONE',  ( 109.7248659292862385, -27.00080518209267311, 84.86479194192601483 ) ) ;
#20886=VERTEX_POINT ( 'NONE', #37213 ) ;
#20888=CARTESIAN_POINT ( 'NONE',  ( 30.48091746481826192, -48.32844715994148999, 300.4678068554150059 ) ) ;
#20890=CARTESIAN_POINT ( 'NONE',  ( 101.1416012009399026, -28.10844496237015733, 50.55562527591095545 ) ) ;
#20891=ORIENTED_EDGE ( 'NONE', *, *, #76871, .F. ) ;
#20892=CARTESIAN_POINT ( 'NONE',  ( 105.5073833390055853, -45.15143093073633196, 11.85241982807799843 ) ) ;
#20894=FACE_OUTER_BOUND ( 'NONE', #52033, .T. ) ;
#20895=CARTESIAN_POINT ( 'NONE',  ( 114.0663967180213803, -29.08153105160599949, 154.4746728949589851 ) ) ;
#20896=DIRECTION ( 'NONE',  ( -4.237773401492740281E-14, 1.000000000000000000, 0.000000000000000000 ) ) ;
#20898=CARTESIAN_POINT ( 'NONE',  ( 97.81168895331838087, -40.51742574516882200, 9.635625275910941312 ) ) ;
#20901=CARTESIAN_POINT ( 'NONE',  ( 117.5177603787924170, -36.12629959281294134, 224.8727681330539667 ) ) ;
#20903=EDGE_LOOP ( 'NONE', ( #53382, #81746, #14366, #61792 ) ) ;
#20904=CARTESIAN_POINT ( 'NONE',  ( 136.5663465660554721, -37.87725565067738387, 7.080220459966729329 ) ) ;
#20906=CARTESIAN_POINT ( 'NONE',  ( 95.98172161192206886, -37.30002307145830542, 117.3794347997199594 ) ) ;
#20908=AXIS2_PLACEMENT_3D ( 'NONE', #42121, #6273, #63018 ) ;
#20909=VECTOR ( 'NONE', #54302, 1000.000000000000000 ) ;
#20910=ORIENTED_EDGE ( 'NONE', *, *, #79874, .T. ) ;
#20912=ORIENTED_EDGE ( 'NONE', *, *, #41642, .T. ) ;
#20913=CIRCLE ( 'NONE', #52816, 2.517499999999998739 ) ;
#20915=CARTESIAN_POINT ( 'NONE',  ( 182.2420472961719895, -31.76306994223730840, -5.074374724088000832 ) ) ;
#20917=LINE ( 'NONE', #48588, #28717 ) ;
#20918=CARTESIAN_POINT ( 'NONE',  ( 106.9948502263972188, -44.89183619263916825, 185.3880903695919642 ) ) ;
#20919=CARTESIAN_POINT ( 'NONE',  ( 100.0093689611455687, -28.97871315454919028, 281.6641967044822650 ) ) ;
#20920=CARTESIAN_POINT ( 'NONE',  ( 113.1765051245399860, -44.75320790169451612, 59.09377906252450430 ) ) ;
#20921=EDGE_CURVE ( 'NONE', #14315, #19682, #84278, .T. ) ;
#20922=EDGE_LOOP ( 'NONE', ( #14212, #38232 ) ) ;
#20924=ADVANCED_FACE ( 'NONE', ( #13425 ), #6603, .T. ) ;
#20928=CARTESIAN_POINT ( 'NONE',  ( 31.56670390244800828, -32.29483332968611364, -5.074374724088000832 ) ) ;
#20929=LINE ( 'NONE', #40470, #58479 ) ;
#20930=CARTESIAN_POINT ( 'NONE',  ( 97.78482178150787263, -40.45120638126190471, 16.62993809196701989 ) ) ;
#20931=DIRECTION ( 'NONE',  ( 0.000000000000000000, 1.000000000000000000, 0.000000000000000000 ) ) ;
#20932=CARTESIAN_POINT ( 'NONE',  ( 107.0664832912750057, -36.72944715993903486, 0.4256252759109709349 ) ) ;
#20933=CARTESIAN_POINT ( 'NONE',  ( 115.3666750469823938, -34.71377145672549602, 208.4381341137909658 ) ) ;
#20934=CARTESIAN_POINT ( 'NONE',  ( 97.24697957573494023, -33.09846756419045022, 66.04419670448297097 ) ) ;
#20937=CARTESIAN_POINT ( 'NONE',  ( 91.06648329127391150, -36.72944715993925513, -4.074374724089044442 ) ) ;
#20938=EDGE_LOOP ( 'NONE', ( #16192, #20912 ) ) ;
#20941=DIRECTION ( 'NONE',  ( -6.524622321627019585E-16, -4.013151879589939944E-16, -1.000000000000000000 ) ) ;
#20942=CARTESIAN_POINT ( 'NONE',  ( 149.4532656544376721, -72.54365454176046057, 361.9756252759100335 ) ) ;
#20944=CIRCLE ( 'NONE', #49974, 2.116999999999993776 ) ;
#20946=PLANE ( 'NONE',  #87261 ) ;
#20947=EDGE_LOOP ( 'NONE', ( #76052, #52346, #22493, #87440 ) ) ;
#20948=CARTESIAN_POINT ( 'NONE',  ( 98.70474251149389033, -42.99264563182325816, 66.83848241876793850 ) ) ;
#20949=AXIS2_PLACEMENT_3D ( 'NONE', #7207, #68536, #41252 ) ;
#20952=CARTESIAN_POINT ( 'NONE',  ( 50.96943157740487607, -34.03355364506408165, 193.9678068554150911 ) ) ;
#20953=CARTESIAN_POINT ( 'NONE',  ( 177.4809174648213173, -48.32844715993478957, 300.4678068554149490 ) ) ;
#20954=ORIENTED_EDGE ( 'NONE', *, *, #26490, .F. ) ;
#20955=CARTESIAN_POINT ( 'NONE',  ( 114.6040617491220246, -30.10671728496298627, 120.3995749443976706 ) ) ;
#20956=LINE ( 'NONE', #27768, #38547 ) ;
#20959=CARTESIAN_POINT ( 'NONE',  ( 117.1846329980857178, -34.12938843674525202, 120.0270538473389479 ) ) ;
#20965=CIRCLE ( 'NONE', #79013, 3.249999999999975131 ) ;
#20966=AXIS2_PLACEMENT_3D ( 'NONE', #82664, #40839, #68116 ) ;
#20968=EDGE_CURVE ( 'NONE', #85809, #1145, #56071, .T. ) ;
#20972=CARTESIAN_POINT ( 'NONE',  ( 102.8912152862170188, -46.22186109533342346, 128.2346728949579528 ) ) ;
#20973=CARTESIAN_POINT ( 'NONE',  ( 32.16397622746000451, -34.03355364505800651, 237.4678068554150059 ) ) ;
#20975=AXIS2_PLACEMENT_3D ( 'NONE', #82304, #45936, #18706 ) ;
#20976=AXIS2_PLACEMENT_3D ( 'NONE', #17302, #23680, #78656 ) ;
#20977=ADVANCED_FACE ( 'NONE', ( #1143 ), #89742, .F. ) ;
#20978=CARTESIAN_POINT ( 'NONE',  ( 115.7579298488886224, -31.01215564512775558, 250.2899109901966028 ) ) ;
#20979=CARTESIAN_POINT ( 'NONE',  ( 162.5667039024470171, -32.29483332968611364, -5.074374724088000832 ) ) ;
#20985=CARTESIAN_POINT ( 'NONE',  ( 107.6181574201208662, -47.08485352040301564, 197.6308633711499567 ) ) ;
#20987=ORIENTED_EDGE ( 'NONE', *, *, #68381, .F. ) ;
#20988=CARTESIAN_POINT ( 'NONE',  ( 115.8989637469753831, -39.93316602039875107, 169.9692023535169483 ) ) ;
#20989=EDGE_CURVE ( 'NONE', #24368, #74810, #18969, .T. ) ;
#20991=CARTESIAN_POINT ( 'NONE',  ( 110.4493835822141676, -45.49486465592072904, 14.28920235351599466 ) ) ;
#20992=DIRECTION ( 'NONE',  ( 0.000000000000000000, 1.000000000000000000, 0.000000000000000000 ) ) ;
#20993=ADVANCED_FACE ( 'NONE', ( #48808 ), #83366, .T. ) ;
#20994=CARTESIAN_POINT ( 'NONE',  ( 108.3328345498486414, -46.73492894964222444, 267.6773957667126069 ) ) ;
#20996=FACE_OUTER_BOUND ( 'NONE', #80597, .T. ) ;
#20998=CARTESIAN_POINT ( 'NONE',  ( 96.87985868497418096, -34.61725761836211035, 216.1641967044819808 ) ) ;
#20999=CARTESIAN_POINT ( 'NONE',  ( 86.06670390244796920, -50.82844715994100682, 198.9178068554149945 ) ) ;
#21000=ORIENTED_EDGE ( 'NONE', *, *, #19752, .T. ) ;
#21001=EDGE_LOOP ( 'NONE', ( #63353, #80425, #64683, #36779 ) ) ;
#21002=EDGE_CURVE ( 'NONE', #73956, #12535, #33856, .T. ) ;
#21007=AXIS2_PLACEMENT_3D ( 'NONE', #37054, #24321, #2094 ) ;
#21009=ORIENTED_EDGE ( 'NONE', *, *, #39155, .T. ) ;
#21010=DIRECTION ( 'NONE',  ( -4.194175870806139918E-14, 1.000000000000000000, 0.000000000000000000 ) ) ;
#21011=AXIS2_PLACEMENT_3D ( 'NONE', #38036, #65727, #3509 ) ;
#21012=CARTESIAN_POINT ( 'NONE',  ( 112.4544618167839332, -45.69580618038663999, 238.0070538473389377 ) ) ;
#21013=ORIENTED_EDGE ( 'NONE', *, *, #78008, .T. ) ;
#21015=DIRECTION ( 'NONE',  ( -1.000000000000000078E-15, 1.000000000000000083E-30, 1.000000000000000000 ) ) ;
#21017=CARTESIAN_POINT ( 'NONE',  ( 112.7718126367562093, -42.56716444297848767, 71.01094751244896486 ) ) ;
#21018=CARTESIAN_POINT ( 'NONE',  ( 109.8617963350518920, -26.66349048206837580, 170.8613395616249591 ) ) ;
#21019=DIRECTION ( 'NONE',  ( -0.000000000000000000, -0.000000000000000000, 1.000000000000000000 ) ) ;
#21020=ORIENTED_EDGE ( 'NONE', *, *, #76862, .T. ) ;
#21021=B_SPLINE_CURVE_WITH_KNOTS ( 'NONE', 3,
 ( #781, #55708, #75298, #83024, #56169, #28478, #14424, #42104, #33945, #83919, #40762, #70270, #68484, #34849, #27145, #82582, #49363, #48009 ),
 .UNSPECIFIED., .F., .F.,
 ( 4, 2, 2, 2, 2, 2, 2, 2, 4 ),
 ( 0.000000000000000000, 0.06250000000899012809, 0.1250000000179802562, 0.1875000000269703704, 0.2500000000359605123, 0.3125000000449506543, 0.3750000000539407408, 0.4375000000629308827, 0.5000000000719210247 ),
 .UNSPECIFIED. ) ;
#21022=ADVANCED_FACE ( 'NONE', ( #49266, #15219 ), #21593, .F. ) ;
#21023=DIRECTION ( 'NONE',  ( 0.000000000000000000, 0.000000000000000000, -1.000000000000000000 ) ) ;
#21028=PLANE ( 'NONE',  #8220 ) ;
#21029=VECTOR ( 'NONE', #73367, 1000.000000000000000 ) ;
#21030=EDGE_LOOP ( 'NONE', ( #81612, #49676, #4868, #40425 ) ) ;
#21032=DIRECTION ( 'NONE',  ( 0.7071067811578790607, 0.7071067812152160847, 0.000000000000000000 ) ) ;
#21033=AXIS2_PLACEMENT_3D ( 'NONE', #18220, #40000, #81372 ) ;
#21034=CARTESIAN_POINT ( 'NONE',  ( 102.7155009198991280, -28.78705314239651969, 99.88575316140996563 ) ) ;
#21036=CARTESIAN_POINT ( 'NONE',  ( 97.14868559305091367, -40.01329441332335790, 241.5813395616249863 ) ) ;
#21038=CARTESIAN_POINT ( 'NONE',  ( 96.69582475441069391, -35.54038568221476879, 206.2356252759109623 ) ) ;
#21039=CARTESIAN_POINT ( 'NONE',  ( 117.9019101119219357, -41.46671778014663801, 54.49848241876792088 ) ) ;
#21040=DIRECTION ( 'NONE',  ( -4.554376769437570034E-14, 1.000000000000000000, 0.000000000000000000 ) ) ;
#21041=CARTESIAN_POINT ( 'NONE',  ( 126.0667039024479550, -14.72944715994094977, 199.5838068554170093 ) ) ;
#21043=VERTEX_POINT ( 'NONE', #62007 ) ;
#21047=CARTESIAN_POINT ( 'NONE',  ( 102.0112516875887252, -27.67497761899947406, 105.4937205140069665 ) ) ;
#21048=ADVANCED_FACE ( 'NONE', ( #56532 ), #680, .F. ) ;
#21049=CARTESIAN_POINT ( 'NONE',  ( 99.46959489307312197, -43.93319290153426238, 81.92991099019597812 ) ) ;
#21050=CARTESIAN_POINT ( 'NONE',  ( 106.5652189068774902, -47.22232703829767786, 247.5384824187679556 ) ) ;
#21051=ORIENTED_EDGE ( 'NONE', *, *, #54255, .F. ) ;
#21052=CARTESIAN_POINT ( 'NONE',  ( 107.2492389712779612, -24.88009754917498739, 230.0641967044819580 ) ) ;
#21054=CARTESIAN_POINT ( 'NONE',  ( 116.3274949261486881, -32.94048995676258329, 25.13562527591095375 ) ) ;
#21055=CARTESIAN_POINT ( 'NONE',  ( 98.05794652679882972, -41.07680959571720081, 27.68475610168817269 ) ) ;
#21057=CARTESIAN_POINT ( 'NONE',  ( 107.8140391369254019, -46.65806076900804555, 277.6356252759110816 ) ) ;
#21058=CYLINDRICAL_SURFACE ( 'NONE', #51426, 2.517500000000000071 ) ;
#21059=CARTESIAN_POINT ( 'NONE',  ( 25.56670390244829250, -48.82844715994168183, 290.7178068554150059 ) ) ;
#21060=DIRECTION ( 'NONE',  ( -0.7071067811865433539, -0.7071067811865516806, -7.071067811865440820E-16 ) ) ;
#21063=CARTESIAN_POINT ( 'NONE',  ( 105.7925720156200384, -26.72498208092823546, 40.17704486214662296 ) ) ;
#21064=CARTESIAN_POINT ( 'NONE',  ( 33.92127028473601769, -29.73316016639540749, -5.074374724088000832 ) ) ;
#21066=EDGE_LOOP ( 'NONE', ( #68230, #31169 ) ) ;
#21067=DIRECTION ( 'NONE',  ( -1.000000000000000078E-15, 1.000000000000000083E-30, 1.000000000000000000 ) ) ;
#21068=CARTESIAN_POINT ( 'NONE',  ( 97.20287302226383019, -40.27875065248429820, 266.6013395616254797 ) ) ;
#21069=CARTESIAN_POINT ( 'NONE',  ( 96.67093460706618657, -35.94617138369610387, 142.2670538473399517 ) ) ;
#21070=CARTESIAN_POINT ( 'NONE',  ( 96.76602677561474763, -40.86443131079876423, 247.6422919425769749 ) ) ;
#21072=CARTESIAN_POINT ( 'NONE',  ( 128.0667039024480118, -50.82844715994100682, 57.91780685541508689 ) ) ;
#21073=CARTESIAN_POINT ( 'NONE',  ( 82.15318967142708573, -34.93816060011965163, 7.482180659748648210 ) ) ;
#21074=CARTESIAN_POINT ( 'NONE',  ( 117.0718980089568078, -35.46249550098277581, 139.9272908994846034 ) ) ;
#21075=VECTOR ( 'NONE', #7961, 1000.000000000000000 ) ;
#21076=FACE_OUTER_BOUND ( 'NONE', #17438, .T. ) ;
#21077=AXIS2_PLACEMENT_3D ( 'NONE', #53538, #12241, #17720 ) ;
#21080=ORIENTED_EDGE ( 'NONE', *, *, #6616, .T. ) ;
#21081=EDGE_CURVE ( 'NONE', #79856, #26963, #42103, .T. ) ;
#21082=CARTESIAN_POINT ( 'NONE',  ( 107.4755550402934148, -45.77628807984756065, 192.0228960185529559 ) ) ;
#21084=ORIENTED_EDGE ( 'NONE', *, *, #18409, .T. ) ;
#21086=EDGE_CURVE ( 'NONE', #22615, #7080, #41548, .T. ) ;
#21087=CARTESIAN_POINT ( 'NONE',  ( 116.7861719071672155, -43.46560779248400763, 159.3441967044829539 ) ) ;
#21088=FACE_OUTER_BOUND ( 'NONE', #42471, .T. ) ;
#21090=PLANE ( 'NONE',  #34186 ) ;
#21092=EDGE_CURVE ( 'NONE', #32624, #3091, #27937, .T. ) ;
#21094=CARTESIAN_POINT ( 'NONE',  ( 102.8368274790082921, -27.91052165842129185, 95.43276813305395478 ) ) ;
#21096=ORIENTED_EDGE ( 'NONE', *, *, #30413, .F. ) ;
#21097=ORIENTED_EDGE ( 'NONE', *, *, #20630, .F. ) ;
#21099=CARTESIAN_POINT ( 'NONE',  ( 99.16631175631914630, -32.71502711089942039, 47.38444044875394923 ) ) ;
#21100=EDGE_CURVE ( 'NONE', #22667, #18476, #18515, .T. ) ;
#21103=AXIS2_PLACEMENT_3D ( 'NONE', #49227, #35156, #41964 ) ;
#21104=CARTESIAN_POINT ( 'NONE',  ( 109.2982854457139297, -26.60236246699155416, 175.8918157521009391 ) ) ;
#21108=ADVANCED_FACE ( 'NONE', ( #26050 ), #60093, .F. ) ;
#21109=AXIS2_PLACEMENT_3D ( 'NONE', #81084, #18835, #46517 ) ;
#21110=DIRECTION ( 'NONE',  ( 1.000000000000000000, 3.083952846180989689E-15, 1.541976423090494844E-15 ) ) ;
#21112=CARTESIAN_POINT ( 'NONE',  ( 95.80265872640100611, -40.33145541733363615, 131.5727681330539554 ) ) ;
#21114=ORIENTED_EDGE ( 'NONE', *, *, #4713, .T. ) ;
#21121=CARTESIAN_POINT ( 'NONE',  ( 102.4736563324128440, -43.47745920372498318, 194.9195189410199589 ) ) ;
#21122=CARTESIAN_POINT ( 'NONE',  ( 49.21213752016101495, -29.73316016639650172, -5.074374724088000832 ) ) ;
#21123=AXIS2_PLACEMENT_3D ( 'NONE', #41484, #70107, #49193 ) ;
#21124=DIRECTION ( 'NONE',  ( 1.000000000000000000, 2.999999999999999839E-15, 1.000000000000000078E-15 ) ) ;
#21126=VERTEX_POINT ( 'NONE', #52370 ) ;
#21128=CARTESIAN_POINT ( 'NONE',  ( 20.03715912545735378, -24.42818131006189830, 249.9678068554150059 ) ) ;
#21129=ORIENTED_EDGE ( 'NONE', *, *, #35470, .F. ) ;
#21130=VERTEX_POINT ( 'NONE', #4714 ) ;
#21131=CARTESIAN_POINT ( 'NONE',  ( 162.5667039024460223, -19.82844715994111340, 342.9256252759119548 ) ) ;
#21133=CARTESIAN_POINT ( 'NONE',  ( 114.5810018449060834, -31.08954144758037685, 260.7825356868496556 ) ) ;
#21134=CARTESIAN_POINT ( 'NONE',  ( 115.0893015243264443, -30.61815127115607638, 180.3443299114694582 ) ) ;
#21135=VERTEX_POINT ( 'NONE', #12419 ) ;
#21136=ADVANCED_FACE ( 'NONE', ( #33307 ), #53686, .F. ) ;
#21137=CARTESIAN_POINT ( 'NONE',  ( 131.3164832912739826, -18.72944715994100662, -5.074374724089004474 ) ) ;
#21142=CARTESIAN_POINT ( 'NONE',  ( 63.03715912545730760, -24.42818131006027826, 300.4678068554150627 ) ) ;
#21143=VECTOR ( 'NONE', #54271, 1000.000000000000000 ) ;
#21145=EDGE_LOOP ( 'NONE', ( #9357, #70152, #76040, #52596 ) ) ;
#21146=EDGE_CURVE ( 'NONE', #53629, #3324, #88558, .T. ) ;
#21147=CARTESIAN_POINT ( 'NONE',  ( 109.3549613941650875, -28.89410453886290142, 257.6680903695913685 ) ) ;
#21148=CARTESIAN_POINT ( 'NONE',  ( 117.2310933634200012, -39.29246586887208537, 123.6299109901969615 ) ) ;
#21149=CARTESIAN_POINT ( 'NONE',  ( 117.3423061886548879, -38.35306328171704848, 113.7013395616249767 ) ) ;
#21152=CARTESIAN_POINT ( 'NONE',  ( 112.2050260072902290, -45.80016191694880234, 208.9870538473389558 ) ) ;
#21153=CARTESIAN_POINT ( 'NONE',  ( 41.56670390244783420, -36.32844715994104234, 249.9678068554150343 ) ) ;
#21154=DIRECTION ( 'NONE',  ( 0.000000000000000000, 0.000000000000000000, -1.000000000000000000 ) ) ;
#21155=EDGE_LOOP ( 'NONE', ( #56642, #50261, #64458, #32963 ) ) ;
#21159=CARTESIAN_POINT ( 'NONE',  ( 41.56648329127399677, 0.2215528400590013880, 78.92562527591199739 ) ) ;
#21161=CARTESIAN_POINT ( 'NONE',  ( 97.07204692338113716, -35.37868373995705440, 137.2189094707525783 ) ) ;
#21163=AXIS2_PLACEMENT_3D ( 'NONE', #39957, #25893, #89016 ) ;
#21165=CARTESIAN_POINT ( 'NONE',  ( 102.0817216996469483, -27.57306688727539168, 145.4727681330539610 ) ) ;
#21167=AXIS2_PLACEMENT_3D ( 'NONE', #74609, #88707, #4683 ) ;
#21168=CARTESIAN_POINT ( 'NONE',  ( 130.5667039024480118, -35.47069715994093997, 218.8274735512161158 ) ) ;
#21169=CARTESIAN_POINT ( 'NONE',  ( 152.0371591254583450, -47.82818131005588214, 249.9678068554149490 ) ) ;
#21170=CARTESIAN_POINT ( 'NONE',  ( 125.0664832912740110, -18.82844715994099971, 284.9256252759119548 ) ) ;
#21172=CARTESIAN_POINT ( 'NONE',  ( 112.1942863616535817, -45.78120396183486918, 208.9870538473389558 ) ) ;
#21173=CARTESIAN_POINT ( 'NONE',  ( 138.0667039024480403, -58.72944715994091069, 239.5838068554170377 ) ) ;
#21175=ORIENTED_EDGE ( 'NONE', *, *, #40460, .T. ) ;
#21177=LINE ( 'NONE', #34791, #48340 ) ;
#21180=CARTESIAN_POINT ( 'NONE',  ( 141.0664832912739826, -8.729447159940995959, 14.67562527591100441 ) ) ;
#21181=CARTESIAN_POINT ( 'NONE',  ( 111.7588773036880383, -27.37059502548119028, 279.7070538473396937 ) ) ;
#21182=VERTEX_POINT ( 'NONE', #31958 ) ;
#21183=FACE_OUTER_BOUND ( 'NONE', #81932, .T. ) ;
#21184=CARTESIAN_POINT ( 'NONE',  ( 114.2686970495659295, -44.29742072815643184, 158.1813395616249807 ) ) ;
#21185=CARTESIAN_POINT ( 'NONE',  ( 100.5507766775973835, -27.80086676837388637, 26.56610146638793779 ) ) ;
#21186=CARTESIAN_POINT ( 'NONE',  ( 117.4696809092536256, -30.95150704042223211, 175.2299109901969700 ) ) ;
#21191=CARTESIAN_POINT ( 'NONE',  ( 193.0371591254584303, -47.82818131005411999, 249.9678068554149775 ) ) ;
#21192=CARTESIAN_POINT ( 'NONE',  ( 116.3212776292296127, -32.94146857471318413, 287.6356252759109680 ) ) ;
#21195=VECTOR ( 'NONE', #53548, 1000.000000000000000 ) ;
#21196=ORIENTED_EDGE ( 'NONE', *, *, #62757, .F. ) ;
#21197=ORIENTED_EDGE ( 'NONE', *, *, #42362, .F. ) ;
#21198=ADVANCED_FACE ( 'NONE', ( #46465 ), #46910, .T. ) ;
#21199=EDGE_LOOP ( 'NONE', ( #15903, #28115, #63679, #5551 ) ) ;
#21200=CARTESIAN_POINT ( 'NONE',  ( 117.2454586689011364, -38.87819698039182015, 59.66133956162595098 ) ) ;
#21204=CARTESIAN_POINT ( 'NONE',  ( 111.4354466870268539, -47.79847022207366081, 168.8756252759109486 ) ) ;
#21206=CARTESIAN_POINT ( 'NONE',  ( 105.0359719168109933, -28.43277227512634298, 284.6895626852196415 ) ) ;
#21207=AXIS2_PLACEMENT_3D ( 'NONE', #44900, #23162, #38101 ) ;
#21210=ORIENTED_EDGE ( 'NONE', *, *, #58909, .F. ) ;
#21211=CARTESIAN_POINT ( 'NONE',  ( 115.0372575077159212, -42.90846256501347966, 108.3022919427452138 ) ) ;
#21213=CARTESIAN_POINT ( 'NONE',  ( 108.4169788036852964, -26.73497112227234140, 160.9689992506304748 ) ) ;
#21215=DIRECTION ( 'NONE',  ( 1.000000000000000000, 4.163336342344333240E-14, 0.000000000000000000 ) ) ;
#21219=LINE ( 'NONE', #29383, #79695 ) ;
#21221=CARTESIAN_POINT ( 'NONE',  ( 112.1867106929447999, -26.95862322015887358, 14.68038718067299442 ) ) ;
#21222=FACE_OUTER_BOUND ( 'NONE', #42262, .T. ) ;
#21224=LINE ( 'NONE', #68476, #31588 ) ;
#21225=CIRCLE ( 'NONE', #16878, 1.000000000000000888 ) ;
#21227=CARTESIAN_POINT ( 'NONE',  ( 102.3683448235669715, -29.46113098739592928, 68.36332846482901004 ) ) ;
#21229=AXIS2_PLACEMENT_3D ( 'NONE', #5761, #12571, #68875 ) ;
#21230=AXIS2_PLACEMENT_3D ( 'NONE', #88594, #5469, #73603 ) ;
#21232=CARTESIAN_POINT ( 'NONE',  ( 80.06648329127399677, -8.729447159940999512, 306.1181252759120071 ) ) ;
#21233=VERTEX_POINT ( 'NONE', #53267 ) ;
#21234=EDGE_LOOP ( 'NONE', ( #7974, #48995, #26305, #29271 ) ) ;
#21235=DIRECTION ( 'NONE',  ( -1.000000000000000078E-15, -1.000000000000000083E-30, 1.000000000000000000 ) ) ;
#21237=EDGE_LOOP ( 'NONE', ( #55679, #72269, #83434, #21702 ) ) ;
#21238=CARTESIAN_POINT ( 'NONE',  ( 34.96670390244654669, -26.71338133339238041, 117.4678068554150485 ) ) ;
#21239=CARTESIAN_POINT ( 'NONE',  ( 100.2959224756171466, -44.18784923124425035, 153.4215833058969736 ) ) ;
#21240=DIRECTION ( 'NONE',  ( 1.000000000000000078E-15, -1.000000000000000000, 0.000000000000000000 ) ) ;
#21241=AXIS2_PLACEMENT_3D ( 'NONE', #60099, #73751, #73295 ) ;
#21242=CARTESIAN_POINT ( 'NONE',  ( 96.77023068570494502, -38.49705603518268049, 87.46133956162493917 ) ) ;
#21243=CARTESIAN_POINT ( 'NONE',  ( 188.5667039024479834, -62.87844715994099687, 134.4678068554150059 ) ) ;
#21245=CARTESIAN_POINT ( 'NONE',  ( 107.0667039024467613, -36.72944715994091780, 196.8538068554170195 ) ) ;
#21246=VERTEX_POINT ( 'NONE', #31502 ) ;
#21247=AXIS2_PLACEMENT_3D ( 'NONE', #66538, #87000, #59709 ) ;
#21248=ORIENTED_EDGE ( 'NONE', *, *, #27932, .F. ) ;
#21250=CARTESIAN_POINT ( 'NONE',  ( 72.26648329127297643, -1.929447159941394263, 352.4506252759079530 ) ) ;
#21252=CARTESIAN_POINT ( 'NONE',  ( 115.9938418408662244, -42.00591315737207054, 283.4137205140066271 ) ) ;
#21253=CARTESIAN_POINT ( 'NONE',  ( 96.58534993179142703, -36.88768535406505578, 132.3384824187679669 ) ) ;
#21256=CARTESIAN_POINT ( 'NONE',  ( 101.7108440984968212, -27.74398881808361850, 81.50419670448295051 ) ) ;
#21257=CARTESIAN_POINT ( 'NONE',  ( 107.0664832912750057, -36.72944715993903486, 9.425625275910970657 ) ) ;
#21258=VERTEX_POINT ( 'NONE', #25142 ) ;
#21259=CARTESIAN_POINT ( 'NONE',  ( 97.12564716885088956, -37.99759042466634895, 116.4282268054463145 ) ) ;
#21260=CARTESIAN_POINT ( 'NONE',  ( 97.81136857581559241, -40.51756142658395987, 157.6353372204761456 ) ) ;
#21265=CARTESIAN_POINT ( 'NONE',  ( 112.1975415602056216, -26.93795424888832812, 14.68038718067299442 ) ) ;
#21266=CARTESIAN_POINT ( 'NONE',  ( 70.14948329127297200, -71.52944715994141234, 352.4506252759078961 ) ) ;
#21268=PLANE ( 'NONE',  #28732 ) ;
#21269=CARTESIAN_POINT ( 'NONE',  ( 111.3857387752846790, -29.74709210828544670, 289.0581341137911409 ) ) ;
#21270=CARTESIAN_POINT ( 'NONE',  ( 115.0888706016519905, -30.61758542023168062, 109.3439634156283091 ) ) ;
#21271=CARTESIAN_POINT ( 'NONE',  ( 98.47430666977648173, -42.65725675464086919, 122.8070538473389490 ) ) ;
#21272=CARTESIAN_POINT ( 'NONE',  ( 104.4899544459507865, -26.97880758620100750, 71.28145860973472736 ) ) ;
#21273=CARTESIAN_POINT ( 'NONE',  ( 172.5664832912729878, -27.82844715994070484, 134.1756252759119832 ) ) ;
#21274=ORIENTED_EDGE ( 'NONE', *, *, #67160, .T. ) ;
#21275=DIRECTION ( 'NONE',  ( 0.7071067811865779928, -0.7071067811865171526, 7.071067811865785947E-16 ) ) ;
#21276=FACE_BOUND ( 'NONE', #23135, .T. ) ;
#21277=CARTESIAN_POINT ( 'NONE',  ( 46.83715912545339677, -47.82818131006086304, 180.4678068554150911 ) ) ;
#21279=EDGE_CURVE ( 'NONE', #50783, #8428, #68315, .T. ) ;
#21282=CARTESIAN_POINT ( 'NONE',  ( 103.7935660395325073, -26.78486678718983072, 165.3299109901969643 ) ) ;
#21283=ORIENTED_EDGE ( 'NONE', *, *, #66622, .T. ) ;
#21284=CARTESIAN_POINT ( 'NONE',  ( 63.03715912545735023, -24.42818131006027826, 249.9678068554150343 ) ) ;
#21285=CARTESIAN_POINT ( 'NONE',  ( 103.7162039098101332, -26.17194585468624624, 201.3089586092439731 ) ) ;
#21286=CARTESIAN_POINT ( 'NONE',  ( 98.61215933031529346, -43.92124142298762735, 72.89943479972099283 ) ) ;
#21289=CARTESIAN_POINT ( 'NONE',  ( 62.56670390244747892, -48.82844715994099971, 300.4678068554150627 ) ) ;
#21293=AXIS2_PLACEMENT_3D ( 'NONE', #86811, #58203, #64577 ) ;
#21294=EDGE_CURVE ( 'NONE', #19859, #51458, #66026, .T. ) ;
#21295=ORIENTED_EDGE ( 'NONE', *, *, #54603, .T. ) ;
#21296=ORIENTED_EDGE ( 'NONE', *, *, #67431, .F. ) ;
#21299=CARTESIAN_POINT ( 'NONE',  ( 114.6054725695487946, -29.52902160936550047, 230.4327681330539690 ) ) ;
#21301=LINE ( 'NONE', #38490, #86143 ) ;
#21303=DIRECTION ( 'NONE',  ( 0.000000000000000000, 0.000000000000000000, 1.000000000000000000 ) ) ;
#21306=AXIS2_PLACEMENT_3D ( 'NONE', #61344, #26831, #69528 ) ;
#21307=CARTESIAN_POINT ( 'NONE',  ( 106.6058666599951152, -25.66223100340348040, 40.09753003781596448 ) ) ;
#21309=ORIENTED_EDGE ( 'NONE', *, *, #71238, .F. ) ;
#21311=CARTESIAN_POINT ( 'NONE',  ( 57.56670390244819657, -48.82844715994039575, 259.7178068554150627 ) ) ;
#21313=CARTESIAN_POINT ( 'NONE',  ( 110.5064767540468011, -26.94654216138288660, 250.8194347997200850 ) ) ;
#21314=CARTESIAN_POINT ( 'NONE',  ( 61.56670390244727287, -23.42844715994043980, 300.4678068554150627 ) ) ;
#21315=EDGE_CURVE ( 'NONE', #37451, #88467, #14211, .T. ) ;
#21316=CARTESIAN_POINT ( 'NONE',  ( 97.87212830949614784, -31.93334231290201330, 86.93181575210095957 ) ) ;
#21318=EDGE_CURVE ( 'NONE', #36953, #21752, #55508, .T. ) ;
#21321=VERTEX_POINT ( 'NONE', #41889 ) ;
#21324=VERTEX_POINT ( 'NONE', #56420 ) ;
#21325=EDGE_LOOP ( 'NONE', ( #54742, #51933, #87938, #63322 ) ) ;
#21327=CARTESIAN_POINT ( 'NONE',  ( 110.1832024441707460, -27.86589328696400969, 251.2511071154212061 ) ) ;
#21328=VECTOR ( 'NONE', #5880, 1000.000000000000000 ) ;
#21329=CARTESIAN_POINT ( 'NONE',  ( 117.0718954873599671, -35.46248236694560063, 193.9272919417280718 ) ) ;
#21331=B_SPLINE_CURVE_WITH_KNOTS ( 'NONE', 3,
 ( #6534, #14253, #19275, #41928, #34229, #33791, #61934, #21063, #48737, #89667, #26982, #26530, #67865, #27417, #55099, #54202, #81964, #75128 ),
 .UNSPECIFIED., .F., .F.,
 ( 4, 2, 2, 2, 2, 2, 2, 2, 4 ),
 ( 0.000000000000000000, 0.06248810027333082107, 0.1249762005466616421, 0.1874643008199924632, 0.2499524010933232843, 0.3124405013666541331, 0.3749286016399849264, 0.4374167019133153866, 0.4999048021866459024 ),
 .UNSPECIFIED. ) ;
#21335=DIRECTION ( 'NONE',  ( 0.000000000000000000, 1.000000000000000000, 0.000000000000000000 ) ) ;
#21336=DIRECTION ( 'NONE',  ( 3.309108161477000101E-13, -1.000000000000000000, 4.100000000000000342E-29 ) ) ;
#21338=CARTESIAN_POINT ( 'NONE',  ( 99.98060178585627966, -44.37649324013435859, 46.98133956162592284 ) ) ;
#21340=CARTESIAN_POINT ( 'NONE',  ( 98.28161005395152472, -38.92874716189901818, 15.95622935188595370 ) ) ;
#21341=DIRECTION ( 'NONE',  ( 0.000000000000000000, 0.000000000000000000, -1.000000000000000000 ) ) ;
#21342=CARTESIAN_POINT ( 'NONE',  ( 98.80555182512723889, -41.96590078842033478, 186.7756252759109543 ) ) ;
#21343=CARTESIAN_POINT ( 'NONE',  ( 57.56670390244829605, -48.82844715994039575, 293.2178068554150627 ) ) ;
#21344=CARTESIAN_POINT ( 'NONE',  ( 172.5664832912740110, -9.303447159940999356, 81.04262527591200183 ) ) ;
#21345=DIRECTION ( 'NONE',  ( 4.299999999999999979E-14, -1.000000000000000000, 0.000000000000000000 ) ) ;
#21346=AXIS2_PLACEMENT_3D ( 'NONE', #38622, #81335, #25896 ) ;
#21348=CARTESIAN_POINT ( 'NONE',  ( 118.5948618896802742, -33.89272371608580414, 10.01848241876795953 ) ) ;
#21350=ORIENTED_EDGE ( 'NONE', *, *, #75910, .F. ) ;
#21352=AXIS2_PLACEMENT_3D ( 'NONE', #32786, #5999, #69109 ) ;
#21353=ORIENTED_EDGE ( 'NONE', *, *, #67419, .F. ) ;
#21354=CARTESIAN_POINT ( 'NONE',  ( 96.59565658895887452, -37.56598942197172164, 97.38991099019594344 ) ) ;
#21356=DIRECTION ( 'NONE',  ( -2.900000000000000265E-14, 2.000000000000000155E-15, -1.000000000000000000 ) ) ;
#21357=AXIS2_PLACEMENT_3D ( 'NONE', #51485, #16994, #44675 ) ;
#21358=VERTEX_POINT ( 'NONE', #21477 ) ;
#21359=CARTESIAN_POINT ( 'NONE',  ( 76.31670390244799762, -50.82844715994100682, 198.9178068554149945 ) ) ;
#21361=ORIENTED_EDGE ( 'NONE', *, *, #88171, .T. ) ;
#21362=CARTESIAN_POINT ( 'NONE',  ( 97.95250717983365973, -32.49412669507731266, 25.56312527591095929 ) ) ;
#21364=CYLINDRICAL_SURFACE ( 'NONE', #84919, 0.5000000000000073275 ) ;
#21366=DIRECTION ( 'NONE',  ( 1.000000000000000000, 4.163336342344333240E-14, 0.000000000000000000 ) ) ;
#21367=CARTESIAN_POINT ( 'NONE',  ( 108.5374814027631203, -28.67222352762033211, 162.7509475124489597 ) ) ;
#21368=CARTESIAN_POINT ( 'NONE',  ( 116.2377588530493995, -41.80555791324388082, 259.4241967044827106 ) ) ;
#21372=AXIS2_PLACEMENT_3D ( 'NONE', #46987, #33383, #27462 ) ;
#21375=ORIENTED_EDGE ( 'NONE', *, *, #72949, .T. ) ;
#21378=DIRECTION ( 'NONE',  ( 1.000000000000000078E-15, -1.000000000000000083E-30, -1.000000000000000000 ) ) ;
#21379=EDGE_CURVE ( 'NONE', #3248, #67028, #84164, .T. ) ;
#21380=DIRECTION ( 'NONE',  ( -0.4808135048159887792, -0.02029144519433677407, 0.8765880622267739897 ) ) ;
#21381=CARTESIAN_POINT ( 'NONE',  ( 112.1393234202593590, -28.01280907429307732, 14.65646064512042912 ) ) ;
#21382=ADVANCED_FACE ( 'NONE', ( #76886, #55963 ), #75089, .T. ) ;
#21384=DIRECTION ( 'NONE',  ( 0.7071067811865514585, -0.7071067811865435759, 7.071067811865211065E-16 ) ) ;
#21385=CARTESIAN_POINT ( 'NONE',  ( 113.5990078486005217, -30.45738264864434441, 188.8457531614099594 ) ) ;
#21386=CARTESIAN_POINT ( 'NONE',  ( 117.0169231590003562, -33.47438763928646210, 89.07848241876791917 ) ) ;
#21389=ORIENTED_EDGE ( 'NONE', *, *, #36573, .F. ) ;
#21392=EDGE_LOOP ( 'NONE', ( #8614, #12946, #73187, #67248 ) ) ;
#21393=ADVANCED_FACE ( 'NONE', ( #1030 ), #54612, .T. ) ;
#21396=ORIENTED_EDGE ( 'NONE', *, *, #73574, .T. ) ;
#21399=DIRECTION ( 'NONE',  ( 0.7071067811865779928, -0.7071067811865171526, 7.071067811865785947E-16 ) ) ;
#21400=VECTOR ( 'NONE', #38821, 1000.000000000000000 ) ;
#21402=FACE_OUTER_BOUND ( 'NONE', #54082, .T. ) ;
#21404=CARTESIAN_POINT ( 'NONE',  ( 96.15435578470099642, -38.63231720721949358, 46.45181575210094138 ) ) ;
#21407=PLANE ( 'NONE',  #20239 ) ;
#21408=PLANE ( 'NONE',  #47137 ) ;
#21410=CARTESIAN_POINT ( 'NONE',  ( 131.3165191078497855, -18.55813574389560117, 3.101427645695946644 ) ) ;
#21411=ORIENTED_EDGE ( 'NONE', *, *, #20811, .T. ) ;
#21413=CARTESIAN_POINT ( 'NONE',  ( 116.3199495083284347, -32.94194616109231077, 85.13562527591095375 ) ) ;
#21414=ADVANCED_FACE ( 'NONE', ( #89628 ), #27383, .T. ) ;
#21416=FACE_OUTER_BOUND ( 'NONE', #5727, .T. ) ;
#21417=CARTESIAN_POINT ( 'NONE',  ( 116.9423613927432939, -33.21572726007214271, 110.0984824187679578 ) ) ;
#21418=AXIS2_PLACEMENT_3D ( 'NONE', #83617, #75456, #5973 ) ;
#21420=DIRECTION ( 'NONE',  ( 0.000000000000000000, 0.000000000000000000, 1.000000000000000000 ) ) ;
#21421=CARTESIAN_POINT ( 'NONE',  ( 182.2738106836199563, -23.19206098993945275, 342.9256252759109884 ) ) ;
#21426=CARTESIAN_POINT ( 'NONE',  ( 109.0694692412632207, -27.15596902575785876, 135.9127681330529640 ) ) ;
#21428=EDGE_LOOP ( 'NONE', ( #64290, #3278, #68899, #23075 ) ) ;
#21429=VECTOR ( 'NONE', #55701, 1000.000000000000000 ) ;
#21430=CARTESIAN_POINT ( 'NONE',  ( 110.7254274611715630, -26.32387412717039155, 250.8194347997206819 ) ) ;
#21431=CARTESIAN_POINT ( 'NONE',  ( 107.0664832912739683, -23.41197657318947378, 305.7008218191032256 ) ) ;
#21433=DIRECTION ( 'NONE',  ( 0.9068632946707805287, -0.4214249218767882610, 8.630465054610985966E-16 ) ) ;
#21435=ADVANCED_FACE ( 'NONE', ( #13758 ), #41443, .T. ) ;
#21437=CARTESIAN_POINT ( 'NONE',  ( 46.83715912545424231, -47.82818131006082751, 300.4678068554150059 ) ) ;
#21439=VECTOR ( 'NONE', #73717, 1000.000000000000000 ) ;
#21442=CARTESIAN_POINT ( 'NONE',  ( 103.7602102885707183, -27.48919103108766748, 190.3499109901969746 ) ) ;
#21444=ORIENTED_EDGE ( 'NONE', *, *, #86284, .F. ) ;
#21445=CARTESIAN_POINT ( 'NONE',  ( 99.18485448662231363, -41.84413841198986006, 143.2282499725629634 ) ) ;
#21447=DIRECTION ( 'NONE',  ( -1.000000000000000078E-15, 1.000000000000000083E-30, 1.000000000000000000 ) ) ;
#21448=CARTESIAN_POINT ( 'NONE',  ( 97.21282778982880757, -39.96427141005798234, 282.5908633711484867 ) ) ;
#21449=LINE ( 'NONE', #89594, #30412 ) ;
#21450=CARTESIAN_POINT ( 'NONE',  ( 116.7948070112746422, -39.38896383652134858, 268.6149319580774204 ) ) ;
#21451=CARTESIAN_POINT ( 'NONE',  ( 162.5667039024486087, -33.35206098992175328, 237.4678068554150059 ) ) ;
#21453=LINE ( 'NONE', #7812, #40070 ) ;
#21454=CARTESIAN_POINT ( 'NONE',  ( 106.8520627977276831, -47.75749532952668375, 227.5489586092439538 ) ) ;
#21455=CARTESIAN_POINT ( 'NONE',  ( 97.07197674641710705, -35.37901635621462759, 171.2185788321773430 ) ) ;
#21457=VERTEX_POINT ( 'NONE', #42781 ) ;
#21460=CARTESIAN_POINT ( 'NONE',  ( 104.4083715469849523, -46.45818331703511461, 123.3633132816207336 ) ) ;
#21462=AXIS2_PLACEMENT_3D ( 'NONE', #72837, #2911, #72405 ) ;
#21464=DIRECTION ( 'NONE',  ( 0.000000000000000000, 1.000000000000000000, 0.000000000000000000 ) ) ;
#21465=ORIENTED_EDGE ( 'NONE', *, *, #53865, .F. ) ;
#21466=CARTESIAN_POINT ( 'NONE',  ( 100.4377198651835101, -44.85950937921091253, 8.032768133053981074 ) ) ;
#21467=CARTESIAN_POINT ( 'NONE',  ( 113.7993967570077700, -26.97709554098909024, 239.5956252759109759 ) ) ;
#21468=ORIENTED_EDGE ( 'NONE', *, *, #21318, .F. ) ;
#21469=LINE ( 'NONE', #63247, #7160 ) ;
#21470=DIRECTION ( 'NONE',  ( 0.000000000000000000, 0.000000000000000000, -1.000000000000000000 ) ) ;
#21472=CARTESIAN_POINT ( 'NONE',  ( 100.4295600883690014, -42.28392062234677695, 69.68713798863895192 ) ) ;
#21473=CARTESIAN_POINT ( 'NONE',  ( 102.9585648456520772, -26.44303807861259870, 171.3908633711489813 ) ) ;
#21474=LINE ( 'NONE', #1483, #63829 ) ;
#21477=CARTESIAN_POINT ( 'NONE',  ( 41.56648329127381203, -18.82844715994071194, 21.92562527591192989 ) ) ;
#21478=ORIENTED_EDGE ( 'NONE', *, *, #52911, .T. ) ;
#21479=ORIENTED_EDGE ( 'NONE', *, *, #53371, .T. ) ;
#21480=CIRCLE ( 'NONE', #15727, 0.5000000000000004441 ) ;
#21481=AXIS2_PLACEMENT_3D ( 'NONE', #52635, #87646, #80396 ) ;
#21483=EDGE_LOOP ( 'NONE', ( #89236, #31328, #21248, #29244 ) ) ;
#21484=ORIENTED_EDGE ( 'NONE', *, *, #77422, .T. ) ;
#21485=FACE_BOUND ( 'NONE', #73555, .T. ) ;
#21486=EDGE_CURVE ( 'NONE', #12604, #8963, #55255, .T. ) ;
#21488=CARTESIAN_POINT ( 'NONE',  ( 105.8382827194499640, -25.33631814701313445, 322.1960590088103800 ) ) ;
#21489=CARTESIAN_POINT ( 'NONE',  ( 115.4947688602672997, -38.28382951093581710, 88.10384839950596358 ) ) ;
#21490=CARTESIAN_POINT ( 'NONE',  ( 104.3185787381473375, -25.99890841748068482, 245.2880062282919482 ) ) ;
#21493=CARTESIAN_POINT ( 'NONE',  ( 116.7748712849171966, -40.56502120445013304, 193.5270538473389479 ) ) ;
#21494=PLANE ( 'NONE',  #7844 ) ;
#21497=ADVANCED_FACE ( 'NONE', ( #9632 ), #21937, .F. ) ;
#21500=AXIS2_PLACEMENT_3D ( 'NONE', #81780, #27241, #48111 ) ;
#21505=CARTESIAN_POINT ( 'NONE',  ( 112.9285164932676224, -28.85859325239445994, 104.5670538473399347 ) ) ;
#21506=CARTESIAN_POINT ( 'NONE',  ( 113.4866449958868770, -46.74994221786862880, 68.02991099019695298 ) ) ;
#21507=CARTESIAN_POINT ( 'NONE',  ( 99.34894212307516170, -29.65511154620466172, 275.7356252759109907 ) ) ;
#21510=CARTESIAN_POINT ( 'NONE',  ( 117.4129020423329450, -35.18752443080737891, 218.9441967044829482 ) ) ;
#21514=CARTESIAN_POINT ( 'NONE',  ( 107.8430805769216931, -46.60421432495259353, 277.6356252759110816 ) ) ;
#21516=CARTESIAN_POINT ( 'NONE',  ( 105.3684880140626063, -25.39599743441489821, 321.1394118018684480 ) ) ;
#21519=DIRECTION ( 'NONE',  ( 1.000000000000000000, 4.299999999999999979E-14, 1.000000000000000078E-15 ) ) ;
#21520=AXIS2_PLACEMENT_3D ( 'NONE', #79482, #38558, #87614 ) ;
#21522=CARTESIAN_POINT ( 'NONE',  ( 102.0670549276872521, -27.97049807736920002, 11.48979194543367477 ) ) ;
#21523=LINE ( 'NONE', #1969, #4241 ) ;
#21524=EDGE_CURVE ( 'NONE', #3733, #16260, #5949, .T. ) ;
#21525=CARTESIAN_POINT ( 'NONE',  ( 41.56648329127499153, -32.07844715994070839, 318.9256252759120116 ) ) ;
#21526=ORIENTED_EDGE ( 'NONE', *, *, #65389, .T. ) ;
#21528=CARTESIAN_POINT ( 'NONE',  ( 96.24499046374883449, -34.36497383161641039, 256.1432443235299843 ) ) ;
#21529=CARTESIAN_POINT ( 'NONE',  ( 114.4628154322623033, -28.51554874119783634, 155.5051490854349652 ) ) ;
#21530=CARTESIAN_POINT ( 'NONE',  ( 99.12701999692106369, -43.51930588094383978, 27.88991099019694175 ) ) ;
#21531=CARTESIAN_POINT ( 'NONE',  ( 179.4595971212889935, -28.98061976758940617, -5.074374724088000832 ) ) ;
#21532=AXIS2_PLACEMENT_3D ( 'NONE', #75859, #13631, #14539 ) ;
#21535=DIRECTION ( 'NONE',  ( -0.7071067811865779928, 0.7071067811865171526, -7.071067811865786933E-16 ) ) ;
#21538=ORIENTED_EDGE ( 'NONE', *, *, #36979, .T. ) ;
#21539=CARTESIAN_POINT ( 'NONE',  ( 112.4313655287739948, -30.08308194412713021, 163.9581341137909476 ) ) ;
#21540=DIRECTION ( 'NONE',  ( 1.000000000000000000, 4.163336342344333240E-14, 0.000000000000000000 ) ) ;
#21542=DIRECTION ( 'NONE',  ( 0.7071067809773443624, -0.7071067813957507830, 7.071067809773451711E-16 ) ) ;
#21543=CARTESIAN_POINT ( 'NONE',  ( 102.9757002774702102, -26.48594595611790581, 171.3908633711489813 ) ) ;
#21544=CARTESIAN_POINT ( 'NONE',  ( 165.3359832912750278, -36.32844715993530826, 180.4678068554150059 ) ) ;
#21546=CARTESIAN_POINT ( 'NONE',  ( 97.07253791766775919, -35.37391747781727247, 87.21837571989119908 ) ) ;
#21548=LINE ( 'NONE', #36059, #78149 ) ;
#21549=CARTESIAN_POINT ( 'NONE',  ( 41.56670390244783420, -36.32844715994104234, 249.9678068554150343 ) ) ;
#21550=ADVANCED_FACE ( 'NONE', ( #50958 ), #2828, .F. ) ;
#21551=CARTESIAN_POINT ( 'NONE',  ( 104.2906771502715628, -46.10805769451172864, 107.3470538473399500 ) ) ;
#21555=CARTESIAN_POINT ( 'NONE',  ( 111.9552019894765493, -28.70592206014574543, 46.06063092494500211 ) ) ;
#21556=CIRCLE ( 'NONE', #22217, 0.5000000000000004441 ) ;
#21558=CARTESIAN_POINT ( 'NONE',  ( 117.2610056464982904, -34.82931580038573571, 199.9851490854349549 ) ) ;
#21559=CARTESIAN_POINT ( 'NONE',  ( 112.0659116737735559, -45.48839623049394731, 37.98979194726469188 ) ) ;
#21560=CARTESIAN_POINT ( 'NONE',  ( 97.33793862645453032, -34.07069176642836794, 56.11362873108982541 ) ) ;
#21561=CARTESIAN_POINT ( 'NONE',  ( 80.06648329127399677, -8.350947159940998787, 7.443125275912000127 ) ) ;
#21563=VECTOR ( 'NONE', #23389, 1000.000000000000000 ) ;
#21564=DIRECTION ( 'NONE',  ( 0.000000000000000000, 0.000000000000000000, 1.000000000000000000 ) ) ;
#21566=CARTESIAN_POINT ( 'NONE',  ( 102.3226935662337098, -26.77152163616654335, 140.4422919425769578 ) ) ;
#21567=VERTEX_POINT ( 'NONE', #35993 ) ;
#21571=ADVANCED_FACE ( 'NONE', ( #70982 ), #8753, .F. ) ;
#21574=VECTOR ( 'NONE', #79503, 1000.000000000000000 ) ;
#21575=CARTESIAN_POINT ( 'NONE',  ( 188.5667039024479834, -48.82844715994099971, 257.2178068554150059 ) ) ;
#21576=DIRECTION ( 'NONE',  ( 0.9068632946707755327, -0.4214249218767993077, 0.000000000000000000 ) ) ;
#21577=CARTESIAN_POINT ( 'NONE',  ( 106.6101046285737510, -27.46188816740816918, 192.9338046553059485 ) ) ;
#21578=ADVANCED_FACE ( 'NONE', ( #36453 ), #49607, .T. ) ;
#21579=CARTESIAN_POINT ( 'NONE',  ( 107.0664832912739399, -36.72944715994095333, 247.7440089327910755 ) ) ;
#21580=DIRECTION ( 'NONE',  ( -1.000000000000000000, 9.376883653928684652E-16, 1.500301384628589584E-15 ) ) ;
#21581=ORIENTED_EDGE ( 'NONE', *, *, #7156, .T. ) ;
#21582=ORIENTED_EDGE ( 'NONE', *, *, #6781, .T. ) ;
#21586=ORIENTED_EDGE ( 'NONE', *, *, #10521, .F. ) ;
#21587=ORIENTED_EDGE ( 'NONE', *, *, #77656, .T. ) ;
#21588=CARTESIAN_POINT ( 'NONE',  ( 82.81648329127398256, -18.72944715994105636, 3.101481641215461327 ) ) ;
#21589=B_SPLINE_CURVE_WITH_KNOTS ( 'NONE', 3,
 ( #3413, #17488, #45168, #3856, #52409, #13357, #54649, #33792, #60588, #20619, #4750, #12017, #89218, #75130, #26531, #26983, #34230, #32433 ),
 .UNSPECIFIED., .F., .F.,
 ( 4, 2, 2, 2, 2, 2, 2, 2, 4 ),
 ( 0.5000000003264866155, 0.5625000002856758163, 0.6250000002448650172, 0.6875000002040541069, 0.7500000001632433078, 0.8125000001224325086, 0.8750000000816215984, 0.9375000000408107992, 1.000000000000000000 ),
 .UNSPECIFIED. ) ;
#21590=CARTESIAN_POINT ( 'NONE',  ( 113.4748355983601300, -30.60888351595189860, 230.8644404487539816 ) ) ;
#21591=CARTESIAN_POINT ( 'NONE',  ( 115.8257729668916909, -31.73060787271685257, 180.2401568395068807 ) ) ;
#21592=ORIENTED_EDGE ( 'NONE', *, *, #62872, .F. ) ;
#21593=PLANE ( 'NONE',  #5884 ) ;
#21594=AXIS2_PLACEMENT_3D ( 'NONE', #5803, #62093, #13505 ) ;
#21596=ORIENTED_EDGE ( 'NONE', *, *, #35027, .F. ) ;
#21597=VERTEX_POINT ( 'NONE', #29188 ) ;
#21598=CARTESIAN_POINT ( 'NONE',  ( 172.5664832912729878, -27.82844715994070484, 135.9256252759119832 ) ) ;
#21600=ORIENTED_EDGE ( 'NONE', *, *, #29310, .F. ) ;
#21601=EDGE_CURVE ( 'NONE', #80351, #84792, #50508, .T. ) ;
#21602=EDGE_CURVE ( 'NONE', #62736, #32451, #89665, .T. ) ;
#21603=CARTESIAN_POINT ( 'NONE',  ( 113.3211896355758057, -31.48460449655562954, 267.1995189410199600 ) ) ;
#21604=CARTESIAN_POINT ( 'NONE',  ( 114.0958560388892380, -44.50609692678638396, 133.1613395616249989 ) ) ;
#21605=EDGE_CURVE ( 'NONE', #60711, #57212, #44129, .T. ) ;
#21606=CARTESIAN_POINT ( 'NONE',  ( 95.51222647996974047, -34.21005103128000968, 106.1556252759109640 ) ) ;
#21608=FILL_AREA_STYLE ('',( #14794 ) ) ;
#21609=CARTESIAN_POINT ( 'NONE',  ( 117.3348620442827865, -34.92864588493001321, 239.9641967044819637 ) ) ;
#21611=DIRECTION ( 'NONE',  ( 0.7071067811865969777, -0.7071067811864980568, 0.000000000000000000 ) ) ;
#21612=ORIENTED_EDGE ( 'NONE', *, *, #20529, .T. ) ;
#21613=DIRECTION ( 'NONE',  ( 0.000000000000000000, 0.000000000000000000, -1.000000000000000000 ) ) ;
#21614=VERTEX_POINT ( 'NONE', #71866 ) ;
#21616=ADVANCED_FACE ( 'NONE', ( #72312 ), #10085, .T. ) ;
#21619=CARTESIAN_POINT ( 'NONE',  ( 97.31303194613644791, -38.96042662333031359, 137.5053956884336230 ) ) ;
#21620=AXIS2_PLACEMENT_3D ( 'NONE', #48682, #41868, #84144 ) ;
#21621=EDGE_CURVE ( 'NONE', #45509, #40542, #20084, .T. ) ;
#21622=ORIENTED_EDGE ( 'NONE', *, *, #1227, .T. ) ;
#21623=CARTESIAN_POINT ( 'NONE',  ( 97.83587340921722841, -31.88353427759474457, 135.9413395616259947 ) ) ;
#21624=CARTESIAN_POINT ( 'NONE',  ( 36.65249034007441509, -48.32844715994130524, 180.4678068554150911 ) ) ;
#21626=CARTESIAN_POINT ( 'NONE',  ( 57.56670390244718760, -42.82844715994040996, 173.2178068554150911 ) ) ;
#21627=PLANE ( 'NONE',  #15773 ) ;
#21628=DIRECTION ( 'NONE',  ( 0.000000000000000000, 0.000000000000000000, 1.000000000000000000 ) ) ;
#21629=CARTESIAN_POINT ( 'NONE',  ( 112.4430884738663394, -45.67687932769430859, 234.0070538473389377 ) ) ;
#21633=ORIENTED_EDGE ( 'NONE', *, *, #80162, .T. ) ;
#21636=DIRECTION ( 'NONE',  ( 0.000000000000000000, 0.000000000000000000, -1.000000000000000000 ) ) ;
#21637=CARTESIAN_POINT ( 'NONE',  ( 112.1393456349457551, -28.01282277704235568, 255.6564586098648988 ) ) ;
#21639=DIRECTION ( 'NONE',  ( -4.237773401492740281E-14, 1.000000000000000000, 0.000000000000000000 ) ) ;
#21640=CARTESIAN_POINT ( 'NONE',  ( 172.5664832912740110, 0.2215528400590013880, 141.0426252759120018 ) ) ;
#21641=ORIENTED_EDGE ( 'NONE', *, *, #1436, .T. ) ;
#21642=DIRECTION ( 'NONE',  ( 1.000000000000000000, 2.999999999999999839E-15, 1.000000000000000078E-15 ) ) ;
#21643=CARTESIAN_POINT ( 'NONE',  ( 95.28658997325378266, -38.28252189325972665, 151.4299109901969871 ) ) ;
#21644=CARTESIAN_POINT ( 'NONE',  ( 101.3842069476886394, -27.98906827703155642, 21.53562527591096298 ) ) ;
#21645=CARTESIAN_POINT ( 'NONE',  ( 97.36167283409557172, -40.65495779399346077, 202.6327681330539860 ) ) ;
#21648=CARTESIAN_POINT ( 'NONE',  ( 83.06670390244796920, -61.87844715994100397, 231.5838068554150198 ) ) ;
#21649=DIRECTION ( 'NONE',  ( 0.000000000000000000, 1.000000000000000000, 0.000000000000000000 ) ) ;
#21651=DIRECTION ( 'NONE',  ( 4.194175870806139918E-14, -1.000000000000000000, 0.000000000000000000 ) ) ;
#21652=CARTESIAN_POINT ( 'NONE',  ( 83.06670390244796920, -61.87844715994100397, 228.3338068554150198 ) ) ;
#21654=DIRECTION ( 'NONE',  ( 1.000000000000000078E-15, -1.000000000000000083E-30, -1.000000000000000000 ) ) ;
#21657=AXIS2_PLACEMENT_3D ( 'NONE', #81278, #12217, #25388 ) ;
#21660=CARTESIAN_POINT ( 'NONE',  ( 111.9186950350129877, -27.52701776748444473, 55.68991099019693536 ) ) ;
#21661=DIRECTION ( 'NONE',  ( -1.000000000000000078E-15, 1.000000000000000083E-30, 1.000000000000000000 ) ) ;
#21662=DIRECTION ( 'NONE',  ( 1.000000000000000078E-15, -1.000000000000000083E-30, -1.000000000000000000 ) ) ;
#21663=CARTESIAN_POINT ( 'NONE',  ( 106.9746138897780696, -47.19771061482636298, 183.5699109901969734 ) ) ;
#21664=CARTESIAN_POINT ( 'NONE',  ( 101.4801710200817126, -30.26808144278882651, 260.0667055423624561 ) ) ;
#21667=ORIENTED_EDGE ( 'NONE', *, *, #58002, .T. ) ;
#21670=DIRECTION ( 'NONE',  ( 0.000000000000000000, 0.000000000000000000, -1.000000000000000000 ) ) ;
#21671=DIRECTION ( 'NONE',  ( 6.831565154159360295E-14, -1.000000000000000000, 0.000000000000000000 ) ) ;
#21672=CARTESIAN_POINT ( 'NONE',  ( 115.8250614324014549, -31.72937732619463702, 160.2398503699754144 ) ) ;
#21673=CARTESIAN_POINT ( 'NONE',  ( 104.4899544453328559, -26.97880758635668030, 75.28145860978439430 ) ) ;
#21677=CYLINDRICAL_SURFACE ( 'NONE', #82613, 5.599999999999994316 ) ;
#21678=CARTESIAN_POINT ( 'NONE',  ( 112.1067112481348858, -26.91823048478329738, 19.71086337114896736 ) ) ;
#21680=VERTEX_POINT ( 'NONE', #60444 ) ;
#21681=CIRCLE ( 'NONE', #10059, 5.800000000000000711 ) ;
#21682=CARTESIAN_POINT ( 'NONE',  ( 113.2454988854073576, -28.75867309995891574, 269.5522919233096104 ) ) ;
#21683=DIRECTION ( 'NONE',  ( -0.000000000000000000, -0.000000000000000000, -1.000000000000000000 ) ) ;
#21684=CARTESIAN_POINT ( 'NONE',  ( 112.9396172237807860, -42.43812354398048114, 96.03094751244795191 ) ) ;
#21685=VECTOR ( 'NONE', #26728, 1000.000000000000000 ) ;
#21688=LINE ( 'NONE', #62104, #49930 ) ;
#21692=VECTOR ( 'NONE', #50693, 1000.000000000000000 ) ;
#21693=FACE_OUTER_BOUND ( 'NONE', #40232, .T. ) ;
#21694=ORIENTED_EDGE ( 'NONE', *, *, #50225, .T. ) ;
#21695=EDGE_LOOP ( 'NONE', ( #46912, #87206, #32661, #33172, #82373, #5269, #22490, #89749 ) ) ;
#21696=COLOUR_RGB ( '', 0.09019608, 0.27058824, 0.51372549) ;
#21697=CARTESIAN_POINT ( 'NONE',  ( 112.8270896756726671, -29.95615083465972006, 135.9472975916109476 ) ) ;
#21699=CIRCLE ( 'NONE', #28901, 10.00000000000000888 ) ;
#21700=CARTESIAN_POINT ( 'NONE',  ( 109.6893229801689813, -47.49076295823797267, 83.75467289495897205 ) ) ;
#21702=ORIENTED_EDGE ( 'NONE', *, *, #46278, .T. ) ;
#21703=VERTEX_POINT ( 'NONE', #59988 ) ;
#21704=ORIENTED_EDGE ( 'NONE', *, *, #59724, .F. ) ;
#21705=ADVANCED_FACE ( 'NONE', ( #4606 ), #25946, .F. ) ;
#21706=AXIS2_PLACEMENT_3D ( 'NONE', #87077, #24843, #18017 ) ;
#21708=ORIENTED_EDGE ( 'NONE', *, *, #2040, .F. ) ;
#21710=CARTESIAN_POINT ( 'NONE',  ( 96.71096103112829212, -32.93116260832594122, 21.03467289495897319 ) ) ;
#21711=CARTESIAN_POINT ( 'NONE',  ( 109.8617963350518920, -26.66349048206837580, 170.8613395616249591 ) ) ;
#21715=CARTESIAN_POINT ( 'NONE',  ( 102.3023240427231570, -27.41686860022338124, 116.4527681330539650 ) ) ;
#21720=CARTESIAN_POINT ( 'NONE',  ( 112.0665211874434988, -45.48806074044107106, 133.9910299359918895 ) ) ;
#21723=LINE ( 'NONE', #63033, #53289 ) ;
#21725=CARTESIAN_POINT ( 'NONE',  ( 96.65879732087768161, -33.00665786158104709, 26.06514908543494613 ) ) ;
#21728=DIRECTION ( 'NONE',  ( 0.000000000000000000, 1.000000000000000000, 0.000000000000000000 ) ) ;
#21729=CARTESIAN_POINT ( 'NONE',  ( 97.00695627739551696, -39.24785929248557892, 16.53372051400697629 ) ) ;
#21730=CARTESIAN_POINT ( 'NONE',  ( 97.81145390679880336, -40.51685147915726048, 111.6355755005379962 ) ) ;
#21731=CARTESIAN_POINT ( 'NONE',  ( 116.7751801856527152, -32.99181816784840748, 135.1184824187679396 ) ) ;
#21733=FACE_OUTER_BOUND ( 'NONE', #86851, .T. ) ;
#21734=EDGE_CURVE ( 'NONE', #67541, #976, #88188, .T. ) ;
#21735=ORIENTED_EDGE ( 'NONE', *, *, #26965, .T. ) ;
#21737=AXIS2_PLACEMENT_3D ( 'NONE', #65115, #2898, #51465 ) ;
#21739=EDGE_CURVE ( 'NONE', #25932, #72034, #10786, .T. ) ;
#21741=ORIENTED_EDGE ( 'NONE', *, *, #24060, .F. ) ;
#21742=AXIS2_PLACEMENT_3D ( 'NONE', #64318, #2087, #56587 ) ;
#21744=CARTESIAN_POINT ( 'NONE',  ( 98.63028220664102719, -30.46987006685205657, 180.8184824187679567 ) ) ;
#21746=CARTESIAN_POINT ( 'NONE',  ( 41.56670390244695312, -36.32844715994109208, 129.9678068554150911 ) ) ;
#21747=CARTESIAN_POINT ( 'NONE',  ( 117.9552932246042332, -34.69990928640298478, 199.9851490854349549 ) ) ;
#21748=CARTESIAN_POINT ( 'NONE',  ( 112.8417677104678063, -27.25086138798909374, 45.62895860924398761 ) ) ;
#21751=DIRECTION ( 'NONE',  ( 4.299999999999999979E-14, -1.000000000000000000, 4.400000000000000367E-29 ) ) ;
#21752=VERTEX_POINT ( 'NONE', #60906 ) ;
#21753=VECTOR ( 'NONE', #41106, 1000.000000000000000 ) ;
#21756=ORIENTED_EDGE ( 'NONE', *, *, #12286, .T. ) ;
#21759=DIRECTION ( 'NONE',  ( -0.7071067811734105257, 0.7071067811996846197, 0.000000000000000000 ) ) ;
#21760=CARTESIAN_POINT ( 'NONE',  ( 100.8484424157226442, -45.14118303587278547, 253.0699109901968882 ) ) ;
#21762=CARTESIAN_POINT ( 'NONE',  ( 135.9115321082997809, -16.68812259378463025, 2.188418746654308578 ) ) ;
#21764=CIRCLE ( 'NONE', #26098, 29.00000000000000000 ) ;
#21765=CYLINDRICAL_SURFACE ( 'NONE', #55445, 3.300000000000000711 ) ;
#21767=CARTESIAN_POINT ( 'NONE',  ( 121.5762960060074960, -43.47224590996763993, 0.7256252759109853567 ) ) ;
#21768=EDGE_CURVE ( 'NONE', #14135, #76504, #22953, .T. ) ;
#21769=CARTESIAN_POINT ( 'NONE',  ( 116.4944971008961261, -32.22846566477972630, 19.18133956162493092 ) ) ;
#21771=ORIENTED_EDGE ( 'NONE', *, *, #36074, .F. ) ;
#21773=CARTESIAN_POINT ( 'NONE',  ( 97.33794773618596707, -34.07063109094482201, 17.11683259552636116 ) ) ;
#21774=ADVANCED_FACE ( 'NONE', ( #68626, #34984 ), #27731, .F. ) ;
#21775=CARTESIAN_POINT ( 'NONE',  ( 104.5747221139661605, -26.66317121150818892, 236.2575300378149734 ) ) ;
#21777=DIRECTION ( 'NONE',  ( 0.3818493186865920541, -0.9242245927363030855, 0.000000000000000000 ) ) ;
#21778=CARTESIAN_POINT ( 'NONE',  ( 109.0694692412632207, -27.15596902575785876, 135.9127681330529640 ) ) ;
#21781=ORIENTED_EDGE ( 'NONE', *, *, #13189, .T. ) ;
#21784=ORIENTED_EDGE ( 'NONE', *, *, #2758, .T. ) ;
#21785=AXIS2_PLACEMENT_3D ( 'NONE', #85926, #50021, #44546 ) ;
#21787=CARTESIAN_POINT ( 'NONE',  ( 110.3188062821955242, -28.45390942821411429, 266.2101547344684604 ) ) ;
#21788=DIRECTION ( 'NONE',  ( -0.7071067811869841124, 0.7071067811861110330, 0.000000000000000000 ) ) ;
#21789=EDGE_CURVE ( 'NONE', #30320, #62271, #33651, .T. ) ;
#21791=CARTESIAN_POINT ( 'NONE',  ( 102.0670549734760044, -27.97049805183234383, 85.48979194136749982 ) ) ;
#21794=VECTOR ( 'NONE', #54019, 1000.000000000000000 ) ;
#21795=LINE ( 'NONE', #83128, #72547 ) ;
#21796=DIRECTION ( 'NONE',  ( -1.000000000000000000, -3.999999999999999995E-14, -1.000000000000000078E-15 ) ) ;
#21797=ORIENTED_EDGE ( 'NONE', *, *, #17918, .F. ) ;
#21798=CARTESIAN_POINT ( 'NONE',  ( 99.29363446503140267, -43.73007054641615809, 56.90991099019593236 ) ) ;
#21800=CARTESIAN_POINT ( 'NONE',  ( 104.7514827670518684, -44.95118086569023319, 21.78099125664900626 ) ) ;
#21802=EDGE_CURVE ( 'NONE', #4000, #45258, #65012, .T. ) ;
#21804=CARTESIAN_POINT ( 'NONE',  ( 116.1939227058878714, -40.33550099034470549, 193.5270538473399426 ) ) ;
#21806=LINE ( 'NONE', #21344, #47628 ) ;
#21809=CARTESIAN_POINT ( 'NONE',  ( 98.40574028604457624, -42.07939390257583767, 7.768006228291934434 ) ) ;
#21811=AXIS2_PLACEMENT_3D ( 'NONE', #36472, #79160, #77807 ) ;
#21814=EDGE_LOOP ( 'NONE', ( #15661, #27160, #61091, #46522 ) ) ;
#21815=CARTESIAN_POINT ( 'NONE',  ( 114.7393473568293700, -44.74971245420289279, 109.1718157521009687 ) ) ;
#21819=VERTEX_POINT ( 'NONE', #62245 ) ;
#21821=CARTESIAN_POINT ( 'NONE',  ( 115.7831076434849251, -41.80230955793731340, 123.4064586049333485 ) ) ;
#21823=DIRECTION ( 'NONE',  ( 0.000000000000000000, 0.000000000000000000, 1.000000000000000000 ) ) ;
#21824=FACE_BOUND ( 'NONE', #19522, .T. ) ;
#21825=FACE_OUTER_BOUND ( 'NONE', #16456, .T. ) ;
#21827=CARTESIAN_POINT ( 'NONE',  ( 112.3492874949901932, -28.18945346073204306, 285.6356252759109680 ) ) ;
#21829=ORIENTED_EDGE ( 'NONE', *, *, #88140, .T. ) ;
#21830=CARTESIAN_POINT ( 'NONE',  ( 152.0371591254585155, -47.82818131005588214, 180.4678068554149775 ) ) ;
#21832=FACE_OUTER_BOUND ( 'NONE', #1163, .T. ) ;
#21833=ORIENTED_EDGE ( 'NONE', *, *, #60116, .F. ) ;
#21834=ORIENTED_EDGE ( 'NONE', *, *, #76339, .T. ) ;
#21836=FACE_BOUND ( 'NONE', #67725, .T. ) ;
#21837=DIRECTION ( 'NONE',  ( 1.017460296392624983E-15, 1.000000000000000000, 0.000000000000000000 ) ) ;
#21840=VECTOR ( 'NONE', #34962, 1000.000000000000000 ) ;
#21841=CARTESIAN_POINT ( 'NONE',  ( 109.1470148533826432, -28.41539336262556503, 199.3038483995049717 ) ) ;
#21842=LINE ( 'NONE', #15479, #73677 ) ;
#21843=DIRECTION ( 'NONE',  ( 0.000000000000000000, 0.000000000000000000, -1.000000000000000000 ) ) ;
#21844=CARTESIAN_POINT ( 'NONE',  ( 115.3018890743646665, -44.17195851134204077, 83.25372051400698581 ) ) ;
#21847=ADVANCED_FACE ( 'NONE', ( #7300 ), #14110, .F. ) ;
#21848=ORIENTED_EDGE ( 'NONE', *, *, #26501, .T. ) ;
#21850=DIRECTION ( 'NONE',  ( -0.000000000000000000, 1.000000000000000000, 0.000000000000000000 ) ) ;
#21851=EDGE_LOOP ( 'NONE', ( #38747, #66681, #12395, #1596, #29492, #53495 ) ) ;
#21852=CARTESIAN_POINT ( 'NONE',  ( 108.4173424463529756, -26.73501367913670279, 49.96897025569050754 ) ) ;
#21853=ORIENTED_EDGE ( 'NONE', *, *, #53773, .F. ) ;
#21855=CARTESIAN_POINT ( 'NONE',  ( 37.36643805256586859, -48.62818131006127231, 180.4678068554150911 ) ) ;
#21856=CARTESIAN_POINT ( 'NONE',  ( 101.9943086291660137, -45.44649556581995142, 273.1560813037751245 ) ) ;
#21858=CARTESIAN_POINT ( 'NONE',  ( 182.5667039024459939, -19.82844715994031048, -5.074374724088000832 ) ) ;
#21860=CARTESIAN_POINT ( 'NONE',  ( 118.7574168473771152, -34.64232270468420438, 48.96705384733895983 ) ) ;
#21861=( BOUNDED_CURVE ( )  B_SPLINE_CURVE ( 3, ( #8646, #49949, #77681, #42241 ),
 .UNSPECIFIED., .F., .T. ) 
 B_SPLINE_CURVE_WITH_KNOTS ( ( 4, 4 ),
 ( 3.141592653592887530, 4.712388980388064752 ),
 .UNSPECIFIED. ) 
 CURVE ( )  GEOMETRIC_REPRESENTATION_ITEM ( )  RATIONAL_B_SPLINE_CURVE ( ( 1.000000000000000000, 0.8047378541242988792, 0.8047378541242988792, 1.000000000000000000 ) ) 
 REPRESENTATION_ITEM ( '' )  );
#21862=DIRECTION ( 'NONE',  ( 0.000000000000000000, 1.000000000000000000, 0.000000000000000000 ) ) ;
#21863=CARTESIAN_POINT ( 'NONE',  ( 194.5667039024482960, -47.82844715993405771, 300.4678068554149490 ) ) ;
#21864=DIRECTION ( 'NONE',  ( -0.000000000000000000, -0.000000000000000000, -1.000000000000000000 ) ) ;
#21865=CARTESIAN_POINT ( 'NONE',  ( 100.8874678611112472, -44.70022135721517742, 142.0522919402655191 ) ) ;
#21867=CARTESIAN_POINT ( 'NONE',  ( 80.06648329127402519, -46.72944715994105991, 1.625625275910943746 ) ) ;
#21868=LINE ( 'NONE', #75137, #48301 ) ;
#21869=CARTESIAN_POINT ( 'NONE',  ( 144.4532657509292335, -72.54478064608022692, 540.9756252759101471 ) ) ;
#21870=CIRCLE ( 'NONE', #40709, 2.517499999999998739 ) ;
#21871=CARTESIAN_POINT ( 'NONE',  ( 108.3220630915710530, -47.10059840840933987, 113.6727681330539639 ) ) ;
#21872=DIRECTION ( 'NONE',  ( 0.9068632946707807507, -0.4214249218767881500, 9.028300618466658994E-16 ) ) ;
#21873=CARTESIAN_POINT ( 'NONE',  ( 126.9629299006805638, -46.62589376934779750, 14.92562527591094046 ) ) ;
#21875=AXIS2_PLACEMENT_3D ( 'NONE', #68200, #62266, #5983 ) ;
#21877=LINE ( 'NONE', #22776, #78175 ) ;
#21878=ADVANCED_FACE ( 'NONE', ( #13216 ), #82722, .F. ) ;
#21879=CARTESIAN_POINT ( 'NONE',  ( 116.4171719250472137, -30.71472603919677624, 140.2813395616249750 ) ) ;
#21880=AXIS2_PLACEMENT_3D ( 'NONE', #1717, #42563, #84401 ) ;
#21881=DIRECTION ( 'NONE',  ( 1.000000000000000000, 0.000000000000000000, 0.000000000000000000 ) ) ;
#21883=CARTESIAN_POINT ( 'NONE',  ( 99.34937008002601999, -28.84845824588786911, 266.7051490854347549 ) ) ;
#21884=DIRECTION ( 'NONE',  ( 1.000000000000000000, 0.000000000000000000, 0.000000000000000000 ) ) ;
#21885=DIRECTION ( 'NONE',  ( 0.9068632946707805287, -0.4214249218767882610, 1.035655806553318316E-15 ) ) ;
#21889=CARTESIAN_POINT ( 'NONE',  ( 172.5664832912740110, -18.82844715994099971, 201.0426252759120018 ) ) ;
#21890=CARTESIAN_POINT ( 'NONE',  ( 101.5632356570520756, -44.81509498605974784, 197.1013395616259913 ) ) ;
#21891=EDGE_LOOP ( 'NONE', ( #57241, #1644, #59323, #5436 ) ) ;
#21892=EDGE_LOOP ( 'NONE', ( #42154, #34873, #25362, #20231 ) ) ;
#21893=CARTESIAN_POINT ( 'NONE',  ( 99.50276801249795255, -32.11225214635365433, 167.3215833058969793 ) ) ;
#21896=CARTESIAN_POINT ( 'NONE',  ( 101.4562479827646371, -44.74122725731964323, 278.0899109901961879 ) ) ;
#21898=EDGE_CURVE ( 'NONE', #64904, #69092, #59221, .T. ) ;
#21899=AXIS2_PLACEMENT_3D ( 'NONE', #83705, #34647, #14669 ) ;
#21900=CARTESIAN_POINT ( 'NONE',  ( 123.6837132603319560, -54.60520651782485402, 218.8274735512161158 ) ) ;
#21903=VECTOR ( 'NONE', #46518, 1000.000000000000000 ) ;
#21906=CARTESIAN_POINT ( 'NONE',  ( 115.4423046205436947, -29.55243945206539280, 229.4022919425779605 ) ) ;
#21908=ORIENTED_EDGE ( 'NONE', *, *, #33286, .F. ) ;
#21910=EDGE_LOOP ( 'NONE', ( #58824, #51697 ) ) ;
#21911=EDGE_CURVE ( 'NONE', #22294, #51499, #55857, .T. ) ;
#21912=ADVANCED_FACE ( 'NONE', ( #88632 ), #40902, .T. ) ;
#21913=CARTESIAN_POINT ( 'NONE',  ( 106.8177105000358154, -25.27021144450689505, 321.3088427749597713 ) ) ;
#21915=CARTESIAN_POINT ( 'NONE',  ( 108.3341841271554244, -46.73478572737850101, 123.6756741429928184 ) ) ;
#21916=DIRECTION ( 'NONE',  ( 1.000000000000000000, 0.000000000000000000, -7.043400939473319300E-33 ) ) ;
#21918=EDGE_CURVE ( 'NONE', #52727, #63584, #51944, .T. ) ;
#21919=CARTESIAN_POINT ( 'NONE',  ( 118.0115280580377402, -34.77548253539075063, 44.96705384733895272 ) ) ;
#21920=CARTESIAN_POINT ( 'NONE',  ( 168.0371591254545649, -48.62818131005519007, 180.4678068554150059 ) ) ;
#21922=AXIS2_PLACEMENT_3D ( 'NONE', #25039, #80024, #81373 ) ;
#21923=CARTESIAN_POINT ( 'NONE',  ( 111.0628700864597533, -47.08446675046669583, 13.85753003781498016 ) ) ;
#21924=CARTESIAN_POINT ( 'NONE',  ( 46.83715912545424231, -47.82818131006082751, 300.4678068554150059 ) ) ;
#21925=EDGE_CURVE ( 'NONE', #26765, #37091, #89807, .T. ) ;
#21926=CARTESIAN_POINT ( 'NONE',  ( 110.8168587353559786, -26.33166992238134085, 249.7889586092445882 ) ) ;
#21927=ORIENTED_EDGE ( 'NONE', *, *, #84015, .F. ) ;
#21928=DIRECTION ( 'NONE',  ( 1.000000000000000078E-15, -1.000000000000000083E-30, -1.000000000000000000 ) ) ;
#21929=CARTESIAN_POINT ( 'NONE',  ( 163.1639762274590169, -34.03355364505800651, -5.074374724088000832 ) ) ;
#21930=CARTESIAN_POINT ( 'NONE',  ( 114.6207320473410931, -43.31440182122523197, 168.2560093401067149 ) ) ;
#21932=CARTESIAN_POINT ( 'NONE',  ( 109.2937122495728772, -44.61120707852311540, 70.61380465530497474 ) ) ;
#21933=CARTESIAN_POINT ( 'NONE',  ( 96.72156277063432128, -35.27346698316355145, 177.2156252759109805 ) ) ;
#21934=AXIS2_PLACEMENT_3D ( 'NONE', #38400, #36644, #85258 ) ;
#21935=DIRECTION ( 'NONE',  ( 1.017460296392624983E-15, 1.000000000000000000, 0.000000000000000000 ) ) ;
#21937=PLANE ( 'NONE',  #30575 ) ;
#21938=ORIENTED_EDGE ( 'NONE', *, *, #20164, .T. ) ;
#21939=ORIENTED_EDGE ( 'NONE', *, *, #42063, .F. ) ;
#21940=DIRECTION ( 'NONE',  ( 0.000000000000000000, 0.000000000000000000, 1.000000000000000000 ) ) ;
#21943=CARTESIAN_POINT ( 'NONE',  ( 80.06648329127401098, -39.47944715994105991, 1.625625275910943746 ) ) ;
#21944=LINE ( 'NONE', #53837, #46009 ) ;
#21945=CARTESIAN_POINT ( 'NONE',  ( 103.9632409301644316, -45.23724106753869734, 96.70861030426696914 ) ) ;
#21946=AXIS2_PLACEMENT_3D ( 'NONE', #35312, #84839, #63027 ) ;
#21947=CARTESIAN_POINT ( 'NONE',  ( 104.5828969173064849, -26.58150870143000688, 285.2670538473396391 ) ) ;
#21949=EDGE_CURVE ( 'NONE', #53017, #3248, #75193, .T. ) ;
#21952=AXIS2_PLACEMENT_3D ( 'NONE', #29097, #57227, #85866 ) ;
#21953=ORIENTED_EDGE ( 'NONE', *, *, #25905, .F. ) ;
#21954=EDGE_CURVE ( 'NONE', #48511, #33376, #84058, .T. ) ;
#21957=EDGE_CURVE ( 'NONE', #55604, #57432, #18584, .T. ) ;
#21958=DIRECTION ( 'NONE',  ( 0.000000000000000000, 0.000000000000000000, -1.000000000000000000 ) ) ;
#21960=CARTESIAN_POINT ( 'NONE',  ( 108.2420053567034017, -46.43931755893584779, 117.6727681330539639 ) ) ;
#21961=CARTESIAN_POINT ( 'NONE',  ( 115.0563813407508889, -43.54951484902237979, 63.26419670448196797 ) ) ;
#21963=EDGE_LOOP ( 'NONE', ( #75267, #74519, #59464, #42601 ) ) ;
#21964=CARTESIAN_POINT ( 'NONE',  ( 110.8168587353559786, -26.33166992238134085, 249.7889586092445882 ) ) ;
#21965=CARTESIAN_POINT ( 'NONE',  ( 182.2300522401149863, -33.89581943344511217, -5.074374724088000832 ) ) ;
#21967=CARTESIAN_POINT ( 'NONE',  ( 25.56670390244797275, -67.87844715994100397, 137.2178068554150059 ) ) ;
#21968=PLANE ( 'NONE',  #38685 ) ;
#21969=DIRECTION ( 'NONE',  ( -0.7071067811865431318, 0.7071067811865517916, -7.071067811865425043E-16 ) ) ;
#21970=FACE_OUTER_BOUND ( 'NONE', #66099, .T. ) ;
#21971=CARTESIAN_POINT ( 'NONE',  ( 105.6456579547864436, -25.35845045263859987, 320.8626788258979445 ) ) ;
#21972=CYLINDRICAL_SURFACE ( 'NONE', #19272, 0.2500000000000039968 ) ;
#21973=DIRECTION ( 'NONE',  ( 0.7071067811865779928, -0.7071067811865171526, 7.071067811865786933E-16 ) ) ;
#21977=CARTESIAN_POINT ( 'NONE',  ( 20.03715912545639100, -24.42818131006202265, 180.4678068554150911 ) ) ;
#21978=CARTESIAN_POINT ( 'NONE',  ( 104.4899544325742369, -26.97880758956900848, 260.2814586108214030 ) ) ;
#21980=CARTESIAN_POINT ( 'NONE',  ( 31.56670390244699931, -19.82844715994111340, 342.9256252759109884 ) ) ;
#21981=CARTESIAN_POINT ( 'NONE',  ( 114.4306803301698778, -27.41265490572180141, 274.5441967044824878 ) ) ;
#21982=CARTESIAN_POINT ( 'NONE',  ( 114.0809025726587436, -44.48955379074138961, 129.1613395616249704 ) ) ;
#21983=CARTESIAN_POINT ( 'NONE',  ( 118.0985323217624057, -37.71894194680212564, 29.74324432352998215 ) ) ;
#21984=FACE_BOUND ( 'NONE', #80796, .T. ) ;
#21987=CARTESIAN_POINT ( 'NONE',  ( 82.26522136040252065, -35.07517613921011446, 7.387586420632111128 ) ) ;
#21988=CARTESIAN_POINT ( 'NONE',  ( 93.94797395270803975, -35.60435878782502783, 296.5517437918485939 ) ) ;
#21989=VECTOR ( 'NONE', #18445, 1000.000000000000000 ) ;
#21991=CARTESIAN_POINT ( 'NONE',  ( 107.0664832912739968, -36.72944715994100306, 287.6356252759109680 ) ) ;
#21993=CARTESIAN_POINT ( 'NONE',  ( 108.5268020718178690, -45.14512305525489921, 167.1352769709339725 ) ) ;
#21994=CARTESIAN_POINT ( 'NONE',  ( 109.6395629035810231, -46.48095453850196179, 187.7817364959817326 ) ) ;
#21995=ORIENTED_EDGE ( 'NONE', *, *, #277, .F. ) ;
#21997=CARTESIAN_POINT ( 'NONE',  ( 117.2886123466743129, -34.79635738071010564, 154.9756252759109714 ) ) ;
#21998=DIRECTION ( 'NONE',  ( -1.000000000000000078E-15, -1.000000000000000083E-30, 1.000000000000000000 ) ) ;
#22000=CARTESIAN_POINT ( 'NONE',  ( 116.3199495083284347, -32.94194616109231077, 85.13562527591095375 ) ) ;
#22001=TOROIDAL_SURFACE ( 'NONE', #36518, 7.799999999999999822, 0.2999999999999999889 ) ;
#22003=FACE_OUTER_BOUND ( 'NONE', #948, .T. ) ;
#22004=CARTESIAN_POINT ( 'NONE',  ( 116.0091996907507905, -30.12340400999213941, 109.3327681330539605 ) ) ;
#22005=ORIENTED_EDGE ( 'NONE', *, *, #8065, .F. ) ;
#22008=ORIENTED_EDGE ( 'NONE', *, *, #61530, .F. ) ;
#22009=CARTESIAN_POINT ( 'NONE',  ( 109.4844142153598057, -45.28606679814626546, 69.22729759161194352 ) ) ;
#22011=CARTESIAN_POINT ( 'NONE',  ( 108.5755967597531679, -27.06580334247545494, 185.9527681330529845 ) ) ;
#22013=DIRECTION ( 'NONE',  ( 1.639958061481212836E-42, -4.100000000000000342E-29, -1.000000000000000000 ) ) ;
#22016=EDGE_CURVE ( 'NONE', #4456, #89731, #8648, .T. ) ;
#22017=AXIS2_PLACEMENT_3D ( 'NONE', #12785, #62258, #75900 ) ;
#22018=DIRECTION ( 'NONE',  ( 0.7071067811865969777, -0.7071067811864980568, 0.000000000000000000 ) ) ;
#22019=EDGE_CURVE ( 'NONE', #77531, #74275, #37235, .T. ) ;
#22020=DIRECTION ( 'NONE',  ( -0.7071067811865779928, 0.7071067811865171526, -6.612322855860441069E-17 ) ) ;
#22022=CARTESIAN_POINT ( 'NONE',  ( 103.2134869792595708, -46.43093390711695889, 117.2756252759109543 ) ) ;
#22024=EDGE_LOOP ( 'NONE', ( #71932, #25948, #17901, #71874 ) ) ;
#22025=AXIS2_PLACEMENT_3D ( 'NONE', #38805, #43830, #80168 ) ;
#22026=ORIENTED_EDGE ( 'NONE', *, *, #49663, .T. ) ;
#22027=EDGE_CURVE ( 'NONE', #2245, #16601, #78135, .T. ) ;
#22028=ADVANCED_FACE ( 'NONE', ( #21832 ), #8192, .T. ) ;
#22030=DIRECTION ( 'NONE',  ( -0.7071067811864671926, -0.7071067811866279529, -7.071067811864976379E-16 ) ) ;
#22031=CARTESIAN_POINT ( 'NONE',  ( 51.34673845256550351, -29.62846900982264842, 313.9678068554150059 ) ) ;
#22032=CARTESIAN_POINT ( 'NONE',  ( 98.55143180905920985, -33.04300857791147195, 208.8195189410199646 ) ) ;
#22034=DIRECTION ( 'NONE',  ( 0.7071067811865597852, -0.7071067811865354713, 0.000000000000000000 ) ) ;
#22036=FACE_OUTER_BOUND ( 'NONE', #15567, .T. ) ;
#22037=ORIENTED_EDGE ( 'NONE', *, *, #83186, .F. ) ;
#22038=ORIENTED_EDGE ( 'NONE', *, *, #33692, .T. ) ;
#22039=ORIENTED_EDGE ( 'NONE', *, *, #47846, .T. ) ;
#22040=VECTOR ( 'NONE', #29561, 1000.000000000000000 ) ;
#22042=EDGE_LOOP ( 'NONE', ( #11469, #43970, #41218, #79058 ) ) ;
#22044=CARTESIAN_POINT ( 'NONE',  ( 31.89136050872298966, -31.76306994223740432, -5.074374724088000832 ) ) ;
#22045=ADVANCED_FACE ( 'NONE', ( #84519 ), #15466, .T. ) ;
#22046=CARTESIAN_POINT ( 'NONE',  ( 116.4296429186904049, -33.01435002197194279, 245.5587261630399780 ) ) ;
#22047=LINE ( 'NONE', #49717, #50716 ) ;
#22049=AXIS2_PLACEMENT_3D ( 'NONE', #49421, #83518, #14932 ) ;
#22051=ADVANCED_FACE ( 'NONE', ( #51282 ), #57214, .T. ) ;
#22054=VERTEX_POINT ( 'NONE', #86281 ) ;
#22055=AXIS2_PLACEMENT_3D ( 'NONE', #57444, #78372, #29314 ) ;
#22056=CARTESIAN_POINT ( 'NONE',  ( 110.8712199137570593, -45.97737147754565967, 112.8870656898620553 ) ) ;
#22057=VERTEX_POINT ( 'NONE', #59443 ) ;
#22059=CARTESIAN_POINT ( 'NONE',  ( 99.09762411907954061, -31.97621503831505407, 278.7166617981628178 ) ) ;
#22060=CARTESIAN_POINT ( 'NONE',  ( 95.99055855653007541, -36.58346519971924948, 156.3280062282919687 ) ) ;
#22061=CARTESIAN_POINT ( 'NONE',  ( 114.0075736764523100, -28.98025818340840942, 114.4956252759109816 ) ) ;
#22062=CARTESIAN_POINT ( 'NONE',  ( 116.5506768258616432, -39.71645928710276507, 249.5838068554167819 ) ) ;
#22063=DIRECTION ( 'NONE',  ( 1.000000000000000000, 4.510281037539819615E-14, 0.000000000000000000 ) ) ;
#22064=CARTESIAN_POINT ( 'NONE',  ( 106.3019393658184129, -47.12646404140136269, 218.5184824187679453 ) ) ;
#22066=PLANE ( 'NONE',  #45120 ) ;
#22070=VECTOR ( 'NONE', #9710, 1000.000000000000000 ) ;
#22071=EDGE_CURVE ( 'NONE', #65869, #7080, #9910, .T. ) ;
#22073=DIRECTION ( 'NONE',  ( 0.000000000000000000, -1.000000000000000000, 0.000000000000000000 ) ) ;
#22074=ADVANCED_FACE ( 'NONE', ( #18117 ), #25379, .T. ) ;
#22075=AXIS2_PLACEMENT_3D ( 'NONE', #54437, #33577, #62173 ) ;
#22076=CIRCLE ( 'NONE', #65556, 3.299999999999999822 ) ;
#22078=CARTESIAN_POINT ( 'NONE',  ( 114.7262375871959392, -43.80158930977980702, 123.2327681330539519 ) ) ;
#22079=LINE ( 'NONE', #56099, #18124 ) ;
#22081=DIRECTION ( 'NONE',  ( 1.000000000000000000, 4.163336342344333240E-14, 0.000000000000000000 ) ) ;
#22083=CARTESIAN_POINT ( 'NONE',  ( 117.1011259092108787, -37.51040938078600107, 58.76384579545401721 ) ) ;
#22084=CARTESIAN_POINT ( 'NONE',  ( 105.7790678824445223, -26.40611305247087870, 266.1756252759109884 ) ) ;
#22086=CARTESIAN_POINT ( 'NONE',  ( 182.4202572930259976, -31.94127993907710206, -5.074374724088000832 ) ) ;
#22087=DIRECTION ( 'NONE',  ( -0.8660253910675258515, -0.0001484127181930297611, 0.5000000000000041078 ) ) ;
#22089=CARTESIAN_POINT ( 'NONE',  ( 115.8254323913364630, -31.73001882733125001, 255.2397919427014585 ) ) ;
#22090=CIRCLE ( 'NONE', #72832, 4.750000000000004441 ) ;
#22092=CARTESIAN_POINT ( 'NONE',  ( 115.0886446791137132, -30.00251675211520919, 269.3813395616250546 ) ) ;
#22095=CARTESIAN_POINT ( 'NONE',  ( 98.07151883162052286, -42.11266039418816121, 161.7556252759109725 ) ) ;
#22096=CARTESIAN_POINT ( 'NONE',  ( 100.4792253034169960, -27.85352395805916359, 31.59657765686396758 ) ) ;
#22097=CARTESIAN_POINT ( 'NONE',  ( 98.51568282078342520, -45.00561318155631341, 187.9384824187679612 ) ) ;
#22099=DIRECTION ( 'NONE',  ( 0.000000000000000000, -1.000000000000000000, 0.000000000000000000 ) ) ;
#22100=CARTESIAN_POINT ( 'NONE',  ( 141.8664832912739939, -71.52944715994085811, 361.9756252759100335 ) ) ;
#22101=DIRECTION ( 'NONE',  ( 1.000000000000000000, 4.299999999999999979E-14, 1.000000000000000078E-15 ) ) ;
#22105=EDGE_CURVE ( 'NONE', #56233, #78479, #39005, .T. ) ;
#22106=CARTESIAN_POINT ( 'NONE',  ( 163.1543517358616668, -31.62489322947754289, 237.4678068554150059 ) ) ;
#22108=ORIENTED_EDGE ( 'NONE', *, *, #57242, .F. ) ;
#22109=CARTESIAN_POINT ( 'NONE',  ( 83.06670390244804025, -51.22944715994108122, 231.5838068554169524 ) ) ;
#22110=ORIENTED_EDGE ( 'NONE', *, *, #84590, .T. ) ;
#22111=CARTESIAN_POINT ( 'NONE',  ( 117.0329088946582630, -32.00354160957723337, 60.19086337114898555 ) ) ;
#22113=LINE ( 'NONE', #85241, #51412 ) ;
#22114=CARTESIAN_POINT ( 'NONE',  ( 101.9632951345543148, -45.91070444983295573, 183.1727681330539781 ) ) ;
#22116=CARTESIAN_POINT ( 'NONE',  ( 100.7827017321902758, -30.20819270671951173, 265.0971817328389761 ) ) ;
#22117=ORIENTED_EDGE ( 'NONE', *, *, #24591, .F. ) ;
#22120=ORIENTED_EDGE ( 'NONE', *, *, #185, .F. ) ;
#22121=AXIS2_PLACEMENT_3D ( 'NONE', #19886, #784, #82585 ) ;
#22123=CARTESIAN_POINT ( 'NONE',  ( 98.30753419365476020, -41.72887549635444060, 106.7397919430594300 ) ) ;
#22125=CARTESIAN_POINT ( 'NONE',  ( 97.07205900541282517, -35.37856870842702506, 162.2189687603248558 ) ) ;
#22126=CARTESIAN_POINT ( 'NONE',  ( 99.09570906993977246, -30.55043176099360025, 75.80229194336320120 ) ) ;
#22127=DIRECTION ( 'NONE',  ( 4.299999999999999979E-14, -1.000000000000000000, 0.000000000000000000 ) ) ;
#22129=CARTESIAN_POINT ( 'NONE',  ( 181.5667039024459939, -22.48495420874030515, -5.074374724088000832 ) ) ;
#22130=EDGE_CURVE ( 'NONE', #49937, #29939, #38994, .T. ) ;
#22131=DIRECTION ( 'NONE',  ( 0.7071067811862279395, -0.7071067811868672059, 7.071067811862286363E-16 ) ) ;
#22133=CARTESIAN_POINT ( 'NONE',  ( 80.06648329127398256, -9.029447159941060619, 1.625625275910943746 ) ) ;
#22134=CARTESIAN_POINT ( 'NONE',  ( 96.85498737197825392, -38.89503640450125488, 31.49276813305495892 ) ) ;
#22135=FACE_OUTER_BOUND ( 'NONE', #87363, .T. ) ;
#22136=AXIS2_PLACEMENT_3D ( 'NONE', #22140, #63450, #76180 ) ;
#22137=ORIENTED_EDGE ( 'NONE', *, *, #19963, .T. ) ;
#22140=CARTESIAN_POINT ( 'NONE',  ( 134.0664832912740110, -8.729447159940999512, 308.6356252759119911 ) ) ;
#22141=CARTESIAN_POINT ( 'NONE',  ( 108.0475348069766284, -44.83298120013808585, 115.4909475124489830 ) ) ;
#22142=EDGE_CURVE ( 'NONE', #44500, #62791, #63652, .T. ) ;
#22143=FACE_BOUND ( 'NONE', #23270, .T. ) ;
#22144=ADVANCED_FACE ( 'NONE', ( #9981 ), #86730, .T. ) ;
#22145=AXIS2_PLACEMENT_3D ( 'NONE', #39797, #47948, #75689 ) ;
#22147=ORIENTED_EDGE ( 'NONE', *, *, #62829, .F. ) ;
#22148=ORIENTED_EDGE ( 'NONE', *, *, #86638, .T. ) ;
#22149=CARTESIAN_POINT ( 'NONE',  ( 98.04152496004225270, -41.04187039268755655, 136.6813859289020741 ) ) ;
#22152=CARTESIAN_POINT ( 'NONE',  ( 98.21222678671237816, -37.09057735734792516, 157.7901547344689845 ) ) ;
#22154=CARTESIAN_POINT ( 'NONE',  ( 98.31807308660266642, -42.43931386104045345, 97.78705384733993355 ) ) ;
#22155=FACE_OUTER_BOUND ( 'NONE', #64758, .T. ) ;
#22156=ORIENTED_EDGE ( 'NONE', *, *, #86809, .F. ) ;
#22161=ORIENTED_EDGE ( 'NONE', *, *, #68606, .T. ) ;
#22162=CARTESIAN_POINT ( 'NONE',  ( 97.60228370312334789, -39.19771807597653179, 276.5299109901972088 ) ) ;
#22163=CARTESIAN_POINT ( 'NONE',  ( 118.9020112566783354, -37.70028621367283961, 184.7613395616249647 ) ) ;
#22165=PLANE ( 'NONE',  #11222 ) ;
#22166=CARTESIAN_POINT ( 'NONE',  ( 102.6976273654655643, -46.88262786655960923, 133.2651490854349561 ) ) ;
#22167=DIRECTION ( 'NONE',  ( 0.9068632946707805287, -0.4214249218767882055, 8.839355291601567287E-16 ) ) ;
#22168=EDGE_LOOP ( 'NONE', ( #62796, #75150, #74287, #87010 ) ) ;
#22169=DIRECTION ( 'NONE',  ( 0.000000000000000000, 0.000000000000000000, -1.000000000000000000 ) ) ;
#22170=VERTEX_POINT ( 'NONE', #18566 ) ;
#22171=CARTESIAN_POINT ( 'NONE',  ( 116.8167403593138687, -34.15142894304322851, 135.0315941499441408 ) ) ;
#22172=EDGE_LOOP ( 'NONE', ( #14769, #35913, #64254, #8402 ) ) ;
#22173=EDGE_CURVE ( 'NONE', #46741, #71950, #10419, .T. ) ;
#22175=CIRCLE ( 'NONE', #84560, 2.117000000000000881 ) ;
#22178=CARTESIAN_POINT ( 'NONE',  ( 97.10456541990245682, -39.80308206185652864, 21.56419670448195092 ) ) ;
#22180=DIRECTION ( 'NONE',  ( 0.000000000000000000, 1.000000000000000000, 0.000000000000000000 ) ) ;
#22181=CARTESIAN_POINT ( 'NONE',  ( 107.0664832912739257, -50.22944715994095333, 315.1356252759112522 ) ) ;
#22182=CARTESIAN_POINT ( 'NONE',  ( 109.4837483930865574, -46.20680252518646114, 47.77562527591094721 ) ) ;
#22183=DIRECTION ( 'NONE',  ( 0.002456323621556914284, -0.5003413983110611696, -0.8658247233767341067 ) ) ;
#22184=CARTESIAN_POINT ( 'NONE',  ( 114.1602155298369325, -45.17592836263234091, 144.1203871806729637 ) ) ;
#22185=CARTESIAN_POINT ( 'NONE',  ( 97.33784130821194935, -34.07106454015703179, 72.11479194342473420 ) ) ;
#22190=CARTESIAN_POINT ( 'NONE',  ( 151.0371591254573502, -24.42818131005593685, 237.4678068554150059 ) ) ;
#22193=CARTESIAN_POINT ( 'NONE',  ( 117.1106518157658343, -39.68263944894788864, 183.5984824187679578 ) ) ;
#22195=DIRECTION ( 'NONE',  ( 3.999999999999999995E-14, -1.000000000000000000, 4.100000000000000342E-29 ) ) ;
#22196=CARTESIAN_POINT ( 'NONE',  ( 96.11533564597472434, -35.06885359281673686, 217.1946728949589840 ) ) ;
#22197=CARTESIAN_POINT ( 'NONE',  ( 106.0723295733845362, -48.58789440604735432, 108.5099109901969712 ) ) ;
#22198=LINE ( 'NONE', #14930, #59191 ) ;
#22200=CARTESIAN_POINT ( 'NONE',  ( 108.3334481036005599, -46.73485935279997960, 77.67729194326504683 ) ) ;
#22201=VERTEX_POINT ( 'NONE', #52604 ) ;
#22202=CIRCLE ( 'NONE', #67162, 2.517499999999998739 ) ;
#22204=VERTEX_POINT ( 'NONE', #46246 ) ;
#22206=VERTEX_POINT ( 'NONE', #73983 ) ;
#22208=CARTESIAN_POINT ( 'NONE',  ( 98.89890862997502552, -29.28198419350761483, 226.7261014663869503 ) ) ;
#22209=CARTESIAN_POINT ( 'NONE',  ( 97.01732288581034425, -36.31871811287255980, 251.2938706393009340 ) ) ;
#22210=CARTESIAN_POINT ( 'NONE',  ( 134.0664832912739826, -15.97944715994100306, 1.625625275910997480 ) ) ;
#22212=CARTESIAN_POINT ( 'NONE',  ( 182.3467384525650061, -29.62846900982231446, 342.9256252759119548 ) ) ;
#22214=CARTESIAN_POINT ( 'NONE',  ( 117.5098600993040066, -37.01623072280121107, 43.80419670448293346 ) ) ;
#22215=ORIENTED_EDGE ( 'NONE', *, *, #50194, .F. ) ;
#22216=ORIENTED_EDGE ( 'NONE', *, *, #33440, .T. ) ;
#22217=AXIS2_PLACEMENT_3D ( 'NONE', #3864, #72900, #5204 ) ;
#22218=CARTESIAN_POINT ( 'NONE',  ( 115.0901107527865150, -30.61920090636028036, 15.34508885633713682 ) ) ;
#22219=CARTESIAN_POINT ( 'NONE',  ( 117.6440909798951253, -33.30491947301820232, 280.0756252759109657 ) ) ;
#22222=AXIS2_PLACEMENT_3D ( 'NONE', #83773, #21998, #69239 ) ;
#22223=CARTESIAN_POINT ( 'NONE',  ( 112.7054497023526238, -28.73785826246146158, 125.5870538473389502 ) ) ;
#22224=EDGE_CURVE ( 'NONE', #57373, #8193, #52164, .T. ) ;
#22228=ORIENTED_EDGE ( 'NONE', *, *, #68466, .T. ) ;
#22229=DIRECTION ( 'NONE',  ( 0.000000000000000000, 1.000000000000000000, 0.000000000000000000 ) ) ;
#22230=EDGE_CURVE ( 'NONE', #78219, #23819, #4942, .T. ) ;
#22231=DIRECTION ( 'NONE',  ( -0.000000000000000000, -0.000000000000000000, -1.000000000000000000 ) ) ;
#22232=ORIENTED_EDGE ( 'NONE', *, *, #55176, .F. ) ;
#22235=CARTESIAN_POINT ( 'NONE',  ( 100.5471494818408189, -29.96373860736636274, 262.1063452106591853 ) ) ;
#22238=CARTESIAN_POINT ( 'NONE',  ( 48.86082318535700608, -35.55794170701751256, 342.9256252759119548 ) ) ;
#22239=FACE_OUTER_BOUND ( 'NONE', #70735, .T. ) ;
#22242=ORIENTED_EDGE ( 'NONE', *, *, #16473, .F. ) ;
#22245=EDGE_LOOP ( 'NONE', ( #53583, #57279 ) ) ;
#22246=CARTESIAN_POINT ( 'NONE',  ( 97.62219055090962172, -32.23153194184447301, 75.97276813305397525 ) ) ;
#22248=CARTESIAN_POINT ( 'NONE',  ( 99.46800687602927837, -39.83949638310546248, 11.05813411379097388 ) ) ;
#22250=CARTESIAN_POINT ( 'NONE',  ( 109.2168187703261282, -26.58475186820026792, 184.9222919425779708 ) ) ;
#22252=CARTESIAN_POINT ( 'NONE',  ( 181.8884939055946006, -32.11662333283960180, 313.9678068554149490 ) ) ;
#22255=CARTESIAN_POINT ( 'NONE',  ( 96.93665061341955891, -39.37131572480267749, 272.5299109901966972 ) ) ;
#22256=CARTESIAN_POINT ( 'NONE',  ( 98.41008151203357102, -41.80409597589088833, 116.7490096102640251 ) ) ;
#22257=ORIENTED_EDGE ( 'NONE', *, *, #86780, .T. ) ;
#22258=VECTOR ( 'NONE', #55650, 1000.000000000000000 ) ;
#22260=ORIENTED_EDGE ( 'NONE', *, *, #38145, .F. ) ;
#22261=CARTESIAN_POINT ( 'NONE',  ( 118.9671133714783480, -36.92893286478360437, 149.8127681330539644 ) ) ;
#22262=FACE_OUTER_BOUND ( 'NONE', #69448, .T. ) ;
#22263=ORIENTED_EDGE ( 'NONE', *, *, #48538, .F. ) ;
#22266=CARTESIAN_POINT ( 'NONE',  ( 116.3201495438094923, -32.94088975182634726, 124.1356252759109537 ) ) ;
#22267=CARTESIAN_POINT ( 'NONE',  ( 194.0371591254575208, -24.42818131005417115, 180.4678068554150343 ) ) ;
#22268=CYLINDRICAL_SURFACE ( 'NONE', #45699, 9.999999999999998224 ) ;
#22269=LINE ( 'NONE', #57663, #36505 ) ;
#22271=CARTESIAN_POINT ( 'NONE',  ( 114.0905851706116181, -46.27390148416495208, 29.08133956162595268 ) ) ;
#22272=CARTESIAN_POINT ( 'NONE',  ( 172.5664832912729878, -27.57844715994070484, 138.9256252759119832 ) ) ;
#22273=ORIENTED_EDGE ( 'NONE', *, *, #23217, .F. ) ;
#22275=CARTESIAN_POINT ( 'NONE',  ( 112.0659081082637840, -45.48839843342108225, 42.98939337566707763 ) ) ;
#22277=ORIENTED_EDGE ( 'NONE', *, *, #17456, .T. ) ;
#22278=ORIENTED_EDGE ( 'NONE', *, *, #77080, .T. ) ;
#22279=CARTESIAN_POINT ( 'NONE',  ( 82.74959284958350736, -19.33856210726131053, 3.004220725470469144 ) ) ;
#22282=EDGE_CURVE ( 'NONE', #67095, #69124, #26278, .T. ) ;
#22283=FACE_BOUND ( 'NONE', #34855, .T. ) ;
#22285=CARTESIAN_POINT ( 'NONE',  ( 102.4276729374712431, -43.93594010915269621, 221.5438483995059755 ) ) ;
#22288=CARTESIAN_POINT ( 'NONE',  ( 117.4149692539380681, -32.71426074976766074, 94.10895860924395606 ) ) ;
#22289=EDGE_LOOP ( 'NONE', ( #74984, #15958, #65831, #60317 ) ) ;
#22290=CARTESIAN_POINT ( 'NONE',  ( 131.4346950876525568, -19.52719034724729497, 6.916533740478841175 ) ) ;
#22291=VERTEX_POINT ( 'NONE', #39897 ) ;
#22293=CARTESIAN_POINT ( 'NONE',  ( 113.6135369627281335, -29.08718243961786598, 275.5131478814660682 ) ) ;
#22294=VERTEX_POINT ( 'NONE', #5853 ) ;
#22297=DIRECTION ( 'NONE',  ( 1.000000000000000000, 0.000000000000000000, 0.000000000000000000 ) ) ;
#22298=CARTESIAN_POINT ( 'NONE',  ( 100.8879627497241387, -44.70063105137227666, 273.0519027137635248 ) ) ;
#22303=CARTESIAN_POINT ( 'NONE',  ( 102.5485826229696329, -27.30952478670668881, 95.43276813305395478 ) ) ;
#22306=DIRECTION ( 'NONE',  ( -1.000000000000000078E-15, 1.000000000000000083E-30, 1.000000000000000000 ) ) ;
#22312=LINE ( 'NONE', #77728, #29883 ) ;
#22313=CARTESIAN_POINT ( 'NONE',  ( 116.6182342972125809, -29.67350615900649657, 105.3327681330539463 ) ) ;
#22314=CARTESIAN_POINT ( 'NONE',  ( 29.56648329127298069, -71.37844715994266664, 342.9256252759109884 ) ) ;
#22317=VECTOR ( 'NONE', #36925, 1000.000000000000000 ) ;
#22321=CARTESIAN_POINT ( 'NONE',  ( 96.71010325458821910, -37.26253042779857338, 117.3794347997199594 ) ) ;
#22322=EDGE_CURVE ( 'NONE', #82906, #69283, #34595, .T. ) ;
#22324=ORIENTED_EDGE ( 'NONE', *, *, #68336, .F. ) ;
#22325=CARTESIAN_POINT ( 'NONE',  ( 115.5963437193832277, -42.63132022635295471, 9.356577656862985037 ) ) ;
#22327=DIRECTION ( 'NONE',  ( 1.000000000000000078E-15, 1.000000000000000083E-30, -1.000000000000000000 ) ) ;
#22328=FACE_OUTER_BOUND ( 'NONE', #11995, .T. ) ;
#22329=EDGE_CURVE ( 'NONE', #16664, #12989, #75332, .T. ) ;
#22331=FACE_BOUND ( 'NONE', #36311, .T. ) ;
#22332=CARTESIAN_POINT ( 'NONE',  ( 99.34779341711919187, -29.80408710710932496, 235.7565776568639819 ) ) ;
#22334=ORIENTED_EDGE ( 'NONE', *, *, #31813, .F. ) ;
#22335=CARTESIAN_POINT ( 'NONE',  ( 113.2524973562852608, -30.34232264463288686, 170.8958690201829711 ) ) ;
#22336=B_SPLINE_CURVE_WITH_KNOTS ( 'NONE', 3,
 ( #15628, #15172, #63317, #21546, #69688, #8360, #49219, #76498, #64221, #70587, #62857, #36057, #50570, #14731, #77852, #55570, #63774, #83320, #70132, #29252, #78312, #43301, #1551, #56937, #71046, #633, #57385, #7459, #28804, #71492, #35600, #42405, #27895, #22000 ),
 .UNSPECIFIED., .F., .F.,
 ( 4, 2, 2, 2, 2, 2, 2, 2, 2, 1, 1, 1, 1, 2, 2, 2, 2, 2, 4 ),
 ( 0.5000923170378537286, 0.5625807774081261758, 0.6250692377783986231, 0.6875576981486710704, 0.7188019283338071830, 0.7500461585189430735, 0.8125346188892145216, 0.8437788490743498571, 0.8594009641669180244, 0.8672120217132019970, 0.8711175504863439834, 0.8730703148729151986, 0.8740466970662008617, 0.8745348881628436377, 0.8750230792594864138, 0.9062673094446147548, 0.9375115396297432069, 0.9687557698148714369, 1.000000000000000000 ),
 .UNSPECIFIED. ) ;
#22337=AXIS2_PLACEMENT_3D ( 'NONE', #23589, #15873, #70382 ) ;
#22338=LINE ( 'NONE', #535, #76270 ) ;
#22339=CARTESIAN_POINT ( 'NONE',  ( 115.9938408324894539, -42.00591253359444011, 279.4137205140056608 ) ) ;
#22340=VECTOR ( 'NONE', #9806, 1000.000000000000000 ) ;
#22342=VECTOR ( 'NONE', #23961, 1000.000000000000000 ) ;
#22343=B_SPLINE_CURVE_WITH_KNOTS ( 'NONE', 3,
 ( #78465, #37557, #43453, #65257, #37996, #86602, #72955, #85280, #72528, #65690, #43902, #23931, #31168, #79802, #50267, #3036, #29405, #51604, #30734, #71194, #23052, #50727, #58865, #64371, #79354, #36667, #24375, #58429, #17556, #84827, #57085, #45233, #2146, #22593, #36212, #1701, #29852, #78009, #15776, #16226, #57540, #37110, #64815, #2597, #30292, #57991, #85723, #23499, #51164 ),
 .UNSPECIFIED., .F., .F.,
 ( 4, 2, 1, 1, 1, 1, 2, 2, 2, 2, 2, 2, 2, 1, 1, 1, 1, 1, 1, 1, 2, 2, 2, 2, 2, 2, 2, 2, 2, 4 ),
 ( 0.5000151698130386180, 0.5005034362487721378, 0.5009917026845057686, 0.5019682355559731413, 0.5039213012989078866, 0.5078274327847773773, 0.5156396957565162475, 0.5312642216999940992, 0.5625132735869494693, 0.6250113773608605428, 0.6875094811347715051, 0.7500075849086826896, 0.7500686182131491853, 0.7501296515176159030, 0.7502517181265497825, 0.7504958513444184298, 0.7509841177801490630, 0.7519606506516048894, 0.7539137163944960029, 0.7578198478802943283, 0.7656321108518988616, 0.7812566367951041535, 0.8125056886815178459, 0.8437547405679315382, 0.8750037924543452306, 0.9062528443407589229, 0.9375018962271726153, 0.9687509481135863076, 0.9843754740567931538, 1.000000000000000000 ),
 .UNSPECIFIED. ) ;
#22344=LINE ( 'NONE', #21900, #24355 ) ;
#22349=CARTESIAN_POINT ( 'NONE',  ( 97.53193330917046922, -39.74923349999438216, 37.57026538729112275 ) ) ;
#22350=EDGE_CURVE ( 'NONE', #27695, #18119, #67996, .T. ) ;
#22351=CARTESIAN_POINT ( 'NONE',  ( 118.0177608886754967, -35.41288285714057338, 238.9337205140059552 ) ) ;
#22352=LINE ( 'NONE', #7814, #61949 ) ;
#22353=ORIENTED_EDGE ( 'NONE', *, *, #6504, .T. ) ;
#22355=CARTESIAN_POINT ( 'NONE',  ( 100.8874678657582677, -44.70022136077002983, 87.05229194071588950 ) ) ;
#22358=DIRECTION ( 'NONE',  ( 0.7071067811865496822, 7.071067811865498013E-16, -0.7071067811865453523 ) ) ;
#22359=CARTESIAN_POINT ( 'NONE',  ( 115.1932381579439948, -43.17108053757041830, 44.30514908543392494 ) ) ;
#22360=DIRECTION ( 'NONE',  ( 0.000000000000000000, 0.000000000000000000, 1.000000000000000000 ) ) ;
#22361=ORIENTED_EDGE ( 'NONE', *, *, #55558, .T. ) ;
#22362=CARTESIAN_POINT ( 'NONE',  ( 111.4336192290781753, -46.24370506310440732, 23.91848241876792969 ) ) ;
#22364=CARTESIAN_POINT ( 'NONE',  ( 117.4915365000037042, -36.80222117025145678, 263.8213395616251660 ) ) ;
#22366=CARTESIAN_POINT ( 'NONE',  ( 78.11989406980549688, -38.67261125150972134, 7.590611884311868174 ) ) ;
#22368=CARTESIAN_POINT ( 'NONE',  ( 31.89136050872298966, -31.76306994223740432, -5.074374724088000832 ) ) ;
#22369=CARTESIAN_POINT ( 'NONE',  ( 107.7548360709104855, -28.10233318731983232, 112.8433284648289430 ) ) ;
#22370=CARTESIAN_POINT ( 'NONE',  ( 98.36161695517027681, -29.88032255785606139, 196.8080062282919869 ) ) ;
#22371=CARTESIAN_POINT ( 'NONE',  ( 57.56670390244832447, -48.82844715994039575, 257.2178068554150627 ) ) ;
#22372=EDGE_LOOP ( 'NONE', ( #32174, #2802, #30724, #72843 ) ) ;
#22373=CARTESIAN_POINT ( 'NONE',  ( 172.5667039024482960, -42.82844715993499563, 180.4678068554150059 ) ) ;
#22377=PLANE ( 'NONE',  #86551 ) ;
#22378=( BOUNDED_CURVE ( )  B_SPLINE_CURVE ( 3, ( #37327, #65909, #78240, #3695 ),
 .UNSPECIFIED., .F., .F. ) 
 B_SPLINE_CURVE_WITH_KNOTS ( ( 4, 4 ),
 ( 4.712388980373003022, 6.283185307170268352 ),
 .UNSPECIFIED. ) 
 CURVE ( )  GEOMETRIC_REPRESENTATION_ITEM ( )  RATIONAL_B_SPLINE_CURVE ( ( 1.000000000000000000, 0.8047378541216103631, 0.8047378541216103631, 1.000000000000000000 ) ) 
 REPRESENTATION_ITEM ( '' )  );
#22379=ORIENTED_EDGE ( 'NONE', *, *, #57788, .F. ) ;
#22380=EDGE_LOOP ( 'NONE', ( #86932, #51662, #79682, #64089 ) ) ;
#22381=CARTESIAN_POINT ( 'NONE',  ( 117.0612621577405008, -38.07784205248298548, 169.7193832652232004 ) ) ;
#22383=ADVANCED_FACE ( 'NONE', ( #13112 ), #12207, .T. ) ;
#22384=CARTESIAN_POINT ( 'NONE',  ( 113.5546853072178237, -29.03447022270776046, 40.51940965636622138 ) ) ;
#22385=CARTESIAN_POINT ( 'NONE',  ( 103.7110576214454341, -44.58420688232069296, 91.67813411379100330 ) ) ;
#22386=CARTESIAN_POINT ( 'NONE',  ( 106.1363778353814666, -47.76712558329867875, 262.4975300378158067 ) ) ;
#22387=FACE_OUTER_BOUND ( 'NONE', #75838, .T. ) ;
#22388=DIRECTION ( 'NONE',  ( 4.299999999999999979E-14, -1.000000000000000000, 4.400000000000000367E-29 ) ) ;
#22389=ORIENTED_EDGE ( 'NONE', *, *, #26906, .F. ) ;
#22391=CYLINDRICAL_SURFACE ( 'NONE', #23253, 0.9999999999999800160 ) ;
#22394=CARTESIAN_POINT ( 'NONE',  ( 102.6513375509277495, -45.45698538002856282, 127.2041967044829960 ) ) ;
#22395=CARTESIAN_POINT ( 'NONE',  ( 113.9459708190624241, -28.01821676562244789, 124.5565776568629559 ) ) ;
#22397=EDGE_LOOP ( 'NONE', ( #83148, #27537 ) ) ;
#22400=CARTESIAN_POINT ( 'NONE',  ( 99.39677155223240845, -28.76988628678374837, 265.6746728949588032 ) ) ;
#22401=AXIS2_PLACEMENT_3D ( 'NONE', #85895, #44517, #31346 ) ;
#22402=CARTESIAN_POINT ( 'NONE',  ( 106.5394234437989667, -24.24056378642895737, 322.0356252759110021 ) ) ;
#22404=VECTOR ( 'NONE', #40136, 1000.000000000000114 ) ;
#22406=FACE_OUTER_BOUND ( 'NONE', #74525, .T. ) ;
#22408=CARTESIAN_POINT ( 'NONE',  ( 49.21213752016101495, -29.73316016639650172, -5.074374724088000832 ) ) ;
#22409=CARTESIAN_POINT ( 'NONE',  ( 105.2934191044239043, -25.40803282519309647, 322.8191631070221774 ) ) ;
#22410=DIRECTION ( 'NONE',  ( -1.000000000000000078E-15, 0.000000000000000000, -1.000000000000000000 ) ) ;
#22415=FACE_BOUND ( 'NONE', #4798, .T. ) ;
#22416=EDGE_CURVE ( 'NONE', #42450, #16685, #5626, .T. ) ;
#22421=CARTESIAN_POINT ( 'NONE',  ( 41.56670390244689628, -36.32844715994109208, 180.4678068554150911 ) ) ;
#22422=CARTESIAN_POINT ( 'NONE',  ( 117.5135424720979103, -36.80237478700602338, 263.8213395616250523 ) ) ;
#22423=CARTESIAN_POINT ( 'NONE',  ( 113.7506423937859807, -44.72972868871420360, 189.1299109901969757 ) ) ;
#22424=CARTESIAN_POINT ( 'NONE',  ( 99.04917799727566319, -44.37196124675453746, 32.92038718067297509 ) ) ;
#22426=CARTESIAN_POINT ( 'NONE',  ( 194.0371591254574923, -24.42818131005417115, 193.9678068554150343 ) ) ;
#22428=EDGE_CURVE ( 'NONE', #61259, #17509, #27619, .T. ) ;
#22429=ORIENTED_EDGE ( 'NONE', *, *, #23977, .F. ) ;
#22430=PLANE ( 'NONE',  #9874 ) ;
#22431=ORIENTED_EDGE ( 'NONE', *, *, #39714, .F. ) ;
#22432=CARTESIAN_POINT ( 'NONE',  ( 97.92582740012257148, -33.45545302834237589, 175.4752769709339759 ) ) ;
#22433=CARTESIAN_POINT ( 'NONE',  ( 115.7803070267097354, -41.80703622889448923, 188.4066082405644522 ) ) ;
#22434=EDGE_LOOP ( 'NONE', ( #29998, #80337, #51838, #5313 ) ) ;
#22435=DIRECTION ( 'NONE',  ( 0.000000000000000000, 0.000000000000000000, -1.000000000000000000 ) ) ;
#22436=CARTESIAN_POINT ( 'NONE',  ( 116.8369567342159456, -40.30247308064090817, 214.5470538473389581 ) ) ;
#22437=DIRECTION ( 'NONE',  ( 1.000000000000000000, 4.299999999999999979E-14, 1.000000000000000078E-15 ) ) ;
#22439=ADVANCED_FACE ( 'NONE', ( #34877 ), #363, .F. ) ;
#22441=CARTESIAN_POINT ( 'NONE',  ( 31.56670390244700641, -22.48495420874110806, -5.074374724088000832 ) ) ;
#22443=CARTESIAN_POINT ( 'NONE',  ( 98.82386243697609984, -31.40279086140550291, 145.8699109901969848 ) ) ;
#22444=ORIENTED_EDGE ( 'NONE', *, *, #59416, .F. ) ;
#22445=ORIENTED_EDGE ( 'NONE', *, *, #89360, .F. ) ;
#22447=CARTESIAN_POINT ( 'NONE',  ( 99.90998525089342763, -42.81722683197487811, 73.33110711542096283 ) ) ;
#22449=CARTESIAN_POINT ( 'NONE',  ( 116.5663773505004315, -40.88766770462209621, 204.4861014663869696 ) ) ;
#22450=CARTESIAN_POINT ( 'NONE',  ( 77.06670390244796920, -50.82844715994100682, 310.9178068554150514 ) ) ;
#22454=CARTESIAN_POINT ( 'NONE',  ( 90.44969454456408187, -53.34645651782490461, 239.5838068554174356 ) ) ;
#22455=EDGE_CURVE ( 'NONE', #36232, #66586, #64388, .T. ) ;
#22456=LINE ( 'NONE', #7919, #10045 ) ;
#22459=CARTESIAN_POINT ( 'NONE',  ( 114.7552509866192452, -44.63809267644818135, 118.2022919425779719 ) ) ;
#22460=VERTEX_POINT ( 'NONE', #9418 ) ;
#22462=ORIENTED_EDGE ( 'NONE', *, *, #2020, .T. ) ;
#22466=EDGE_CURVE ( 'NONE', #85489, #57830, #81046, .T. ) ;
#22467=CARTESIAN_POINT ( 'NONE',  ( 108.3334480829778812, -46.73485935560395177, 78.67729194162538420 ) ) ;
#22469=CARTESIAN_POINT ( 'NONE',  ( 107.2048247310825388, -44.91868093929326022, 210.4080903695909512 ) ) ;
#22471=CYLINDRICAL_SURFACE ( 'NONE', #29110, 0.2500000000000046074 ) ;
#22472=B_SPLINE_CURVE_WITH_KNOTS ( 'NONE', 3,
 ( #19828, #49308, #8446, #30228, #71575, #43388, #77939, #15261, #22982, #72013, #85655, #35687, #15711, #21637, #64307, #22525, #22089, #71129 ),
 .UNSPECIFIED., .F., .F.,
 ( 4, 2, 2, 2, 2, 2, 2, 2, 4 ),
 ( 0.4999999994038420992, 0.5624999994783618229, 0.6249999995528815466, 0.6874999996274013814, 0.7499999997019211051, 0.8124999997764408288, 0.8749999998509605525, 0.9374999999254802763, 1.000000000000000000 ),
 .UNSPECIFIED. ) ;
#22473=CARTESIAN_POINT ( 'NONE',  ( 102.6975360555999259, -46.88284006984166297, 137.2651490854349561 ) ) ;
#22474=CARTESIAN_POINT ( 'NONE',  ( 41.56648329127399677, -9.303447159940999356, 18.92562527591200094 ) ) ;
#22477=VERTEX_POINT ( 'NONE', #78029 ) ;
#22478=CONICAL_SURFACE ( 'NONE', #73217, 1.624999999999987566, 1.029744258676650093 ) ;
#22480=FACE_OUTER_BOUND ( 'NONE', #45825, .T. ) ;
#22485=CARTESIAN_POINT ( 'NONE',  ( 98.65401097786960349, -39.51487139837627893, 238.0130118773259653 ) ) ;
#22488=CARTESIAN_POINT ( 'NONE',  ( 116.6298083638390324, -39.11748333416112899, 9.635625275910943088 ) ) ;
#22489=PLANE ( 'NONE',  #83666 ) ;
#22490=ORIENTED_EDGE ( 'NONE', *, *, #75488, .T. ) ;
#22491=ORIENTED_EDGE ( 'NONE', *, *, #68381, .T. ) ;
#22492=CARTESIAN_POINT ( 'NONE',  ( 110.8546043978908244, -45.98418316275319029, 112.8856366702089247 ) ) ;
#22493=ORIENTED_EDGE ( 'NONE', *, *, #16299, .T. ) ;
#22494=ORIENTED_EDGE ( 'NONE', *, *, #48420, .F. ) ;
#22495=VECTOR ( 'NONE', #84308, 1000.000000000000000 ) ;
#22496=CARTESIAN_POINT ( 'NONE',  ( 101.6725443455464131, -43.49748584897681525, 269.8471379886391901 ) ) ;
#22497=CARTESIAN_POINT ( 'NONE',  ( 98.64801509901850807, -30.48302769619336416, 180.8184824187679567 ) ) ;
#22498=CARTESIAN_POINT ( 'NONE',  ( 97.81366378802354689, -42.73395665195503312, 146.7965776568629508 ) ) ;
#22499=DIRECTION ( 'NONE',  ( -1.000000000000000000, -3.999999999999999995E-14, -1.000000000000000078E-15 ) ) ;
#22500=CARTESIAN_POINT ( 'NONE',  ( 99.75313521292756036, -29.29995004827394212, 221.6956252759109702 ) ) ;
#22501=CARTESIAN_POINT ( 'NONE',  ( 179.4595971212720258, -26.00627455219131789, 117.4678068554150627 ) ) ;
#22502=DIRECTION ( 'NONE',  ( -0.9825752044165969590, -0.1858654558159821002, 0.000000000000000000 ) ) ;
#22503=EDGE_LOOP ( 'NONE', ( #39508, #19455, #49964, #5022, #36418 ) ) ;
#22504=CARTESIAN_POINT ( 'NONE',  ( 19.56670390244739721, -25.42844715994192129, 249.9678068554150059 ) ) ;
#22505=ORIENTED_EDGE ( 'NONE', *, *, #69003, .T. ) ;
#22507=AXIS2_PLACEMENT_3D ( 'NONE', #21830, #77235, #14567 ) ;
#22508=CARTESIAN_POINT ( 'NONE',  ( 116.4168962126584717, -41.43863437684461104, 203.4556252759109611 ) ) ;
#22510=EDGE_CURVE ( 'NONE', #76954, #16276, #49839, .T. ) ;
#22511=CARTESIAN_POINT ( 'NONE',  ( 117.7037197400453437, -39.73414628438690244, 143.6194347997209775 ) ) ;
#22514=CARTESIAN_POINT ( 'NONE',  ( 165.3359832912750278, -36.32844715993530826, 117.4678068554150485 ) ) ;
#22515=CARTESIAN_POINT ( 'NONE',  ( 123.6837132603318992, -23.41243780205710578, 239.5838068554165545 ) ) ;
#22516=EDGE_CURVE ( 'NONE', #55318, #2603, #20145, .T. ) ;
#22518=CARTESIAN_POINT ( 'NONE',  ( 100.3900607503748574, -44.18760341221117471, 56.99518173324602799 ) ) ;
#22519=CARTESIAN_POINT ( 'NONE',  ( 112.4780167374715631, -46.34085331822165443, 253.9965776568634510 ) ) ;
#22522=DIRECTION ( 'NONE',  ( 0.000000000000000000, 1.000000000000000000, 0.000000000000000000 ) ) ;
#22524=CARTESIAN_POINT ( 'NONE',  ( 151.5667039024485518, -48.82844715993590512, 180.4678068554149775 ) ) ;
#22525=CARTESIAN_POINT ( 'NONE',  ( 115.0889047221861290, -30.61763667734028971, 255.3439586094922618 ) ) ;
#22526=EDGE_CURVE ( 'NONE', #68501, #61899, #14455, .T. ) ;
#22528=DIRECTION ( 'NONE',  ( 0.000000000000000000, 0.000000000000000000, -1.000000000000000000 ) ) ;
#22531=LINE ( 'NONE', #83407, #39355 ) ;
#22532=CARTESIAN_POINT ( 'NONE',  ( 95.54500964991285628, -39.60862429916534211, 166.5213395616259788 ) ) ;
#22533=CARTESIAN_POINT ( 'NONE',  ( 117.3534687869931048, -38.62661931536851512, 84.68133956162593279 ) ) ;
#22534=CARTESIAN_POINT ( 'NONE',  ( 113.7132347973738575, -45.61866494189415988, 184.0994347997199725 ) ) ;
#22536=DIRECTION ( 'NONE',  ( -0.000000000000000000, 0.000000000000000000, -1.000000000000000000 ) ) ;
#22539=DIRECTION ( 'NONE',  ( -1.000000000000000000, 1.774213772886706994E-13, 0.000000000000000000 ) ) ;
#22542=EDGE_CURVE ( 'NONE', #48576, #50846, #7629, .T. ) ;
#22545=VECTOR ( 'NONE', #39506, 1000.000000000000000 ) ;
#22547=AXIS2_PLACEMENT_3D ( 'NONE', #58219, #85948, #60894 ) ;
#22548=EDGE_CURVE ( 'NONE', #28811, #40401, #39889, .T. ) ;
#22550=VERTEX_POINT ( 'NONE', #58446 ) ;
#22551=AXIS2_PLACEMENT_3D ( 'NONE', #13924, #41603, #291 ) ;
#22552=DIRECTION ( 'NONE',  ( 1.000000000000000078E-15, 0.000000000000000000, 1.000000000000000000 ) ) ;
#22553=VERTEX_POINT ( 'NONE', #45257 ) ;
#22554=CARTESIAN_POINT ( 'NONE',  ( 95.37363933861288956, -34.96150835630653120, 67.20705384733894050 ) ) ;
#22556=EDGE_CURVE ( 'NONE', #14017, #50559, #46141, .T. ) ;
#22557=AXIS2_PLACEMENT_3D ( 'NONE', #83102, #83536, #20855 ) ;
#22558=FACE_OUTER_BOUND ( 'NONE', #61135, .T. ) ;
#22559=CARTESIAN_POINT ( 'NONE',  ( 101.7473938980672870, -45.74611303501656323, 158.1527681330539963 ) ) ;
#22560=AXIS2_PLACEMENT_3D ( 'NONE', #64550, #30913, #37740 ) ;
#22561=CARTESIAN_POINT ( 'NONE',  ( 98.74870792914448714, -34.66384430100242753, 275.5552769709340737 ) ) ;
#22562=ORIENTED_EDGE ( 'NONE', *, *, #17207, .F. ) ;
#22563=ORIENTED_EDGE ( 'NONE', *, *, #57579, .F. ) ;
#22564=ORIENTED_EDGE ( 'NONE', *, *, #22428, .F. ) ;
#22566=CARTESIAN_POINT ( 'NONE',  ( 120.0664832912739399, -36.72944715994095333, 293.6356252759106837 ) ) ;
#22567=DIRECTION ( 'NONE',  ( 4.299999999999999979E-14, -1.000000000000000000, 4.400000000000000367E-29 ) ) ;
#22572=PLANE ( 'NONE',  #55820 ) ;
#22573=CARTESIAN_POINT ( 'NONE',  ( 156.5667039024480971, -42.82844715993568485, 293.2178068554149490 ) ) ;
#22574=CARTESIAN_POINT ( 'NONE',  ( 118.0600790064084293, -37.62648441163795354, 38.77372051400595865 ) ) ;
#22575=ORIENTED_EDGE ( 'NONE', *, *, #59881, .F. ) ;
#22578=ADVANCED_FACE ( 'NONE', ( #65278 ), #4837, .F. ) ;
#22580=CARTESIAN_POINT ( 'NONE',  ( 98.90423600646026614, -36.64316113183544843, 109.1366617981629474 ) ) ;
#22581=AXIS2_PLACEMENT_3D ( 'NONE', #75127, #20617, #82411 ) ;
#22582=B_SPLINE_CURVE_WITH_KNOTS ( 'NONE', 3,
 ( #52924, #11648, #72965, #67048, #60212, #23509, #78914, #44360, #72089, #47927, #62019, #13881, #12091, #27065, #81154, #53386, #60666, #75667, #33869, #75215, #13437, #68847, #20257, #12996, #69299, #40227, #39775, #54284, #7070, #81605, #68402, #18900, #89753, #20700, #53835, #12540, #61125, #27503, #54735, #47482, #82048, #25712, #46584, #74762, #41564, #6618, #34767, #55180, #82940, #19801, #87947, #48368, #88854, #40682, #82498, #32971, #88405, #41123, #76102, #74322, #34314, #67488, #5275, #26167, #6181, #19355, #47027, #26608, #61565, #67945, #89301, #5733, #33424, #35659, #62915, #77455, #84740, #70189, #27950, #22062, #86396, #28396 ),
 .UNSPECIFIED., .F., .F.,
 ( 4, 2, 2, 2, 2, 2, 2, 2, 2, 2, 2, 2, 2, 2, 2, 2, 2, 2, 2, 2, 2, 2, 2, 2, 2, 2, 2, 2, 2, 2, 2, 2, 2, 2, 2, 2, 2, 2, 2, 2, 4 ),
 ( 6.083641046005872842E-05, 0.0002295799514885608656, 0.0003983234925170630095, 0.0007358105745741082802, 0.001410784738688156213, 0.002760733066916254246, 0.004110681395144351845, 0.005460629723372451179, 0.006810578051600549646, 0.008160526379828647245, 0.009510474708056746579, 0.01086042303628484418, 0.01356031969274100642, 0.01626021634919716866, 0.01693519051331119837, 0.01761016467742522809, 0.01896011300565331181, 0.01963508716976735541, 0.02031006133388139553, 0.02166000966210947579, 0.02300995799033755604, 0.02435990631856564323, 0.02570985464679372695, 0.02705980297502181414, 0.02840975130324989439, 0.02975969963147798159, 0.03043467379559202171, 0.03110964795970606531, 0.03245959628793418372, 0.03380954461616231255, 0.03515949294439044137, 0.03650944127261857020, 0.03785938960084669902, 0.03920933792907482784, 0.04055928625730294973, 0.04190923458553107855, 0.04258420874964514297, 0.04292169583170216129, 0.04309043937273064617, 0.04317481114324489555, 0.04325918291375914493 ),
 .UNSPECIFIED. ) ;
#22583=LINE ( 'NONE', #1689, #68819 ) ;
#22584=CARTESIAN_POINT ( 'NONE',  ( 83.06670390244801183, -42.97311385574013798, 231.5838068554169524 ) ) ;
#22586=VERTEX_POINT ( 'NONE', #32082 ) ;
#22587=CARTESIAN_POINT ( 'NONE',  ( 97.81469011401388514, -40.51612824417846070, 136.6360017533206417 ) ) ;
#22588=VERTEX_POINT ( 'NONE', #39352 ) ;
#22590=CARTESIAN_POINT ( 'NONE',  ( 99.59846494627726088, -31.90336481815605296, 142.3015833058969974 ) ) ;
#22591=DIRECTION ( 'NONE',  ( 1.000000000000000078E-15, -1.000000000000000083E-30, -1.000000000000000000 ) ) ;
#22592=CARTESIAN_POINT ( 'NONE',  ( 98.13097783494514204, -43.27482323654912477, 102.8175300378159847 ) ) ;
#22593=CARTESIAN_POINT ( 'NONE',  ( 111.4877917169584975, -45.70509539860793780, 17.94068519067145928 ) ) ;
#22595=VERTEX_POINT ( 'NONE', #73420 ) ;
#22596=AXIS2_PLACEMENT_3D ( 'NONE', #28803, #23350, #85127 ) ;
#22597=VECTOR ( 'NONE', #72820, 1000.000000000000000 ) ;
#22600=ORIENTED_EDGE ( 'NONE', *, *, #49776, .F. ) ;
#22602=CARTESIAN_POINT ( 'NONE',  ( 117.0750736332619937, -31.98354782443029620, 64.19086337114899266 ) ) ;
#22603=ORIENTED_EDGE ( 'NONE', *, *, #54882, .F. ) ;
#22604=CARTESIAN_POINT ( 'NONE',  ( 115.7453557663426409, -41.23947501269460503, 288.4441967044829767 ) ) ;
#22605=CARTESIAN_POINT ( 'NONE',  ( 101.9739164908862961, -45.89159533563675808, 183.1727681330539781 ) ) ;
#22606=CARTESIAN_POINT ( 'NONE',  ( 165.6738106836042732, -28.98061976758451053, 313.9678068554149490 ) ) ;
#22608=CARTESIAN_POINT ( 'NONE',  ( 113.9169062821921727, -28.05502007051373070, 120.5565776568639507 ) ) ;
#22610=VERTEX_POINT ( 'NONE', #67057 ) ;
#22613=EDGE_LOOP ( 'NONE', ( #48117, #53434, #46357, #89816 ) ) ;
#22615=VERTEX_POINT ( 'NONE', #32520 ) ;
#22616=ADVANCED_FACE ( 'NONE', ( #3490 ), #52934, .T. ) ;
#22617=VERTEX_POINT ( 'NONE', #66151 ) ;
#22618=DIRECTION ( 'NONE',  ( 1.000000000000000000, 2.999999999999999839E-15, 1.000000000000000078E-15 ) ) ;
#22620=CARTESIAN_POINT ( 'NONE',  ( 101.3840881871039272, -27.98888560156178329, 25.53562527591096654 ) ) ;
#22621=LINE ( 'NONE', #70769, #11239 ) ;
#22623=ADVANCED_FACE ( 'NONE', ( #9870 ), #38895, .F. ) ;
#22626=EDGE_CURVE ( 'NONE', #5764, #19968, #30758, .T. ) ;
#22627=CARTESIAN_POINT ( 'NONE',  ( 97.00151786184777336, -41.45262973156714992, 61.67562527591097421 ) ) ;
#22628=CARTESIAN_POINT ( 'NONE',  ( 149.4430470701762772, -12.91565541735124256, 394.9756252759100903 ) ) ;
#22629=CARTESIAN_POINT ( 'NONE',  ( 117.6812658759004222, -39.72780374360937827, 139.6194347997199827 ) ) ;
#22631=CARTESIAN_POINT ( 'NONE',  ( 188.5667039024479834, -65.37844715994100397, 137.2178068554150059 ) ) ;
#22632=ORIENTED_EDGE ( 'NONE', *, *, #19246, .F. ) ;
#22633=CARTESIAN_POINT ( 'NONE',  ( 107.0664832912739257, -49.72944715994096043, 315.6356252759111953 ) ) ;
#22634=EDGE_CURVE ( 'NONE', #77176, #36098, #25269, .T. ) ;
#22637=ORIENTED_EDGE ( 'NONE', *, *, #9911, .T. ) ;
#22640=CARTESIAN_POINT ( 'NONE',  ( 107.9218747862861250, -47.19940893231376577, 177.6413395616249886 ) ) ;
#22641=EDGE_LOOP ( 'NONE', ( #28046, #22232, #27832, #63941 ) ) ;
#22643=DIRECTION ( 'NONE',  ( 0.7071067811865160424, 0.7071067811865791031, 0.000000000000000000 ) ) ;
#22644=CARTESIAN_POINT ( 'NONE',  ( 100.6242249862060731, -26.75349815150567778, 216.5327681330539633 ) ) ;
#22645=CARTESIAN_POINT ( 'NONE',  ( 98.29982688861167617, -42.45122269429050021, 97.78705384733993355 ) ) ;
#22649=EDGE_LOOP ( 'NONE', ( #66351, #38772, #74744, #62524 ) ) ;
#22650=ADVANCED_FACE ( 'NONE', ( #17133, #80704 ), #78922, .F. ) ;
#22651=CIRCLE ( 'NONE', #44331, 13.16666666666670160 ) ;
#22653=EDGE_CURVE ( 'NONE', #87303, #24776, #18453, .T. ) ;
#22656=FACE_OUTER_BOUND ( 'NONE', #85121, .T. ) ;
#22657=CARTESIAN_POINT ( 'NONE',  ( 115.4598468997141509, -29.53740796227222987, 225.4022919425769658 ) ) ;
#22658=LINE ( 'NONE', #50331, #6947 ) ;
#22660=ADVANCED_FACE ( 'NONE', ( #38018 ), #87509, .T. ) ;
#22661=CARTESIAN_POINT ( 'NONE',  ( 46.83715912545429205, -47.82818131006082751, 249.9678068554150343 ) ) ;
#22662=CARTESIAN_POINT ( 'NONE',  ( 107.8173249548519692, -46.71069529603006032, 277.6356222035115024 ) ) ;
#22665=CARTESIAN_POINT ( 'NONE',  ( 99.12668881670464316, -43.51958910750428089, 31.88991099019594699 ) ) ;
#22666=EDGE_LOOP ( 'NONE', ( #82162, #41997, #82084, #58423 ) ) ;
#22667=VERTEX_POINT ( 'NONE', #86623 ) ;
#22668=AXIS2_PLACEMENT_3D ( 'NONE', #63335, #1112, #7478 ) ;
#22670=VECTOR ( 'NONE', #38628, 1000.000000000000000 ) ;
#22671=CARTESIAN_POINT ( 'NONE',  ( 41.56648329127499153, -32.07844715994070839, 143.6756252759119832 ) ) ;
#22672=VECTOR ( 'NONE', #8264, 1000.000000000000000 ) ;
#22674=CARTESIAN_POINT ( 'NONE',  ( 106.8506556707825013, -46.50783423188139665, 268.5584824187674258 ) ) ;
#22676=CARTESIAN_POINT ( 'NONE',  ( 98.98846131648984681, -42.30253745798191289, 122.8070538473389490 ) ) ;
#22677=DIRECTION ( 'NONE',  ( 0.000000000000000000, 1.000000000000000000, 0.000000000000000000 ) ) ;
#22678=EDGE_LOOP ( 'NONE', ( #6471, #29423, #70987 ) ) ;
#22680=CARTESIAN_POINT ( 'NONE',  ( 77.33253968407632328, -36.38436945697863933, 3.076560175368444838 ) ) ;
#22682=ORIENTED_EDGE ( 'NONE', *, *, #11663, .F. ) ;
#22683=EDGE_CURVE ( 'NONE', #44005, #75042, #79819, .T. ) ;
#22686=CARTESIAN_POINT ( 'NONE',  ( 99.05427501747529107, -38.42862543901446060, 29.31094751244794949 ) ) ;
#22687=DIRECTION ( 'NONE',  ( 1.000000000000000078E-15, 1.000000000000000083E-30, -1.000000000000000000 ) ) ;
#22690=CARTESIAN_POINT ( 'NONE',  ( 142.8821648370248170, -72.54478064608022692, 394.9756252759102040 ) ) ;
#22692=CARTESIAN_POINT ( 'NONE',  ( 90.44969454456406766, -22.62993780205715311, 229.5838068554169809 ) ) ;
#22693=FACE_OUTER_BOUND ( 'NONE', #25412, .T. ) ;
#22695=CARTESIAN_POINT ( 'NONE',  ( 110.1579966911880888, -46.68583080861444756, 97.81562527591097478 ) ) ;
#22696=VERTEX_POINT ( 'NONE', #45688 ) ;
#22697=CARTESIAN_POINT ( 'NONE',  ( 109.8440526342893975, -45.34906309516006928, 57.25908649474392575 ) ) ;
#22698=CARTESIAN_POINT ( 'NONE',  ( 48.79742451361993716, -36.32844715994080786, 117.4678068554150485 ) ) ;
#22699=CARTESIAN_POINT ( 'NONE',  ( 112.1511370651177231, -26.84216853020813076, 169.6984824187689469 ) ) ;
#22701=DIRECTION ( 'NONE',  ( 0.7071067811865192621, 0.7071067811865758834, 7.071067811865185427E-16 ) ) ;
#22704=LINE ( 'NONE', #8626, #33420 ) ;
#22705=CARTESIAN_POINT ( 'NONE',  ( 117.5348948014565593, -36.80252384088669260, 259.8213395616249386 ) ) ;
#22706=VERTEX_POINT ( 'NONE', #75998 ) ;
#22707=EDGE_CURVE ( 'NONE', #32919, #33505, #35097, .T. ) ;
#22708=CARTESIAN_POINT ( 'NONE',  ( 48.45959712128998120, -28.98061976758942748, 342.9256252759109884 ) ) ;
#22710=CARTESIAN_POINT ( 'NONE',  ( 97.79748285543813324, -31.86337989110288405, 131.9413395616259947 ) ) ;
#22714=ORIENTED_EDGE ( 'NONE', *, *, #74307, .T. ) ;
#22715=CARTESIAN_POINT ( 'NONE',  ( 115.0372574689094023, -42.90846261676750828, 123.3022919376508071 ) ) ;
#22716=CARTESIAN_POINT ( 'NONE',  ( 97.81413906161476746, -40.51632882248723888, 267.6361360915977343 ) ) ;
#22718=CARTESIAN_POINT ( 'NONE',  ( 100.4501120178094453, -50.96720088627028389, 0.4256252759109639960 ) ) ;
#22719=LINE ( 'NONE', #77677, #9853 ) ;
#22720=CARTESIAN_POINT ( 'NONE',  ( 97.35162482889903401, -32.85093483786611301, 37.02419670448292521 ) ) ;
#22721=DIRECTION ( 'NONE',  ( 1.000000000000000000, 4.299999999999999979E-14, 1.000000000000000078E-15 ) ) ;
#22725=CARTESIAN_POINT ( 'NONE',  ( 105.7154676722796722, -46.72385723303512606, 42.46848526305529248 ) ) ;
#22726=VERTEX_POINT ( 'NONE', #20598 ) ;
#22727=ORIENTED_EDGE ( 'NONE', *, *, #72352, .F. ) ;
#22729=VECTOR ( 'NONE', #497, 1000.000000000000000 ) ;
#22730=CARTESIAN_POINT ( 'NONE',  ( 82.80053463576300032, -19.07423037057760240, 3.076719480831280329 ) ) ;
#22732=CARTESIAN_POINT ( 'NONE',  ( 61.56670390244727287, -23.42844715994043980, 300.4678068554150627 ) ) ;
#22733=DIRECTION ( 'NONE',  ( 0.000000000000000000, 0.000000000000000000, -1.000000000000000000 ) ) ;
#22735=ADVANCED_FACE ( 'NONE', ( #62804 ), #82837, .T. ) ;
#22737=CARTESIAN_POINT ( 'NONE',  ( 62.03715912545639100, -23.42818131006021787, 129.9678068554150911 ) ) ;
#22738=EDGE_CURVE ( 'NONE', #76957, #51167, #41216, .T. ) ;
#22739=CARTESIAN_POINT ( 'NONE',  ( 98.95796485450003388, -39.41423029504880304, 241.0038483995049603 ) ) ;
#22741=CARTESIAN_POINT ( 'NONE',  ( 98.73996931189277859, -42.96625968561437503, 62.83848241876793850 ) ) ;
#22742=CARTESIAN_POINT ( 'NONE',  ( 150.5667039024473866, -25.42844715993594562, 249.9678068554149490 ) ) ;
#22743=CARTESIAN_POINT ( 'NONE',  ( 95.43890296797121664, -34.19406290021405681, 106.1556252759109640 ) ) ;
#22744=EDGE_LOOP ( 'NONE', ( #5590, #79885 ) ) ;
#22745=LINE ( 'NONE', #50420, #24851 ) ;
#22746=VERTEX_POINT ( 'NONE', #55521 ) ;
#22748=FACE_BOUND ( 'NONE', #19124, .T. ) ;
#22749=CYLINDRICAL_SURFACE ( 'NONE', #78988, 2.749999999999974687 ) ;
#22750=VERTEX_POINT ( 'NONE', #583 ) ;
#22752=ADVANCED_FACE ( 'NONE', ( #18909 ), #83717, .T. ) ;
#22753=ORIENTED_EDGE ( 'NONE', *, *, #23933, .T. ) ;
#22754=CARTESIAN_POINT ( 'NONE',  ( 84.06648329127399677, -18.72966777111522063, 17.92562527591199739 ) ) ;
#22755=CARTESIAN_POINT ( 'NONE',  ( 98.30759644065037151, -41.72902612734809225, 272.7393669437288395 ) ) ;
#22756=AXIS2_PLACEMENT_3D ( 'NONE', #20141, #26948, #41010 ) ;
#22757=DIRECTION ( 'NONE',  ( -4.299999999999999979E-14, 1.000000000000000000, 0.000000000000000000 ) ) ;
#22759=CIRCLE ( 'NONE', #66643, 1.499999999999987788 ) ;
#22760=CARTESIAN_POINT ( 'NONE',  ( 97.24554646791794710, -31.60649478380229382, 90.93181575210196854 ) ) ;
#22762=DIRECTION ( 'NONE',  ( -4.237773401492740281E-14, 1.000000000000000000, 0.000000000000000000 ) ) ;
#22764=CARTESIAN_POINT ( 'NONE',  ( 142.8698897858160706, -0.9167816978817300289, 396.9756252759102040 ) ) ;
#22767=CARTESIAN_POINT ( 'NONE',  ( 114.0395979133839575, -29.51747486401405851, 120.4639116022243570 ) ) ;
#22768=CARTESIAN_POINT ( 'NONE',  ( 97.06107108209303647, -37.99641183811671397, 156.4272919325953239 ) ) ;
#22770=CARTESIAN_POINT ( 'NONE',  ( 114.7874576214283167, -44.67122033332078246, 114.2022919425779719 ) ) ;
#22771=CARTESIAN_POINT ( 'NONE',  ( 177.3246001664172695, -48.34074026909179622, 300.4678068554149490 ) ) ;
#22772=LINE ( 'NONE', #70920, #44155 ) ;
#22773=DIRECTION ( 'NONE',  ( -8.839355291601565315E-16, -1.000000000000000000, 0.000000000000000000 ) ) ;
#22775=EDGE_LOOP ( 'NONE', ( #40207, #17569, #24778, #2028 ) ) ;
#22776=CARTESIAN_POINT ( 'NONE',  ( 76.06670390244796920, -26.72944715994109899, 239.5838068554169809 ) ) ;
#22777=CARTESIAN_POINT ( 'NONE',  ( 114.4768422515204094, -30.34587328852060395, 180.3927681330529538 ) ) ;
#22780=CARTESIAN_POINT ( 'NONE',  ( 114.9268010244024225, -42.60560063232393446, 24.31562527591096767 ) ) ;
#22781=CARTESIAN_POINT ( 'NONE',  ( 88.17226027475679473, -58.72944715994100306, 239.5838068554174924 ) ) ;
#22782=CARTESIAN_POINT ( 'NONE',  ( 156.5667039024482676, -42.82844715993568485, 259.7178068554149490 ) ) ;
#22785=DIRECTION ( 'NONE',  ( -1.000000000000000078E-15, 1.000000000000000083E-30, 1.000000000000000000 ) ) ;
#22787=CARTESIAN_POINT ( 'NONE',  ( 116.2522929705883712, -40.08866370952549829, 218.5470538473399529 ) ) ;
#22788=VERTEX_POINT ( 'NONE', #7406 ) ;
#22791=CARTESIAN_POINT ( 'NONE',  ( 112.6322303140947838, -44.29905650357037672, 179.5006309249449430 ) ) ;
#22792=VECTOR ( 'NONE', #83745, 1000.000000000000000 ) ;
#22795=CARTESIAN_POINT ( 'NONE',  ( 102.7262891916532084, -29.00345248032369483, 56.91586902018297423 ) ) ;
#22796=VECTOR ( 'NONE', #33053, 1000.000000000000000 ) ;
#22798=EDGE_CURVE ( 'NONE', #67480, #15446, #13775, .T. ) ;
#22799=CARTESIAN_POINT ( 'NONE',  ( 104.4076873786489159, -46.45796789277314076, 267.3648837029242600 ) ) ;
#22800=CARTESIAN_POINT ( 'NONE',  ( 85.35814995794051185, 12.92155284005802685, 335.5992267699911054 ) ) ;
#22801=ORIENTED_EDGE ( 'NONE', *, *, #19498, .T. ) ;
#22802=PLANE ( 'NONE',  #53 ) ;
#22803=DIRECTION ( 'NONE',  ( 0.7071067811575898476, -0.7071067812155052978, 0.000000000000000000 ) ) ;
#22804=CARTESIAN_POINT ( 'NONE',  ( 99.41296134609922319, -28.78668791560518514, 265.6746728949588032 ) ) ;
#22805=CARTESIAN_POINT ( 'NONE',  ( 97.60818021318179660, -39.98327219696195556, 171.5903219849872698 ) ) ;
#22806=EDGE_LOOP ( 'NONE', ( #88053, #78577 ) ) ;
#22807=EDGE_LOOP ( 'NONE', ( #46592, #27072, #15871, #40206 ) ) ;
#22810=CARTESIAN_POINT ( 'NONE',  ( 97.86644135638643149, -40.64890597622355273, 122.6464849464893945 ) ) ;
#22813=AXIS2_PLACEMENT_3D ( 'NONE', #41343, #54066, #48157 ) ;
#22814=CARTESIAN_POINT ( 'NONE',  ( 112.4622727538958316, -27.87370092883246286, 45.62895860924398761 ) ) ;
#22817=ADVANCED_FACE ( 'NONE', ( #13333 ), #21494, .T. ) ;
#22818=CARTESIAN_POINT ( 'NONE',  ( 100.9155127638074703, -46.91653085812070856, 48.14419670448194211 ) ) ;
#22819=CARTESIAN_POINT ( 'NONE',  ( 188.5667039024482960, -48.82844715993431350, 259.7178068554150059 ) ) ;
#22820=CARTESIAN_POINT ( 'NONE',  ( 116.5366478410923463, -42.42989196264584706, 278.3832443235298797 ) ) ;
#22821=ORIENTED_EDGE ( 'NONE', *, *, #87919, .F. ) ;
#22825=CARTESIAN_POINT ( 'NONE',  ( 98.00070950526129820, -34.75266269402447250, 103.9738046553059547 ) ) ;
#22826=CARTESIAN_POINT ( 'NONE',  ( 101.4135918642175369, -46.25467808933209568, 203.1622919425779514 ) ) ;
#22827=DIRECTION ( 'NONE',  ( 0.000000000000000000, 1.000000000000000000, 0.000000000000000000 ) ) ;
#22828=ORIENTED_EDGE ( 'NONE', *, *, #17511, .F. ) ;
#22829=CARTESIAN_POINT ( 'NONE',  ( 51.06648329127400388, 25.62155284005901379, 333.4006252759110112 ) ) ;
#22831=AXIS2_PLACEMENT_3D ( 'NONE', #79295, #17054, #73795 ) ;
#22833=DIRECTION ( 'NONE',  ( -6.524622321627019585E-16, -3.741823817616790462E-31, -1.000000000000000000 ) ) ;
#22834=EDGE_LOOP ( 'NONE', ( #70701, #38384, #38052, #11439 ) ) ;
#22835=ORIENTED_EDGE ( 'NONE', *, *, #57005, .T. ) ;
#22837=CARTESIAN_POINT ( 'NONE',  ( 107.7709757720581649, -26.73284657607137405, 41.02040754495594399 ) ) ;
#22838=ADVANCED_FACE ( 'NONE', ( #7850 ), #25722, .F. ) ;
#22839=CARTESIAN_POINT ( 'NONE',  ( 108.4402549024021312, -27.77817906387560143, 144.3657531614099412 ) ) ;
#22840=CARTESIAN_POINT ( 'NONE',  ( 99.31672145811513985, -28.81511631862888123, 270.7051490854347549 ) ) ;
#22841=EDGE_CURVE ( 'NONE', #88945, #74932, #42350, .T. ) ;
#22842=LINE ( 'NONE', #85075, #19450 ) ;
#22844=ORIENTED_EDGE ( 'NONE', *, *, #27141, .T. ) ;
#22846=ORIENTED_EDGE ( 'NONE', *, *, #61192, .F. ) ;
#22848=CIRCLE ( 'NONE', #15650, 1.000000000000000888 ) ;
#22850=CARTESIAN_POINT ( 'NONE',  ( 142.8832909413445122, -79.11588146349311046, 361.9756252759100335 ) ) ;
#22851=CARTESIAN_POINT ( 'NONE',  ( 111.0995558192250456, -25.53287967237518430, 99.80133956162498521 ) ) ;
#22852=VECTOR ( 'NONE', #80964, 1000.000000000000000 ) ;
#22854=ORIENTED_EDGE ( 'NONE', *, *, #78349, .T. ) ;
#22855=CIRCLE ( 'NONE', #37302, 13.50000000000000533 ) ;
#22856=CARTESIAN_POINT ( 'NONE',  ( 110.7331673686684610, -26.30186281216086996, 254.8194347997205682 ) ) ;
#22857=DIRECTION ( 'NONE',  ( 0.000000000000000000, 1.000000000000000000, 0.000000000000000000 ) ) ;
#22859=CARTESIAN_POINT ( 'NONE',  ( 45.77381068350376125, -48.62134037888161231, 180.4678068554150911 ) ) ;
#22860=DIRECTION ( 'NONE',  ( 1.000000000000000078E-15, -1.000000000000000083E-30, -1.000000000000000000 ) ) ;
#22863=PLANE ( 'NONE',  #26408 ) ;
#22864=CYLINDRICAL_SURFACE ( 'NONE', #55352, 2.500000000000002220 ) ;
#22865=LINE ( 'NONE', #51864, #17952 ) ;
#22869=DIRECTION ( 'NONE',  ( 2.900000000000000265E-14, -2.000000000000000155E-15, 1.000000000000000000 ) ) ;
#22870=CARTESIAN_POINT ( 'NONE',  ( 31.71315051186898870, -31.94127993907790852, -5.074374724088000832 ) ) ;
#22872=VERTEX_POINT ( 'NONE', #1944 ) ;
#22873=LINE ( 'NONE', #78290, #17713 ) ;
#22874=CARTESIAN_POINT ( 'NONE',  ( 105.1555015486555078, -47.05240725173535310, 12.42991099019596923 ) ) ;
#22875=CARTESIAN_POINT ( 'NONE',  ( 104.5626002042890974, -48.31241677248981858, 178.4070538473399665 ) ) ;
#22876=CARTESIAN_POINT ( 'NONE',  ( 111.1374431767090414, -47.03053892029802796, 18.88800622829195319 ) ) ;
#22877=VECTOR ( 'NONE', #80891, 1000.000000000000000 ) ;
#22879=LINE ( 'NONE', #76936, #33392 ) ;
#22884=LINE ( 'NONE', #63762, #70832 ) ;
#22886=CARTESIAN_POINT ( 'NONE',  ( 116.6363502066642468, -38.74961609181404043, 59.66133956162394725 ) ) ;
#22887=DIRECTION ( 'NONE',  ( 1.000000000000000078E-15, 1.000000000000000083E-30, -1.000000000000000000 ) ) ;
#22889=CARTESIAN_POINT ( 'NONE',  ( 101.9934276907083444, -45.44595233133192380, 48.15644075925013823 ) ) ;
#22890=CARTESIAN_POINT ( 'NONE',  ( 108.1794352217186201, -47.07304438381563472, 198.6613395616249989 ) ) ;
#22892=CARTESIAN_POINT ( 'NONE',  ( 98.54783405468135982, -41.97727565318817966, 146.7658588207967796 ) ) ;
#22893=DIRECTION ( 'NONE',  ( -0.000000000000000000, -0.000000000000000000, 1.000000000000000000 ) ) ;
#22894=LINE ( 'NONE', #77396, #68829 ) ;
#22895=FACE_OUTER_BOUND ( 'NONE', #58720, .T. ) ;
#22896=CARTESIAN_POINT ( 'NONE',  ( 111.0136030271875285, -45.91768036457248314, 97.89935017080178170 ) ) ;
#22897=CARTESIAN_POINT ( 'NONE',  ( 98.36735121233621726, -42.37464764417353535, 146.7965776568640024 ) ) ;
#22898=ORIENTED_EDGE ( 'NONE', *, *, #4635, .T. ) ;
#22900=ADVANCED_FACE ( 'NONE', ( #50066 ), #36467, .T. ) ;
#22901=VECTOR ( 'NONE', #75879, 1000.000000000000000 ) ;
#22902=CARTESIAN_POINT ( 'NONE',  ( 115.8905597133153549, -37.54428082998141747, 75.18444044875394638 ) ) ;
#22904=CARTESIAN_POINT ( 'NONE',  ( 114.1395267584829014, -29.97404255306821241, 230.4327681330529742 ) ) ;
#22905=LINE ( 'NONE', #17414, #23073 ) ;
#22906=CARTESIAN_POINT ( 'NONE',  ( 36.23715912545430484, -47.82818131006125384, 237.4678068554150059 ) ) ;
#22910=CARTESIAN_POINT ( 'NONE',  ( 21.56670390244635271, -23.42844715994195326, 117.4678068554150343 ) ) ;
#22912=CARTESIAN_POINT ( 'NONE',  ( 114.4473569665854313, -28.53271593493105485, 159.5051490854349652 ) ) ;
#22914=ORIENTED_EDGE ( 'NONE', *, *, #27206, .T. ) ;
#22915=ORIENTED_EDGE ( 'NONE', *, *, #89073, .F. ) ;
#22918=CARTESIAN_POINT ( 'NONE',  ( 97.78494223251618678, -40.45150674683588932, 131.6299638674549897 ) ) ;
#22920=CARTESIAN_POINT ( 'NONE',  ( 111.7906875226637879, -43.98084836425640276, 220.8661856076869583 ) ) ;
#22921=CIRCLE ( 'NONE', #34493, 11.45913725231036118 ) ;
#22922=VECTOR ( 'NONE', #52, 1000.000000000000000 ) ;
#22923=EDGE_CURVE ( 'NONE', #37352, #12546, #56885, .T. ) ;
#22925=CARTESIAN_POINT ( 'NONE',  ( 95.67500926166044906, -33.46221576448694890, 141.1041967044829732 ) ) ;
#22927=VERTEX_POINT ( 'NONE', #72327 ) ;
#22928=VERTEX_POINT ( 'NONE', #9644 ) ;
#22929=ORIENTED_EDGE ( 'NONE', *, *, #36908, .T. ) ;
#22930=B_SPLINE_CURVE_WITH_KNOTS ( 'NONE', 3,
 ( #68481, #62882, #56053, #50142, #28831, #77423, #42877, #70611, #56963, #84704, #22467, #36976, #24245, #31483, #9722, #86040, #58313, #23809 ),
 .UNSPECIFIED., .F., .F.,
 ( 4, 2, 2, 2, 2, 2, 2, 2, 4 ),
 ( 0.000000000000000000, 0.06250000004081082694, 0.1250000000816216539, 0.1875000001224324808, 0.2500000001632433078, 0.3125000002040541069, 0.3750000002448649616, 0.4375000002856758163, 0.5000000003264866155 ),
 .UNSPECIFIED. ) ;
#22931=AXIS2_PLACEMENT_3D ( 'NONE', #77091, #84811, #48895 ) ;
#22932=LINE ( 'NONE', #7498, #21563 ) ;
#22933=ORIENTED_EDGE ( 'NONE', *, *, #30837, .T. ) ;
#22936=DIRECTION ( 'NONE',  ( -4.237773401492740281E-14, 1.000000000000000000, 0.000000000000000000 ) ) ;
#22937=CARTESIAN_POINT ( 'NONE',  ( 100.4929819111635538, -30.01635508975405031, 267.1368214011352507 ) ) ;
#22940=CARTESIAN_POINT ( 'NONE',  ( 109.6430113662638064, -46.48008694528652995, 272.7814585466231847 ) ) ;
#22943=VECTOR ( 'NONE', #62716, 1000.000000000000114 ) ;
#22944=CARTESIAN_POINT ( 'NONE',  ( 111.4213356664735386, -44.07558929780552148, 9.635625275910941312 ) ) ;
#22945=DIRECTION ( 'NONE',  ( 0.000000000000000000, 0.000000000000000000, -1.000000000000000000 ) ) ;
#22946=EDGE_LOOP ( 'NONE', ( #45727, #89350 ) ) ;
#22949=CARTESIAN_POINT ( 'NONE',  ( 116.9125557316235557, -38.73407091525943002, 113.6668860931665108 ) ) ;
#22951=EDGE_LOOP ( 'NONE', ( #25198, #82846, #61046, #10950 ) ) ;
#22952=ADVANCED_FACE ( 'NONE', ( #22387 ), #51401, .T. ) ;
#22953=CIRCLE ( 'NONE', #44699, 2.117000000000000881 ) ;
#22954=CARTESIAN_POINT ( 'NONE',  ( 114.3408732721816534, -41.20596775705023163, 17.80956268521999419 ) ) ;
#22955=CARTESIAN_POINT ( 'NONE',  ( 114.2686970495659295, -44.29742072815643184, 158.1813395616249807 ) ) ;
#22956=CARTESIAN_POINT ( 'NONE',  ( 117.5859182825552978, -33.41202194707543782, 129.0575300378159795 ) ) ;
#22957=CARTESIAN_POINT ( 'NONE',  ( 194.5667039024479834, -48.82844715994099971, 300.9178068554150514 ) ) ;
#22958=CARTESIAN_POINT ( 'NONE',  ( 97.47313694375068849, -40.89946378256092174, 227.6527681330539679 ) ) ;
#22964=ORIENTED_EDGE ( 'NONE', *, *, #49533, .F. ) ;
#22965=ORIENTED_EDGE ( 'NONE', *, *, #5335, .F. ) ;
#22967=CARTESIAN_POINT ( 'NONE',  ( 107.2439172579031919, -47.23279478401654075, 212.5899109901969837 ) ) ;
#22969=CARTESIAN_POINT ( 'NONE',  ( 117.4874684240972300, -40.41484487456647656, 178.5680062282919778 ) ) ;
#22970=LINE ( 'NONE', #35222, #42751 ) ;
#22971=CARTESIAN_POINT ( 'NONE',  ( 134.4383386548979331, -33.97944715994099596, 8.225625275910996237 ) ) ;
#22972=CARTESIAN_POINT ( 'NONE',  ( 32.25690895537066183, -33.54226604285041446, 313.9678068554150059 ) ) ;
#22974=CARTESIAN_POINT ( 'NONE',  ( 107.0664832912739399, -36.72944715994095333, 290.1356252759106837 ) ) ;
#22975=CARTESIAN_POINT ( 'NONE',  ( 101.3060704567421624, -26.40153104436181053, 251.4813395616249920 ) ) ;
#22978=CARTESIAN_POINT ( 'NONE',  ( 97.06115611282757527, -37.99685616894899454, 272.4268914305668545 ) ) ;
#22979=EDGE_CURVE ( 'NONE', #29605, #17228, #22842, .T. ) ;
#22980=DIRECTION ( 'NONE',  ( -0.7071067811865170416, -0.7071067811865778818, -7.071067811865474347E-16 ) ) ;
#22981=EDGE_CURVE ( 'NONE', #44492, #44045, #64173, .T. ) ;
#22982=CARTESIAN_POINT ( 'NONE',  ( 102.0670549422599294, -27.97049806924179549, 256.4897919441917793 ) ) ;
#22983=CARTESIAN_POINT ( 'NONE',  ( 107.0664832912739968, -36.72944715994100306, 287.6356252759109680 ) ) ;
#22984=CARTESIAN_POINT ( 'NONE',  ( 98.59159163785028568, -35.76670619840676579, 195.5838068554172082 ) ) ;
#22985=ORIENTED_EDGE ( 'NONE', *, *, #38503, .F. ) ;
#22987=CARTESIAN_POINT ( 'NONE',  ( 97.74263787230347589, -41.52050856888216401, 196.7041967044819728 ) ) ;
#22988=CARTESIAN_POINT ( 'NONE',  ( 106.6603377114791300, -26.31227224467070158, 81.10705384733896040 ) ) ;
#22989=CARTESIAN_POINT ( 'NONE',  ( 117.1100247017212723, -39.68245506451066262, 179.5984824187679294 ) ) ;
#22991=DIRECTION ( 'NONE',  ( 0.000000000000000000, 0.000000000000000000, 1.000000000000000000 ) ) ;
#22992=DIRECTION ( 'NONE',  ( 1.000000000000000000, 4.163336342344333240E-14, 0.000000000000000000 ) ) ;
#22993=CARTESIAN_POINT ( 'NONE',  ( 182.0374245136140132, -23.42844715993459559, 313.9678068554149490 ) ) ;
#22996=EDGE_LOOP ( 'NONE', ( #48629, #80672, #68449, #19435, #80218, #10306 ) ) ;
#22998=CIRCLE ( 'NONE', #88212, 4.749999999999976907 ) ;
#23001=ORIENTED_EDGE ( 'NONE', *, *, #66951, .F. ) ;
#23002=CARTESIAN_POINT ( 'NONE',  ( 113.3792027166817320, -43.22269317268541755, 117.6248007804579458 ) ) ;
#23005=VERTEX_POINT ( 'NONE', #71443 ) ;
#23006=CARTESIAN_POINT ( 'NONE',  ( 112.7897778137181746, -47.07797880090539167, 98.97848241876793907 ) ) ;
#23007=CARTESIAN_POINT ( 'NONE',  ( 180.3521107875639871, -35.65087443492551245, -5.074374724088000832 ) ) ;
#23009=DIRECTION ( 'NONE',  ( 4.299999999999999979E-14, -1.000000000000000000, 4.400000000000000367E-29 ) ) ;
#23010=CYLINDRICAL_SURFACE ( 'NONE', #50557, 2.750000000000002665 ) ;
#23011=VECTOR ( 'NONE', #58842, 1000.000000000000000 ) ;
#23013=CARTESIAN_POINT ( 'NONE',  ( 100.8224265971272615, -29.20115443902020047, 40.62705384733994407 ) ) ;
#23014=ORIENTED_EDGE ( 'NONE', *, *, #1441, .T. ) ;
#23016=VERTEX_POINT ( 'NONE', #43251 ) ;
#23017=DIRECTION ( 'NONE',  ( -1.500809167996645702E-15, 0.7071067811865391350, 0.7071067811865560104 ) ) ;
#23022=DIRECTION ( 'NONE',  ( 0.000000000000000000, 0.000000000000000000, -1.000000000000000000 ) ) ;
#23024=VECTOR ( 'NONE', #25838, 1000.000000000000000 ) ;
#23027=CARTESIAN_POINT ( 'NONE',  ( 115.9265467165008232, -42.18176083994495684, 18.38705384733896153 ) ) ;
#23028=ORIENTED_EDGE ( 'NONE', *, *, #4088, .T. ) ;
#23029=CARTESIAN_POINT ( 'NONE',  ( 97.31584336463156149, -39.30597463869850117, 271.5314584984529347 ) ) ;
#23031=PLANE ( 'NONE',  #88839 ) ;
#23032=CARTESIAN_POINT ( 'NONE',  ( 108.9785397593094132, -44.66504833944034658, 130.5823760838769658 ) ) ;
#23033=VECTOR ( 'NONE', #66209, 1000.000000000000000 ) ;
#23035=EDGE_CURVE ( 'NONE', #35978, #68568, #39737, .T. ) ;
#23036=LINE ( 'NONE', #69157, #3522 ) ;
#23038=VERTEX_POINT ( 'NONE', #60003 ) ;
#23039=ORIENTED_EDGE ( 'NONE', *, *, #45907, .T. ) ;
#23041=CARTESIAN_POINT ( 'NONE',  ( 21.56670390244701707, -23.42844715994183957, 249.9678068554150059 ) ) ;
#23042=ORIENTED_EDGE ( 'NONE', *, *, #40737, .T. ) ;
#23045=CARTESIAN_POINT ( 'NONE',  ( 102.7466871476783581, -44.50128676613118728, 183.6044404487539623 ) ) ;
#23047=EDGE_CURVE ( 'NONE', #8827, #20097, #87735, .T. ) ;
#23048=CYLINDRICAL_SURFACE ( 'NONE', #61217, 1.000000000002049694 ) ;
#23049=CARTESIAN_POINT ( 'NONE',  ( 108.0361718062294614, -25.69563957016125855, 105.9946728949589811 ) ) ;
#23050=CARTESIAN_POINT ( 'NONE',  ( 108.4174893140138352, -26.73503593703446057, 119.9689586043175211 ) ) ;
#23051=ADVANCED_FACE ( 'NONE', ( #45476 ), #80484, .T. ) ;
#23052=CARTESIAN_POINT ( 'NONE',  ( 110.8537921787340252, -45.98451557629201147, 17.88556681916309898 ) ) ;
#23056=ORIENTED_EDGE ( 'NONE', *, *, #37824, .F. ) ;
#23058=ADVANCED_FACE ( 'NONE', ( #19147 ), #86850, .F. ) ;
#23059=CARTESIAN_POINT ( 'NONE',  ( 114.8623915286450199, -39.24071799505598079, 156.3966617981629668 ) ) ;
#23060=VECTOR ( 'NONE', #22701, 1000.000000000000000 ) ;
#23061=CARTESIAN_POINT ( 'NONE',  ( 103.9507802182147600, -47.35902078718802954, 62.33753003781600199 ) ) ;
#23062=ORIENTED_EDGE ( 'NONE', *, *, #57983, .F. ) ;
#23063=CARTESIAN_POINT ( 'NONE',  ( 101.3960830062750063, -28.00733582429760204, 25.53562527591096654 ) ) ;
#23064=CARTESIAN_POINT ( 'NONE',  ( 97.65507918845807467, -41.26406199109977280, 167.6841967044829573 ) ) ;
#23065=EDGE_CURVE ( 'NONE', #16664, #86561, #53628, .T. ) ;
#23066=B_SPLINE_CURVE_WITH_KNOTS ( 'NONE', 3,
 ( #39776, #60668, #40228, #32972, #6619, #5735, #89754, #13438, #26168, #55629, #34768, #75216, #53836, #34315, #55181, #33425, #89302, #88855, #62472, #82941, #68848, #81606, #12092, #83377, #48369, #76103, #74763, #13882, #12542, #26609, #67489 ),
 .UNSPECIFIED., .F., .F.,
 ( 4, 2, 2, 1, 2, 2, 2, 2, 2, 2, 2, 1, 1, 2, 2, 2, 4 ),
 ( 0.000000000000000000, 0.1249999999999597267, 0.1874999999999392708, 0.2187499999999290290, 0.2343749999999237554, 0.2499999999999185096, 0.3749999999999280575, 0.4374999999999334421, 0.4999999999999388267, 0.6249999999999505951, 0.6874999999999609201, 0.7187499999999670264, 0.7343749999999702460, 0.7421874999999727995, 0.7499999999999753530, 0.8749999999999876765, 1.000000000000000000 ),
 .UNSPECIFIED. ) ;
#23069=CARTESIAN_POINT ( 'NONE',  ( 98.84006766826026080, -28.19945879207355688, 111.6870538473389587 ) ) ;
#23070=EDGE_CURVE ( 'NONE', #83877, #32492, #46821, .T. ) ;
#23071=DIRECTION ( 'NONE',  ( 0.000000000000000000, 0.000000000000000000, 1.000000000000000000 ) ) ;
#23072=ORIENTED_EDGE ( 'NONE', *, *, #302, .T. ) ;
#23073=VECTOR ( 'NONE', #45097, 999.9999999999998863 ) ;
#23075=ORIENTED_EDGE ( 'NONE', *, *, #48631, .F. ) ;
#23077=CARTESIAN_POINT ( 'NONE',  ( 116.7954517155124563, -39.38667583240329151, 134.6155541235699786 ) ) ;
#23082=CARTESIAN_POINT ( 'NONE',  ( 117.0539912639601852, -31.99354471700374702, 64.19086337114899266 ) ) ;
#23085=CARTESIAN_POINT ( 'NONE',  ( 71.25416588882602298, -72.55705569728901594, 540.9756252759101471 ) ) ;
#23086=CARTESIAN_POINT ( 'NONE',  ( 111.6283393632454448, -28.07768985461828848, 59.68991099019693536 ) ) ;
#23087=DIRECTION ( 'NONE',  ( 0.000000000000000000, 0.000000000000000000, -1.000000000000000000 ) ) ;
#23088=CARTESIAN_POINT ( 'NONE',  ( 101.7806060443209049, -45.68981339355057969, 158.1527681330539963 ) ) ;
#23090=CARTESIAN_POINT ( 'NONE',  ( 51.24204729617298426, -31.76306994223730840, -5.074374724088000832 ) ) ;
#23092=AXIS2_PLACEMENT_3D ( 'NONE', #26285, #19024, #60342 ) ;
#23093=CARTESIAN_POINT ( 'NONE',  ( 167.2371591254543262, -47.82818131005522844, 237.4678068554150059 ) ) ;
#23095=CARTESIAN_POINT ( 'NONE',  ( 116.3176178399231873, -32.93748434060082531, 55.13562527591098217 ) ) ;
#23099=LINE ( 'NONE', #85324, #52000 ) ;
#23100=CARTESIAN_POINT ( 'NONE',  ( 109.6166107820099569, -26.53883167775938645, 199.8813395616249977 ) ) ;
#23101=VERTEX_POINT ( 'NONE', #35000 ) ;
#23102=CARTESIAN_POINT ( 'NONE',  ( 179.4595971212720258, -26.00627455219131789, -5.074374724088000832 ) ) ;
#23103=CARTESIAN_POINT ( 'NONE',  ( 116.6256809191353909, -40.94358996305180654, 249.4956252759109532 ) ) ;
#23104=CARTESIAN_POINT ( 'NONE',  ( 101.4776230940428832, -27.87746311998561666, 106.5241967044819944 ) ) ;
#23107=CARTESIAN_POINT ( 'NONE',  ( 104.4880348644471724, -26.97933548612494903, 191.2814020040040930 ) ) ;
#23111=ORIENTED_EDGE ( 'NONE', *, *, #37857, .F. ) ;
#23112=ORIENTED_EDGE ( 'NONE', *, *, #70006, .T. ) ;
#23114=DIRECTION ( 'NONE',  ( 0.000000000000000000, 0.000000000000000000, 1.000000000000000000 ) ) ;
#23115=CARTESIAN_POINT ( 'NONE',  ( 96.91437895093065436, -34.20831442473366479, 272.1327681330538439 ) ) ;
#23117=CARTESIAN_POINT ( 'NONE',  ( 131.3165191078497855, -36.55813574389619447, 3.101427645695960411 ) ) ;
#23119=DIRECTION ( 'NONE',  ( -0.7071067812160279908, 0.7071067811570671546, -2.899137802744091193E-29 ) ) ;
#23122=CARTESIAN_POINT ( 'NONE',  ( 113.9904334582008545, -30.89236017996071837, 223.7943245899819829 ) ) ;
#23123=ORIENTED_EDGE ( 'NONE', *, *, #8384, .F. ) ;
#23127=FACE_BOUND ( 'NONE', #39204, .T. ) ;
#23128=CARTESIAN_POINT ( 'NONE',  ( 130.0664832912740110, -18.82844715994099971, 17.92562527591199739 ) ) ;
#23129=CARTESIAN_POINT ( 'NONE',  ( 112.0124476237220676, -28.73397683645143275, 285.6356252759109680 ) ) ;
#23130=LINE ( 'NONE', #63542, #15354 ) ;
#23132=CARTESIAN_POINT ( 'NONE',  ( 116.9310496459149391, -33.53114825773884178, 130.0880062282909648 ) ) ;
#23135=EDGE_LOOP ( 'NONE', ( #25322, #61329 ) ) ;
#23136=DIRECTION ( 'NONE',  ( -2.999999999999999839E-15, 1.000000000000000000, -2.999999999999999900E-30 ) ) ;
#23137=DIRECTION ( 'NONE',  ( 1.000000000000000000, 0.000000000000000000, 0.000000000000000000 ) ) ;
#23140=DIRECTION ( 'NONE',  ( 0.000000000000000000, 1.000000000000000000, 0.000000000000000000 ) ) ;
#23141=CARTESIAN_POINT ( 'NONE',  ( 116.0742395100671871, -34.51300936444170020, 11.83666179816295028 ) ) ;
#23143=EDGE_CURVE ( 'NONE', #66655, #6347, #61360, .T. ) ;
#23144=EDGE_CURVE ( 'NONE', #88451, #79790, #75903, .T. ) ;
#23147=VECTOR ( 'NONE', #18574, 1000.000000000000000 ) ;
#23148=CARTESIAN_POINT ( 'NONE',  ( 117.0608701673778000, -38.08062519847543115, 194.7189615153010323 ) ) ;
#23149=ORIENTED_EDGE ( 'NONE', *, *, #53149, .F. ) ;
#23152=DIRECTION ( 'NONE',  ( 0.000000000000000000, 1.000000000000000000, 0.000000000000000000 ) ) ;
#23154=CARTESIAN_POINT ( 'NONE',  ( 107.2322097935746541, -25.67722466037449536, 80.07657765686299456 ) ) ;
#23155=VERTEX_POINT ( 'NONE', #49064 ) ;
#23156=CARTESIAN_POINT ( 'NONE',  ( 109.7746843348460857, -45.37110888865593239, 52.22861030426695095 ) ) ;
#23157=EDGE_CURVE ( 'NONE', #57151, #48918, #32472, .T. ) ;
#23158=CARTESIAN_POINT ( 'NONE',  ( 112.0396642006261629, -45.43305334282853636, 88.98868781504944536 ) ) ;
#23159=CARTESIAN_POINT ( 'NONE',  ( 108.7386892141029477, -46.36620816325537930, 167.7127681330539701 ) ) ;
#23161=EDGE_CURVE ( 'NONE', #70284, #24618, #27746, .T. ) ;
#23162=DIRECTION ( 'NONE',  ( -0.000000000000000000, 1.000000000000000000, 0.000000000000000000 ) ) ;
#23164=AXIS2_PLACEMENT_3D ( 'NONE', #89826, #82569, #39848 ) ;
#23165=CARTESIAN_POINT ( 'NONE',  ( 111.7933198282062364, -46.77516514641244783, 283.9146728949586418 ) ) ;
#23167=ADVANCED_FACE ( 'NONE', ( #55429 ), #49518, .T. ) ;
#23168=ORIENTED_EDGE ( 'NONE', *, *, #78750, .F. ) ;
#23169=DIRECTION ( 'NONE',  ( 0.9834602067019604377, 0.1811243270069963496, 0.000000000000000000 ) ) ;
#23170=EDGE_LOOP ( 'NONE', ( #12626, #71446, #68115, #67746, #19481 ) ) ;
#23171=CARTESIAN_POINT ( 'NONE',  ( 112.1411864721344642, -47.49320580990715968, 133.9270538473399768 ) ) ;
#23174=VERTEX_POINT ( 'NONE', #40479 ) ;
#23175=ORIENTED_EDGE ( 'NONE', *, *, #13406, .F. ) ;
#23176=EDGE_CURVE ( 'NONE', #46082, #10162, #68196, .T. ) ;
#23178=CYLINDRICAL_SURFACE ( 'NONE', #55041, 9.999999999999998224 ) ;
#23179=AXIS2_PLACEMENT_3D ( 'NONE', #83676, #20992, #48669 ) ;
#23180=FACE_OUTER_BOUND ( 'NONE', #74332, .T. ) ;
#23181=CARTESIAN_POINT ( 'NONE',  ( 98.48461633480658861, -41.42146110206444121, 221.7241967044829494 ) ) ;
#23183=PLANE ( 'NONE',  #87265 ) ;
#23185=CARTESIAN_POINT ( 'NONE',  ( 98.42378885047078541, -42.06819960529416136, 7.768006228291934434 ) ) ;
#23186=EDGE_CURVE ( 'NONE', #15468, #71887, #83180, .T. ) ;
#23188=ORIENTED_EDGE ( 'NONE', *, *, #44679, .F. ) ;
#23189=CARTESIAN_POINT ( 'NONE',  ( 103.3374434664356869, -27.45071444193263588, 171.3805643286247573 ) ) ;
#23190=CIRCLE ( 'NONE', #73920, 0.5000000000000004441 ) ;
#23193=ORIENTED_EDGE ( 'NONE', *, *, #36979, .F. ) ;
#23194=VECTOR ( 'NONE', #28515, 1000.000000000000000 ) ;
#23195=VECTOR ( 'NONE', #88727, 1000.000000000000000 ) ;
#23196=DIRECTION ( 'NONE',  ( 1.000000000000000000, 0.000000000000000000, 0.000000000000000000 ) ) ;
#23197=LINE ( 'NONE', #76787, #71610 ) ;
#23198=CARTESIAN_POINT ( 'NONE',  ( 96.21411768969875311, -32.03111041547175120, 211.0013395616249738 ) ) ;
#23199=FACE_BOUND ( 'NONE', #37981, .T. ) ;
#23200=DIRECTION ( 'NONE',  ( -1.000000000000000000, -3.999999999999999995E-14, -1.000000000000000078E-15 ) ) ;
#23201=CARTESIAN_POINT ( 'NONE',  ( 116.0662231142348162, -35.72080775710429634, 233.3257531614099776 ) ) ;
#23202=CYLINDRICAL_SURFACE ( 'NONE', #5479, 0.2500000000000002220 ) ;
#23203=CARTESIAN_POINT ( 'NONE',  ( 115.6551466294303054, -43.65033472170370032, 39.27467289495895386 ) ) ;
#23204=CARTESIAN_POINT ( 'NONE',  ( 41.56648329127499153, -36.32844715994070839, 263.6756252759120116 ) ) ;
#23205=CARTESIAN_POINT ( 'NONE',  ( 109.7815504499144339, -47.49240650911489325, 92.78514908543495210 ) ) ;
#23206=ORIENTED_EDGE ( 'NONE', *, *, #71346, .F. ) ;
#23207=CARTESIAN_POINT ( 'NONE',  ( 131.6545875264049528, -20.05177997654004685, 7.178113714829589043 ) ) ;
#23208=VERTEX_POINT ( 'NONE', #49968 ) ;
#23209=VECTOR ( 'NONE', #84276, 1000.000000000000000 ) ;
#23210=DIRECTION ( 'NONE',  ( -1.000000000000000078E-15, 1.000000000000000083E-30, 1.000000000000000000 ) ) ;
#23211=CARTESIAN_POINT ( 'NONE',  ( 103.2774390132985047, -27.47508908009983841, 276.3857178017252068 ) ) ;
#23212=ORIENTED_EDGE ( 'NONE', *, *, #20870, .F. ) ;
#23213=ADVANCED_FACE ( 'NONE', ( #77254 ), #43155, .F. ) ;
#23214=PLANE ( 'NONE',  #28754 ) ;
#23215=VERTEX_POINT ( 'NONE', #35905 ) ;
#23217=EDGE_CURVE ( 'NONE', #63602, #5603, #62578, .T. ) ;
#23219=DIRECTION ( 'NONE',  ( 1.000000000000000000, 4.163336342344333240E-14, 0.000000000000000000 ) ) ;
#23221=CARTESIAN_POINT ( 'NONE',  ( 108.5410937779726623, -26.38672566707733225, 104.9641967044819779 ) ) ;
#23222=AXIS2_PLACEMENT_3D ( 'NONE', #26001, #18733, #80987 ) ;
#23224=DIRECTION ( 'NONE',  ( 1.000000000000000000, 0.000000000000000000, 0.000000000000000000 ) ) ;
#23227=CIRCLE ( 'NONE', #13019, 1.000000000000000888 ) ;
#23230=CARTESIAN_POINT ( 'NONE',  ( 142.0664832912740394, -45.72944715994099596, 14.67562527591100441 ) ) ;
#23232=DIRECTION ( 'NONE',  ( 0.000000000000000000, 0.000000000000000000, 1.000000000000000000 ) ) ;
#23233=CARTESIAN_POINT ( 'NONE',  ( 83.06670390244796920, -58.35344715994099829, 234.8338068554150198 ) ) ;
#23234=DIRECTION ( 'NONE',  ( 1.000000000000000078E-15, -1.000000000000000083E-30, -1.000000000000000000 ) ) ;
#23235=VECTOR ( 'NONE', #40081, 1000.000000000000114 ) ;
#23236=ADVANCED_FACE ( 'NONE', ( #58572 ), #22749, .F. ) ;
#23237=ORIENTED_EDGE ( 'NONE', *, *, #81628, .T. ) ;
#23239=CARTESIAN_POINT ( 'NONE',  ( 103.2204921605864314, -27.09891563476517717, 171.3908633711489813 ) ) ;
#23242=CIRCLE ( 'NONE', #56523, 2.749999999999974687 ) ;
#23243=CARTESIAN_POINT ( 'NONE',  ( 116.7468388360763925, -38.12735696270775065, 24.71276813305395237 ) ) ;
#23244=FACE_OUTER_BOUND ( 'NONE', #63403, .T. ) ;
#23245=DIRECTION ( 'NONE',  ( -0.7071067811865249242, 0.7071067811865702213, -7.071067811865256424E-16 ) ) ;
#23246=CARTESIAN_POINT ( 'NONE',  ( 115.7813681005709583, -41.80524612504061821, 13.40677487158930070 ) ) ;
#23247=VECTOR ( 'NONE', #30239, 1000.000000000000000 ) ;
#23248=LINE ( 'NONE', #84573, #12339 ) ;
#23249=CARTESIAN_POINT ( 'NONE',  ( 101.2091419812964830, -45.28691980162484754, 242.1108633711499465 ) ) ;
#23250=ORIENTED_EDGE ( 'NONE', *, *, #2758, .F. ) ;
#23252=CARTESIAN_POINT ( 'NONE',  ( 107.5663136956459738, -46.11170142552477813, 194.0625356868489462 ) ) ;
#23253=AXIS2_PLACEMENT_3D ( 'NONE', #9212, #8311, #2847 ) ;
#23254=DIRECTION ( 'NONE',  ( 4.299999999999999979E-14, -1.000000000000000000, 4.400000000000000367E-29 ) ) ;
#23255=CARTESIAN_POINT ( 'NONE',  ( 107.1760646772892756, -27.86850643495606406, 31.49872616304000417 ) ) ;
#23257=EDGE_CURVE ( 'NONE', #57874, #69697, #41281, .T. ) ;
#23258=EDGE_CURVE ( 'NONE', #52915, #83877, #1852, .T. ) ;
#23259=DIRECTION ( 'NONE',  ( 1.000000000000000000, -9.073094938289460781E-13, 0.000000000000000000 ) ) ;
#23260=AXIS2_PLACEMENT_3D ( 'NONE', #41440, #28264, #55959 ) ;
#23262=ORIENTED_EDGE ( 'NONE', *, *, #11256, .T. ) ;
#23263=FACE_OUTER_BOUND ( 'NONE', #9995, .T. ) ;
#23265=DIRECTION ( 'NONE',  ( -1.000000000000000000, -5.512527431108013646E-15, 0.000000000000000000 ) ) ;
#23267=CARTESIAN_POINT ( 'NONE',  ( 100.2615012876617726, -45.41023301258256595, 277.0594347997204636 ) ) ;
#23270=EDGE_LOOP ( 'NONE', ( #16680, #88831 ) ) ;
#23271=EDGE_CURVE ( 'NONE', #49742, #63793, #49978, .T. ) ;
#23272=CARTESIAN_POINT ( 'NONE',  ( 116.3212776292269268, -32.94146857470660450, 84.13562527591095375 ) ) ;
#23273=CARTESIAN_POINT ( 'NONE',  ( 41.56648329127399677, -18.82844715994099971, 321.0426252759119734 ) ) ;
#23274=VECTOR ( 'NONE', #54419, 1000.000000000000000 ) ;
#23276=DIRECTION ( 'NONE',  ( -0.7071067811865483499, -0.7071067811865466846, -7.071067811865491110E-16 ) ) ;
#23277=CARTESIAN_POINT ( 'NONE',  ( 101.7353989658871853, -28.52926574618699362, 21.53562527591096298 ) ) ;
#23281=CARTESIAN_POINT ( 'NONE',  ( 103.4621965996249600, -25.38836122657986394, 51.32133956162493149 ) ) ;
#23283=CARTESIAN_POINT ( 'NONE',  ( 96.97860658150185031, -39.36037357437717787, 276.5299109901967540 ) ) ;
#23284=ORIENTED_EDGE ( 'NONE', *, *, #80695, .F. ) ;
#23285=EDGE_CURVE ( 'NONE', #56395, #28751, #57245, .T. ) ;
#23286=LINE ( 'NONE', #78694, #81151 ) ;
#23287=CARTESIAN_POINT ( 'NONE',  ( 109.6439838910708318, -46.47984676037744833, 18.78209685499881587 ) ) ;
#23288=CARTESIAN_POINT ( 'NONE',  ( 46.03715912545348488, -48.62818131006090283, 129.9678068554150911 ) ) ;
#23289=CARTESIAN_POINT ( 'NONE',  ( 104.8330862573783122, -27.72345643971313578, 88.08809036959192440 ) ) ;
#23290=CARTESIAN_POINT ( 'NONE',  ( 104.4482647075962518, -26.61598136914473400, 196.2784824187679362 ) ) ;
#23292=VERTEX_POINT ( 'NONE', #39025 ) ;
#23294=VECTOR ( 'NONE', #59514, 1000.000000000000000 ) ;
#23297=FACE_BOUND ( 'NONE', #76435, .T. ) ;
#23298=VERTEX_POINT ( 'NONE', #18587 ) ;
#23299=VERTEX_POINT ( 'NONE', #17263 ) ;
#23300=LINE ( 'NONE', #50965, #62820 ) ;
#23301=CARTESIAN_POINT ( 'NONE',  ( 108.5087116869628545, -26.80026332916055765, 40.96182968949694470 ) ) ;
#23302=CARTESIAN_POINT ( 'NONE',  ( 112.8135049847298461, -43.08742197748514968, 132.5838483995059676 ) ) ;
#23303=CARTESIAN_POINT ( 'NONE',  ( 99.36516439250377175, -29.66998179773359823, 275.7356252759109907 ) ) ;
#23305=DIRECTION ( 'NONE',  ( 1.000000000000000078E-15, -1.000000000000000083E-30, -1.000000000000000000 ) ) ;
#23307=CARTESIAN_POINT ( 'NONE',  ( 103.2790308240917483, -27.47443741155154484, 136.3855809319543653 ) ) ;
#23309=LINE ( 'NONE', #78717, #24709 ) ;
#23310=CARTESIAN_POINT ( 'NONE',  ( 108.3323352706075582, -46.73498566967406731, 32.67742174073810446 ) ) ;
#23313=CIRCLE ( 'NONE', #59507, 2.117000000000007987 ) ;
#23315=ORIENTED_EDGE ( 'NONE', *, *, #85399, .T. ) ;
#23316=CARTESIAN_POINT ( 'NONE',  ( 99.33304576907053729, -28.83178728225833609, 270.7051490854348685 ) ) ;
#23317=CARTESIAN_POINT ( 'NONE',  ( 100.5706289694924607, -28.47478668554837000, 11.60705384733995515 ) ) ;
#23318=CARTESIAN_POINT ( 'NONE',  ( 99.04406185220089753, -42.84125763159654099, 117.8439586084165285 ) ) ;
#23319=B_SPLINE_CURVE_WITH_KNOTS ( 'NONE', 3,
 ( #27167, #5387, #69407, #33086, #7182, #67608, #20366, #74876, #6723, #89863, #55295, #60784, #88518, #806, #15789, #70752, #8526, #2607 ),
 .UNSPECIFIED., .F., .F.,
 ( 4, 2, 2, 2, 2, 2, 2, 2, 4 ),
 ( 0.000000000000000000, 0.06249843091306516579, 0.1249968618261303316, 0.1874952927391954904, 0.2499937236522606632, 0.3124921545653258081, 0.3749905854783909809, 0.4374890163914561536, 0.4999874473045213263 ),
 .UNSPECIFIED. ) ;
#23322=DIRECTION ( 'NONE',  ( 0.000000000000000000, 0.000000000000000000, -1.000000000000000000 ) ) ;
#23323=CARTESIAN_POINT ( 'NONE',  ( 107.0664832912739399, -36.72944715994095333, 293.1356252759106837 ) ) ;
#23324=DIRECTION ( 'NONE',  ( -6.524622321627019585E-16, -4.013151879589939944E-16, -1.000000000000000000 ) ) ;
#23328=CARTESIAN_POINT ( 'NONE',  ( 143.0664832912740110, -8.729447159940999512, 17.92562527591199739 ) ) ;
#23329=CARTESIAN_POINT ( 'NONE',  ( 136.8164806451553659, -36.72944715939129168, 6.749772901088312516 ) ) ;
#23330=CARTESIAN_POINT ( 'NONE',  ( 100.2327115992702176, -45.44695862323239055, 277.0594347997204068 ) ) ;
#23331=CARTESIAN_POINT ( 'NONE',  ( 116.7952044851831488, -40.57305441194377948, 189.5270538473389479 ) ) ;
#23332=CARTESIAN_POINT ( 'NONE',  ( 100.4515265478786574, -44.84261285976553779, 8.032768133053981074 ) ) ;
#23333=AXIS2_PLACEMENT_3D ( 'NONE', #34220, #4739, #20609 ) ;
#23334=LINE ( 'NONE', #51000, #43556 ) ;
#23335=CARTESIAN_POINT ( 'NONE',  ( 19.56670390244734747, -25.42844715994192129, 300.4678068554150059 ) ) ;
#23336=CARTESIAN_POINT ( 'NONE',  ( 80.94673009889058335, -34.12360705087682788, 1.744847597651331572 ) ) ;
#23337=EDGE_CURVE ( 'NONE', #85061, #31872, #44944, .T. ) ;
#23342=CARTESIAN_POINT ( 'NONE',  ( 97.35459460924926134, -38.14118110200429612, 62.44133956162495025 ) ) ;
#23346=CARTESIAN_POINT ( 'NONE',  ( 63.03715912545729338, -24.42818131006027826, 313.9678068554150059 ) ) ;
#23347=CARTESIAN_POINT ( 'NONE',  ( 107.6532706963292441, -47.74396045468172645, 193.6308633711489620 ) ) ;
#23348=LINE ( 'NONE', #29687, #20783 ) ;
#23349=CARTESIAN_POINT ( 'NONE',  ( 107.0664832912749915, -36.72944715993903486, 25.56312527591096995 ) ) ;
#23350=DIRECTION ( 'NONE',  ( -1.000000000000000078E-15, 0.000000000000000000, -1.000000000000000000 ) ) ;
#23351=DIRECTION ( 'NONE',  ( -1.000000000000000078E-15, 1.000000000000000083E-30, 1.000000000000000000 ) ) ;
#23352=PLANE ( 'NONE',  #60725 ) ;
#23353=CARTESIAN_POINT ( 'NONE',  ( 111.0847094670297110, -45.88713190444605772, 97.90550790398889092 ) ) ;
#23354=CARTESIAN_POINT ( 'NONE',  ( 98.98846131648976154, -42.30253745798197684, 126.8070538473399580 ) ) ;
#23355=ORIENTED_EDGE ( 'NONE', *, *, #77383, .F. ) ;
#23356=ORIENTED_EDGE ( 'NONE', *, *, #61112, .F. ) ;
#23357=CARTESIAN_POINT ( 'NONE',  ( 115.6007127221643032, -39.11591036577164004, 95.04158330589696391 ) ) ;
#23360=CARTESIAN_POINT ( 'NONE',  ( 97.71246005893831921, -41.20616857227587815, 212.6937205140059461 ) ) ;
#23363=CARTESIAN_POINT ( 'NONE',  ( 21.03715912545739641, -47.82818131006197149, 180.4678068554150911 ) ) ;
#23364=EDGE_CURVE ( 'NONE', #28401, #14757, #32529, .T. ) ;
#23365=DIRECTION ( 'NONE',  ( 0.000000000000000000, 0.000000000000000000, -1.000000000000000000 ) ) ;
#23367=EDGE_CURVE ( 'NONE', #12231, #12481, #12230, .T. ) ;
#23369=CARTESIAN_POINT ( 'NONE',  ( 114.1602155298370036, -45.17592836263241196, 148.1203871806719405 ) ) ;
#23370=EDGE_CURVE ( 'NONE', #23101, #45090, #87666, .T. ) ;
#23371=ORIENTED_EDGE ( 'NONE', *, *, #75361, .F. ) ;
#23373=VECTOR ( 'NONE', #31679, 1000.000000000000000 ) ;
#23374=ADVANCED_FACE ( 'NONE', ( #74003 ), #31316, .F. ) ;
#23375=CARTESIAN_POINT ( 'NONE',  ( 172.5664832912729878, -27.82844715994070484, 78.92562527591199739 ) ) ;
#23376=CARTESIAN_POINT ( 'NONE',  ( 77.44501272126919389, -17.89730640218066426, 2.921034946746040806 ) ) ;
#23378=DIRECTION ( 'NONE',  ( 0.7071067708032332533, 0.0001211784769705727632, 0.7071067811865479058 ) ) ;
#23379=CARTESIAN_POINT ( 'NONE',  ( 108.8441613132982155, -28.76266695291210951, 222.7195189410199703 ) ) ;
#23381=CARTESIAN_POINT ( 'NONE',  ( 142.0664832912739541, -9.729447159941033263, -4.970821333495754502 ) ) ;
#23382=CARTESIAN_POINT ( 'NONE',  ( 98.43480628652092435, -29.82486610537253569, 195.7775300378159784 ) ) ;
#23383=LINE ( 'NONE', #51051, #41684 ) ;
#23384=VERTEX_POINT ( 'NONE', #4067 ) ;
#23387=EDGE_CURVE ( 'NONE', #20562, #67881, #87639, .T. ) ;
#23388=AXIS2_PLACEMENT_3D ( 'NONE', #40687, #54288, #82052 ) ;
#23389=DIRECTION ( 'NONE',  ( -0.7071067811865753283, 0.7071067811865197061, -7.071067811865760309E-16 ) ) ;
#23390=ORIENTED_EDGE ( 'NONE', *, *, #45794, .F. ) ;
#23391=CARTESIAN_POINT ( 'NONE',  ( 97.81469011401388514, -40.51612824417846070, 136.6360017533206417 ) ) ;
#23392=CARTESIAN_POINT ( 'NONE',  ( 131.4524275574070771, -35.85322059724929034, 6.943211687812413935 ) ) ;
#23393=AXIS2_PLACEMENT_3D ( 'NONE', #57572, #78498, #16258 ) ;
#23394=CARTESIAN_POINT ( 'NONE',  ( 111.0382984267975246, -28.80776997321336097, 276.1387261630399621 ) ) ;
#23396=EDGE_LOOP ( 'NONE', ( #80519, #77804, #83632, #89183 ) ) ;
#23397=CARTESIAN_POINT ( 'NONE',  ( 115.0808484473774485, -41.07790926377064267, 9.635625275910941312 ) ) ;
#23398=FACE_OUTER_BOUND ( 'NONE', #24932, .T. ) ;
#23400=ORIENTED_EDGE ( 'NONE', *, *, #89800, .F. ) ;
#23404=CARTESIAN_POINT ( 'NONE',  ( 111.2703484347609333, -28.70728902343469002, 14.10289601855296837 ) ) ;
#23405=CARTESIAN_POINT ( 'NONE',  ( 114.9818473740405835, -29.91084206771912690, 184.3927681330539770 ) ) ;
#23407=CARTESIAN_POINT ( 'NONE',  ( 114.4965984691701664, -29.44205611023136626, 149.4441967044819819 ) ) ;
#23408=CARTESIAN_POINT ( 'NONE',  ( 64.67079002020508938, -0.9301828534102468682, 394.9756252759101471 ) ) ;
#23409=CARTESIAN_POINT ( 'NONE',  ( 104.8412801004068058, -26.50840007386317509, 256.2470538473397141 ) ) ;
#23410=CARTESIAN_POINT ( 'NONE',  ( 117.0718565137653968, -35.46215913205921311, 99.92773310503083906 ) ) ;
#23413=VERTEX_POINT ( 'NONE', #39479 ) ;
#23414=ORIENTED_EDGE ( 'NONE', *, *, #51318, .T. ) ;
#23415=AXIS2_PLACEMENT_3D ( 'NONE', #61881, #42768, #55949 ) ;
#23417=AXIS2_PLACEMENT_3D ( 'NONE', #45354, #17675, #73074 ) ;
#23418=CARTESIAN_POINT ( 'NONE',  ( 107.5678864575881590, -47.81824684668375625, 192.6003871806729535 ) ) ;
#23419=ORIENTED_EDGE ( 'NONE', *, *, #36368, .T. ) ;
#23420=CARTESIAN_POINT ( 'NONE',  ( 114.2535261088984981, -44.28147934099003180, 158.1813395616249807 ) ) ;
#23421=DIRECTION ( 'NONE',  ( 0.02150753337723812844, 0.0009076677972192511400, 0.9997682742251809973 ) ) ;
#23422=EDGE_CURVE ( 'NONE', #12231, #2137, #86751, .T. ) ;
#23423=CARTESIAN_POINT ( 'NONE',  ( 136.4578062354202359, -35.36823420008745700, 7.200493380652632780 ) ) ;
#23424=CARTESIAN_POINT ( 'NONE',  ( 48.45959712128975383, -28.98061976758959801, 117.4678068554150485 ) ) ;
#23426=CARTESIAN_POINT ( 'NONE',  ( 80.06648329127399677, 0.2215528400590013880, 308.6356252759119911 ) ) ;
#23427=CARTESIAN_POINT ( 'NONE',  ( 97.63514171170974976, -41.12017164899855715, 252.6727681330536655 ) ) ;
#23428=PLANE ( 'NONE',  #55297 ) ;
#23429=CARTESIAN_POINT ( 'NONE',  ( 144.4532657278588204, -72.54451140298851897, 540.9756252759101471 ) ) ;
#23431=DIRECTION ( 'NONE',  ( -1.000000000000000000, -4.299999999999999979E-14, -1.000000000000000078E-15 ) ) ;
#23432=CARTESIAN_POINT ( 'NONE',  ( 108.3334481168079435, -46.73485935100409705, 258.6772919443159253 ) ) ;
#23433=CARTESIAN_POINT ( 'NONE',  ( 172.5664832912740110, -32.07844715994070839, 78.92562527591199739 ) ) ;
#23434=AXIS2_PLACEMENT_3D ( 'NONE', #27907, #55137, #14749 ) ;
#23435=CARTESIAN_POINT ( 'NONE',  ( 112.8728595368667698, -42.45837713832621318, 195.5838068554166966 ) ) ;
#23436=VERTEX_POINT ( 'NONE', #60355 ) ;
#23437=DIRECTION ( 'NONE',  ( 0.000000000000000000, 1.000000000000000000, 0.000000000000000000 ) ) ;
#23438=CARTESIAN_POINT ( 'NONE',  ( 106.4823715260129688, -24.86804634255730662, 195.1156252759109861 ) ) ;
#23439=CARTESIAN_POINT ( 'NONE',  ( 101.0662023700742935, -27.44663458233410935, 66.54514908543495721 ) ) ;
#23440=CARTESIAN_POINT ( 'NONE',  ( 116.8358708857152095, -40.58912082693117185, 189.5270538473389479 ) ) ;
#23443=CARTESIAN_POINT ( 'NONE',  ( 116.3212776292296127, -32.94146857471318413, 287.6356252759109680 ) ) ;
#23445=CARTESIAN_POINT ( 'NONE',  ( 164.7830935719630361, -29.99615139349950965, -5.074374724088000832 ) ) ;
#23446=DIRECTION ( 'NONE',  ( 0.000000000000000000, 0.000000000000000000, -1.000000000000000000 ) ) ;
#23447=VERTEX_POINT ( 'NONE', #80838 ) ;
#23448=AXIS2_PLACEMENT_3D ( 'NONE', #53311, #46953, #39702 ) ;
#23450=EDGE_CURVE ( 'NONE', #67268, #25932, #55954, .T. ) ;
#23452=ORIENTED_EDGE ( 'NONE', *, *, #53586, .T. ) ;
#23453=CARTESIAN_POINT ( 'NONE',  ( 103.9030524752275397, -44.69467205304180624, 116.6981341137909567 ) ) ;
#23455=ORIENTED_EDGE ( 'NONE', *, *, #29044, .T. ) ;
#23456=CARTESIAN_POINT ( 'NONE',  ( 115.1498815335950638, -43.27828968249928465, 84.28419670448195689 ) ) ;
#23460=DIRECTION ( 'NONE',  ( 1.000000000000000078E-15, 1.000000000000000083E-30, -1.000000000000000000 ) ) ;
#23461=CARTESIAN_POINT ( 'NONE',  ( 110.8778723976570433, -46.37372517399798255, 22.88800622829195675 ) ) ;
#23463=ORIENTED_EDGE ( 'NONE', *, *, #4713, .F. ) ;
#23466=CARTESIAN_POINT ( 'NONE',  ( 193.0371591254583734, -47.82818131005421947, 313.9678068554149490 ) ) ;
#23467=CARTESIAN_POINT ( 'NONE',  ( 109.7248659245813656, -27.00080518071327162, 115.8647919423142696 ) ) ;
#23468=CARTESIAN_POINT ( 'NONE',  ( 71.25416588882602298, -72.55705569728901594, 540.9756252759101471 ) ) ;
#23470=CARTESIAN_POINT ( 'NONE',  ( 97.07208927141411436, -35.37826970552124095, 52.21955069277615991 ) ) ;
#23472=CIRCLE ( 'NONE', #19087, 11.45913725231036118 ) ;
#23474=CARTESIAN_POINT ( 'NONE',  ( 112.9508454419806043, -28.15023113465287352, 44.59848241876795782 ) ) ;
#23478=B_SPLINE_CURVE_WITH_KNOTS ( 'NONE', 3,
 ( #45018, #65481, #10077, #79128, #1924, #37782, #8747, #10515, #31393, #23287, #44121, #3267, #70975, #30958, #72746, #43685, #9624, #65036, #64592, #38220, #3700, #59090, #78695, #58645, #2819, #2374, #24594 ),
 .UNSPECIFIED., .F., .F.,
 ( 4, 2, 2, 2, 2, 2, 2, 2, 2, 2, 1, 1, 1, 2, 4 ),
 ( 0.000000000000000000, 0.06250761762232094620, 0.1250152352446418924, 0.1875228528669628247, 0.2500304704892837848, 0.3125380881116047727, 0.3750457057339256495, 0.4375533233562466373, 0.4688071321674068814, 0.4844340365729870035, 0.4922474887757767870, 0.4961542148771715399, 0.4981075779278690274, 0.4990842594532179377, 0.5000609409785667925 ),
 .UNSPECIFIED. ) ;
#23481=CARTESIAN_POINT ( 'NONE',  ( 103.6457284375485131, -44.67924975648479347, 135.0833284648299752 ) ) ;
#23482=B_SPLINE_CURVE_WITH_KNOTS ( 'NONE', 3,
 ( #19370, #74779, #34329, #39789, #40245, #33439, #61143, #54299, #82066, #62929, #36594, #16149, #69762, #63846, #35676, #70206, #42923, #1629 ),
 .UNSPECIFIED., .F., .F.,
 ( 4, 2, 2, 2, 2, 2, 2, 2, 4 ),
 ( 0.000000000000000000, 0.06249998643239338542, 0.1249999728647867708, 0.1874999592971801632, 0.2499999457295735417, 0.3124999321619669201, 0.3749999185943603264, 0.4374999050267536771, 0.4999998914591470833 ),
 .UNSPECIFIED. ) ;
#23483=VECTOR ( 'NONE', #7071, 1000.000000000000000 ) ;
#23484=CARTESIAN_POINT ( 'NONE',  ( 102.0647649218796289, -27.97183332977936132, 95.49000569952723083 ) ) ;
#23485=DIRECTION ( 'NONE',  ( -3.999999999999999995E-14, 1.000000000000000000, -4.100000000000000342E-29 ) ) ;
#23487=ORIENTED_EDGE ( 'NONE', *, *, #77936, .F. ) ;
#23488=ADVANCED_FACE ( 'NONE', ( #48065 ), #51394, .T. ) ;
#23489=CARTESIAN_POINT ( 'NONE',  ( 98.54782867203449825, -41.97726770183525957, 136.7656906696263093 ) ) ;
#23490=ORIENTED_EDGE ( 'NONE', *, *, #33998, .F. ) ;
#23491=ORIENTED_EDGE ( 'NONE', *, *, #25292, .T. ) ;
#23494=CARTESIAN_POINT ( 'NONE',  ( 98.87114546532168902, -41.32433164768560374, 178.1768214011349585 ) ) ;
#23496=CARTESIAN_POINT ( 'NONE',  ( 102.2923668651898339, -27.39740514546159389, 116.4527681330539650 ) ) ;
#23497=CARTESIAN_POINT ( 'NONE',  ( 48.16670390244496502, -26.71338133339251542, 342.9256252759109884 ) ) ;
#23498=AXIS2_PLACEMENT_3D ( 'NONE', #22421, #41933, #29232 ) ;
#23499=CARTESIAN_POINT ( 'NONE',  ( 116.5679076829705707, -33.54432202151119924, 19.08379224916496497 ) ) ;
#23500=ORIENTED_EDGE ( 'NONE', *, *, #8384, .T. ) ;
#23502=ORIENTED_EDGE ( 'NONE', *, *, #49056, .T. ) ;
#23504=CIRCLE ( 'NONE', #48095, 3.300000000000000711 ) ;
#23505=CARTESIAN_POINT ( 'NONE',  ( 99.90434330870786539, -40.64524553156628173, 219.5423760838769738 ) ) ;
#23506=CARTESIAN_POINT ( 'NONE',  ( 113.5198117145332475, -28.51355303769357619, 79.54705384733995288 ) ) ;
#23507=ORIENTED_EDGE ( 'NONE', *, *, #57918, .T. ) ;
#23508=CARTESIAN_POINT ( 'NONE',  ( 118.0600790064084293, -37.62648441163795354, 38.77372051400595865 ) ) ;
#23509=CARTESIAN_POINT ( 'NONE',  ( 112.4324277152178837, -28.68226574489724001, 249.5838068554168956 ) ) ;
#23510=CARTESIAN_POINT ( 'NONE',  ( 130.0664832912740110, -18.72922654876706972, 284.9256252759119548 ) ) ;
#23512=CARTESIAN_POINT ( 'NONE',  ( 97.98655846647217516, -41.85169789442448263, 132.7356252759109623 ) ) ;
#23513=CIRCLE ( 'NONE', #36607, 27.99999999999999645 ) ;
#23514=CARTESIAN_POINT ( 'NONE',  ( 123.0079629938350223, -38.09664315643626509, 302.4856252759109907 ) ) ;
#23515=ORIENTED_EDGE ( 'NONE', *, *, #1668, .T. ) ;
#23519=CARTESIAN_POINT ( 'NONE',  ( 193.0371591254583450, -47.82818131005411999, 249.9678068554149775 ) ) ;
#23522=FACE_OUTER_BOUND ( 'NONE', #6594, .T. ) ;
#23523=CARTESIAN_POINT ( 'NONE',  ( 103.1466689443337117, -27.50432134387084560, 131.3959253572286627 ) ) ;
#23524=CARTESIAN_POINT ( 'NONE',  ( 96.92094985624760284, -32.34227964863599425, 61.01372051400599616 ) ) ;
#23526=EDGE_CURVE ( 'NONE', #65464, #83730, #55761, .T. ) ;
#23527=DIRECTION ( 'NONE',  ( 0.000000000000000000, -1.000000000000000000, 0.000000000000000000 ) ) ;
#23529=CARTESIAN_POINT ( 'NONE',  ( 116.1466984671188385, -33.09446055034462120, 54.12991099019798469 ) ) ;
#23530=CARTESIAN_POINT ( 'NONE',  ( 72.31648329127402519, -45.62589376934781882, -5.074374724089063982 ) ) ;
#23531=CARTESIAN_POINT ( 'NONE',  ( 108.5866130067098254, -47.05677245125736619, 138.6927681330539883 ) ) ;
#23532=DIRECTION ( 'NONE',  ( 1.000000000000000000, 4.163336342344333240E-14, 0.000000000000000000 ) ) ;
#23533=CARTESIAN_POINT ( 'NONE',  ( 165.9667039024473922, -26.71338133338714016, 313.9678068554149490 ) ) ;
#23539=CARTESIAN_POINT ( 'NONE',  ( 115.4232488078209258, -30.42301107085752321, 219.3413395616249773 ) ) ;
#23541=CARTESIAN_POINT ( 'NONE',  ( 98.34968923854172829, -31.65687136160358506, 145.9064846611762505 ) ) ;
#23542=CARTESIAN_POINT ( 'NONE',  ( 116.9053397700284478, -41.81689336946376301, 239.4346728949589647 ) ) ;
#23543=CARTESIAN_POINT ( 'NONE',  ( 109.6947933286257353, -47.51320739032397000, 83.75467289495897205 ) ) ;
#23546=CARTESIAN_POINT ( 'NONE',  ( 104.4076956878168261, -46.45797032905074531, 263.3648843889448585 ) ) ;
#23548=ADVANCED_FACE ( 'NONE', ( #14012 ), #83077, .T. ) ;
#23549=ORIENTED_EDGE ( 'NONE', *, *, #35839, .T. ) ;
#23550=VERTEX_POINT ( 'NONE', #21277 ) ;
#23552=VERTEX_POINT ( 'NONE', #81736 ) ;
#23554=CARTESIAN_POINT ( 'NONE',  ( 118.1029919389229406, -36.12161712796727642, 269.8822919425776945 ) ) ;
#23555=DIRECTION ( 'NONE',  ( 0.9963424814100678706, -0.08544974978095865037, 0.000000000000000000 ) ) ;
#23556=CARTESIAN_POINT ( 'NONE',  ( 132.8830524875708363, -34.24700279812689274, 1.845048209623704416 ) ) ;
#23557=ADVANCED_FACE ( 'NONE', ( #35338 ), #89432, .T. ) ;
#23563=CARTESIAN_POINT ( 'NONE',  ( 114.6950545185401609, -40.57145610743049247, 202.8781341137909635 ) ) ;
#23566=ORIENTED_EDGE ( 'NONE', *, *, #64796, .F. ) ;
#23569=DIRECTION ( 'NONE',  ( 0.000000000000000000, 0.000000000000000000, 1.000000000000000000 ) ) ;
#23570=CARTESIAN_POINT ( 'NONE',  ( 110.8541901428846899, -45.98435271355759824, 182.8856010440399018 ) ) ;
#23572=CARTESIAN_POINT ( 'NONE',  ( 99.81116105471878086, -29.32005551970522461, 266.7051490854344706 ) ) ;
#23573=CIRCLE ( 'NONE', #74318, 2.500000000000002220 ) ;
#23576=EDGE_CURVE ( 'NONE', #80585, #89702, #15184, .T. ) ;
#23578=EDGE_LOOP ( 'NONE', ( #2379, #12616, #49463, #41291, #4782 ) ) ;
#23579=FACE_OUTER_BOUND ( 'NONE', #81614, .T. ) ;
#23582=CARTESIAN_POINT ( 'NONE',  ( 110.3993955946342993, -29.27817736879564237, 22.55951894101998434 ) ) ;
#23583=CARTESIAN_POINT ( 'NONE',  ( 136.7978637535031226, -18.40984252624964412, 6.777538624682987844 ) ) ;
#23586=EDGE_LOOP ( 'NONE', ( #19447, #62535, #13875, #83312 ) ) ;
#23589=CARTESIAN_POINT ( 'NONE',  ( 107.0664832912739968, -36.72944715994100306, -2.364374724089013391 ) ) ;
#23590=VECTOR ( 'NONE', #34017, 1000.000000000000000 ) ;
#23591=EDGE_LOOP ( 'NONE', ( #6103, #67600, #48759, #9391 ) ) ;
#23592=CARTESIAN_POINT ( 'NONE',  ( 113.3425240358415778, -27.63052414531908596, 89.60800622829195561 ) ) ;
#23595=CARTESIAN_POINT ( 'NONE',  ( 99.48186602960301173, -30.66774701162068695, 45.21241982807700310 ) ) ;
#23596=EDGE_CURVE ( 'NONE', #40553, #58657, #28994, .T. ) ;
#23598=CARTESIAN_POINT ( 'NONE',  ( 98.75489364002905290, -33.65605228111792968, 62.47586902018298360 ) ) ;
#23599=CARTESIAN_POINT ( 'NONE',  ( 90.44969454456408187, -50.04645651782490745, 239.5838068554174356 ) ) ;
#23600=DIRECTION ( 'NONE',  ( 1.000000000000000000, 8.163404592831600092E-16, 1.020425574103949962E-15 ) ) ;
#23603=CARTESIAN_POINT ( 'NONE',  ( 118.7569292017688696, -34.64240976163905827, 44.96705384733895272 ) ) ;
#23607=CARTESIAN_POINT ( 'NONE',  ( 128.0667039024480118, -50.82844715994100682, 250.9178068554150514 ) ) ;
#23609=CARTESIAN_POINT ( 'NONE',  ( 113.8717716195138792, -28.72781827743602889, 135.5156252759109634 ) ) ;
#23613=B_SPLINE_CURVE_WITH_KNOTS ( 'NONE', 3,
 ( #46163, #73895, #11679, #39372, #60248, #65728, #10333, #87980, #67520, #25740, #58905, #53416, #81183, #18932, #74348, #12118, #39801, #5309, #32999, #81633, #3510, #44838, #31208, #86642, #52080, #24415, #79840, #17597 ),
 .UNSPECIFIED., .F., .F.,
 ( 4, 2, 2, 2, 2, 2, 2, 2, 2, 2, 1, 1, 1, 1, 2, 4 ),
 ( 0.000000000000000000, 0.06251128867752057949, 0.1250225773550411590, 0.1875338660325617246, 0.2500451547100823180, 0.3125564433876029113, 0.3750677320651234492, 0.4375790207426440426, 0.4688346650814042005, 0.4844624872507840574, 0.4922763983354739303, 0.4961833538778187003, 0.4981368316489910852, 0.4991135705345771667, 0.4996019399773705127, 0.5000903094201638588 ),
 .UNSPECIFIED. ) ;
#23614=FACE_OUTER_BOUND ( 'NONE', #63731, .T. ) ;
#23615=DIRECTION ( 'NONE',  ( 1.000000000000000000, 6.493183223601999383E-14, -1.022247060195607093E-42 ) ) ;
#23616=CARTESIAN_POINT ( 'NONE',  ( 107.2322476904469966, -46.54200526979099095, 212.5899109901969837 ) ) ;
#23619=DIRECTION ( 'NONE',  ( 0.000000000000000000, 0.000000000000000000, -1.000000000000000000 ) ) ;
#23620=CARTESIAN_POINT ( 'NONE',  ( 110.2841144599940577, -46.64559811412390644, 8.827053847339950465 ) ) ;
#23621=AXIS2_PLACEMENT_3D ( 'NONE', #80117, #53699, #5595 ) ;
#23622=CARTESIAN_POINT ( 'NONE',  ( 33.91903122894598965, -35.91149509761181235, -5.074374724088000832 ) ) ;
#23623=ORIENTED_EDGE ( 'NONE', *, *, #16357, .F. ) ;
#23625=DIRECTION ( 'NONE',  ( -1.000000000000000078E-15, 1.000000000000000083E-30, 1.000000000000000000 ) ) ;
#23626=ORIENTED_EDGE ( 'NONE', *, *, #39219, .F. ) ;
#23628=CARTESIAN_POINT ( 'NONE',  ( 97.80791547859365664, -40.51903635482080546, 112.6360621818907077 ) ) ;
#23629=CARTESIAN_POINT ( 'NONE',  ( 118.6297112294784029, -39.20734283244436114, 258.6584824187679033 ) ) ;
#23630=CARTESIAN_POINT ( 'NONE',  ( 72.25757238336808541, -1.944390235229867425, 361.9756252759101471 ) ) ;
#23631=DIRECTION ( 'NONE',  ( 1.000000000000000000, 4.237773401492740281E-14, 0.000000000000000000 ) ) ;
#23633=CARTESIAN_POINT ( 'NONE',  ( 98.11275290507195734, -35.37173493080541675, 220.6171817328389864 ) ) ;
#23634=CYLINDRICAL_SURFACE ( 'NONE', #89645, 12.99999999999999822 ) ;
#23635=CARTESIAN_POINT ( 'NONE',  ( 106.6078071710152244, -25.70885557892973949, 36.09753003781596448 ) ) ;
#23637=CARTESIAN_POINT ( 'NONE',  ( 117.7486274683349308, -39.74683136594191524, 143.6194347997209775 ) ) ;
#23638=VERTEX_POINT ( 'NONE', #43938 ) ;
#23639=DIRECTION ( 'NONE',  ( 1.054009200593500181E-15, 1.000000000000000000, 0.000000000000000000 ) ) ;
#23640=EDGE_LOOP ( 'NONE', ( #25966, #72582, #26147, #988 ) ) ;
#23642=CARTESIAN_POINT ( 'NONE',  ( 97.81281252356875200, -40.52015776331121089, 277.6356251289804504 ) ) ;
#23644=DIRECTION ( 'NONE',  ( 0.000000000000000000, 1.000000000000000000, 0.000000000000000000 ) ) ;
#23646=CARTESIAN_POINT ( 'NONE',  ( 251.6756888531239156, -13.32818131005263140, 117.4678068554150627 ) ) ;
#23647=CARTESIAN_POINT ( 'NONE',  ( 107.0664832912739541, -36.72944715994095333, 309.2406250056037038 ) ) ;
#23648=DIRECTION ( 'NONE',  ( 0.000000000000000000, 0.000000000000000000, 1.000000000000000000 ) ) ;
#23650=CARTESIAN_POINT ( 'NONE',  ( 106.6594718829666704, -26.29006472227095870, 85.10705384733896040 ) ) ;
#23654=PLANE ( 'NONE',  #58258 ) ;
#23657=EDGE_LOOP ( 'NONE', ( #43430, #88808, #27637, #24276 ) ) ;
#23660=VECTOR ( 'NONE', #39286, 1000.000000000000000 ) ;
#23661=CARTESIAN_POINT ( 'NONE',  ( 172.5664832912729878, -27.57844715994070484, 18.92562527591200094 ) ) ;
#23668=CARTESIAN_POINT ( 'NONE',  ( 88.17226027475707895, -14.72944715994102616, 249.5838068554175777 ) ) ;
#23670=VECTOR ( 'NONE', #14994, 1000.000000000000000 ) ;
#23671=ORIENTED_EDGE ( 'NONE', *, *, #22798, .F. ) ;
#23672=CARTESIAN_POINT ( 'NONE',  ( 182.0667039024480118, -32.29483332968430886, -5.074374724088000832 ) ) ;
#23674=CARTESIAN_POINT ( 'NONE',  ( 102.3610132369663432, -45.97051510703448685, 168.2137205140059564 ) ) ;
#23676=EDGE_LOOP ( 'NONE', ( #14838, #1695, #59674, #50258 ) ) ;
#23677=CARTESIAN_POINT ( 'NONE',  ( 106.3024736416176950, -26.94527301088420046, 21.13848241876792144 ) ) ;
#23678=DIRECTION ( 'NONE',  ( 2.900000000000000265E-14, -2.000000000000000155E-15, 1.000000000000000000 ) ) ;
#23680=DIRECTION ( 'NONE',  ( 0.000000000000000000, 1.000000000000000000, 0.000000000000000000 ) ) ;
#23681=EDGE_CURVE ( 'NONE', #10148, #52594, #1288, .T. ) ;
#23682=ORIENTED_EDGE ( 'NONE', *, *, #260, .F. ) ;
#23683=CARTESIAN_POINT ( 'NONE',  ( 99.09606710607866376, -30.54995432804265576, 30.80247099595620952 ) ) ;
#23684=CARTESIAN_POINT ( 'NONE',  ( 98.48461633480658861, -41.42146110206444121, 221.7241967044829494 ) ) ;
#23687=CARTESIAN_POINT ( 'NONE',  ( 107.4908894006829172, -46.11541567637532069, 189.0320594963729661 ) ) ;
#23688=AXIS2_PLACEMENT_3D ( 'NONE', #74000, #59904, #25399 ) ;
#23689=DIRECTION ( 'NONE',  ( 0.000000000000000000, 0.000000000000000000, 1.000000000000000000 ) ) ;
#23690=CARTESIAN_POINT ( 'NONE',  ( 106.1501016865858844, -27.91533782510476058, 46.59015473446797984 ) ) ;
#23693=VECTOR ( 'NONE', #25813, 1000.000000000000114 ) ;
#23695=DIRECTION ( 'NONE',  ( 0.000000000000000000, 0.000000000000000000, 1.000000000000000000 ) ) ;
#23697=PLANE ( 'NONE',  #87070 ) ;
#23698=DIRECTION ( 'NONE',  ( 2.999999999999999839E-15, -1.000000000000000000, 2.999999999999999900E-30 ) ) ;
#23700=CARTESIAN_POINT ( 'NONE',  ( 118.0844448206164827, -36.21142561920247971, 268.8518157521015723 ) ) ;
#23702=ORIENTED_EDGE ( 'NONE', *, *, #76061, .F. ) ;
#23705=CARTESIAN_POINT ( 'NONE',  ( 80.06648329127399677, 0.2215528400590013880, 311.1531252759119752 ) ) ;
#23707=CARTESIAN_POINT ( 'NONE',  ( 172.5664832912740110, 0.2215528400590013880, 18.92562527591200094 ) ) ;
#23709=CARTESIAN_POINT ( 'NONE',  ( 96.85055626654755656, -38.51091292166574220, 42.45181575209999636 ) ) ;
#23711=ORIENTED_EDGE ( 'NONE', *, *, #88059, .T. ) ;
#23712=CARTESIAN_POINT ( 'NONE',  ( 95.20983985305964836, -35.71400682071400468, 32.25848241876794020 ) ) ;
#23713=DIRECTION ( 'NONE',  ( 1.000000000000000000, 0.000000000000000000, 1.261617073437676668E-15 ) ) ;
#23714=AXIS2_PLACEMENT_3D ( 'NONE', #40392, #54439, #5440 ) ;
#23715=CARTESIAN_POINT ( 'NONE',  ( 104.5881283732255156, -26.60288457357396652, 285.2670538473396391 ) ) ;
#23716=VERTEX_POINT ( 'NONE', #71235 ) ;
#23718=CARTESIAN_POINT ( 'NONE',  ( 82.81644824798257787, -18.55833207211307112, 3.101428811465905877 ) ) ;
#23719=DIRECTION ( 'NONE',  ( -0.0001713722455994998422, 0.9999999853157766072, 0.000000000000000000 ) ) ;
#23721=CARTESIAN_POINT ( 'NONE',  ( 113.0492235774716363, -42.98306560958572931, 110.9899951314959594 ) ) ;
#23722=CARTESIAN_POINT ( 'NONE',  ( 115.0562973506820157, -29.05819712879207017, 185.4232443235299570 ) ) ;
#23724=DIRECTION ( 'NONE',  ( 0.7071067811571474238, 0.7071067812159476107, 0.000000000000000000 ) ) ;
#23725=ORIENTED_EDGE ( 'NONE', *, *, #32024, .F. ) ;
#23729=AXIS2_PLACEMENT_3D ( 'NONE', #27010, #27449, #82889 ) ;
#23730=CYLINDRICAL_SURFACE ( 'NONE', #56030, 2.030000000001872529 ) ;
#23731=ORIENTED_EDGE ( 'NONE', *, *, #75735, .T. ) ;
#23732=VERTEX_POINT ( 'NONE', #23095 ) ;
#23734=CARTESIAN_POINT ( 'NONE',  ( 115.8238408366701009, -31.72726729926949574, 24.24004256710726679 ) ) ;
#23735=CARTESIAN_POINT ( 'NONE',  ( 112.1993679394656453, -43.55657132036190404, 142.5124198280769576 ) ) ;
#23736=CARTESIAN_POINT ( 'NONE',  ( 116.6022279875747216, -42.36549642380604297, 283.4137205140060018 ) ) ;
#23739=CARTESIAN_POINT ( 'NONE',  ( 108.5522760911612465, -26.80684647353728778, 135.9583350980946364 ) ) ;
#23741=LINE ( 'NONE', #36010, #34826 ) ;
#23747=EDGE_LOOP ( 'NONE', ( #17654, #7284, #7816, #42509 ) ) ;
#23748=CARTESIAN_POINT ( 'NONE',  ( 106.1383370350330324, -47.74387551462719159, 262.4975300378158636 ) ) ;
#23749=CARTESIAN_POINT ( 'NONE',  ( 115.4796304032075653, -43.01888039838633659, 24.31562527591096767 ) ) ;
#23750=AXIS2_PLACEMENT_3D ( 'NONE', #72656, #66260, #79034 ) ;
#23751=DIRECTION ( 'NONE',  ( 0.000000000000000000, 0.000000000000000000, -1.000000000000000000 ) ) ;
#23752=EDGE_CURVE ( 'NONE', #52709, #76080, #73893, .T. ) ;
#23755=CARTESIAN_POINT ( 'NONE',  ( 51.06670390244899238, -32.29483332968430886, -5.074374724088000832 ) ) ;
#23757=CARTESIAN_POINT ( 'NONE',  ( 37.36643805256657913, -48.62818131006090994, 249.9678068554150343 ) ) ;
#23758=CARTESIAN_POINT ( 'NONE',  ( 131.7293641403265099, -38.17925173418004192, 7.255518600575052268 ) ) ;
#23759=EDGE_CURVE ( 'NONE', #72082, #10437, #44837, .T. ) ;
#23760=CARTESIAN_POINT ( 'NONE',  ( 162.8913605087219878, -31.76306994223740432, -5.074374724088000832 ) ) ;
#23762=DIRECTION ( 'NONE',  ( 0.000000000000000000, 0.000000000000000000, 1.000000000000000000 ) ) ;
#23763=ADVANCED_FACE ( 'NONE', ( #65298 ), #23971, .T. ) ;
#23764=LINE ( 'NONE', #51432, #84452 ) ;
#23765=CARTESIAN_POINT ( 'NONE',  ( 118.6196304926710212, -33.88663714441439367, 14.01848241876796308 ) ) ;
#23766=CARTESIAN_POINT ( 'NONE',  ( 98.09065366798802188, -42.10120877535955231, 157.7556252759109725 ) ) ;
#23767=CARTESIAN_POINT ( 'NONE',  ( 110.3609615670502535, -25.32029891922833897, 60.85276813305395649 ) ) ;
#23768=DIRECTION ( 'NONE',  ( 0.000000000000000000, 0.000000000000000000, 1.000000000000000000 ) ) ;
#23769=DIRECTION ( 'NONE',  ( 0.000000000000000000, 0.000000000000000000, -1.000000000000000000 ) ) ;
#23770=CARTESIAN_POINT ( 'NONE',  ( 82.58883806303516906, -35.63381004753058789, 2.797770231023114729 ) ) ;
#23772=AXIS2_PLACEMENT_3D ( 'NONE', #63110, #82686, #7264 ) ;
#23773=CIRCLE ( 'NONE', #17908, 0.4999999999999994449 ) ;
#23775=CARTESIAN_POINT ( 'NONE',  ( 100.9546728744814601, -28.70702568005829391, 186.5939586030299608 ) ) ;
#23776=ORIENTED_EDGE ( 'NONE', *, *, #73173, .F. ) ;
#23777=EDGE_CURVE ( 'NONE', #76504, #14135, #10816, .T. ) ;
#23778=CARTESIAN_POINT ( 'NONE',  ( 98.84777479348176144, -29.24180311599948467, 76.73848241876795839 ) ) ;
#23779=PLANE ( 'NONE',  #80578 ) ;
#23780=ORIENTED_EDGE ( 'NONE', *, *, #4141, .T. ) ;
#23782=CARTESIAN_POINT ( 'NONE',  ( 112.0653985349986357, -45.48868239570060723, 48.98974552996795495 ) ) ;
#23783=CARTESIAN_POINT ( 'NONE',  ( 117.7539631054256972, -31.66723592997637482, 210.1784824187679703 ) ) ;
#23784=LINE ( 'NONE', #51448, #77390 ) ;
#23785=DIRECTION ( 'NONE',  ( 0.9068632946707805287, -0.4214249218767882610, 1.035655806553318316E-15 ) ) ;
#23787=DIRECTION ( 'NONE',  ( 1.000000000000000078E-15, 1.000000000000000083E-30, -1.000000000000000000 ) ) ;
#23790=CARTESIAN_POINT ( 'NONE',  ( 110.8719906046491559, -45.97705236736918977, 97.88713169491219901 ) ) ;
#23791=CARTESIAN_POINT ( 'NONE',  ( 102.9676436823273917, -46.25511244710201453, 137.2651490854349561 ) ) ;
#23792=ORIENTED_EDGE ( 'NONE', *, *, #13347, .F. ) ;
#23793=ORIENTED_EDGE ( 'NONE', *, *, #25207, .F. ) ;
#23794=CARTESIAN_POINT ( 'NONE',  ( 116.2382276885637538, -38.76798346032508391, 100.0720594963729866 ) ) ;
#23795=CARTESIAN_POINT ( 'NONE',  ( 128.0667039024481539, -16.72944715994115583, 239.5838068554164408 ) ) ;
#23796=CARTESIAN_POINT ( 'NONE',  ( 107.2379402074490855, -25.61267671046461558, 226.0641967044819580 ) ) ;
#23797=CARTESIAN_POINT ( 'NONE',  ( 41.56670390244777735, -36.32844715994104234, 300.4678068554150059 ) ) ;
#23798=CARTESIAN_POINT ( 'NONE',  ( 113.8679580013058654, -39.89013407401493794, 9.125625275910969947 ) ) ;
#23802=DIRECTION ( 'NONE',  ( -1.000000000000000000, 0.000000000000000000, 8.252657816380299978E-16 ) ) ;
#23804=CARTESIAN_POINT ( 'NONE',  ( 97.69433714244404143, -41.24514667321086847, 171.6841967044819626 ) ) ;
#23807=CARTESIAN_POINT ( 'NONE',  ( 72.06648329127403940, -56.72944715994105991, -4.824374724089063982 ) ) ;
#23809=CARTESIAN_POINT ( 'NONE',  ( 97.81169182074827972, -40.51741433969252881, 77.63574375254798099 ) ) ;
#23810=CARTESIAN_POINT ( 'NONE',  ( 98.54748562642340914, -41.97671081279658978, 102.7657787019688271 ) ) ;
#23812=AXIS2_PLACEMENT_3D ( 'NONE', #60475, #32324, #88221 ) ;
#23813=DIRECTION ( 'NONE',  ( -1.000000000000000078E-15, 1.000000000000000083E-30, 1.000000000000000000 ) ) ;
#23815=CARTESIAN_POINT ( 'NONE',  ( 97.76227787611212250, -41.51041654567812600, 196.7041967044819728 ) ) ;
#23816=LINE ( 'NONE', #49705, #9751 ) ;
#23817=ORIENTED_EDGE ( 'NONE', *, *, #32138, .T. ) ;
#23819=VERTEX_POINT ( 'NONE', #32542 ) ;
#23821=DIRECTION ( 'NONE',  ( 1.000000000000000000, 0.000000000000000000, 0.000000000000000000 ) ) ;
#23822=DIRECTION ( 'NONE',  ( -1.000000000000000078E-15, 1.000000000000000083E-30, 1.000000000000000000 ) ) ;
#23823=CARTESIAN_POINT ( 'NONE',  ( 113.8567361903355675, -31.03552547285496388, 265.8130118773257777 ) ) ;
#23824=CARTESIAN_POINT ( 'NONE',  ( 45.77381068356938698, -48.62134037881676818, 249.9678068554150343 ) ) ;
#23826=EDGE_CURVE ( 'NONE', #39335, #56383, #11678, .T. ) ;
#23827=CARTESIAN_POINT ( 'NONE',  ( 115.8395158816858981, -40.05665934170760067, 9.635625275910941312 ) ) ;
#23829=ORIENTED_EDGE ( 'NONE', *, *, #2529, .F. ) ;
#23830=ORIENTED_EDGE ( 'NONE', *, *, #49672, .T. ) ;
#23831=EDGE_CURVE ( 'NONE', #47474, #9456, #25290, .T. ) ;
#23832=AXIS2_PLACEMENT_3D ( 'NONE', #55045, #54147, #48685 ) ;
#23833=DIRECTION ( 'NONE',  ( 4.194175870806139918E-14, -1.000000000000000000, 0.000000000000000000 ) ) ;
#23834=CIRCLE ( 'NONE', #60036, 1.000000000000000888 ) ;
#23836=ORIENTED_EDGE ( 'NONE', *, *, #19913, .F. ) ;
#23837=VECTOR ( 'NONE', #37141, 1000.000000000000000 ) ;
#23838=CARTESIAN_POINT ( 'NONE',  ( 98.68252487213293023, -38.50746385042646125, 30.91527697093399141 ) ) ;
#23839=CIRCLE ( 'NONE', #25240, 2.517500000000005844 ) ;
#23840=CARTESIAN_POINT ( 'NONE',  ( 95.88624405714097065, -32.72491640434669335, 176.0527681330539735 ) ) ;
#23841=CARTESIAN_POINT ( 'NONE',  ( 111.7842945758856672, -25.88553347519904335, 134.7499109901969518 ) ) ;
#23843=CARTESIAN_POINT ( 'NONE',  ( 162.5667039024460223, -22.48495420874110806, -5.074374724088000832 ) ) ;
#23844=CARTESIAN_POINT ( 'NONE',  ( 118.0816017896457453, -32.35888884030432422, 245.1270538473389706 ) ) ;
#23845=DIRECTION ( 'NONE',  ( 1.639958061481212836E-42, -4.100000000000000342E-29, -1.000000000000000000 ) ) ;
#23848=ORIENTED_EDGE ( 'NONE', *, *, #77057, .F. ) ;
#23850=CARTESIAN_POINT ( 'NONE',  ( 109.3681991936945508, -25.87058038976459429, 184.9222919425779708 ) ) ;
#23851=VERTEX_POINT ( 'NONE', #3958 ) ;
#23852=CARTESIAN_POINT ( 'NONE',  ( 104.5625478726873894, -48.31265885861421339, 182.4070538473399665 ) ) ;
#23853=CARTESIAN_POINT ( 'NONE',  ( 41.56648329127381203, -27.82844715994070484, 321.9256252759120116 ) ) ;
#23854=LINE ( 'NONE', #25623, #17417 ) ;
#23858=CARTESIAN_POINT ( 'NONE',  ( 98.36549455146196408, -40.29075363668730603, 7.635625275910939536 ) ) ;
#23859=CYLINDRICAL_SURFACE ( 'NONE', #22025, 0.4999999999999989453 ) ;
#23861=DIRECTION ( 'NONE',  ( 0.9242245927363031965, 0.3818493186865917766, 0.000000000000000000 ) ) ;
#23862=FACE_OUTER_BOUND ( 'NONE', #41345, .T. ) ;
#23866=CARTESIAN_POINT ( 'NONE',  ( 107.0664832912739968, 0.2215528400590083269, 336.6506252759110112 ) ) ;
#23867=CARTESIAN_POINT ( 'NONE',  ( 100.8056940436082698, -41.93424458468394533, 195.5838068554169809 ) ) ;
#23869=EDGE_CURVE ( 'NONE', #13668, #78028, #55790, .T. ) ;
#23870=CARTESIAN_POINT ( 'NONE',  ( 135.7779513194053891, -20.88977919477191492, 7.751962620090911749 ) ) ;
#23871=CARTESIAN_POINT ( 'NONE',  ( 108.6784406349466110, -26.40724015326817664, 189.9527681330539792 ) ) ;
#23872=CARTESIAN_POINT ( 'NONE',  ( 115.2072660578295284, -44.20618685261739245, 74.22324432352993995 ) ) ;
#23873=CARTESIAN_POINT ( 'NONE',  ( 106.5652502036378593, -47.22167190867460818, 243.5384824187679556 ) ) ;
#23874=CARTESIAN_POINT ( 'NONE',  ( 188.5667039024479834, -62.87844715994099687, 175.9678068554150059 ) ) ;
#23875=LINE ( 'NONE', #51545, #47493 ) ;
#23876=DIRECTION ( 'NONE',  ( 1.000000000000000078E-15, -1.000000000000000000, 0.000000000000000000 ) ) ;
#23877=CARTESIAN_POINT ( 'NONE',  ( 164.9190312289453004, -35.91149509760637670, 313.9678068554149490 ) ) ;
#23880=ORIENTED_EDGE ( 'NONE', *, *, #89740, .T. ) ;
#23881=VECTOR ( 'NONE', #27313, 1000.000000000000000 ) ;
#23882=DIRECTION ( 'NONE',  ( -4.237773401492740281E-14, 1.000000000000000000, 0.000000000000000000 ) ) ;
#23884=ORIENTED_EDGE ( 'NONE', *, *, #14229, .F. ) ;
#23886=EDGE_CURVE ( 'NONE', #49295, #85439, #58903, .T. ) ;
#23887=CARTESIAN_POINT ( 'NONE',  ( 107.2856214976012552, -28.19082255356615008, 119.4781341137909578 ) ) ;
#23889=ORIENTED_EDGE ( 'NONE', *, *, #14489, .T. ) ;
#23890=CARTESIAN_POINT ( 'NONE',  ( 96.05879824974444148, -41.05137697672054742, 92.62419670448296927 ) ) ;
#23893=DIRECTION ( 'NONE',  ( 0.000000000000000000, 1.000000000000000000, 1.914177628664063178E-15 ) ) ;
#23894=CARTESIAN_POINT ( 'NONE',  ( 117.5198883494731632, -40.51604253578042858, 23.54991099019792955 ) ) ;
#23895=VERTEX_POINT ( 'NONE', #17596 ) ;
#23896=ORIENTED_EDGE ( 'NONE', *, *, #47538, .T. ) ;
#23897=ORIENTED_EDGE ( 'NONE', *, *, #59388, .F. ) ;
#23898=VECTOR ( 'NONE', #40731, 1000.000000000000000 ) ;
#23899=AXIS2_PLACEMENT_3D ( 'NONE', #65088, #85997, #23769 ) ;
#23900=DIRECTION ( 'NONE',  ( 1.000000000000000000, 4.299999999999999979E-14, 1.000000000000000078E-15 ) ) ;
#23902=DIRECTION ( 'NONE',  ( 0.000000000000000000, 0.000000000000000000, 1.000000000000000000 ) ) ;
#23905=DIRECTION ( 'NONE',  ( -0.7071067811864671926, -0.7071067811866279529, -7.071067811864664779E-16 ) ) ;
#23906=CARTESIAN_POINT ( 'NONE',  ( 194.0371591254573502, -24.89890238294407965, 249.9678068554149775 ) ) ;
#23912=CARTESIAN_POINT ( 'NONE',  ( 115.0059970501927182, -43.50650750775904640, 63.26419670448196797 ) ) ;
#23916=CARTESIAN_POINT ( 'NONE',  ( 163.5667039024460223, -18.82844715994111340, 330.9333219726761399 ) ) ;
#23917=CARTESIAN_POINT ( 'NONE',  ( 108.2186271136511095, -28.64846388872622285, 102.7823760838769687 ) ) ;
#23918=EDGE_CURVE ( 'NONE', #45771, #31400, #31170, .T. ) ;
#23919=VECTOR ( 'NONE', #53296, 1000.000000000000000 ) ;
#23920=CARTESIAN_POINT ( 'NONE',  ( 97.80514285669603680, -40.50139878960715834, 96.63424722611091511 ) ) ;
#23923=VERTEX_POINT ( 'NONE', #38467 ) ;
#23924=CARTESIAN_POINT ( 'NONE',  ( 172.5667039024478413, -36.32844715993500273, 249.9678068554149775 ) ) ;
#23925=ORIENTED_EDGE ( 'NONE', *, *, #36298, .T. ) ;
#23927=CARTESIAN_POINT ( 'NONE',  ( 113.7913652599847438, -30.16800768036728542, 190.8853928297069444 ) ) ;
#23929=CARTESIAN_POINT ( 'NONE',  ( 104.9584626277977577, -25.04276672576827778, 121.2184824187679766 ) ) ;
#23930=CARTESIAN_POINT ( 'NONE',  ( 20.03715912545745326, -46.82818131006192175, 180.4678068554150911 ) ) ;
#23931=CARTESIAN_POINT ( 'NONE',  ( 99.08976676173786302, -42.79577391424577115, 16.84398999344881176 ) ) ;
#23932=ORIENTED_EDGE ( 'NONE', *, *, #34011, .T. ) ;
#23933=EDGE_CURVE ( 'NONE', #77606, #63506, #59358, .T. ) ;
#23935=ORIENTED_EDGE ( 'NONE', *, *, #78216, .T. ) ;
#23936=ORIENTED_EDGE ( 'NONE', *, *, #44010, .T. ) ;
#23937=CARTESIAN_POINT ( 'NONE',  ( 113.3093514795881589, -30.73549005055465955, 187.2414237029249477 ) ) ;
#23938=CARTESIAN_POINT ( 'NONE',  ( 97.26762016986505444, -33.10609988230974920, 66.04419670448297097 ) ) ;
#23940=CARTESIAN_POINT ( 'NONE',  ( 116.7068942081672276, -31.36975501082240569, 29.24229194257799236 ) ) ;
#23942=LINE ( 'NONE', #25259, #16211 ) ;
#23943=CARTESIAN_POINT ( 'NONE',  ( 107.0079280548302592, -25.26905977990648466, 323.4874463521242092 ) ) ;
#23944=CARTESIAN_POINT ( 'NONE',  ( 108.0069324954157537, -26.34569400419502827, 151.0041967044829505 ) ) ;
#23947=CARTESIAN_POINT ( 'NONE',  ( 134.0664832912740110, -41.22944715994101017, 4.925625275910997303 ) ) ;
#23948=ORIENTED_CLOSED_SHELL ( 'NONE', *, #35820, .F. );
#23954=DIRECTION ( 'NONE',  ( 0.9068632946707805287, -0.4214249218767880389, 9.068632946707802473E-16 ) ) ;
#23956=CARTESIAN_POINT ( 'NONE',  ( 51.23005224011598102, -33.89581943344511217, -5.074374724088000832 ) ) ;
#23957=CARTESIAN_POINT ( 'NONE',  ( 107.8683683300076837, -26.33502505738635691, 70.01562527591099183 ) ) ;
#23958=DIRECTION ( 'NONE',  ( -1.000000000000000000, -4.163336342344275811E-14, 0.000000000000000000 ) ) ;
#23959=AXIS2_PLACEMENT_3D ( 'NONE', #76879, #62784, #6484 ) ;
#23960=DIRECTION ( 'NONE',  ( -1.000000000000000078E-15, -9.367723249499513438E-31, 1.000000000000000000 ) ) ;
#23961=DIRECTION ( 'NONE',  ( 0.000000000000000000, 1.000000000000000000, 0.000000000000000000 ) ) ;
#23962=CARTESIAN_POINT ( 'NONE',  ( 104.2296407737279509, -46.70397019442136610, 67.36800622829292706 ) ) ;
#23963=DIRECTION ( 'NONE',  ( 1.000000000000000000, 0.000000000000000000, -0.000000000000000000 ) ) ;
#23964=CARTESIAN_POINT ( 'NONE',  ( 117.4654710391979222, -40.40706546494229201, 174.5680062282919778 ) ) ;
#23967=DIRECTION ( 'NONE',  ( 3.999999999999999995E-14, -1.000000000000000000, 4.100000000000000342E-29 ) ) ;
#23968=ORIENTED_EDGE ( 'NONE', *, *, #37643, .F. ) ;
#23969=DIRECTION ( 'NONE',  ( 1.000000000000000000, 0.000000000000000000, 1.261617073437676668E-15 ) ) ;
#23970=VECTOR ( 'NONE', #52090, 1000.000000000000000 ) ;
#23971=PLANE ( 'NONE',  #89160 ) ;
#23972=EDGE_CURVE ( 'NONE', #59961, #67197, #26635, .T. ) ;
#23974=DIRECTION ( 'NONE',  ( 3.999999999999999995E-14, -1.000000000000000000, 4.100000000000000342E-29 ) ) ;
#23975=CARTESIAN_POINT ( 'NONE',  ( 97.01576029581003979, -41.44069443601846814, 211.6632443235299945 ) ) ;
#23976=ORIENTED_EDGE ( 'NONE', *, *, #3959, .F. ) ;
#23977=EDGE_CURVE ( 'NONE', #49045, #83730, #53864, .T. ) ;
#23978=DIRECTION ( 'NONE',  ( 0.000000000000000000, 0.000000000000000000, 1.000000000000000000 ) ) ;
#23979=CARTESIAN_POINT ( 'NONE',  ( 103.0821958934680111, -47.91639064866039632, 248.3041967044829619 ) ) ;
#23980=CARTESIAN_POINT ( 'NONE',  ( 107.2328990581281687, -25.63125793145087172, 76.07657765686298035 ) ) ;
#23981=DIRECTION ( 'NONE',  ( -2.999999999999999839E-15, 1.000000000000000000, -2.999999999999999900E-30 ) ) ;
#23982=CARTESIAN_POINT ( 'NONE',  ( 97.81021718220807770, -40.51802218317752846, 192.6354414398782353 ) ) ;
#23983=CIRCLE ( 'NONE', #19616, 10.04999999999999361 ) ;
#23993=CARTESIAN_POINT ( 'NONE',  ( 95.23138046818854718, -37.33356364299761054, 267.3670538473395482 ) ) ;
#23995=ADVANCED_FACE ( 'NONE', ( #27090 ), #20724, .T. ) ;
#23996=CARTESIAN_POINT ( 'NONE',  ( 131.4596324495014130, -35.85248396559212125, 2.902015641457837969 ) ) ;
#24000=CARTESIAN_POINT ( 'NONE',  ( 109.5125757112413822, -28.00996883845181173, 219.2933722090289734 ) ) ;
#24001=ORIENTED_EDGE ( 'NONE', *, *, #2414, .F. ) ;
#24002=VERTEX_POINT ( 'NONE', #40257 ) ;
#24003=AXIS2_PLACEMENT_3D ( 'NONE', #6398, #75454, #33660 ) ;
#24005=PLANE ( 'NONE',  #60100 ) ;
#24006=AXIS2_PLACEMENT_3D ( 'NONE', #86765, #39931, #5434 ) ;
#24007=CARTESIAN_POINT ( 'NONE',  ( 97.81221995309677197, -40.51872308918434840, 181.6357364503598433 ) ) ;
#24008=CARTESIAN_POINT ( 'NONE',  ( 97.40014589274353796, -35.23768424668793386, 262.2041967044816602 ) ) ;
#24009=DIRECTION ( 'NONE',  ( -0.9068632946707805287, 0.4214249218767882610, -9.068632946707800501E-16 ) ) ;
#24010=CARTESIAN_POINT ( 'NONE',  ( 115.8238554372424289, -31.72729253430197360, 174.2400402683865650 ) ) ;
#24012=ORIENTED_EDGE ( 'NONE', *, *, #24168, .F. ) ;
#24013=CARTESIAN_POINT ( 'NONE',  ( 107.9683749031584341, -26.74872499883632315, 56.00468566283465321 ) ) ;
#24016=CARTESIAN_POINT ( 'NONE',  ( 113.6264423535256043, -41.63348889605062908, 26.13380465530496011 ) ) ;
#24019=AXIS2_PLACEMENT_3D ( 'NONE', #89254, #67899, #55133 ) ;
#24021=AXIS2_PLACEMENT_3D ( 'NONE', #3159, #72199, #9084 ) ;
#24023=CARTESIAN_POINT ( 'NONE',  ( 72.06648329127401098, -45.72944715994106701, 14.92562527591093691 ) ) ;
#24024=CYLINDRICAL_SURFACE ( 'NONE', #35804, 7.499999999999996447 ) ;
#24025=AXIS2_PLACEMENT_3D ( 'NONE', #6545, #34242, #19288 ) ;
#24030=CARTESIAN_POINT ( 'NONE',  ( 96.71459513300293054, -38.23421233548538112, 66.44133956162495735 ) ) ;
#24031=ORIENTED_EDGE ( 'NONE', *, *, #45758, .F. ) ;
#24032=CARTESIAN_POINT ( 'NONE',  ( 114.0365971503568119, -41.66641429710976752, 52.75813411379098739 ) ) ;
#24034=CARTESIAN_POINT ( 'NONE',  ( 117.0564912681829952, -35.80799090043529276, 89.89887535740403735 ) ) ;
#24035=CARTESIAN_POINT ( 'NONE',  ( 114.0372341014417543, -43.02906291645705039, 79.68539282970694160 ) ) ;
#24036=DIRECTION ( 'NONE',  ( -2.981567257902526681E-15, 0.8571673007021100021, 0.5150380749100580413 ) ) ;
#24040=CARTESIAN_POINT ( 'NONE',  ( 116.7472758669860013, -31.34730438484761805, 25.24229194257798881 ) ) ;
#24041=DIRECTION ( 'NONE',  ( 0.9999999853157766072, 0.0001713722456143214551, 0.000000000000000000 ) ) ;
#24042=ORIENTED_EDGE ( 'NONE', *, *, #51117, .T. ) ;
#24044=EDGE_LOOP ( 'NONE', ( #83251, #50689, #70231, #65490 ) ) ;
#24045=CARTESIAN_POINT ( 'NONE',  ( 97.96923373944615321, -30.37039525599472256, 156.8289586092439549 ) ) ;
#24047=CARTESIAN_POINT ( 'NONE',  ( 78.80082187617171030, -21.17731672736319126, 1.873071027758830054 ) ) ;
#24048=ORIENTED_EDGE ( 'NONE', *, *, #79771, .F. ) ;
#24049=AXIS2_PLACEMENT_3D ( 'NONE', #5441, #87217, #39050 ) ;
#24050=ORIENTED_EDGE ( 'NONE', *, *, #7042, .T. ) ;
#24052=CARTESIAN_POINT ( 'NONE',  ( 63.03715912545826683, -46.82818131006018092, 237.4678068554150059 ) ) ;
#24053=CARTESIAN_POINT ( 'NONE',  ( 107.2379402074490429, -25.61267671046441308, 230.0641967044829812 ) ) ;
#24054=CARTESIAN_POINT ( 'NONE',  ( 97.77504362009293004, -40.42681596862870208, 126.6273886944452016 ) ) ;
#24055=CARTESIAN_POINT ( 'NONE',  ( 99.04406178308130393, -42.84125754196290359, 187.8439585994789809 ) ) ;
#24056=CARTESIAN_POINT ( 'NONE',  ( 96.17756896972203151, -38.62826926382330583, 42.45181575210199298 ) ) ;
#24057=CARTESIAN_POINT ( 'NONE',  ( 99.50455959988217103, -43.30559304351280048, 42.89599952138878081 ) ) ;
#24058=ORIENTED_EDGE ( 'NONE', *, *, #52546, .T. ) ;
#24059=CARTESIAN_POINT ( 'NONE',  ( 97.70650162570946407, -40.25115913408279766, 172.6128377269262728 ) ) ;
#24060=EDGE_CURVE ( 'NONE', #33552, #46749, #55651, .T. ) ;
#24063=CIRCLE ( 'NONE', #74825, 1.000000000000000888 ) ;
#24065=CARTESIAN_POINT ( 'NONE',  ( 117.0724333545735902, -35.46694875580925554, 114.9279293202101968 ) ) ;
#24066=CARTESIAN_POINT ( 'NONE',  ( 98.95962429139160577, -30.20966935044058488, 240.7870538473399620 ) ) ;
#24069=DIRECTION ( 'NONE',  ( 1.000000000000000000, 0.000000000000000000, 0.000000000000000000 ) ) ;
#24070=DIRECTION ( 'NONE',  ( -0.9254794337955620787, -0.3787978585227822492, 0.000000000000000000 ) ) ;
#24071=CARTESIAN_POINT ( 'NONE',  ( 102.6292086192877946, -44.02785282196147421, 246.5638483995049626 ) ) ;
#24073=CARTESIAN_POINT ( 'NONE',  ( 117.2454586689011364, -38.87819698039182015, 59.66133956162595098 ) ) ;
#24075=CARTESIAN_POINT ( 'NONE',  ( 118.9539009387050186, -36.16544432761327954, 118.8641967044819836 ) ) ;
#24076=ORIENTED_EDGE ( 'NONE', *, *, #3231, .F. ) ;
#24077=CARTESIAN_POINT ( 'NONE',  ( 181.8764988495248929, -33.54226604284360036, 193.9678068554150059 ) ) ;
#24081=CARTESIAN_POINT ( 'NONE',  ( 103.4822561620420487, -27.39340619187812820, 276.3681719739503819 ) ) ;
#24083=ORIENTED_EDGE ( 'NONE', *, *, #73804, .F. ) ;
#24084=CARTESIAN_POINT ( 'NONE',  ( 97.33774635339761971, -34.07140301938782301, 51.11481945842477614 ) ) ;
#24087=CARTESIAN_POINT ( 'NONE',  ( 116.3212776292295842, -32.94146857471309886, 45.13562527591097506 ) ) ;
#24089=VECTOR ( 'NONE', #64677, 1000.000000000000000 ) ;
#24090=VERTEX_POINT ( 'NONE', #88433 ) ;
#24091=CARTESIAN_POINT ( 'NONE',  ( 116.5534958752826213, -32.35418074550542400, 104.1699109901969535 ) ) ;
#24094=AXIS2_PLACEMENT_3D ( 'NONE', #75516, #32823, #68698 ) ;
#24095=DIRECTION ( 'NONE',  ( 1.000000000000000078E-15, -1.000000000000000000, 0.000000000000000000 ) ) ;
#24096=DIRECTION ( 'NONE',  ( 0.000000000000000000, 0.000000000000000000, 1.000000000000000000 ) ) ;
#24099=EDGE_CURVE ( 'NONE', #51053, #9116, #75246, .T. ) ;
#24102=FACE_OUTER_BOUND ( 'NONE', #38317, .T. ) ;
#24103=EDGE_CURVE ( 'NONE', #72149, #51651, #19380, .T. ) ;
#24107=CARTESIAN_POINT ( 'NONE',  ( 182.4202572930400095, -33.70561438051981185, 117.4678068554150627 ) ) ;
#24111=CARTESIAN_POINT ( 'NONE',  ( 101.9936211249197555, -45.44607164413606171, 33.15645862599451021 ) ) ;
#24112=CARTESIAN_POINT ( 'NONE',  ( 116.4077482568849007, -39.73851878533132975, 154.5784824187679476 ) ) ;
#24115=CARTESIAN_POINT ( 'NONE',  ( 116.1702204287673794, -31.76348745224625958, 20.21181575210096071 ) ) ;
#24116=DIRECTION ( 'NONE',  ( 1.000000000000000000, 6.145690160522439356E-16, 0.000000000000000000 ) ) ;
#24118=CARTESIAN_POINT ( 'NONE',  ( 172.5664832912729878, -18.82844715994071194, 318.9256252759120116 ) ) ;
#24119=VERTEX_POINT ( 'NONE', #5308 ) ;
#24121=ORIENTED_EDGE ( 'NONE', *, *, #51904, .F. ) ;
#24123=CARTESIAN_POINT ( 'NONE',  ( 104.1527054293246550, -27.79712248444839773, 206.7711071154209606 ) ) ;
#24124=CARTESIAN_POINT ( 'NONE',  ( 194.5667039024479834, -40.82844715993405771, 300.4678068554149490 ) ) ;
#24125=CARTESIAN_POINT ( 'NONE',  ( 115.2933828064165311, -33.43605939358163681, 50.56158330589693861 ) ) ;
#24129=FACE_OUTER_BOUND ( 'NONE', #19696, .T. ) ;
#24132=CARTESIAN_POINT ( 'NONE',  ( 33.96670390244699433, -28.27351298637401200, -5.074374724088000832 ) ) ;
#24134=CARTESIAN_POINT ( 'NONE',  ( 115.3062145713272599, -45.21207857638187022, 268.1899109901965517 ) ) ;
#24135=CARTESIAN_POINT ( 'NONE',  ( 79.06648329127300201, -36.72944715994189835, 361.9756252759079871 ) ) ;
#24136=ORIENTED_EDGE ( 'NONE', *, *, #64977, .F. ) ;
#24137=PLANE ( 'NONE',  #88011 ) ;
#24138=LINE ( 'NONE', #86812, #4101 ) ;
#24140=DIRECTION ( 'NONE',  ( 1.000000000000000078E-15, -1.000000000000000000, 0.000000000000000000 ) ) ;
#24141=AXIS2_PLACEMENT_3D ( 'NONE', #36550, #77429, #64252 ) ;
#24142=CARTESIAN_POINT ( 'NONE',  ( 106.8507155540331013, -47.82678659975260160, 223.5489586092439538 ) ) ;
#24143=AXIS2_PLACEMENT_3D ( 'NONE', #72725, #79107, #43211 ) ;
#24146=VECTOR ( 'NONE', #59121, 1000.000000000000000 ) ;
#24147=CARTESIAN_POINT ( 'NONE',  ( 110.3857440325295443, -47.32095349711466525, 48.80610146638797175 ) ) ;
#24149=LINE ( 'NONE', #51375, #30846 ) ;
#24150=AXIS2_PLACEMENT_3D ( 'NONE', #10490, #23695, #10929 ) ;
#24151=CARTESIAN_POINT ( 'NONE',  ( 111.4804840314119758, -26.59568808167472653, 284.7375300378156453 ) ) ;
#24153=EDGE_LOOP ( 'NONE', ( #43871, #58380, #9682, #27263 ) ) ;
#24154=EDGE_CURVE ( 'NONE', #38408, #16560, #63083, .T. ) ;
#24155=CARTESIAN_POINT ( 'NONE',  ( 107.0664832912739968, 25.62155284005901379, 339.0006252759110339 ) ) ;
#24158=CARTESIAN_POINT ( 'NONE',  ( 100.1260263088618103, -41.89964850235647020, 109.6661856076859607 ) ) ;
#24159=CARTESIAN_POINT ( 'NONE',  ( 112.4656099449901916, -45.71435824391657832, 234.0070538473389377 ) ) ;
#24161=LINE ( 'NONE', #51384, #69658 ) ;
#24162=ORIENTED_EDGE ( 'NONE', *, *, #46876, .F. ) ;
#24163=EDGE_CURVE ( 'NONE', #61077, #88430, #74695, .T. ) ;
#24164=VECTOR ( 'NONE', #83709, 999.9999999999998863 ) ;
#24165=CARTESIAN_POINT ( 'NONE',  ( 188.5667039024479834, -58.35344715994099829, 295.9678068554150059 ) ) ;
#24167=ORIENTED_EDGE ( 'NONE', *, *, #21802, .T. ) ;
#24168=EDGE_CURVE ( 'NONE', #58062, #7066, #80540, .T. ) ;
#24169=DIRECTION ( 'NONE',  ( 0.7071067811865101582, 0.7071067811865849873, 0.000000000000000000 ) ) ;
#24171=ORIENTED_EDGE ( 'NONE', *, *, #515, .F. ) ;
#24172=CARTESIAN_POINT ( 'NONE',  ( 100.8880764000450370, -44.70071190640118886, 168.0529670008384926 ) ) ;
#24173=ADVANCED_FACE ( 'NONE', ( #77039 ), #70670, .F. ) ;
#24174=CARTESIAN_POINT ( 'NONE',  ( 103.2796802074614817, -27.47417168924152620, 41.38552508622479564 ) ) ;
#24175=CARTESIAN_POINT ( 'NONE',  ( 106.2553484193443865, -46.40481216151710697, 111.9324198280769735 ) ) ;
#24176=CARTESIAN_POINT ( 'NONE',  ( 115.9827728363227664, -42.21636132903250171, 18.38705384733896153 ) ) ;
#24178=DIRECTION ( 'NONE',  ( 4.554376769437570034E-14, -1.000000000000000000, 0.000000000000000000 ) ) ;
#24179=ADVANCED_FACE ( 'NONE', ( #36605 ), #49754, .F. ) ;
#24181=CYLINDRICAL_SURFACE ( 'NONE', #18565, 3.250000000000002665 ) ;
#24182=VERTEX_POINT ( 'NONE', #35233 ) ;
#24184=DIRECTION ( 'NONE',  ( 0.000000000000000000, 0.000000000000000000, -1.000000000000000000 ) ) ;
#24185=CARTESIAN_POINT ( 'NONE',  ( 51.56670390244799762, -33.35206098992650681, -5.074374724088000832 ) ) ;
#24186=CARTESIAN_POINT ( 'NONE',  ( 63.03715912545640521, -24.89890238295017255, 180.4678068554151196 ) ) ;
#24187=ORIENTED_EDGE ( 'NONE', *, *, #49991, .F. ) ;
#24188=CARTESIAN_POINT ( 'NONE',  ( 116.5821416419259435, -42.35362450032752690, 283.4137205140060587 ) ) ;
#24189=CARTESIAN_POINT ( 'NONE',  ( 116.8105015878075079, -31.41422314659176607, 20.21181575210195902 ) ) ;
#24192=DIRECTION ( 'NONE',  ( 0.000000000000000000, 0.000000000000000000, -1.000000000000000000 ) ) ;
#24193=DIRECTION ( 'NONE',  ( 1.000000000000000078E-15, -1.000000000000000083E-30, -1.000000000000000000 ) ) ;
#24195=EDGE_CURVE ( 'NONE', #69092, #64904, #3632, .T. ) ;
#24197=ADVANCED_FACE ( 'NONE', ( #7987 ), #70216, .T. ) ;
#24198=CARTESIAN_POINT ( 'NONE',  ( 112.0663155181265580, -45.48817100771776722, 162.9896579463498369 ) ) ;
#24199=EDGE_CURVE ( 'NONE', #29616, #45, #43836, .T. ) ;
#24200=PLANE ( 'NONE',  #5165 ) ;
#24201=CARTESIAN_POINT ( 'NONE',  ( 118.2557925370599179, -40.78261322564650015, 23.54991099019593292 ) ) ;
#24202=CARTESIAN_POINT ( 'NONE',  ( 113.5650955083461326, -44.92635950737134465, 164.1099109901969655 ) ) ;
#24203=CARTESIAN_POINT ( 'NONE',  ( 117.2880962612577349, -38.88719764259226253, 59.66133956162595098 ) ) ;
#24204=EDGE_CURVE ( 'NONE', #32492, #60843, #50655, .T. ) ;
#24205=CIRCLE ( 'NONE', #11083, 3.299999999999997158 ) ;
#24206=FACE_OUTER_BOUND ( 'NONE', #74682, .T. ) ;
#24207=CARTESIAN_POINT ( 'NONE',  ( 105.7154773334175815, -46.72385839260719109, 47.46895860948406920 ) ) ;
#24208=CARTESIAN_POINT ( 'NONE',  ( 81.12494507884905204, -34.19118199975294203, 1.799893109327175500 ) ) ;
#24209=AXIS2_PLACEMENT_3D ( 'NONE', #86480, #58311, #51474 ) ;
#24212=FACE_OUTER_BOUND ( 'NONE', #67695, .T. ) ;
#24214=CARTESIAN_POINT ( 'NONE',  ( 97.54819157151555942, -32.61351373332772852, 57.01372051400599616 ) ) ;
#24215=CARTESIAN_POINT ( 'NONE',  ( 194.0371591254573218, -24.42818131005407878, 249.9678068554149775 ) ) ;
#24218=CARTESIAN_POINT ( 'NONE',  ( 103.6457867198658391, -26.24313906103854066, 206.3394347997209763 ) ) ;
#24219=DIRECTION ( 'NONE',  ( 0.000000000000000000, 1.000000000000000000, 0.000000000000000000 ) ) ;
#24221=FACE_BOUND ( 'NONE', #19902, .T. ) ;
#24223=DIRECTION ( 'NONE',  ( -4.237773401492740281E-14, 1.000000000000000000, 0.000000000000000000 ) ) ;
#24224=CYLINDRICAL_SURFACE ( 'NONE', #81995, 9.999999999999998224 ) ;
#24226=CARTESIAN_POINT ( 'NONE',  ( 109.3575602964533431, -46.23809593081423941, 132.7641967044829698 ) ) ;
#24227=ORIENTED_EDGE ( 'NONE', *, *, #53761, .F. ) ;
#24228=EDGE_LOOP ( 'NONE', ( #66641, #40463, #74879, #25918 ) ) ;
#24229=CARTESIAN_POINT ( 'NONE',  ( 97.72568451978753501, -37.74236564027221874, 77.83205949637394383 ) ) ;
#24231=CYLINDRICAL_SURFACE ( 'NONE', #70450, 2.749999999999974687 ) ;
#24232=CARTESIAN_POINT ( 'NONE',  ( 100.2051353121705546, -29.75912871662447756, 221.6956252759109702 ) ) ;
#24235=PLANE ( 'NONE',  #77169 ) ;
#24238=CARTESIAN_POINT ( 'NONE',  ( 184.5664832912740110, 25.62155284005901379, 323.8756252759109202 ) ) ;
#24240=CARTESIAN_POINT ( 'NONE',  ( 113.3182355088851381, -45.04474967211709924, 143.0899109901969553 ) ) ;
#24241=ORIENTED_EDGE ( 'NONE', *, *, #41359, .F. ) ;
#24245=CARTESIAN_POINT ( 'NONE',  ( 104.4081006469831578, -46.45808913634610349, 78.36479194142131632 ) ) ;
#24246=CARTESIAN_POINT ( 'NONE',  ( 115.7830029644259611, -41.80249729622526189, 104.4064416391778565 ) ) ;
#24247=AXIS2_PLACEMENT_3D ( 'NONE', #68990, #26748, #41709 ) ;
#24248=CARTESIAN_POINT ( 'NONE',  ( 142.0664832912740110, -9.729447159940995959, -4.824374724088994704 ) ) ;
#24249=ADVANCED_FACE ( 'NONE', ( #718 ), #64306, .F. ) ;
#24250=CARTESIAN_POINT ( 'NONE',  ( 112.4862084254573631, -26.19061110901967382, 169.6984824187679521 ) ) ;
#24252=CARTESIAN_POINT ( 'NONE',  ( 135.2499210002644361, -39.21189388395509923, 8.006199623927603426 ) ) ;
#24256=EDGE_CURVE ( 'NONE', #4393, #78803, #77479, .T. ) ;
#24257=CARTESIAN_POINT ( 'NONE',  ( 97.81801690659570170, -40.53285193764387628, 62.63741732645588911 ) ) ;
#24260=CARTESIAN_POINT ( 'NONE',  ( 103.0821812797523194, -45.97846664716049503, 283.6844404487542874 ) ) ;
#24262=CARTESIAN_POINT ( 'NONE',  ( 50.88849390559499142, -32.11662333284530746, 342.9256252759119548 ) ) ;
#24266=CARTESIAN_POINT ( 'NONE',  ( 108.9246099533292238, -44.86580503303185452, 9.635625275910941312 ) ) ;
#24267=CARTESIAN_POINT ( 'NONE',  ( 82.81648064515530905, -18.72944715939135207, 6.749772901088279653 ) ) ;
#24269=ORIENTED_EDGE ( 'NONE', *, *, #44119, .F. ) ;
#24270=EDGE_CURVE ( 'NONE', #35318, #18758, #48530, .T. ) ;
#24271=AXIS2_PLACEMENT_3D ( 'NONE', #4639, #72349, #38259 ) ;
#24274=CIRCLE ( 'NONE', #46018, 16.00000000000090239 ) ;
#24276=ORIENTED_EDGE ( 'NONE', *, *, #43628, .T. ) ;
#24279=CARTESIAN_POINT ( 'NONE',  ( 110.3271547037548004, -45.17815799167961899, 17.28003887569495944 ) ) ;
#24280=CARTESIAN_POINT ( 'NONE',  ( 114.9947137121727820, -28.99390558034420451, 194.4537205140059370 ) ) ;
#24281=CARTESIAN_POINT ( 'NONE',  ( 102.0922439024870982, -27.59239485085791088, 145.4727681330539610 ) ) ;
#24283=CARTESIAN_POINT ( 'NONE',  ( 115.6952998724001560, -42.57974731087075071, 269.3527681330536439 ) ) ;
#24284=CARTESIAN_POINT ( 'NONE',  ( 98.30749083302823976, -41.72877197732193366, 97.74043806258440270 ) ) ;
#24287=EDGE_CURVE ( 'NONE', #68689, #88451, #31993, .T. ) ;
#24288=ORIENTED_EDGE ( 'NONE', *, *, #29123, .F. ) ;
#24289=AXIS2_PLACEMENT_3D ( 'NONE', #50132, #30154, #28351 ) ;
#24290=ADVANCED_FACE ( 'NONE', ( #44275 ), #37927, .T. ) ;
#24292=CARTESIAN_POINT ( 'NONE',  ( 98.63028220664102719, -30.46987006685205657, 180.8184824187679567 ) ) ;
#24293=VERTEX_POINT ( 'NONE', #10656 ) ;
#24294=CARTESIAN_POINT ( 'NONE',  ( 114.2400596693416475, -45.14401474321602592, 153.1508633711489722 ) ) ;
#24295=CARTESIAN_POINT ( 'NONE',  ( 97.31587469920060585, -39.30605313440615589, 266.5315195702721667 ) ) ;
#24296=CARTESIAN_POINT ( 'NONE',  ( 73.06648329127401098, -46.72944715994108122, 14.82207188531766029 ) ) ;
#24297=LINE ( 'NONE', #79719, #52203 ) ;
#24298=CARTESIAN_POINT ( 'NONE',  ( 123.0079629938350223, -38.09664315643626509, 293.9356252759109793 ) ) ;
#24300=CARTESIAN_POINT ( 'NONE',  ( 37.03715912545349198, -48.62818131006128652, 117.4678068554150485 ) ) ;
#24301=CARTESIAN_POINT ( 'NONE',  ( 110.0853110376240664, -46.03288293484944660, 8.827053847338950376 ) ) ;
#24303=DIRECTION ( 'NONE',  ( 0.000000000000000000, 0.000000000000000000, 1.000000000000000000 ) ) ;
#24304=CYLINDRICAL_SURFACE ( 'NONE', #62959, 4.875000000000017764 ) ;
#24306=FACE_OUTER_BOUND ( 'NONE', #46014, .T. ) ;
#24307=CARTESIAN_POINT ( 'NONE',  ( 126.9629299006806065, -46.62589376934779750, -5.074374724088961841 ) ) ;
#24308=CARTESIAN_POINT ( 'NONE',  ( 104.9500019498489252, -44.48156792823318995, 195.5838068554170377 ) ) ;
#24309=ORIENTED_EDGE ( 'NONE', *, *, #55474, .T. ) ;
#24310=CARTESIAN_POINT ( 'NONE',  ( 149.4430470701762488, -12.91565541735124256, 378.4756252759100335 ) ) ;
#24311=CARTESIAN_POINT ( 'NONE',  ( 117.5094658089964241, -40.42262428419060427, 178.5680062282919778 ) ) ;
#24312=CARTESIAN_POINT ( 'NONE',  ( 98.09687384527185827, -31.41638835794072193, 81.90133956162493689 ) ) ;
#24313=CARTESIAN_POINT ( 'NONE',  ( 117.3777842326014706, -34.92111847156615312, 239.9641967044819637 ) ) ;
#24317=DIRECTION ( 'NONE',  ( 1.000000000000000000, 0.000000000000000000, 0.000000000000000000 ) ) ;
#24319=DIRECTION ( 'NONE',  ( 0.000000000000000000, 1.000000000000000000, 0.000000000000000000 ) ) ;
#24321=DIRECTION ( 'NONE',  ( -1.000000000000000078E-15, 1.000000000000000000, 0.000000000000000000 ) ) ;
#24322=ORIENTED_EDGE ( 'NONE', *, *, #2946, .F. ) ;
#24324=CARTESIAN_POINT ( 'NONE',  ( 99.03715563995052662, -32.54106229299839725, 90.35432458998199934 ) ) ;
#24326=EDGE_LOOP ( 'NONE', ( #82026, #34743, #10675, #86111 ) ) ;
#24327=CARTESIAN_POINT ( 'NONE',  ( 97.24623519876082867, -31.70684325556598893, 91.96229194257693962 ) ) ;
#24330=ADVANCED_FACE ( 'NONE', ( #38810 ), #52406, .F. ) ;
#24331=CARTESIAN_POINT ( 'NONE',  ( 182.0667039024480118, -32.29483332968430886, -5.074374724088000832 ) ) ;
#24333=CARTESIAN_POINT ( 'NONE',  ( 109.4546162266718454, -25.87086512622375878, 29.90419670448296685 ) ) ;
#24334=ORIENTED_EDGE ( 'NONE', *, *, #87426, .T. ) ;
#24337=EDGE_CURVE ( 'NONE', #68275, #74036, #77688, .T. ) ;
#24339=AXIS2_PLACEMENT_3D ( 'NONE', #56933, #22435, #15624 ) ;
#24340=CARTESIAN_POINT ( 'NONE',  ( 20.03715912545644073, -24.42818131006202265, 129.9678068554150627 ) ) ;
#24341=DIRECTION ( 'NONE',  ( -4.237773401492740281E-14, 1.000000000000000000, 0.000000000000000000 ) ) ;
#24342=LINE ( 'NONE', #43875, #84061 ) ;
#24344=DIRECTION ( 'NONE',  ( 0.000000000000000000, 0.000000000000000000, 1.000000000000000000 ) ) ;
#24346=DIRECTION ( 'NONE',  ( 0.000000000000000000, -1.000000000000000000, 0.000000000000000000 ) ) ;
#24349=CARTESIAN_POINT ( 'NONE',  ( 106.9276426037745011, -26.29176787048580266, 60.08705384733897858 ) ) ;
#24350=ORIENTED_EDGE ( 'NONE', *, *, #24943, .F. ) ;
#24352=CIRCLE ( 'NONE', #37443, 0.5000000000000016653 ) ;
#24355=VECTOR ( 'NONE', #70492, 1000.000000000000000 ) ;
#24358=CARTESIAN_POINT ( 'NONE',  ( 100.1874667927473439, -32.28399744105692548, 143.6880903695909524 ) ) ;
#24360=EDGE_CURVE ( 'NONE', #63598, #44371, #46049, .T. ) ;
#24362=DIRECTION ( 'NONE',  ( -1.000000000000000000, -4.299999999999999979E-14, -1.000000000000000078E-15 ) ) ;
#24363=ORIENTED_EDGE ( 'NONE', *, *, #22979, .T. ) ;
#24364=ORIENTED_EDGE ( 'NONE', *, *, #20576, .F. ) ;
#24365=PLANE ( 'NONE',  #7581 ) ;
#24366=EDGE_CURVE ( 'NONE', #59170, #19054, #74678, .T. ) ;
#24367=EDGE_LOOP ( 'NONE', ( #77806, #14373, #81585, #24930 ) ) ;
#24368=VERTEX_POINT ( 'NONE', #54201 ) ;
#24369=CARTESIAN_POINT ( 'NONE',  ( 115.7580415341064111, -34.85356206270782309, 180.4272975916109374 ) ) ;
#24373=CARTESIAN_POINT ( 'NONE',  ( 102.0670550486025121, -27.97049800993343993, 120.4897919345716133 ) ) ;
#24374=AXIS2_PLACEMENT_3D ( 'NONE', #62840, #76935, #1075 ) ;
#24375=CARTESIAN_POINT ( 'NONE',  ( 110.8567118704325623, -45.98332038337609617, 17.88581783518143453 ) ) ;
#24376=VERTEX_POINT ( 'NONE', #26087 ) ;
#24377=EDGE_CURVE ( 'NONE', #26375, #40569, #89666, .T. ) ;
#24378=VERTEX_POINT ( 'NONE', #41480 ) ;
#24380=EDGE_CURVE ( 'NONE', #19753, #9456, #5194, .T. ) ;
#24381=B_SPLINE_CURVE_WITH_KNOTS ( 'NONE', 3,
 ( #15923, #9550, #71339, #64515, #56784, #29999, #85869, #64958, #84533, #22290, #76794, #57689, #9111, #85432, #23207, #50874, #44044, #71779, #78612, #37255, #30442, #58137, #943, #59901, #31311, #52623, #11320, #4516, #65832, #66731, #52180, #87192, #38139, #10436, #16811, #3616, #87633, #39021 ),
 .UNSPECIFIED., .F., .F.,
 ( 4, 2, 2, 1, 2, 2, 2, 2, 1, 1, 2, 2, 2, 1, 2, 2, 1, 2, 1, 2, 2, 4 ),
 ( 0.000000000000000000, 0.04166793602358854348, 0.05208492002948607313, 0.05729341203243450142, 0.05989765803390947191, 0.06250190403538444239, 0.08333587204719075658, 0.1041698400589970708, 0.1145868240649016850, 0.1197953160678549983, 0.1223995620693313774, 0.1250038080708077703, 0.1666717440944421869, 0.1770887281003535874, 0.1822972201033092876, 0.1875057121062650156, 0.2083396801180918412, 0.2291736481299186945, 0.2395906321358344804, 0.2447991241387921235, 0.2500076161417498222, 0.3333434881890884882 ),
 .UNSPECIFIED. ) ;
#24382=CARTESIAN_POINT ( 'NONE',  ( 111.0898924481313941, -43.83169361959101451, 210.8052332267339750 ) ) ;
#24384=CARTESIAN_POINT ( 'NONE',  ( 107.3215719809018083, -25.65558735872630081, 75.04610146638695767 ) ) ;
#24385=CARTESIAN_POINT ( 'NONE',  ( 111.3142535964730797, -27.23286288913589459, 24.74133956162494030 ) ) ;
#24389=CARTESIAN_POINT ( 'NONE',  ( 96.65005459693196599, -37.15429219901626823, 157.3584824187679487 ) ) ;
#24391=ORIENTED_EDGE ( 'NONE', *, *, #47744, .T. ) ;
#24393=EDGE_LOOP ( 'NONE', ( #18438, #12321, #45767, #61571 ) ) ;
#24395=DIRECTION ( 'NONE',  ( 0.000000000000000000, 1.000000000000000000, 0.000000000000000000 ) ) ;
#24396=DIRECTION ( 'NONE',  ( 0.000000000000000000, 0.000000000000000000, -1.000000000000000000 ) ) ;
#24398=CIRCLE ( 'NONE', #73800, 5.599999999999994316 ) ;
#24403=CARTESIAN_POINT ( 'NONE',  ( 104.0426969376867987, -47.36127689622573200, 67.36800622829191809 ) ) ;
#24406=CARTESIAN_POINT ( 'NONE',  ( 100.8874678934932518, -44.70022138198631012, 73.05229194346932786 ) ) ;
#24407=CARTESIAN_POINT ( 'NONE',  ( 116.7343647603066614, -32.97833357388812914, 94.10895860924495082 ) ) ;
#24409=CARTESIAN_POINT ( 'NONE',  ( 97.78191787992085438, -41.50032452247405246, 192.7041967044819728 ) ) ;
#24410=CARTESIAN_POINT ( 'NONE',  ( 113.2418788616994618, -28.75590518149876118, 59.55265118002041902 ) ) ;
#24412=ORIENTED_EDGE ( 'NONE', *, *, #34723, .F. ) ;
#24413=DIRECTION ( 'NONE',  ( 0.7071067811743789733, -0.7071067811987160612, 0.000000000000000000 ) ) ;
#24415=CARTESIAN_POINT ( 'NONE',  ( 97.80441965743102628, -40.49963042538360725, 136.6344769046315832 ) ) ;
#24416=CIRCLE ( 'NONE', #75181, 11.45913725231036118 ) ;
#24418=CARTESIAN_POINT ( 'NONE',  ( 114.8468557742592822, -29.67128889090990640, 209.4127681330539872 ) ) ;
#24420=CARTESIAN_POINT ( 'NONE',  ( 97.75843951370882223, -40.38502501680090973, 146.6242685447254246 ) ) ;
#24421=CARTESIAN_POINT ( 'NONE',  ( 100.8354465997397540, -45.15876371340904427, 253.0699109901969450 ) ) ;
#24422=CARTESIAN_POINT ( 'NONE',  ( 117.2645927648968183, -42.86211997589052203, 124.3956252759109731 ) ) ;
#24423=CIRCLE ( 'NONE', #86791, 11.45913725231036118 ) ;
#24424=CARTESIAN_POINT ( 'NONE',  ( 105.8028360693176495, -26.72358448476759918, 251.1828494030555703 ) ) ;
#24425=VECTOR ( 'NONE', #51308, 1000.000000000000114 ) ;
#24427=CARTESIAN_POINT ( 'NONE',  ( 82.51464772713113405, -37.98222059078202761, 7.138441653511359952 ) ) ;
#24429=CARTESIAN_POINT ( 'NONE',  ( 188.5667039024481255, -42.82844715993431350, 257.2178068554150059 ) ) ;
#24434=ORIENTED_EDGE ( 'NONE', *, *, #14623, .F. ) ;
#24436=CARTESIAN_POINT ( 'NONE',  ( 116.1395517938576347, -31.55217135963209785, 285.2384824187680579 ) ) ;
#24437=DIRECTION ( 'NONE',  ( 1.000000000000000000, 0.000000000000000000, 0.000000000000000000 ) ) ;
#24438=CARTESIAN_POINT ( 'NONE',  ( 132.5731111080349649, -34.41810224487143444, 1.981704920702773043 ) ) ;
#24439=CARTESIAN_POINT ( 'NONE',  ( 34.33598329127477911, -36.32844715994133367, 237.4678068554150059 ) ) ;
#24441=AXIS2_PLACEMENT_3D ( 'NONE', #4584, #25023, #45883 ) ;
#24442=CARTESIAN_POINT ( 'NONE',  ( 102.2605585157881194, -43.79055321879850027, 196.5238483995059937 ) ) ;
#24443=ORIENTED_EDGE ( 'NONE', *, *, #3124, .F. ) ;
#24446=ORIENTED_EDGE ( 'NONE', *, *, #52906, .T. ) ;
#24447=EDGE_CURVE ( 'NONE', #50547, #77225, #75585, .T. ) ;
#24448=CARTESIAN_POINT ( 'NONE',  ( 51.27381068362099370, -23.19206098993950604, -5.074374724088000832 ) ) ;
#24449=DIRECTION ( 'NONE',  ( 0.000000000000000000, -1.000000000000000000, 0.000000000000000000 ) ) ;
#24450=DIRECTION ( 'NONE',  ( 0.000000000000000000, 1.000000000000000000, 0.000000000000000000 ) ) ;
#24451=CARTESIAN_POINT ( 'NONE',  ( 98.80858115845356338, -33.43260291865056644, 37.45586902018299469 ) ) ;
#24455=ORIENTED_EDGE ( 'NONE', *, *, #7060, .F. ) ;
#24459=CARTESIAN_POINT ( 'NONE',  ( 162.7866693523300796, -36.02818131005322044, 117.4678068554150485 ) ) ;
#24460=CARTESIAN_POINT ( 'NONE',  ( 112.5662596640460720, -44.20262526656594559, 30.89951894101994156 ) ) ;
#24461=AXIS2_PLACEMENT_3D ( 'NONE', #51878, #17391, #59154 ) ;
#24462=CONICAL_SURFACE ( 'NONE', #75232, 1.258750000000002922, 1.029744258676650093 ) ;
#24465=EDGE_CURVE ( 'NONE', #67541, #17862, #47181, .T. ) ;
#24466=FACE_OUTER_BOUND ( 'NONE', #22996, .T. ) ;
#24471=EDGE_CURVE ( 'NONE', #60222, #9337, #79122, .T. ) ;
#24473=CARTESIAN_POINT ( 'NONE',  ( 98.14942788562998999, -43.26130833009477783, 106.8175300378159704 ) ) ;
#24475=EDGE_CURVE ( 'NONE', #34264, #85910, #19274, .T. ) ;
#24476=CARTESIAN_POINT ( 'NONE',  ( 115.5202298134134367, -37.95022619834508504, 28.13527697093398672 ) ) ;
#24478=DIRECTION ( 'NONE',  ( -0.7071067811865501263, 0.7071067811865449082, -7.071067811865501957E-16 ) ) ;
#24479=CARTESIAN_POINT ( 'NONE',  ( 99.97388925556708728, -42.04201607304819532, 63.27015473446895300 ) ) ;
#24480=CARTESIAN_POINT ( 'NONE',  ( 115.7823355676851946, -41.80361319518412699, 14.40633917731446445 ) ) ;
#24481=EDGE_CURVE ( 'NONE', #59994, #61557, #9473, .T. ) ;
#24482=CARTESIAN_POINT ( 'NONE',  ( 46.83715912545345361, -47.82818131006086304, 117.4678068554150485 ) ) ;
#24483=LINE ( 'NONE', #24922, #36819 ) ;
#24484=CARTESIAN_POINT ( 'NONE',  ( 116.4941038412854510, -32.22865339830268283, 15.18133956162492915 ) ) ;
#24486=VERTEX_POINT ( 'NONE', #46948 ) ;
#24487=CARTESIAN_POINT ( 'NONE',  ( 156.5667039024484666, -42.82844715993568485, 139.7178068554149775 ) ) ;
#24489=CARTESIAN_POINT ( 'NONE',  ( 77.61460381940941033, -19.97617057400826468, 2.716753174556971295 ) ) ;
#24491=ORIENTED_EDGE ( 'NONE', *, *, #57290, .F. ) ;
#24492=EDGE_CURVE ( 'NONE', #35045, #66245, #74238, .T. ) ;
#24494=CARTESIAN_POINT ( 'NONE',  ( 109.9476544338203325, -26.76763818355050262, 214.8403871806739289 ) ) ;
#24495=CARTESIAN_POINT ( 'NONE',  ( 168.3595971213392772, -48.62134037882587023, 180.4678068554150059 ) ) ;
#24496=CARTESIAN_POINT ( 'NONE',  ( 112.0659115689755083, -45.48839629194433343, 188.9897919376950028 ) ) ;
#24497=CARTESIAN_POINT ( 'NONE',  ( 103.9574082008755198, -47.33640867427461529, 58.33753003781600199 ) ) ;
#24498=CARTESIAN_POINT ( 'NONE',  ( 98.38030477604230839, -41.69506886831626957, 42.73974658533858673 ) ) ;
#24499=ORIENTED_EDGE ( 'NONE', *, *, #53074, .F. ) ;
#24500=CARTESIAN_POINT ( 'NONE',  ( 115.1227284505533959, -30.77440371158323629, 170.3330730039945706 ) ) ;
#24501=DIRECTION ( 'NONE',  ( 0.7071067811865460184, 0.000000000000000000, 0.7071067811865487940 ) ) ;
#24504=LINE ( 'NONE', #32190, #15546 ) ;
#24506=CARTESIAN_POINT ( 'NONE',  ( 118.0585799961421429, -32.36802338489820841, 249.1270538473389706 ) ) ;
#24507=DIRECTION ( 'NONE',  ( -1.000000000000000000, -4.510281037539694659E-14, 0.000000000000000000 ) ) ;
#24509=CARTESIAN_POINT ( 'NONE',  ( 78.98444042533921561, -39.25772566032940603, 1.807989669955163414 ) ) ;
#24510=CARTESIAN_POINT ( 'NONE',  ( 114.8821461825539245, -40.17495804977037466, 252.9181341137911545 ) ) ;
#24512=CARTESIAN_POINT ( 'NONE',  ( 115.1498815335950638, -43.27828968249928465, 84.28419670448195689 ) ) ;
#24514=CARTESIAN_POINT ( 'NONE',  ( 116.9458863120112539, -40.19413502446316500, 133.5584824187679658 ) ) ;
#24516=CARTESIAN_POINT ( 'NONE',  ( 25.56670390244797275, -58.35344715994099829, 295.9678068554150059 ) ) ;
#24517=ORIENTED_EDGE ( 'NONE', *, *, #24575, .F. ) ;
#24518=DIRECTION ( 'NONE',  ( 0.000000000000000000, 0.000000000000000000, -1.000000000000000000 ) ) ;
#24519=CARTESIAN_POINT ( 'NONE',  ( 194.5667039024480403, -40.82844715993405771, 249.9678068554149775 ) ) ;
#24520=EDGE_LOOP ( 'NONE', ( #62448, #61644, #1293, #6392 ) ) ;
#24523=CARTESIAN_POINT ( 'NONE',  ( 117.1490187775317793, -39.54886983357372543, 98.60991099019594230 ) ) ;
#24529=LINE ( 'NONE', #3198, #51062 ) ;
#24530=ORIENTED_EDGE ( 'NONE', *, *, #64063, .F. ) ;
#24532=CARTESIAN_POINT ( 'NONE',  ( 109.2596401224901541, -46.98022400537049492, 107.7441967044829880 ) ) ;
#24534=DIRECTION ( 'NONE',  ( 0.000000000000000000, 0.000000000000000000, -1.000000000000000000 ) ) ;
#24535=EDGE_CURVE ( 'NONE', #31678, #52430, #13355, .T. ) ;
#24536=CARTESIAN_POINT ( 'NONE',  ( 162.7131505118679797, -31.94127993907790852, -5.074374724088000832 ) ) ;
#24537=CARTESIAN_POINT ( 'NONE',  ( 141.8664832912739939, -71.52944715994085811, 361.9756252759100335 ) ) ;
#24538=ORIENTED_EDGE ( 'NONE', *, *, #53290, .F. ) ;
#24539=AXIS2_PLACEMENT_3D ( 'NONE', #52700, #65480, #66357 ) ;
#24541=CARTESIAN_POINT ( 'NONE',  ( 107.0664832912739968, -0.2185775633790978945, 330.8831252759119934 ) ) ;
#24542=LINE ( 'NONE', #87216, #32358 ) ;
#24543=VECTOR ( 'NONE', #38858, 1000.000000000000000 ) ;
#24544=DIRECTION ( 'NONE',  ( -0.7071067811864691910, -0.7071067811866257324, -7.071067811864685486E-16 ) ) ;
#24545=LINE ( 'NONE', #52208, #79901 ) ;
#24546=FACE_BOUND ( 'NONE', #5819, .T. ) ;
#24548=EDGE_LOOP ( 'NONE', ( #64182, #5003 ) ) ;
#24550=CARTESIAN_POINT ( 'NONE',  ( 104.4081008449446983, -46.45808918883411565, 33.36479195756466254 ) ) ;
#24551=CARTESIAN_POINT ( 'NONE',  ( 96.81359797424460112, -35.17473563989039320, 217.1946728949579608 ) ) ;
#24552=AXIS2_PLACEMENT_3D ( 'NONE', #69084, #82284, #14118 ) ;
#24553=B_SPLINE_CURVE_WITH_KNOTS ( 'NONE', 3,
 ( #52705, #80465, #45904, #39110, #54505, #47702, #82268, #20920, #5958, #34538, #27728, #68623, #6387, #61338, #82718, #75442, #40897, #69066, #40456, #61781, #20479, #14104, #7296, #67719, #76324, #48149, #62241, #83163, #6835 ),
 .UNSPECIFIED., .F., .F.,
 ( 4, 2, 2, 2, 2, 2, 2, 2, 2, 2, 1, 1, 1, 1, 1, 2, 4 ),
 ( 0.000000000000000000, 0.06250186912378230542, 0.1250037382475646108, 0.1875056073713469162, 0.2500074764951292217, 0.3125093456189115271, 0.3750112147426938325, 0.4375130838664761379, 0.4687640184283670686, 0.4843894857093126172, 0.4922022193497853082, 0.4961085861700220145, 0.4980617695801402012, 0.4990383612851991835, 0.4995266571377283693, 0.4997708050639932953, 0.5000149529902581103 ),
 .UNSPECIFIED. ) ;
#24556=CARTESIAN_POINT ( 'NONE',  ( 114.5308976578478166, -43.10096916487045604, 59.26419670448196086 ) ) ;
#24558=CARTESIAN_POINT ( 'NONE',  ( 165.6738106836196494, -26.00627455219358453, 342.9256252759109884 ) ) ;
#24559=EDGE_CURVE ( 'NONE', #17862, #65985, #47397, .T. ) ;
#24563=EDGE_LOOP ( 'NONE', ( #38432, #73467, #40851, #77224 ) ) ;
#24564=CARTESIAN_POINT ( 'NONE',  ( 98.23266987703472353, -35.71659467859123538, 202.6672975916109465 ) ) ;
#24567=CARTESIAN_POINT ( 'NONE',  ( 152.4409905591762708, -0.9151414768250908383, 394.9756252759102040 ) ) ;
#24568=DIRECTION ( 'NONE',  ( 0.000000000000000000, 0.000000000000000000, -1.000000000000000000 ) ) ;
#24569=ORIENTED_EDGE ( 'NONE', *, *, #57475, .T. ) ;
#24571=CARTESIAN_POINT ( 'NONE',  ( 71.24189083761808661, -0.9290567490904538817, 540.9756252759101471 ) ) ;
#24572=ORIENTED_EDGE ( 'NONE', *, *, #74802, .T. ) ;
#24573=CARTESIAN_POINT ( 'NONE',  ( 111.8540205700169139, -46.00543295620339990, 272.9556252759110180 ) ) ;
#24574=DIRECTION ( 'NONE',  ( 0.000000000000000000, 0.000000000000000000, -1.000000000000000000 ) ) ;
#24575=EDGE_CURVE ( 'NONE', #59746, #23716, #29839, .T. ) ;
#24576=ORIENTED_EDGE ( 'NONE', *, *, #87650, .T. ) ;
#24577=AXIS2_PLACEMENT_3D ( 'NONE', #34116, #63178, #56347 ) ;
#24578=FACE_OUTER_BOUND ( 'NONE', #89172, .T. ) ;
#24582=CARTESIAN_POINT ( 'NONE',  ( 110.5132149073354242, -26.84445748292755951, 205.8099109901969541 ) ) ;
#24585=CIRCLE ( 'NONE', #60885, 3.000000000000002665 ) ;
#24587=CARTESIAN_POINT ( 'NONE',  ( 96.14773132834588409, -38.72402830165600562, 47.48229194257797303 ) ) ;
#24588=LINE ( 'NONE', #17772, #20740 ) ;
#24589=EDGE_LOOP ( 'NONE', ( #89184, #26245, #24058, #1600 ) ) ;
#24591=EDGE_CURVE ( 'NONE', #42455, #17322, #80605, .T. ) ;
#24593=CARTESIAN_POINT ( 'NONE',  ( 78.34779240610842521, -38.87777042261290461, 7.743969477056507955 ) ) ;
#24594=CARTESIAN_POINT ( 'NONE',  ( 97.81483072311490901, -40.51614641965803543, 17.63529977666319937 ) ) ;
#24596=CARTESIAN_POINT ( 'NONE',  ( 100.8868511195287567, -44.69971074744904627, 152.0528254920112943 ) ) ;
#24597=CARTESIAN_POINT ( 'NONE',  ( 114.6841822258597148, -33.79680514827971649, 136.9366617981629588 ) ) ;
#24598=CARTESIAN_POINT ( 'NONE',  ( 106.5662934289835988, -47.19983425457502335, 243.5384824187679556 ) ) ;
#24602=CARTESIAN_POINT ( 'NONE',  ( 135.3687878533317246, -39.15209318185264209, 1.893168666202053041 ) ) ;
#24604=ORIENTED_EDGE ( 'NONE', *, *, #2861, .T. ) ;
#24606=EDGE_LOOP ( 'NONE', ( #10294, #23711 ) ) ;
#24608=DIRECTION ( 'NONE',  ( 1.000000000000000000, 1.261617073437676668E-15, 1.261617073437676668E-15 ) ) ;
#24610=CARTESIAN_POINT ( 'NONE',  ( 51.56670390244899238, -32.29483332968450782, -5.074374724088000832 ) ) ;
#24611=VECTOR ( 'NONE', #83956, 1000.000000000000000 ) ;
#24612=CARTESIAN_POINT ( 'NONE',  ( 116.7648798213666623, -36.26930322673007367, 118.2867055423629807 ) ) ;
#24613=CARTESIAN_POINT ( 'NONE',  ( 118.1222316836501705, -37.72106760768119216, 33.74324432352998571 ) ) ;
#24615=CARTESIAN_POINT ( 'NONE',  ( 164.9190312289449878, -35.91149509761181235, -5.074374724088000832 ) ) ;
#24616=VERTEX_POINT ( 'NONE', #84203 ) ;
#24618=VERTEX_POINT ( 'NONE', #83744 ) ;
#24624=CARTESIAN_POINT ( 'NONE',  ( 97.21658504226680009, -33.31410993950169086, 286.0613395616252888 ) ) ;
#24625=CARTESIAN_POINT ( 'NONE',  ( 111.0628700864597533, -47.08446675046669583, 13.85753003781498016 ) ) ;
#24626=CARTESIAN_POINT ( 'NONE',  ( 138.0667039024480971, -58.72944715994091069, 199.5838068554170093 ) ) ;
#24628=DIRECTION ( 'NONE',  ( 0.000000000000000000, 0.000000000000000000, -1.000000000000000000 ) ) ;
#24629=DIRECTION ( 'NONE',  ( 0.9963424814100680926, -0.08544974978095730422, 0.000000000000000000 ) ) ;
#24630=DIRECTION ( 'NONE',  ( 0.000000000000000000, 0.000000000000000000, -1.000000000000000000 ) ) ;
#24632=LINE ( 'NONE', #52299, #72132 ) ;
#24633=CARTESIAN_POINT ( 'NONE',  ( 115.0376101259158901, -42.90801517561737910, 163.3021728873967788 ) ) ;
#24636=CARTESIAN_POINT ( 'NONE',  ( 96.64524470886469487, -32.90705862865544162, 21.03467289495897319 ) ) ;
#24637=CARTESIAN_POINT ( 'NONE',  ( 114.8139851684208992, -29.70110827795256014, 205.4127681330539872 ) ) ;
#24638=CARTESIAN_POINT ( 'NONE',  ( 96.69317630666223806, -38.23732580652426094, 62.44133956162495025 ) ) ;
#24640=CARTESIAN_POINT ( 'NONE',  ( 128.0667039024480118, -58.72944715994110254, 310.9178068554150514 ) ) ;
#24641=DIRECTION ( 'NONE',  ( -0.7071067811869841124, 0.7071067811861110330, 0.000000000000000000 ) ) ;
#24642=AXIS2_PLACEMENT_3D ( 'NONE', #88965, #88077, #41236 ) ;
#24645=CARTESIAN_POINT ( 'NONE',  ( 102.0670550238970407, -27.97049802371184768, 186.4897919368071939 ) ) ;
#24646=ORIENTED_EDGE ( 'NONE', *, *, #2061, .F. ) ;
#24647=CARTESIAN_POINT ( 'NONE',  ( 106.8551140066829817, -47.84553036069057441, 73.56133956162396714 ) ) ;
#24650=FACE_OUTER_BOUND ( 'NONE', #20947, .T. ) ;
#24652=LINE ( 'NONE', #23346, #50449 ) ;
#24653=CARTESIAN_POINT ( 'NONE',  ( 113.7851844261089695, -26.99768152489570738, 235.5956252759109759 ) ) ;
#24654=DIRECTION ( 'NONE',  ( 1.000000000000000000, 4.163336342344333240E-14, 0.000000000000000000 ) ) ;
#24656=CARTESIAN_POINT ( 'NONE',  ( 168.0371591254543375, -48.62818131005499822, 300.4678068554149490 ) ) ;
#24657=CARTESIAN_POINT ( 'NONE',  ( 193.5667039024485803, -48.82844715993409324, 180.4678068554150343 ) ) ;
#24659=ADVANCED_FACE ( 'NONE', ( #55542 ), #62830, .F. ) ;
#24660=DIRECTION ( 'NONE',  ( -0.9254794337955620787, -0.3787978585227822492, 0.000000000000000000 ) ) ;
#24663=CARTESIAN_POINT ( 'NONE',  ( 116.6769215743980936, -34.91203320259893417, 158.9756252759109714 ) ) ;
#24665=ORIENTED_EDGE ( 'NONE', *, *, #89661, .T. ) ;
#24666=EDGE_CURVE ( 'NONE', #77124, #54148, #44266, .T. ) ;
#24667=CARTESIAN_POINT ( 'NONE',  ( 99.30241108408027628, -32.39570601076609080, 107.3530118773259545 ) ) ;
#24668=CYLINDRICAL_SURFACE ( 'NONE', #61724, 9.999999999999998224 ) ;
#24669=CARTESIAN_POINT ( 'NONE',  ( 109.9476544338203041, -26.76763818355061986, 210.8403871806729626 ) ) ;
#24670=DIRECTION ( 'NONE',  ( 0.000000000000000000, 0.000000000000000000, 1.000000000000000000 ) ) ;
#24672=EDGE_CURVE ( 'NONE', #16560, #38408, #57371, .T. ) ;
#24674=VECTOR ( 'NONE', #78388, 1000.000000000000000 ) ;
#24677=CARTESIAN_POINT ( 'NONE',  ( 134.0664832912740110, -46.42944715994100591, -0.5743747240890021422 ) ) ;
#24679=CARTESIAN_POINT ( 'NONE',  ( 108.9412587213991088, -26.46057952311815953, 164.9327681330529742 ) ) ;
#24680=ORIENTED_EDGE ( 'NONE', *, *, #73167, .T. ) ;
#24682=ORIENTED_EDGE ( 'NONE', *, *, #15204, .F. ) ;
#24686=CARTESIAN_POINT ( 'NONE',  ( 62.03715912545838762, -47.82818131006021645, 249.9678068554150343 ) ) ;
#24688=CARTESIAN_POINT ( 'NONE',  ( 105.7154619534882016, -46.72385643955875878, 268.4689573849462363 ) ) ;
#24689=CARTESIAN_POINT ( 'NONE',  ( 97.67451187568107684, -41.25469890874477841, 171.6841967044819626 ) ) ;
#24690=DIRECTION ( 'NONE',  ( -1.000000000000000078E-15, 1.000000000000000083E-30, 1.000000000000000000 ) ) ;
#24692=ORIENTED_EDGE ( 'NONE', *, *, #5701, .T. ) ;
#24693=ORIENTED_EDGE ( 'NONE', *, *, #75266, .T. ) ;
#24694=AXIS2_PLACEMENT_3D ( 'NONE', #10380, #3122, #78987 ) ;
#24698=ADVANCED_FACE ( 'NONE', ( #38158 ), #2284, .F. ) ;
#24699=CARTESIAN_POINT ( 'NONE',  ( 109.6422123260156383, -46.48028807993739520, 163.7813936359489162 ) ) ;
#24701=CARTESIAN_POINT ( 'NONE',  ( 98.11614316284976667, -39.58741349592436620, 277.9920594963732015 ) ) ;
#24702=AXIS2_PLACEMENT_3D ( 'NONE', #44622, #65530, #80511 ) ;
#24704=ORIENTED_EDGE ( 'NONE', *, *, #86919, .F. ) ;
#24705=EDGE_CURVE ( 'NONE', #21703, #13421, #67653, .T. ) ;
#24706=CARTESIAN_POINT ( 'NONE',  ( 99.66264782090949836, -39.75983002812326106, 9.635625275910941312 ) ) ;
#24709=VECTOR ( 'NONE', #16470, 1000.000000000000000 ) ;
#24710=ORIENTED_EDGE ( 'NONE', *, *, #59303, .F. ) ;
#24712=VERTEX_POINT ( 'NONE', #32223 ) ;
#24714=CARTESIAN_POINT ( 'NONE',  ( 112.1371669992097964, -28.01157492980850350, 155.6564172018965166 ) ) ;
#24715=CARTESIAN_POINT ( 'NONE',  ( 113.9308110932664704, -41.86102644448636312, 27.73813411379200033 ) ) ;
#24716=AXIS2_PLACEMENT_3D ( 'NONE', #22272, #15461, #43581 ) ;
#24717=CARTESIAN_POINT ( 'NONE',  ( 101.3369781660191222, -46.20933176663394448, 202.1318157521019430 ) ) ;
#24718=CARTESIAN_POINT ( 'NONE',  ( 108.6716496925947126, -26.45072611336619772, 189.9527681330539792 ) ) ;
#24720=CARTESIAN_POINT ( 'NONE',  ( 106.5673366543293383, -47.17799660047543853, 243.5384824187679556 ) ) ;
#24721=CARTESIAN_POINT ( 'NONE',  ( 97.81413651554109379, -40.51640884438177181, 97.63607350422876152 ) ) ;
#24722=CARTESIAN_POINT ( 'NONE',  ( 182.2300522401177432, -33.89581943343662118, 237.4678068554150059 ) ) ;
#24723=ORIENTED_EDGE ( 'NONE', *, *, #38969, .F. ) ;
#24726=DIRECTION ( 'NONE',  ( -0.7071067811865453523, -0.7071067811865496822, -7.071067811865460542E-16 ) ) ;
#24727=CARTESIAN_POINT ( 'NONE',  ( 104.1736071946568103, -26.63078081164005440, 225.2984824187679749 ) ) ;
#24729=CARTESIAN_POINT ( 'NONE',  ( 99.10121394234140269, -45.50393173043428163, 156.9899109901969609 ) ) ;
#24730=CARTESIAN_POINT ( 'NONE',  ( 165.9667039024459996, -26.71338133339301635, 342.9256252759109884 ) ) ;
#24736=CARTESIAN_POINT ( 'NONE',  ( 105.2810544170623359, -46.37316503544239765, 8.429910990195965681 ) ) ;
#24737=DIRECTION ( 'NONE',  ( 0.000000000000000000, 1.000000000000000000, 0.000000000000000000 ) ) ;
#24738=CYLINDRICAL_SURFACE ( 'NONE', #61275, 2.750000000000002665 ) ;
#24742=LINE ( 'NONE', #37929, #3904 ) ;
#24743=DIRECTION ( 'NONE',  ( 0.000000000000000000, 0.000000000000000000, -1.000000000000000000 ) ) ;
#24744=CARTESIAN_POINT ( 'NONE',  ( 112.8613057705799605, -28.86133510866265084, 195.5838068554167819 ) ) ;
#24745=ORIENTED_EDGE ( 'NONE', *, *, #12685, .T. ) ;
#24746=CARTESIAN_POINT ( 'NONE',  ( 101.4133560641720067, -46.25507541695031222, 207.1622919425779514 ) ) ;
#24747=CARTESIAN_POINT ( 'NONE',  ( 114.7713543040237454, -44.65465650488444993, 114.2022919425779719 ) ) ;
#24748=CARTESIAN_POINT ( 'NONE',  ( 100.6107886340239901, -26.73269172650989489, 216.5327681330539633 ) ) ;
#24749=CYLINDRICAL_SURFACE ( 'NONE', #60681, 0.9999999999999800160 ) ;
#24750=DIRECTION ( 'NONE',  ( 2.999999999999999839E-15, -1.000000000000000000, 2.999999999999999900E-30 ) ) ;
#24751=VECTOR ( 'NONE', #55600, 1000.000000000000000 ) ;
#24753=CARTESIAN_POINT ( 'NONE',  ( 106.8019215826475943, -46.78094778693688482, 38.55552475618427621 ) ) ;
#24755=FACE_OUTER_BOUND ( 'NONE', #1833, .T. ) ;
#24756=CARTESIAN_POINT ( 'NONE',  ( 115.0910585283885865, -30.62042626667451728, 64.34441744103244787 ) ) ;
#24757=B_SPLINE_CURVE_WITH_KNOTS ( 'NONE', 3,
 ( #41599, #68440, #27543, #49316, #727, #7999, #35695, #69782, #63408, #33905, #1191, #56584, #62510, #40716, #83411, #69333, #41156, #34801 ),
 .UNSPECIFIED., .F., .F.,
 ( 4, 2, 2, 2, 2, 2, 2, 2, 4 ),
 ( 0.4999999957683650686, 0.5624999962973193934, 0.6249999968262738292, 0.6874999973552281540, 0.7499999978841824788, 0.8124999984131369146, 0.8749999989420912394, 0.9374999994710455642, 1.000000000000000000 ),
 .UNSPECIFIED. ) ;
#24758=ORIENTED_EDGE ( 'NONE', *, *, #29409, .F. ) ;
#24759=EDGE_CURVE ( 'NONE', #29576, #74086, #52991, .T. ) ;
#24761=CARTESIAN_POINT ( 'NONE',  ( 100.5019087779429015, -42.19410572027086914, 116.3009912566479471 ) ) ;
#24762=EDGE_CURVE ( 'NONE', #61450, #37451, #28320, .T. ) ;
#24765=CARTESIAN_POINT ( 'NONE',  ( 107.6020193903983966, -26.30459096080998904, 91.03562527591097364 ) ) ;
#24767=AXIS2_PLACEMENT_3D ( 'NONE', #78879, #38847, #30706 ) ;
#24768=VECTOR ( 'NONE', #87662, 1000.000000000000000 ) ;
#24769=CARTESIAN_POINT ( 'NONE',  ( 20.03715912545644073, -24.42818131006202265, 129.9678068554150627 ) ) ;
#24770=EDGE_CURVE ( 'NONE', #61077, #16601, #59918, .T. ) ;
#24771=EDGE_CURVE ( 'NONE', #10976, #14667, #60204, .T. ) ;
#24773=DIRECTION ( 'NONE',  ( 0.7071067811865525687, -0.7071067811865425767, 7.071067811865533512E-16 ) ) ;
#24774=CARTESIAN_POINT ( 'NONE',  ( 106.3024736416914493, -26.94527301106431949, 25.13848241876892686 ) ) ;
#24776=VERTEX_POINT ( 'NONE', #52200 ) ;
#24778=ORIENTED_EDGE ( 'NONE', *, *, #88789, .T. ) ;
#24779=ADVANCED_FACE ( 'NONE', ( #46737 ), #25416, .T. ) ;
#24781=CARTESIAN_POINT ( 'NONE',  ( 106.1376555893193370, -47.80867374849567852, 108.5099109901959622 ) ) ;
#24783=DIRECTION ( 'NONE',  ( -1.000000000000000000, -4.299999999999999979E-14, -1.000000000000000078E-15 ) ) ;
#24784=ADVANCED_FACE ( 'NONE', ( #73115 ), #67195, .F. ) ;
#24786=VECTOR ( 'NONE', #19910, 1000.000000000000000 ) ;
#24787=DIRECTION ( 'NONE',  ( 0.000000000000000000, 0.000000000000000000, -1.000000000000000000 ) ) ;
#24789=LINE ( 'NONE', #57621, #67575 ) ;
#24790=CARTESIAN_POINT ( 'NONE',  ( 115.7104945841387718, -43.58108136993647719, 48.30514908543492680 ) ) ;
#24791=EDGE_LOOP ( 'NONE', ( #31592, #40648, #52683, #22682 ) ) ;
#24793=ORIENTED_EDGE ( 'NONE', *, *, #16790, .F. ) ;
#24794=CARTESIAN_POINT ( 'NONE',  ( 33.96670390244737803, -26.71338133339334320, 313.9678068554150059 ) ) ;
#24795=CYLINDRICAL_SURFACE ( 'NONE', #35939, 9.999999999999998224 ) ;
#24797=CARTESIAN_POINT ( 'NONE',  ( 108.7381085716129263, -28.73974155568626898, 137.7309475124479548 ) ) ;
#24798=ADVANCED_FACE ( 'NONE', ( #32677 ), #33129, .T. ) ;
#24799=AXIS2_PLACEMENT_3D ( 'NONE', #29627, #78701, #2381 ) ;
#24801=ORIENTED_EDGE ( 'NONE', *, *, #49803, .T. ) ;
#24802=ORIENTED_EDGE ( 'NONE', *, *, #64363, .F. ) ;
#24803=CYLINDRICAL_SURFACE ( 'NONE', #49625, 2.030000000001311644 ) ;
#24804=AXIS2_PLACEMENT_3D ( 'NONE', #76377, #29570, #84104 ) ;
#24805=ORIENTED_EDGE ( 'NONE', *, *, #10224, .F. ) ;
#24808=VECTOR ( 'NONE', #39814, 1000.000000000000000 ) ;
#24809=EDGE_CURVE ( 'NONE', #1463, #34216, #25869, .T. ) ;
#24810=CARTESIAN_POINT ( 'NONE',  ( 103.4772640228778329, -44.83165572645120278, 173.6758690201829438 ) ) ;
#24812=EDGE_CURVE ( 'NONE', #45647, #56272, #19052, .T. ) ;
#24814=DIRECTION ( 'NONE',  ( 3.999999999999999995E-14, -1.000000000000000000, 4.100000000000000342E-29 ) ) ;
#24816=VERTEX_POINT ( 'NONE', #66296 ) ;
#24818=CIRCLE ( 'NONE', #26241, 1.000000000000000888 ) ;
#24820=ORIENTED_EDGE ( 'NONE', *, *, #44744, .F. ) ;
#24821=CARTESIAN_POINT ( 'NONE',  ( 111.7322531227442681, -44.01858407219413039, 215.8357094172109782 ) ) ;
#24822=CARTESIAN_POINT ( 'NONE',  ( 96.00011186464382718, -37.20993085831212710, 116.3489586092439652 ) ) ;
#24823=CARTESIAN_POINT ( 'NONE',  ( 96.68076663292303863, -33.01451620012163346, 26.06514908543494613 ) ) ;
#24824=DIRECTION ( 'NONE',  ( 1.000000000000000000, 1.387778780781444413E-14, 0.000000000000000000 ) ) ;
#24825=DIRECTION ( 'NONE',  ( -0.4214249218767883165, -0.9068632946707806397, -4.214249218767892389E-16 ) ) ;
#24827=CARTESIAN_POINT ( 'NONE',  ( 102.0510343613854189, -46.57928231165939081, 168.2137205140059564 ) ) ;
#24829=ORIENTED_EDGE ( 'NONE', *, *, #38708, .T. ) ;
#24831=EDGE_LOOP ( 'NONE', ( #29147, #16366, #43525, #56182 ) ) ;
#24832=ORIENTED_EDGE ( 'NONE', *, *, #35769, .T. ) ;
#24833=DIRECTION ( 'NONE',  ( 0.000000000000000000, 0.000000000000000000, 1.000000000000000000 ) ) ;
#24837=EDGE_CURVE ( 'NONE', #55506, #45213, #38595, .T. ) ;
#24838=CARTESIAN_POINT ( 'NONE',  ( 120.3338511921238876, -37.86730215311064995, 299.5571190294419921 ) ) ;
#24839=ORIENTED_EDGE ( 'NONE', *, *, #71341, .F. ) ;
#24841=CARTESIAN_POINT ( 'NONE',  ( 96.65640405957751113, -37.29272404675901242, 76.36991099019697060 ) ) ;
#24843=DIRECTION ( 'NONE',  ( 0.000000000000000000, 1.000000000000000000, 0.000000000000000000 ) ) ;
#24844=DIRECTION ( 'NONE',  ( 0.000000000000000000, 0.000000000000000000, -1.000000000000000000 ) ) ;
#24845=CARTESIAN_POINT ( 'NONE',  ( 96.75683229781650141, -37.84742820979680289, 81.40038718067398804 ) ) ;
#24846=CARTESIAN_POINT ( 'NONE',  ( 154.4409905298078058, -0.9147987323338667709, 540.9756252759101471 ) ) ;
#24847=CARTESIAN_POINT ( 'NONE',  ( 102.0615167388205293, -46.55869598106821883, 168.2137205140059564 ) ) ;
#24849=DIRECTION ( 'NONE',  ( 0.000000000000000000, 0.000000000000000000, -1.000000000000000000 ) ) ;
#24850=EDGE_LOOP ( 'NONE', ( #72084, #7236, #86933, #56789 ) ) ;
#24851=VECTOR ( 'NONE', #78163, 1000.000000000000000 ) ;
#24852=DIRECTION ( 'NONE',  ( 1.000000000000000078E-15, 1.000000000000000083E-30, -1.000000000000000000 ) ) ;
#24853=CARTESIAN_POINT ( 'NONE',  ( 71.23990787207000608, 10.64204399490126463, 542.9756252759101471 ) ) ;
#24856=DIRECTION ( 'NONE',  ( 0.000000000000000000, 0.000000000000000000, 1.000000000000000000 ) ) ;
#24857=CARTESIAN_POINT ( 'NONE',  ( 96.09181007874647662, -35.06528625842698688, 221.1946728949589840 ) ) ;
#24858=ORIENTED_EDGE ( 'NONE', *, *, #16145, .T. ) ;
#24859=CARTESIAN_POINT ( 'NONE',  ( 100.9544530942022362, -28.70718995531744255, 145.5939800926359737 ) ) ;
#24860=CARTESIAN_POINT ( 'NONE',  ( 96.99552470177088992, -33.95220897389439330, 247.1127681330539758 ) ) ;
#24861=CARTESIAN_POINT ( 'NONE',  ( 99.02072372077822138, -43.42711337151016693, 112.8784824187679732 ) ) ;
#24863=CARTESIAN_POINT ( 'NONE',  ( 81.44716491654075696, -39.11090284777883852, 7.925007058955602091 ) ) ;
#24864=ADVANCED_FACE ( 'NONE', ( #24974 ), #45835, .T. ) ;
#24865=FACE_OUTER_BOUND ( 'NONE', #86060, .T. ) ;
#24867=ORIENTED_EDGE ( 'NONE', *, *, #27713, .F. ) ;
#24868=EDGE_CURVE ( 'NONE', #19039, #54183, #82042, .T. ) ;
#24870=EDGE_CURVE ( 'NONE', #79942, #51804, #22651, .T. ) ;
#24871=EDGE_LOOP ( 'NONE', ( #46399, #57555, #45225, #26750, #21084, #12425 ) ) ;
#24872=CIRCLE ( 'NONE', #10408, 0.5000000000000004441 ) ;
#24874=ORIENTED_EDGE ( 'NONE', *, *, #52438, .F. ) ;
#24875=CARTESIAN_POINT ( 'NONE',  ( 37.06648329127298780, 12.92155284005730387, 355.9756252759109998 ) ) ;
#24876=CARTESIAN_POINT ( 'NONE',  ( 97.81168895331678925, -40.51742574516946860, 7.635625275910939536 ) ) ;
#24878=CARTESIAN_POINT ( 'NONE',  ( 133.3151098752258292, -34.05633243510672514, 1.690787911851882264 ) ) ;
#24880=DIRECTION ( 'NONE',  ( -4.299999999999999979E-14, 1.000000000000000000, -4.128053709984630540E-29 ) ) ;
#24881=CARTESIAN_POINT ( 'NONE',  ( 113.2461701916471810, -28.75918670901990382, 149.5525716684902022 ) ) ;
#24883=CARTESIAN_POINT ( 'NONE',  ( 115.8412394166662835, -32.57321297090945933, 213.6009912566489675 ) ) ;
#24885=ORIENTED_EDGE ( 'NONE', *, *, #68671, .T. ) ;
#24887=EDGE_CURVE ( 'NONE', #893, #59432, #7726, .T. ) ;
#24888=VECTOR ( 'NONE', #69406, 1000.000000000000000 ) ;
#24890=CARTESIAN_POINT ( 'NONE',  ( 110.8544820967422311, -45.98423322291753124, 182.8856261428530843 ) ) ;
#24891=CARTESIAN_POINT ( 'NONE',  ( 41.56648329127399677, -9.303447159940999356, 198.9256252759119832 ) ) ;
#24892=CARTESIAN_POINT ( 'NONE',  ( 107.1760646772892756, -27.86850643495606406, 31.49872616304000417 ) ) ;
#24895=DIRECTION ( 'NONE',  ( 0.7071067811575828532, -0.7071067812155121812, 0.000000000000000000 ) ) ;
#24898=EDGE_CURVE ( 'NONE', #623, #68369, #49031, .T. ) ;
#24901=CARTESIAN_POINT ( 'NONE',  ( 103.4307397011154279, -27.41362630817958035, 56.37257573100154673 ) ) ;
#24904=CARTESIAN_POINT ( 'NONE',  ( 100.5332814249895108, -41.62301430380158962, 64.65666179816298609 ) ) ;
#24905=VECTOR ( 'NONE', #57363, 1000.000000000000000 ) ;
#24906=CARTESIAN_POINT ( 'NONE',  ( 46.48091746482126041, -48.32844715994084339, 300.4678068554150059 ) ) ;
#24907=PLANE ( 'NONE',  #43256 ) ;
#24908=CONICAL_SURFACE ( 'NONE', #75691, 1.258750000000002922, 1.029744258676650093 ) ;
#24910=ORIENTED_EDGE ( 'NONE', *, *, #55049, .F. ) ;
#24911=FACE_OUTER_BOUND ( 'NONE', #75288, .T. ) ;
#24913=ORIENTED_EDGE ( 'NONE', *, *, #51497, .T. ) ;
#24914=CARTESIAN_POINT ( 'NONE',  ( 114.7715153371978687, -44.65482214316887877, 118.2022919425779719 ) ) ;
#24915=ORIENTED_EDGE ( 'NONE', *, *, #45725, .T. ) ;
#24916=CARTESIAN_POINT ( 'NONE',  ( 114.5755952152626946, -32.65889807719148052, 68.64384839950594142 ) ) ;
#24918=CARTESIAN_POINT ( 'NONE',  ( 114.7653520042265143, -30.23343873216411026, 70.81586902018300123 ) ) ;
#24919=CARTESIAN_POINT ( 'NONE',  ( 135.5598545223736551, -21.04079274303778391, 1.981704437708090127 ) ) ;
#24922=CARTESIAN_POINT ( 'NONE',  ( 71.06648329127399677, -18.82844715994099971, -5.074374724088000832 ) ) ;
#24923=CARTESIAN_POINT ( 'NONE',  ( 112.8297475082234484, -27.27058933724656953, 45.62895860924398761 ) ) ;
#24924=CARTESIAN_POINT ( 'NONE',  ( 36.23715912545338114, -47.82818131006131779, 193.9678068554150911 ) ) ;
#24929=VERTEX_POINT ( 'NONE', #28612 ) ;
#24930=ORIENTED_EDGE ( 'NONE', *, *, #88059, .F. ) ;
#24931=VECTOR ( 'NONE', #32007, 1000.000000000000000 ) ;
#24932=EDGE_LOOP ( 'NONE', ( #39770, #72412, #47932, #21587 ) ) ;
#24933=CARTESIAN_POINT ( 'NONE',  ( 110.4719531740380347, -47.31314961125950447, 207.8241967044829721 ) ) ;
#24934=CARTESIAN_POINT ( 'NONE',  ( 97.73888860506711751, -40.33520859504945832, 126.6195452632120038 ) ) ;
#24935=CARTESIAN_POINT ( 'NONE',  ( 113.1782937269942124, -44.75186862722408421, 189.0939586048054935 ) ) ;
#24936=CARTESIAN_POINT ( 'NONE',  ( 115.0226255289246922, -43.52070134976005988, 59.26419670448196086 ) ) ;
#24937=CARTESIAN_POINT ( 'NONE',  ( 117.0608842944984644, -38.08055299089861023, 44.71895066874647995 ) ) ;
#24939=CARTESIAN_POINT ( 'NONE',  ( 172.5664832912740110, -32.07844715994070839, 138.9256252759119832 ) ) ;
#24940=EDGE_CURVE ( 'NONE', #49158, #6301, #14640, .T. ) ;
#24943=EDGE_CURVE ( 'NONE', #14978, #50013, #71915, .T. ) ;
#24945=DIRECTION ( 'NONE',  ( -0.7071067811734105257, 0.7071067811996846197, 0.000000000000000000 ) ) ;
#24946=CARTESIAN_POINT ( 'NONE',  ( 115.7579298488887076, -31.01215564512770229, 254.2899109901966028 ) ) ;
#24948=CARTESIAN_POINT ( 'NONE',  ( 48.86082318535593316, -35.55794170701788204, 117.4678068554150485 ) ) ;
#24949=DIRECTION ( 'NONE',  ( -4.299999999999999979E-14, 1.000000000000000000, -4.400000000000000367E-29 ) ) ;
#24950=CARTESIAN_POINT ( 'NONE',  ( 98.83240126976802742, -34.45875894154226415, 250.5352769709339782 ) ) ;
#24952=CARTESIAN_POINT ( 'NONE',  ( 98.11562048848820439, -31.42749274529986536, 81.90133956162493689 ) ) ;
#24954=CARTESIAN_POINT ( 'NONE',  ( 112.1415033342358640, -47.49387789398046067, 137.9270538473389820 ) ) ;
#24956=CARTESIAN_POINT ( 'NONE',  ( 126.0667039024479266, -14.72944715994094977, 239.5838068554170377 ) ) ;
#24957=ORIENTED_EDGE ( 'NONE', *, *, #66928, .T. ) ;
#24958=DIRECTION ( 'NONE',  ( 4.299999999999999979E-14, -1.000000000000000000, 4.400000000000000367E-29 ) ) ;
#24961=CARTESIAN_POINT ( 'NONE',  ( 135.0140782791278582, -34.14703303315379657, 1.764000745016856886 ) ) ;
#24963=CARTESIAN_POINT ( 'NONE',  ( 37.56670390244749314, -48.82844715994126261, 129.9678068554150911 ) ) ;
#24964=CARTESIAN_POINT ( 'NONE',  ( 103.3467460430879612, -47.18776626161088927, 102.3165776568629752 ) ) ;
#24965=VERTEX_POINT ( 'NONE', #23497 ) ;
#24966=DIRECTION ( 'NONE',  ( 1.000000000000000078E-15, 0.000000000000000000, -1.000000000000000000 ) ) ;
#24968=AXIS2_PLACEMENT_3D ( 'NONE', #28095, #83528, #76257 ) ;
#24972=CARTESIAN_POINT ( 'NONE',  ( 104.9583746955643448, -25.04227923723010463, 125.2184824187689856 ) ) ;
#24974=FACE_OUTER_BOUND ( 'NONE', #13053, .T. ) ;
#24975=DIRECTION ( 'NONE',  ( 0.7071067811575898476, -0.7071067812155052978, 0.000000000000000000 ) ) ;
#24979=EDGE_CURVE ( 'NONE', #30195, #47060, #3034, .T. ) ;
#24983=EDGE_CURVE ( 'NONE', #81368, #22460, #17114, .T. ) ;
#24984=AXIS2_PLACEMENT_3D ( 'NONE', #27411, #15598, #7872 ) ;
#24985=LINE ( 'NONE', #18611, #63196 ) ;
#24986=ADVANCED_FACE ( 'NONE', ( #3919, #40670, #53376, #73399 ), #81141, .T. ) ;
#24989=DIRECTION ( 'NONE',  ( 0.000000000000000000, 0.000000000000000000, -1.000000000000000000 ) ) ;
#24992=B_SPLINE_CURVE_WITH_KNOTS ( 'NONE', 3,
 ( #3891, #72497, #85695, #3005, #2571, #50697, #86576, #78438, #30271, #71170, #30707, #58403, #44772, #23470, #10696, #9376, #8945, #52012, #64786, #57959, #29828, #71613, #3449, #10264, #65231, #72050, #57059, #79772 ),
 .UNSPECIFIED., .F., .F.,
 ( 4, 2, 1, 1, 1, 1, 2, 2, 2, 2, 2, 2, 2, 2, 2, 4 ),
 ( 0.5000913810681943961, 0.5005795730788700215, 0.5010677650895456470, 0.5020441491108970089, 0.5039969171535993997, 0.5079024532390044033, 0.5157135254098140775, 0.5313356697514330929, 0.5625799584346710125, 0.6250685358011466297, 0.6875571131676221359, 0.7500456905340977531, 0.8125342679005732593, 0.8750228452670488766, 0.9375114226335243828, 1.000000000000000000 ),
 .UNSPECIFIED. ) ;
#24993=CARTESIAN_POINT ( 'NONE',  ( 112.0659117286329547, -45.48839619832590131, 33.98979195227510530 ) ) ;
#24994=CARTESIAN_POINT ( 'NONE',  ( 112.7271506738795779, -45.41826929060054852, 219.0480062282919960 ) ) ;
#24997=EDGE_LOOP ( 'NONE', ( #53412, #49010, #9813, #66366 ) ) ;
#24998=CIRCLE ( 'NONE', #65649, 3.250000000000002665 ) ;
#24999=CARTESIAN_POINT ( 'NONE',  ( 99.61812512063050917, -43.94476044465307751, 37.95086337114900488 ) ) ;
#25000=FACE_OUTER_BOUND ( 'NONE', #63211, .T. ) ;
#25002=DIRECTION ( 'NONE',  ( 1.000000000000000000, 0.000000000000000000, 0.000000000000000000 ) ) ;
#25003=ORIENTED_EDGE ( 'NONE', *, *, #6931, .F. ) ;
#25006=VERTEX_POINT ( 'NONE', #88841 ) ;
#25007=CARTESIAN_POINT ( 'NONE',  ( 108.9963713912396912, -28.08052754339530921, 221.3330118773259585 ) ) ;
#25008=VECTOR ( 'NONE', #87040, 1000.000000000000000 ) ;
#25012=CARTESIAN_POINT ( 'NONE',  ( 81.20961857873525958, -39.23068377182526234, 1.829869271362388750 ) ) ;
#25013=ORIENTED_EDGE ( 'NONE', *, *, #53114, .T. ) ;
#25014=DIRECTION ( 'NONE',  ( 0.000000000000000000, 0.000000000000000000, 1.000000000000000000 ) ) ;
#25015=CARTESIAN_POINT ( 'NONE',  ( 182.2420472961719895, -31.76306994223730840, 117.4678068554150627 ) ) ;
#25016=ORIENTED_EDGE ( 'NONE', *, *, #60959, .F. ) ;
#25017=CARTESIAN_POINT ( 'NONE',  ( 116.1584957626482435, -43.02035883463254606, 13.35657765686298859 ) ) ;
#25019=ORIENTED_EDGE ( 'NONE', *, *, #46905, .T. ) ;
#25020=CARTESIAN_POINT ( 'NONE',  ( 114.1044565855118265, -40.86425766668616433, 236.2223760838769806 ) ) ;
#25023=DIRECTION ( 'NONE',  ( -1.000000000000000000, -4.299999999999999979E-14, -1.000000000000000078E-15 ) ) ;
#25025=ADVANCED_FACE ( 'NONE', ( #17986 ), #80681, .F. ) ;
#25026=CARTESIAN_POINT ( 'NONE',  ( 97.72358123494467463, -41.53030082902068898, 192.7041967044819728 ) ) ;
#25028=ORIENTED_EDGE ( 'NONE', *, *, #70409, .T. ) ;
#25029=VECTOR ( 'NONE', #66492, 1000.000000000000000 ) ;
#25030=CARTESIAN_POINT ( 'NONE',  ( 100.2704505754038706, -46.49802187830721323, 83.09276813305294240 ) ) ;
#25031=DIRECTION ( 'NONE',  ( 0.000000000000000000, 0.000000000000000000, 1.000000000000000000 ) ) ;
#25034=EDGE_LOOP ( 'NONE', ( #26075, #72504 ) ) ;
#25036=VECTOR ( 'NONE', #34674, 1000.000000000000000 ) ;
#25037=CARTESIAN_POINT ( 'NONE',  ( 81.33214528238656271, -16.28157797492746184, 1.873071231918668200 ) ) ;
#25038=CYLINDRICAL_SURFACE ( 'NONE', #44220, 0.5000000000000007772 ) ;
#25039=CARTESIAN_POINT ( 'NONE',  ( 107.0664832912739968, -36.72944715994100306, 287.6356252759109680 ) ) ;
#25040=CARTESIAN_POINT ( 'NONE',  ( 98.94907028073869526, -37.58812756235333552, 124.2280903695919818 ) ) ;
#25041=CARTESIAN_POINT ( 'NONE',  ( 118.0739042565516712, -35.49579832924209910, 229.9032443235299468 ) ) ;
#25042=CARTESIAN_POINT ( 'NONE',  ( 194.5664832912729878, -81.37844715994266664, 361.9756252759109998 ) ) ;
#25043=VERTEX_POINT ( 'NONE', #11172 ) ;
#25044=CARTESIAN_POINT ( 'NONE',  ( 135.1908702341735591, -39.23918067504811091, 1.822998012175016003 ) ) ;
#25045=VERTEX_POINT ( 'NONE', #32063 ) ;
#25046=VERTEX_POINT ( 'NONE', #74309 ) ;
#25049=ORIENTED_EDGE ( 'NONE', *, *, #21739, .T. ) ;
#25050=ORIENTED_EDGE ( 'NONE', *, *, #51778, .F. ) ;
#25051=FACE_OUTER_BOUND ( 'NONE', #31974, .T. ) ;
#25052=CARTESIAN_POINT ( 'NONE',  ( 19.56670390244734747, -25.42844715994192129, 300.4678068554150059 ) ) ;
#25053=CARTESIAN_POINT ( 'NONE',  ( 97.07201598029109846, -35.37898882807422751, 26.21900220677386528 ) ) ;
#25054=CARTESIAN_POINT ( 'NONE',  ( 116.7762654731291860, -36.89220852042034693, 153.2352769709339668 ) ) ;
#25055=CARTESIAN_POINT ( 'NONE',  ( 104.2289649446409783, -46.80690502001216657, 22.35848241876792031 ) ) ;
#25056=VERTEX_POINT ( 'NONE', #66580 ) ;
#25057=AXIS2_PLACEMENT_3D ( 'NONE', #78423, #37066, #81548 ) ;
#25059=ORIENTED_EDGE ( 'NONE', *, *, #52790, .T. ) ;
#25060=ORIENTED_CLOSED_SHELL ( 'NONE', *, #47417, .F. );
#25061=DIRECTION ( 'NONE',  ( 0.000000000000000000, 1.000000000000000000, 0.000000000000000000 ) ) ;
#25062=ORIENTED_EDGE ( 'NONE', *, *, #56339, .T. ) ;
#25063=CARTESIAN_POINT ( 'NONE',  ( 97.04329235580377144, -37.22002798420894720, 167.3652492753220145 ) ) ;
#25064=CARTESIAN_POINT ( 'NONE',  ( 109.6418137192420517, -46.48038841143647915, 32.78157913610764496 ) ) ;
#25066=AXIS2_PLACEMENT_3D ( 'NONE', #60427, #88174, #53144 ) ;
#25067=FACE_BOUND ( 'NONE', #18428, .T. ) ;
#25069=CARTESIAN_POINT ( 'NONE',  ( 118.5953454549360231, -33.89261193510051839, 14.01848241876796308 ) ) ;
#25070=CARTESIAN_POINT ( 'NONE',  ( 111.3409431244321439, -27.17319409035083666, 20.74133956162494030 ) ) ;
#25073=DIRECTION ( 'NONE',  ( -0.7071067811865774377, 0.7071067811865175967, -7.071067811865782003E-16 ) ) ;
#25074=DIRECTION ( 'NONE',  ( 4.299999999999999979E-14, -1.000000000000000000, 0.000000000000000000 ) ) ;
#25076=EDGE_CURVE ( 'NONE', #829, #20800, #47472, .T. ) ;
#25077=CARTESIAN_POINT ( 'NONE',  ( 116.3212776292296127, -32.94146857471318413, 10.13562527591094309 ) ) ;
#25079=CARTESIAN_POINT ( 'NONE',  ( 103.5840655562901134, -46.60261447156455716, 57.30705384733997221 ) ) ;
#25080=CARTESIAN_POINT ( 'NONE',  ( 114.1247157756359769, -29.05716968555177004, 195.4841967044819739 ) ) ;
#25081=CARTESIAN_POINT ( 'NONE',  ( 96.69309474412473548, -37.96640669985919914, 37.42133956162496844 ) ) ;
#25082=ADVANCED_FACE ( 'NONE', ( #75201 ), #39766, .T. ) ;
#25084=LINE ( 'NONE', #37835, #47203 ) ;
#25085=CARTESIAN_POINT ( 'NONE',  ( 81.08070086926755948, -34.17316201338597637, 1.785258157648824895 ) ) ;
#25089=DIRECTION ( 'NONE',  ( -4.237773401492740281E-14, 1.000000000000000000, 0.000000000000000000 ) ) ;
#25090=ORIENTED_EDGE ( 'NONE', *, *, #16385, .T. ) ;
#25092=CARTESIAN_POINT ( 'NONE',  ( 104.3903674582245742, -25.93822912171390982, 86.26991099019598153 ) ) ;
#25095=ORIENTED_EDGE ( 'NONE', *, *, #27141, .F. ) ;
#25096=CYLINDRICAL_SURFACE ( 'NONE', #63035, 9.999999999999998224 ) ;
#25097=CARTESIAN_POINT ( 'NONE',  ( 101.4165038149807572, -45.50681337102567880, 218.1213395616249784 ) ) ;
#25098=CARTESIAN_POINT ( 'NONE',  ( 105.8694971003958614, -26.37070548771162493, 321.6188579224977389 ) ) ;
#25099=CYLINDRICAL_SURFACE ( 'NONE', #20273, 11.45913725231036118 ) ;
#25102=FACE_OUTER_BOUND ( 'NONE', #34864, .T. ) ;
#25103=CARTESIAN_POINT ( 'NONE',  ( 132.1570028294962924, -38.71057579844590180, 2.232988688758104967 ) ) ;
#25105=CARTESIAN_POINT ( 'NONE',  ( 98.56701561008806323, -30.78824967682747271, 160.8289586092449497 ) ) ;
#25106=ORIENTED_EDGE ( 'NONE', *, *, #27357, .F. ) ;
#25108=CARTESIAN_POINT ( 'NONE',  ( 104.5515342781392008, -45.22670024980423165, 103.7787261630399911 ) ) ;
#25109=DIRECTION ( 'NONE',  ( 4.237773401492740281E-14, -1.000000000000000000, 0.000000000000000000 ) ) ;
#25110=CARTESIAN_POINT ( 'NONE',  ( 97.40014589274353796, -35.23768424668793386, 262.2041967044816602 ) ) ;
#25113=CARTESIAN_POINT ( 'NONE',  ( 162.7866693523280048, -29.62846900982320264, 342.9256252759119548 ) ) ;
#25121=CARTESIAN_POINT ( 'NONE',  ( 96.76471471792625323, -35.27954033865438532, 181.2156252759109805 ) ) ;
#25125=CARTESIAN_POINT ( 'NONE',  ( 102.0670550280536446, -27.97049802139369135, 151.4897919364310894 ) ) ;
#25126=LINE ( 'NONE', #79675, #58082 ) ;
#25127=DIRECTION ( 'NONE',  ( -1.000000000000000000, -8.163404592831600092E-16, -1.020425574103949962E-15 ) ) ;
#25132=CARTESIAN_POINT ( 'NONE',  ( 113.7507820938996872, -44.72989589602062210, 193.1299109901969757 ) ) ;
#25133=FACE_OUTER_BOUND ( 'NONE', #38950, .T. ) ;
#25135=ORIENTED_EDGE ( 'NONE', *, *, #65535, .F. ) ;
#25137=CARTESIAN_POINT ( 'NONE',  ( 194.0371591254575492, -24.42818131005407167, 129.9678068554150343 ) ) ;
#25138=CARTESIAN_POINT ( 'NONE',  ( 107.0664832912739683, -18.82844715994099971, 199.5838068554169809 ) ) ;
#25139=CARTESIAN_POINT ( 'NONE',  ( 115.6923476351215641, -37.43328618085965331, 36.59189989340094940 ) ) ;
#25140=DIRECTION ( 'NONE',  ( 1.000000000000000078E-15, -1.000000000000000000, 0.000000000000000000 ) ) ;
#25142=CARTESIAN_POINT ( 'NONE',  ( 180.2121375201600131, -29.73316016639650172, 117.4678068554150627 ) ) ;
#25143=CARTESIAN_POINT ( 'NONE',  ( 82.19340217263071224, -16.98608769072388824, 7.448832051633130114 ) ) ;
#25144=ORIENTED_EDGE ( 'NONE', *, *, #77180, .T. ) ;
#25146=AXIS2_PLACEMENT_3D ( 'NONE', #75692, #13460, #7544 ) ;
#25148=CARTESIAN_POINT ( 'NONE',  ( 41.56648329127399677, 0.2215528400590013880, 316.8086252759120498 ) ) ;
#25149=VERTEX_POINT ( 'NONE', #25700 ) ;
#25150=ORIENTED_EDGE ( 'NONE', *, *, #6536, .T. ) ;
#25151=CARTESIAN_POINT ( 'NONE',  ( 100.9536334643962903, -28.70783906175504896, 156.5938426686704759 ) ) ;
#25152=CARTESIAN_POINT ( 'NONE',  ( 106.6171843113225606, -27.68451483556421522, 44.55051506617196821 ) ) ;
#25153=CARTESIAN_POINT ( 'NONE',  ( 97.38146765292194118, -40.64695096355149673, 206.6327681330539860 ) ) ;
#25154=CARTESIAN_POINT ( 'NONE',  ( 114.4473569665854313, -28.53271593493105485, 159.5051490854349652 ) ) ;
#25155=DIRECTION ( 'NONE',  ( 1.000000000000000078E-15, 1.000000000000000083E-30, -1.000000000000000000 ) ) ;
#25156=CARTESIAN_POINT ( 'NONE',  ( 99.39693184722126773, -28.77005263954443492, 261.6746728949588032 ) ) ;
#25157=DIRECTION ( 'NONE',  ( -0.04216478779797398074, 0.9991106698809455455, 0.000000000000000000 ) ) ;
#25158=DIRECTION ( 'NONE',  ( 0.7071067812123270624, 0.7071067811607679721, 0.000000000000000000 ) ) ;
#25159=EDGE_CURVE ( 'NONE', #14582, #67680, #74750, .T. ) ;
#25160=ORIENTED_EDGE ( 'NONE', *, *, #65974, .T. ) ;
#25161=EDGE_CURVE ( 'NONE', #69894, #26619, #60654, .T. ) ;
#25162=ORIENTED_EDGE ( 'NONE', *, *, #67160, .F. ) ;
#25163=DIRECTION ( 'NONE',  ( 1.000000000000000000, -5.337610695313248426E-16, 0.000000000000000000 ) ) ;
#25164=CARTESIAN_POINT ( 'NONE',  ( 115.8924960319658055, -44.71257290243538307, 233.2413395616259493 ) ) ;
#25165=ORIENTED_EDGE ( 'NONE', *, *, #39495, .T. ) ;
#25166=CARTESIAN_POINT ( 'NONE',  ( 100.0080109101350985, -27.21007462382121744, 185.5841967044829630 ) ) ;
#25168=CIRCLE ( 'NONE', #62907, 2.749999999999974687 ) ;
#25170=ADVANCED_FACE ( 'NONE', ( #32502 ), #4817, .T. ) ;
#25171=CARTESIAN_POINT ( 'NONE',  ( 162.5667039024470171, -33.35206098992711077, 342.9256252759109884 ) ) ;
#25172=DIRECTION ( 'NONE',  ( 0.000000000000000000, 0.000000000000000000, 1.000000000000000000 ) ) ;
#25173=CARTESIAN_POINT ( 'NONE',  ( 97.94068279941657806, -40.34109379996354505, 277.6356252759109111 ) ) ;
#25174=DIRECTION ( 'NONE',  ( 5.512527431108029424E-15, -1.000000000000000000, 0.000000000000000000 ) ) ;
#25175=CARTESIAN_POINT ( 'NONE',  ( 109.2074818670226222, -48.35976665079980563, 273.7213395616252569 ) ) ;
#25176=FACE_OUTER_BOUND ( 'NONE', #64574, .T. ) ;
#25177=DIRECTION ( 'NONE',  ( 1.000000000000000000, 0.000000000000000000, 9.462128050782575008E-16 ) ) ;
#25178=LINE ( 'NONE', #52840, #28119 ) ;
#25179=AXIS2_PLACEMENT_3D ( 'NONE', #43260, #84633, #7412 ) ;
#25180=DIRECTION ( 'NONE',  ( -8.252657816380299978E-16, -2.773339119917620066E-31, -1.000000000000000000 ) ) ;
#25181=DIRECTION ( 'NONE',  ( -3.201858731750027727E-15, 1.000000000000000000, -3.201858731750027724E-30 ) ) ;
#25183=CARTESIAN_POINT ( 'NONE',  ( 134.0664832912740110, -8.350947159940998787, 293.6356252759119911 ) ) ;
#25185=VERTEX_POINT ( 'NONE', #40116 ) ;
#25186=CARTESIAN_POINT ( 'NONE',  ( 136.5307003794597449, -19.95069274173234675, 7.120636252907847741 ) ) ;
#25187=CARTESIAN_POINT ( 'NONE',  ( 104.1796880194223576, -26.65200820554803585, 225.2984824187679749 ) ) ;
#25188=CARTESIAN_POINT ( 'NONE',  ( 98.85791787721181834, -43.21333385077131339, 87.85848241876792031 ) ) ;
#25189=CARTESIAN_POINT ( 'NONE',  ( 106.8507155540331013, -47.82678659975260160, 223.5489586092439538 ) ) ;
#25190=DIRECTION ( 'NONE',  ( -1.000000000000000078E-15, 1.000000000000000083E-30, 1.000000000000000000 ) ) ;
#25191=DIRECTION ( 'NONE',  ( 0.000000000000000000, 0.000000000000000000, 1.000000000000000000 ) ) ;
#25192=LINE ( 'NONE', #23443, #27561 ) ;
#25193=CARTESIAN_POINT ( 'NONE',  ( 116.3376065436754203, -32.98135602958129908, 40.13195101788765840 ) ) ;
#25194=CARTESIAN_POINT ( 'NONE',  ( 131.0667039024480118, -58.35344715994099829, 228.3338068554150198 ) ) ;
#25196=CARTESIAN_POINT ( 'NONE',  ( 131.5325842222575545, -19.79809288067805539, 2.811527366592877275 ) ) ;
#25198=ORIENTED_EDGE ( 'NONE', *, *, #12792, .F. ) ;
#25199=CARTESIAN_POINT ( 'NONE',  ( 107.8370078009992028, -28.22187835749811313, 154.4267055423619581 ) ) ;
#25200=EDGE_CURVE ( 'NONE', #27479, #78184, #85026, .T. ) ;
#25203=CARTESIAN_POINT ( 'NONE',  ( 97.33783051261163166, -34.07110767403877816, 91.11349398838056857 ) ) ;
#25204=CARTESIAN_POINT ( 'NONE',  ( 117.1049515565468226, -33.87427183379793405, 145.0470538473399529 ) ) ;
#25206=EDGE_CURVE ( 'NONE', #69283, #74946, #25564, .T. ) ;
#25207=EDGE_CURVE ( 'NONE', #73831, #86897, #26972, .T. ) ;
#25208=DIRECTION ( 'NONE',  ( -0.7071067811868619879, -0.7071067811862330466, -7.071067811868613027E-16 ) ) ;
#25210=LINE ( 'NONE', #81553, #48319 ) ;
#25211=ADVANCED_FACE ( 'NONE', ( #39231 ), #86506, .T. ) ;
#25212=CARTESIAN_POINT ( 'NONE',  ( 115.6651410650259066, -32.06827565682259262, 69.22133956162596746 ) ) ;
#25213=ORIENTED_EDGE ( 'NONE', *, *, #76468, .F. ) ;
#25217=LINE ( 'NONE', #17523, #15280 ) ;
#25218=CARTESIAN_POINT ( 'NONE',  ( 98.56701561008813428, -30.78824967682752245, 156.8289586092439549 ) ) ;
#25219=CARTESIAN_POINT ( 'NONE',  ( 97.81480632908598238, -40.51613010894325839, 171.6358981596145270 ) ) ;
#25220=AXIS2_PLACEMENT_3D ( 'NONE', #49617, #34208, #6960 ) ;
#25221=CARTESIAN_POINT ( 'NONE',  ( 53.35959712126198440, -48.62134037875358672, 129.9678068554150911 ) ) ;
#25222=DIRECTION ( 'NONE',  ( 0.000000000000000000, 1.000000000000000000, 0.000000000000000000 ) ) ;
#25225=DIRECTION ( 'NONE',  ( 0.000000000000000000, 0.000000000000000000, -1.000000000000000000 ) ) ;
#25226=CARTESIAN_POINT ( 'NONE',  ( 101.7220374796296909, -27.76276858577399409, 85.50419670448295051 ) ) ;
#25227=ORIENTED_EDGE ( 'NONE', *, *, #73583, .T. ) ;
#25228=ORIENTED_EDGE ( 'NONE', *, *, #11710, .F. ) ;
#25231=CARTESIAN_POINT ( 'NONE',  ( 95.60734603896359829, -36.72944715994100306, 309.2406250056037038 ) ) ;
#25232=CARTESIAN_POINT ( 'NONE',  ( 98.88612577743202792, -36.32393613343754879, 169.1052332267339580 ) ) ;
#25234=CIRCLE ( 'NONE', #62981, 0.5000000000000004441 ) ;
#25235=ADVANCED_FACE ( 'NONE', ( #18335 ), #74211, .T. ) ;
#25236=CARTESIAN_POINT ( 'NONE',  ( 119.5435152932140426, -31.57448135767196362, 289.6356252759106837 ) ) ;
#25237=ORIENTED_EDGE ( 'NONE', *, *, #38423, .F. ) ;
#25239=DIRECTION ( 'NONE',  ( 0.7071067811864671926, 0.7071067811866279529, 6.612322855854137577E-17 ) ) ;
#25240=AXIS2_PLACEMENT_3D ( 'NONE', #23426, #10650, #64737 ) ;
#25241=ORIENTED_EDGE ( 'NONE', *, *, #72157, .F. ) ;
#25244=CARTESIAN_POINT ( 'NONE',  ( 100.2828564484647274, -30.98100942051235052, 212.1987261630399360 ) ) ;
#25245=DIRECTION ( 'NONE',  ( 4.194175870806139918E-14, -1.000000000000000000, 0.000000000000000000 ) ) ;
#25251=ORIENTED_EDGE ( 'NONE', *, *, #4944, .T. ) ;
#25254=CARTESIAN_POINT ( 'NONE',  ( 104.5243549119882829, -45.65320838865366682, 215.1738046553059860 ) ) ;
#25256=CARTESIAN_POINT ( 'NONE',  ( 117.3932167392688655, -32.72270067050601483, 94.10895860924395606 ) ) ;
#25257=CARTESIAN_POINT ( 'NONE',  ( 104.0490797691969647, -47.33883444496888160, 67.36800622829191809 ) ) ;
#25258=CARTESIAN_POINT ( 'NONE',  ( 116.8184952045819500, -34.15823809959283608, 254.0314695188159533 ) ) ;
#25259=CARTESIAN_POINT ( 'NONE',  ( 97.81168895331838087, -40.51742574516882200, 287.6356252759109680 ) ) ;
#25260=CARTESIAN_POINT ( 'NONE',  ( 134.0664832912740110, -46.42944715994100591, 4.925625275910997303 ) ) ;
#25261=CARTESIAN_POINT ( 'NONE',  ( 117.4572939498068820, -40.49840382496243052, 169.5375300378159693 ) ) ;
#25266=VERTEX_POINT ( 'NONE', #11534 ) ;
#25268=ORIENTED_EDGE ( 'NONE', *, *, #56884, .F. ) ;
#25269=LINE ( 'NONE', #18007, #11456 ) ;
#25271=ORIENTED_EDGE ( 'NONE', *, *, #8710, .T. ) ;
#25272=ADVANCED_FACE ( 'NONE', ( #3382 ), #12067, .F. ) ;
#25273=DIRECTION ( 'NONE',  ( 0.7071067811571474238, 0.7071067812159476107, 0.000000000000000000 ) ) ;
#25275=( BOUNDED_CURVE ( )  B_SPLINE_CURVE ( 3, ( #88785, #20186, #75141, #81975 ),
 .UNSPECIFIED., .F., .T. ) 
 B_SPLINE_CURVE_WITH_KNOTS ( ( 4, 4 ),
 ( 2.074222157386416767E-12, 1.570796326797197162 ),
 .UNSPECIFIED. ) 
 CURVE ( )  GEOMETRIC_REPRESENTATION_ITEM ( )  RATIONAL_B_SPLINE_CURVE ( ( 1.000000000000000000, 0.8047378541243116468, 0.8047378541243116468, 1.000000000000000000 ) ) 
 REPRESENTATION_ITEM ( '' )  );
#25277=CARTESIAN_POINT ( 'NONE',  ( 102.9709959788349636, -46.31662683568885086, 92.25562527591097250 ) ) ;
#25279=AXIS2_PLACEMENT_3D ( 'NONE', #70781, #70325, #8553 ) ;
#25282=DIRECTION ( 'NONE',  ( 1.000000000000000078E-15, -1.000000000000000083E-30, -1.000000000000000000 ) ) ;
#25283=CARTESIAN_POINT ( 'NONE',  ( 116.4859054502389881, -39.36344060769046393, 98.60991099019695127 ) ) ;
#25285=CARTESIAN_POINT ( 'NONE',  ( 102.9757002774702102, -26.48594595611790581, 171.3908633711489813 ) ) ;
#25287=DIRECTION ( 'NONE',  ( -0.0001211784769825758571, 0.7071067708032323651, 0.7071067811865486830 ) ) ;
#25288=ORIENTED_EDGE ( 'NONE', *, *, #82913, .T. ) ;
#25290=LINE ( 'NONE', #24853, #70357 ) ;
#25291=DIRECTION ( 'NONE',  ( 2.900000000000000265E-14, -2.000000000000000155E-15, 1.000000000000000000 ) ) ;
#25292=EDGE_CURVE ( 'NONE', #35473, #43151, #47816, .T. ) ;
#25294=CARTESIAN_POINT ( 'NONE',  ( 100.7967938542458199, -45.88935316334050185, 242.1108633711489517 ) ) ;
#25295=ORIENTED_EDGE ( 'NONE', *, *, #4689, .T. ) ;
#25296=CARTESIAN_POINT ( 'NONE',  ( 97.81168736999980240, -40.51740164104307240, 32.63591986563997693 ) ) ;
#25297=CARTESIAN_POINT ( 'NONE',  ( 118.2085198165198676, -40.76548936363617059, 19.54991099019698453 ) ) ;
#25298=CARTESIAN_POINT ( 'NONE',  ( 103.4533635841105479, -46.55483943026052174, 138.2956252759109645 ) ) ;
#25299=FACE_OUTER_BOUND ( 'NONE', #39730, .T. ) ;
#25300=CARTESIAN_POINT ( 'NONE',  ( 82.81058719979546368, -36.91414947189120710, 6.758631288822928518 ) ) ;
#25302=LINE ( 'NONE', #38051, #77016 ) ;
#25303=ORIENTED_EDGE ( 'NONE', *, *, #78800, .T. ) ;
#25304=AXIS2_PLACEMENT_3D ( 'NONE', #42101, #1239, #6696 ) ;
#25305=VECTOR ( 'NONE', #32333, 1000.000000000000000 ) ;
#25306=AXIS2_PLACEMENT_3D ( 'NONE', #16151, #85206, #9326 ) ;
#25309=AXIS2_PLACEMENT_3D ( 'NONE', #85208, #29333, #76580 ) ;
#25310=CIRCLE ( 'NONE', #10977, 2.750000000000002665 ) ;
#25312=CARTESIAN_POINT ( 'NONE',  ( 138.8167039024479834, -50.82844715994100682, 58.80080685541479824 ) ) ;
#25313=CARTESIAN_POINT ( 'NONE',  ( 115.5933672690473912, -28.53551910654245205, 35.43562527591098643 ) ) ;
#25314=CARTESIAN_POINT ( 'NONE',  ( 61.56670390244730839, -23.42844715994043980, 249.9678068554150343 ) ) ;
#25319=ADVANCED_FACE ( 'NONE', ( #81933, #20144 ), #75098, .T. ) ;
#25320=CARTESIAN_POINT ( 'NONE',  ( 98.21912858861395534, -34.79631884261151242, 255.5657531614102709 ) ) ;
#25321=EDGE_LOOP ( 'NONE', ( #61169, #74273, #36051, #34605 ) ) ;
#25322=ORIENTED_EDGE ( 'NONE', *, *, #7188, .T. ) ;
#25323=VERTEX_POINT ( 'NONE', #88743 ) ;
#25324=DIRECTION ( 'NONE',  ( -0.000000000000000000, 1.000000000000000000, 0.000000000000000000 ) ) ;
#25325=CARTESIAN_POINT ( 'NONE',  ( 116.7485963143377461, -34.15446243945111604, 184.0333798272055503 ) ) ;
#25326=DIRECTION ( 'NONE',  ( 0.000000000000000000, 0.000000000000000000, -1.000000000000000000 ) ) ;
#25327=CARTESIAN_POINT ( 'NONE',  ( 114.9896934147946013, -32.69399539773264252, 40.63301187732598407 ) ) ;
#25329=DIRECTION ( 'NONE',  ( 1.000000000000000078E-15, -1.000000000000000083E-30, -1.000000000000000000 ) ) ;
#25330=CARTESIAN_POINT ( 'NONE',  ( 96.81359797424451585, -35.17473563989037899, 221.1946728949589840 ) ) ;
#25332=ORIENTED_EDGE ( 'NONE', *, *, #8194, .T. ) ;
#25335=CARTESIAN_POINT ( 'NONE',  ( 106.2223766104409037, -28.61050573088338922, 47.97666179816295795 ) ) ;
#25337=CARTESIAN_POINT ( 'NONE',  ( 135.2364670978548986, -16.23881677343959495, 8.012604157991546572 ) ) ;
#25338=AXIS2_PLACEMENT_3D ( 'NONE', #8668, #36366, #37258 ) ;
#25340=CARTESIAN_POINT ( 'NONE',  ( 98.30752845723139899, -41.72886325947258968, 192.7396747606553049 ) ) ;
#25341=ORIENTED_EDGE ( 'NONE', *, *, #4248, .T. ) ;
#25342=DIRECTION ( 'NONE',  ( -0.000000000000000000, -0.000000000000000000, 1.000000000000000000 ) ) ;
#25344=ORIENTED_EDGE ( 'NONE', *, *, #81789, .T. ) ;
#25345=CARTESIAN_POINT ( 'NONE',  ( 117.8566403422286299, -39.12769616061267186, 103.6403871806729455 ) ) ;
#25346=ORIENTED_EDGE ( 'NONE', *, *, #55189, .T. ) ;
#25347=CARTESIAN_POINT ( 'NONE',  ( 115.4237413257435918, -38.49363815508749553, 63.08384839950497991 ) ) ;
#25348=CARTESIAN_POINT ( 'NONE',  ( 172.5664832912740110, -32.07844715994070839, 323.6756252759119548 ) ) ;
#25349=CARTESIAN_POINT ( 'NONE',  ( 98.25403324269851169, -37.66165033158306130, 122.8415833058969469 ) ) ;
#25350=CARTESIAN_POINT ( 'NONE',  ( 165.6738106836199904, -26.00627455219321860, 342.9256252759119548 ) ) ;
#25351=FACE_OUTER_BOUND ( 'NONE', #80122, .T. ) ;
#25352=ADVANCED_FACE ( 'NONE', ( #21485, #75992 ), #28275, .F. ) ;
#25353=CARTESIAN_POINT ( 'NONE',  ( 99.11086226171772751, -44.43615201859483932, 37.95086337114900488 ) ) ;
#25355=ORIENTED_EDGE ( 'NONE', *, *, #51396, .T. ) ;
#25356=CARTESIAN_POINT ( 'NONE',  ( 98.30762054419153628, -41.72908882781142381, 256.7397536183686384 ) ) ;
#25357=CIRCLE ( 'NONE', #36980, 6.571100913904396101 ) ;
#25358=VERTEX_POINT ( 'NONE', #27389 ) ;
#25361=AXIS2_PLACEMENT_3D ( 'NONE', #55250, #48428, #27123 ) ;
#25362=ORIENTED_EDGE ( 'NONE', *, *, #27128, .T. ) ;
#25363=ORIENTED_EDGE ( 'NONE', *, *, #26660, .F. ) ;
#25364=EDGE_CURVE ( 'NONE', #25889, #47935, #16420, .T. ) ;
#25366=AXIS2_PLACEMENT_3D ( 'NONE', #70555, #84644, #36485 ) ;
#25371=CARTESIAN_POINT ( 'NONE',  ( 115.4101910119110386, -30.57141770992054219, 259.3203871806734355 ) ) ;
#25372=CARTESIAN_POINT ( 'NONE',  ( 51.56670390244699576, -22.48495420874030515, -5.074374724088000832 ) ) ;
#25374=CARTESIAN_POINT ( 'NONE',  ( 103.5987781142019202, -46.56090220241721767, 53.30705384733997221 ) ) ;
#25375=CARTESIAN_POINT ( 'NONE',  ( 101.9932059899096402, -45.44583378561615916, 43.15642108796611609 ) ) ;
#25377=CARTESIAN_POINT ( 'NONE',  ( 108.4174567856275075, -26.73502315347771230, 114.9708767927032227 ) ) ;
#25379=CYLINDRICAL_SURFACE ( 'NONE', #83964, 10.00000000000000355 ) ;
#25380=VECTOR ( 'NONE', #54115, 1000.000000000000000 ) ;
#25381=ORIENTED_EDGE ( 'NONE', *, *, #20989, .F. ) ;
#25382=EDGE_CURVE ( 'NONE', #69025, #837, #61392, .T. ) ;
#25384=FACE_OUTER_BOUND ( 'NONE', #74312, .T. ) ;
#25385=CARTESIAN_POINT ( 'NONE',  ( 106.5683798796750779, -47.15615894637593897, 247.5384824187679556 ) ) ;
#25386=PLANE ( 'NONE',  #14167 ) ;
#25387=AXIS2_PLACEMENT_3D ( 'NONE', #73771, #39250, #45587 ) ;
#25388=DIRECTION ( 'NONE',  ( -1.000000000000000000, -4.238735976179846264E-15, 0.000000000000000000 ) ) ;
#25389=CARTESIAN_POINT ( 'NONE',  ( 77.61460381940304387, -37.97617057399400409, 2.716753174564080275 ) ) ;
#25391=CARTESIAN_POINT ( 'NONE',  ( 99.00226700525801959, -39.63126001020209799, 266.0238483995056527 ) ) ;
#25392=CARTESIAN_POINT ( 'NONE',  ( 163.1639762274590169, -34.03355364505800651, -5.074374724088000832 ) ) ;
#25393=CARTESIAN_POINT ( 'NONE',  ( 112.5028774994481466, -27.85959465031284310, 90.63848241876793566 ) ) ;
#25395=CARTESIAN_POINT ( 'NONE',  ( 111.8142338872566626, -25.81671781287135303, 134.7499109901969518 ) ) ;
#25398=ORIENTED_EDGE ( 'NONE', *, *, #27135, .F. ) ;
#25399=DIRECTION ( 'NONE',  ( 0.000000000000000000, 0.000000000000000000, -1.000000000000000000 ) ) ;
#25400=CARTESIAN_POINT ( 'NONE',  ( 112.1393456299127251, -28.01282277393797315, 65.65645861032975006 ) ) ;
#25402=VERTEX_POINT ( 'NONE', #82380 ) ;
#25403=ADVANCED_FACE ( 'NONE', ( #62356 ), #61451, .T. ) ;
#25404=CARTESIAN_POINT ( 'NONE',  ( 97.80798526467157217, -40.50836769862076636, 51.63484613625869457 ) ) ;
#25405=CARTESIAN_POINT ( 'NONE',  ( 106.0722674988897296, -48.58863484196640314, 112.5099109901969712 ) ) ;
#25407=CARTESIAN_POINT ( 'NONE',  ( 83.56670390244801183, -39.24694715994107952, 229.5838068554169524 ) ) ;
#25408=DIRECTION ( 'NONE',  ( 1.000000000000000078E-15, -1.000000000000000083E-30, -1.000000000000000000 ) ) ;
#25409=CYLINDRICAL_SURFACE ( 'NONE', #34356, 1.000000000000000888 ) ;
#25410=AXIS2_PLACEMENT_3D ( 'NONE', #68634, #82729, #22733 ) ;
#25411=FACE_OUTER_BOUND ( 'NONE', #72274, .T. ) ;
#25412=EDGE_LOOP ( 'NONE', ( #18005, #2934, #5564, #65611 ) ) ;
#25413=CARTESIAN_POINT ( 'NONE',  ( 117.6033054121008945, -33.31318886634804954, 134.0880062282919880 ) ) ;
#25415=AXIS2_PLACEMENT_3D ( 'NONE', #66061, #10222, #65627 ) ;
#25416=PLANE ( 'NONE',  #21077 ) ;
#25417=DIRECTION ( 'NONE',  ( -1.000000000000000000, -4.299999999999999979E-14, -1.000000000000000078E-15 ) ) ;
#25418=EDGE_LOOP ( 'NONE', ( #21129, #2653, #65861, #215 ) ) ;
#25419=ORIENTED_EDGE ( 'NONE', *, *, #81440, .F. ) ;
#25423=CARTESIAN_POINT ( 'NONE',  ( 116.3279290549545806, -32.94269076977911226, 60.13562527591098927 ) ) ;
#25424=CARTESIAN_POINT ( 'NONE',  ( 52.65249034007825912, -48.32844715994060181, 300.4678068554150059 ) ) ;
#25427=CARTESIAN_POINT ( 'NONE',  ( 97.80797205823303386, -40.50833534217826326, 181.6348433549487424 ) ) ;
#25428=AXIS2_PLACEMENT_3D ( 'NONE', #13274, #68686, #41843 ) ;
#25432=CARTESIAN_POINT ( 'NONE',  ( 48.16670390244701139, -28.27351298637280408, -5.074374724088000832 ) ) ;
#25433=CARTESIAN_POINT ( 'NONE',  ( 112.6540662323891837, -44.79745133516134104, 199.0584824187679374 ) ) ;
#25434=CARTESIAN_POINT ( 'NONE',  ( 73.06648329127396835, -8.729447159941065237, 14.92562527591093691 ) ) ;
#25435=VERTEX_POINT ( 'NONE', #35092 ) ;
#25437=CARTESIAN_POINT ( 'NONE',  ( 96.86520444330115254, -38.59296402346411980, 47.48229194257691432 ) ) ;
#25438=CARTESIAN_POINT ( 'NONE',  ( 116.9157166719834606, -38.71740874140498789, 53.66822714426762531 ) ) ;
#25440=VECTOR ( 'NONE', #76717, 1000.000000000000000 ) ;
#25442=ORIENTED_EDGE ( 'NONE', *, *, #41288, .T. ) ;
#25445=VERTEX_POINT ( 'NONE', #41013 ) ;
#25446=VERTEX_POINT ( 'NONE', #68734 ) ;
#25447=AXIS2_PLACEMENT_3D ( 'NONE', #46303, #45853, #53560 ) ;
#25448=CARTESIAN_POINT ( 'NONE',  ( 101.6176986403717279, -43.71793944654686470, 228.4815833058969758 ) ) ;
#25450=CARTESIAN_POINT ( 'NONE',  ( 97.81847922488930180, -40.53401570104637841, 52.63663032143116993 ) ) ;
#25452=AXIS2_PLACEMENT_3D ( 'NONE', #65082, #15605, #86434 ) ;
#25453=CARTESIAN_POINT ( 'NONE',  ( 105.7154772353844265, -46.72385838015826920, 153.4689586016793612 ) ) ;
#25454=CARTESIAN_POINT ( 'NONE',  ( 82.46407580264985882, -38.08864647353023258, 2.654395117673051363 ) ) ;
#25455=EDGE_LOOP ( 'NONE', ( #16629, #13243, #19620, #39576 ) ) ;
#25456=DIRECTION ( 'NONE',  ( 0.7071067811865506814, -0.7071067811865443531, 7.071067811865500971E-16 ) ) ;
#25458=EDGE_LOOP ( 'NONE', ( #63808, #49487, #87362, #88859 ) ) ;
#25459=CARTESIAN_POINT ( 'NONE',  ( 118.2087526870871415, -40.76557371769158777, 23.54991099019593292 ) ) ;
#25461=VECTOR ( 'NONE', #46570, 1000.000000000000000 ) ;
#25462=ORIENTED_EDGE ( 'NONE', *, *, #78641, .F. ) ;
#25463=CARTESIAN_POINT ( 'NONE',  ( 105.9433607271350439, -44.81451498420922519, 255.2852332267341353 ) ) ;
#25467=DIRECTION ( 'NONE',  ( 9.351236661543306751E-17, -3.725950533538267725E-29, -1.000000000000000000 ) ) ;
#25469=CARTESIAN_POINT ( 'NONE',  ( 108.1864281049355867, -47.13803512191609713, 198.6613395616249989 ) ) ;
#25472=CARTESIAN_POINT ( 'NONE',  ( 101.6884573362309823, -27.70642928270265060, 81.50419670448295051 ) ) ;
#25473=ORIENTED_EDGE ( 'NONE', *, *, #42132, .F. ) ;
#25475=EDGE_CURVE ( 'NONE', #81368, #65933, #74440, .T. ) ;
#25476=ADVANCED_FACE ( 'NONE', ( #29634 ), #85524, .F. ) ;
#25477=ORIENTED_EDGE ( 'NONE', *, *, #75735, .F. ) ;
#25479=CARTESIAN_POINT ( 'NONE',  ( 99.09507348882181077, -30.55127953124965146, 160.8021594487345851 ) ) ;
#25480=CARTESIAN_POINT ( 'NONE',  ( 184.5667039024483245, -48.82844715993448403, 300.4678068554149490 ) ) ;
#25482=CARTESIAN_POINT ( 'NONE',  ( 112.6324121799619462, -43.35677846492738041, 145.9385665600669881 ) ) ;
#25483=CARTESIAN_POINT ( 'NONE',  ( 96.11533564597472434, -35.06885359281673686, 217.1946728949589840 ) ) ;
#25484=FACE_OUTER_BOUND ( 'NONE', #88293, .T. ) ;
#25485=VERTEX_POINT ( 'NONE', #77794 ) ;
#25487=EDGE_CURVE ( 'NONE', #84817, #80206, #23300, .T. ) ;
#25490=ORIENTED_EDGE ( 'NONE', *, *, #55670, .T. ) ;
#25491=AXIS2_PLACEMENT_3D ( 'NONE', #64114, #1884, #67221 ) ;
#25494=VECTOR ( 'NONE', #69139, 1000.000000000000000 ) ;
#25497=LINE ( 'NONE', #38233, #1894 ) ;
#25500=FACE_BOUND ( 'NONE', #26716, .T. ) ;
#25501=ADVANCED_FACE ( 'NONE', ( #43246, #15114 ), #42790, .F. ) ;
#25502=CARTESIAN_POINT ( 'NONE',  ( 108.5268020718178690, -45.14512305525489921, 167.1352769709339725 ) ) ;
#25503=CARTESIAN_POINT ( 'NONE',  ( 118.1298445534695531, -37.63217702543061449, 38.77372051400595865 ) ) ;
#25511=CYLINDRICAL_SURFACE ( 'NONE', #87939, 0.2499999999999941991 ) ;
#25512=CARTESIAN_POINT ( 'NONE',  ( 116.5661000126995361, -33.54017338482336186, 134.0841521534302387 ) ) ;
#25515=EDGE_LOOP ( 'NONE', ( #89009, #79425, #55986, #51990 ) ) ;
#25516=CARTESIAN_POINT ( 'NONE',  ( 116.7476796835742192, -31.34707987858772427, 29.24229194257799236 ) ) ;
#25517=CARTESIAN_POINT ( 'NONE',  ( 97.24759266268939939, -33.09869426670887549, 62.04419670448196911 ) ) ;
#25518=CIRCLE ( 'NONE', #24049, 3.000000000000002665 ) ;
#25521=CARTESIAN_POINT ( 'NONE',  ( 193.0374249753376432, -23.42844715993431848, 193.9678068554150343 ) ) ;
#25523=CARTESIAN_POINT ( 'NONE',  ( 50.96943157743499597, -34.03355364505720360, 237.4678068554150059 ) ) ;
#25524=CARTESIAN_POINT ( 'NONE',  ( 106.8487982878802427, -25.26971417141049869, 322.7516258301318999 ) ) ;
#25526=ORIENTED_EDGE ( 'NONE', *, *, #9133, .F. ) ;
#25527=CARTESIAN_POINT ( 'NONE',  ( 112.8421283165351809, -27.25026954951128388, 49.62895860924498947 ) ) ;
#25528=CARTESIAN_POINT ( 'NONE',  ( 117.1921950572609603, -41.16159581679399793, 204.4861014663869696 ) ) ;
#25529=CARTESIAN_POINT ( 'NONE',  ( 101.9498695335308014, -27.62134513440381411, 56.48419670448296159 ) ) ;
#25530=CARTESIAN_POINT ( 'NONE',  ( 98.15104113905631777, -41.26173906225317722, 171.7005789228540777 ) ) ;
#25531=CARTESIAN_POINT ( 'NONE',  ( 107.0664832912739968, -36.72944715994100306, -2.114374724089040924 ) ) ;
#25534=CARTESIAN_POINT ( 'NONE',  ( 97.81170999498195329, -40.51745678363457159, 187.6351607544849287 ) ) ;
#25536=CARTESIAN_POINT ( 'NONE',  ( 107.5699729851651938, -26.92841289699918050, 91.03562527591097364 ) ) ;
#25539=CARTESIAN_POINT ( 'NONE',  ( 97.49318720818088480, -40.89074837367928694, 227.6527681330539679 ) ) ;
#25540=DIRECTION ( 'NONE',  ( 0.000000000000000000, 0.000000000000000000, 1.000000000000000000 ) ) ;
#25541=CARTESIAN_POINT ( 'NONE',  ( 75.25757238336808541, -1.944390235229870978, 361.9756252759101471 ) ) ;
#25542=LINE ( 'NONE', #11478, #60230 ) ;
#25543=CARTESIAN_POINT ( 'NONE',  ( 102.0670549500623991, -27.97049806489031809, 46.48979194346625832 ) ) ;
#25544=CARTESIAN_POINT ( 'NONE',  ( 133.0522658619989613, -39.28573230649611503, 1.785258109343265565 ) ) ;
#25547=CARTESIAN_POINT ( 'NONE',  ( 101.2684584845351736, -45.32493232151070828, 152.0918157521019509 ) ) ;
#25548=ORIENTED_EDGE ( 'NONE', *, *, #83576, .F. ) ;
#25550=AXIS2_PLACEMENT_3D ( 'NONE', #14300, #84247, #34728 ) ;
#25551=CARTESIAN_POINT ( 'NONE',  ( 115.3364322588818851, -33.54570361940938739, 135.5501547344689754 ) ) ;
#25553=CARTESIAN_POINT ( 'NONE',  ( 36.23715912545339535, -47.82818131006131779, 180.4678068554150911 ) ) ;
#25555=CARTESIAN_POINT ( 'NONE',  ( 116.8464009251321301, -35.91275531464980730, 249.8927681330532664 ) ) ;
#25557=AXIS2_PLACEMENT_3D ( 'NONE', #5925, #46322, #81348 ) ;
#25558=CARTESIAN_POINT ( 'NONE',  ( 19.56648329127400032, 0.2215528400590083269, 323.8756252759109202 ) ) ;
#25561=CARTESIAN_POINT ( 'NONE',  ( 180.3164832912740110, 12.92155284005802507, 336.5756252759111362 ) ) ;
#25562=DIRECTION ( 'NONE',  ( 1.000000000000000000, 4.510281037539819615E-14, 0.000000000000000000 ) ) ;
#25564=B_SPLINE_CURVE_WITH_KNOTS ( 'NONE', 3,
 ( #53727, #46918, #52813, #10629, #66033, #18791, #31513, #25151, #72862, #3823, #87839, #80586, #79702, #24714, #58768, #17455, #59220, #86950 ),
 .UNSPECIFIED., .F., .F.,
 ( 4, 2, 2, 2, 2, 2, 2, 2, 4 ),
 ( 0.5000310696403432731, 0.5625271859353003778, 0.6250233022302574826, 0.6875194185252144763, 0.7500155348201715810, 0.8125116511151286858, 0.8750077674100857905, 0.9375038837050428953, 1.000000000000000000 ),
 .UNSPECIFIED. ) ;
#25566=CARTESIAN_POINT ( 'NONE',  ( 114.9485010938853975, -29.93956786141545834, 184.3927681330539770 ) ) ;
#25567=CARTESIAN_POINT ( 'NONE',  ( 99.09567284741018511, -30.55045004867509562, 170.8014589425313829 ) ) ;
#25568=ORIENTED_EDGE ( 'NONE', *, *, #22526, .F. ) ;
#25569=ORIENTED_EDGE ( 'NONE', *, *, #24099, .F. ) ;
#25571=CARTESIAN_POINT ( 'NONE',  ( 82.50377070432760718, -20.00325133682503420, 7.150416387935383256 ) ) ;
#25572=CARTESIAN_POINT ( 'NONE',  ( 97.06105352154311561, -37.99632076813814052, 186.4277894213790034 ) ) ;
#25573=CARTESIAN_POINT ( 'NONE',  ( 160.5667039024426401, -48.82844715994099971, 300.4678068554149490 ) ) ;
#25575=CARTESIAN_POINT ( 'NONE',  ( 105.7963341568336517, -26.72446301096675469, 95.17754999580937181 ) ) ;
#25576=VERTEX_POINT ( 'NONE', #21943 ) ;
#25578=CIRCLE ( 'NONE', #37199, 4.874999999999990230 ) ;
#25579=CARTESIAN_POINT ( 'NONE',  ( 100.6562259211013384, -44.95110337444964443, 232.0499109901969632 ) ) ;
#25581=EDGE_LOOP ( 'NONE', ( #42632, #19291 ) ) ;
#25583=EDGE_LOOP ( 'NONE', ( #22005, #81131, #64350, #3599 ) ) ;
#25584=EDGE_CURVE ( 'NONE', #36668, #85068, #51393, .T. ) ;
#25585=CARTESIAN_POINT ( 'NONE',  ( 103.5075036784956239, -46.12099098172097200, 63.28861473418663763 ) ) ;
#25586=DIRECTION ( 'NONE',  ( 1.000000000000000000, 0.000000000000000000, 0.000000000000000000 ) ) ;
#25588=CARTESIAN_POINT ( 'NONE',  ( 97.82528646310512954, -40.55050253551667083, 166.6384714708592867 ) ) ;
#25589=CARTESIAN_POINT ( 'NONE',  ( 99.26659991834783625, -39.13601125124746716, 19.38237608387593980 ) ) ;
#25590=CARTESIAN_POINT ( 'NONE',  ( 102.3833470591291785, -26.69184581432750747, 131.4118157521009778 ) ) ;
#25591=FACE_OUTER_BOUND ( 'NONE', #37673, .T. ) ;
#25593=EDGE_CURVE ( 'NONE', #44341, #72437, #43700, .T. ) ;
#25595=CARTESIAN_POINT ( 'NONE',  ( 80.43833865491315294, -15.97944715994106524, 8.225625275910944723 ) ) ;
#25596=EDGE_LOOP ( 'NONE', ( #66686, #73263, #31398, #55415 ) ) ;
#25599=ORIENTED_EDGE ( 'NONE', *, *, #24771, .T. ) ;
#25600=EDGE_LOOP ( 'NONE', ( #23490, #70330, #6515, #70436 ) ) ;
#25603=CARTESIAN_POINT ( 'NONE',  ( 111.7785660440950011, -28.99582275371927764, 49.05146744712496343 ) ) ;
#25604=CARTESIAN_POINT ( 'NONE',  ( 102.2269548454591046, -45.98824451103227062, 212.1927681330539599 ) ) ;
#25605=CARTESIAN_POINT ( 'NONE',  ( 116.6407469026009238, -40.79910830432095281, 168.5070538473399608 ) ) ;
#25607=CARTESIAN_POINT ( 'NONE',  ( 97.84500235132117041, -40.59787897505477616, 21.64223743672927469 ) ) ;
#25608=CARTESIAN_POINT ( 'NONE',  ( 104.7405551043178633, -47.51155644559842273, 28.41943479971997988 ) ) ;
#25611=ORIENTED_EDGE ( 'NONE', *, *, #54699, .T. ) ;
#25612=ORIENTED_EDGE ( 'NONE', *, *, #42431, .F. ) ;
#25616=VECTOR ( 'NONE', #34677, 1000.000000000000114 ) ;
#25617=CARTESIAN_POINT ( 'NONE',  ( 113.2461215947159161, -45.18040784396236376, 228.0784824187679760 ) ) ;
#25619=VECTOR ( 'NONE', #21341, 1000.000000000000000 ) ;
#25620=CARTESIAN_POINT ( 'NONE',  ( 101.3490469528152715, -46.18936307759902604, 202.1318157521019430 ) ) ;
#25621=CARTESIAN_POINT ( 'NONE',  ( 131.3164832912740110, -36.72944715994100306, -5.074374724089004474 ) ) ;
#25623=CARTESIAN_POINT ( 'NONE',  ( 141.0664832912740394, -46.72944715994099596, 14.92562527591100618 ) ) ;
#25624=DIRECTION ( 'NONE',  ( 0.000000000000000000, 1.000000000000000000, 0.000000000000000000 ) ) ;
#25625=CARTESIAN_POINT ( 'NONE',  ( 115.1362341769185917, -35.67412036042625800, 277.6356252759107974 ) ) ;
#25627=DIRECTION ( 'NONE',  ( 1.000000000000000078E-15, -1.000000000000000083E-30, -1.000000000000000000 ) ) ;
#25633=CARTESIAN_POINT ( 'NONE',  ( 101.1312616121724659, -28.98109996770097396, 195.5838068554168103 ) ) ;
#25635=CARTESIAN_POINT ( 'NONE',  ( 71.24102794365336422, 4.106145706013555774, 542.9756252759101471 ) ) ;
#25636=CARTESIAN_POINT ( 'NONE',  ( 110.1440020323170330, -26.08875547494869451, 214.8403871806729342 ) ) ;
#25637=CARTESIAN_POINT ( 'NONE',  ( 114.7074080197622976, -44.71632701241580321, 109.1718157521009687 ) ) ;
#25638=CARTESIAN_POINT ( 'NONE',  ( 115.2859307195537326, -30.18890446381676540, 240.3613395616249875 ) ) ;
#25639=CARTESIAN_POINT ( 'NONE',  ( 162.5667039024481255, -33.35206098992175328, 313.9678068554149490 ) ) ;
#25641=AXIS2_PLACEMENT_3D ( 'NONE', #1489, #22833, #44584 ) ;
#25642=PLANE ( 'NONE',  #66714 ) ;
#25645=DIRECTION ( 'NONE',  ( -0.9963424814100680926, 0.08544974978095698503, 0.000000000000000000 ) ) ;
#25646=CARTESIAN_POINT ( 'NONE',  ( 35.44148329127400388, 12.92155284005802685, 335.5992267699910485 ) ) ;
#25648=EDGE_CURVE ( 'NONE', #71480, #15206, #86160, .T. ) ;
#25651=CARTESIAN_POINT ( 'NONE',  ( 115.4001863486352022, -38.60401951598402803, 148.0724198280769883 ) ) ;
#25653=ORIENTED_EDGE ( 'NONE', *, *, #82058, .F. ) ;
#25654=CARTESIAN_POINT ( 'NONE',  ( 168.0371591254543091, -48.62818131005519717, 313.9678068554149490 ) ) ;
#25655=CARTESIAN_POINT ( 'NONE',  ( 117.1882713363356174, -39.28166824301211335, 119.6299109901969615 ) ) ;
#25658=CARTESIAN_POINT ( 'NONE',  ( 161.4809174648185888, -48.32844715993547169, 129.9678068554149775 ) ) ;
#25659=CARTESIAN_POINT ( 'NONE',  ( 116.7951252719045101, -39.38782978815772395, 109.6147919427310171 ) ) ;
#25660=CARTESIAN_POINT ( 'NONE',  ( 113.1080853710608238, -29.03773216254911915, 79.54705384733995288 ) ) ;
#25661=VERTEX_POINT ( 'NONE', #4613 ) ;
#25663=VECTOR ( 'NONE', #63973, 1000.000000000000000 ) ;
#25664=ORIENTED_EDGE ( 'NONE', *, *, #41255, .F. ) ;
#25665=EDGE_CURVE ( 'NONE', #55229, #37453, #87725, .T. ) ;
#25666=CARTESIAN_POINT ( 'NONE',  ( 25.56670390244797275, -62.87844715994099687, 293.2178068554150627 ) ) ;
#25667=CARTESIAN_POINT ( 'NONE',  ( 114.0056865186721922, -29.02320718445401226, 155.5051490854339704 ) ) ;
#25668=DIRECTION ( 'NONE',  ( 0.000000000000000000, 0.000000000000000000, -1.000000000000000000 ) ) ;
#25669=LINE ( 'NONE', #46090, #56653 ) ;
#25670=DIRECTION ( 'NONE',  ( 1.000000000000000000, 4.299999999999999979E-14, 1.000000000000000078E-15 ) ) ;
#25672=DIRECTION ( 'NONE',  ( 0.000000000000000000, 0.000000000000000000, -1.000000000000000000 ) ) ;
#25674=CARTESIAN_POINT ( 'NONE',  ( 117.3173117416417739, -32.65705981835808558, 99.13943479972098771 ) ) ;
#25675=VERTEX_POINT ( 'NONE', #53620 ) ;
#25677=EDGE_CURVE ( 'NONE', #27344, #47300, #59891, .T. ) ;
#25679=AXIS2_PLACEMENT_3D ( 'NONE', #80292, #45718, #18038 ) ;
#25680=CARTESIAN_POINT ( 'NONE',  ( 172.5664832912740110, -9.303447159940999356, 18.92562527591200094 ) ) ;
#25681=VECTOR ( 'NONE', #22677, 1000.000000000000000 ) ;
#25683=CARTESIAN_POINT ( 'NONE',  ( 97.86260780209082100, -37.94289672904660193, 149.2480903695909547 ) ) ;
#25684=CIRCLE ( 'NONE', #21352, 0.5000000000000004441 ) ;
#25687=CYLINDRICAL_SURFACE ( 'NONE', #35870, 0.9999999999992039701 ) ;
#25690=DIRECTION ( 'NONE',  ( -6.524622321627019585E-16, -3.741823817616790462E-31, -1.000000000000000000 ) ) ;
#25696=CARTESIAN_POINT ( 'NONE',  ( 99.68253537205306714, -30.91964177047806217, 197.2396785439919711 ) ) ;
#25697=PLANE ( 'NONE',  #63205 ) ;
#25698=VECTOR ( 'NONE', #37534, 1000.000000000000000 ) ;
#25700=CARTESIAN_POINT ( 'NONE',  ( 191.6377717143134873, -48.82844715994099971, 13.84673904354932006 ) ) ;
#25702=CARTESIAN_POINT ( 'NONE',  ( 116.3212776292296127, -32.94146857471318413, 287.6356252759109680 ) ) ;
#25705=CIRCLE ( 'NONE', #79426, 7.500000000000007105 ) ;
#25706=ORIENTED_EDGE ( 'NONE', *, *, #74207, .T. ) ;
#25707=EDGE_LOOP ( 'NONE', ( #84139, #50917, #70251, #49414, #9606, #5915 ) ) ;
#25708=ADVANCED_FACE ( 'NONE', ( #38671 ), #30972, .T. ) ;
#25709=CARTESIAN_POINT ( 'NONE',  ( 115.2284764178246661, -36.04786338006340429, 251.7109475124485414 ) ) ;
#25710=CARTESIAN_POINT ( 'NONE',  ( 97.24554646791794710, -31.60649478380229382, 90.93181575210196854 ) ) ;
#25711=CARTESIAN_POINT ( 'NONE',  ( 107.3204973292724276, -25.70223992296332582, 75.04610146638695767 ) ) ;
#25712=CARTESIAN_POINT ( 'NONE',  ( 100.2186905329472353, -40.88491400341852966, 249.5838068554171230 ) ) ;
#25713=EDGE_CURVE ( 'NONE', #21182, #12019, #64274, .T. ) ;
#25714=CARTESIAN_POINT ( 'NONE',  ( 184.5664832912740110, 25.62155284005901379, 328.6381252759109088 ) ) ;
#25716=CARTESIAN_POINT ( 'NONE',  ( 110.6962928707952756, -48.01036458606073865, 203.8241967044819489 ) ) ;
#25718=ORIENTED_EDGE ( 'NONE', *, *, #37362, .T. ) ;
#25720=ORIENTED_EDGE ( 'NONE', *, *, #30410, .F. ) ;
#25721=VERTEX_POINT ( 'NONE', #5057 ) ;
#25722=PLANE ( 'NONE',  #75993 ) ;
#25725=AXIS2_PLACEMENT_3D ( 'NONE', #87877, #58807, #80624 ) ;
#25727=CARTESIAN_POINT ( 'NONE',  ( 97.06114394585299010, -37.99679135525541795, 92.42732210906062562 ) ) ;
#25728=CARTESIAN_POINT ( 'NONE',  ( 112.8018845221357367, -47.09986945403115044, 102.9784824187679817 ) ) ;
#25729=CYLINDRICAL_SURFACE ( 'NONE', #40210, 0.5000000000000073275 ) ;
#25730=DIRECTION ( 'NONE',  ( -1.000000000000000000, 0.000000000000000000, 0.000000000000000000 ) ) ;
#25731=LINE ( 'NONE', #18464, #22342 ) ;
#25733=CARTESIAN_POINT ( 'NONE',  ( 97.81269203708822602, -40.51987569166981018, 56.63541895716551267 ) ) ;
#25734=CARTESIAN_POINT ( 'NONE',  ( 96.76471471792635271, -35.27954033865441374, 177.2156252759109805 ) ) ;
#25735=CARTESIAN_POINT ( 'NONE',  ( 41.56648329127499153, -36.32844715994070839, 138.9256252759119832 ) ) ;
#25737=ORIENTED_EDGE ( 'NONE', *, *, #65804, .T. ) ;
#25740=CARTESIAN_POINT ( 'NONE',  ( 102.0677916066047857, -27.97004931035759867, 135.4896765091952489 ) ) ;
#25742=CARTESIAN_POINT ( 'NONE',  ( 96.76538361991065074, -40.86468949728195099, 251.6422919425776001 ) ) ;
#25743=ORIENTED_EDGE ( 'NONE', *, *, #406, .F. ) ;
#25744=DIRECTION ( 'NONE',  ( 0.000000000000000000, 0.000000000000000000, -1.000000000000000000 ) ) ;
#25745=CARTESIAN_POINT ( 'NONE',  ( 115.6732227570775819, -30.74586734987101622, 275.3099109901965562 ) ) ;
#25746=CARTESIAN_POINT ( 'NONE',  ( 117.0748215982922176, -30.29170057715430531, 140.2813395616249750 ) ) ;
#25747=PLANE ( 'NONE',  #83880 ) ;
#25752=ORIENTED_EDGE ( 'NONE', *, *, #47737, .T. ) ;
#25754=AXIS2_PLACEMENT_3D ( 'NONE', #11594, #18387, #12485 ) ;
#25755=ADVANCED_FACE ( 'NONE', ( #58659 ), #31405, .F. ) ;
#25756=ORIENTED_EDGE ( 'NONE', *, *, #4192, .F. ) ;
#25759=CARTESIAN_POINT ( 'NONE',  ( 112.0659116130450030, -45.48839626610337916, 72.98979194171874951 ) ) ;
#25760=CARTESIAN_POINT ( 'NONE',  ( 114.8031991714176741, -43.68443766454699073, 34.24419670448197905 ) ) ;
#25764=VECTOR ( 'NONE', #52234, 1000.000000000000114 ) ;
#25766=DIRECTION ( 'NONE',  ( 0.000000000000000000, 0.000000000000000000, 1.000000000000000000 ) ) ;
#25768=CARTESIAN_POINT ( 'NONE',  ( 111.4808447759429413, -44.07556959346039349, 237.4295626852199632 ) ) ;
#25771=ORIENTED_EDGE ( 'NONE', *, *, #77057, .T. ) ;
#25772=VECTOR ( 'NONE', #69127, 1000.000000000000000 ) ;
#25773=EDGE_CURVE ( 'NONE', #5538, #28440, #25497, .T. ) ;
#25775=CARTESIAN_POINT ( 'NONE',  ( 117.0518796628545601, -35.94349769466420241, 183.8890245146588995 ) ) ;
#25776=CARTESIAN_POINT ( 'NONE',  ( 97.81168895331838087, -40.51742574516882200, 287.6356252759109680 ) ) ;
#25777=DIRECTION ( 'NONE',  ( 0.000000000000000000, 0.000000000000000000, -1.000000000000000000 ) ) ;
#25779=CARTESIAN_POINT ( 'NONE',  ( 115.2782656938782821, -32.16401669718150202, 25.67396425827794815 ) ) ;
#25780=CARTESIAN_POINT ( 'NONE',  ( 130.0664832912740110, -14.47844715994100007, 284.9256252759119548 ) ) ;
#25781=EDGE_CURVE ( 'NONE', #62123, #22667, #59011, .T. ) ;
#25782=CARTESIAN_POINT ( 'NONE',  ( 116.7892270726677140, -35.66563809581925426, 278.9127681330543851 ) ) ;
#25783=LINE ( 'NONE', #53909, #39949 ) ;
#25784=ADVANCED_FACE ( 'NONE', ( #25051 ), #20759, .T. ) ;
#25785=ORIENTED_EDGE ( 'NONE', *, *, #58502, .F. ) ;
#25786=ADVANCED_FACE ( 'NONE', ( #25954 ), #28011, .T. ) ;
#25788=AXIS2_PLACEMENT_3D ( 'NONE', #49819, #21240, #35294 ) ;
#25790=CARTESIAN_POINT ( 'NONE',  ( 109.7208934110032743, -44.96686374295461519, 55.65475703625794068 ) ) ;
#25791=VECTOR ( 'NONE', #26099, 1000.000000000000000 ) ;
#25792=EDGE_CURVE ( 'NONE', #86125, #73517, #52272, .T. ) ;
#25793=EDGE_CURVE ( 'NONE', #82312, #75243, #75893, .T. ) ;
#25794=CARTESIAN_POINT ( 'NONE',  ( 134.4383386549280317, -15.97944715994100839, 8.225625275911001566 ) ) ;
#25795=ADVANCED_FACE ( 'NONE', ( #27736 ), #74995, .T. ) ;
#25796=DIRECTION ( 'NONE',  ( 0.000000000000000000, 0.000000000000000000, -1.000000000000000000 ) ) ;
#25798=ORIENTED_EDGE ( 'NONE', *, *, #9209, .F. ) ;
#25799=CARTESIAN_POINT ( 'NONE',  ( 83.56670390244801183, -39.24694715994102268, 219.5838068554169809 ) ) ;
#25801=EDGE_CURVE ( 'NONE', #60102, #9112, #7724, .T. ) ;
#25802=ORIENTED_EDGE ( 'NONE', *, *, #27128, .F. ) ;
#25803=CARTESIAN_POINT ( 'NONE',  ( 117.3640430381357334, -38.35649778030718693, 113.7013395616249767 ) ) ;
#25804=VERTEX_POINT ( 'NONE', #7304 ) ;
#25805=CARTESIAN_POINT ( 'NONE',  ( 112.2681825743621431, -29.31628353742046755, 84.00003887569602057 ) ) ;
#25806=EDGE_CURVE ( 'NONE', #62879, #34580, #20929, .T. ) ;
#25807=CARTESIAN_POINT ( 'NONE',  ( 194.5664832912739826, 15.62155284005900491, 328.6381252759109088 ) ) ;
#25808=CARTESIAN_POINT ( 'NONE',  ( 99.48689454471329441, -42.28159629070200509, 103.2492023535159831 ) ) ;
#25809=DIRECTION ( 'NONE',  ( 4.299999999999999979E-14, -1.000000000000000000, 0.000000000000000000 ) ) ;
#25812=CARTESIAN_POINT ( 'NONE',  ( 108.9892323659770170, -46.99785963944585632, 78.72419670448194040 ) ) ;
#25813=DIRECTION ( 'NONE',  ( -0.7071067811865779928, 0.7071067811865171526, -7.071067811865475333E-16 ) ) ;
#25818=AXIS2_PLACEMENT_3D ( 'NONE', #65509, #17806, #52287 ) ;
#25820=ORIENTED_EDGE ( 'NONE', *, *, #82033, .T. ) ;
#25825=ORIENTED_EDGE ( 'NONE', *, *, #29698, .T. ) ;
#25826=CARTESIAN_POINT ( 'NONE',  ( 116.3159835831962852, -41.41832011455028351, 248.4651490854349731 ) ) ;
#25827=EDGE_CURVE ( 'NONE', #16260, #3733, #59952, .T. ) ;
#25828=CARTESIAN_POINT ( 'NONE',  ( 97.44427603289686601, -39.46115625027057661, 126.5460739273663364 ) ) ;
#25829=CARTESIAN_POINT ( 'NONE',  ( 100.8874677950680478, -44.70022130669426730, 188.0522919337000758 ) ) ;
#25830=CARTESIAN_POINT ( 'NONE',  ( 96.71481148478426348, -38.23418088628295664, 62.44133956162495025 ) ) ;
#25832=ADVANCED_FACE ( 'NONE', ( #55419 ), #7786, .T. ) ;
#25834=CARTESIAN_POINT ( 'NONE',  ( 165.3359832912748004, -36.32844715993531537, 300.4678068554149490 ) ) ;
#25835=AXIS2_PLACEMENT_3D ( 'NONE', #18984, #46212, #74396 ) ;
#25838=DIRECTION ( 'NONE',  ( 0.000000000000000000, 0.000000000000000000, 1.000000000000000000 ) ) ;
#25839=ORIENTED_EDGE ( 'NONE', *, *, #51796, .F. ) ;
#25841=CARTESIAN_POINT ( 'NONE',  ( 72.26648329127297643, -1.929447159941394263, 352.4506252759079530 ) ) ;
#25842=CARTESIAN_POINT ( 'NONE',  ( 117.4970320020027259, -36.54623693216564106, 288.8413395616252615 ) ) ;
#25843=CARTESIAN_POINT ( 'NONE',  ( 51.06670390244799762, -33.35206098992630075, -5.074374724088000832 ) ) ;
#25846=CARTESIAN_POINT ( 'NONE',  ( 111.4459538621439805, -44.65616828817710626, 252.3886103042673028 ) ) ;
#25848=CARTESIAN_POINT ( 'NONE',  ( 100.3128846869253294, -46.43702735306945328, 83.09276813305294240 ) ) ;
#25850=CARTESIAN_POINT ( 'NONE',  ( 117.8461808354131080, -34.08161713018977679, 164.0061014663869798 ) ) ;
#25851=VERTEX_POINT ( 'NONE', #41792 ) ;
#25853=ORIENTED_EDGE ( 'NONE', *, *, #44785, .T. ) ;
#25854=AXIS2_PLACEMENT_3D ( 'NONE', #16795, #927, #65815 ) ;
#25856=FACE_OUTER_BOUND ( 'NONE', #33775, .T. ) ;
#25857=CARTESIAN_POINT ( 'NONE',  ( 134.7196861477233654, -34.05633243510673935, 1.689562801603117892 ) ) ;
#25860=CARTESIAN_POINT ( 'NONE',  ( 117.0653594338693892, -39.95035295773606521, 158.5784824187679476 ) ) ;
#25862=DIRECTION ( 'NONE',  ( 0.000000000000000000, 1.000000000000000000, 0.000000000000000000 ) ) ;
#25864=DIRECTION ( 'NONE',  ( 1.000000000000000000, 0.000000000000000000, -7.043400939473319300E-33 ) ) ;
#25866=CARTESIAN_POINT ( 'NONE',  ( 32.09598329127702243, -23.42844715994121785, 313.9678068554150059 ) ) ;
#25869=LINE ( 'NONE', #3635, #86376 ) ;
#25872=ORIENTED_EDGE ( 'NONE', *, *, #6962, .F. ) ;
#25873=DIRECTION ( 'NONE',  ( -3.360405532702990443E-14, 1.000000000000000000, 0.000000000000000000 ) ) ;
#25875=DIRECTION ( 'NONE',  ( -1.000000000000000078E-15, 1.000000000000000083E-30, 1.000000000000000000 ) ) ;
#25878=CARTESIAN_POINT ( 'NONE',  ( 112.1390831963027637, -28.01267242204366781, 104.6564824957334423 ) ) ;
#25880=CARTESIAN_POINT ( 'NONE',  ( 111.2668257968264527, -46.89591768004029149, 292.6356252759106837 ) ) ;
#25882=ORIENTED_EDGE ( 'NONE', *, *, #47966, .T. ) ;
#25885=CARTESIAN_POINT ( 'NONE',  ( 123.6837132603319418, -50.82895651782485658, 229.5838068554170093 ) ) ;
#25887=CARTESIAN_POINT ( 'NONE',  ( 99.57924082623978279, -30.38476633542330774, 211.7670538473389570 ) ) ;
#25888=CARTESIAN_POINT ( 'NONE',  ( 106.5646857698207981, -25.28130207810567498, 321.1698005525342978 ) ) ;
#25889=VERTEX_POINT ( 'NONE', #62702 ) ;
#25891=EDGE_CURVE ( 'NONE', #59432, #628, #58540, .T. ) ;
#25892=CARTESIAN_POINT ( 'NONE',  ( 115.5638989210037124, -29.55965564860111527, 70.38419670448092802 ) ) ;
#25893=DIRECTION ( 'NONE',  ( 9.351236661543306751E-17, -3.725950533538267725E-29, -1.000000000000000000 ) ) ;
#25896=DIRECTION ( 'NONE',  ( -5.551115123125777653E-14, -1.000000000000000000, 0.000000000000000000 ) ) ;
#25897=EDGE_CURVE ( 'NONE', #35135, #34504, #14115, .T. ) ;
#25900=EDGE_CURVE ( 'NONE', #64418, #3248, #34547, .T. ) ;
#25904=CARTESIAN_POINT ( 'NONE',  ( 101.6974430329241272, -44.43982537643711339, 233.5120594963729559 ) ) ;
#25905=EDGE_CURVE ( 'NONE', #27387, #4960, #32400, .T. ) ;
#25909=DIRECTION ( 'NONE',  ( 1.000000000000000078E-15, 0.000000000000000000, 1.000000000000000000 ) ) ;
#25911=FACE_OUTER_BOUND ( 'NONE', #66121, .T. ) ;
#25912=ORIENTED_EDGE ( 'NONE', *, *, #61778, .F. ) ;
#25913=LINE ( 'NONE', #87690, #66762 ) ;
#25915=ORIENTED_EDGE ( 'NONE', *, *, #71963, .T. ) ;
#25916=CARTESIAN_POINT ( 'NONE',  ( 96.58568816239599641, -40.17018292043295702, 286.5908633711491120 ) ) ;
#25917=ORIENTED_EDGE ( 'NONE', *, *, #20404, .T. ) ;
#25918=ORIENTED_EDGE ( 'NONE', *, *, #32811, .F. ) ;
#25919=CARTESIAN_POINT ( 'NONE',  ( 105.3241794147103008, -28.72650611001668608, 258.0652332267344491 ) ) ;
#25921=CARTESIAN_POINT ( 'NONE',  ( 113.6473777113568531, -44.00994186338857617, 133.1613395616259936 ) ) ;
#25922=DIRECTION ( 'NONE',  ( 0.000000000000000000, 0.000000000000000000, 1.000000000000000000 ) ) ;
#25924=CYLINDRICAL_SURFACE ( 'NONE', #44743, 2.030000000001869864 ) ;
#25925=CIRCLE ( 'NONE', #73766, 2.500000000000002220 ) ;
#25926=EDGE_CURVE ( 'NONE', #78352, #16601, #88640, .T. ) ;
#25927=CARTESIAN_POINT ( 'NONE',  ( 95.35923950155199691, -38.86288465644625489, 197.4699109901969791 ) ) ;
#25928=DIRECTION ( 'NONE',  ( 0.000000000000000000, 0.000000000000000000, -1.000000000000000000 ) ) ;
#25930=CARTESIAN_POINT ( 'NONE',  ( 118.8919219083537797, -35.39899076563189340, 79.91562527591095488 ) ) ;
#25931=CARTESIAN_POINT ( 'NONE',  ( 128.5967921371759815, -18.82844715994100682, 342.9256252759109884 ) ) ;
#25932=VERTEX_POINT ( 'NONE', #19576 ) ;
#25933=EDGE_LOOP ( 'NONE', ( #82683, #68929, #82920, #36848 ) ) ;
#25934=EDGE_LOOP ( 'NONE', ( #47419, #24680, #15054, #36044 ) ) ;
#25935=CARTESIAN_POINT ( 'NONE',  ( 77.31648329127401098, -36.72944715994107412, 3.101481641215480867 ) ) ;
#25936=DIRECTION ( 'NONE',  ( 1.000000000000000078E-15, -1.000000000000000083E-30, -1.000000000000000000 ) ) ;
#25937=CARTESIAN_POINT ( 'NONE',  ( 41.56648329127399677, -9.303447159940999356, 258.9256252759120116 ) ) ;
#25938=CARTESIAN_POINT ( 'NONE',  ( 114.9723337227840005, -34.69788249897437993, 121.8452332267339671 ) ) ;
#25939=CARTESIAN_POINT ( 'NONE',  ( 100.8102337077607871, -45.86971777371983450, 238.1108633711489517 ) ) ;
#25940=DIRECTION ( 'NONE',  ( 0.000000000000000000, 0.000000000000000000, -1.000000000000000000 ) ) ;
#25942=ORIENTED_EDGE ( 'NONE', *, *, #36522, .T. ) ;
#25944=CIRCLE ( 'NONE', #75289, 16.00000000000000000 ) ;
#25945=EDGE_CURVE ( 'NONE', #1529, #58575, #8200, .T. ) ;
#25946=CYLINDRICAL_SURFACE ( 'NONE', #6982, 2.116999999999980009 ) ;
#25947=ORIENTED_EDGE ( 'NONE', *, *, #40374, .T. ) ;
#25948=ORIENTED_EDGE ( 'NONE', *, *, #62994, .T. ) ;
#25949=AXIS2_PLACEMENT_3D ( 'NONE', #40052, #75491, #53661 ) ;
#25950=AXIS2_PLACEMENT_3D ( 'NONE', #17326, #37320, #43220 ) ;
#25952=ORIENTED_EDGE ( 'NONE', *, *, #46278, .F. ) ;
#25953=ORIENTED_EDGE ( 'NONE', *, *, #53674, .T. ) ;
#25954=FACE_OUTER_BOUND ( 'NONE', #61290, .T. ) ;
#25956=FACE_OUTER_BOUND ( 'NONE', #57361, .T. ) ;
#25957=CARTESIAN_POINT ( 'NONE',  ( 107.7643578131546178, -45.27140672887451700, 177.0638483995059858 ) ) ;
#25958=CARTESIAN_POINT ( 'NONE',  ( 99.03195499373370581, -44.38837911315224716, 36.92038718067297509 ) ) ;
#25960=EDGE_LOOP ( 'NONE', ( #58948, #24745, #34211, #85868 ) ) ;
#25962=DIRECTION ( 'NONE',  ( -1.000000000000000078E-15, 0.000000000000000000, -1.000000000000000000 ) ) ;
#25963=ORIENTED_EDGE ( 'NONE', *, *, #40976, .F. ) ;
#25964=VECTOR ( 'NONE', #24670, 1000.000000000000000 ) ;
#25965=CARTESIAN_POINT ( 'NONE',  ( 142.8821648370248170, -72.54478064608022692, 394.9756252759102040 ) ) ;
#25966=ORIENTED_EDGE ( 'NONE', *, *, #28378, .T. ) ;
#25967=CARTESIAN_POINT ( 'NONE',  ( 103.1366983212326573, -27.50878891356330769, 166.3966305085834847 ) ) ;
#25969=CARTESIAN_POINT ( 'NONE',  ( 99.50471754548186709, -43.30576767929590432, 131.8960681784909070 ) ) ;
#25971=CARTESIAN_POINT ( 'NONE',  ( 51.56670390244683944, -33.35206098992668444, 117.4678068554150485 ) ) ;
#25973=CARTESIAN_POINT ( 'NONE',  ( 100.5838780899822922, -28.49162262467549667, 15.60705384733995871 ) ) ;
#25974=CARTESIAN_POINT ( 'NONE',  ( 101.0411209824609813, -27.40783209567417700, 66.54514908543495721 ) ) ;
#25977=DIRECTION ( 'NONE',  ( 0.000000000000000000, 0.000000000000000000, -1.000000000000000000 ) ) ;
#25978=CARTESIAN_POINT ( 'NONE',  ( 132.7628207310659150, -39.15113447712369776, 7.957506268078478939 ) ) ;
#25979=AXIS2_PLACEMENT_3D ( 'NONE', #40803, #19926, #7638 ) ;
#25980=CARTESIAN_POINT ( 'NONE',  ( 102.3363410760962608, -27.82220188792448567, 121.4623623916829587 ) ) ;
#25982=ORIENTED_EDGE ( 'NONE', *, *, #24337, .T. ) ;
#25983=CARTESIAN_POINT ( 'NONE',  ( 115.7653496281367325, -43.62456195820889349, 48.30514908543492680 ) ) ;
#25984=CARTESIAN_POINT ( 'NONE',  ( 112.2050260072902290, -45.80016191694880234, 208.9870538473389558 ) ) ;
#25985=CARTESIAN_POINT ( 'NONE',  ( 101.7448744985357223, -27.01524695604527082, 96.46324432352997746 ) ) ;
#25986=CARTESIAN_POINT ( 'NONE',  ( 115.0386160834107017, -42.90673886385352631, 173.2986915154965004 ) ) ;
#25988=CARTESIAN_POINT ( 'NONE',  ( 191.6377717143134873, -67.87844715994100397, 307.9888746672805269 ) ) ;
#25989=CIRCLE ( 'NONE', #43417, 3.250000000000002665 ) ;
#25991=EDGE_CURVE ( 'NONE', #65338, #72917, #23197, .T. ) ;
#25995=CARTESIAN_POINT ( 'NONE',  ( 112.9285164932675514, -28.85859325239454165, 100.5670538473389684 ) ) ;
#25997=EDGE_LOOP ( 'NONE', ( #42336, #14586, #72056, #19319 ) ) ;
#25999=CARTESIAN_POINT ( 'NONE',  ( 116.9047011640239759, -41.71676023082950735, 244.4651490854349731 ) ) ;
#26000=CARTESIAN_POINT ( 'NONE',  ( 115.7827659893201968, -41.80290719135400934, 254.4082417524339235 ) ) ;
#26001=CARTESIAN_POINT ( 'NONE',  ( 90.44969454456408187, -53.34645651782490461, 239.5838068554174356 ) ) ;
#26003=CARTESIAN_POINT ( 'NONE',  ( 97.33784131839850318, -34.07106450384809193, 82.11479194044655117 ) ) ;
#26004=AXIS2_PLACEMENT_3D ( 'NONE', #22100, #48861, #8001 ) ;
#26005=CARTESIAN_POINT ( 'NONE',  ( 131.3165190107490048, -36.90078909148135011, 3.101427792080953871 ) ) ;
#26006=ADVANCED_FACE ( 'NONE', ( #83613 ), #14573, .F. ) ;
#26008=CARTESIAN_POINT ( 'NONE',  ( 97.38117110781242047, -35.36630255995240191, 181.2156252759109805 ) ) ;
#26009=EDGE_LOOP ( 'NONE', ( #42873, #64008, #23111, #70368 ) ) ;
#26011=CIRCLE ( 'NONE', #4223, 12.99999999999999822 ) ;
#26012=CARTESIAN_POINT ( 'NONE',  ( 108.6971488411468414, -45.98241724535997577, 119.1349166392299566 ) ) ;
#26013=TOROIDAL_SURFACE ( 'NONE', #88396, 15.69999999999999929, 0.2999999999999999889 ) ;
#26014=ADVANCED_FACE ( 'NONE', ( #7744 ), #85420, .T. ) ;
#26015=CARTESIAN_POINT ( 'NONE',  ( 33.92127028473601769, -29.73316016639540749, 313.9678068554150059 ) ) ;
#26016=CARTESIAN_POINT ( 'NONE',  ( 98.19951187208815213, -40.85743130997446571, 252.6727681330533812 ) ) ;
#26017=LINE ( 'NONE', #20102, #46222 ) ;
#26019=ADVANCED_FACE ( 'NONE', ( #49054 ), #15913, .T. ) ;
#26020=FACE_OUTER_BOUND ( 'NONE', #86363, .T. ) ;
#26021=VECTOR ( 'NONE', #27270, 1000.000000000000000 ) ;
#26022=DIRECTION ( 'NONE',  ( -1.000000000000000000, 0.000000000000000000, 0.000000000000000000 ) ) ;
#26026=CARTESIAN_POINT ( 'NONE',  ( 116.3308458273176456, -44.07926308385601999, 198.2927681330539542 ) ) ;
#26027=CARTESIAN_POINT ( 'NONE',  ( 116.3212776292296127, -32.94146857471318413, 287.6356252759109680 ) ) ;
#26029=ORIENTED_EDGE ( 'NONE', *, *, #88719, .F. ) ;
#26031=CARTESIAN_POINT ( 'NONE',  ( 78.82300719539804845, -16.27587548316634525, 1.868342134758776307 ) ) ;
#26032=AXIS2_PLACEMENT_3D ( 'NONE', #1641, #28427, #29342 ) ;
#26036=ORIENTED_EDGE ( 'NONE', *, *, #9182, .F. ) ;
#26037=CARTESIAN_POINT ( 'NONE',  ( 113.1764815558486390, -44.75322278302650147, 63.09378032628466570 ) ) ;
#26038=CARTESIAN_POINT ( 'NONE',  ( 107.2492389712779612, -24.88009754917498739, 230.0641967044819580 ) ) ;
#26039=DIRECTION ( 'NONE',  ( -0.9254794337955620787, -0.3787978585227822492, 0.000000000000000000 ) ) ;
#26040=ORIENTED_EDGE ( 'NONE', *, *, #20432, .F. ) ;
#26043=CARTESIAN_POINT ( 'NONE',  ( 184.5667039024480118, -67.87844715994100397, 300.9178068554150514 ) ) ;
#26044=CARTESIAN_POINT ( 'NONE',  ( 113.1774532810855760, -44.75249673545214080, 164.0938759193286955 ) ) ;
#26045=CARTESIAN_POINT ( 'NONE',  ( 98.96120113019971143, -37.69594967233602034, 39.23951894101995919 ) ) ;
#26046=CARTESIAN_POINT ( 'NONE',  ( 103.4608836344597194, -46.53438966646587005, 138.2956252759109645 ) ) ;
#26047=DIRECTION ( 'NONE',  ( 1.000000000000000078E-15, -1.000000000000000000, 0.000000000000000000 ) ) ;
#26048=VERTEX_POINT ( 'NONE', #1387 ) ;
#26050=FACE_OUTER_BOUND ( 'NONE', #48493, .T. ) ;
#26052=LINE ( 'NONE', #46911, #44475 ) ;
#26054=ORIENTED_EDGE ( 'NONE', *, *, #4031, .F. ) ;
#26055=APPLICATION_CONTEXT ( 'automotive_design' ) ;
#26057=ORIENTED_EDGE ( 'NONE', *, *, #39314, .F. ) ;
#26058=ORIENTED_EDGE ( 'NONE', *, *, #44285, .F. ) ;
#26060=CARTESIAN_POINT ( 'NONE',  ( 100.2301541646454552, -41.85006585248910937, 66.26099125664796929 ) ) ;
#26061=CARTESIAN_POINT ( 'NONE',  ( 99.27200920372420967, -29.77297264586844960, 190.7470538473399415 ) ) ;
#26063=CARTESIAN_POINT ( 'NONE',  ( 101.7806060443208480, -45.68981339355064364, 162.1527681330539679 ) ) ;
#26064=CARTESIAN_POINT ( 'NONE',  ( 110.1478212817822424, -46.33253055760241068, 22.82345756811338333 ) ) ;
#26065=CARTESIAN_POINT ( 'NONE',  ( 104.5881800117806932, -26.60309611811081254, 281.2670538473395823 ) ) ;
#26067=DIRECTION ( 'NONE',  ( 0.7071067811873671394, 0.7071067811857280061, -2.899137802861369224E-29 ) ) ;
#26068=ORIENTED_EDGE ( 'NONE', *, *, #66512, .T. ) ;
#26069=CIRCLE ( 'NONE', #37686, 2.999999999999947153 ) ;
#26072=EDGE_CURVE ( 'NONE', #28588, #45463, #51269, .T. ) ;
#26074=CARTESIAN_POINT ( 'NONE',  ( 118.0975507117283883, -35.49314816969329200, 233.9032443235299752 ) ) ;
#26075=ORIENTED_EDGE ( 'NONE', *, *, #61535, .F. ) ;
#26076=CARTESIAN_POINT ( 'NONE',  ( 114.9651742339629976, -29.92520496456729262, 184.3927681330539770 ) ) ;
#26077=DIRECTION ( 'NONE',  ( 0.000000000000000000, 0.000000000000000000, 1.000000000000000000 ) ) ;
#26079=DIRECTION ( 'NONE',  ( 0.000000000000000000, 0.000000000000000000, 1.000000000000000000 ) ) ;
#26080=CARTESIAN_POINT ( 'NONE',  ( 116.8785659245552466, -39.03624075203685351, 29.64421603613703482 ) ) ;
#26081=CARTESIAN_POINT ( 'NONE',  ( 98.33459205555250549, -35.67394987134639450, 277.6356252759110816 ) ) ;
#26084=DIRECTION ( 'NONE',  ( -0.9254794337955621897, -0.3787978585227819717, 0.000000000000000000 ) ) ;
#26087=CARTESIAN_POINT ( 'NONE',  ( 80.06648329127399677, -9.029447159941060619, 1.625625275910943746 ) ) ;
#26093=DIRECTION ( 'NONE',  ( 0.000000000000000000, 0.000000000000000000, -1.000000000000000000 ) ) ;
#26094=CARTESIAN_POINT ( 'NONE',  ( 103.6313148537710305, -26.19877486694289459, 210.3394347997209763 ) ) ;
#26095=CARTESIAN_POINT ( 'NONE',  ( 117.8564148307409596, -39.12764603782969886, 99.64038718067195077 ) ) ;
#26096=CARTESIAN_POINT ( 'NONE',  ( 100.2187443247741783, -45.46477599873944797, 273.0594347997206910 ) ) ;
#26097=CARTESIAN_POINT ( 'NONE',  ( 83.56670390244801183, -36.72944715994108122, 219.5838068554169809 ) ) ;
#26098=AXIS2_PLACEMENT_3D ( 'NONE', #6173, #33861, #83827 ) ;
#26099=DIRECTION ( 'NONE',  ( 0.000000000000000000, 0.000000000000000000, 1.000000000000000000 ) ) ;
#26103=CARTESIAN_POINT ( 'NONE',  ( 133.3217830637437658, -21.37853523628597330, 1.709393643970599674 ) ) ;
#26104=ORIENTED_EDGE ( 'NONE', *, *, #29872, .T. ) ;
#26105=VERTEX_POINT ( 'NONE', #63152 ) ;
#26106=EDGE_CURVE ( 'NONE', #59488, #48723, #56775, .T. ) ;
#26108=CARTESIAN_POINT ( 'NONE',  ( 115.7032693465968975, -34.00573701374007385, 128.4800388756959819 ) ) ;
#26110=ORIENTED_EDGE ( 'NONE', *, *, #72891, .F. ) ;
#26111=LINE ( 'NONE', #54223, #88076 ) ;
#26113=CARTESIAN_POINT ( 'NONE',  ( 102.7067583520261138, -46.86140753836539119, 133.2651490854349561 ) ) ;
#26114=CYLINDRICAL_SURFACE ( 'NONE', #86032, 2.030000000001807248 ) ;
#26115=ADVANCED_FACE ( 'NONE', ( #21836, #36797 ), #35893, .F. ) ;
#26118=EDGE_CURVE ( 'NONE', #66670, #84435, #49507, .T. ) ;
#26120=CARTESIAN_POINT ( 'NONE',  ( 106.0550521757682816, -27.00111521709620277, 50.15848241876896907 ) ) ;
#26121=ORIENTED_EDGE ( 'NONE', *, *, #66281, .F. ) ;
#26124=EDGE_LOOP ( 'NONE', ( #57038, #21411, #58241, #49966, #45037, #31511 ) ) ;
#26126=CARTESIAN_POINT ( 'NONE',  ( 104.0088209277215867, -27.43890701233904394, 161.3299109901969643 ) ) ;
#26128=DIRECTION ( 'NONE',  ( 0.000000000000000000, 0.000000000000000000, -1.000000000000000000 ) ) ;
#26131=EDGE_CURVE ( 'NONE', #8047, #44005, #49298, .T. ) ;
#26133=VECTOR ( 'NONE', #64453, 1000.000000000000000 ) ;
#26134=DIRECTION ( 'NONE',  ( -0.7071067811865175967, -0.7071067811865774377, -7.071067811865168663E-16 ) ) ;
#26135=CARTESIAN_POINT ( 'NONE',  ( 72.06648329127396835, -8.979447159941065237, 14.67562527591093513 ) ) ;
#26136=CARTESIAN_POINT ( 'NONE',  ( 117.3497117099304745, -32.73958051198272301, 94.10895860924395606 ) ) ;
#26139=AXIS2_PLACEMENT_3D ( 'NONE', #68224, #13258, #88677 ) ;
#26140=DIRECTION ( 'NONE',  ( 0.000000000000000000, 0.000000000000000000, -1.000000000000000000 ) ) ;
#26142=LINE ( 'NONE', #87917, #33647 ) ;
#26143=CARTESIAN_POINT ( 'NONE',  ( 107.5257129551532813, -44.87112140103544533, 150.4395189410199407 ) ) ;
#26145=EDGE_LOOP ( 'NONE', ( #20742, #9470, #19398, #69954 ) ) ;
#26146=ORIENTED_EDGE ( 'NONE', *, *, #46420, .T. ) ;
#26147=ORIENTED_EDGE ( 'NONE', *, *, #53074, .T. ) ;
#26148=VERTEX_POINT ( 'NONE', #17247 ) ;
#26150=CARTESIAN_POINT ( 'NONE',  ( 77.59226090855182179, -19.93375462387231067, 7.110117206099022980 ) ) ;
#26151=CARTESIAN_POINT ( 'NONE',  ( 115.8610455727973090, -35.41879699190349129, 215.3758690201829609 ) ) ;
#26152=DIRECTION ( 'NONE',  ( 1.000000000000000000, 0.000000000000000000, 0.000000000000000000 ) ) ;
#26157=ORIENTED_EDGE ( 'NONE', *, *, #45360, .F. ) ;
#26158=VERTEX_POINT ( 'NONE', #51735 ) ;
#26159=DIRECTION ( 'NONE',  ( 0.000000000000000000, 0.000000000000000000, 1.000000000000000000 ) ) ;
#26160=ORIENTED_EDGE ( 'NONE', *, *, #3030, .T. ) ;
#26162=ADVANCED_FACE ( 'NONE', ( #86285 ), #44928, .F. ) ;
#26164=CARTESIAN_POINT ( 'NONE',  ( 111.7906875226637879, -43.98084836425640276, 220.8661856076869583 ) ) ;
#26165=CARTESIAN_POINT ( 'NONE',  ( 98.07775226919108036, -31.40506188283435307, 85.90133956162493689 ) ) ;
#26166=CARTESIAN_POINT ( 'NONE',  ( 117.2454586689012359, -38.87819698039184146, 63.66133956162494911 ) ) ;
#26167=CARTESIAN_POINT ( 'NONE',  ( 111.9916049118937877, -43.86739420629758257, 249.5838068554168672 ) ) ;
#26168=CARTESIAN_POINT ( 'NONE',  ( 133.0080215814353721, -16.19118199975284611, 8.051357469095140829 ) ) ;
#26170=CARTESIAN_POINT ( 'NONE',  ( 117.4263761885577537, -30.97555849962366281, 175.2299109901969700 ) ) ;
#26171=CARTESIAN_POINT ( 'NONE',  ( 48.16670390244701139, -26.71338133339251542, -5.074374724088000832 ) ) ;
#26172=VERTEX_POINT ( 'NONE', #59887 ) ;
#26173=DIRECTION ( 'NONE',  ( -1.000000000000000000, -4.299999999999999979E-14, -1.000000000000000078E-15 ) ) ;
#26175=ORIENTED_EDGE ( 'NONE', *, *, #4165, .F. ) ;
#26178=VERTEX_POINT ( 'NONE', #73086 ) ;
#26179=LINE ( 'NONE', #47494, #67848 ) ;
#26180=EDGE_CURVE ( 'NONE', #58422, #27248, #35326, .T. ) ;
#26182=CARTESIAN_POINT ( 'NONE',  ( 103.2788000081581288, -47.11369209158109328, 97.28610146638693834 ) ) ;
#26184=CARTESIAN_POINT ( 'NONE',  ( 107.0664832912739968, 0.2215528400590083269, 330.1506252759110680 ) ) ;
#26185=PLANE ( 'NONE',  #48430 ) ;
#26188=CARTESIAN_POINT ( 'NONE',  ( 97.93839266929580845, -41.72010113774604889, 217.7241967044829494 ) ) ;
#26189=LINE ( 'NONE', #46609, #68433 ) ;
#26190=CARTESIAN_POINT ( 'NONE',  ( 179.4595971212720258, -26.00627455219132500, 342.9256252759109884 ) ) ;
#26191=VERTEX_POINT ( 'NONE', #45806 ) ;
#26197=CARTESIAN_POINT ( 'NONE',  ( 106.5652189068774902, -47.22232703829767786, 247.5384824187679556 ) ) ;
#26198=ORIENTED_EDGE ( 'NONE', *, *, #22322, .F. ) ;
#26199=CARTESIAN_POINT ( 'NONE',  ( 104.5038485128689416, -27.03369106489477502, 195.2819955450332827 ) ) ;
#26200=CARTESIAN_POINT ( 'NONE',  ( 105.3204089162997263, -26.45171782723944176, 11.20991099019697046 ) ) ;
#26201=CARTESIAN_POINT ( 'NONE',  ( 98.80568095843470644, -28.16380313737984764, 111.6870538473389587 ) ) ;
#26204=LINE ( 'NONE', #20735, #85550 ) ;
#26205=CYLINDRICAL_SURFACE ( 'NONE', #87821, 2.500000000000002220 ) ;
#26206=CARTESIAN_POINT ( 'NONE',  ( 98.34985895919700738, -31.65658473072328860, 190.9064586020228660 ) ) ;
#26207=ORIENTED_EDGE ( 'NONE', *, *, #35823, .T. ) ;
#26208=VERTEX_POINT ( 'NONE', #9985 ) ;
#26209=ORIENTED_EDGE ( 'NONE', *, *, #8956, .T. ) ;
#26210=ORIENTED_EDGE ( 'NONE', *, *, #39242, .T. ) ;
#26211=DIRECTION ( 'NONE',  ( 0.7071067811865473507, 0.7071067811865476838, 0.000000000000000000 ) ) ;
#26212=CARTESIAN_POINT ( 'NONE',  ( 105.4244226815142298, -47.00233879195495490, 33.44991099019695469 ) ) ;
#26213=LINE ( 'NONE', #60719, #84661 ) ;
#26217=DIRECTION ( 'NONE',  ( 0.000000000000000000, 0.000000000000000000, -1.000000000000000000 ) ) ;
#26218=CARTESIAN_POINT ( 'NONE',  ( 109.4611421171680945, -28.53056059958231216, 259.2724198280769770 ) ) ;
#26220=ORIENTED_EDGE ( 'NONE', *, *, #5272, .F. ) ;
#26223=CARTESIAN_POINT ( 'NONE',  ( 98.04154813939969415, -41.04191879011435162, 101.6816083635749379 ) ) ;
#26226=CARTESIAN_POINT ( 'NONE',  ( 115.8371248229627639, -37.99598801341877419, 25.14444044875396855 ) ) ;
#26229=ADVANCED_FACE ( 'NONE', ( #25384 ), #31298, .F. ) ;
#26231=CARTESIAN_POINT ( 'NONE',  ( 97.31589510082254435, -39.30610152985839534, 176.5314694035164678 ) ) ;
#26233=CARTESIAN_POINT ( 'NONE',  ( 96.91794407517402021, -34.59732685048006573, 261.1737205140070159 ) ) ;
#26235=DIRECTION ( 'NONE',  ( -4.299999999999999979E-14, 1.000000000000000000, -4.128053709984630540E-29 ) ) ;
#26237=CARTESIAN_POINT ( 'NONE',  ( 165.3359832912740046, -36.32844715994100682, 117.4678068554150485 ) ) ;
#26238=CIRCLE ( 'NONE', #13217, 1.000000000000000888 ) ;
#26240=CARTESIAN_POINT ( 'NONE',  ( 98.66659878002396056, -40.67125783036974696, 59.49380465530595785 ) ) ;
#26241=AXIS2_PLACEMENT_3D ( 'NONE', #47698, #6383, #68619 ) ;
#26242=PLANE ( 'NONE',  #55139 ) ;
#26243=CARTESIAN_POINT ( 'NONE',  ( 172.5664832912729878, -18.82844715994071194, 198.9256252759119832 ) ) ;
#26245=ORIENTED_EDGE ( 'NONE', *, *, #39421, .T. ) ;
#26246=DIRECTION ( 'NONE',  ( 0.000000000000000000, 0.000000000000000000, 1.000000000000000000 ) ) ;
#26249=CARTESIAN_POINT ( 'NONE',  ( 97.93239114460148187, -31.63098981178377755, 110.9213395616259703 ) ) ;
#26250=ORIENTED_EDGE ( 'NONE', *, *, #52522, .F. ) ;
#26251=CARTESIAN_POINT ( 'NONE',  ( 115.1845888671227556, -34.07379402343466523, 88.50099125664800681 ) ) ;
#26253=DIRECTION ( 'NONE',  ( -0.7071067811578587436, 0.7071067812152364018, 0.000000000000000000 ) ) ;
#26254=CARTESIAN_POINT ( 'NONE',  ( 116.2382276885637538, -38.76798346032508391, 100.0720594963729866 ) ) ;
#26255=DIRECTION ( 'NONE',  ( 0.000000000000000000, 1.000000000000000000, 0.000000000000000000 ) ) ;
#26256=DIRECTION ( 'NONE',  ( 0.000000000000000000, 0.000000000000000000, -1.000000000000000000 ) ) ;
#26257=CARTESIAN_POINT ( 'NONE',  ( 117.2880962612577349, -38.88719764259226253, 59.66133956162595098 ) ) ;
#26258=VECTOR ( 'NONE', #42595, 1000.000000000000114 ) ;
#26260=CARTESIAN_POINT ( 'NONE',  ( 116.8172185371468146, -34.15328862580971503, 259.0314398403625091 ) ) ;
#26262=FACE_OUTER_BOUND ( 'NONE', #85504, .T. ) ;
#26266=VECTOR ( 'NONE', #23071, 1000.000000000000000 ) ;
#26267=LINE ( 'NONE', #46237, #70254 ) ;
#26269=CARTESIAN_POINT ( 'NONE',  ( 101.1405520526759574, -45.23956608920065037, 237.0803871806729717 ) ) ;
#26270=CARTESIAN_POINT ( 'NONE',  ( 117.2592865896494345, -39.02220311275136311, 144.6499109901969859 ) ) ;
#26273=CARTESIAN_POINT ( 'NONE',  ( 98.85791787721181834, -43.21333385077131339, 87.85848241876792031 ) ) ;
#26274=AXIS2_PLACEMENT_3D ( 'NONE', #35783, #50763, #55754 ) ;
#26275=CARTESIAN_POINT ( 'NONE',  ( 163.5667039024460223, -22.48495420874110806, -5.074374724088000832 ) ) ;
#26276=ORIENTED_EDGE ( 'NONE', *, *, #86903, .F. ) ;
#26277=CARTESIAN_POINT ( 'NONE',  ( 180.3503142329326465, -29.99615139350787629, 342.9256252759109884 ) ) ;
#26278=LINE ( 'NONE', #20812, #47672 ) ;
#26279=ORIENTED_EDGE ( 'NONE', *, *, #39630, .F. ) ;
#26280=LINE ( 'NONE', #88527, #2581 ) ;
#26281=EDGE_CURVE ( 'NONE', #7509, #57079, #72214, .T. ) ;
#26283=CARTESIAN_POINT ( 'NONE',  ( 110.9847977634196496, -46.36662828626499078, 282.8841967044824628 ) ) ;
#26285=CARTESIAN_POINT ( 'NONE',  ( 30.48091746481835429, -49.32844715994148288, 249.9678068554150059 ) ) ;
#26287=CARTESIAN_POINT ( 'NONE',  ( 114.1362055435773613, -41.52268812998874381, 272.7752769709339304 ) ) ;
#26288=CARTESIAN_POINT ( 'NONE',  ( 97.72316397745180439, -40.29463414041478586, 101.6170128052498995 ) ) ;
#26289=CARTESIAN_POINT ( 'NONE',  ( 97.24623519876082867, -31.70684325556598893, 91.96229194257693962 ) ) ;
#26290=CYLINDRICAL_SURFACE ( 'NONE', #58179, 3.000000000000002665 ) ;
#26291=CARTESIAN_POINT ( 'NONE',  ( 95.86269369446621624, -32.71648115089089259, 176.0527681330539735 ) ) ;
#26296=CARTESIAN_POINT ( 'NONE',  ( 32.15435173583699680, -31.62489322948790971, 237.4678068554150059 ) ) ;
#26297=CIRCLE ( 'NONE', #66875, 2.116999999999980009 ) ;
#26298=CARTESIAN_POINT ( 'NONE',  ( 115.8254323908916206, -31.73001882624620862, 65.23979194279471017 ) ) ;
#26300=ORIENTED_EDGE ( 'NONE', *, *, #65601, .F. ) ;
#26303=DIRECTION ( 'NONE',  ( -0.7071067811861110330, -0.7071067811869841124, 0.000000000000000000 ) ) ;
#26304=CARTESIAN_POINT ( 'NONE',  ( 114.2703446987665643, -45.17953892438131192, 153.1508633711489722 ) ) ;
#26305=ORIENTED_EDGE ( 'NONE', *, *, #29682, .T. ) ;
#26307=DIRECTION ( 'NONE',  ( -1.000000000000000078E-15, 1.000000000000000083E-30, 1.000000000000000000 ) ) ;
#26308=AXIS2_PLACEMENT_3D ( 'NONE', #12800, #88657, #7323 ) ;
#26310=EDGE_CURVE ( 'NONE', #51954, #84121, #53958, .T. ) ;
#26311=PLANE ( 'NONE',  #56827 ) ;
#26312=ORIENTED_EDGE ( 'NONE', *, *, #19175, .T. ) ;
#26313=VECTOR ( 'NONE', #2606, 1000.000000000000000 ) ;
#26318=ORIENTED_EDGE ( 'NONE', *, *, #18781, .T. ) ;
#26319=DIRECTION ( 'NONE',  ( 0.9068632946707807507, -0.4214249218767881500, 1.031805784967618114E-15 ) ) ;
#26321=LINE ( 'NONE', #46744, #26598 ) ;
#26323=CARTESIAN_POINT ( 'NONE',  ( 116.3262419368496978, -32.93860311337579105, 160.1356252759109680 ) ) ;
#26326=DIRECTION ( 'NONE',  ( 1.000000000000000000, -1.332267629550186637E-12, 0.000000000000000000 ) ) ;
#26327=CARTESIAN_POINT ( 'NONE',  ( 109.7247516442869539, -27.00077167917759979, 179.8648013270537263 ) ) ;
#26328=AXIS2_PLACEMENT_3D ( 'NONE', #64747, #38816, #87427 ) ;
#26329=VERTEX_POINT ( 'NONE', #4947 ) ;
#26330=DIRECTION ( 'NONE',  ( -1.000000000000000000, -4.299999999999999979E-14, -1.000000000000000078E-15 ) ) ;
#26331=CARTESIAN_POINT ( 'NONE',  ( 109.8674951572811267, -26.74480306206640989, 215.8708633711489711 ) ) ;
#26332=CIRCLE ( 'NONE', #35018, 13.16666666666670160 ) ;
#26333=FACE_OUTER_BOUND ( 'NONE', #86659, .T. ) ;
#26335=ADVANCED_FACE ( 'NONE', ( #89418 ), #6289, .F. ) ;
#26336=CARTESIAN_POINT ( 'NONE',  ( 100.4186822966650539, -43.90371905523895890, 42.98133956162492098 ) ) ;
#26337=CARTESIAN_POINT ( 'NONE',  ( 110.8601161811647273, -45.98192586914924362, 52.88611059975448825 ) ) ;
#26338=EDGE_CURVE ( 'NONE', #22610, #46354, #74887, .T. ) ;
#26339=DIRECTION ( 'NONE',  ( -0.7071067811865516806, 0.7071067811865434649, -7.071067811865511818E-16 ) ) ;
#26341=EDGE_CURVE ( 'NONE', #77150, #75223, #55306, .T. ) ;
#26343=VERTEX_POINT ( 'NONE', #82617 ) ;
#26347=ORIENTED_EDGE ( 'NONE', *, *, #49988, .T. ) ;
#26348=CARTESIAN_POINT ( 'NONE',  ( 101.7595872045747285, -44.48272901101389465, 238.5425356868499591 ) ) ;
#26349=CARTESIAN_POINT ( 'NONE',  ( 100.8876536524146843, -44.70040499368899134, 53.05193493111340786 ) ) ;
#26350=CARTESIAN_POINT ( 'NONE',  ( 177.0664832912740110, 12.92155284005802685, 336.5756252759111362 ) ) ;
#26351=CARTESIAN_POINT ( 'NONE',  ( 116.8171228687850203, -34.15291832615506706, 155.0314586087714588 ) ) ;
#26357=ORIENTED_EDGE ( 'NONE', *, *, #54204, .T. ) ;
#26358=CARTESIAN_POINT ( 'NONE',  ( 116.5620552962771654, -42.34175257684902505, 283.4137205140060587 ) ) ;
#26359=ORIENTED_EDGE ( 'NONE', *, *, #11856, .F. ) ;
#26360=EDGE_LOOP ( 'NONE', ( #20309, #37997 ) ) ;
#26361=CARTESIAN_POINT ( 'NONE',  ( 99.66640463149437323, -40.17452507577532117, 254.4909475124484857 ) ) ;
#26363=CARTESIAN_POINT ( 'NONE',  ( 118.1851208724672233, -36.91582462397655462, 153.8127681330539644 ) ) ;
#26368=CARTESIAN_POINT ( 'NONE',  ( 105.1027920011780452, -26.44660240447466037, 231.2270538473399597 ) ) ;
#26370=VERTEX_POINT ( 'NONE', #20378 ) ;
#26371=VECTOR ( 'NONE', #69748, 1000.000000000000000 ) ;
#26372=CARTESIAN_POINT ( 'NONE',  ( 107.2328990581281687, -25.63125793145087172, 76.07657765686298035 ) ) ;
#26373=CYLINDRICAL_SURFACE ( 'NONE', #45342, 5.599999999999994316 ) ;
#26374=ORIENTED_EDGE ( 'NONE', *, *, #78663, .T. ) ;
#26375=VERTEX_POINT ( 'NONE', #75337 ) ;
#26376=EDGE_LOOP ( 'NONE', ( #12700, #65458, #62976, #54628, #56325 ) ) ;
#26378=DIRECTION ( 'NONE',  ( 5.512527431108029424E-15, -1.000000000000000000, 0.000000000000000000 ) ) ;
#26379=DIRECTION ( 'NONE',  ( -1.000000000000000000, -4.299999999999999979E-14, -9.351236661543306751E-17 ) ) ;
#26381=CARTESIAN_POINT ( 'NONE',  ( 112.6831787765100898, -43.31780159632685212, 150.9690427505439914 ) ) ;
#26382=CARTESIAN_POINT ( 'NONE',  ( 100.1631548973110739, -45.39139052332982516, 268.0289586092443415 ) ) ;
#26384=CARTESIAN_POINT ( 'NONE',  ( 41.56670390244804025, -42.82844715994103524, 300.4678068554150059 ) ) ;
#26387=DIRECTION ( 'NONE',  ( 1.000000000000000000, 0.000000000000000000, 0.000000000000000000 ) ) ;
#26389=CIRCLE ( 'NONE', #20568, 2.517500000000005844 ) ;
#26390=VERTEX_POINT ( 'NONE', #27178 ) ;
#26392=FACE_BOUND ( 'NONE', #69630, .T. ) ;
#26394=VERTEX_POINT ( 'NONE', #6734 ) ;
#26396=CARTESIAN_POINT ( 'NONE',  ( 162.8913605087228404, -31.76306994223244118, 117.4678068554150485 ) ) ;
#26398=EDGE_CURVE ( 'NONE', #60336, #67129, #40355, .T. ) ;
#26399=DIRECTION ( 'NONE',  ( -2.900000000000000265E-14, 2.000000000000000155E-15, -1.000000000000000000 ) ) ;
#26401=CARTESIAN_POINT ( 'NONE',  ( 115.4001863486352022, -38.60401951598402803, 148.0724198280769883 ) ) ;
#26403=CARTESIAN_POINT ( 'NONE',  ( 100.9151287000745896, -46.91716693487881429, 52.14419670448194921 ) ) ;
#26404=DIRECTION ( 'NONE',  ( -0.000000000000000000, -0.000000000000000000, 1.000000000000000000 ) ) ;
#26406=ADVANCED_FACE ( 'NONE', ( #61682 ), #68070, .T. ) ;
#26408=AXIS2_PLACEMENT_3D ( 'NONE', #50539, #78281, #9225 ) ;
#26409=ORIENTED_EDGE ( 'NONE', *, *, #64862, .T. ) ;
#26410=ADVANCED_FACE ( 'NONE', ( #33542 ), #34432, .T. ) ;
#26411=ADVANCED_FACE ( 'NONE', ( #68966 ), #62142, .F. ) ;
#26413=VECTOR ( 'NONE', #45665, 1000.000000000000000 ) ;
#26417=CARTESIAN_POINT ( 'NONE',  ( 110.9845004553952208, -45.93008197751423438, 132.8968334499706145 ) ) ;
#26418=EDGE_CURVE ( 'NONE', #17652, #31120, #48481, .T. ) ;
#26420=VERTEX_POINT ( 'NONE', #81275 ) ;
#26421=CARTESIAN_POINT ( 'NONE',  ( 96.63682800883232460, -32.99879952304045361, 26.06514908543494613 ) ) ;
#26422=CARTESIAN_POINT ( 'NONE',  ( 97.58291127976856671, -32.21282489450084086, 71.97276813305397525 ) ) ;
#26423=EDGE_CURVE ( 'NONE', #52268, #78030, #85622, .T. ) ;
#26426=CARTESIAN_POINT ( 'NONE',  ( 63.03715912545644784, -24.42818131006017168, 117.4678068554150485 ) ) ;
#26427=DIRECTION ( 'NONE',  ( 0.000000000000000000, 0.000000000000000000, 1.000000000000000000 ) ) ;
#26428=CARTESIAN_POINT ( 'NONE',  ( 188.5667039024479834, -62.87844715994099687, 173.2178068554149775 ) ) ;
#26432=ORIENTED_EDGE ( 'NONE', *, *, #48011, .F. ) ;
#26433=CARTESIAN_POINT ( 'NONE',  ( 97.73303842741869119, -31.98671872394393034, 50.95276813305294183 ) ) ;
#26434=CARTESIAN_POINT ( 'NONE',  ( 116.9955931624231624, -33.48136526131695234, 85.07848241876791917 ) ) ;
#26436=CARTESIAN_POINT ( 'NONE',  ( 101.9941904926150613, -45.44642369002148286, 172.1539441930640635 ) ) ;
#26437=DIRECTION ( 'NONE',  ( -6.524622321627019585E-16, -3.741823817616790462E-31, -1.000000000000000000 ) ) ;
#26438=CARTESIAN_POINT ( 'NONE',  ( 31.71315051186932621, -31.94127993907824958, 342.9256252759109884 ) ) ;
#26440=ORIENTED_EDGE ( 'NONE', *, *, #39337, .F. ) ;
#26441=CARTESIAN_POINT ( 'NONE',  ( 103.5913876162975953, -46.49993820617270757, 98.31657765686297523 ) ) ;
#26443=EDGE_LOOP ( 'NONE', ( #24031, #34413, #10209, #45027 ) ) ;
#26444=CARTESIAN_POINT ( 'NONE',  ( 115.8368392028493190, -44.66223131803943858, 229.2413395616249545 ) ) ;
#26445=CARTESIAN_POINT ( 'NONE',  ( 116.3136297247243078, -32.94478793390952376, 255.1356252759109395 ) ) ;
#26446=CARTESIAN_POINT ( 'NONE',  ( 29.56670390244797630, -48.82844715994099971, 310.9178068554150514 ) ) ;
#26447=DIRECTION ( 'NONE',  ( -6.831565154159360295E-14, 1.000000000000000000, 0.000000000000000000 ) ) ;
#26448=CARTESIAN_POINT ( 'NONE',  ( 115.8254323924586231, -31.73001883007492552, 80.23979194246547308 ) ) ;
#26449=VECTOR ( 'NONE', #35282, 1000.000000000000000 ) ;
#26450=EDGE_CURVE ( 'NONE', #8036, #28811, #35323, .T. ) ;
#26451=CARTESIAN_POINT ( 'NONE',  ( 131.5867845949876198, -37.92005462650919156, 2.747931806398446586 ) ) ;
#26452=CARTESIAN_POINT ( 'NONE',  ( 25.56670390244744695, -48.82844715994178841, 173.2178068554150627 ) ) ;
#26453=EDGE_CURVE ( 'NONE', #87386, #25446, #42136, .T. ) ;
#26454=CARTESIAN_POINT ( 'NONE',  ( 102.9544237342423969, -27.85507949283293527, 180.4213395616259845 ) ) ;
#26457=CARTESIAN_POINT ( 'NONE',  ( 116.0270257299131487, -33.90363670229466919, 125.4892023535159638 ) ) ;
#26458=VECTOR ( 'NONE', #13887, 1000.000000000000000 ) ;
#26460=CARTESIAN_POINT ( 'NONE',  ( 100.6033219294153724, -44.83909144599376617, 268.0289586092438867 ) ) ;
#26463=AXIS2_PLACEMENT_3D ( 'NONE', #6640, #76124, #39367 ) ;
#26466=CARTESIAN_POINT ( 'NONE',  ( 164.9667039024459996, -26.71338133339301635, -5.074374724088000832 ) ) ;
#26468=CARTESIAN_POINT ( 'NONE',  ( 117.4654710391980217, -40.40706546494233464, 178.5680062282919778 ) ) ;
#26469=CARTESIAN_POINT ( 'NONE',  ( 115.0900420730608147, -30.61910110487549019, 169.3437578978403337 ) ) ;
#26470=ORIENTED_EDGE ( 'NONE', *, *, #39941, .T. ) ;
#26471=EDGE_LOOP ( 'NONE', ( #33693, #5255, #15069, #22026 ) ) ;
#26473=CARTESIAN_POINT ( 'NONE',  ( 77.59184326793636899, -17.51852171451485063, 2.740177351661285954 ) ) ;
#26474=DIRECTION ( 'NONE',  ( 4.299999999999999979E-14, -1.000000000000000000, 4.400000000000000367E-29 ) ) ;
#26475=DIRECTION ( 'NONE',  ( 0.02150753337723862457, 0.0009076677972192722819, 0.9997682742251809973 ) ) ;
#26476=DIRECTION ( 'NONE',  ( 0.000000000000000000, 1.000000000000000000, 0.000000000000000000 ) ) ;
#26477=VERTEX_POINT ( 'NONE', #8538 ) ;
#26479=CARTESIAN_POINT ( 'NONE',  ( 115.3881169701508327, -30.44952332473371115, 219.3413395616249773 ) ) ;
#26481=CIRCLE ( 'NONE', #43863, 16.00000000000000000 ) ;
#26483=DIRECTION ( 'NONE',  ( 1.000000000000000078E-15, 0.000000000000000000, -1.000000000000000000 ) ) ;
#26484=CARTESIAN_POINT ( 'NONE',  ( 98.30750600249929505, -41.72880667514048980, 162.7397860246828714 ) ) ;
#26485=CARTESIAN_POINT ( 'NONE',  ( 101.5184502652259084, -42.71685524349225460, 44.79951894101996857 ) ) ;
#26486=CARTESIAN_POINT ( 'NONE',  ( 117.7011894673193382, -39.82593390098057284, 134.5889586092439743 ) ) ;
#26487=CARTESIAN_POINT ( 'NONE',  ( 172.5664832912740110, -32.07844715994070839, 14.17562527591199917 ) ) ;
#26488=EDGE_LOOP ( 'NONE', ( #54926, #44763, #31465, #37856 ) ) ;
#26489=DIRECTION ( 'NONE',  ( 1.000000000000000078E-15, 1.000000000000000083E-30, -1.000000000000000000 ) ) ;
#26490=EDGE_CURVE ( 'NONE', #6493, #45463, #15803, .T. ) ;
#26491=CARTESIAN_POINT ( 'NONE',  ( 100.7388752691453391, -44.57574992080446918, 67.03815598159052058 ) ) ;
#26492=VERTEX_POINT ( 'NONE', #2171 ) ;
#26493=VERTEX_POINT ( 'NONE', #1726 ) ;
#26494=AXIS2_PLACEMENT_3D ( 'NONE', #45893, #32734, #82257 ) ;
#26495=B_SPLINE_CURVE_WITH_KNOTS ( 'NONE', 3,
 ( #4104, #31804, #64999, #50459, #43645, #30035, #58178, #71383, #9148, #50912, #57728, #85469, #23246, #9588, #85908, #39517, #60847, #33600 ),
 .UNSPECIFIED., .F., .F.,
 ( 4, 2, 2, 2, 2, 2, 2, 2, 4 ),
 ( 0.000000000000000000, 0.1250000000000000000, 0.2500000000000000000, 0.3750000000000000000, 0.5000000000000000000, 0.6250000000000000000, 0.7500000000000000000, 0.8750000000000000000, 1.000000000000000000 ),
 .UNSPECIFIED. ) ;
#26496=CARTESIAN_POINT ( 'NONE',  ( 160.7738106836348777, -48.62134037874901082, 249.9678068554149490 ) ) ;
#26497=EDGE_LOOP ( 'NONE', ( #13466, #58443, #44263, #64325 ) ) ;
#26498=EDGE_LOOP ( 'NONE', ( #75004, #49737, #63763, #70702, #67026, #33976 ) ) ;
#26499=DIRECTION ( 'NONE',  ( 1.000000000000000000, 4.163336342344333240E-14, 0.000000000000000000 ) ) ;
#26500=EDGE_CURVE ( 'NONE', #20871, #44627, #78488, .T. ) ;
#26501=EDGE_CURVE ( 'NONE', #68029, #16276, #78035, .T. ) ;
#26502=CARTESIAN_POINT ( 'NONE',  ( 104.9561144943094035, -45.03597746244296474, 46.80099125664899162 ) ) ;
#26503=CARTESIAN_POINT ( 'NONE',  ( 96.78703652860848194, -40.85599721901744630, 251.6422919425777138 ) ) ;
#26504=EDGE_CURVE ( 'NONE', #34907, #71626, #15972, .T. ) ;
#26505=CARTESIAN_POINT ( 'NONE',  ( 108.8451227504523331, -46.97957433935484772, 167.7127681330539701 ) ) ;
#26506=DIRECTION ( 'NONE',  ( 0.000000000000000000, 0.000000000000000000, 1.000000000000000000 ) ) ;
#26507=CARTESIAN_POINT ( 'NONE',  ( 111.4063510358307241, -46.18429848020799255, 23.91848241876792969 ) ) ;
#26508=CARTESIAN_POINT ( 'NONE',  ( 32.06670390244800473, -33.35206098992711077, -5.074374724088000832 ) ) ;
#26509=CARTESIAN_POINT ( 'NONE',  ( 71.06648329127399677, -18.82844715994099971, 17.92562527591199739 ) ) ;
#26511=EDGE_LOOP ( 'NONE', ( #23880, #84669 ) ) ;
#26512=EDGE_CURVE ( 'NONE', #42491, #66495, #14909, .T. ) ;
#26513=CIRCLE ( 'NONE', #84578, 4.750000000000004441 ) ;
#26515=CARTESIAN_POINT ( 'NONE',  ( 100.7967938542458199, -45.88935316334050185, 242.1108633711489517 ) ) ;
#26517=CARTESIAN_POINT ( 'NONE',  ( 110.6963687344609184, -48.01060035924083280, 207.8241967044819489 ) ) ;
#26518=DIRECTION ( 'NONE',  ( 0.000000000000000000, 0.000000000000000000, -1.000000000000000000 ) ) ;
#26521=CARTESIAN_POINT ( 'NONE',  ( 117.0885360161528439, -37.77856303987432796, 29.74381011534493524 ) ) ;
#26522=CARTESIAN_POINT ( 'NONE',  ( 99.08811452206278148, -33.58219759109908864, 277.6356252759111385 ) ) ;
#26523=DIRECTION ( 'NONE',  ( -4.237773401492740281E-14, 1.000000000000000000, 0.000000000000000000 ) ) ;
#26525=DIRECTION ( 'NONE',  ( 1.000000000000000000, 4.299999999999999979E-14, 1.000000000000000078E-15 ) ) ;
#26528=DIRECTION ( 'NONE',  ( 0.000000000000000000, 1.000000000000000000, 0.000000000000000000 ) ) ;
#26529=DIRECTION ( 'NONE',  ( 0.7071067811571474238, 0.7071067812159476107, 0.000000000000000000 ) ) ;
#26530=CARTESIAN_POINT ( 'NONE',  ( 99.09330906164119313, -30.55363432604262286, 40.80189661388796196 ) ) ;
#26531=CARTESIAN_POINT ( 'NONE',  ( 113.2454987006837968, -28.75867294695902743, 75.55229194230558676 ) ) ;
#26533=CARTESIAN_POINT ( 'NONE',  ( 100.8523774812658900, -29.53301242784285563, 195.5838068554162135 ) ) ;
#26536=CARTESIAN_POINT ( 'NONE',  ( 98.82177599387378564, -29.33213395062421469, 235.7565776568629872 ) ) ;
#26537=CARTESIAN_POINT ( 'NONE',  ( 111.0825168487035626, -25.58018305758348632, 95.80133956162495679 ) ) ;
#26538=CARTESIAN_POINT ( 'NONE',  ( 99.50795136241276850, -29.43516104912357179, 246.7156252759109520 ) ) ;
#26540=DIRECTION ( 'NONE',  ( 1.000000000000000000, 4.299999999999999979E-14, 1.000000000000000078E-15 ) ) ;
#26543=FACE_OUTER_BOUND ( 'NONE', #32893, .T. ) ;
#26544=CARTESIAN_POINT ( 'NONE',  ( 131.7155263566516226, -20.16021090639161528, 2.608895778942307508 ) ) ;
#26546=ORIENTED_EDGE ( 'NONE', *, *, #35732, .T. ) ;
#26547=CARTESIAN_POINT ( 'NONE',  ( 115.2323353771322445, -31.47685829367418009, 143.7038483995059721 ) ) ;
#26551=LINE ( 'NONE', #25654, #27177 ) ;
#26552=CARTESIAN_POINT ( 'NONE',  ( 99.70004787478436015, -45.98060041612298221, 118.0413395616259606 ) ) ;
#26553=DIRECTION ( 'NONE',  ( 0.000000000000000000, 0.000000000000000000, -1.000000000000000000 ) ) ;
#26554=CARTESIAN_POINT ( 'NONE',  ( 165.2748236753140247, -30.08671355700301575, -5.074374724088000832 ) ) ;
#26557=EDGE_CURVE ( 'NONE', #40401, #86883, #58939, .T. ) ;
#26558=CARTESIAN_POINT ( 'NONE',  ( 97.58158007118568378, -32.53714515026960896, 55.98324432352996638 ) ) ;
#26559=ORIENTED_EDGE ( 'NONE', *, *, #77893, .T. ) ;
#26560=EDGE_LOOP ( 'NONE', ( #9479, #34759, #68245, #79405 ) ) ;
#26561=ORIENTED_EDGE ( 'NONE', *, *, #6017, .F. ) ;
#26562=VECTOR ( 'NONE', #24773, 999.9999999999998863 ) ;
#26564=CARTESIAN_POINT ( 'NONE',  ( 97.98063455390173715, -41.72806076336409120, 172.7146728949579710 ) ) ;
#26565=DIRECTION ( 'NONE',  ( 0.7071067811865473507, 0.000000000000000000, -0.7071067811865476838 ) ) ;
#26566=DIRECTION ( 'NONE',  ( 0.000000000000000000, 0.000000000000000000, 1.000000000000000000 ) ) ;
#26567=CARTESIAN_POINT ( 'NONE',  ( 172.5664832912729878, -27.82844715994070484, 194.1756252759119832 ) ) ;
#26568=LINE ( 'NONE', #47887, #43064 ) ;
#26569=LINE ( 'NONE', #54694, #12967 ) ;
#26571=CARTESIAN_POINT ( 'NONE',  ( 108.9812119692459049, -46.95502683147942236, 82.72419670448194040 ) ) ;
#26572=VERTEX_POINT ( 'NONE', #16691 ) ;
#26573=VERTEX_POINT ( 'NONE', #2620 ) ;
#26576=DIRECTION ( 'NONE',  ( 0.000000000000000000, 0.000000000000000000, 1.000000000000000000 ) ) ;
#26579=CARTESIAN_POINT ( 'NONE',  ( 104.4487311862825578, -28.48030787377049577, 203.1271379886389639 ) ) ;
#26582=AXIS2_PLACEMENT_3D ( 'NONE', #82728, #37, #83171 ) ;
#26584=ORIENTED_EDGE ( 'NONE', *, *, #89380, .T. ) ;
#26585=ORIENTED_EDGE ( 'NONE', *, *, #2430, .T. ) ;
#26587=CARTESIAN_POINT ( 'NONE',  ( 80.06648329127399677, -8.729447159940999512, 308.6356252759119911 ) ) ;
#26589=VERTEX_POINT ( 'NONE', #38901 ) ;
#26592=CARTESIAN_POINT ( 'NONE',  ( 98.85146132857330770, -40.05235142642286661, 203.0644404487539703 ) ) ;
#26593=DIRECTION ( 'NONE',  ( 1.000000000000000078E-15, -1.000000000000000083E-30, -1.000000000000000000 ) ) ;
#26595=ORIENTED_EDGE ( 'NONE', *, *, #51403, .T. ) ;
#26596=ORIENTED_EDGE ( 'NONE', *, *, #28995, .F. ) ;
#26598=VECTOR ( 'NONE', #81316, 1000.000000000000000 ) ;
#26599=ORIENTED_EDGE ( 'NONE', *, *, #81399, .T. ) ;
#26600=ORIENTED_EDGE ( 'NONE', *, *, #89227, .F. ) ;
#26601=ADVANCED_FACE ( 'NONE', ( #9877 ), #45696, .T. ) ;
#26603=CARTESIAN_POINT ( 'NONE',  ( 104.9194883499490061, -28.34545421100826346, 243.1061856076869958 ) ) ;
#26605=CARTESIAN_POINT ( 'NONE',  ( 96.67713595657845360, -37.82845849995531040, 126.4099109901969626 ) ) ;
#26606=EDGE_CURVE ( 'NONE', #42662, #84235, #30323, .T. ) ;
#26607=CARTESIAN_POINT ( 'NONE',  ( 97.64212626138829876, -32.24102647341085515, 75.97276813305397525 ) ) ;
#26608=CARTESIAN_POINT ( 'NONE',  ( 114.1404429899671555, -42.27958953989512025, 249.5838068554168672 ) ) ;
#26609=CARTESIAN_POINT ( 'NONE',  ( 131.3165190107488627, -18.55810522839977139, 6.749822759740949252 ) ) ;
#26610=CARTESIAN_POINT ( 'NONE',  ( 105.8259002483207922, -25.33766151058717142, 321.6188579224977389 ) ) ;
#26611=CARTESIAN_POINT ( 'NONE',  ( 96.19138854833354912, -32.02127024200479610, 207.0013395616249738 ) ) ;
#26612=PLANE ( 'NONE',  #23388 ) ;
#26613=ORIENTED_EDGE ( 'NONE', *, *, #65535, .T. ) ;
#26614=CARTESIAN_POINT ( 'NONE',  ( 168.0371591254543944, -48.62818131005519717, 249.9678068554149775 ) ) ;
#26615=ORIENTED_EDGE ( 'NONE', *, *, #86119, .T. ) ;
#26616=EDGE_CURVE ( 'NONE', #73652, #27672, #17140, .T. ) ;
#26617=VERTEX_POINT ( 'NONE', #44373 ) ;
#26618=CARTESIAN_POINT ( 'NONE',  ( 71.24189083761808661, -0.9290567490904538817, 540.9756252759101471 ) ) ;
#26619=VERTEX_POINT ( 'NONE', #23956 ) ;
#26620=AXIS2_PLACEMENT_3D ( 'NONE', #33954, #89849, #5829 ) ;
#26622=CARTESIAN_POINT ( 'NONE',  ( 193.0371591254586576, -47.82818131005411999, 129.9678068554150343 ) ) ;
#26623=CARTESIAN_POINT ( 'NONE',  ( 117.8755673099929453, -39.04089478637848032, 108.6708633711489824 ) ) ;
#26625=CARTESIAN_POINT ( 'NONE',  ( 136.7925547069167749, -36.36732994130177588, 6.785344856283919590 ) ) ;
#26626=CARTESIAN_POINT ( 'NONE',  ( 150.5667039024476139, -25.42844715993593852, 129.9678068554149775 ) ) ;
#26627=CARTESIAN_POINT ( 'NONE',  ( 116.8171228667634125, -34.15291832121570792, 145.0314586091961928 ) ) ;
#26629=CARTESIAN_POINT ( 'NONE',  ( 100.6697571656888499, -44.93374849542860971, 228.0499109901969348 ) ) ;
#26631=DIRECTION ( 'NONE',  ( 2.056463827196271584E-15, -0.8571673007021100021, 0.5150380749100580413 ) ) ;
#26635=LINE ( 'NONE', #19827, #47112 ) ;
#26636=CYLINDRICAL_SURFACE ( 'NONE', #37179, 10.00000000000000355 ) ;
#26637=DIRECTION ( 'NONE',  ( -1.000000000000000000, -3.999999999999999995E-14, -1.000000000000000078E-15 ) ) ;
#26638=CARTESIAN_POINT ( 'NONE',  ( 116.6462162596975389, -40.95264290462791479, 253.4956252759109532 ) ) ;
#26639=VERTEX_POINT ( 'NONE', #86628 ) ;
#26640=CARTESIAN_POINT ( 'NONE',  ( 110.4848523211437339, -27.30132240271888122, 194.7993133264554046 ) ) ;
#26641=CARTESIAN_POINT ( 'NONE',  ( 96.34427168469159142, -39.41376207380771746, 12.53372051400597442 ) ) ;
#26642=CARTESIAN_POINT ( 'NONE',  ( 108.6553284749260229, -25.75107874774626993, 145.9737205140069420 ) ) ;
#26644=CARTESIAN_POINT ( 'NONE',  ( 108.4175022753835691, -26.73504371419085501, 100.9690269479842613 ) ) ;
#26646=DIRECTION ( 'NONE',  ( 0.000000000000000000, 0.000000000000000000, -1.000000000000000000 ) ) ;
#26648=LINE ( 'NONE', #68445, #65592 ) ;
#26650=VECTOR ( 'NONE', #67972, 1000.000000000000000 ) ;
#26651=AXIS2_PLACEMENT_3D ( 'NONE', #46811, #61348, #89077 ) ;
#26652=ORIENTED_EDGE ( 'NONE', *, *, #85815, .T. ) ;
#26654=ORIENTED_EDGE ( 'NONE', *, *, #38191, .T. ) ;
#26655=CARTESIAN_POINT ( 'NONE',  ( 172.5664832912740110, -9.303447159940999356, 261.0426252759119734 ) ) ;
#26656=CARTESIAN_POINT ( 'NONE',  ( 99.14404768239424470, -44.40400490628089614, 37.95086337114900488 ) ) ;
#26658=CARTESIAN_POINT ( 'NONE',  ( 162.5667039024460223, -19.82844715994111340, -5.074374724088000832 ) ) ;
#26659=CARTESIAN_POINT ( 'NONE',  ( 131.0667039024480118, -67.87844715994100397, 207.5838068554149913 ) ) ;
#26660=EDGE_CURVE ( 'NONE', #32398, #85160, #81825, .T. ) ;
#26661=CARTESIAN_POINT ( 'NONE',  ( 111.5095219758393483, -44.62071306430618023, 257.4190864947434534 ) ) ;
#26662=ORIENTED_EDGE ( 'NONE', *, *, #87246, .F. ) ;
#26666=CARTESIAN_POINT ( 'NONE',  ( 128.2586590417343189, -60.54728653293321372, 361.9756252759100903 ) ) ;
#26667=VECTOR ( 'NONE', #41613, 1000.000000000000000 ) ;
#26668=CARTESIAN_POINT ( 'NONE',  ( 99.08985340457110169, -42.79589214074761117, 101.8442426276604493 ) ) ;
#26669=EDGE_CURVE ( 'NONE', #14785, #56383, #83916, .T. ) ;
#26670=CARTESIAN_POINT ( 'NONE',  ( 107.0664832912750057, -36.72944715993903486, 9.125625275910969947 ) ) ;
#26671=CARTESIAN_POINT ( 'NONE',  ( 107.0664832912739399, -36.72944715994095333, 312.6356252759112522 ) ) ;
#26673=VECTOR ( 'NONE', #72924, 1000.000000000000000 ) ;
#26675=CARTESIAN_POINT ( 'NONE',  ( 104.9788083641148688, -27.14010996210884485, 260.2470538473402826 ) ) ;
#26678=CARTESIAN_POINT ( 'NONE',  ( 97.81168895331838087, -40.51742574516882200, 287.6356252759109680 ) ) ;
#26679=CYLINDRICAL_SURFACE ( 'NONE', #10498, 3.000000000000002665 ) ;
#26680=CARTESIAN_POINT ( 'NONE',  ( 114.2426363300227763, -32.83938885940727204, 67.03951894101994924 ) ) ;
#26682=CARTESIAN_POINT ( 'NONE',  ( 97.79834864326036836, -40.48469191151001922, 131.6328120007984808 ) ) ;
#26684=CARTESIAN_POINT ( 'NONE',  ( 97.81021718220807770, -40.51802218317752846, 192.6354414398782353 ) ) ;
#26686=CARTESIAN_POINT ( 'NONE',  ( 78.15700282949505606, -34.74831852143766042, 7.618261863062902428 ) ) ;
#26688=CARTESIAN_POINT ( 'NONE',  ( 117.1261863205049423, -33.86823216992616636, 149.0470538473389581 ) ) ;
#26689=VERTEX_POINT ( 'NONE', #60682 ) ;
#26691=CARTESIAN_POINT ( 'NONE',  ( 115.6883067454668463, -38.90345035940969609, 120.0615833058969457 ) ) ;
#26692=LINE ( 'NONE', #81247, #56056 ) ;
#26694=CARTESIAN_POINT ( 'NONE',  ( 97.26802889450139844, -33.10625101732204456, 62.04419670448196911 ) ) ;
#26695=CARTESIAN_POINT ( 'NONE',  ( 31.71315051185399270, -33.70561438052121161, 117.4678068554150485 ) ) ;
#26696=CARTESIAN_POINT ( 'NONE',  ( 163.0664832912739826, 0.2215528400590083269, 333.4006252759110112 ) ) ;
#26697=VERTEX_POINT ( 'NONE', #26622 ) ;
#26705=CARTESIAN_POINT ( 'NONE',  ( 107.4826147187165333, -46.50135945624624156, 237.6099109901969655 ) ) ;
#26706=CARTESIAN_POINT ( 'NONE',  ( 114.5431187036783740, -28.56067750227894564, 150.4746728949579619 ) ) ;
#26708=LINE ( 'NONE', #54842, #43108 ) ;
#26710=CARTESIAN_POINT ( 'NONE',  ( 107.6031410145815528, -26.28275719304336633, 91.03562527591097364 ) ) ;
#26711=CARTESIAN_POINT ( 'NONE',  ( 100.9563739204374855, -28.70569515775407510, 96.59303380014206653 ) ) ;
#26712=ORIENTED_EDGE ( 'NONE', *, *, #82036, .T. ) ;
#26713=DIRECTION ( 'NONE',  ( 0.7071067811868687603, 0.7071067811862262742, 7.071067811868681067E-16 ) ) ;
#26715=CARTESIAN_POINT ( 'NONE',  ( 41.56648329127398966, -18.82844715994071194, 318.9256252759120116 ) ) ;
#26716=EDGE_LOOP ( 'NONE', ( #29750, #69022 ) ) ;
#26719=AXIS2_PLACEMENT_3D ( 'NONE', #70228, #43400, #78410 ) ;
#26720=VECTOR ( 'NONE', #88672, 1000.000000000000000 ) ;
#26722=CARTESIAN_POINT ( 'NONE',  ( 100.0388059118472341, -29.01104360887432776, 285.6641967044823787 ) ) ;
#26723=CARTESIAN_POINT ( 'NONE',  ( 34.27482367531500529, -30.08671355700301575, 342.9256252759119548 ) ) ;
#26726=LINE ( 'NONE', #54409, #35991 ) ;
#26727=CARTESIAN_POINT ( 'NONE',  ( 100.9534786964907482, -28.35269599622599301, 30.56610146638794134 ) ) ;
#26728=DIRECTION ( 'NONE',  ( 0.000000000000000000, 0.000000000000000000, 1.000000000000000000 ) ) ;
#26729=CARTESIAN_POINT ( 'NONE',  ( 109.2504006710444173, -46.93703897017532967, 103.7441967044829880 ) ) ;
#26730=DIRECTION ( 'NONE',  ( 0.000000000000000000, 0.000000000000000000, -1.000000000000000000 ) ) ;
#26731=CARTESIAN_POINT ( 'NONE',  ( 98.82181093208917844, -30.27703119756231942, 155.7984824187679465 ) ) ;
#26735=ORIENTED_EDGE ( 'NONE', *, *, #71354, .T. ) ;
#26738=AXIS2_PLACEMENT_3D ( 'NONE', #54121, #11928, #12834 ) ;
#26739=PLANE ( 'NONE',  #60968 ) ;
#26740=EDGE_CURVE ( 'NONE', #3336, #48583, #17450, .T. ) ;
#26741=CARTESIAN_POINT ( 'NONE',  ( 136.4599941731065655, -35.37149686612711719, 2.653088969733340630 ) ) ;
#26742=VERTEX_POINT ( 'NONE', #18459 ) ;
#26743=CARTESIAN_POINT ( 'NONE',  ( 97.31571814629074879, -39.30557183317851155, 62.53186119129362908 ) ) ;
#26744=CARTESIAN_POINT ( 'NONE',  ( 96.56283406263658264, -36.88802528585984675, 136.3384824187679385 ) ) ;
#26745=ORIENTED_EDGE ( 'NONE', *, *, #56837, .T. ) ;
#26746=CARTESIAN_POINT ( 'NONE',  ( 41.56648329127499153, -32.07844715994070839, 323.6756252759119548 ) ) ;
#26748=DIRECTION ( 'NONE',  ( 0.000000000000000000, 1.000000000000000000, 0.000000000000000000 ) ) ;
#26750=ORIENTED_EDGE ( 'NONE', *, *, #5196, .T. ) ;
#26752=ORIENTED_EDGE ( 'NONE', *, *, #33842, .T. ) ;
#26754=EDGE_LOOP ( 'NONE', ( #28495, #84375, #31267, #86075 ) ) ;
#26757=CARTESIAN_POINT ( 'NONE',  ( 115.7831076504716634, -41.80230954540643040, 158.4064586060680995 ) ) ;
#26758=DIRECTION ( 'NONE',  ( -0.9254794337955620787, -0.3787978585227822492, 0.000000000000000000 ) ) ;
#26759=CARTESIAN_POINT ( 'NONE',  ( 80.06648329127402519, -46.72944715994105991, 8.225625275910942946 ) ) ;
#26761=CARTESIAN_POINT ( 'NONE',  ( 97.81061268084424398, -40.51479618546458994, 181.6353987547717566 ) ) ;
#26763=ORIENTED_EDGE ( 'NONE', *, *, #7536, .F. ) ;
#26764=AXIS2_PLACEMENT_3D ( 'NONE', #24537, #52201, #45397 ) ;
#26765=VERTEX_POINT ( 'NONE', #42353 ) ;
#26766=DIRECTION ( 'NONE',  ( 4.299999999999999979E-14, -1.000000000000000000, 4.400000000000000367E-29 ) ) ;
#26767=VECTOR ( 'NONE', #73440, 1000.000000000000000 ) ;
#26768=DIRECTION ( 'NONE',  ( -4.237773401492740281E-14, 1.000000000000000000, 0.000000000000000000 ) ) ;
#26769=EDGE_CURVE ( 'NONE', #7132, #78594, #82701, .T. ) ;
#26770=CARTESIAN_POINT ( 'NONE',  ( 114.9950743857440756, -30.04541929558971702, 220.3718157521009573 ) ) ;
#26773=CARTESIAN_POINT ( 'NONE',  ( 104.2906771502716055, -46.10805769451163627, 103.3470538473389411 ) ) ;
#26774=CARTESIAN_POINT ( 'NONE',  ( 111.4697974980132642, -45.71384261549509631, 52.93909454086460187 ) ) ;
#26778=LINE ( 'NONE', #27684, #26921 ) ;
#26779=ORIENTED_EDGE ( 'NONE', *, *, #18893, .F. ) ;
#26780=ORIENTED_EDGE ( 'NONE', *, *, #52510, .F. ) ;
#26781=CARTESIAN_POINT ( 'NONE',  ( 97.77711562652216060, -35.32084007268648662, 217.6263452106589682 ) ) ;
#26783=CARTESIAN_POINT ( 'NONE',  ( 98.04129441745654105, -41.04138963897023018, 52.68073796447941248 ) ) ;
#26785=CIRCLE ( 'NONE', #2110, 2.750000000000002665 ) ;
#26788=CIRCLE ( 'NONE', #13703, 0.5000000000000004441 ) ;
#26789=DIRECTION ( 'NONE',  ( 0.000000000000000000, 0.000000000000000000, -1.000000000000000000 ) ) ;
#26790=CARTESIAN_POINT ( 'NONE',  ( 82.81651833456541567, -36.90056224776740379, 3.101534470965026546 ) ) ;
#26791=AXIS2_PLACEMENT_3D ( 'NONE', #5190, #67858, #61034 ) ;
#26795=CARTESIAN_POINT ( 'NONE',  ( 97.81168895331838087, -40.51742574516882200, 287.6356252759109680 ) ) ;
#26796=EDGE_LOOP ( 'NONE', ( #87390, #80934, #1812, #55235, #14835 ) ) ;
#26797=CARTESIAN_POINT ( 'NONE',  ( 101.9604343285081569, -27.64015156285208974, 60.48419670448296159 ) ) ;
#26799=CARTESIAN_POINT ( 'NONE',  ( 113.8860208566381544, -32.24350986527421981, 252.1080903695913662 ) ) ;
#26802=CARTESIAN_POINT ( 'NONE',  ( 116.5042510202519708, -34.04512512578503447, 149.0470538473399529 ) ) ;
#26804=FACE_OUTER_BOUND ( 'NONE', #59467, .T. ) ;
#26805=CARTESIAN_POINT ( 'NONE',  ( 46.83715912545337545, -47.82818131006086304, 193.9678068554150911 ) ) ;
#26806=DIRECTION ( 'NONE',  ( 0.000000000000000000, 0.000000000000000000, -1.000000000000000000 ) ) ;
#26807=CARTESIAN_POINT ( 'NONE',  ( 98.86476787746175887, -29.25085353348518424, 226.7261014663869503 ) ) ;
#26808=CARTESIAN_POINT ( 'NONE',  ( 193.0371591254572934, -23.42818131005412496, 249.9678068554149775 ) ) ;
#26809=ORIENTED_EDGE ( 'NONE', *, *, #22981, .T. ) ;
#26810=CARTESIAN_POINT ( 'NONE',  ( 97.58291127976856671, -32.21282489450084086, 71.97276813305397525 ) ) ;
#26811=DIRECTION ( 'NONE',  ( -4.237773401492740281E-14, 1.000000000000000000, 0.000000000000000000 ) ) ;
#26813=ORIENTED_EDGE ( 'NONE', *, *, #11337, .F. ) ;
#26815=ORIENTED_EDGE ( 'NONE', *, *, #77509, .T. ) ;
#26817=DIRECTION ( 'NONE',  ( 0.7071067811575828532, -0.7071067812155121812, 0.000000000000000000 ) ) ;
#26822=CARTESIAN_POINT ( 'NONE',  ( 98.33113000137380766, -33.60062404821446336, 173.8709475124489359 ) ) ;
#26823=CARTESIAN_POINT ( 'NONE',  ( 101.0741685120301412, -45.28686133165523131, 278.0899109901965858 ) ) ;
#26827=DIRECTION ( 'NONE',  ( -0.000000000000000000, 1.000000000000000000, 0.000000000000000000 ) ) ;
#26829=ORIENTED_EDGE ( 'NONE', *, *, #25781, .F. ) ;
#26831=DIRECTION ( 'NONE',  ( 0.000000000000000000, 0.000000000000000000, 1.000000000000000000 ) ) ;
#26833=ORIENTED_EDGE ( 'NONE', *, *, #52348, .F. ) ;
#26839=CARTESIAN_POINT ( 'NONE',  ( 104.3962608544918993, -28.61612207615715775, 164.7524198280769667 ) ) ;
#26840=CARTESIAN_POINT ( 'NONE',  ( 101.1165878437261227, -28.07204926635110098, 50.55562527591095545 ) ) ;
#26841=EDGE_CURVE ( 'NONE', #43365, #2670, #2933, .T. ) ;
#26844=CARTESIAN_POINT ( 'NONE',  ( 184.5667039024483813, -48.82844715993448403, 249.9678068554149775 ) ) ;
#26845=ORIENTED_EDGE ( 'NONE', *, *, #72456, .T. ) ;
#26846=ADVANCED_FACE ( 'NONE', ( #29643 ), #22391, .F. ) ;
#26850=EDGE_CURVE ( 'NONE', #23101, #30005, #9648, .T. ) ;
#26852=CARTESIAN_POINT ( 'NONE',  ( 110.8867401108072812, -45.97098272926901785, 132.8884009179573695 ) ) ;
#26853=DIRECTION ( 'NONE',  ( -0.000000000000000000, 1.000000000000000000, 0.000000000000000000 ) ) ;
#26854=VECTOR ( 'NONE', #80200, 1000.000000000000000 ) ;
#26855=VERTEX_POINT ( 'NONE', #8770 ) ;
#26856=CARTESIAN_POINT ( 'NONE',  ( 116.7655018478977951, -32.84674153052576884, 54.12991099019698282 ) ) ;
#26858=CARTESIAN_POINT ( 'NONE',  ( 109.9229042994399492, -46.83780379245977343, 68.79562527591099297 ) ) ;
#26859=VECTOR ( 'NONE', #81216, 1000.000000000000000 ) ;
#26861=VECTOR ( 'NONE', #76423, 1000.000000000000000 ) ;
#26863=CARTESIAN_POINT ( 'NONE',  ( 142.8698897858160706, -0.9167816978817300289, 394.9756252759102040 ) ) ;
#26868=CARTESIAN_POINT ( 'NONE',  ( 107.0664832912739541, -36.72944715994095333, 309.2406250056037038 ) ) ;
#26873=CARTESIAN_POINT ( 'NONE',  ( 117.3602503114455402, -32.64000144215158628, 95.13943479972097350 ) ) ;
#26874=CARTESIAN_POINT ( 'NONE',  ( 97.92339844016763095, -40.78107841467939920, 171.6585333637830502 ) ) ;
#26875=DIRECTION ( 'NONE',  ( -7.723290606088049820E-15, 0.000000000000000000, -1.000000000000000000 ) ) ;
#26877=AXIS2_PLACEMENT_3D ( 'NONE', #627, #15165, #14725 ) ;
#26880=DIRECTION ( 'NONE',  ( 1.000000000000000000, 4.163336342344333240E-14, 0.000000000000000000 ) ) ;
#26881=EDGE_LOOP ( 'NONE', ( #35819, #34796 ) ) ;
#26883=CARTESIAN_POINT ( 'NONE',  ( 99.34849973496659459, -28.72665311504493246, 111.6870538473389587 ) ) ;
#26885=ORIENTED_EDGE ( 'NONE', *, *, #24377, .F. ) ;
#26886=CARTESIAN_POINT ( 'NONE',  ( 117.4695305279093986, -36.80206755349690440, 259.8213395616249386 ) ) ;
#26887=CARTESIAN_POINT ( 'NONE',  ( 142.8698897858160706, -0.9167816978817300289, 542.9756252759101471 ) ) ;
#26888=CARTESIAN_POINT ( 'NONE',  ( 111.2428885491283239, -45.81710051344609980, 147.9192755852553205 ) ) ;
#26890=CARTESIAN_POINT ( 'NONE',  ( 116.3212776292293995, -32.94146857471265122, 80.13562527591095375 ) ) ;
#26893=CARTESIAN_POINT ( 'NONE',  ( 117.1144258088630750, -31.97015794161411861, 214.1784824187679419 ) ) ;
#26894=ORIENTED_EDGE ( 'NONE', *, *, #5793, .F. ) ;
#26896=AXIS2_PLACEMENT_3D ( 'NONE', #62471, #42019, #69747 ) ;
#26897=CARTESIAN_POINT ( 'NONE',  ( 103.0256836488564716, -28.24720316769774797, 136.8739642582779652 ) ) ;
#26898=LINE ( 'NONE', #18745, #32692 ) ;
#26899=EDGE_CURVE ( 'NONE', #34034, #752, #72580, .T. ) ;
#26900=CARTESIAN_POINT ( 'NONE',  ( 116.8470136369841725, -36.79772195930840439, 259.8213395616247681 ) ) ;
#26902=AXIS2_PLACEMENT_3D ( 'NONE', #65850, #66750, #53084 ) ;
#26904=EDGE_CURVE ( 'NONE', #52724, #28401, #23741, .T. ) ;
#26906=EDGE_CURVE ( 'NONE', #86805, #81323, #88526, .T. ) ;
#26907=DIRECTION ( 'NONE',  ( 1.000000000000000078E-15, -1.000000000000000083E-30, -1.000000000000000000 ) ) ;
#26908=DIRECTION ( 'NONE',  ( 0.000000000000000000, 0.000000000000000000, -1.000000000000000000 ) ) ;
#26909=CARTESIAN_POINT ( 'NONE',  ( 31.71315051186735801, -31.94127993907786589, 193.9678068554150911 ) ) ;
#26910=CARTESIAN_POINT ( 'NONE',  ( 104.4591861284129948, -26.65816784528755790, 200.2784824187679362 ) ) ;
#26911=DIRECTION ( 'NONE',  ( 0.9254794337955621897, 0.3787978585227821382, 0.000000000000000000 ) ) ;
#26913=ORIENTED_EDGE ( 'NONE', *, *, #348, .F. ) ;
#26914=EDGE_CURVE ( 'NONE', #87649, #31858, #60950, .T. ) ;
#26915=EDGE_CURVE ( 'NONE', #39062, #62015, #72332, .T. ) ;
#26917=CARTESIAN_POINT ( 'NONE',  ( 81.91398979885782694, -20.77444411302980853, 7.664507283826766049 ) ) ;
#26918=CARTESIAN_POINT ( 'NONE',  ( 117.0715937733379093, -35.45994745709830198, 124.9267458150729482 ) ) ;
#26921=VECTOR ( 'NONE', #54463, 1000.000000000000000 ) ;
#26925=AXIS2_PLACEMENT_3D ( 'NONE', #71491, #64654, #8359 ) ;
#26927=AXIS2_PLACEMENT_3D ( 'NONE', #57394, #85137, #57847 ) ;
#26928=AXIS2_PLACEMENT_3D ( 'NONE', #29523, #36337, #16341 ) ;
#26929=EDGE_CURVE ( 'NONE', #36112, #26158, #23309, .T. ) ;
#26930=CARTESIAN_POINT ( 'NONE',  ( 106.8516092256838306, -47.78082339050276772, 227.5489586092439538 ) ) ;
#26931=VERTEX_POINT ( 'NONE', #45925 ) ;
#26932=VECTOR ( 'NONE', #50669, 1000.000000000000000 ) ;
#26933=FACE_OUTER_BOUND ( 'NONE', #17118, .T. ) ;
#26935=CARTESIAN_POINT ( 'NONE',  ( 21.03689327557615130, -23.42844715994197813, 180.4678068554150911 ) ) ;
#26936=CARTESIAN_POINT ( 'NONE',  ( 156.5667039024485518, -48.82844715993568485, 173.2178068554149775 ) ) ;
#26937=EDGE_CURVE ( 'NONE', #80043, #5970, #66780, .T. ) ;
#26938=CARTESIAN_POINT ( 'NONE',  ( 101.1433531317129280, -42.34605246296819558, 79.74809036959096886 ) ) ;
#26939=CARTESIAN_POINT ( 'NONE',  ( 117.5090302172161500, -40.42247023647522752, 174.5680062282919778 ) ) ;
#26940=AXIS2_PLACEMENT_3D ( 'NONE', #31910, #9692, #3330 ) ;
#26941=LINE ( 'NONE', #19676, #37758 ) ;
#26943=CIRCLE ( 'NONE', #6656, 10.04999999999999361 ) ;
#26945=CARTESIAN_POINT ( 'NONE',  ( 112.9065472848678127, -44.95407874994433683, 68.06887155916673748 ) ) ;
#26946=EDGE_LOOP ( 'NONE', ( #18649, #24569, #8024, #53072 ) ) ;
#26947=VERTEX_POINT ( 'NONE', #74113 ) ;
#26948=DIRECTION ( 'NONE',  ( -0.000000000000000000, 1.000000000000000000, 0.000000000000000000 ) ) ;
#26950=ORIENTED_EDGE ( 'NONE', *, *, #71550, .F. ) ;
#26953=CARTESIAN_POINT ( 'NONE',  ( 109.7600704110825802, -27.40125247274746556, 64.27527697093398729 ) ) ;
#26954=CARTESIAN_POINT ( 'NONE',  ( 98.82177599387378564, -29.33213395062421469, 235.7565776568629872 ) ) ;
#26955=EDGE_CURVE ( 'NONE', #8825, #43693, #59564, .T. ) ;
#26956=CARTESIAN_POINT ( 'NONE',  ( 113.0874441278155871, -45.97130050132146550, 223.0480062282919675 ) ) ;
#26957=CARTESIAN_POINT ( 'NONE',  ( 71.06648329127310149, -18.82844715994099971, 81.92562527591198318 ) ) ;
#26958=CARTESIAN_POINT ( 'NONE',  ( 116.7496603916996207, -31.44741115753631178, 20.21181575210195902 ) ) ;
#26960=CARTESIAN_POINT ( 'NONE',  ( 25.56670390244797275, -65.37844715994100397, 132.3428068554150343 ) ) ;
#26961=CARTESIAN_POINT ( 'NONE',  ( 117.0724591054688517, -35.46716173184821486, 94.92691977030953865 ) ) ;
#26962=ADVANCED_FACE ( 'NONE', ( #32772 ), #52728, .F. ) ;
#26963=VERTEX_POINT ( 'NONE', #81405 ) ;
#26964=ORIENTED_EDGE ( 'NONE', *, *, #83725, .T. ) ;
#26965=EDGE_CURVE ( 'NONE', #64372, #62172, #23313, .T. ) ;
#26966=CARTESIAN_POINT ( 'NONE',  ( 99.11394507416765975, -43.38496525699394368, 71.86895860924497015 ) ) ;
#26967=CARTESIAN_POINT ( 'NONE',  ( 100.2700262342886219, -46.49863182355969116, 87.09276813305393716 ) ) ;
#26968=CARTESIAN_POINT ( 'NONE',  ( 96.93601811142059432, -39.37148068186442629, 276.5299109901966403 ) ) ;
#26970=CARTESIAN_POINT ( 'NONE',  ( 109.3585227812971539, -25.91623105973918939, 184.9222919425779708 ) ) ;
#26971=CARTESIAN_POINT ( 'NONE',  ( 109.7248658851862047, -27.00080516916434092, 34.86479194556028460 ) ) ;
#26972=CIRCLE ( 'NONE', #66118, 2.117000000000000881 ) ;
#26973=CYLINDRICAL_SURFACE ( 'NONE', #23333, 2.750000000000002665 ) ;
#26974=CARTESIAN_POINT ( 'NONE',  ( 20.03715912545732891, -24.95799193693189721, 300.4678068554150059 ) ) ;
#26975=DIRECTION ( 'NONE',  ( 1.000000000000000000, 4.272717921125146745E-14, 0.000000000000000000 ) ) ;
#26976=CARTESIAN_POINT ( 'NONE',  ( 109.6970437850230979, -45.56375468492142744, 277.6356252759109680 ) ) ;
#26977=CARTESIAN_POINT ( 'NONE',  ( 107.0664832912739399, -36.72944715994095333, 315.1356252759112522 ) ) ;
#26980=DIRECTION ( 'NONE',  ( -1.000000000000000078E-15, 1.000000000000000083E-30, 1.000000000000000000 ) ) ;
#26981=DIRECTION ( 'NONE',  ( 0.000000000000000000, 0.000000000000000000, -1.000000000000000000 ) ) ;
#26982=CARTESIAN_POINT ( 'NONE',  ( 100.9507452397097467, -28.71010058181673230, 40.59361269664083949 ) ) ;
#26983=CARTESIAN_POINT ( 'NONE',  ( 115.0889047249108614, -30.61763668143413497, 75.34395860910829867 ) ) ;
#26986=CARTESIAN_POINT ( 'NONE',  ( 32.25690895537100289, -33.54226604285010893, -5.074374724088000832 ) ) ;
#26987=CARTESIAN_POINT ( 'NONE',  ( 107.2496247454619152, -24.85508506706595000, 230.0641967044819580 ) ) ;
#26988=CARTESIAN_POINT ( 'NONE',  ( 97.83606632657298974, -31.88363555591887533, 131.9413395616259947 ) ) ;
#26989=CARTESIAN_POINT ( 'NONE',  ( 110.9086127847465377, -26.95314644129561543, 265.7784824187680783 ) ) ;
#26990=CARTESIAN_POINT ( 'NONE',  ( 25.56670390244797275, -58.35344715994099829, 257.2178068554150059 ) ) ;
#26992=CARTESIAN_POINT ( 'NONE',  ( 194.5667039024483529, -47.82844715993405771, 249.9678068554149775 ) ) ;
#26994=FACE_OUTER_BOUND ( 'NONE', #30845, .T. ) ;
#26995=DIRECTION ( 'NONE',  ( 0.7071067811989671936, 0.7071067811741279519, 6.612322855971028274E-17 ) ) ;
#26996=DIRECTION ( 'NONE',  ( -3.062684205862500216E-15, 0.000000000000000000, 1.000000000000000000 ) ) ;
#26998=AXIS2_PLACEMENT_3D ( 'NONE', #10542, #24184, #58245 ) ;
#27001=VERTEX_POINT ( 'NONE', #5069 ) ;
#27002=CARTESIAN_POINT ( 'NONE',  ( 103.2375202873391800, -28.52263824056898756, 134.8343245899819465 ) ) ;
#27003=DIRECTION ( 'NONE',  ( 0.000000000000000000, 0.000000000000000000, -1.000000000000000000 ) ) ;
#27004=ORIENTED_EDGE ( 'NONE', *, *, #41697, .T. ) ;
#27005=CARTESIAN_POINT ( 'NONE',  ( 150.5667039024485234, -47.82844715993594065, 180.4678068554149775 ) ) ;
#27006=CARTESIAN_POINT ( 'NONE',  ( 109.5033840998383994, -46.84330794493973826, 128.7641967044819751 ) ) ;
#27007=CARTESIAN_POINT ( 'NONE',  ( 100.8868115320050549, -44.69967795324804882, 148.0528215568805308 ) ) ;
#27009=DIRECTION ( 'NONE',  ( 1.000000000000000000, 3.999999999999999995E-14, 1.000000000000000078E-15 ) ) ;
#27010=CARTESIAN_POINT ( 'NONE',  ( 83.06670390244796920, -61.87844715994100397, 231.5838068554150198 ) ) ;
#27012=CARTESIAN_POINT ( 'NONE',  ( 112.3909220325769667, -27.83061929752856400, 54.65943479972096242 ) ) ;
#27013=ORIENTED_EDGE ( 'NONE', *, *, #64063, .T. ) ;
#27016=LINE ( 'NONE', #82450, #54449 ) ;
#27017=CARTESIAN_POINT ( 'NONE',  ( 116.6093774848465472, -38.87601340171671893, 144.6499109901959628 ) ) ;
#27019=CIRCLE ( 'NONE', #5296, 2.116999999999980009 ) ;
#27020=LINE ( 'NONE', #74280, #61000 ) ;
#27021=EDGE_CURVE ( 'NONE', #76097, #26390, #66386, .T. ) ;
#27022=FACE_OUTER_BOUND ( 'NONE', #21892, .T. ) ;
#27025=EDGE_CURVE ( 'NONE', #15206, #51994, #55705, .T. ) ;
#27026=LINE ( 'NONE', #67010, #30348 ) ;
#27027=DIRECTION ( 'NONE',  ( 6.524622321627019585E-16, 3.741823817616790462E-31, 1.000000000000000000 ) ) ;
#27028=CARTESIAN_POINT ( 'NONE',  ( 113.4926247784321021, -28.54816540729036589, 79.54705384733995288 ) ) ;
#27029=ORIENTED_EDGE ( 'NONE', *, *, #55501, .T. ) ;
#27030=VERTEX_POINT ( 'NONE', #41807 ) ;
#27031=ORIENTED_EDGE ( 'NONE', *, *, #82115, .T. ) ;
#27032=EDGE_CURVE ( 'NONE', #30851, #37640, #7319, .T. ) ;
#27033=DIRECTION ( 'NONE',  ( -1.000000000000000000, -4.299999999999999979E-14, -1.000000000000000078E-15 ) ) ;
#27036=CARTESIAN_POINT ( 'NONE',  ( 110.4730825863185260, -45.36026475776040456, 170.6938046553059678 ) ) ;
#27038=CARTESIAN_POINT ( 'NONE',  ( 37.35959712141614375, -48.62134037890901084, 300.4678068554150059 ) ) ;
#27039=ORIENTED_EDGE ( 'NONE', *, *, #40460, .F. ) ;
#27040=EDGE_LOOP ( 'NONE', ( #76642, #81011 ) ) ;
#27041=ORIENTED_EDGE ( 'NONE', *, *, #69440, .T. ) ;
#27042=CARTESIAN_POINT ( 'NONE',  ( 131.0667039024480118, -64.87844715994098976, 213.1838068554149856 ) ) ;
#27043=CARTESIAN_POINT ( 'NONE',  ( 136.6734006051289612, -19.60624470235256567, 2.902100967938342269 ) ) ;
#27044=ORIENTED_EDGE ( 'NONE', *, *, #15866, .T. ) ;
#27046=DIRECTION ( 'NONE',  ( -0.7071067812163264188, 0.7071067811567686157, -7.071067812162960697E-16 ) ) ;
#27047=B_SPLINE_CURVE_WITH_KNOTS ( 'NONE', 3,
 ( #32983, #60680, #82061, #67959, #81617, #5746, #56095, #84304, #37806, #76572, #21619, #65505, #30542, #21161, #77026, #14353, #58242, #86411, #48380, #23307, #10100, #37353, #69758, #9646, #58667, #3288, #83844, #7528, #13892, #56561, #28408, #85970, #27961, #55639, #2844, #62926, #78715, #34779, #48832, #23739, #14804, #51405, #49294, #50974, #65062, #79158, #704, #16918, #72330 ),
 .UNSPECIFIED., .F., .F.,
 ( 4, 2, 1, 1, 1, 1, 2, 2, 2, 2, 2, 2, 2, 1, 1, 1, 1, 1, 1, 1, 2, 2, 2, 2, 2, 2, 2, 2, 2, 4 ),
 ( 0.5000151141236341967, 0.5005033806137728636, 0.5009916471039114194, 0.5019681800841889752, 0.5039212460447435316, 0.5078273779658523113, 0.5156396418080697597, 0.5312641694925048785, 0.5625132248613745611, 0.6250113355991141484, 0.6875094463368538467, 0.7500075570745934339, 0.7500685903858610448, 0.7501296236971285447, 0.7502516903196607689, 0.7504958235647252174, 0.7509840900548254705, 0.7519606230349995535, 0.7539136889953474974, 0.7578198209160560417, 0.7656320847574735744, 0.7812566124403086398, 0.8125056678059787707, 0.8437547231716489016, 0.8750037785373191435, 0.9062528339029893854, 0.9375018892686595162, 0.9687509446343296471, 0.9843754723171647125, 1.000000000000000000 ),
 .UNSPECIFIED. ) ;
#27049=CARTESIAN_POINT ( 'NONE',  ( 99.81674604704261355, -31.63341061165540680, 202.2701547344679796 ) ) ;
#27051=CARTESIAN_POINT ( 'NONE',  ( 142.8821648370248170, -72.54478064608022692, 542.9756252759101471 ) ) ;
#27052=EDGE_CURVE ( 'NONE', #68551, #50389, #50, .T. ) ;
#27054=VECTOR ( 'NONE', #28242, 1000.000000000000000 ) ;
#27055=ORIENTED_EDGE ( 'NONE', *, *, #46600, .F. ) ;
#27058=AXIS2_PLACEMENT_3D ( 'NONE', #61095, #26140, #12512 ) ;
#27059=DIRECTION ( 'NONE',  ( 0.000000000000000000, 0.000000000000000000, 1.000000000000000000 ) ) ;
#27060=EDGE_LOOP ( 'NONE', ( #83538, #87104, #7967, #75191 ) ) ;
#27061=ORIENTED_EDGE ( 'NONE', *, *, #81598, .T. ) ;
#27062=CARTESIAN_POINT ( 'NONE',  ( 104.9869425053901892, -28.32846893322983917, 238.0757094172099642 ) ) ;
#27063=CARTESIAN_POINT ( 'NONE',  ( 100.8733315758915552, -45.91070206092880568, 152.0918157521009562 ) ) ;
#27064=CARTESIAN_POINT ( 'NONE',  ( 98.22092589535427010, -43.31882777834842813, 111.8480062282919647 ) ) ;
#27065=CARTESIAN_POINT ( 'NONE',  ( 108.4649749756400183, -27.96694839443428293, 249.5838068554169524 ) ) ;
#27067=CARTESIAN_POINT ( 'NONE',  ( 103.7231914492017637, -26.19396519929847145, 201.3089586092439731 ) ) ;
#27068=CARTESIAN_POINT ( 'NONE',  ( 98.20858259865026696, -41.48711566647967430, 276.7185663392993433 ) ) ;
#27069=VERTEX_POINT ( 'NONE', #33226 ) ;
#27072=ORIENTED_EDGE ( 'NONE', *, *, #17586, .F. ) ;
#27076=ORIENTED_EDGE ( 'NONE', *, *, #55792, .T. ) ;
#27077=DIRECTION ( 'NONE',  ( 0.000000000000000000, 0.000000000000000000, -1.000000000000000000 ) ) ;
#27078=AXIS2_PLACEMENT_3D ( 'NONE', #26618, #54743, #52935 ) ;
#27079=CARTESIAN_POINT ( 'NONE',  ( 114.0222564360173720, -28.96386602133403798, 114.4956252759109816 ) ) ;
#27082=DIRECTION ( 'NONE',  ( 0.000000000000000000, 0.000000000000000000, -1.000000000000000000 ) ) ;
#27085=CARTESIAN_POINT ( 'NONE',  ( 117.2062538965839309, -41.07097622818925942, 209.5165776568640013 ) ) ;
#27086=DIRECTION ( 'NONE',  ( 0.000000000000000000, 0.000000000000000000, 1.000000000000000000 ) ) ;
#27089=DIRECTION ( 'NONE',  ( 0.7071067811861589947, -0.7071067811869361508, 0.000000000000000000 ) ) ;
#27090=FACE_OUTER_BOUND ( 'NONE', #69040, .T. ) ;
#27091=CARTESIAN_POINT ( 'NONE',  ( 151.0371591254575776, -24.42818131005592264, 117.4678068554150485 ) ) ;
#27092=DIRECTION ( 'NONE',  ( 4.299999999999999979E-14, -1.000000000000000000, 4.400000000000000367E-29 ) ) ;
#27094=CARTESIAN_POINT ( 'NONE',  ( 97.51966259852430596, -43.83486848311488160, 261.8356252759109566 ) ) ;
#27095=ORIENTED_EDGE ( 'NONE', *, *, #35099, .F. ) ;
#27097=CARTESIAN_POINT ( 'NONE',  ( 102.2921677216391174, -27.39701587636625391, 120.4527681330539792 ) ) ;
#27098=CARTESIAN_POINT ( 'NONE',  ( 95.20664489286731680, -37.33482625718801273, 267.3670538473395482 ) ) ;
#27099=CARTESIAN_POINT ( 'NONE',  ( 100.8606736390591720, -45.92946726319084405, 148.0918157521009562 ) ) ;
#27102=FACE_OUTER_BOUND ( 'NONE', #63378, .T. ) ;
#27103=FACE_OUTER_BOUND ( 'NONE', #36524, .T. ) ;
#27104=CARTESIAN_POINT ( 'NONE',  ( 97.07207207411279626, -35.37844109237227741, 191.2189586007484934 ) ) ;
#27105=DIRECTION ( 'NONE',  ( -0.7071067811864693020, -0.7071067811866258435, 2.899137802865049595E-29 ) ) ;
#27109=ORIENTED_EDGE ( 'NONE', *, *, #45076, .T. ) ;
#27110=ORIENTED_EDGE ( 'NONE', *, *, #26904, .F. ) ;
#27112=LINE ( 'NONE', #47979, #39489 ) ;
#27113=CARTESIAN_POINT ( 'NONE',  ( 112.1067112481348431, -26.91823048478340397, 15.71086337114896381 ) ) ;
#27117=AXIS2_PLACEMENT_3D ( 'NONE', #37895, #43351, #22945 ) ;
#27118=CARTESIAN_POINT ( 'NONE',  ( 101.8914336387190502, -44.16123909860101548, 236.5028960185529456 ) ) ;
#27122=CIRCLE ( 'NONE', #57592, 0.4999999999999933387 ) ;
#27123=DIRECTION ( 'NONE',  ( -3.201858731750027727E-15, 1.000000000000000000, -3.201858731750027724E-30 ) ) ;
#27124=CARTESIAN_POINT ( 'NONE',  ( 113.1784658275440449, -44.75174020452156753, 103.0937353791139799 ) ) ;
#27125=LINE ( 'NONE', #79536, #51302 ) ;
#27126=CARTESIAN_POINT ( 'NONE',  ( 97.81168895331838087, -40.51742574516882200, 287.6356252759109680 ) ) ;
#27128=EDGE_CURVE ( 'NONE', #54496, #2932, #55876, .T. ) ;
#27129=CARTESIAN_POINT ( 'NONE',  ( 134.0664832912740110, -8.350947159940998787, 4.925625275911999168 ) ) ;
#27131=CARTESIAN_POINT ( 'NONE',  ( 194.0371591254573218, -24.42818131005417825, 237.4678068554150059 ) ) ;
#27132=CARTESIAN_POINT ( 'NONE',  ( 114.8131502045276449, -44.70447909941025699, 268.1899109901970633 ) ) ;
#27133=CARTESIAN_POINT ( 'NONE',  ( 20.03715912545737510, -24.95799193693189721, 249.9678068554150059 ) ) ;
#27135=EDGE_CURVE ( 'NONE', #62140, #41893, #47732, .T. ) ;
#27137=AXIS2_PLACEMENT_3D ( 'NONE', #209, #27909, #41523 ) ;
#27138=AXIS2_PLACEMENT_3D ( 'NONE', #52711, #74095, #80472 ) ;
#27140=CARTESIAN_POINT ( 'NONE',  ( 111.5571307036148312, -44.84917726517733882, 100.7966617981629582 ) ) ;
#27141=EDGE_CURVE ( 'NONE', #25851, #20875, #71163, .T. ) ;
#27143=CYLINDRICAL_SURFACE ( 'NONE', #89118, 6.571100913904396990 ) ;
#27144=EDGE_CURVE ( 'NONE', #45997, #45134, #61010, .T. ) ;
#27145=CARTESIAN_POINT ( 'NONE',  ( 97.07207205845678288, -35.37844120283712357, 46.21895860954398927 ) ) ;
#27147=CARTESIAN_POINT ( 'NONE',  ( 77.53592152231070145, -35.65293368212927305, 7.043713522541964700 ) ) ;
#27148=EDGE_LOOP ( 'NONE', ( #19623, #52228, #64569, #11878 ) ) ;
#27149=CARTESIAN_POINT ( 'NONE',  ( 102.3126588425671315, -26.75045724741508124, 140.4422919425769578 ) ) ;
#27152=CARTESIAN_POINT ( 'NONE',  ( 115.7982244386701609, -33.26055366603426933, 95.57110711542094350 ) ) ;
#27155=CARTESIAN_POINT ( 'NONE',  ( 117.1124756048696440, -32.06433792440376607, 55.16038718067301261 ) ) ;
#27156=VECTOR ( 'NONE', #42947, 1000.000000000000000 ) ;
#27160=ORIENTED_EDGE ( 'NONE', *, *, #8281, .F. ) ;
#27161=ORIENTED_EDGE ( 'NONE', *, *, #45886, .T. ) ;
#27162=DIRECTION ( 'NONE',  ( 1.000000000000000000, 0.000000000000000000, 0.000000000000000000 ) ) ;
#27163=VERTEX_POINT ( 'NONE', #27301 ) ;
#27164=CARTESIAN_POINT ( 'NONE',  ( 116.0161715043950466, -40.67488961668907166, 253.4956252759109532 ) ) ;
#27165=CARTESIAN_POINT ( 'NONE',  ( 107.6542194910912684, -47.14941140656445384, 148.6213395616249784 ) ) ;
#27167=CARTESIAN_POINT ( 'NONE',  ( 116.3192736897089645, -32.94707975126958388, 130.1356252759109680 ) ) ;
#27168=CARTESIAN_POINT ( 'NONE',  ( 97.62238793418175931, -32.23162594710754547, 71.97276813305397525 ) ) ;
#27169=CARTESIAN_POINT ( 'NONE',  ( 107.0664832912739968, 25.62155284005901379, 333.4006252759110112 ) ) ;
#27170=ORIENTED_EDGE ( 'NONE', *, *, #74601, .F. ) ;
#27171=CARTESIAN_POINT ( 'NONE',  ( 194.0371591254582881, -46.82818131005407736, 249.9678068554149775 ) ) ;
#27172=DIRECTION ( 'NONE',  ( 0.9068632946707807507, -0.4214249218767880945, 8.673617379884035472E-16 ) ) ;
#27177=VECTOR ( 'NONE', #81985, 1000.000000000000114 ) ;
#27178=CARTESIAN_POINT ( 'NONE',  ( 130.5667039024481255, -40.02944715994102154, 249.5838068554162987 ) ) ;
#27179=CARTESIAN_POINT ( 'NONE',  ( 105.7790678824445081, -26.40611305247077567, 270.1756252759109884 ) ) ;
#27180=DIRECTION ( 'NONE',  ( -0.7071067811865506814, 0.7071067811865443531, -7.071067811865500971E-16 ) ) ;
#27184=CARTESIAN_POINT ( 'NONE',  ( 100.9974734301594310, -29.01720366022859565, 15.60705384733995871 ) ) ;
#27186=CARTESIAN_POINT ( 'NONE',  ( 96.66103594285313250, -37.56076609107801545, 97.38991099019594344 ) ) ;
#27187=CARTESIAN_POINT ( 'NONE',  ( 122.8585116216235065, -38.08382569396911776, 302.6356252759109680 ) ) ;
#27188=CARTESIAN_POINT ( 'NONE',  ( 100.8602861511969024, -45.93004170815812159, 152.0918157521009562 ) ) ;
#27189=FACE_OUTER_BOUND ( 'NONE', #69874, .T. ) ;
#27190=VERTEX_POINT ( 'NONE', #34559 ) ;
#27192=DIRECTION ( 'NONE',  ( -0.000000000000000000, 1.000000000000000000, 0.000000000000000000 ) ) ;
#27196=CARTESIAN_POINT ( 'NONE',  ( 109.2104764766756517, -26.48201038666214657, 139.9127681330539872 ) ) ;
#27198=DIRECTION ( 'NONE',  ( -4.237773401492740281E-14, 1.000000000000000000, 0.000000000000000000 ) ) ;
#27199=AXIS2_PLACEMENT_3D ( 'NONE', #70950, #43659, #84130 ) ;
#27201=CIRCLE ( 'NONE', #60505, 15.69999999999999574 ) ;
#27203=DIRECTION ( 'NONE',  ( 3.062684205862500216E-15, 0.000000000000000000, -1.000000000000000000 ) ) ;
#27204=ORIENTED_EDGE ( 'NONE', *, *, #43370, .T. ) ;
#27205=VECTOR ( 'NONE', #74613, 1000.000000000000000 ) ;
#27206=EDGE_CURVE ( 'NONE', #6607, #593, #27622, .T. ) ;
#27207=ORIENTED_EDGE ( 'NONE', *, *, #46702, .F. ) ;
#27208=ORIENTED_EDGE ( 'NONE', *, *, #16740, .T. ) ;
#27209=ORIENTED_EDGE ( 'NONE', *, *, #66414, .F. ) ;
#27211=CARTESIAN_POINT ( 'NONE',  ( 99.28081699872726062, -30.36252297428069724, 250.7808459398054310 ) ) ;
#27212=FACE_OUTER_BOUND ( 'NONE', #44581, .T. ) ;
#27213=CARTESIAN_POINT ( 'NONE',  ( 21.03715912545746036, -47.82818131006197149, 117.4678068554150485 ) ) ;
#27215=LINE ( 'NONE', #76264, #50069 ) ;
#27216=ORIENTED_EDGE ( 'NONE', *, *, #78333, .F. ) ;
#27221=CARTESIAN_POINT ( 'NONE',  ( 113.3831382903590566, -27.58002901871528323, 235.5956252759109759 ) ) ;
#27222=EDGE_CURVE ( 'NONE', #53871, #29598, #78431, .T. ) ;
#27224=CARTESIAN_POINT ( 'NONE',  ( 103.5913876162975953, -46.49993820617270757, 98.31657765686297523 ) ) ;
#27228=CARTESIAN_POINT ( 'NONE',  ( 114.7529613671623139, -30.30768866273729500, 20.38027562559657113 ) ) ;
#27229=ORIENTED_EDGE ( 'NONE', *, *, #87034, .F. ) ;
#27233=EDGE_LOOP ( 'NONE', ( #35938, #54002, #11056, #33174 ) ) ;
#27235=CARTESIAN_POINT ( 'NONE',  ( 131.3164832912740110, -36.72944715994100306, 3.101481641215535046 ) ) ;
#27236=CARTESIAN_POINT ( 'NONE',  ( 114.3671945862968045, -31.65384462053443571, 275.7415833058969952 ) ) ;
#27237=CIRCLE ( 'NONE', #30167, 5.035202529042104302 ) ;
#27239=VECTOR ( 'NONE', #48309, 1000.000000000000000 ) ;
#27241=DIRECTION ( 'NONE',  ( 0.000000000000000000, 0.000000000000000000, 1.000000000000000000 ) ) ;
#27242=EDGE_CURVE ( 'NONE', #65418, #16063, #50428, .T. ) ;
#27244=ORIENTED_EDGE ( 'NONE', *, *, #64099, .T. ) ;
#27246=CONICAL_SURFACE ( 'NONE', #85376, 1.571100913904388552, 1.047197551196592302 ) ;
#27247=CARTESIAN_POINT ( 'NONE',  ( 113.1764918811396399, -44.75321505856369697, 184.0943504403222164 ) ) ;
#27248=VERTEX_POINT ( 'NONE', #63621 ) ;
#27249=CARTESIAN_POINT ( 'NONE',  ( 117.0539912639601852, -31.99354471700374702, 64.19086337114899266 ) ) ;
#27250=ORIENTED_EDGE ( 'NONE', *, *, #15570, .F. ) ;
#27251=CARTESIAN_POINT ( 'NONE',  ( 113.9883325317156135, -31.53436023685440048, 262.1690427505439516 ) ) ;
#27253=DIRECTION ( 'NONE',  ( 3.360405532702990443E-14, -1.000000000000000000, 0.000000000000000000 ) ) ;
#27254=CARTESIAN_POINT ( 'NONE',  ( 97.31342953368660176, -35.99458159538090030, 146.2670538473399517 ) ) ;
#27258=CARTESIAN_POINT ( 'NONE',  ( 181.8764988495247223, -33.54226604284360747, 237.4678068554150059 ) ) ;
#27259=VECTOR ( 'NONE', #74774, 999.9999999999998863 ) ;
#27261=CARTESIAN_POINT ( 'NONE',  ( 110.0014563237810137, -26.68062070874399438, 255.8499109901966051 ) ) ;
#27263=ORIENTED_EDGE ( 'NONE', *, *, #17191, .F. ) ;
#27264=EDGE_LOOP ( 'NONE', ( #88375, #69526, #50354, #3199 ) ) ;
#27265=CARTESIAN_POINT ( 'NONE',  ( 113.8847749867171046, -44.67324210339663182, 104.1413395616249744 ) ) ;
#27267=VERTEX_POINT ( 'NONE', #57698 ) ;
#27269=ORIENTED_EDGE ( 'NONE', *, *, #43674, .T. ) ;
#27270=DIRECTION ( 'NONE',  ( 0.000000000000000000, -1.000000000000000000, 0.000000000000000000 ) ) ;
#27271=CARTESIAN_POINT ( 'NONE',  ( 107.0664832912739541, -23.56278049327425350, 357.5272416190308604 ) ) ;
#27272=CARTESIAN_POINT ( 'NONE',  ( 128.8897065959775432, -58.55267046464430791, -5.074374724089007138 ) ) ;
#27273=DIRECTION ( 'NONE',  ( 0.000000000000000000, 0.000000000000000000, -1.000000000000000000 ) ) ;
#27274=CARTESIAN_POINT ( 'NONE',  ( 99.93348902297414327, -31.82829241803101894, 163.6776141791149826 ) ) ;
#27275=CARTESIAN_POINT ( 'NONE',  ( 100.2329966457367334, -45.44659500335379221, 273.0594347997205773 ) ) ;
#27276=FACE_OUTER_BOUND ( 'NONE', #19683, .T. ) ;
#27277=ORIENTED_EDGE ( 'NONE', *, *, #76061, .T. ) ;
#27279=VECTOR ( 'NONE', #38750, 1000.000000000000000 ) ;
#27280=DIRECTION ( 'NONE',  ( -0.7071067811865462405, 0.000000000000000000, 0.7071067811865486830 ) ) ;
#27281=EDGE_CURVE ( 'NONE', #21126, #25185, #84982, .T. ) ;
#27282=ORIENTED_EDGE ( 'NONE', *, *, #10741, .T. ) ;
#27283=AXIS2_PLACEMENT_3D ( 'NONE', #57209, #77230, #15459 ) ;
#27285=LINE ( 'NONE', #34990, #83691 ) ;
#27288=DIRECTION ( 'NONE',  ( 0.7071067812152160847, -0.7071067811578790607, 0.000000000000000000 ) ) ;
#27289=CARTESIAN_POINT ( 'NONE',  ( 97.33781463699185110, -34.07115960914099162, 16.11479949169054393 ) ) ;
#27291=CARTESIAN_POINT ( 'NONE',  ( 83.73314995794039817, 12.92155284005802685, 349.2756252759109543 ) ) ;
#27292=DIRECTION ( 'NONE',  ( 0.7071067811571474238, 0.7071067812159476107, 0.000000000000000000 ) ) ;
#27293=CARTESIAN_POINT ( 'NONE',  ( 100.0898434420045788, -43.48201142159524579, 191.3609912566489584 ) ) ;
#27294=CARTESIAN_POINT ( 'NONE',  ( 112.7839950898761288, -27.91685089337277503, 69.61848241876793963 ) ) ;
#27297=CARTESIAN_POINT ( 'NONE',  ( 51.23005224011698289, -33.89581943344334292, 313.9678068554150059 ) ) ;
#27298=VERTEX_POINT ( 'NONE', #30006 ) ;
#27299=CARTESIAN_POINT ( 'NONE',  ( 109.7235518845674136, -27.00045683442361266, 260.8648104962068146 ) ) ;
#27301=CARTESIAN_POINT ( 'NONE',  ( 135.9998166246059839, 12.92155284005730387, 361.9756252759109998 ) ) ;
#27303=CARTESIAN_POINT ( 'NONE',  ( 105.7145417833327343, -46.72371677956441260, 132.4689531747473268 ) ) ;
#27304=AXIS2_PLACEMENT_3D ( 'NONE', #67098, #39392, #12142 ) ;
#27306=ORIENTED_EDGE ( 'NONE', *, *, #71944, .T. ) ;
#27309=CARTESIAN_POINT ( 'NONE',  ( 110.3610989901968651, -25.31982300743893077, 64.85276813305395649 ) ) ;
#27311=CARTESIAN_POINT ( 'NONE',  ( 142.0664832912740394, -45.72944715994099596, 14.67562527591100441 ) ) ;
#27313=DIRECTION ( 'NONE',  ( -0.9999999853157766072, -0.0001713722456127291416, 9.999999853157765648E-16 ) ) ;
#27314=EDGE_LOOP ( 'NONE', ( #58735, #77257 ) ) ;
#27315=AXIS2_PLACEMENT_3D ( 'NONE', #64578, #17324, #85935 ) ;
#27321=ORIENTED_EDGE ( 'NONE', *, *, #48420, .T. ) ;
#27322=CARTESIAN_POINT ( 'NONE',  ( 97.60264960697516301, -32.22222542080420027, 71.97276813305397525 ) ) ;
#27323=CIRCLE ( 'NONE', #89724, 3.000000000000002665 ) ;
#27324=CIRCLE ( 'NONE', #70854, 16.00000000000000000 ) ;
#27325=CARTESIAN_POINT ( 'NONE',  ( 89.17003477451882532, -56.47944715994104570, 14.92562527591095289 ) ) ;
#27326=CARTESIAN_POINT ( 'NONE',  ( 41.56648329127381203, -27.82844715994070484, 141.9256252759119832 ) ) ;
#27330=CARTESIAN_POINT ( 'NONE',  ( 105.4244293397739085, -47.72525222749315787, 143.4584824187679715 ) ) ;
#27331=AXIS2_PLACEMENT_3D ( 'NONE', #48152, #475, #89525 ) ;
#27332=CYLINDRICAL_SURFACE ( 'NONE', #74736, 2.517500000000005844 ) ;
#27333=ORIENTED_EDGE ( 'NONE', *, *, #56541, .F. ) ;
#27334=CARTESIAN_POINT ( 'NONE',  ( 100.2624651760415873, -28.85963121439202794, 256.6441967044821695 ) ) ;
#27337=CARTESIAN_POINT ( 'NONE',  ( 165.2725846195380086, -35.55794170701810941, -5.074374724088000832 ) ) ;
#27338=ADVANCED_FACE ( 'NONE', ( #29108 ), #35909, .F. ) ;
#27339=PLANE ( 'NONE',  #77527 ) ;
#27340=DIRECTION ( 'NONE',  ( 1.000000000000000000, 0.000000000000000000, 0.000000000000000000 ) ) ;
#27341=CARTESIAN_POINT ( 'NONE',  ( 131.3164832912739826, -18.72944715994100662, -5.074374724089004474 ) ) ;
#27342=CARTESIAN_POINT ( 'NONE',  ( 114.4888877093246293, -29.48743791597849651, 194.4537205140069318 ) ) ;
#27344=VERTEX_POINT ( 'NONE', #44053 ) ;
#27346=VECTOR ( 'NONE', #82888, 1000.000000000000000 ) ;
#27347=CARTESIAN_POINT ( 'NONE',  ( 103.4772640228778329, -44.83165572645120278, 173.6758690201829438 ) ) ;
#27349=CARTESIAN_POINT ( 'NONE',  ( 102.6690082227317475, -46.93785447722112281, 283.2527681330534506 ) ) ;
#27350=DIRECTION ( 'NONE',  ( -1.000000000000000000, 0.000000000000000000, 0.000000000000000000 ) ) ;
#27351=PLANE ( 'NONE',  #10177 ) ;
#27353=EDGE_CURVE ( 'NONE', #46749, #87063, #85687, .T. ) ;
#27354=DIRECTION ( 'NONE',  ( 0.000000000000000000, 0.000000000000000000, -1.000000000000000000 ) ) ;
#27355=CARTESIAN_POINT ( 'NONE',  ( 97.81168895331838087, -40.51742574516882200, 11.63562527591094309 ) ) ;
#27357=EDGE_CURVE ( 'NONE', #7162, #77531, #15029, .T. ) ;
#27358=CARTESIAN_POINT ( 'NONE',  ( 100.6697571656888073, -44.93374849542868787, 232.0499109901969632 ) ) ;
#27359=CARTESIAN_POINT ( 'NONE',  ( 116.3170820643562564, -32.94538914428453324, 169.1356252759109680 ) ) ;
#27360=EDGE_LOOP ( 'NONE', ( #24913, #35818, #52664, #71095 ) ) ;
#27361=EDGE_LOOP ( 'NONE', ( #27550, #47759, #43996, #84252 ) ) ;
#27364=CARTESIAN_POINT ( 'NONE',  ( 82.49755700851123663, -20.01506174167580099, 7.157201688891981384 ) ) ;
#27365=CARTESIAN_POINT ( 'NONE',  ( 102.0674957170151060, -27.97023961310380713, 185.4902194784735912 ) ) ;
#27366=DIRECTION ( 'NONE',  ( -0.7071067811865634489, 0.7071067811865315855, -7.071067811865641980E-16 ) ) ;
#27369=ORIENTED_EDGE ( 'NONE', *, *, #32998, .T. ) ;
#27370=CARTESIAN_POINT ( 'NONE',  ( 116.8105015878075079, -31.41422314659176607, 20.21181575210195902 ) ) ;
#27371=CARTESIAN_POINT ( 'NONE',  ( 115.5175571194294122, -29.60495148624196204, 224.3718157521009573 ) ) ;
#27372=VERTEX_POINT ( 'NONE', #49972 ) ;
#27373=CIRCLE ( 'NONE', #20126, 2.500000000000002220 ) ;
#27374=CARTESIAN_POINT ( 'NONE',  ( 172.5664832912729878, -27.57844715994070484, 135.9256252759119832 ) ) ;
#27375=CARTESIAN_POINT ( 'NONE',  ( 123.0664832912757163, -36.72944715993921960, -4.074374724089013355 ) ) ;
#27377=CARTESIAN_POINT ( 'NONE',  ( 104.3513172347134770, -44.42734293102004273, 55.12523322673396109 ) ) ;
#27378=AXIS2_PLACEMENT_3D ( 'NONE', #71940, #31471, #51463 ) ;
#27379=CARTESIAN_POINT ( 'NONE',  ( 98.14969091592392658, -31.28627964566590336, 166.8899109901969950 ) ) ;
#27380=DIRECTION ( 'NONE',  ( 0.000000000000000000, 0.000000000000000000, -1.000000000000000000 ) ) ;
#27381=ORIENTED_EDGE ( 'NONE', *, *, #42995, .F. ) ;
#27383=CYLINDRICAL_SURFACE ( 'NONE', #77007, 0.5000000000000079936 ) ;
#27385=ORIENTED_EDGE ( 'NONE', *, *, #32422, .T. ) ;
#27386=LINE ( 'NONE', #33759, #58949 ) ;
#27387=VERTEX_POINT ( 'NONE', #1407 ) ;
#27388=ORIENTED_EDGE ( 'NONE', *, *, #62886, .T. ) ;
#27389=CARTESIAN_POINT ( 'NONE',  ( 97.81170255947417047, -40.51743869465033754, 117.6354096206635518 ) ) ;
#27391=CARTESIAN_POINT ( 'NONE',  ( 108.8595479556035599, -45.11020018309576329, 107.1667055423619672 ) ) ;
#27392=CARTESIAN_POINT ( 'NONE',  ( 114.6215443236117153, -29.51367161159714314, 234.4327681330539690 ) ) ;
#27393=CARTESIAN_POINT ( 'NONE',  ( 117.1710321396411416, -41.15233254730030410, 208.4861014663869696 ) ) ;
#27395=CARTESIAN_POINT ( 'NONE',  ( 118.5467753794658705, -33.90456151647279626, 10.01848241876795953 ) ) ;
#27397=FACE_OUTER_BOUND ( 'NONE', #57611, .T. ) ;
#27398=ORIENTED_EDGE ( 'NONE', *, *, #5142, .T. ) ;
#27400=CARTESIAN_POINT ( 'NONE',  ( 107.2219638487720488, -26.36052190073617041, 80.07657765686398932 ) ) ;
#27401=CARTESIAN_POINT ( 'NONE',  ( 110.3680388590993573, -25.29578946207851331, 64.85276813305395649 ) ) ;
#27402=CARTESIAN_POINT ( 'NONE',  ( 111.7588773036880383, -27.37059502548119028, 279.7070538473396937 ) ) ;
#27403=EDGE_LOOP ( 'NONE', ( #82702, #40510, #51761, #15678, #43959, #32129, #81770, #40014, #10512, #17426, #39566, #61094, #34525, #50934, #84237, #10483, #4886, #252, #2599, #73911, #22110, #42043, #37175, #86568, #67554, #7508, #46013, #77450, #30908, #4002, #47988, #56757, #71653, #32506, #10894, #56193, #36093, #41089, #77018, #59457, #25019, #68448, #42425, #23817, #82213, #1169, #66013, #46168, #58860, #16215, #70151, #31691, #81898, #17785, #36624, #63880, #55113, #61236, #66956, #1272, #42520, #60606, #43263, #14888, #68323, #44399, #61765, #58579, #17264, #58046, #83181, #14643, #52624, #50963, #52241, #57888, #22117, #52096, #48424, #9048, #70285, #45507, #28643, #43745, #19556, #76690, #75472, #16441, #31236, #55772, #69626, #32120 ) ) ;
#27405=CARTESIAN_POINT ( 'NONE',  ( 113.0255487838780937, -46.03904575001691768, 218.0175300378159591 ) ) ;
#27406=CARTESIAN_POINT ( 'NONE',  ( 163.0664832912739826, 12.92155284005902516, 333.4006252759110112 ) ) ;
#27407=CARTESIAN_POINT ( 'NONE',  ( 53.35959712126142307, -48.62134037875158299, 180.4678068554151196 ) ) ;
#27408=DIRECTION ( 'NONE',  ( 0.000000000000000000, 1.000000000000000000, 0.000000000000000000 ) ) ;
#27409=CARTESIAN_POINT ( 'NONE',  ( 114.1839641476628913, -41.30284314992755412, 277.6356252759110248 ) ) ;
#27410=DIRECTION ( 'NONE',  ( 1.000000000000000000, 8.673617379883546378E-16, 9.757819552368989676E-16 ) ) ;
#27411=CARTESIAN_POINT ( 'NONE',  ( 188.5667039024479834, -67.87844715994100397, 137.2178068554150059 ) ) ;
#27413=LINE ( 'NONE', #69657, #38310 ) ;
#27414=B_SPLINE_CURVE_WITH_KNOTS ( 'NONE', 3,
 ( #41747, #27692, #75404, #34944, #42201, #20440, #6796, #69030, #55370, #70376, #6352, #76741, #56730, #13175, #8148, #63100, #14522, #48550 ),
 .UNSPECIFIED., .F., .F.,
 ( 4, 2, 2, 2, 2, 2, 2, 2, 4 ),
 ( 0.000000000000000000, 0.06249937177560595247, 0.1249987435512119049, 0.1874981153268178713, 0.2499974871024238099, 0.3124968588780297485, 0.3749962306536357426, 0.4374956024292416812, 0.4999949742048476198 ),
 .UNSPECIFIED. ) ;
#27415=ADVANCED_FACE ( 'NONE', ( #15932 ), #2752, .F. ) ;
#27416=CARTESIAN_POINT ( 'NONE',  ( 71.24025061656124080, 8.642044024269713631, 394.9756252759102040 ) ) ;
#27417=CARTESIAN_POINT ( 'NONE',  ( 97.33724564666434276, -34.07349040010189611, 41.11432248975863502 ) ) ;
#27418=EDGE_CURVE ( 'NONE', #20886, #1757, #65363, .T. ) ;
#27420=CARTESIAN_POINT ( 'NONE',  ( 172.5664832912740110, 0.2215528400590013880, 316.8086252759120498 ) ) ;
#27421=EDGE_LOOP ( 'NONE', ( #62160, #42508, #58511, #66658, #13249 ) ) ;
#27422=TOROIDAL_SURFACE ( 'NONE', #46270, 15.84999999999999964, 0.1499999999999999944 ) ;
#27423=EDGE_CURVE ( 'NONE', #2591, #23447, #84260, .T. ) ;
#27424=FACE_OUTER_BOUND ( 'NONE', #68414, .T. ) ;
#27425=CARTESIAN_POINT ( 'NONE',  ( 112.5009111935468411, -46.38151608383146396, 257.9965776568635647 ) ) ;
#27426=CARTESIAN_POINT ( 'NONE',  ( 95.31164914186729220, -38.27921806354234491, 147.4299109901969871 ) ) ;
#27427=CARTESIAN_POINT ( 'NONE',  ( 106.1344768297789329, -47.78968505587090476, 258.4975300378158636 ) ) ;
#27429=DIRECTION ( 'NONE',  ( 0.9963424814100680926, -0.08544974978095730422, 0.000000000000000000 ) ) ;
#27430=CARTESIAN_POINT ( 'NONE',  ( 172.5664832912729878, -27.82844715994070484, 318.9256252759120116 ) ) ;
#27431=DIRECTION ( 'NONE',  ( -0.7071067811865171526, -0.7071067811865779928, -6.612322855854603498E-17 ) ) ;
#27432=EDGE_CURVE ( 'NONE', #60265, #70284, #79054, .T. ) ;
#27437=DIRECTION ( 'NONE',  ( -0.7071067811865764385, 0.7071067811865187069, -7.071067811865771156E-16 ) ) ;
#27439=CARTESIAN_POINT ( 'NONE',  ( 108.1312808730283166, -45.72271566404705112, 162.1048007804579640 ) ) ;
#27443=CARTESIAN_POINT ( 'NONE',  ( 48.79742451362098166, -36.32844715994040996, 342.9256252759119548 ) ) ;
#27444=CARTESIAN_POINT ( 'NONE',  ( 109.3536845750984128, -25.93905639472658819, 180.9222919425779708 ) ) ;
#27446=EDGE_CURVE ( 'NONE', #54334, #87716, #87645, .T. ) ;
#27447=DIRECTION ( 'NONE',  ( 0.000000000000000000, 0.000000000000000000, 1.000000000000000000 ) ) ;
#27449=DIRECTION ( 'NONE',  ( 0.000000000000000000, 1.000000000000000000, 0.000000000000000000 ) ) ;
#27451=CARTESIAN_POINT ( 'NONE',  ( 113.0229309284916752, -28.24065945027244595, 84.57753003781698453 ) ) ;
#27452=ORIENTED_EDGE ( 'NONE', *, *, #68600, .F. ) ;
#27456=CARTESIAN_POINT ( 'NONE',  ( 102.2986265273211615, -45.30740241592380357, 183.1727681330529833 ) ) ;
#27457=CARTESIAN_POINT ( 'NONE',  ( 172.5664832912728457, -18.82844715994071194, 261.9256252759119548 ) ) ;
#27458=CARTESIAN_POINT ( 'NONE',  ( 112.1400925610924730, -28.01325243291391232, 54.65557868090081683 ) ) ;
#27460=AXIS2_PLACEMENT_3D ( 'NONE', #26508, #66946, #81052 ) ;
#27462=DIRECTION ( 'NONE',  ( 0.000000000000000000, -1.000000000000000000, 0.000000000000000000 ) ) ;
#27463=EDGE_CURVE ( 'NONE', #7579, #30851, #32214, .T. ) ;
#27464=LINE ( 'NONE', #48784, #33250 ) ;
#27467=CARTESIAN_POINT ( 'NONE',  ( 102.6254653968535990, -46.82603978519644272, 132.2346728949579528 ) ) ;
#27469=ORIENTED_EDGE ( 'NONE', *, *, #42507, .F. ) ;
#27470=VERTEX_POINT ( 'NONE', #37717 ) ;
#27471=EDGE_CURVE ( 'NONE', #75399, #72082, #19044, .T. ) ;
#27472=CARTESIAN_POINT ( 'NONE',  ( 88.06670390244791236, -14.72944715994105991, 239.5838068554169809 ) ) ;
#27476=CARTESIAN_POINT ( 'NONE',  ( 102.5899018517108772, -44.13627803831183627, 199.9499951314959674 ) ) ;
#27477=AXIS2_PLACEMENT_3D ( 'NONE', #5348, #88476, #46200 ) ;
#27479=VERTEX_POINT ( 'NONE', #10885 ) ;
#27482=VECTOR ( 'NONE', #82898, 1000.000000000000000 ) ;
#27483=DIRECTION ( 'NONE',  ( -0.000000000000000000, -0.000000000000000000, -1.000000000000000000 ) ) ;
#27484=EDGE_LOOP ( 'NONE', ( #45146, #58612, #52030, #32948 ) ) ;
#27487=CARTESIAN_POINT ( 'NONE',  ( 100.0731593717985106, -30.45489967868845227, 232.1882499725639661 ) ) ;
#27489=ORIENTED_EDGE ( 'NONE', *, *, #70185, .F. ) ;
#27490=DIRECTION ( 'NONE',  ( 1.000000000000000078E-15, 1.000000000000000083E-30, -1.000000000000000000 ) ) ;
#27493=ORIENTED_EDGE ( 'NONE', *, *, #2020, .F. ) ;
#27495=VERTEX_POINT ( 'NONE', #59468 ) ;
#27499=CARTESIAN_POINT ( 'NONE',  ( 111.2851091291901042, -43.74983776777182953, 235.8252332267339852 ) ) ;
#27501=CARTESIAN_POINT ( 'NONE',  ( 98.43795593625375773, -42.68233540891471023, 126.8070538473389490 ) ) ;
#27502=CARTESIAN_POINT ( 'NONE',  ( 104.1140010245780445, -46.70499295924816607, 107.3470538473389411 ) ) ;
#27503=CARTESIAN_POINT ( 'NONE',  ( 99.21395805206054774, -38.40459780144472290, 249.5838068554171514 ) ) ;
#27504=CYLINDRICAL_SURFACE ( 'NONE', #1754, 4.874999999999990230 ) ;
#27505=( GEOMETRIC_REPRESENTATION_CONTEXT ( 3 ) GLOBAL_UNCERTAINTY_ASSIGNED_CONTEXT ( ( #594 ) ) GLOBAL_UNIT_ASSIGNED_CONTEXT ( ( #15036, #84545, #31332 ) ) REPRESENTATION_CONTEXT ( 'NONE', 'WORKASPACE' ) );
#27506=CARTESIAN_POINT ( 'NONE',  ( 96.04670619665022002, -35.87009084903410638, 187.2765776568629406 ) ) ;
#27507=CARTESIAN_POINT ( 'NONE',  ( 164.9190312289449878, -35.91149509761181235, 193.9678068554150059 ) ) ;
#27516=LINE ( 'NONE', #53399, #63512 ) ;
#27518=CARTESIAN_POINT ( 'NONE',  ( 113.3314600845033482, -45.06233935626208620, 143.0899109901969553 ) ) ;
#27525=CARTESIAN_POINT ( 'NONE',  ( 110.4916936757735186, -26.90617889774112825, 205.8099109901969541 ) ) ;
#27526=CARTESIAN_POINT ( 'NONE',  ( 20.03715912545737510, -24.95799193693189721, 249.9678068554150059 ) ) ;
#27529=VECTOR ( 'NONE', #5750, 1000.000000000000000 ) ;
#27530=CARTESIAN_POINT ( 'NONE',  ( 162.8913605087219878, -31.76306994223740432, 117.4678068554150627 ) ) ;
#27533=DIRECTION ( 'NONE',  ( 1.000000000000000078E-15, 1.000000000000000083E-30, -1.000000000000000000 ) ) ;
#27534=ADVANCED_FACE ( 'NONE', ( #39032 ), #72681, .T. ) ;
#27535=DIRECTION ( 'NONE',  ( 0.000000000000000000, 0.000000000000000000, 1.000000000000000000 ) ) ;
#27536=CARTESIAN_POINT ( 'NONE',  ( 105.1007409166104054, -25.80476224416663200, 275.2061014663870537 ) ) ;
#27537=ORIENTED_EDGE ( 'NONE', *, *, #74129, .F. ) ;
#27538=EDGE_CURVE ( 'NONE', #59703, #18271, #66743, .T. ) ;
#27539=CARTESIAN_POINT ( 'NONE',  ( 101.1158614047228070, -28.69863163947533735, 195.5838086201111992 ) ) ;
#27540=CARTESIAN_POINT ( 'NONE',  ( 99.03713458771083822, -43.41345219906346387, 116.8784824187679732 ) ) ;
#27541=CARTESIAN_POINT ( 'NONE',  ( 96.95674990518240577, -32.26097187787489418, 51.98324432352996638 ) ) ;
#27542=CARTESIAN_POINT ( 'NONE',  ( 97.34161151642148013, -42.07962167312376067, 172.7146728949589942 ) ) ;
#27543=CARTESIAN_POINT ( 'NONE',  ( 97.06107112666785497, -37.99641220746794090, 32.42729196197263519 ) ) ;
#27544=DIRECTION ( 'NONE',  ( 1.000000000000000078E-15, -1.000000000000000083E-30, -1.000000000000000000 ) ) ;
#27545=AXIS2_PLACEMENT_3D ( 'NONE', #45534, #54136, #39634 ) ;
#27546=DIRECTION ( 'NONE',  ( -1.000000000000000000, -6.493183223601999383E-14, -1.000000000000000078E-15 ) ) ;
#27548=CARTESIAN_POINT ( 'NONE',  ( 116.3135867418571650, -32.94878190598771539, 189.1356252759109680 ) ) ;
#27549=DIRECTION ( 'NONE',  ( 0.000000000000000000, 0.000000000000000000, 1.000000000000000000 ) ) ;
#27550=ORIENTED_EDGE ( 'NONE', *, *, #40858, .F. ) ;
#27552=EDGE_CURVE ( 'NONE', #60401, #44708, #3625, .T. ) ;
#27553=ORIENTED_EDGE ( 'NONE', *, *, #3237, .F. ) ;
#27555=VECTOR ( 'NONE', #84690, 1000.000000000000000 ) ;
#27556=ORIENTED_EDGE ( 'NONE', *, *, #23918, .T. ) ;
#27557=CARTESIAN_POINT ( 'NONE',  ( 134.5667039024480118, -50.82844715994100682, 280.9178068554149945 ) ) ;
#27558=CARTESIAN_POINT ( 'NONE',  ( 116.6546583390152279, -32.60254457569000408, 75.14991099019697174 ) ) ;
#27561=VECTOR ( 'NONE', #79741, 1000.000000000000000 ) ;
#27562=FACE_OUTER_BOUND ( 'NONE', #82490, .T. ) ;
#27563=CARTESIAN_POINT ( 'NONE',  ( 116.8358708857152095, -40.58912082693117185, 189.5270538473389479 ) ) ;
#27565=CARTESIAN_POINT ( 'NONE',  ( 98.95807093800334542, -41.73853705562144967, 11.76800622829293808 ) ) ;
#27569=VECTOR ( 'NONE', #70767, 1000.000000000000000 ) ;
#27570=EDGE_LOOP ( 'NONE', ( #68234, #41846, #25490, #89053, #84469 ) ) ;
#27572=CARTESIAN_POINT ( 'NONE',  ( 116.3262419368496978, -32.93860311337579105, 160.1356252759109680 ) ) ;
#27573=CARTESIAN_POINT ( 'NONE',  ( 109.7260717835659563, -27.00112607981847290, 19.86400788967373998 ) ) ;
#27574=DIRECTION ( 'NONE',  ( 0.000000000000000000, 1.000000000000000000, 0.000000000000000000 ) ) ;
#27576=DIRECTION ( 'NONE',  ( 0.000000000000000000, 0.000000000000000000, -1.000000000000000000 ) ) ;
#27577=VECTOR ( 'NONE', #8293, 1000.000000000000000 ) ;
#27579=CARTESIAN_POINT ( 'NONE',  ( 115.6529839569025455, -41.48189714014875307, 263.4241967044829948 ) ) ;
#27580=CARTESIAN_POINT ( 'NONE',  ( 193.0374249753376432, -23.42844715993431848, 193.9678068554150343 ) ) ;
#27581=ORIENTED_EDGE ( 'NONE', *, *, #88734, .T. ) ;
#27582=ADVANCED_FACE ( 'NONE', ( #45389 ), #18143, .F. ) ;
#27584=AXIS2_PLACEMENT_3D ( 'NONE', #50307, #8552, #56679 ) ;
#27586=DIRECTION ( 'NONE',  ( 1.387778780781444492E-15, 0.000000000000000000, -1.000000000000000000 ) ) ;
#27587=CARTESIAN_POINT ( 'NONE',  ( 98.46239236780679960, -37.66247686286469332, 79.21856656006798403 ) ) ;
#27590=DIRECTION ( 'NONE',  ( 0.000000000000000000, 1.000000000000000000, 0.000000000000000000 ) ) ;
#27591=EDGE_LOOP ( 'NONE', ( #54698, #59494, #49061, #89436 ) ) ;
#27592=CARTESIAN_POINT ( 'NONE',  ( 77.55659459556528645, -35.60518703965896492, 7.068229416970963186 ) ) ;
#27594=CARTESIAN_POINT ( 'NONE',  ( 118.9178230750475649, -36.92810663041961305, 153.8127681330539644 ) ) ;
#27596=CARTESIAN_POINT ( 'NONE',  ( 99.04406189553675688, -42.84125768779406229, 67.84395861402028061 ) ) ;
#27597=CARTESIAN_POINT ( 'NONE',  ( 99.34829255622855726, -41.08350393070648465, 133.1672975916119697 ) ) ;
#27598=CARTESIAN_POINT ( 'NONE',  ( 194.0371591254573502, -24.89890238294407965, 249.9678068554149775 ) ) ;
#27600=CARTESIAN_POINT ( 'NONE',  ( 107.3215613407866584, -25.65604926530302166, 71.04610146638795243 ) ) ;
#27601=EDGE_CURVE ( 'NONE', #30540, #87253, #67186, .T. ) ;
#27602=CARTESIAN_POINT ( 'NONE',  ( 117.0718954858506038, -35.46248235908498714, 84.92729194235329260 ) ) ;
#27603=ORIENTED_EDGE ( 'NONE', *, *, #80368, .F. ) ;
#27606=ORIENTED_EDGE ( 'NONE', *, *, #73041, .T. ) ;
#27609=ORIENTED_EDGE ( 'NONE', *, *, #44468, .T. ) ;
#27610=CARTESIAN_POINT ( 'NONE',  ( 116.8729656461675148, -36.55725972750698105, 288.8413395616257731 ) ) ;
#27611=CARTESIAN_POINT ( 'NONE',  ( 101.9613826146451885, -46.55915482862852173, 163.1832443235299763 ) ) ;
#27613=CARTESIAN_POINT ( 'NONE',  ( 97.31584371250237098, -39.30597598563051065, 142.5314586081371147 ) ) ;
#27614=CARTESIAN_POINT ( 'NONE',  ( 97.22566771925157525, -31.69632393854739760, 91.96229194257693962 ) ) ;
#27615=FACE_OUTER_BOUND ( 'NONE', #62197, .T. ) ;
#27616=ORIENTED_EDGE ( 'NONE', *, *, #27538, .F. ) ;
#27619=LINE ( 'NONE', #55302, #14318 ) ;
#27621=ORIENTED_EDGE ( 'NONE', *, *, #84101, .T. ) ;
#27622=CIRCLE ( 'NONE', #21875, 16.00000000000090239 ) ;
#27624=DIRECTION ( 'NONE',  ( -6.524622321627019585E-16, -4.013151879589939944E-16, -1.000000000000000000 ) ) ;
#27625=CARTESIAN_POINT ( 'NONE',  ( 115.3062145713272599, -45.21207857638187022, 268.1899109901965517 ) ) ;
#27626=DIRECTION ( 'NONE',  ( 1.000000000000000078E-15, -1.000000000000000083E-30, -1.000000000000000000 ) ) ;
#27628=CARTESIAN_POINT ( 'NONE',  ( 141.0664832912740110, -8.729447159940896483, 14.82207188531772957 ) ) ;
#27629=LINE ( 'NONE', #53963, #67892 ) ;
#27631=CARTESIAN_POINT ( 'NONE',  ( 110.9231077663976066, -44.92578233336853799, 287.3371817328388147 ) ) ;
#27632=CARTESIAN_POINT ( 'NONE',  ( 116.1804594027163517, -40.96476762480074996, 6.826283056785800163 ) ) ;
#27633=CARTESIAN_POINT ( 'NONE',  ( 103.3702027031294648, -47.12181610991854086, 98.31657765686297523 ) ) ;
#27635=CARTESIAN_POINT ( 'NONE',  ( 107.6554820827327461, -47.17179587048914158, 152.6213395616249500 ) ) ;
#27637=ORIENTED_EDGE ( 'NONE', *, *, #45866, .F. ) ;
#27638=CIRCLE ( 'NONE', #18952, 2.517500000000005844 ) ;
#27639=DIRECTION ( 'NONE',  ( 0.000000000000000000, -1.000000000000000000, 0.000000000000000000 ) ) ;
#27640=EDGE_CURVE ( 'NONE', #80786, #23384, #67641, .T. ) ;
#27641=FACE_BOUND ( 'NONE', #89433, .T. ) ;
#27645=CARTESIAN_POINT ( 'NONE',  ( 117.7486274683349308, -39.74683136594191524, 143.6194347997209775 ) ) ;
#27646=VERTEX_POINT ( 'NONE', #47174 ) ;
#27648=CARTESIAN_POINT ( 'NONE',  ( 101.4135918642175369, -46.25467808933209568, 203.1622919425779514 ) ) ;
#27651=LINE ( 'NONE', #89441, #64835 ) ;
#27656=EDGE_LOOP ( 'NONE', ( #80474, #16810, #11390, #34051, #38172, #19813 ) ) ;
#27657=EDGE_CURVE ( 'NONE', #82307, #37791, #7213, .T. ) ;
#27662=DIRECTION ( 'NONE',  ( 1.639958061481212836E-42, -4.100000000000000342E-29, -1.000000000000000000 ) ) ;
#27663=CARTESIAN_POINT ( 'NONE',  ( 101.4253818664906959, -46.23481170842615740, 203.1622919425779514 ) ) ;
#27664=CARTESIAN_POINT ( 'NONE',  ( 77.31648329127402519, -36.72944715994107412, -5.074374724089059541 ) ) ;
#27665=CARTESIAN_POINT ( 'NONE',  ( 135.0140782791311551, -16.14703303315377880, 1.764000745017878069 ) ) ;
#27666=B_SPLINE_CURVE_WITH_KNOTS ( 'NONE', 3,
 ( #39657, #11061, #4257, #60541, #25588, #80572, #31952, #66926, #4707, #32386, #60088, #87824, #53261, #81030, #46459, #11973, #32846, #13752, #15101, #75979, #41882, #42776, #84157, #34639, #47803, #20580, #48247, #34183, #55055, #20129, #62344, #83700, #40999, #69618, #82815, #69167, #63249, #35077, #41437, #21930, #61888, #75539, #70519, #6937, #13312, #42331, #124, #68719, #27823, #55502 ),
 .UNSPECIFIED., .F., .F.,
 ( 4, 2, 1, 1, 1, 1, 1, 2, 2, 2, 2, 2, 2, 2, 1, 1, 1, 1, 1, 1, 1, 2, 2, 2, 2, 2, 2, 2, 2, 2, 4 ),
 ( 0.5000148065476123227, 0.5002589399428646333, 0.5005030733381169439, 0.5009913401286217871, 0.5019678737096311405, 0.5039209408716495142, 0.5078270751956860396, 0.5156393438437590904, 0.5312638811399049699, 0.5625129557321965068, 0.6250111049167789146, 0.6875092541013613223, 0.7500074032859437301, 0.7500684366347565302, 0.7501294699835694413, 0.7502515366812014808, 0.7504956700764423561, 0.7509839368669025683, 0.7519604704478229928, 0.7539135376096571806, 0.7578196719333130105, 0.7656319405806258915, 0.7812564778752518757, 0.8125055524645015126, 0.8437546270537512605, 0.8750037016430010084, 0.9062527762322506453, 0.9375018508215002822, 0.9687509254107500301, 0.9843754627053750150, 1.000000000000000000 ),
 .UNSPECIFIED. ) ;
#27669=CARTESIAN_POINT ( 'NONE',  ( 20.56670390244833158, -48.82844715994187368, 249.9678068554150059 ) ) ;
#27672=VERTEX_POINT ( 'NONE', #68093 ) ;
#27674=FACE_OUTER_BOUND ( 'NONE', #2187, .T. ) ;
#27675=DIRECTION ( 'NONE',  ( 0.7071067811865516806, -0.7071067811865434649, 7.071067811865511818E-16 ) ) ;
#27676=CARTESIAN_POINT ( 'NONE',  ( 97.40895461294502411, -34.98419235835276453, 237.1841967044819626 ) ) ;
#27678=CARTESIAN_POINT ( 'NONE',  ( 102.0841886111852688, -27.63463957783716651, 96.46324432352997746 ) ) ;
#27681=CARTESIAN_POINT ( 'NONE',  ( 115.1188116510141128, -30.76893447370202139, 20.33360764784250208 ) ) ;
#27682=AXIS2_PLACEMENT_3D ( 'NONE', #71255, #1306, #36271 ) ;
#27683=EDGE_LOOP ( 'NONE', ( #30737, #29118, #75522, #32618, #76434, #15389, #64611, #88332, #85353, #38240, #82362, #48608, #11370, #70577, #82651, #63418, #38392, #80158, #30370, #41551, #31009, #84221, #59569, #84338, #67190, #6136, #65853, #11174, #74473, #89284, #30884, #69449, #9945, #53652, #64707, #61325, #29034, #1146, #77022, #46230, #13388, #82990, #39671, #69180, #69937, #42062, #66931, #16182 ) ) ;
#27684=CARTESIAN_POINT ( 'NONE',  ( 45.56670390244828184, -48.82844715994087892, 300.4678068554150059 ) ) ;
#27687=EDGE_CURVE ( 'NONE', #18505, #42340, #61266, .T. ) ;
#27689=CARTESIAN_POINT ( 'NONE',  ( 107.8719782714504873, -26.68843711164719323, 261.4444404487539941 ) ) ;
#27690=AXIS2_PLACEMENT_3D ( 'NONE', #838, #28527, #35793 ) ;
#27691=CARTESIAN_POINT ( 'NONE',  ( 172.5664832912729878, -27.82844715994070484, 138.9256252759119832 ) ) ;
#27692=CARTESIAN_POINT ( 'NONE',  ( 115.8251266376895074, -31.72949007719681092, 139.2398401005303299 ) ) ;
#27694=LINE ( 'NONE', #8153, #45894 ) ;
#27695=VERTEX_POINT ( 'NONE', #34901 ) ;
#27697=CARTESIAN_POINT ( 'NONE',  ( 97.81170003938157720, -40.51743348276853851, 42.63567940883270069 ) ) ;
#27698=VERTEX_POINT ( 'NONE', #62613 ) ;
#27699=CARTESIAN_POINT ( 'NONE',  ( 97.80902780829600829, -29.33079837672297074, 45.78991099019697231 ) ) ;
#27700=ORIENTED_EDGE ( 'NONE', *, *, #45860, .F. ) ;
#27701=CARTESIAN_POINT ( 'NONE',  ( 114.4813385407417741, -41.19272473522806166, 276.2014237029247852 ) ) ;
#27702=VECTOR ( 'NONE', #56323, 1000.000000000000000 ) ;
#27703=CARTESIAN_POINT ( 'NONE',  ( 117.0611684525443650, -38.07849049335855085, 128.7190349916091066 ) ) ;
#27704=CARTESIAN_POINT ( 'NONE',  ( 116.9310496459150244, -33.53114825773879915, 134.0880062282919880 ) ) ;
#27705=EDGE_CURVE ( 'NONE', #21321, #24090, #88987, .T. ) ;
#27708=PLANE ( 'NONE',  #5723 ) ;
#27710=CARTESIAN_POINT ( 'NONE',  ( 96.20418022731425367, -34.44737123974878301, 257.1737205140064475 ) ) ;
#27711=PLANE ( 'NONE',  #89179 ) ;
#27713=EDGE_CURVE ( 'NONE', #8740, #50121, #48071, .T. ) ;
#27716=CARTESIAN_POINT ( 'NONE',  ( 109.2641226286370824, -47.00117516105910198, 103.7441967044829880 ) ) ;
#27718=VERTEX_POINT ( 'NONE', #54425 ) ;
#27719=EDGE_LOOP ( 'NONE', ( #49376, #77465, #88450, #30685 ) ) ;
#27720=ORIENTED_EDGE ( 'NONE', *, *, #76037, .F. ) ;
#27722=CARTESIAN_POINT ( 'NONE',  ( 172.5664832912729878, -27.82844715994070484, 18.92562527591200094 ) ) ;
#27725=DIRECTION ( 'NONE',  ( -1.000000000000000078E-15, 1.000000000000000083E-30, 1.000000000000000000 ) ) ;
#27726=CARTESIAN_POINT ( 'NONE',  ( 114.8576755932693487, -34.29489411463138282, 171.8852332267339591 ) ) ;
#27727=CARTESIAN_POINT ( 'NONE',  ( 96.51501197915654018, -40.09867661842082498, 277.5603871806729899 ) ) ;
#27728=CARTESIAN_POINT ( 'NONE',  ( 108.3317990709242480, -46.73504955168621677, 58.67715742008988400 ) ) ;
#27730=CARTESIAN_POINT ( 'NONE',  ( 80.54920390244802775, -43.72944715994108833, 231.5838068554169524 ) ) ;
#27731=PLANE ( 'NONE',  #73696 ) ;
#27732=ORIENTED_EDGE ( 'NONE', *, *, #61778, .T. ) ;
#27733=ORIENTED_EDGE ( 'NONE', *, *, #60852, .F. ) ;
#27735=CARTESIAN_POINT ( 'NONE',  ( 36.23715912545344509, -47.82818131006131779, 129.9678068554150911 ) ) ;
#27736=FACE_OUTER_BOUND ( 'NONE', #2199, .T. ) ;
#27737=CARTESIAN_POINT ( 'NONE',  ( 109.7248310533103819, -27.00079495799194973, 14.86479478277475863 ) ) ;
#27738=DIRECTION ( 'NONE',  ( 1.000000000000000078E-15, -1.000000000000000083E-30, -1.000000000000000000 ) ) ;
#27739=DIRECTION ( 'NONE',  ( 0.000000000000000000, 0.000000000000000000, 1.000000000000000000 ) ) ;
#27741=CARTESIAN_POINT ( 'NONE',  ( 115.0373743241724327, -39.87857374794037923, 192.9495626852199450 ) ) ;
#27742=CARTESIAN_POINT ( 'NONE',  ( 107.3221093067165128, -25.63226107660779007, 75.04610146638695767 ) ) ;
#27744=VERTEX_POINT ( 'NONE', #47626 ) ;
#27745=EDGE_CURVE ( 'NONE', #69050, #45263, #40820, .T. ) ;
#27746=LINE ( 'NONE', #76799, #51333 ) ;
#27750=ADVANCED_FACE ( 'NONE', ( #68542 ), #6311, .F. ) ;
#27752=CARTESIAN_POINT ( 'NONE',  ( 182.3467384525650061, -29.62846900982231446, -5.074374724088000832 ) ) ;
#27753=LINE ( 'NONE', #84084, #48754 ) ;
#27754=CARTESIAN_POINT ( 'NONE',  ( 116.3185006702053244, -32.93849971620830530, 275.1356252759109680 ) ) ;
#27757=ORIENTED_EDGE ( 'NONE', *, *, #76446, .T. ) ;
#27759=CARTESIAN_POINT ( 'NONE',  ( 117.1128946550982732, -32.06414332788899912, 59.16038718067295576 ) ) ;
#27761=FACE_OUTER_BOUND ( 'NONE', #69057, .T. ) ;
#27762=CARTESIAN_POINT ( 'NONE',  ( 128.0667039024480118, -48.82844715994099971, 198.9178068554149945 ) ) ;
#27763=CARTESIAN_POINT ( 'NONE',  ( 57.56670390244829605, -48.82844715994039575, 293.2178068554150627 ) ) ;
#27764=ORIENTED_EDGE ( 'NONE', *, *, #28406, .T. ) ;
#27766=AXIS2_PLACEMENT_3D ( 'NONE', #80384, #65404, #86745 ) ;
#27768=CARTESIAN_POINT ( 'NONE',  ( 184.5667039024486087, -48.82844715993447693, 129.9678068554150059 ) ) ;
#27769=DIRECTION ( 'NONE',  ( 0.000000000000000000, 0.000000000000000000, 1.000000000000000000 ) ) ;
#27771=CARTESIAN_POINT ( 'NONE',  ( 117.6173583669683040, -42.17933576662011319, 89.44705384733997278 ) ) ;
#27772=DIRECTION ( 'NONE',  ( 0.000000000000000000, 0.000000000000000000, 1.000000000000000000 ) ) ;
#27776=ORIENTED_EDGE ( 'NONE', *, *, #36572, .T. ) ;
#27777=CARTESIAN_POINT ( 'NONE',  ( 112.9441315310008918, -44.54716313336194844, 139.0899109901959605 ) ) ;
#27778=LINE ( 'NONE', #7345, #82019 ) ;
#27779=EDGE_LOOP ( 'NONE', ( #56418, #78714, #75814, #55871 ) ) ;
#27780=CIRCLE ( 'NONE', #64043, 3.000000000000002665 ) ;
#27781=CARTESIAN_POINT ( 'NONE',  ( 99.39760893136107711, -29.69972230079153519, 271.7356252759109907 ) ) ;
#27783=CARTESIAN_POINT ( 'NONE',  ( 61.56670390244634916, -23.42844715994043270, 180.4678068554151196 ) ) ;
#27785=DIRECTION ( 'NONE',  ( -4.825893423866870279E-33, 0.000000000000000000, 1.000000000000000000 ) ) ;
#27788=CARTESIAN_POINT ( 'NONE',  ( 112.7790632652332050, -27.19118669266615740, 204.6470538473399756 ) ) ;
#27789=EDGE_LOOP ( 'NONE', ( #2513, #32382, #26104, #69073 ) ) ;
#27790=CIRCLE ( 'NONE', #80011, 1.000000000000000888 ) ;
#27792=ADVANCED_FACE ( 'NONE', ( #20836 ), #41704, .T. ) ;
#27793=CARTESIAN_POINT ( 'NONE',  ( 111.9232213988593827, -44.14162454355680865, 174.4701547344689629 ) ) ;
#27794=AXIS2_PLACEMENT_3D ( 'NONE', #19907, #28052, #47142 ) ;
#27796=CARTESIAN_POINT ( 'NONE',  ( 102.2363890476183599, -29.29987999758196793, 21.96729759161197748 ) ) ;
#27799=CARTESIAN_POINT ( 'NONE',  ( 98.30751288258193199, -41.72882199423717253, 266.7398595753476798 ) ) ;
#27800=CARTESIAN_POINT ( 'NONE',  ( 131.0667039024480118, -61.87844715994100397, 207.5838068554149913 ) ) ;
#27802=FACE_OUTER_BOUND ( 'NONE', #58553, .T. ) ;
#27803=CARTESIAN_POINT ( 'NONE',  ( 106.9407056411434951, -47.75886249174727283, 232.5794347997199907 ) ) ;
#27804=LINE ( 'NONE', #34618, #50344 ) ;
#27810=CARTESIAN_POINT ( 'NONE',  ( 97.81442241246865876, -40.52410417640054874, 122.6357492958329374 ) ) ;
#27811=DIRECTION ( 'NONE',  ( 0.000000000000000000, 0.000000000000000000, -1.000000000000000000 ) ) ;
#27812=VECTOR ( 'NONE', #57816, 1000.000000000000114 ) ;
#27813=DIRECTION ( 'NONE',  ( 0.000000000000000000, 0.000000000000000000, 1.000000000000000000 ) ) ;
#27814=ORIENTED_EDGE ( 'NONE', *, *, #16336, .T. ) ;
#27817=CARTESIAN_POINT ( 'NONE',  ( 98.38769172161842391, -42.09058819985752109, 7.768006228291934434 ) ) ;
#27818=CARTESIAN_POINT ( 'NONE',  ( 96.76314818047262634, -35.13937921927007579, 266.2041967044821149 ) ) ;
#27819=ORIENTED_EDGE ( 'NONE', *, *, #71848, .T. ) ;
#27820=AXIS2_PLACEMENT_3D ( 'NONE', #49855, #14468, #84418 ) ;
#27821=CARTESIAN_POINT ( 'NONE',  ( 77.33333279747652966, -37.08363404521340101, 6.775960187534254331 ) ) ;
#27823=CARTESIAN_POINT ( 'NONE',  ( 116.5674885483476402, -33.54335893859623496, 169.0838757843391136 ) ) ;
#27825=CARTESIAN_POINT ( 'NONE',  ( 115.0531750927473951, -38.41541278395968817, 61.47951894101993986 ) ) ;
#27826=CARTESIAN_POINT ( 'NONE',  ( 117.8230732226064532, -34.08729308082334342, 160.0061014663869798 ) ) ;
#27828=CARTESIAN_POINT ( 'NONE',  ( 41.56648329127399677, 0.2215528400590013880, 18.92562527591200094 ) ) ;
#27831=VERTEX_POINT ( 'NONE', #57126 ) ;
#27832=ORIENTED_EDGE ( 'NONE', *, *, #57793, .T. ) ;
#27834=EDGE_LOOP ( 'NONE', ( #32768, #3287, #42788, #14069 ) ) ;
#27837=ADVANCED_FACE ( 'NONE', ( #69883 ), #76699, .F. ) ;
#27838=CARTESIAN_POINT ( 'NONE',  ( 115.5093363421805606, -33.45364150533647063, 93.53146744712398686 ) ) ;
#27839=CARTESIAN_POINT ( 'NONE',  ( 100.8099727397313217, -45.87009904342127697, 242.1108633711489517 ) ) ;
#27840=CARTESIAN_POINT ( 'NONE',  ( 116.3579325164319869, -41.40893824611053020, 203.4556252759109611 ) ) ;
#27841=CARTESIAN_POINT ( 'NONE',  ( 109.6376038899290393, -46.81002275840752702, 43.77562527591094721 ) ) ;
#27842=CARTESIAN_POINT ( 'NONE',  ( 20.03715912545824906, -46.82818131006190043, 249.9678068554150059 ) ) ;
#27844=CARTESIAN_POINT ( 'NONE',  ( 115.0351357599961375, -42.91115358527014934, 94.30202127052717742 ) ) ;
#27845=EDGE_CURVE ( 'NONE', #70274, #11434, #29898, .T. ) ;
#27850=CARTESIAN_POINT ( 'NONE',  ( 101.8448680821487073, -28.45912855063583891, 110.5241967044829892 ) ) ;
#27851=CARTESIAN_POINT ( 'NONE',  ( 118.0484485056734769, -38.34478726580598362, 73.72229194257801055 ) ) ;
#27852=CARTESIAN_POINT ( 'NONE',  ( 115.9443088281525149, -30.06633247050010382, 264.3508633711492735 ) ) ;
#27854=CARTESIAN_POINT ( 'NONE',  ( 117.4744730450754560, -36.12879772292662039, 228.8727681330539667 ) ) ;
#27855=FACE_OUTER_BOUND ( 'NONE', #79483, .T. ) ;
#27858=DIRECTION ( 'NONE',  ( 0.000000000000000000, 1.000000000000000000, 0.000000000000000000 ) ) ;
#27859=DIRECTION ( 'NONE',  ( -1.000000000000000078E-15, 1.000000000000000083E-30, 1.000000000000000000 ) ) ;
#27860=CARTESIAN_POINT ( 'NONE',  ( 106.5510518188671227, -25.28190781890620542, 320.5359728645732389 ) ) ;
#27862=B_SPLINE_CURVE_WITH_KNOTS ( 'NONE', 3,
 ( #84773, #35247, #2542, #63874, #77953, #14833, #62956, #84332, #43401, #83415, #28438, #15274, #57032, #77494, #50218, #42951, #8920, #42501 ),
 .UNSPECIFIED., .F., .F.,
 ( 4, 2, 2, 2, 2, 2, 2, 2, 4 ),
 ( 0.000000000000000000, 0.06249999995315230761, 0.1249999999063046152, 0.1874999998594569228, 0.2499999998126092304, 0.3124999997657615380, 0.3749999997189138456, 0.4374999996720661533, 0.4999999996252184609 ),
 .UNSPECIFIED. ) ;
#27863=DIRECTION ( 'NONE',  ( 1.000000000000000078E-15, 1.000000000000000083E-30, -1.000000000000000000 ) ) ;
#27864=ADVANCED_FACE ( 'NONE', ( #9013 ), #57584, .F. ) ;
#27865=CARTESIAN_POINT ( 'NONE',  ( 90.44969454456403923, -20.11243780205715481, 239.5838068554169809 ) ) ;
#27866=ADVANCED_FACE ( 'NONE', ( #78509 ), #52288, .F. ) ;
#27867=CARTESIAN_POINT ( 'NONE',  ( 20.03715912545820288, -46.82818131006180096, 300.4678068554150059 ) ) ;
#27869=CIRCLE ( 'NONE', #85932, 0.5000000000000004441 ) ;
#27870=LINE ( 'NONE', #77370, #68969 ) ;
#27872=FACE_BOUND ( 'NONE', #59784, .T. ) ;
#27873=CARTESIAN_POINT ( 'NONE',  ( 109.9663390834669912, -48.24573355310754152, 242.7727681330539724 ) ) ;
#27874=CARTESIAN_POINT ( 'NONE',  ( 102.0818258798731506, -27.57325825325154867, 141.4727681330539895 ) ) ;
#27875=CARTESIAN_POINT ( 'NONE',  ( 118.7023651333632159, -39.22291191012653400, 254.6584824187681022 ) ) ;
#27876=LINE ( 'NONE', #20627, #40240 ) ;
#27878=CARTESIAN_POINT ( 'NONE',  ( 82.80005790026068269, -36.42904715602206522, 6.774297104452852381 ) ) ;
#27881=DIRECTION ( 'NONE',  ( -0.9834602067153815907, -0.1811243269341220596, 0.000000000000000000 ) ) ;
#27882=AXIS2_PLACEMENT_3D ( 'NONE', #47488, #53841, #82054 ) ;
#27884=CYLINDRICAL_SURFACE ( 'NONE', #27304, 9.999999999999998224 ) ;
#27885=VERTEX_POINT ( 'NONE', #8558 ) ;
#27887=CARTESIAN_POINT ( 'NONE',  ( 100.6939357996894557, -31.04202505589751837, 190.1695626852199439 ) ) ;
#27888=DIRECTION ( 'NONE',  ( -2.999999999999999839E-15, 1.000000000000000000, -2.999999999999999900E-30 ) ) ;
#27889=EDGE_LOOP ( 'NONE', ( #26600, #53703, #23792, #41445 ) ) ;
#27890=CARTESIAN_POINT ( 'NONE',  ( 164.9190312289449878, -35.91149509761181235, -5.074374724088000832 ) ) ;
#27891=CARTESIAN_POINT ( 'NONE',  ( 98.18688568738953393, -31.30898482519909365, 166.8899109901969950 ) ) ;
#27892=DIRECTION ( 'NONE',  ( -0.0001713722455994998422, 0.9999999853157766072, 0.000000000000000000 ) ) ;
#27893=DIRECTION ( 'NONE',  ( -4.237773401492740281E-14, 1.000000000000000000, 0.000000000000000000 ) ) ;
#27895=CARTESIAN_POINT ( 'NONE',  ( 116.0343967343886504, -32.24059753838103859, 85.19573006588439057 ) ) ;
#27897=DIRECTION ( 'NONE',  ( 0.7071067811865758834, -0.7071067811865192621, 7.071067811865765240E-16 ) ) ;
#27898=CARTESIAN_POINT ( 'NONE',  ( 108.4470127171752125, -27.04659769318750762, 104.9641967044829869 ) ) ;
#27902=CARTESIAN_POINT ( 'NONE',  ( 106.9482176359816634, -27.83854490981203256, 56.51872616303998598 ) ) ;
#27903=PLANE ( 'NONE',  #41370 ) ;
#27904=CARTESIAN_POINT ( 'NONE',  ( 97.99937763885738207, -40.39701179870334613, 202.6327681330529629 ) ) ;
#27907=CARTESIAN_POINT ( 'NONE',  ( 41.56648329127398966, -27.82844715994070484, 78.92562527591199739 ) ) ;
#27908=EDGE_CURVE ( 'NONE', #28327, #8825, #1294, .T. ) ;
#27909=DIRECTION ( 'NONE',  ( 0.000000000000000000, 0.000000000000000000, -1.000000000000000000 ) ) ;
#27910=CIRCLE ( 'NONE', #68574, 0.5000000000000073275 ) ;
#27911=DIRECTION ( 'NONE',  ( 1.000000000000000078E-15, -1.000000000000000083E-30, -1.000000000000000000 ) ) ;
#27913=CARTESIAN_POINT ( 'NONE',  ( 99.70004787478420383, -45.98060041612311721, 122.0413395616249659 ) ) ;
#27914=EDGE_LOOP ( 'NONE', ( #73979, #34940, #6964, #76147, #68824, #64288, #71338, #84818, #10416, #68186, #42179, #53112, #86580, #10718, #71184, #29498 ) ) ;
#27916=VERTEX_POINT ( 'NONE', #2643 ) ;
#27917=LINE ( 'NONE', #16100, #38652 ) ;
#27918=FACE_OUTER_BOUND ( 'NONE', #40727, .T. ) ;
#27920=CARTESIAN_POINT ( 'NONE',  ( 115.1682430951150735, -35.73384980259207566, 191.7423760838769908 ) ) ;
#27923=CARTESIAN_POINT ( 'NONE',  ( 179.1667039024460166, -28.27351298637280408, -5.074374724088000832 ) ) ;
#27924=CARTESIAN_POINT ( 'NONE',  ( 48.45959712127301344, -26.00627455219131789, 313.9678068554150059 ) ) ;
#27925=ORIENTED_EDGE ( 'NONE', *, *, #58031, .T. ) ;
#27930=VERTEX_POINT ( 'NONE', #84428 ) ;
#27931=LINE ( 'NONE', #76538, #75365 ) ;
#27932=EDGE_CURVE ( 'NONE', #6555, #71592, #36258, .T. ) ;
#27933=AXIS2_PLACEMENT_3D ( 'NONE', #69718, #34736, #62443 ) ;
#27934=CARTESIAN_POINT ( 'NONE',  ( 104.7356562592608498, -27.62759180600148667, 241.7196785439919609 ) ) ;
#27935=ADVANCED_FACE ( 'NONE', ( #58038 ), #8106, .F. ) ;
#27937=LINE ( 'NONE', #42004, #18896 ) ;
#27939=VERTEX_POINT ( 'NONE', #48958 ) ;
#27941=CONICAL_SURFACE ( 'NONE', #12000, 1.258750000000002922, 1.029744258676650093 ) ;
#27942=LINE ( 'NONE', #75207, #69606 ) ;
#27945=ADVANCED_FACE ( 'NONE', ( #56222 ), #78058, .F. ) ;
#27946=VECTOR ( 'NONE', #31098, 1000.000000000000000 ) ;
#27947=CARTESIAN_POINT ( 'NONE',  ( 105.9433607271350439, -44.81451498420922519, 255.2852332267341353 ) ) ;
#27948=CARTESIAN_POINT ( 'NONE',  ( 108.7467888895124162, -25.78085441620226348, 144.9432443235299672 ) ) ;
#27949=CARTESIAN_POINT ( 'NONE',  ( 110.1514708964275968, -46.66481413883396812, 97.81562527591097478 ) ) ;
#27950=CARTESIAN_POINT ( 'NONE',  ( 116.4947067722135188, -39.72538118426291476, 249.5838068554167819 ) ) ;
#27951=DIRECTION ( 'NONE',  ( 2.900000000000000265E-14, -2.000000000000000155E-15, 1.000000000000000000 ) ) ;
#27952=CARTESIAN_POINT ( 'NONE',  ( 113.7992560408602145, -26.97729936261201900, 235.5956252759109759 ) ) ;
#27953=CARTESIAN_POINT ( 'NONE',  ( 160.5667039024429243, -48.82844715994099971, 129.9678068554149775 ) ) ;
#27954=ADVANCED_FACE ( 'NONE', ( #43046 ), #63969, .T. ) ;
#27955=LINE ( 'NONE', #70651, #208 ) ;
#27958=ORIENTED_EDGE ( 'NONE', *, *, #17456, .F. ) ;
#27959=EDGE_LOOP ( 'NONE', ( #23355, #68983, #35646, #66886 ) ) ;
#27961=CARTESIAN_POINT ( 'NONE',  ( 103.6874411509537595, -27.31610070321936234, 136.3507228384528105 ) ) ;
#27962=CARTESIAN_POINT ( 'NONE',  ( 97.57106248370669732, -31.07117258718254149, 130.9108633711489915 ) ) ;
#27966=CARTESIAN_POINT ( 'NONE',  ( 162.9033555647783658, -33.89581943343814174, 313.9678068554149490 ) ) ;
#27968=CARTESIAN_POINT ( 'NONE',  ( 103.6457867198658391, -26.24313906103854066, 206.3394347997209763 ) ) ;
#27969=DIRECTION ( 'NONE',  ( -0.04216478779797398074, 0.9991106698809455455, 0.000000000000000000 ) ) ;
#27974=VECTOR ( 'NONE', #1549, 1000.000000000000000 ) ;
#27976=ADVANCED_FACE ( 'NONE', ( #30779 ), #65305, .T. ) ;
#27977=DIRECTION ( 'NONE',  ( 0.000000000000000000, 1.000000000000000000, 0.000000000000000000 ) ) ;
#27978=EDGE_CURVE ( 'NONE', #31607, #68056, #31665, .T. ) ;
#27979=DIRECTION ( 'NONE',  ( 0.000000000000000000, 0.000000000000000000, 1.000000000000000000 ) ) ;
#27980=CARTESIAN_POINT ( 'NONE',  ( 105.7708979221677197, -26.34060099707374292, 270.1756252759109884 ) ) ;
#27981=VERTEX_POINT ( 'NONE', #25296 ) ;
#27983=CARTESIAN_POINT ( 'NONE',  ( 114.2552021840540846, -45.16177683379865471, 153.1508633711489722 ) ) ;
#27984=CARTESIAN_POINT ( 'NONE',  ( 107.1953983157108041, -26.30515493630308654, 31.06705384733893283 ) ) ;
#27985=CARTESIAN_POINT ( 'NONE',  ( 114.3743266858445935, -29.18402207539437399, 170.4641967044829585 ) ) ;
#27986=EDGE_CURVE ( 'NONE', #59735, #65816, #19865, .T. ) ;
#27987=CYLINDRICAL_SURFACE ( 'NONE', #18413, 9.999999999999998224 ) ;
#27989=CARTESIAN_POINT ( 'NONE',  ( 50.96943157743499597, -34.03355364505720360, 313.9678068554150059 ) ) ;
#27993=ORIENTED_EDGE ( 'NONE', *, *, #48300, .T. ) ;
#27994=CIRCLE ( 'NONE', #78786, 2.750000000000002665 ) ;
#27995=CARTESIAN_POINT ( 'NONE',  ( 21.03715912545824551, -47.82818131006186491, 300.4678068554150059 ) ) ;
#27996=EDGE_LOOP ( 'NONE', ( #5231, #23731, #24434, #70641 ) ) ;
#27999=CARTESIAN_POINT ( 'NONE',  ( 107.8666756518570793, -26.35696637107995954, 66.01562527591097762 ) ) ;
#28000=PLANE ( 'NONE',  #65819 ) ;
#28002=CARTESIAN_POINT ( 'NONE',  ( 109.8676264040644526, -26.64249633179236909, 170.8613395616249591 ) ) ;
#28003=CARTESIAN_POINT ( 'NONE',  ( 101.4793796374089965, -43.85664460571122447, 276.4819436376007502 ) ) ;
#28004=ORIENTED_EDGE ( 'NONE', *, *, #81789, .F. ) ;
#28008=CARTESIAN_POINT ( 'NONE',  ( 80.06648329127398256, -8.729447159941058132, 4.925625275910944012 ) ) ;
#28010=FACE_OUTER_BOUND ( 'NONE', #53846, .T. ) ;
#28011=TOROIDAL_SURFACE ( 'NONE', #78810, 13.50000000000000000, 0.5000000000000000000 ) ;
#28015=VECTOR ( 'NONE', #16327, 1000.000000000000000 ) ;
#28016=CARTESIAN_POINT ( 'NONE',  ( 41.56648329127398966, -27.82844715994070484, 18.92562527591200094 ) ) ;
#28017=CARTESIAN_POINT ( 'NONE',  ( 163.0664832912739826, 19.62155284005901024, 333.4006252759110112 ) ) ;
#28018=CARTESIAN_POINT ( 'NONE',  ( 100.5643946202652330, -27.81952766013690237, 30.56610146638794134 ) ) ;
#28020=ORIENTED_EDGE ( 'NONE', *, *, #74936, .T. ) ;
#28022=DIRECTION ( 'NONE',  ( -1.000000000000000000, 6.036837696399408848E-13, 0.000000000000000000 ) ) ;
#28023=CARTESIAN_POINT ( 'NONE',  ( 115.1349747707284479, -33.59889284931170295, 91.92713798863898944 ) ) ;
#28025=AXIS2_PLACEMENT_3D ( 'NONE', #77726, #43622, #8688 ) ;
#28026=EDGE_CURVE ( 'NONE', #88995, #70782, #58469, .T. ) ;
#28027=FACE_OUTER_BOUND ( 'NONE', #71865, .T. ) ;
#28031=ADVANCED_FACE ( 'NONE', ( #10339 ), #67083, .F. ) ;
#28032=FACE_OUTER_BOUND ( 'NONE', #63560, .T. ) ;
#28035=EDGE_CURVE ( 'NONE', #84376, #68878, #52526, .T. ) ;
#28037=CARTESIAN_POINT ( 'NONE',  ( 98.17580767689473475, -36.86367352702462341, 132.7701547344679511 ) ) ;
#28039=CARTESIAN_POINT ( 'NONE',  ( 75.31670390244798341, -57.40094715994099772, 63.03480685541479289 ) ) ;
#28040=CARTESIAN_POINT ( 'NONE',  ( 113.3555096308132022, -27.61169779702804306, 85.60800622829195561 ) ) ;
#28042=LINE ( 'NONE', #35752, #19855 ) ;
#28043=ORIENTED_EDGE ( 'NONE', *, *, #86522, .T. ) ;
#28046=ORIENTED_EDGE ( 'NONE', *, *, #81708, .F. ) ;
#28047=ADVANCED_FACE ( 'NONE', ( #34344 ), #82085, .F. ) ;
#28048=PLANE ( 'NONE',  #32560 ) ;
#28049=VERTEX_POINT ( 'NONE', #60254 ) ;
#28050=CARTESIAN_POINT ( 'NONE',  ( 105.9660763718858618, -46.48152545022894344, 282.4870538473400643 ) ) ;
#28051=CARTESIAN_POINT ( 'NONE',  ( 102.3833470591291785, -26.69184581432750747, 131.4118157521009778 ) ) ;
#28052=DIRECTION ( 'NONE',  ( -2.900000000000000265E-14, 2.000000000000000155E-15, -1.000000000000000000 ) ) ;
#28053=CARTESIAN_POINT ( 'NONE',  ( 100.9546728181673245, -28.70702572214929305, 141.5939586085704036 ) ) ;
#28054=CARTESIAN_POINT ( 'NONE',  ( 96.79170515468972269, -38.49336940632627346, 87.46133956162493917 ) ) ;
#28057=VERTEX_POINT ( 'NONE', #33902 ) ;
#28059=CARTESIAN_POINT ( 'NONE',  ( 163.0664832912739826, -8.350947159940998787, 333.4006252759120343 ) ) ;
#28061=CONICAL_SURFACE ( 'NONE', #78873, 3.299999999999999822, 0.7853981633974602694 ) ;
#28063=CARTESIAN_POINT ( 'NONE',  ( 97.81461822720238786, -40.51595288653417981, 132.6359866545674890 ) ) ;
#28064=CARTESIAN_POINT ( 'NONE',  ( 97.80902780829600829, -29.33079837672297074, 45.78991099019697231 ) ) ;
#28065=CARTESIAN_POINT ( 'NONE',  ( 156.5667039024485803, -48.82844715993568485, 134.7178068554149775 ) ) ;
#28068=CARTESIAN_POINT ( 'NONE',  ( 110.8778723976570433, -46.37372517399798255, 22.88800622829195675 ) ) ;
#28070=CARTESIAN_POINT ( 'NONE',  ( 96.66376384204026806, -36.61947630124858932, 107.3184824187679567 ) ) ;
#28073=EDGE_LOOP ( 'NONE', ( #895, #80470, #39549, #33285 ) ) ;
#28075=CARTESIAN_POINT ( 'NONE',  ( 172.5664832912740110, -18.82844715994099971, 316.8086252759120498 ) ) ;
#28077=ORIENTED_EDGE ( 'NONE', *, *, #28549, .F. ) ;
#28078=EDGE_CURVE ( 'NONE', #18676, #69089, #59890, .T. ) ;
#28079=DIRECTION ( 'NONE',  ( 2.775557561562888827E-14, -1.000000000000000000, 0.000000000000000000 ) ) ;
#28080=CARTESIAN_POINT ( 'NONE',  ( 112.5090891374639313, -26.14611880238131647, 169.6984824187679521 ) ) ;
#28083=CARTESIAN_POINT ( 'NONE',  ( 110.0582552220427175, -26.06480902925029497, 215.8708633711489711 ) ) ;
#28084=EDGE_CURVE ( 'NONE', #667, #79585, #5314, .T. ) ;
#28088=ORIENTED_EDGE ( 'NONE', *, *, #61770, .T. ) ;
#28092=ORIENTED_EDGE ( 'NONE', *, *, #54370, .F. ) ;
#28093=VECTOR ( 'NONE', #81218, 1000.000000000000000 ) ;
#28095=CARTESIAN_POINT ( 'NONE',  ( 41.56670390244777735, -36.32844715994104234, 300.4678068554150059 ) ) ;
#28096=CARTESIAN_POINT ( 'NONE',  ( 116.9253062793529665, -41.72720563489927770, 244.4651490854349731 ) ) ;
#28097=CARTESIAN_POINT ( 'NONE',  ( 84.06648329127399677, -14.47844715994100007, 17.92562527591199739 ) ) ;
#28098=CARTESIAN_POINT ( 'NONE',  ( 135.7756147485513907, -16.57277681852953677, 2.101554741600898613 ) ) ;
#28099=CARTESIAN_POINT ( 'NONE',  ( 32.06670390244800473, -33.35206098992711077, -5.074374724088000832 ) ) ;
#28100=FACE_OUTER_BOUND ( 'NONE', #47164, .T. ) ;
#28101=CYLINDRICAL_SURFACE ( 'NONE', #22557, 9.999999999999998224 ) ;
#28102=CARTESIAN_POINT ( 'NONE',  ( 107.1956731390977779, -26.28293224109629733, 35.06705384733893283 ) ) ;
#28106=CARTESIAN_POINT ( 'NONE',  ( 89.06648138392532132, -56.72944715994137255, 14.82207188531717001 ) ) ;
#28107=CARTESIAN_POINT ( 'NONE',  ( 97.75826863619981566, -40.38458993153165011, 17.62397050589623859 ) ) ;
#28108=CARTESIAN_POINT ( 'NONE',  ( 106.9482321581270270, -47.09886382165559127, 228.5794347997199907 ) ) ;
#28110=CARTESIAN_POINT ( 'NONE',  ( 116.7176835877704093, -38.50936494796416554, 84.68133956162493803 ) ) ;
#28112=CARTESIAN_POINT ( 'NONE',  ( 97.60785906575104320, -39.98233608924685001, 22.59004718401966372 ) ) ;
#28113=EDGE_LOOP ( 'NONE', ( #74327, #50156, #86931, #37945 ) ) ;
#28114=DIRECTION ( 'NONE',  ( 0.000000000000000000, 0.000000000000000000, -1.000000000000000000 ) ) ;
#28115=ORIENTED_EDGE ( 'NONE', *, *, #43112, .F. ) ;
#28118=CARTESIAN_POINT ( 'NONE',  ( 111.0382984267975246, -28.80776997321336097, 276.1387261630399621 ) ) ;
#28119=VECTOR ( 'NONE', #80614, 1000.000000000000000 ) ;
#28120=CARTESIAN_POINT ( 'NONE',  ( 112.0659115712803668, -45.48839629059288825, 192.9897919379049256 ) ) ;
#28126=FACE_OUTER_BOUND ( 'NONE', #29309, .T. ) ;
#28127=ORIENTED_EDGE ( 'NONE', *, *, #68982, .F. ) ;
#28130=CARTESIAN_POINT ( 'NONE',  ( 116.7943018416943062, -39.39076309558235067, 184.6151407780641307 ) ) ;
#28131=EDGE_LOOP ( 'NONE', ( #46066, #81540, #32497, #46002, #64286, #9997 ) ) ;
#28132=CARTESIAN_POINT ( 'NONE',  ( 110.4566641872556403, -47.25017721759432732, 57.83657765686300678 ) ) ;
#28134=CARTESIAN_POINT ( 'NONE',  ( 114.5169583807067966, -41.13300932163210177, 281.2318998934008505 ) ) ;
#28137=CARTESIAN_POINT ( 'NONE',  ( 99.07755742602699911, -44.46178485432853478, 191.9384824187689560 ) ) ;
#28139=LINE ( 'NONE', #34959, #4131 ) ;
#28140=CARTESIAN_POINT ( 'NONE',  ( 46.83715912545424231, -47.82818131006082751, 300.4678068554150059 ) ) ;
#28141=DIRECTION ( 'NONE',  ( 3.999999999999999995E-14, -1.000000000000000000, 4.100000000000000342E-29 ) ) ;
#28142=CARTESIAN_POINT ( 'NONE',  ( 112.5120184049100089, -46.40124356417671692, 253.9965776568635647 ) ) ;
#28143=CARTESIAN_POINT ( 'NONE',  ( 109.7881854341049177, -46.37695241868441087, 117.7973390980168205 ) ) ;
#28144=EDGE_CURVE ( 'NONE', #11510, #80206, #48399, .T. ) ;
#28145=ORIENTED_EDGE ( 'NONE', *, *, #5223, .F. ) ;
#28146=DIRECTION ( 'NONE',  ( -4.237773401492740281E-14, 1.000000000000000000, 0.000000000000000000 ) ) ;
#28147=VECTOR ( 'NONE', #41427, 1000.000000000000000 ) ;
#28149=CARTESIAN_POINT ( 'NONE',  ( 113.1020477030913582, -28.17579636167772605, 125.5870538473399591 ) ) ;
#28151=AXIS2_PLACEMENT_3D ( 'NONE', #16611, #3870, #73343 ) ;
#28152=VECTOR ( 'NONE', #87520, 1000.000000000000000 ) ;
#28153=ORIENTED_EDGE ( 'NONE', *, *, #46579, .F. ) ;
#28154=ORIENTED_EDGE ( 'NONE', *, *, #4996, .F. ) ;
#28155=ORIENTED_EDGE ( 'NONE', *, *, #35643, .T. ) ;
#28158=DIRECTION ( 'NONE',  ( 1.639958061481212836E-42, -4.100000000000000342E-29, -1.000000000000000000 ) ) ;
#28159=CARTESIAN_POINT ( 'NONE',  ( 163.0667039024470171, -33.35206098992711077, -5.074374724088000832 ) ) ;
#28162=CARTESIAN_POINT ( 'NONE',  ( 50.56670390244699576, -18.82844715994031048, -5.074374724088000832 ) ) ;
#28163=CARTESIAN_POINT ( 'NONE',  ( 99.97311099609123630, -31.77112186149751949, 158.6471379886389741 ) ) ;
#28164=CARTESIAN_POINT ( 'NONE',  ( 96.54178838847580835, -40.18459672615917100, 282.5908633711491120 ) ) ;
#28165=EDGE_CURVE ( 'NONE', #39822, #62232, #75620, .T. ) ;
#28166=CARTESIAN_POINT ( 'NONE',  ( 19.56670390244829605, -47.82844715994191631, 249.9678068554150059 ) ) ;
#28170=ORIENTED_EDGE ( 'NONE', *, *, #22329, .F. ) ;
#28171=ORIENTED_EDGE ( 'NONE', *, *, #26512, .T. ) ;
#28176=CARTESIAN_POINT ( 'NONE',  ( 49.35211078757041747, -35.65087443489839814, 193.9678068554150911 ) ) ;
#28177=CARTESIAN_POINT ( 'NONE',  ( 98.60840819187967554, -35.53902818534925245, 180.6381341137909544 ) ) ;
#28178=CARTESIAN_POINT ( 'NONE',  ( 98.61163144626758026, -43.92169047526947168, 76.89943479971999807 ) ) ;
#28179=ORIENTED_EDGE ( 'NONE', *, *, #7035, .T. ) ;
#28183=ORIENTED_EDGE ( 'NONE', *, *, #59116, .F. ) ;
#28188=ADVANCED_FACE ( 'NONE', ( #33456 ), #61160, .T. ) ;
#28189=DIRECTION ( 'NONE',  ( 0.7071067811865514585, -0.7071067811865435759, 7.071067811865522665E-16 ) ) ;
#28190=AXIS2_PLACEMENT_3D ( 'NONE', #27763, #55443, #89555 ) ;
#28193=CARTESIAN_POINT ( 'NONE',  ( 104.0363141061766186, -47.38371934748259662, 67.36800622829191809 ) ) ;
#28198=DIRECTION ( 'NONE',  ( -4.299999999999999979E-14, 1.000000000000000000, -4.100000000000000342E-29 ) ) ;
#28199=CARTESIAN_POINT ( 'NONE',  ( 132.6481957738584754, -16.37139167074703039, 1.944749297856041670 ) ) ;
#28201=CARTESIAN_POINT ( 'NONE',  ( 106.3701732919943055, -26.72731777573979883, 121.1301100331873926 ) ) ;
#28202=CARTESIAN_POINT ( 'NONE',  ( 83.06670390244796920, -64.87844715994098976, 237.1838068554150141 ) ) ;
#28203=FACE_OUTER_BOUND ( 'NONE', #54331, .T. ) ;
#28206=CARTESIAN_POINT ( 'NONE',  ( 104.9584626277977577, -25.04276672576827778, 121.2184824187679766 ) ) ;
#28208=DIRECTION ( 'NONE',  ( -1.000000000000000078E-15, 1.000000000000000083E-30, 1.000000000000000000 ) ) ;
#28209=LINE ( 'NONE', #49096, #36426 ) ;
#28211=CIRCLE ( 'NONE', #73205, 9.571100913904325935 ) ;
#28212=AXIS2_PLACEMENT_3D ( 'NONE', #966, #21420, #35029 ) ;
#28214=VECTOR ( 'NONE', #74232, 1000.000000000000000 ) ;
#28216=CARTESIAN_POINT ( 'NONE',  ( 111.8077268321493278, -46.78591733285061594, 133.9270538473389536 ) ) ;
#28218=ORIENTED_EDGE ( 'NONE', *, *, #37722, .T. ) ;
#28221=CARTESIAN_POINT ( 'NONE',  ( 111.7292870705843342, -27.42961193919087748, 275.7070538473395800 ) ) ;
#28222=CARTESIAN_POINT ( 'NONE',  ( 25.56670390244797275, -62.87844715994099687, 173.2178068554149775 ) ) ;
#28223=DIRECTION ( 'NONE',  ( -0.7071067811865671127, -0.7071067811865279218, -7.071067811865664660E-16 ) ) ;
#28228=CARTESIAN_POINT ( 'NONE',  ( 97.48942487598446860, -34.74365074496812156, 216.1641967044829755 ) ) ;
#28230=ORIENTED_EDGE ( 'NONE', *, *, #19432, .F. ) ;
#28231=CARTESIAN_POINT ( 'NONE',  ( 99.92577194148378794, -31.43111053364522434, 177.2501547344679693 ) ) ;
#28232=DIRECTION ( 'NONE',  ( 0.000000000000000000, 0.000000000000000000, 1.000000000000000000 ) ) ;
#28233=CARTESIAN_POINT ( 'NONE',  ( 114.7948027157550399, -42.07682430429896669, 9.788249972563944468 ) ) ;
#28234=CARTESIAN_POINT ( 'NONE',  ( 134.0664832912739826, -18.72944715994100306, 14.92562527591099908 ) ) ;
#28235=AXIS2_PLACEMENT_3D ( 'NONE', #67391, #75117, #62374 ) ;
#28236=EDGE_CURVE ( 'NONE', #59735, #64543, #7554, .T. ) ;
#28237=ADVANCED_FACE ( 'NONE', ( #42493 ), #77486, .F. ) ;
#28241=ADVANCED_FACE ( 'NONE', ( #21183 ), #1186, .F. ) ;
#28242=DIRECTION ( 'NONE',  ( 0.7071067810573865575, 0.7071067813157084769, 7.071067810574170182E-16 ) ) ;
#28243=CARTESIAN_POINT ( 'NONE',  ( 110.0457755916377778, -26.10929462018208369, 219.8708633711489711 ) ) ;
#28250=CARTESIAN_POINT ( 'NONE',  ( 99.08956020682818178, -42.79551379493017293, 122.8430804584095455 ) ) ;
#28252=EDGE_CURVE ( 'NONE', #48540, #44152, #22531, .T. ) ;
#28255=VECTOR ( 'NONE', #48393, 999.9999999999998863 ) ;
#28256=CARTESIAN_POINT ( 'NONE',  ( 116.6059430675273063, -40.93488859202243901, 253.4956252759109532 ) ) ;
#28258=EDGE_CURVE ( 'NONE', #74870, #86147, #14740, .T. ) ;
#28259=CARTESIAN_POINT ( 'NONE',  ( 77.76764265987422675, -38.23887630718186159, 7.293197373623000246 ) ) ;
#28260=DIRECTION ( 'NONE',  ( -0.9254794337955620787, -0.3787978585227822492, 0.000000000000000000 ) ) ;
#28262=CARTESIAN_POINT ( 'NONE',  ( 108.5688297718456852, -44.75270591617022831, 80.54237608387698799 ) ) ;
#28263=CARTESIAN_POINT ( 'NONE',  ( 95.99102054923815786, -36.58347128883620059, 152.3280062282919971 ) ) ;
#28264=DIRECTION ( 'NONE',  ( 0.000000000000000000, 1.000000000000000000, 0.000000000000000000 ) ) ;
#28268=VERTEX_POINT ( 'NONE', #42941 ) ;
#28271=CARTESIAN_POINT ( 'NONE',  ( 172.5667039024478413, -36.32844715993500273, 249.9678068554149775 ) ) ;
#28272=AXIS2_PLACEMENT_3D ( 'NONE', #42523, #62536, #56610 ) ;
#28273=VERTEX_POINT ( 'NONE', #63404 ) ;
#28275=PLANE ( 'NONE',  #84641 ) ;
#28277=CARTESIAN_POINT ( 'NONE',  ( 106.5510518188671227, -25.28190781890620542, 320.5359728645732389 ) ) ;
#28278=CARTESIAN_POINT ( 'NONE',  ( 98.07131787375925569, -37.77809840677601017, 85.85337220902894728 ) ) ;
#28280=CARTESIAN_POINT ( 'NONE',  ( 115.4777400244682042, -29.52207584268309759, 229.4022919425779605 ) ) ;
#28282=CARTESIAN_POINT ( 'NONE',  ( 117.3921119255897452, -35.46056622170122097, 193.9241967044829664 ) ) ;
#28283=DIRECTION ( 'NONE',  ( -0.7071067811865165975, -0.7071067811865784369, -7.071067811865158803E-16 ) ) ;
#28286=CARTESIAN_POINT ( 'NONE',  ( 108.4144577094060082, -26.73465142943761919, 90.96919997473116837 ) ) ;
#28287=CARTESIAN_POINT ( 'NONE',  ( 130.0664832912740110, -18.82844715994099971, 284.9256252759119548 ) ) ;
#28289=CARTESIAN_POINT ( 'NONE',  ( 97.81443832832722762, -40.51607714565724905, 56.63519146330476417 ) ) ;
#28291=CARTESIAN_POINT ( 'NONE',  ( 109.1197153606379970, -46.32621810461561296, 107.7441967044829880 ) ) ;
#28292=CARTESIAN_POINT ( 'NONE',  ( 104.0299312746664526, -47.40616179873944702, 67.36800622829191809 ) ) ;
#28293=CARTESIAN_POINT ( 'NONE',  ( 115.8130859178907599, -30.97587361506452197, 254.2899109901966028 ) ) ;
#28294=ORIENTED_EDGE ( 'NONE', *, *, #80079, .T. ) ;
#28295=CARTESIAN_POINT ( 'NONE',  ( 115.3881169701508327, -30.44952332473371115, 219.3413395616249773 ) ) ;
#28298=FACE_OUTER_BOUND ( 'NONE', #80131, .T. ) ;
#28299=CARTESIAN_POINT ( 'NONE',  ( 108.4861102935399089, -46.16112076858227908, 277.6356252759110816 ) ) ;
#28300=CYLINDRICAL_SURFACE ( 'NONE', #25366, 3.000000000000002665 ) ;
#28302=FACE_OUTER_BOUND ( 'NONE', #37342, .T. ) ;
#28303=CARTESIAN_POINT ( 'NONE',  ( 151.5667039024536678, -48.82844715994099971, 180.4678068554149775 ) ) ;
#28305=CARTESIAN_POINT ( 'NONE',  ( 90.44969454456408187, -23.41243780205710578, 239.5838068554175209 ) ) ;
#28308=ORIENTED_EDGE ( 'NONE', *, *, #38503, .T. ) ;
#28310=CARTESIAN_POINT ( 'NONE',  ( 105.7736212422599777, -26.36243834887274673, 270.1756252759109884 ) ) ;
#28311=CARTESIAN_POINT ( 'NONE',  ( 117.3100215237039805, -34.79230872694400034, 154.9756252759109714 ) ) ;
#28312=CARTESIAN_POINT ( 'NONE',  ( 96.63726304471626349, -32.99895513370901057, 22.06514908543494258 ) ) ;
#28314=CARTESIAN_POINT ( 'NONE',  ( 20.03715912545645139, -24.42818131006202265, 117.4678068554150485 ) ) ;
#28315=CARTESIAN_POINT ( 'NONE',  ( 80.80620050779884878, -34.05355276379768981, 8.162233076795734732 ) ) ;
#28316=CARTESIAN_POINT ( 'NONE',  ( 100.8873625800001719, -44.70014081962553831, 138.0522817664394495 ) ) ;
#28320=CIRCLE ( 'NONE', #37096, 2.517500000000005844 ) ;
#28323=ORIENTED_EDGE ( 'NONE', *, *, #5909, .F. ) ;
#28325=CARTESIAN_POINT ( 'NONE',  ( 108.9443472801882393, -27.87019791606706320, 184.3448007804579447 ) ) ;
#28327=VERTEX_POINT ( 'NONE', #62947 ) ;
#28328=DIRECTION ( 'NONE',  ( 4.299999999999999979E-14, -1.000000000000000000, 4.400000000000000367E-29 ) ) ;
#28329=CARTESIAN_POINT ( 'NONE',  ( 109.8501361970267425, -26.70547878262040342, 170.8613395616249591 ) ) ;
#28330=DIRECTION ( 'NONE',  ( 0.000000000000000000, 0.000000000000000000, 1.000000000000000000 ) ) ;
#28334=DIRECTION ( 'NONE',  ( 0.000000000000000000, 0.000000000000000000, 1.000000000000000000 ) ) ;
#28335=CARTESIAN_POINT ( 'NONE',  ( 114.1038288540493539, -43.56973530630605751, 98.21276813305496489 ) ) ;
#28336=VERTEX_POINT ( 'NONE', #77045 ) ;
#28337=ORIENTED_EDGE ( 'NONE', *, *, #62192, .T. ) ;
#28338=EDGE_LOOP ( 'NONE', ( #87921, #8518, #40513, #13096 ) ) ;
#28340=CARTESIAN_POINT ( 'NONE',  ( 98.26727195740441800, -38.00851302551287603, 62.87301187732596475 ) ) ;
#28343=VECTOR ( 'NONE', #74603, 1000.000000000000000 ) ;
#28344=CARTESIAN_POINT ( 'NONE',  ( 106.5196382177907140, -25.62481104856566105, 191.1156252759109861 ) ) ;
#28345=CARTESIAN_POINT ( 'NONE',  ( 98.30753425284424907, -41.72887559872005170, 36.73979195237785689 ) ) ;
#28346=CIRCLE ( 'NONE', #51555, 2.116999999999993776 ) ;
#28347=CARTESIAN_POINT ( 'NONE',  ( 134.0664832912740110, -36.72944715994100306, -5.074374724089001809 ) ) ;
#28351=DIRECTION ( 'NONE',  ( 8.755702086949183871E-16, 1.000000000000000000, 0.000000000000000000 ) ) ;
#28355=CARTESIAN_POINT ( 'NONE',  ( 109.1969564574039282, -26.54663071456422330, 139.9127681330539872 ) ) ;
#28359=ORIENTED_EDGE ( 'NONE', *, *, #1720, .T. ) ;
#28361=EDGE_CURVE ( 'NONE', #4530, #67525, #43694, .T. ) ;
#28365=FACE_OUTER_BOUND ( 'NONE', #7225, .T. ) ;
#28366=VECTOR ( 'NONE', #66767, 1000.000000000000000 ) ;
#28367=CARTESIAN_POINT ( 'NONE',  ( 103.0873890296785333, -43.88832256772609952, 184.9909475124489688 ) ) ;
#28368=FACE_OUTER_BOUND ( 'NONE', #81054, .T. ) ;
#28370=DIRECTION ( 'NONE',  ( -4.299999999999999979E-14, 1.000000000000000000, -4.400000000000000367E-29 ) ) ;
#28372=VERTEX_POINT ( 'NONE', #63865 ) ;
#28378=EDGE_CURVE ( 'NONE', #38559, #51120, #30233, .T. ) ;
#28379=CARTESIAN_POINT ( 'NONE',  ( 134.0664832912740110, 0.2215528400590013880, 308.6356252759119911 ) ) ;
#28380=AXIS2_PLACEMENT_3D ( 'NONE', #44638, #86013, #65545 ) ;
#28381=CARTESIAN_POINT ( 'NONE',  ( 105.8471956337337190, -45.50678253122700312, 253.8987261630398677 ) ) ;
#28384=CARTESIAN_POINT ( 'NONE',  ( 182.4202572930265660, -31.94127993907054730, 313.9678068554149490 ) ) ;
#28385=AXIS2_PLACEMENT_3D ( 'NONE', #8201, #29536, #77689 ) ;
#28387=ORIENTED_EDGE ( 'NONE', *, *, #58077, .F. ) ;
#28388=ORIENTED_EDGE ( 'NONE', *, *, #66454, .T. ) ;
#28389=CARTESIAN_POINT ( 'NONE',  ( 107.0664832912749915, -36.72944715993903486, 25.56312527591096995 ) ) ;
#28391=VERTEX_POINT ( 'NONE', #2971 ) ;
#28392=VERTEX_POINT ( 'NONE', #86985 ) ;
#28393=CARTESIAN_POINT ( 'NONE',  ( 101.7278717236064836, -30.55458258274888905, 258.4623760838770750 ) ) ;
#28394=CARTESIAN_POINT ( 'NONE',  ( 112.1308356434906273, -47.47125106351535351, 137.9270538473389820 ) ) ;
#28395=CARTESIAN_POINT ( 'NONE',  ( 117.5733473178508319, -42.15660255127708211, 93.44705384733897802 ) ) ;
#28396=CARTESIAN_POINT ( 'NONE',  ( 116.6018603435394141, -39.73108032723776972, 249.5838075904518121 ) ) ;
#28397=FACE_OUTER_BOUND ( 'NONE', #87573, .T. ) ;
#28398=CARTESIAN_POINT ( 'NONE',  ( 103.3035667682879932, -27.00715593367326406, 211.3699109901969848 ) ) ;
#28400=CYLINDRICAL_SURFACE ( 'NONE', #13250, 0.5000000000000197620 ) ;
#28401=VERTEX_POINT ( 'NONE', #78844 ) ;
#28403=VERTEX_POINT ( 'NONE', #57926 ) ;
#28405=LINE ( 'NONE', #42918, #77923 ) ;
#28406=EDGE_CURVE ( 'NONE', #30159, #50189, #65194, .T. ) ;
#28407=CIRCLE ( 'NONE', #5262, 4.750000000000000888 ) ;
#28408=CARTESIAN_POINT ( 'NONE',  ( 103.3880255802097849, -27.43047095121296408, 136.3762285854526795 ) ) ;
#28411=AXIS2_PLACEMENT_3D ( 'NONE', #17310, #71393, #57281 ) ;
#28412=CARTESIAN_POINT ( 'NONE',  ( 98.28068559441094010, -31.05177188324158166, 145.8699109901969848 ) ) ;
#28413=CARTESIAN_POINT ( 'NONE',  ( 107.2792697713003776, -24.20934055526686279, 321.5865679059475610 ) ) ;
#28414=CIRCLE ( 'NONE', #79214, 12.99999999999999822 ) ;
#28415=EDGE_CURVE ( 'NONE', #75208, #73048, #13095, .T. ) ;
#28416=DIRECTION ( 'NONE',  ( -0.9254794337955620787, -0.3787978585227822492, 0.000000000000000000 ) ) ;
#28417=DIRECTION ( 'NONE',  ( 1.000000000000000000, 4.299999999999999979E-14, 1.000000000000000078E-15 ) ) ;
#28419=CARTESIAN_POINT ( 'NONE',  ( 110.1997925270103309, -46.26506069963132006, 57.82863803721590301 ) ) ;
#28420=CARTESIAN_POINT ( 'NONE',  ( 96.79426660377265534, -34.87310936442968057, 237.1841967044819626 ) ) ;
#28423=ORIENTED_EDGE ( 'NONE', *, *, #29604, .T. ) ;
#28426=DIRECTION ( 'NONE',  ( 1.000000000000000000, 4.163336342344333240E-14, 0.000000000000000000 ) ) ;
#28427=DIRECTION ( 'NONE',  ( -1.000000000000000000, -1.000000000000000078E-15, -1.000000000000000078E-15 ) ) ;
#28428=CARTESIAN_POINT ( 'NONE',  ( 102.3593652026347343, -47.65646955129418672, 287.2527681330535643 ) ) ;
#28431=CARTESIAN_POINT ( 'NONE',  ( 108.5930441862165026, -47.10046404026961397, 142.6927681330539883 ) ) ;
#28432=CARTESIAN_POINT ( 'NONE',  ( 99.12745497205600032, -44.42007846243786418, 37.95086337114900488 ) ) ;
#28433=CARTESIAN_POINT ( 'NONE',  ( 118.9671133714783480, -36.92893286478360437, 149.8127681330539644 ) ) ;
#28435=CARTESIAN_POINT ( 'NONE',  ( 80.06648329127402519, -36.72944715994107412, -5.074374724089057764 ) ) ;
#28436=CIRCLE ( 'NONE', #69098, 13.63963572536219715 ) ;
#28437=CARTESIAN_POINT ( 'NONE',  ( 48.16670390244661348, -28.27351298637380950, 117.4678068554150485 ) ) ;
#28438=CARTESIAN_POINT ( 'NONE',  ( 100.9546728224220260, -28.70702571896925903, 70.59395860815119761 ) ) ;
#28440=VERTEX_POINT ( 'NONE', #4310 ) ;
#28441=CARTESIAN_POINT ( 'NONE',  ( 107.0664832912739968, -18.82844715994099971, 168.9256252759119832 ) ) ;
#28442=ADVANCED_FACE ( 'NONE', ( #18369 ), #3860, .F. ) ;
#28443=VECTOR ( 'NONE', #12248, 1000.000000000000000 ) ;
#28444=ORIENTED_EDGE ( 'NONE', *, *, #43160, .T. ) ;
#28445=ORIENTED_EDGE ( 'NONE', *, *, #31813, .T. ) ;
#28446=FACE_OUTER_BOUND ( 'NONE', #8616, .T. ) ;
#28448=CARTESIAN_POINT ( 'NONE',  ( 116.7246412902988908, -32.86309880586080823, 50.12991099019698282 ) ) ;
#28449=CARTESIAN_POINT ( 'NONE',  ( 177.3246001664175537, -48.34074026909178912, 129.9678068554150059 ) ) ;
#28450=CARTESIAN_POINT ( 'NONE',  ( 73.06670390244801183, -50.82844715994100682, 250.9178068554160461 ) ) ;
#28451=EDGE_CURVE ( 'NONE', #61548, #11120, #52414, .T. ) ;
#28452=CARTESIAN_POINT ( 'NONE',  ( 95.86339321018937198, -32.71673170297378164, 172.0527681330539735 ) ) ;
#28453=CARTESIAN_POINT ( 'NONE',  ( 115.5572469886287479, -35.80043457063792545, 278.3352769709341032 ) ) ;
#28454=ORIENTED_EDGE ( 'NONE', *, *, #31010, .F. ) ;
#28455=EDGE_LOOP ( 'NONE', ( #1903, #29819 ) ) ;
#28456=ORIENTED_EDGE ( 'NONE', *, *, #71101, .T. ) ;
#28458=DIRECTION ( 'NONE',  ( -1.000200923085726652E-15, -1.000000000000000000, 0.000000000000000000 ) ) ;
#28459=CYLINDRICAL_SURFACE ( 'NONE', #37637, 0.5000000000000079936 ) ;
#28460=CARTESIAN_POINT ( 'NONE',  ( 97.33780276779580731, -34.07122131011711730, 162.1148046345169860 ) ) ;
#28461=CARTESIAN_POINT ( 'NONE',  ( 105.7995184814174934, -26.72403496660779254, 75.17729194306866702 ) ) ;
#28463=CARTESIAN_POINT ( 'NONE',  ( 181.9790560690580037, -31.62489322948711035, -5.074374724088000832 ) ) ;
#28465=DIRECTION ( 'NONE',  ( 0.000000000000000000, 0.000000000000000000, 1.000000000000000000 ) ) ;
#28466=CARTESIAN_POINT ( 'NONE',  ( 111.3142535964730797, -27.23286288913589459, 24.74133956162494030 ) ) ;
#28467=ADVANCED_FACE ( 'NONE', ( #16602 ), #51540, .F. ) ;
#28468=CARTESIAN_POINT ( 'NONE',  ( 167.6524903400753033, -48.32844715993521589, 300.4678068554149490 ) ) ;
#28470=DIRECTION ( 'NONE',  ( -0.7071067811865475727, 0.000000000000000000, -0.7071067811865475727 ) ) ;
#28471=AXIS2_PLACEMENT_3D ( 'NONE', #5374, #4484, #33072 ) ;
#28472=CARTESIAN_POINT ( 'NONE',  ( 165.6738106836030227, -28.98061976758901892, -5.074374724088000832 ) ) ;
#28473=CARTESIAN_POINT ( 'NONE',  ( 103.5365535965830475, -29.36946602085958702, 93.25094751244894553 ) ) ;
#28474=VECTOR ( 'NONE', #34616, 1000.000000000000000 ) ;
#28478=CARTESIAN_POINT ( 'NONE',  ( 109.7248659201067795, -27.00080517940160973, 44.86479194268253679 ) ) ;
#28480=ORIENTED_EDGE ( 'NONE', *, *, #77940, .T. ) ;
#28481=EDGE_CURVE ( 'NONE', #69245, #32266, #20511, .T. ) ;
#28482=DIRECTION ( 'NONE',  ( 0.000000000000000000, 0.000000000000000000, -1.000000000000000000 ) ) ;
#28485=EDGE_CURVE ( 'NONE', #73586, #35967, #60859, .T. ) ;
#28486=CARTESIAN_POINT ( 'NONE',  ( 115.3364322588818851, -33.54570361940938739, 135.5501547344689754 ) ) ;
#28489=CARTESIAN_POINT ( 'NONE',  ( 116.9423613927432939, -33.21572726007214271, 110.0984824187679578 ) ) ;
#28491=ORIENTED_EDGE ( 'NONE', *, *, #89810, .T. ) ;
#28492=ORIENTED_EDGE ( 'NONE', *, *, #43040, .T. ) ;
#28493=ORIENTED_EDGE ( 'NONE', *, *, #66302, .T. ) ;
#28494=DIRECTION ( 'NONE',  ( 0.4214249218767882055, 0.9068632946707806397, 4.214249218767890910E-16 ) ) ;
#28495=ORIENTED_EDGE ( 'NONE', *, *, #39851, .F. ) ;
#28496=CARTESIAN_POINT ( 'NONE',  ( 101.6204011159889831, -47.22657592904994317, 17.19562527591095247 ) ) ;
#28497=CARTESIAN_POINT ( 'NONE',  ( 95.38360599640527937, -38.85844429501600672, 197.4699109901969791 ) ) ;
#28499=LINE ( 'NONE', #56190, #37296 ) ;
#28500=CARTESIAN_POINT ( 'NONE',  ( 102.3127581962668273, -26.75066580571964536, 136.4422919425779526 ) ) ;
#28502=VERTEX_POINT ( 'NONE', #25635 ) ;
#28509=CARTESIAN_POINT ( 'NONE',  ( 116.1584957626482435, -43.02035883463254606, 13.35657765686298859 ) ) ;
#28511=EDGE_CURVE ( 'NONE', #75837, #42151, #37943, .T. ) ;
#28512=CARTESIAN_POINT ( 'NONE',  ( 141.0664832912740394, -46.72944715994099596, -5.074374724088994704 ) ) ;
#28514=CARTESIAN_POINT ( 'NONE',  ( 97.72045520820927322, -39.61305636501506910, 21.56419670448295278 ) ) ;
#28515=DIRECTION ( 'NONE',  ( -4.237773401492740281E-14, 1.000000000000000000, 0.000000000000000000 ) ) ;
#28516=CARTESIAN_POINT ( 'NONE',  ( 96.03721982003250446, -36.58408020053186505, 152.3280062282919971 ) ) ;
#28518=FACE_OUTER_BOUND ( 'NONE', #46807, .T. ) ;
#28520=FACE_OUTER_BOUND ( 'NONE', #34825, .T. ) ;
#28521=FACE_BOUND ( 'NONE', #8549, .T. ) ;
#28525=CARTESIAN_POINT ( 'NONE',  ( 96.57452018799374116, -36.20934681947932177, 171.2870538473399620 ) ) ;
#28526=ORIENTED_EDGE ( 'NONE', *, *, #25945, .T. ) ;
#28527=DIRECTION ( 'NONE',  ( 1.000000000000000078E-15, -1.000000000000000083E-30, -1.000000000000000000 ) ) ;
#28528=CARTESIAN_POINT ( 'NONE',  ( 110.2625522973084600, -26.74624433126517076, 230.8299109901969643 ) ) ;
#28529=CARTESIAN_POINT ( 'NONE',  ( 103.5842829832543686, -46.60199803408937669, 53.30705384733997221 ) ) ;
#28533=CARTESIAN_POINT ( 'NONE',  ( 72.26648329127297643, -71.52944715994141234, 352.4506252759078961 ) ) ;
#28535=CIRCLE ( 'NONE', #38709, 2.750000000000002665 ) ;
#28539=AXIS2_PLACEMENT_3D ( 'NONE', #76185, #8045, #48444 ) ;
#28540=ADVANCED_FACE ( 'NONE', ( #60591 ), #81528, .F. ) ;
#28542=ORIENTED_EDGE ( 'NONE', *, *, #31624, .F. ) ;
#28546=CARTESIAN_POINT ( 'NONE',  ( 112.4543492094282726, -45.69561878580546477, 234.0070538473389377 ) ) ;
#28547=CARTESIAN_POINT ( 'NONE',  ( 97.40471326410413155, -39.52310482453168561, 251.5503829890487566 ) ) ;
#28548=CARTESIAN_POINT ( 'NONE',  ( 135.9759635523877819, -16.74831825236557137, 2.232988539014289397 ) ) ;
#28549=EDGE_CURVE ( 'NONE', #55608, #14919, #85812, .T. ) ;
#28550=ADVANCED_FACE ( 'NONE', ( #34234 ), #5200, .F. ) ;
#28551=LINE ( 'NONE', #15396, #4703 ) ;
#28552=LINE ( 'NONE', #75819, #60168 ) ;
#28554=CIRCLE ( 'NONE', #51759, 1.000000000000000888 ) ;
#28555=CARTESIAN_POINT ( 'NONE',  ( 105.9861246248700439, -26.33814362677674836, 50.15848241876796720 ) ) ;
#28558=ADVANCED_FACE ( 'NONE', ( #87872 ), #5656, .T. ) ;
#28561=LINE ( 'NONE', #56248, #41235 ) ;
#28562=CARTESIAN_POINT ( 'NONE',  ( 97.60782674972406880, -39.98224406465867986, 17.58997982183609210 ) ) ;
#28564=CARTESIAN_POINT ( 'NONE',  ( 112.1213531720969883, -45.14146623880446185, 234.0070538473389377 ) ) ;
#28565=CARTESIAN_POINT ( 'NONE',  ( 63.06670390244732971, -24.92844715994017690, 300.4678068554150627 ) ) ;
#28566=CARTESIAN_POINT ( 'NONE',  ( 106.8551140066829817, -47.84553036069057441, 73.56133956162396714 ) ) ;
#28568=EDGE_CURVE ( 'NONE', #18287, #63937, #19716, .T. ) ;
#28569=CARTESIAN_POINT ( 'NONE',  ( 103.3069155499675986, -27.46306005310784926, 21.38318458331234240 ) ) ;
#28570=EDGE_LOOP ( 'NONE', ( #62211, #39441, #64662, #74872 ) ) ;
#28576=CARTESIAN_POINT ( 'NONE',  ( 98.30854254679421445, -35.37787306724802505, 262.6358690201826676 ) ) ;
#28577=VECTOR ( 'NONE', #48506, 1000.000000000000000 ) ;
#28578=DIRECTION ( 'NONE',  ( 0.000000000000000000, 0.000000000000000000, 1.000000000000000000 ) ) ;
#28580=CARTESIAN_POINT ( 'NONE',  ( 141.0664832912739826, -8.729447159940995959, 14.92562527591100618 ) ) ;
#28582=VERTEX_POINT ( 'NONE', #68324 ) ;
#28584=ADVANCED_FACE ( 'NONE', ( #32437 ), #6104, .T. ) ;
#28586=ORIENTED_EDGE ( 'NONE', *, *, #12157, .T. ) ;
#28587=CARTESIAN_POINT ( 'NONE',  ( 116.7450715690984140, -32.85492016819326722, 54.12991099019698282 ) ) ;
#28588=VERTEX_POINT ( 'NONE', #20179 ) ;
#28590=CARTESIAN_POINT ( 'NONE',  ( 101.7664832247249365, -29.99442739451795958, 15.02956268521998773 ) ) ;
#28591=EDGE_CURVE ( 'NONE', #22872, #85451, #61938, .T. ) ;
#28592=CARTESIAN_POINT ( 'NONE',  ( 41.56648329127499153, -32.07844715994070839, 318.9256252759120116 ) ) ;
#28593=CARTESIAN_POINT ( 'NONE',  ( 96.73459541816642115, -35.84013382243347223, 186.2461014663879837 ) ) ;
#28594=DIRECTION ( 'NONE',  ( -3.999999999999999995E-14, 1.000000000000000000, -4.100000000000000342E-29 ) ) ;
#28595=VECTOR ( 'NONE', #65636, 1000.000000000000000 ) ;
#28596=DIRECTION ( 'NONE',  ( -0.7071067811868619879, -0.7071067811862330466, -7.071067811868613027E-16 ) ) ;
#28597=LINE ( 'NONE', #13632, #14420 ) ;
#28598=ADVANCED_FACE ( 'NONE', ( #27424 ), #82866, .T. ) ;
#28600=CARTESIAN_POINT ( 'NONE',  ( 45.76696975232771081, -48.62818131006071098, 180.4678068554150911 ) ) ;
#28601=CARTESIAN_POINT ( 'NONE',  ( 97.17561725847181719, -33.29990440931864271, 282.0613395616252888 ) ) ;
#28604=CARTESIAN_POINT ( 'NONE',  ( 136.4975570085112793, -38.01506174167548835, 7.157201688892038227 ) ) ;
#28605=CIRCLE ( 'NONE', #53207, 2.750000000000002665 ) ;
#28606=ORIENTED_EDGE ( 'NONE', *, *, #53149, .T. ) ;
#28607=CARTESIAN_POINT ( 'NONE',  ( 117.3817195963474518, -32.63147225404833307, 95.13943479972097350 ) ) ;
#28610=VECTOR ( 'NONE', #16107, 1000.000000000000000 ) ;
#28612=CARTESIAN_POINT ( 'NONE',  ( 130.5667039024480118, -34.21194715994104740, 219.5838068554170093 ) ) ;
#28613=ORIENTED_EDGE ( 'NONE', *, *, #3076, .F. ) ;
#28614=VERTEX_POINT ( 'NONE', #21980 ) ;
#28615=CARTESIAN_POINT ( 'NONE',  ( 97.81170242524891023, -40.51743837274789684, 121.6354095930283137 ) ) ;
#28616=DIRECTION ( 'NONE',  ( 0.000000000000000000, 0.000000000000000000, 1.000000000000000000 ) ) ;
#28617=DIRECTION ( 'NONE',  ( 0.000000000000000000, 0.000000000000000000, 1.000000000000000000 ) ) ;
#28619=CARTESIAN_POINT ( 'NONE',  ( 172.5664832912740110, -18.82844715994099971, 18.92562527591200094 ) ) ;
#28620=CARTESIAN_POINT ( 'NONE',  ( 99.06589935993768847, -44.35602157064030848, 32.92038718067297509 ) ) ;
#28621=CARTESIAN_POINT ( 'NONE',  ( 88.17226027475679473, -14.72944715994100484, 239.5838068554175777 ) ) ;
#28631=FACE_OUTER_BOUND ( 'NONE', #9301, .T. ) ;
#28634=LINE ( 'NONE', #20040, #89857 ) ;
#28636=CARTESIAN_POINT ( 'NONE',  ( 99.14828105993673546, -39.93229045078558670, 206.0552769709339884 ) ) ;
#28638=CARTESIAN_POINT ( 'NONE',  ( 117.1490187775317793, -39.54886983357372543, 98.60991099019594230 ) ) ;
#28643=ORIENTED_EDGE ( 'NONE', *, *, #44249, .F. ) ;
#28644=CARTESIAN_POINT ( 'NONE',  ( 113.2454418602651600, -28.75862586841305557, 49.55229777713112327 ) ) ;
#28647=LINE ( 'NONE', #51, #22729 ) ;
#28648=CARTESIAN_POINT ( 'NONE',  ( 109.6447271640448378, -46.47965470880307493, 273.7811528438442679 ) ) ;
#28649=VECTOR ( 'NONE', #13086, 1000.000000000000000 ) ;
#28650=VECTOR ( 'NONE', #32442, 1000.000000000000000 ) ;
#28652=ORIENTED_EDGE ( 'NONE', *, *, #2529, .T. ) ;
#28653=CARTESIAN_POINT ( 'NONE',  ( 98.57199122844706096, -43.83852907894476658, 71.86895860924397539 ) ) ;
#28655=DIRECTION ( 'NONE',  ( -0.9963424814100688698, 0.08544974978094983797, 0.000000000000000000 ) ) ;
#28658=ADVANCED_FACE ( 'NONE', ( #76025, #27872 ), #36035, .T. ) ;
#28659=CARTESIAN_POINT ( 'NONE',  ( 131.4596324495014699, -17.85248396559163808, 2.902015641457815764 ) ) ;
#28663=CARTESIAN_POINT ( 'NONE',  ( 182.5667039024480118, -32.29483332968450782, -5.074374724088000832 ) ) ;
#28666=CARTESIAN_POINT ( 'NONE',  ( 107.3345073157536689, -26.28600797661530208, 116.0556252759109555 ) ) ;
#28668=AXIS2_PLACEMENT_3D ( 'NONE', #32513, #46134, #79812 ) ;
#28669=CARTESIAN_POINT ( 'NONE',  ( 107.0664832912750057, -36.72944715993903486, 6.826283056785790393 ) ) ;
#28670=FACE_OUTER_BOUND ( 'NONE', #39399, .T. ) ;
#28672=EDGE_CURVE ( 'NONE', #65123, #54206, #71021, .T. ) ;
#28674=ORIENTED_EDGE ( 'NONE', *, *, #57102, .T. ) ;
#28677=ADVANCED_FACE ( 'NONE', ( #7436 ), #76476, .T. ) ;
#28678=CARTESIAN_POINT ( 'NONE',  ( 111.5019814087853405, -26.53443175268790100, 130.7499109901969518 ) ) ;
#28680=VERTEX_POINT ( 'NONE', #1070 ) ;
#28682=CARTESIAN_POINT ( 'NONE',  ( 101.3060704567421624, -26.40153104436181053, 251.4813395616249920 ) ) ;
#28683=DIRECTION ( 'NONE',  ( 0.000000000000000000, 0.000000000000000000, 1.000000000000000000 ) ) ;
#28688=VECTOR ( 'NONE', #82385, 1000.000000000000000 ) ;
#28691=VECTOR ( 'NONE', #62316, 1000.000000000000000 ) ;
#28692=CIRCLE ( 'NONE', #41764, 15.84999999999999964 ) ;
#28693=CARTESIAN_POINT ( 'NONE',  ( 103.8504807240352790, -26.87063827031080621, 210.3394347997209763 ) ) ;
#28694=ORIENTED_EDGE ( 'NONE', *, *, #43289, .F. ) ;
#28695=ORIENTED_EDGE ( 'NONE', *, *, #84432, .F. ) ;
#28696=ADVANCED_FACE ( 'NONE', ( #42382 ), #64200, .T. ) ;
#28697=CARTESIAN_POINT ( 'NONE',  ( 115.2219208674478352, -40.19601845633869175, 164.9387261630399450 ) ) ;
#28699=DIRECTION ( 'NONE',  ( 2.999999999999999839E-15, -1.000000000000000000, 2.999999999999999900E-30 ) ) ;
#28700=CARTESIAN_POINT ( 'NONE',  ( 109.8015415646094226, -45.15840846867854452, 9.258726163039964874 ) ) ;
#28701=DIRECTION ( 'NONE',  ( -0.000000000000000000, -0.000000000000000000, 1.000000000000000000 ) ) ;
#28702=CARTESIAN_POINT ( 'NONE',  ( 127.0664832912740394, -46.72944715994101017, -4.824374724089008915 ) ) ;
#28703=CARTESIAN_POINT ( 'NONE',  ( 107.3366192906461549, -25.27349273040127997, 322.1637998480665033 ) ) ;
#28704=LINE ( 'NONE', #56391, #88443 ) ;
#28706=CARTESIAN_POINT ( 'NONE',  ( 117.7539631054257967, -31.66723592997632863, 214.1784824187679419 ) ) ;
#28708=ORIENTED_EDGE ( 'NONE', *, *, #65373, .T. ) ;
#28709=ORIENTED_EDGE ( 'NONE', *, *, #74921, .T. ) ;
#28710=EDGE_CURVE ( 'NONE', #50783, #33306, #77373, .T. ) ;
#28711=CARTESIAN_POINT ( 'NONE',  ( 106.5646857698207981, -25.28130207810567498, 321.1698005525342978 ) ) ;
#28712=CARTESIAN_POINT ( 'NONE',  ( 82.81519967300323515, -18.82419990105044860, 6.751707299519896566 ) ) ;
#28713=LINE ( 'NONE', #55489, #17112 ) ;
#28714=CARTESIAN_POINT ( 'NONE',  ( 131.0667039024480118, -42.97311385573999587, 231.5838068554170093 ) ) ;
#28717=VECTOR ( 'NONE', #82715, 1000.000000000000000 ) ;
#28718=CARTESIAN_POINT ( 'NONE',  ( 97.33063402535807995, -33.15845140301009053, 17.03467289495797132 ) ) ;
#28719=PLANE ( 'NONE',  #51352 ) ;
#28721=CARTESIAN_POINT ( 'NONE',  ( 97.06313332029375829, -39.81586545721199144, 17.56419670448195092 ) ) ;
#28723=CARTESIAN_POINT ( 'NONE',  ( 103.9392425780951754, -26.78422740453794404, 250.3184824187678714 ) ) ;
#28724=VERTEX_POINT ( 'NONE', #11347 ) ;
#28725=CARTESIAN_POINT ( 'NONE',  ( 77.86687873443747776, -38.38871026384816076, 7.389079501587738186 ) ) ;
#28726=FACE_OUTER_BOUND ( 'NONE', #4112, .T. ) ;
#28728=CARTESIAN_POINT ( 'NONE',  ( 113.7275377883433549, -41.44750597731145092, 51.15380465530594734 ) ) ;
#28729=CARTESIAN_POINT ( 'NONE',  ( 116.6808514842340259, -40.81615526105927927, 164.5070538473399608 ) ) ;
#28731=ORIENTED_EDGE ( 'NONE', *, *, #75745, .T. ) ;
#28732=AXIS2_PLACEMENT_3D ( 'NONE', #34437, #48941, #14463 ) ;
#28734=ORIENTED_EDGE ( 'NONE', *, *, #51509, .T. ) ;
#28735=VERTEX_POINT ( 'NONE', #59925 ) ;
#28736=EDGE_CURVE ( 'NONE', #64255, #52806, #22873, .T. ) ;
#28737=CIRCLE ( 'NONE', #75165, 2.117000000000000881 ) ;
#28739=DIRECTION ( 'NONE',  ( 1.000000000000000000, 4.299999999999999979E-14, 1.000000000000000078E-15 ) ) ;
#28741=VERTEX_POINT ( 'NONE', #39501 ) ;
#28742=ORIENTED_EDGE ( 'NONE', *, *, #38715, .F. ) ;
#28745=CARTESIAN_POINT ( 'NONE',  ( 98.02882863141191194, -40.27788709084830998, 96.04670554236294322 ) ) ;
#28746=CARTESIAN_POINT ( 'NONE',  ( 116.5566381636777322, -42.44192488244189576, 278.3832443235297660 ) ) ;
#28747=CIRCLE ( 'NONE', #59200, 1.000000000000000888 ) ;
#28748=DIRECTION ( 'NONE',  ( 0.000000000000000000, 0.000000000000000000, -1.000000000000000000 ) ) ;
#28749=CARTESIAN_POINT ( 'NONE',  ( 84.06648329127399677, -18.72966777111504300, 199.5838068554169524 ) ) ;
#28751=VERTEX_POINT ( 'NONE', #65083 ) ;
#28753=AXIS2_PLACEMENT_3D ( 'NONE', #26243, #12624, #25796 ) ;
#28754=AXIS2_PLACEMENT_3D ( 'NONE', #9117, #50426, #50880 ) ;
#28756=DIRECTION ( 'NONE',  ( 0.000000000000000000, -1.000000000000000000, 0.000000000000000000 ) ) ;
#28758=CARTESIAN_POINT ( 'NONE',  ( 116.5394839232220505, -34.29517225379350975, 124.0270538473399426 ) ) ;
#28759=CARTESIAN_POINT ( 'NONE',  ( 115.2011789175540741, -43.31984874952732412, 88.28419670448195689 ) ) ;
#28760=CARTESIAN_POINT ( 'NONE',  ( 95.18116725028646385, -37.33612674980418689, 271.3670538473392639 ) ) ;
#28763=CARTESIAN_POINT ( 'NONE',  ( 111.6085881668573450, -46.11327973307566452, 247.9356252759109509 ) ) ;
#28764=FACE_OUTER_BOUND ( 'NONE', #7604, .T. ) ;
#28767=CARTESIAN_POINT ( 'NONE',  ( 98.17570384001206207, -41.31031557640367424, 27.70558999709250614 ) ) ;
#28771=DIRECTION ( 'NONE',  ( 1.000000000000000000, 3.999999999999999995E-14, 1.000000000000000078E-15 ) ) ;
#28772=EDGE_CURVE ( 'NONE', #59006, #60222, #26389, .T. ) ;
#28773=FACE_OUTER_BOUND ( 'NONE', #8886, .T. ) ;
#28775=EDGE_CURVE ( 'NONE', #394, #58704, #79180, .T. ) ;
#28778=DIRECTION ( 'NONE',  ( 0.000000000000000000, 0.000000000000000000, 1.000000000000000000 ) ) ;
#28779=LINE ( 'NONE', #50093, #48645 ) ;
#28780=VERTEX_POINT ( 'NONE', #2866 ) ;
#28781=EDGE_CURVE ( 'NONE', #26329, #44492, #33653, .T. ) ;
#28783=CARTESIAN_POINT ( 'NONE',  ( 95.20615018136085439, -37.33485150947186781, 271.3670538473392639 ) ) ;
#28784=CARTESIAN_POINT ( 'NONE',  ( 117.7034974245586483, -39.73408348695345182, 139.6194347997199827 ) ) ;
#28785=CARTESIAN_POINT ( 'NONE',  ( 106.2504415414193488, -26.27893178022805998, 21.13848241876792144 ) ) ;
#28787=AXIS2_PLACEMENT_3D ( 'NONE', #35857, #36319, #49018 ) ;
#28788=DIRECTION ( 'NONE',  ( -0.000000000000000000, -0.000000000000000000, 1.000000000000000000 ) ) ;
#28789=CARTESIAN_POINT ( 'NONE',  ( 82.41409441627625654, -35.29397280665990166, 7.245803660790303802 ) ) ;
#28793=ORIENTED_EDGE ( 'NONE', *, *, #76452, .T. ) ;
#28796=EDGE_CURVE ( 'NONE', #80581, #45331, #4982, .T. ) ;
#28797=CARTESIAN_POINT ( 'NONE',  ( 98.60840819187967554, -35.53902818534925245, 180.6381341137909544 ) ) ;
#28799=VERTEX_POINT ( 'NONE', #4539 ) ;
#28801=CARTESIAN_POINT ( 'NONE',  ( 96.64068249873270133, -36.21262657180042766, 167.2870538473399620 ) ) ;
#28802=CARTESIAN_POINT ( 'NONE',  ( 116.8183451804401045, -34.15765563543617134, 150.0318682641123758 ) ) ;
#28803=CARTESIAN_POINT ( 'NONE',  ( 107.0620278373210255, -36.73691869758540207, 361.9756252759100903 ) ) ;
#28804=CARTESIAN_POINT ( 'NONE',  ( 113.4728681846144127, -29.02320129775888446, 85.52423081353769874 ) ) ;
#28808=CARTESIAN_POINT ( 'NONE',  ( 98.87588542518393808, -42.07524381596793006, 101.7870538473399620 ) ) ;
#28809=VERTEX_POINT ( 'NONE', #30563 ) ;
#28810=ORIENTED_EDGE ( 'NONE', *, *, #42086, .F. ) ;
#28811=VERTEX_POINT ( 'NONE', #50548 ) ;
#28812=VECTOR ( 'NONE', #74484, 1000.000000000000000 ) ;
#28813=CARTESIAN_POINT ( 'NONE',  ( 116.3507336416864746, -38.17139756410392692, 65.12348806780198629 ) ) ;
#28816=CARTESIAN_POINT ( 'NONE',  ( 96.73459541816653484, -35.84013382243349355, 182.2461014663859658 ) ) ;
#28817=CARTESIAN_POINT ( 'NONE',  ( 116.3121618740066623, -32.93870344941997530, 39.13562527591096796 ) ) ;
#28818=CYLINDRICAL_SURFACE ( 'NONE', #5906, 2.116999999999980009 ) ;
#28822=LINE ( 'NONE', #6577, #31810 ) ;
#28824=CARTESIAN_POINT ( 'NONE',  ( 98.85726102317293851, -28.21728661942034577, 115.6870538473389587 ) ) ;
#28825=ORIENTED_EDGE ( 'NONE', *, *, #65411, .F. ) ;
#28829=CARTESIAN_POINT ( 'NONE',  ( 36.23715912545344509, -47.82818131006131779, 129.9678068554150911 ) ) ;
#28830=VECTOR ( 'NONE', #77482, 1000.000000000000000 ) ;
#28831=CARTESIAN_POINT ( 'NONE',  ( 116.7951252704057907, -39.38782979425321429, 79.61479194223753098 ) ) ;
#28834=CARTESIAN_POINT ( 'NONE',  ( 115.0224139972512063, -40.13592505470528238, 211.3347570362579404 ) ) ;
#28835=CARTESIAN_POINT ( 'NONE',  ( 160.7738106836362419, -48.62134037874780290, 180.4678068554150059 ) ) ;
#28836=DIRECTION ( 'NONE',  ( -0.9999999853157766072, -0.0001713722456127291416, 9.999999853157765648E-16 ) ) ;
#28837=EDGE_LOOP ( 'NONE', ( #60886, #41265 ) ) ;
#28838=ORIENTED_EDGE ( 'NONE', *, *, #23047, .T. ) ;
#28839=VERTEX_POINT ( 'NONE', #32228 ) ;
#28840=AXIS2_PLACEMENT_3D ( 'NONE', #35317, #37130, #2614 ) ;
#28842=VERTEX_POINT ( 'NONE', #58262 ) ;
#28844=PLANE ( 'NONE',  #7220 ) ;
#28845=CARTESIAN_POINT ( 'NONE',  ( 98.98570259493575918, -42.74373749968300729, 258.2672975916112819 ) ) ;
#28846=LINE ( 'NONE', #43347, #23209 ) ;
#28847=VERTEX_POINT ( 'NONE', #23329 ) ;
#28848=CARTESIAN_POINT ( 'NONE',  ( 41.56648329127399677, -18.82844715994099971, 198.9256252759119832 ) ) ;
#28852=VERTEX_POINT ( 'NONE', #60377 ) ;
#28854=CARTESIAN_POINT ( 'NONE',  ( 91.27445496092437338, -35.37506862591278889, 302.4856252759109907 ) ) ;
#28856=EDGE_LOOP ( 'NONE', ( #4811, #28526, #53955, #13814 ) ) ;
#28857=CARTESIAN_POINT ( 'NONE',  ( 106.4091095994060652, -45.35897697767001091, 265.3461856076867207 ) ) ;
#28858=CARTESIAN_POINT ( 'NONE',  ( 101.7582431991767464, -45.72772181880441167, 162.1527681330539679 ) ) ;
#28859=CARTESIAN_POINT ( 'NONE',  ( 96.05093434719793777, -37.29646042206077539, 121.3794347997209684 ) ) ;
#28860=CARTESIAN_POINT ( 'NONE',  ( 41.56670390244777735, -36.32844715994104234, 300.4678068554150059 ) ) ;
#28861=SURFACE_STYLE_USAGE ( .BOTH. , #7962 ) ;
#28862=CARTESIAN_POINT ( 'NONE',  ( 118.7901020289055225, -38.45900758189035429, 219.7099109901969882 ) ) ;
#28864=PLANE ( 'NONE',  #46613 ) ;
#28865=ORIENTED_EDGE ( 'NONE', *, *, #9184, .T. ) ;
#28869=ORIENTED_EDGE ( 'NONE', *, *, #42187, .F. ) ;
#28871=VECTOR ( 'NONE', #34025, 1000.000000000000000 ) ;
#28872=CARTESIAN_POINT ( 'NONE',  ( 25.56670390244719115, -42.82844715994178131, 173.2178068554150627 ) ) ;
#28873=AXIS2_PLACEMENT_3D ( 'NONE', #28140, #68605, #14540 ) ;
#28875=CARTESIAN_POINT ( 'NONE',  ( 103.2053365856880873, -46.45145584090948176, 117.2756252759109543 ) ) ;
#28877=CARTESIAN_POINT ( 'NONE',  ( 134.0664832912739826, -33.97944715994100306, 8.225625275910998013 ) ) ;
#28878=FACE_OUTER_BOUND ( 'NONE', #15744, .T. ) ;
#28880=FACE_BOUND ( 'NONE', #59588, .T. ) ;
#28881=CARTESIAN_POINT ( 'NONE',  ( 110.8089421659425540, -26.35361831834165969, 245.7889586092439629 ) ) ;
#28883=EDGE_CURVE ( 'NONE', #72034, #68380, #23764, .T. ) ;
#28885=CARTESIAN_POINT ( 'NONE',  ( 171.4664832912730219, 12.92155284005730387, 355.9756252759109998 ) ) ;
#28887=ADVANCED_FACE ( 'NONE', ( #18608 ), #88116, .T. ) ;
#28889=ADVANCED_FACE ( 'NONE', ( #66755 ), #46290, .T. ) ;
#28890=DIRECTION ( 'NONE',  ( 0.000000000000000000, 0.000000000000000000, -1.000000000000000000 ) ) ;
#28891=VECTOR ( 'NONE', #65672, 1000.000000000000000 ) ;
#28892=CARTESIAN_POINT ( 'NONE',  ( 84.06648329127399677, -14.47844715994100007, 284.9256252759119548 ) ) ;
#28893=CARTESIAN_POINT ( 'NONE',  ( 112.8431189249872091, -28.80713414957965313, 195.5838068554226084 ) ) ;
#28895=EDGE_CURVE ( 'NONE', #20709, #60678, #32150, .T. ) ;
#28896=DIRECTION ( 'NONE',  ( 1.000000000000000078E-15, 0.000000000000000000, -1.000000000000000000 ) ) ;
#28897=CARTESIAN_POINT ( 'NONE',  ( 100.8733315758915552, -45.91070206092880568, 152.0918157521009562 ) ) ;
#28898=CARTESIAN_POINT ( 'NONE',  ( 118.0831039394318083, -37.62836316206458065, 34.77372051400695341 ) ) ;
#28899=CARTESIAN_POINT ( 'NONE',  ( 117.2699639542694001, -41.09825485984158178, 209.5165776568640013 ) ) ;
#28901=AXIS2_PLACEMENT_3D ( 'NONE', #56458, #76927, #14705 ) ;
#28903=CARTESIAN_POINT ( 'NONE',  ( 37.35959712144415334, -48.62134037893600436, 249.9678068554150343 ) ) ;
#28909=ORIENTED_EDGE ( 'NONE', *, *, #85470, .T. ) ;
#28910=EDGE_LOOP ( 'NONE', ( #67263, #84122, #28218, #35834 ) ) ;
#28913=DIRECTION ( 'NONE',  ( 0.000000000000000000, 1.000000000000000000, 0.000000000000000000 ) ) ;
#28914=VERTEX_POINT ( 'NONE', #68107 ) ;
#28915=CARTESIAN_POINT ( 'NONE',  ( 109.9050689397999605, -46.77468768478695438, 68.79562527591099297 ) ) ;
#28918=CARTESIAN_POINT ( 'NONE',  ( 117.5308098062252498, -40.43017262224169883, 174.5680062282919778 ) ) ;
#28919=CARTESIAN_POINT ( 'NONE',  ( 101.2965385564679792, -30.39239502954603367, 285.0867055423626084 ) ) ;
#28921=AXIS2_PLACEMENT_3D ( 'NONE', #210, #27911, #14752 ) ;
#28922=EDGE_LOOP ( 'NONE', ( #18905, #88214, #42442, #14996 ) ) ;
#28924=ORIENTED_EDGE ( 'NONE', *, *, #72373, .F. ) ;
#28927=CARTESIAN_POINT ( 'NONE',  ( 109.7243363830542364, -27.00066479321645829, 160.8648351248226334 ) ) ;
#28928=CARTESIAN_POINT ( 'NONE',  ( 108.4174892472081808, -26.73503592690951436, 74.96895860963714142 ) ) ;
#28929=CARTESIAN_POINT ( 'NONE',  ( 188.5667039024486087, -48.82844715993430640, 139.7178068554150059 ) ) ;
#28932=DIRECTION ( 'NONE',  ( 0.000000000000000000, 0.000000000000000000, 1.000000000000000000 ) ) ;
#28933=CARTESIAN_POINT ( 'NONE',  ( 112.1705331031350994, -27.62378402076933526, 34.66991099019695355 ) ) ;
#28935=ORIENTED_EDGE ( 'NONE', *, *, #62484, .F. ) ;
#28936=CIRCLE ( 'NONE', #33262, 2.750000000000002665 ) ;
#28937=CARTESIAN_POINT ( 'NONE',  ( 97.06107093643949213, -37.99641063121843843, 271.4272918366033309 ) ) ;
#28938=FACE_OUTER_BOUND ( 'NONE', #8082, .T. ) ;
#28940=CARTESIAN_POINT ( 'NONE',  ( 106.2913146648166531, -45.97580021205838818, 110.3280903695919903 ) ) ;
#28942=CIRCLE ( 'NONE', #37690, 4.874999999999990230 ) ;
#28945=DIRECTION ( 'NONE',  ( 0.000000000000000000, 0.000000000000000000, -1.000000000000000000 ) ) ;
#28946=EDGE_LOOP ( 'NONE', ( #17016, #83368, #18633, #18767 ) ) ;
#28947=ORIENTED_EDGE ( 'NONE', *, *, #1142, .F. ) ;
#28948=VECTOR ( 'NONE', #23615, 1000.000000000000000 ) ;
#28949=CARTESIAN_POINT ( 'NONE',  ( 20.56670390244833158, -48.82844715994187368, 249.9678068554150059 ) ) ;
#28950=VERTEX_POINT ( 'NONE', #55778 ) ;
#28951=ORIENTED_EDGE ( 'NONE', *, *, #13070, .F. ) ;
#28953=CARTESIAN_POINT ( 'NONE',  ( 98.22997538087754776, -36.06364078424440578, 142.6987261630399644 ) ) ;
#28955=AXIS2_PLACEMENT_3D ( 'NONE', #66244, #79472, #47020 ) ;
#28956=CARTESIAN_POINT ( 'NONE',  ( 117.1274056176845733, -39.54282605291903252, 94.60991099019693706 ) ) ;
#28957=DIRECTION ( 'NONE',  ( -0.000000000000000000, -0.000000000000000000, -1.000000000000000000 ) ) ;
#28959=EDGE_CURVE ( 'NONE', #13820, #36065, #80096, .T. ) ;
#28960=ORIENTED_EDGE ( 'NONE', *, *, #57215, .F. ) ;
#28961=EDGE_LOOP ( 'NONE', ( #4933, #84913, #88861, #82785 ) ) ;
#28963=DIRECTION ( 'NONE',  ( 0.000000000000000000, 0.000000000000000000, 1.000000000000000000 ) ) ;
#28964=ORIENTED_EDGE ( 'NONE', *, *, #57579, .T. ) ;
#28965=CARTESIAN_POINT ( 'NONE',  ( 112.1867106929447999, -26.95862322015887358, 14.68038718067299442 ) ) ;
#28966=CARTESIAN_POINT ( 'NONE',  ( 113.6994007951720107, -45.60016365472323230, 184.0994347997199725 ) ) ;
#28968=CARTESIAN_POINT ( 'NONE',  ( 163.0664832912739826, 22.62155284005901024, 327.8006252759110453 ) ) ;
#28969=CARTESIAN_POINT ( 'NONE',  ( 102.3931144830280715, -26.71278082505766704, 131.4118157521009778 ) ) ;
#28970=DIRECTION ( 'NONE',  ( -0.02150753337724187197, -0.0009076677972194977960, -0.9997682742251811083 ) ) ;
#28972=CARTESIAN_POINT ( 'NONE',  ( 97.07195551945122247, -35.37924153545726114, 116.2203645627087099 ) ) ;
#28973=ORIENTED_EDGE ( 'NONE', *, *, #63061, .T. ) ;
#28974=CARTESIAN_POINT ( 'NONE',  ( 99.50479149024018000, -43.30586258244627373, 132.8967665784813903 ) ) ;
#28975=VERTEX_POINT ( 'NONE', #89000 ) ;
#28980=CARTESIAN_POINT ( 'NONE',  ( 110.5552498863747246, -46.59121243395724576, 37.84705384733994293 ) ) ;
#28983=CARTESIAN_POINT ( 'NONE',  ( 104.4081006704565908, -46.45808914256989652, 73.36479194333554688 ) ) ;
#28984=CARTESIAN_POINT ( 'NONE',  ( 110.1509004715571791, -26.04776408289588474, 64.85276813305395649 ) ) ;
#28985=DIRECTION ( 'NONE',  ( -0.9254794337955620787, -0.3787978585227822492, 0.000000000000000000 ) ) ;
#28986=CARTESIAN_POINT ( 'NONE',  ( 114.2249171546290967, -45.12625265263328345, 149.1508633711489722 ) ) ;
#28987=CARTESIAN_POINT ( 'NONE',  ( 108.4174892476684704, -26.73503592697917597, 70.96895860960096059 ) ) ;
#28989=CARTESIAN_POINT ( 'NONE',  ( 130.1657039024480582, -18.82844715994099971, 168.9256252759120116 ) ) ;
#28993=CARTESIAN_POINT ( 'NONE',  ( 99.99294959284291906, -33.44233276930008714, 9.125625275910962841 ) ) ;
#28994=LINE ( 'NONE', #72115, #68861 ) ;
#28995=EDGE_CURVE ( 'NONE', #85897, #26492, #40904, .T. ) ;
#28997=CARTESIAN_POINT ( 'NONE',  ( 25.56670390244744695, -48.82844715994178841, 173.2178068554150627 ) ) ;
#28998=CARTESIAN_POINT ( 'NONE',  ( 96.60586043895887087, -37.15609470439714102, 161.3584824187679487 ) ) ;
#29001=CARTESIAN_POINT ( 'NONE',  ( 105.1068790668079203, -26.46800427226792962, 231.2270538473399597 ) ) ;
#29002=CARTESIAN_POINT ( 'NONE',  ( 116.5728860035299164, -32.34523831224304047, 100.1699109901969535 ) ) ;
#29004=CARTESIAN_POINT ( 'NONE',  ( 46.32460016641637424, -48.34074026909789268, 180.4678068554150911 ) ) ;
#29006=CARTESIAN_POINT ( 'NONE',  ( 72.26648329127297643, -71.52944715994142655, 342.9256252759110453 ) ) ;
#29009=ORIENTED_EDGE ( 'NONE', *, *, #71557, .F. ) ;
#29011=ADVANCED_FACE ( 'NONE', ( #82202 ), #88561, .T. ) ;
#29012=CIRCLE ( 'NONE', #13061, 2.117000000000000881 ) ;
#29013=ORIENTED_EDGE ( 'NONE', *, *, #37803, .T. ) ;
#29015=CARTESIAN_POINT ( 'NONE',  ( 103.9393079366161032, -26.78443525705497663, 246.3184824187679567 ) ) ;
#29020=CARTESIAN_POINT ( 'NONE',  ( 176.7738106835046779, -48.62134037887552296, 300.4678068554149490 ) ) ;
#29021=DIRECTION ( 'NONE',  ( 0.7071067811865171526, 0.7071067811865779928, 7.071067811865162747E-16 ) ) ;
#29022=DIRECTION ( 'NONE',  ( 0.000000000000000000, 0.000000000000000000, 1.000000000000000000 ) ) ;
#29023=CARTESIAN_POINT ( 'NONE',  ( 96.63682800883232460, -32.99879952304045361, 26.06514908543494613 ) ) ;
#29024=ORIENTED_EDGE ( 'NONE', *, *, #68447, .T. ) ;
#29027=CARTESIAN_POINT ( 'NONE',  ( 108.4189123056540609, -26.73521668993834055, 15.97197629934867358 ) ) ;
#29028=CARTESIAN_POINT ( 'NONE',  ( 100.4593337790148837, -29.47290724209160828, 281.6641967044818671 ) ) ;
#29030=CARTESIAN_POINT ( 'NONE',  ( 25.56670390244748603, -48.82844715994178841, 134.7178068554150627 ) ) ;
#29031=CARTESIAN_POINT ( 'NONE',  ( 98.32242264099485851, -42.30440888850449710, 137.7661014663869992 ) ) ;
#29033=CARTESIAN_POINT ( 'NONE',  ( 107.0664832912750057, -36.72944715993903486, 9.425625275910970657 ) ) ;
#29034=ORIENTED_EDGE ( 'NONE', *, *, #74084, .F. ) ;
#29035=CARTESIAN_POINT ( 'NONE',  ( 116.8172847295623598, -34.15354512507032325, 180.0314075673595937 ) ) ;
#29036=CARTESIAN_POINT ( 'NONE',  ( 97.70650630222581867, -40.25117133593911234, 57.61283866776680185 ) ) ;
#29037=ORIENTED_EDGE ( 'NONE', *, *, #6855, .F. ) ;
#29041=CARTESIAN_POINT ( 'NONE',  ( 109.5509076938284068, -28.22321920626787062, 256.2815833058970725 ) ) ;
#29042=DIRECTION ( 'NONE',  ( 0.000000000000000000, 0.000000000000000000, 1.000000000000000000 ) ) ;
#29043=CARTESIAN_POINT ( 'NONE',  ( 51.34673845256487823, -36.02818131005847135, 193.9678068554150911 ) ) ;
#29044=EDGE_CURVE ( 'NONE', #76131, #9747, #74924, .T. ) ;
#29045=CARTESIAN_POINT ( 'NONE',  ( 97.06107109413245837, -37.99641193787602589, 86.42729194052971309 ) ) ;
#29047=EDGE_LOOP ( 'NONE', ( #8839, #71526, #83882, #68263 ) ) ;
#29048=AXIS2_PLACEMENT_3D ( 'NONE', #49117, #28701, #50018 ) ;
#29051=ORIENTED_EDGE ( 'NONE', *, *, #41289, .F. ) ;
#29052=CARTESIAN_POINT ( 'NONE',  ( 101.7107321646854246, -27.74380102040660390, 85.50419670448295051 ) ) ;
#29053=ORIENTED_EDGE ( 'NONE', *, *, #44822, .F. ) ;
#29054=CARTESIAN_POINT ( 'NONE',  ( 98.56159230830689921, -41.41319107723295900, 26.14956268521895311 ) ) ;
#29055=CARTESIAN_POINT ( 'NONE',  ( 116.3254862984629909, -32.93730789470958342, 129.1356252759109680 ) ) ;
#29056=CARTESIAN_POINT ( 'NONE',  ( 113.8941270090217444, -29.67983328691845557, 174.4641967044829585 ) ) ;
#29057=CARTESIAN_POINT ( 'NONE',  ( 34.67381068360400320, -28.98061976758901181, 342.9256252759109884 ) ) ;
#29060=LINE ( 'NONE', #35860, #100 ) ;
#29061=CARTESIAN_POINT ( 'NONE',  ( 116.1773114014176969, -43.03338396708490166, 9.356577656862985037 ) ) ;
#29065=CARTESIAN_POINT ( 'NONE',  ( 188.5667039024479834, -67.87844715994100397, 293.2178068554150627 ) ) ;
#29066=VERTEX_POINT ( 'NONE', #40829 ) ;
#29067=CARTESIAN_POINT ( 'NONE',  ( 117.2057360052074415, -34.12396560160815540, 120.0270538473389479 ) ) ;
#29068=ADVANCED_FACE ( 'NONE', ( #6322 ), #89910, .F. ) ;
#29070=ORIENTED_EDGE ( 'NONE', *, *, #17511, .T. ) ;
#29071=EDGE_LOOP ( 'NONE', ( #83372, #6642 ) ) ;
#29074=CARTESIAN_POINT ( 'NONE',  ( 29.56648329127400388, 15.62155284005900491, 328.6381252759109088 ) ) ;
#29077=DIRECTION ( 'NONE',  ( 0.000000000000000000, 0.000000000000000000, -1.000000000000000000 ) ) ;
#29078=PLANE ( 'NONE',  #14193 ) ;
#29079=CARTESIAN_POINT ( 'NONE',  ( 97.07537224739735393, -33.75284044148263973, 27.09562527591097236 ) ) ;
#29080=ADVANCED_FACE ( 'NONE', ( #76710 ), #75815, .F. ) ;
#29084=EDGE_CURVE ( 'NONE', #30532, #52826, #81537, .T. ) ;
#29085=AXIS2_PLACEMENT_3D ( 'NONE', #56214, #83966, #41251 ) ;
#29086=CARTESIAN_POINT ( 'NONE',  ( 194.5667039024485234, -47.82844715993405060, 180.4678068554150343 ) ) ;
#29087=ORIENTED_EDGE ( 'NONE', *, *, #17423, .F. ) ;
#29088=ORIENTED_EDGE ( 'NONE', *, *, #61140, .F. ) ;
#29089=CARTESIAN_POINT ( 'NONE',  ( 168.0371591254543944, -48.62818131005519007, 237.4678068554150059 ) ) ;
#29091=ADVANCED_FACE ( 'NONE', ( #7669 ), #81752, .T. ) ;
#29094=AXIS2_PLACEMENT_3D ( 'NONE', #448, #28141, #47237 ) ;
#29095=CARTESIAN_POINT ( 'NONE',  ( 106.5889295881363950, -27.03189230550456656, 194.5381341137909601 ) ) ;
#29097=CARTESIAN_POINT ( 'NONE',  ( 163.0664832912739826, -0.2185775633789972805, 333.4006252759120343 ) ) ;
#29098=CARTESIAN_POINT ( 'NONE',  ( 103.8276485124378183, -46.72253193893131140, 82.32705384733995402 ) ) ;
#29099=ORIENTED_EDGE ( 'NONE', *, *, #53251, .T. ) ;
#29100=CARTESIAN_POINT ( 'NONE',  ( 172.5664832912728457, -18.82844715994071194, 141.9256252759118979 ) ) ;
#29101=ORIENTED_EDGE ( 'NONE', *, *, #22173, .F. ) ;
#29102=VECTOR ( 'NONE', #24319, 1000.000000000000000 ) ;
#29103=CARTESIAN_POINT ( 'NONE',  ( 106.0291822676640408, -26.77097407813891650, 276.1590324519580122 ) ) ;
#29104=EDGE_CURVE ( 'NONE', #73470, #34867, #7527, .T. ) ;
#29106=CARTESIAN_POINT ( 'NONE',  ( 167.2371591254545820, -47.82818131005522133, 117.4678068554150485 ) ) ;
#29107=ORIENTED_EDGE ( 'NONE', *, *, #46285, .T. ) ;
#29108=FACE_OUTER_BOUND ( 'NONE', #2278, .T. ) ;
#29110=AXIS2_PLACEMENT_3D ( 'NONE', #2022, #29282, #22034 ) ;
#29113=CARTESIAN_POINT ( 'NONE',  ( 98.84041870859987000, -43.22715631800404879, 91.85848241876892928 ) ) ;
#29118=ORIENTED_EDGE ( 'NONE', *, *, #4599, .T. ) ;
#29121=EDGE_CURVE ( 'NONE', #18060, #63362, #77610, .T. ) ;
#29122=CARTESIAN_POINT ( 'NONE',  ( 105.7995185446386444, -26.72403495942892349, 155.1772919380402129 ) ) ;
#29123=EDGE_CURVE ( 'NONE', #64715, #17090, #29460, .T. ) ;
#29124=DIRECTION ( 'NONE',  ( 0.000000000000000000, 0.000000000000000000, -1.000000000000000000 ) ) ;
#29125=CIRCLE ( 'NONE', #68282, 10.00000000000002487 ) ;
#29126=CARTESIAN_POINT ( 'NONE',  ( 114.0366484478682310, -28.94779845652852757, 110.4956252759109816 ) ) ;
#29127=ADVANCED_FACE ( 'NONE', ( #22656 ), #64874, .F. ) ;
#29129=CYLINDRICAL_SURFACE ( 'NONE', #28212, 0.5000000000000031086 ) ;
#29134=CARTESIAN_POINT ( 'NONE',  ( 96.37928053093618530, -33.66421044892481262, 137.1041967044819501 ) ) ;
#29136=FACE_OUTER_BOUND ( 'NONE', #13219, .T. ) ;
#29137=ORIENTED_EDGE ( 'NONE', *, *, #49043, .F. ) ;
#29138=CARTESIAN_POINT ( 'NONE',  ( 110.0853110376240664, -46.03288293484944660, 8.827053847338950376 ) ) ;
#29139=DIRECTION ( 'NONE',  ( -0.7071067811856560636, -0.7071067811874389708, 0.000000000000000000 ) ) ;
#29141=LINE ( 'NONE', #1882, #85047 ) ;
#29143=CARTESIAN_POINT ( 'NONE',  ( 63.03715912545639100, -24.42818131006017168, 180.4678068554151196 ) ) ;
#29144=CARTESIAN_POINT ( 'NONE',  ( 123.6837132603318423, -20.11243780205705534, 239.5838068554170377 ) ) ;
#29145=CARTESIAN_POINT ( 'NONE',  ( 107.4826147187165333, -46.50135945624624156, 237.6099109901969655 ) ) ;
#29146=EDGE_LOOP ( 'NONE', ( #57435, #2382 ) ) ;
#29147=ORIENTED_EDGE ( 'NONE', *, *, #3689, .F. ) ;
#29148=CARTESIAN_POINT ( 'NONE',  ( 98.18569924386140713, -36.28921507361370402, 167.7187261630399462 ) ) ;
#29149=CARTESIAN_POINT ( 'NONE',  ( 131.3167039024479834, -50.82844715994100682, 198.9178068554149945 ) ) ;
#29150=CARTESIAN_POINT ( 'NONE',  ( 101.4552306925257454, -43.61128330217721327, 8.464440448754938728 ) ) ;
#29152=DIRECTION ( 'NONE',  ( 1.000000000000000000, 1.261617073437676668E-15, 9.462128050782575008E-16 ) ) ;
#29153=DIRECTION ( 'NONE',  ( 0.000000000000000000, -1.000000000000000000, 0.000000000000000000 ) ) ;
#29155=LINE ( 'NONE', #41857, #17364 ) ;
#29156=CARTESIAN_POINT ( 'NONE',  ( 97.79822847042071032, -40.48439528968561518, 37.63249612555365786 ) ) ;
#29157=CARTESIAN_POINT ( 'NONE',  ( 113.0129699484216133, -46.01939436189644539, 218.0175300378159591 ) ) ;
#29158=CARTESIAN_POINT ( 'NONE',  ( 97.81480632908598238, -40.51613010894325839, 171.6358981596145270 ) ) ;
#29159=VERTEX_POINT ( 'NONE', #850 ) ;
#29160=VECTOR ( 'NONE', #78412, 1000.000000000000000 ) ;
#29164=CARTESIAN_POINT ( 'NONE',  ( 112.0669571316796151, -45.48782181672719815, 123.9881978270240950 ) ) ;
#29165=LINE ( 'NONE', #64580, #33208 ) ;
#29167=CARTESIAN_POINT ( 'NONE',  ( 96.86520444330115254, -38.59296402346411980, 47.48229194257691432 ) ) ;
#29169=VERTEX_POINT ( 'NONE', #43060 ) ;
#29170=CIRCLE ( 'NONE', #84305, 2.500000000000002220 ) ;
#29172=EDGE_CURVE ( 'NONE', #76706, #65464, #88787, .T. ) ;
#29174=CARTESIAN_POINT ( 'NONE',  ( 111.1275225509982505, -27.12762490620188771, 244.7584824187679544 ) ) ;
#29181=CARTESIAN_POINT ( 'NONE',  ( 109.1158479366964684, -45.13783758831200998, 85.57285227435401964 ) ) ;
#29182=CARTESIAN_POINT ( 'NONE',  ( 103.7162039098101332, -26.17194585468624624, 201.3089586092439731 ) ) ;
#29187=EDGE_CURVE ( 'NONE', #87997, #46741, #9458, .T. ) ;
#29188=CARTESIAN_POINT ( 'NONE',  ( 138.0667039024479550, -26.72944715994091069, 239.5838068554170377 ) ) ;
#29191=AXIS2_PLACEMENT_3D ( 'NONE', #21746, #56685, #63507 ) ;
#29192=VERTEX_POINT ( 'NONE', #56698 ) ;
#29194=FACE_OUTER_BOUND ( 'NONE', #46671, .T. ) ;
#29196=ORIENTED_EDGE ( 'NONE', *, *, #18301, .T. ) ;
#29198=ADVANCED_FACE ( 'NONE', ( #63071 ), #70799, .T. ) ;
#29199=CARTESIAN_POINT ( 'NONE',  ( 98.34984597051438016, -31.65660619317119640, 41.90638639042374791 ) ) ;
#29200=CARTESIAN_POINT ( 'NONE',  ( 113.7853715510712789, -42.80144937323932908, 82.67622935188595079 ) ) ;
#29202=CARTESIAN_POINT ( 'NONE',  ( 117.4518178387850895, -35.59314106485747686, 278.9127681330539872 ) ) ;
#29205=CIRCLE ( 'NONE', #79988, 0.5000000000000004441 ) ;
#29206=EDGE_CURVE ( 'NONE', #68878, #13709, #20430, .T. ) ;
#29207=EDGE_LOOP ( 'NONE', ( #37131, #16904 ) ) ;
#29208=EDGE_LOOP ( 'NONE', ( #30376, #39389 ) ) ;
#29211=LINE ( 'NONE', #49624, #75960 ) ;
#29212=CARTESIAN_POINT ( 'NONE',  ( 116.7274023843879718, -38.25590632018516857, 113.7013395616259857 ) ) ;
#29213=CARTESIAN_POINT ( 'NONE',  ( 117.2063690954211808, -34.12380291655402687, 124.0270538473399426 ) ) ;
#29214=CARTESIAN_POINT ( 'NONE',  ( 117.5632142390390555, -36.54506796471968499, 288.8413395616251478 ) ) ;
#29215=ORIENTED_EDGE ( 'NONE', *, *, #66563, .T. ) ;
#29216=CARTESIAN_POINT ( 'NONE',  ( 96.68196755257399388, -35.80810936406337674, 231.2556252759109725 ) ) ;
#29217=DIRECTION ( 'NONE',  ( 2.999999999999999839E-15, -1.000000000000000000, 2.999999999999999900E-30 ) ) ;
#29219=DIRECTION ( 'NONE',  ( 1.000000000000000000, 4.163336342344333240E-14, 0.000000000000000000 ) ) ;
#29222=CARTESIAN_POINT ( 'NONE',  ( 105.1030388873302854, -25.43975401280837900, 322.2645585102944779 ) ) ;
#29227=CARTESIAN_POINT ( 'NONE',  ( 116.3212776292296127, -32.94146857471318413, 287.6356252759109680 ) ) ;
#29228=DIRECTION ( 'NONE',  ( 0.000000000000000000, 0.000000000000000000, -1.000000000000000000 ) ) ;
#29230=CARTESIAN_POINT ( 'NONE',  ( 100.9546727909157511, -28.70702574251799533, 260.5939586112514803 ) ) ;
#29231=VERTEX_POINT ( 'NONE', #84887 ) ;
#29232=DIRECTION ( 'NONE',  ( 1.000000000000000000, 4.299999999999999979E-14, 1.000000000000000078E-15 ) ) ;
#29233=CARTESIAN_POINT ( 'NONE',  ( 101.6391055438642894, -45.65636906804281381, 247.1413395616249602 ) ) ;
#29234=CARTESIAN_POINT ( 'NONE',  ( 98.26135236841564335, -42.31085888804770434, 182.7756252759109543 ) ) ;
#29235=CARTESIAN_POINT ( 'NONE',  ( 95.23451729606020422, -35.71612027476381002, 32.25848241876794020 ) ) ;
#29237=VECTOR ( 'NONE', #87205, 1000.000000000000000 ) ;
#29238=CARTESIAN_POINT ( 'NONE',  ( 72.26648329127297643, -71.52944715994141234, 361.9756252759109998 ) ) ;
#29239=CARTESIAN_POINT ( 'NONE',  ( 99.04406186115555499, -42.84125764320888408, 46.84395860957398128 ) ) ;
#29243=DIRECTION ( 'NONE',  ( -4.237773401492740281E-14, 1.000000000000000000, 0.000000000000000000 ) ) ;
#29244=ORIENTED_EDGE ( 'NONE', *, *, #12391, .F. ) ;
#29245=CARTESIAN_POINT ( 'NONE',  ( 107.7643578131546178, -45.27140672887451700, 177.0638483995059858 ) ) ;
#29246=CARTESIAN_POINT ( 'NONE',  ( 99.04370088267752692, -42.84071521736686350, 186.8444288791077668 ) ) ;
#29248=DIRECTION ( 'NONE',  ( -0.9963424814100680926, 0.08544974978095698503, 0.000000000000000000 ) ) ;
#29249=CARTESIAN_POINT ( 'NONE',  ( 97.44537786355549258, -42.12371753947135744, 177.7451490854349743 ) ) ;
#29250=CARTESIAN_POINT ( 'NONE',  ( 118.5256205435843526, -36.72944715994100306, 277.6356252759110248 ) ) ;
#29252=CARTESIAN_POINT ( 'NONE',  ( 110.6700764351487578, -27.40068518752502413, 85.78334170510873946 ) ) ;
#29254=FACE_OUTER_BOUND ( 'NONE', #36445, .T. ) ;
#29255=DIRECTION ( 'NONE',  ( 0.000000000000000000, 0.000000000000000000, -1.000000000000000000 ) ) ;
#29256=CARTESIAN_POINT ( 'NONE',  ( 112.4472966703649348, -46.45872411559678028, 102.9784824187679817 ) ) ;
#29257=ORIENTED_EDGE ( 'NONE', *, *, #62192, .F. ) ;
#29260=CARTESIAN_POINT ( 'NONE',  ( 101.8597501770084364, -45.35270844728685802, 48.57586902018196184 ) ) ;
#29262=CARTESIAN_POINT ( 'NONE',  ( 97.28849942844340148, -36.49606577720026479, 192.3070538473389490 ) ) ;
#29263=CARTESIAN_POINT ( 'NONE',  ( 115.7831076883988146, -41.80230947738378688, 38.40645861222698443 ) ) ;
#29264=CARTESIAN_POINT ( 'NONE',  ( 142.0664832912740110, -8.729447159940995959, -4.824374724088994704 ) ) ;
#29266=AXIS2_PLACEMENT_3D ( 'NONE', #38032, #23967, #86191 ) ;
#29267=CARTESIAN_POINT ( 'NONE',  ( 107.0664832912739968, -36.72944715994100306, 287.6356252759109680 ) ) ;
#29268=DIRECTION ( 'NONE',  ( 0.000000000000000000, 0.000000000000000000, 1.000000000000000000 ) ) ;
#29270=CARTESIAN_POINT ( 'NONE',  ( 114.7100688122353063, -43.78666090992615523, 123.2327681330539519 ) ) ;
#29271=ORIENTED_EDGE ( 'NONE', *, *, #52324, .F. ) ;
#29273=AXIS2_PLACEMENT_3D ( 'NONE', #45162, #24737, #44272 ) ;
#29274=ORIENTED_EDGE ( 'NONE', *, *, #34961, .T. ) ;
#29277=DIRECTION ( 'NONE',  ( 1.000000000000000000, 4.237773401492740281E-14, 0.000000000000000000 ) ) ;
#29278=B_SPLINE_CURVE_WITH_KNOTS ( 'NONE', 3,
 ( #75031, #32332, #87766, #18720, #89115, #81860, #33247, #26874, #61829, #25530, #19177, #46846, #54550, #5556, #53203, #26436, #67306, #89563, #60484, #80972, #82766, #88233, #25986, #46403, #45947, #47303, #73686, #12821, #43178 ),
 .UNSPECIFIED., .F., .F.,
 ( 4, 2, 1, 1, 1, 1, 1, 2, 2, 2, 2, 2, 2, 2, 2, 2, 4 ),
 ( 0.5000605868651970543, 0.5003046979067664601, 0.5005488089483359770, 0.5010370310314751219, 0.5020134751977542997, 0.5039663635303122113, 0.5078721401954277015, 0.5156836935256587928, 0.5313068001861211975, 0.5625530135070464510, 0.6250454401488969580, 0.6875378667907473540, 0.7500302934325979720, 0.8125227200744484790, 0.8750151467162989860, 0.9375075733581494930, 1.000000000000000000 ),
 .UNSPECIFIED. ) ;
#29280=CARTESIAN_POINT ( 'NONE',  ( 104.3825147926133354, -28.50161402210781603, 208.1576141791150008 ) ) ;
#29282=DIRECTION ( 'NONE',  ( -0.7071067811865483499, -0.7071067811865466846, -7.071067811865491110E-16 ) ) ;
#29283=EDGE_CURVE ( 'NONE', #53694, #22477, #75544, .T. ) ;
#29284=CARTESIAN_POINT ( 'NONE',  ( 111.7942743463426609, -25.86259492108981206, 134.7499109901969518 ) ) ;
#29286=CARTESIAN_POINT ( 'NONE',  ( 179.7974245136200011, -36.32844715994040996, 117.4678068554150627 ) ) ;
#29287=VERTEX_POINT ( 'NONE', #25312 ) ;
#29289=ORIENTED_EDGE ( 'NONE', *, *, #73052, .F. ) ;
#29290=CIRCLE ( 'NONE', #87313, 2.750000000000002665 ) ;
#29294=EDGE_LOOP ( 'NONE', ( #10527, #58476, #64711, #26735 ) ) ;
#29295=DIRECTION ( 'NONE',  ( -0.7071067812159692600, -0.7071067811571258854, 2.899137802744100722E-29 ) ) ;
#29297=CARTESIAN_POINT ( 'NONE',  ( 115.4467593082293178, -40.97768201889641659, 244.8968214011349573 ) ) ;
#29298=EDGE_CURVE ( 'NONE', #63362, #24618, #4434, .T. ) ;
#29300=VERTEX_POINT ( 'NONE', #46635 ) ;
#29302=CARTESIAN_POINT ( 'NONE',  ( 116.3379421530591884, -39.39079624489408360, 9.635625275910941312 ) ) ;
#29303=DIRECTION ( 'NONE',  ( 1.387778780781444492E-15, 0.000000000000000000, -1.000000000000000000 ) ) ;
#29306=EDGE_CURVE ( 'NONE', #28582, #34717, #39289, .T. ) ;
#29307=CARTESIAN_POINT ( 'NONE',  ( 111.0058300909787761, -45.92119593049321935, 112.8986727163515269 ) ) ;
#29309=EDGE_LOOP ( 'NONE', ( #55909, #88139, #61273 ) ) ;
#29310=EDGE_CURVE ( 'NONE', #68446, #83210, #80302, .T. ) ;
#29311=CARTESIAN_POINT ( 'NONE',  ( 113.9883325317156135, -31.53436023685440048, 262.1690427505439516 ) ) ;
#29312=CARTESIAN_POINT ( 'NONE',  ( 108.8526476014722277, -47.02293932800507292, 167.7127681330539701 ) ) ;
#29313=CARTESIAN_POINT ( 'NONE',  ( 109.5033840998384136, -46.84330794493983774, 132.7641967044819751 ) ) ;
#29314=DIRECTION ( 'NONE',  ( -0.9254794337955620787, -0.3787978585227823602, 0.000000000000000000 ) ) ;
#29315=CARTESIAN_POINT ( 'NONE',  ( 104.4105741502040701, -26.00004237129247642, 236.2575300378159682 ) ) ;
#29316=CARTESIAN_POINT ( 'NONE',  ( 30.48091746481746611, -48.32844715994156815, 129.9678068554150627 ) ) ;
#29326=CARTESIAN_POINT ( 'NONE',  ( 98.34291691341793751, -29.86560907334282788, 200.8080062282919869 ) ) ;
#29328=CARTESIAN_POINT ( 'NONE',  ( 108.5898285964631640, -47.07861824576353627, 142.6927681330539883 ) ) ;
#29329=CARTESIAN_POINT ( 'NONE',  ( 41.56648329127399677, -18.82844715994099971, 76.80862527591200717 ) ) ;
#29333=DIRECTION ( 'NONE',  ( 0.000000000000000000, 0.000000000000000000, 1.000000000000000000 ) ) ;
#29334=CARTESIAN_POINT ( 'NONE',  ( 106.5683798796750779, -47.15615894637585370, 243.5384824187679556 ) ) ;
#29337=CIRCLE ( 'NONE', #22145, 2.517499999999998739 ) ;
#29338=CARTESIAN_POINT ( 'NONE',  ( 107.3241674272228892, -25.27320757387406402, 321.5865679059475610 ) ) ;
#29339=DIRECTION ( 'NONE',  ( -0.7071067811567173234, 0.7071067812163779331, 0.000000000000000000 ) ) ;
#29340=CARTESIAN_POINT ( 'NONE',  ( 115.7831076753790143, -41.80230950073445939, 259.4064586101131908 ) ) ;
#29342=DIRECTION ( 'NONE',  ( 0.000000000000000000, 0.000000000000000000, -1.000000000000000000 ) ) ;
#29343=CARTESIAN_POINT ( 'NONE',  ( 114.4461924768642405, -27.39302975889309266, 274.5441967044824878 ) ) ;
#29346=CARTESIAN_POINT ( 'NONE',  ( 101.7582431991767464, -45.72772181880441167, 162.1527681330539679 ) ) ;
#29347=CARTESIAN_POINT ( 'NONE',  ( 116.9748844278823015, -33.48813965163778050, 85.07848241876791917 ) ) ;
#29348=CARTESIAN_POINT ( 'NONE',  ( 113.7785824165150643, -44.76317014998476651, 189.1299109901969757 ) ) ;
#29350=ADVANCED_FACE ( 'NONE', ( #74367, #37618 ), #52097, .F. ) ;
#29351=DIRECTION ( 'NONE',  ( 1.639958061481212836E-42, -4.100000000000000342E-29, -1.000000000000000000 ) ) ;
#29352=CARTESIAN_POINT ( 'NONE',  ( 33.78309357196401663, -29.99615139349950965, -5.074374724088000832 ) ) ;
#29354=DIRECTION ( 'NONE',  ( 1.000000000000000000, 0.000000000000000000, 0.000000000000000000 ) ) ;
#29355=CARTESIAN_POINT ( 'NONE',  ( 71.25580610988301089, -82.12815647064932989, 394.9756252759102040 ) ) ;
#29357=FACE_OUTER_BOUND ( 'NONE', #62259, .T. ) ;
#29358=ORIENTED_EDGE ( 'NONE', *, *, #48571, .F. ) ;
#29360=CARTESIAN_POINT ( 'NONE',  ( 172.5664832912740110, -32.07844715994070839, 78.92562527591199739 ) ) ;
#29362=CIRCLE ( 'NONE', #81631, 0.5000000000000004441 ) ;
#29363=CARTESIAN_POINT ( 'NONE',  ( 96.67837842349544530, -37.29153504031420141, 72.36991099019596163 ) ) ;
#29364=DIRECTION ( 'NONE',  ( 0.000000000000000000, 0.000000000000000000, -1.000000000000000000 ) ) ;
#29366=DIRECTION ( 'NONE',  ( 1.000000000000000000, 0.000000000000000000, 0.000000000000000000 ) ) ;
#29368=CARTESIAN_POINT ( 'NONE',  ( 98.22454660805831850, -42.33418938753942484, 182.7756252759109543 ) ) ;
#29370=CARTESIAN_POINT ( 'NONE',  ( 98.72788526414296939, -31.75567473670096774, 280.3209912566482558 ) ) ;
#29371=ORIENTED_EDGE ( 'NONE', *, *, #39402, .F. ) ;
#29375=EDGE_CURVE ( 'NONE', #44052, #74767, #74110, .T. ) ;
#29376=DIRECTION ( 'NONE',  ( -1.000000000000000000, -2.756263715554006823E-15, 0.000000000000000000 ) ) ;
#29377=CARTESIAN_POINT ( 'NONE',  ( 179.1667039024439703, -26.71338133339251542, 342.9256252759109884 ) ) ;
#29378=CARTESIAN_POINT ( 'NONE',  ( 113.2449868381543894, -28.75828141597592591, 160.5523427473990239 ) ) ;
#29382=DIRECTION ( 'NONE',  ( 0.000000000000000000, 0.000000000000000000, -1.000000000000000000 ) ) ;
#29383=CARTESIAN_POINT ( 'NONE',  ( 72.06648329127402519, -45.72944715994106701, -4.824374724089063982 ) ) ;
#29384=CARTESIAN_POINT ( 'NONE',  ( 97.09625384711483775, -33.75906160244644383, 31.09562527591097592 ) ) ;
#29385=ORIENTED_EDGE ( 'NONE', *, *, #60273, .F. ) ;
#29386=CYLINDRICAL_SURFACE ( 'NONE', #33020, 10.00000000000000888 ) ;
#29388=CARTESIAN_POINT ( 'NONE',  ( 99.83919217201646745, -32.93524248800951426, 133.7595189410199623 ) ) ;
#29390=EDGE_CURVE ( 'NONE', #36063, #20396, #63940, .T. ) ;
#29391=CARTESIAN_POINT ( 'NONE',  ( 97.33746229064173860, -34.07254350826487155, 96.11491520920078813 ) ) ;
#29393=AXIS2_PLACEMENT_3D ( 'NONE', #69208, #6980, #15143 ) ;
#29394=DIRECTION ( 'NONE',  ( -1.000000000000000000, -5.512527431108013646E-15, 0.000000000000000000 ) ) ;
#29395=VERTEX_POINT ( 'NONE', #51664 ) ;
#29399=EDGE_LOOP ( 'NONE', ( #20891, #23725, #25825, #27925, #71084 ) ) ;
#29401=CARTESIAN_POINT ( 'NONE',  ( 116.0874278420761527, -39.35605806303598797, 135.0206309249449532 ) ) ;
#29402=EDGE_CURVE ( 'NONE', #67223, #49327, #4404, .T. ) ;
#29403=DIRECTION ( 'NONE',  ( 1.639958061481212836E-42, -4.100000000000000342E-29, -1.000000000000000000 ) ) ;
#29404=CARTESIAN_POINT ( 'NONE',  ( 102.9625221110550513, -46.33646342331733337, 88.25562527591095829 ) ) ;
#29405=CARTESIAN_POINT ( 'NONE',  ( 105.7149664547234806, -46.72378104326954684, 17.46898624714683024 ) ) ;
#29406=ORIENTED_EDGE ( 'NONE', *, *, #26450, .F. ) ;
#29408=ORIENTED_EDGE ( 'NONE', *, *, #52115, .T. ) ;
#29409=EDGE_CURVE ( 'NONE', #36232, #12855, #53435, .T. ) ;
#29410=CIRCLE ( 'NONE', #45399, 2.749999999999974687 ) ;
#29411=CARTESIAN_POINT ( 'NONE',  ( 96.05424466460999611, -37.92361698284899774, 81.40038718067299328 ) ) ;
#29412=ORIENTED_EDGE ( 'NONE', *, *, #37503, .T. ) ;
#29413=CARTESIAN_POINT ( 'NONE',  ( 114.5610390845466355, -30.44493693613343765, 269.3813395616256798 ) ) ;
#29414=CARTESIAN_POINT ( 'NONE',  ( 116.3696522983621549, -44.11004992080503229, 194.2927681330539542 ) ) ;
#29415=CARTESIAN_POINT ( 'NONE',  ( 21.56670390244604718, -23.42844715994195326, 180.4678068554150911 ) ) ;
#29417=CARTESIAN_POINT ( 'NONE',  ( 113.9864041344766861, -28.11035927269328738, 115.5261014663869474 ) ) ;
#29419=VERTEX_POINT ( 'NONE', #55236 ) ;
#29420=CARTESIAN_POINT ( 'NONE',  ( 66.20668838251407351, -0.9299196430550271675, 542.9756252759101471 ) ) ;
#29421=VERTEX_POINT ( 'NONE', #20745 ) ;
#29423=ORIENTED_EDGE ( 'NONE', *, *, #28035, .T. ) ;
#29424=VERTEX_POINT ( 'NONE', #41611 ) ;
#29425=AXIS2_PLACEMENT_3D ( 'NONE', #16333, #37672, #71308 ) ;
#29426=DIRECTION ( 'NONE',  ( -0.7071067811865614505, -0.7071067811865336949, 0.000000000000000000 ) ) ;
#29428=CARTESIAN_POINT ( 'NONE',  ( 112.1813298990327183, -27.60452245592377807, 34.66991099019695355 ) ) ;
#29429=DIRECTION ( 'NONE',  ( -0.7071067811855830110, -0.7071067811875120235, 0.000000000000000000 ) ) ;
#29430=DIRECTION ( 'NONE',  ( 1.000000000000000000, 4.299999999999999979E-14, 1.000000000000000078E-15 ) ) ;
#29431=CARTESIAN_POINT ( 'NONE',  ( 101.9936209501908309, -45.44607154402763172, 73.15645861009139139 ) ) ;
#29432=CARTESIAN_POINT ( 'NONE',  ( 106.5519926023875712, -26.37212682281782250, 45.12800622829394115 ) ) ;
#29434=CARTESIAN_POINT ( 'NONE',  ( 114.4473569665853603, -28.53271593493113301, 155.5051490854349652 ) ) ;
#29435=CARTESIAN_POINT ( 'NONE',  ( 115.0889047233127513, -30.61763667903340291, 70.34395860933346967 ) ) ;
#29436=CARTESIAN_POINT ( 'NONE',  ( 107.0664832912730020, -36.72944715994189835, 361.9756252759079871 ) ) ;
#29438=CARTESIAN_POINT ( 'NONE',  ( 72.26949937496598864, -71.54137415153812185, 361.9756252759101471 ) ) ;
#29441=ORIENTED_EDGE ( 'NONE', *, *, #64830, .F. ) ;
#29442=CARTESIAN_POINT ( 'NONE',  ( 193.0374249753376432, -23.42844715993431848, 180.4678068554150343 ) ) ;
#29443=CARTESIAN_POINT ( 'NONE',  ( 114.9985205141181837, -29.89647917087096118, 184.3927681330539770 ) ) ;
#29445=CARTESIAN_POINT ( 'NONE',  ( 51.56670390244699576, -19.82844715994031048, -5.074374724088000832 ) ) ;
#29446=CARTESIAN_POINT ( 'NONE',  ( 103.8129894719335624, -48.15035030529833904, 213.3556252759109668 ) ) ;
#29447=CARTESIAN_POINT ( 'NONE',  ( 117.3964687521579293, -38.63454956243933225, 84.68133956162593279 ) ) ;
#29450=CARTESIAN_POINT ( 'NONE',  ( 97.33765849503933509, -34.07180872970644003, 192.1146941698899582 ) ) ;
#29451=CARTESIAN_POINT ( 'NONE',  ( 134.0664832912740110, 0.2215528400590013880, 306.1181252759120071 ) ) ;
#29452=ORIENTED_EDGE ( 'NONE', *, *, #3086, .F. ) ;
#29455=EDGE_CURVE ( 'NONE', #30532, #70798, #88454, .T. ) ;
#29457=EDGE_LOOP ( 'NONE', ( #74072, #3272, #17410, #8671, #51182 ) ) ;
#29458=AXIS2_PLACEMENT_3D ( 'NONE', #41477, #55994, #43272 ) ;
#29459=ORIENTED_EDGE ( 'NONE', *, *, #17987, .F. ) ;
#29460=LINE ( 'NONE', #9026, #37994 ) ;
#29461=CARTESIAN_POINT ( 'NONE',  ( 111.1274376763295635, -27.12782558180003889, 240.7584824187679544 ) ) ;
#29462=CARTESIAN_POINT ( 'NONE',  ( 172.5664832912740110, 0.2215528400590013880, 136.8086252759119645 ) ) ;
#29463=CARTESIAN_POINT ( 'NONE',  ( 136.5763721200466989, -17.60518726038198167, 2.783021291310912027 ) ) ;
#29464=DIRECTION ( 'NONE',  ( 1.000000000000000078E-15, -1.000000000000000083E-30, -1.000000000000000000 ) ) ;
#29465=CARTESIAN_POINT ( 'NONE',  ( 156.5667039024483529, -48.82844715993569196, 290.7178068554149490 ) ) ;
#29466=DIRECTION ( 'NONE',  ( 0.9068632946707805287, -0.4214249218767882610, 8.630465054610985966E-16 ) ) ;
#29467=CARTESIAN_POINT ( 'NONE',  ( 115.4624701790509391, -43.00605189524043936, 28.31562527591097123 ) ) ;
#29472=CARTESIAN_POINT ( 'NONE',  ( 51.03742451361310373, -23.42844715994068849, 193.9678068554150911 ) ) ;
#29475=CARTESIAN_POINT ( 'NONE',  ( 105.8561066403589308, -27.02385992090132305, 266.1756252759109884 ) ) ;
#29476=DIRECTION ( 'NONE',  ( 4.299999999999999979E-14, -1.000000000000000000, 4.400000000000000367E-29 ) ) ;
#29477=AXIS2_PLACEMENT_3D ( 'NONE', #14729, #190, #76044 ) ;
#29478=CARTESIAN_POINT ( 'NONE',  ( 116.2961327041337825, -39.96626766897446714, 129.5584824187679658 ) ) ;
#29479=CARTESIAN_POINT ( 'NONE',  ( 117.0720918726942301, -35.46411075774014421, 28.92716242642622504 ) ) ;
#29482=CARTESIAN_POINT ( 'NONE',  ( 77.44501272126922231, -35.89730640218657243, 2.921034946746044803 ) ) ;
#29484=ORIENTED_EDGE ( 'NONE', *, *, #46767, .T. ) ;
#29486=CARTESIAN_POINT ( 'NONE',  ( 109.5858817268311611, -44.49374890974875285, 10.64523322673399619 ) ) ;
#29487=VECTOR ( 'NONE', #27897, 1000.000000000000000 ) ;
#29488=CARTESIAN_POINT ( 'NONE',  ( 51.06648329127400388, 19.62155284005901024, 339.0006252759110339 ) ) ;
#29489=CARTESIAN_POINT ( 'NONE',  ( 115.0889047252626511, -30.61763668196338628, 84.34395860905816278 ) ) ;
#29490=EDGE_CURVE ( 'NONE', #70034, #17117, #27112, .T. ) ;
#29491=DIRECTION ( 'NONE',  ( 0.000000000000000000, 0.000000000000000000, -1.000000000000000000 ) ) ;
#29492=ORIENTED_EDGE ( 'NONE', *, *, #26398, .F. ) ;
#29493=DIRECTION ( 'NONE',  ( -1.000000000000000078E-15, 1.000000000000000083E-30, 1.000000000000000000 ) ) ;
#29494=DIRECTION ( 'NONE',  ( 0.000000000000000000, 0.000000000000000000, -1.000000000000000000 ) ) ;
#29495=EDGE_CURVE ( 'NONE', #28780, #18226, #12592, .T. ) ;
#29497=CARTESIAN_POINT ( 'NONE',  ( 103.2788000081581288, -47.11369209158109328, 97.28610146638693834 ) ) ;
#29498=ORIENTED_EDGE ( 'NONE', *, *, #79126, .T. ) ;
#29499=EDGE_CURVE ( 'NONE', #2385, #57151, #85744, .T. ) ;
#29500=CARTESIAN_POINT ( 'NONE',  ( 102.3843679657495329, -43.41581164733459985, 279.9080903695913776 ) ) ;
#29502=CARTESIAN_POINT ( 'NONE',  ( 113.2095242374420252, -45.08419629851117350, 183.0689586092449588 ) ) ;
#29504=EDGE_CURVE ( 'NONE', #71916, #17169, #3055, .T. ) ;
#29508=CARTESIAN_POINT ( 'NONE',  ( 99.36487284946518628, -28.73678208742278173, 261.6746728949589169 ) ) ;
#29509=CARTESIAN_POINT ( 'NONE',  ( 111.8140854152826336, -45.56118024207201955, 117.9710264827728707 ) ) ;
#29510=ORIENTED_EDGE ( 'NONE', *, *, #32592, .F. ) ;
#29511=AXIS2_PLACEMENT_3D ( 'NONE', #73891, #88878, #5759 ) ;
#29512=DIRECTION ( 'NONE',  ( 0.000000000000000000, 1.000000000000000000, 0.000000000000000000 ) ) ;
#29514=CARTESIAN_POINT ( 'NONE',  ( 116.8361817273313790, -32.96833395228159702, 135.1184824187679396 ) ) ;
#29515=DIRECTION ( 'NONE',  ( 1.000000000000000078E-15, -1.000000000000000083E-30, -1.000000000000000000 ) ) ;
#29516=VECTOR ( 'NONE', #71435, 999.9999999999998863 ) ;
#29518=ORIENTED_EDGE ( 'NONE', *, *, #86112, .T. ) ;
#29519=ORIENTED_EDGE ( 'NONE', *, *, #72322, .F. ) ;
#29521=CARTESIAN_POINT ( 'NONE',  ( 116.7951252620880922, -39.38782982808247368, 123.6147919394983887 ) ) ;
#29523=CARTESIAN_POINT ( 'NONE',  ( 83.06670390244796920, -58.72944715994098885, 231.5838068554150198 ) ) ;
#29527=CARTESIAN_POINT ( 'NONE',  ( 97.48672026426986292, -32.61689163886055809, 12.00419670448293985 ) ) ;
#29532=ORIENTED_EDGE ( 'NONE', *, *, #36985, .F. ) ;
#29533=DIRECTION ( 'NONE',  ( -0.7071067811571960515, 0.7071067812158990940, 0.000000000000000000 ) ) ;
#29534=VECTOR ( 'NONE', #55675, 1000.000000000000000 ) ;
#29535=DIRECTION ( 'NONE',  ( 0.000000000000000000, -1.000000000000000000, 0.000000000000000000 ) ) ;
#29536=DIRECTION ( 'NONE',  ( 0.000000000000000000, 1.000000000000000000, 0.000000000000000000 ) ) ;
#29537=CARTESIAN_POINT ( 'NONE',  ( 107.0664832912739968, -18.82844715994099971, 168.9256252759119832 ) ) ;
#29538=CARTESIAN_POINT ( 'NONE',  ( 63.03715912545730760, -24.42818131006017879, 300.4678068554150627 ) ) ;
#29539=CARTESIAN_POINT ( 'NONE',  ( 111.4808447759429413, -44.07556959346039349, 237.4295626852199632 ) ) ;
#29540=CARTESIAN_POINT ( 'NONE',  ( 131.0667039024480118, -61.87844715994100397, 231.5838068554150198 ) ) ;
#29541=CARTESIAN_POINT ( 'NONE',  ( 115.7104945841387007, -43.58108136993639903, 44.30514908543492680 ) ) ;
#29543=CARTESIAN_POINT ( 'NONE',  ( 97.50197496249766971, -32.47188371672483242, 100.9927681330539713 ) ) ;
#29545=DIRECTION ( 'NONE',  ( -0.1811243269278930978, 0.9834602067165288952, 0.000000000000000000 ) ) ;
#29546=VERTEX_POINT ( 'NONE', #89805 ) ;
#29547=CARTESIAN_POINT ( 'NONE',  ( 98.34985888866438586, -31.65658484983705634, 66.90645861293477026 ) ) ;
#29548=CARTESIAN_POINT ( 'NONE',  ( 141.0667039024479834, -58.72944715994110254, 198.9178068554149945 ) ) ;
#29550=CARTESIAN_POINT ( 'NONE',  ( 107.0664832912739968, -8.729447159940999512, 284.9256252759119548 ) ) ;
#29551=ORIENTED_EDGE ( 'NONE', *, *, #65386, .F. ) ;
#29552=CARTESIAN_POINT ( 'NONE',  ( 172.5667039024480118, -36.32844715993499563, 180.4678068554150059 ) ) ;
#29553=CARTESIAN_POINT ( 'NONE',  ( 99.04424376774331051, -42.84153041693851804, 272.8435455337404960 ) ) ;
#29554=ADVANCED_FACE ( 'NONE', ( #5781 ), #33472, .F. ) ;
#29556=CARTESIAN_POINT ( 'NONE',  ( 107.0664832912739968, -8.350947159940998787, 335.9181252759120184 ) ) ;
#29558=CARTESIAN_POINT ( 'NONE',  ( 96.05424466460999611, -37.92361698284899774, 81.40038718067299328 ) ) ;
#29559=PRESENTATION_STYLE_ASSIGNMENT (( #16828 ) ) ;
#29561=DIRECTION ( 'NONE',  ( 0.000000000000000000, 1.000000000000000000, 0.000000000000000000 ) ) ;
#29562=DIRECTION ( 'NONE',  ( -0.7071067811865517916, 0.000000000000000000, -0.7071067811865431318 ) ) ;
#29564=DIRECTION ( 'NONE',  ( -1.000000000000000000, -4.299999999999999979E-14, -9.351236661543306751E-17 ) ) ;
#29565=DIRECTION ( 'NONE',  ( 0.7071067811865475727, -0.7071067811865475727, 0.000000000000000000 ) ) ;
#29566=DIRECTION ( 'NONE',  ( 4.194175870806139918E-14, -1.000000000000000000, 0.000000000000000000 ) ) ;
#29567=CARTESIAN_POINT ( 'NONE',  ( 98.82287431334749783, -28.18163096472671469, 111.6870538473389587 ) ) ;
#29568=CARTESIAN_POINT ( 'NONE',  ( 90.44969454456416713, -53.34645651782494724, 218.0711402470150801 ) ) ;
#29569=DIRECTION ( 'NONE',  ( 4.194175870806139918E-14, -1.000000000000000000, 0.000000000000000000 ) ) ;
#29570=DIRECTION ( 'NONE',  ( -1.000000000000000078E-15, 0.000000000000000000, 1.000000000000000000 ) ) ;
#29571=VECTOR ( 'NONE', #80503, 1000.000000000000000 ) ;
#29573=DIRECTION ( 'NONE',  ( 0.7071067811865449082, 0.7071067811865501263, 7.071067811865448709E-16 ) ) ;
#29574=CARTESIAN_POINT ( 'NONE',  ( 116.2045471004837083, -43.06251688283437318, 159.3441967044819592 ) ) ;
#29575=DIRECTION ( 'NONE',  ( 0.000000000000000000, 0.000000000000000000, 1.000000000000000000 ) ) ;
#29576=VERTEX_POINT ( 'NONE', #84359 ) ;
#29577=CARTESIAN_POINT ( 'NONE',  ( 101.9462946551393543, -46.59843102978671681, 13.19562527591094891 ) ) ;
#29584=CARTESIAN_POINT ( 'NONE',  ( 117.3624379696767335, -35.49166588079122420, 238.9337205140069500 ) ) ;
#29585=ORIENTED_EDGE ( 'NONE', *, *, #43798, .T. ) ;
#29587=CARTESIAN_POINT ( 'NONE',  ( 116.1701677112242237, -32.41741342456931818, 210.6101547344689777 ) ) ;
#29588=AXIS2_PLACEMENT_3D ( 'NONE', #1796, #43097, #43993 ) ;
#29589=CARTESIAN_POINT ( 'NONE',  ( 72.25757238336808541, -1.944390235229867425, 361.9756252759101471 ) ) ;
#29590=CARTESIAN_POINT ( 'NONE',  ( 115.5880482615279163, -32.77224410791782816, 55.59205949637296840 ) ) ;
#29591=CONICAL_SURFACE ( 'NONE', #62978, 1.625000000000001332, 1.029744258676650093 ) ;
#29594=CIRCLE ( 'NONE', #32490, 3.250000000000002665 ) ;
#29595=CARTESIAN_POINT ( 'NONE',  ( 107.0664832912739541, -36.72944715994095333, 305.0306255462182321 ) ) ;
#29596=CARTESIAN_POINT ( 'NONE',  ( 192.5667039024475002, -23.42844715993433624, 129.9678068554150343 ) ) ;
#29598=VERTEX_POINT ( 'NONE', #28463 ) ;
#29600=CYLINDRICAL_SURFACE ( 'NONE', #64797, 0.5000000000000031086 ) ;
#29601=CARTESIAN_POINT ( 'NONE',  ( 104.3301552612371381, -26.04411461992200927, 245.2880062282919482 ) ) ;
#29602=DIRECTION ( 'NONE',  ( -0.000000000000000000, 1.000000000000000000, 0.000000000000000000 ) ) ;
#29604=EDGE_CURVE ( 'NONE', #46083, #58766, #317, .T. ) ;
#29605=VERTEX_POINT ( 'NONE', #13947 ) ;
#29606=CARTESIAN_POINT ( 'NONE',  ( 108.3334480785710383, -46.73485935620319509, 87.67729194127437609 ) ) ;
#29608=CARTESIAN_POINT ( 'NONE',  ( 100.8873238325640784, -44.70013431002061566, 123.0511152429078123 ) ) ;
#29610=CARTESIAN_POINT ( 'NONE',  ( 100.9534786964906345, -28.35269599622561643, 26.56610146638693948 ) ) ;
#29611=LINE ( 'NONE', #15996, #87680 ) ;
#29613=CARTESIAN_POINT ( 'NONE',  ( 106.9267702420067678, -26.22618599733332090, 56.08705384733997334 ) ) ;
#29615=CARTESIAN_POINT ( 'NONE',  ( 105.1595199372206793, -47.03071207059073799, 12.42991099019596923 ) ) ;
#29616=VERTEX_POINT ( 'NONE', #56153 ) ;
#29617=EDGE_CURVE ( 'NONE', #30791, #57079, #71212, .T. ) ;
#29618=DIRECTION ( 'NONE',  ( 0.7071067810573865575, 0.7071067813157084769, 7.071067810573858582E-16 ) ) ;
#29621=CARTESIAN_POINT ( 'NONE',  ( 48.45959712127301344, -26.00627455219131789, -5.074374724088000832 ) ) ;
#29622=EDGE_CURVE ( 'NONE', #40569, #53148, #42529, .T. ) ;
#29623=CARTESIAN_POINT ( 'NONE',  ( 101.7674321979440606, -44.34626990135510738, 84.91094751244793315 ) ) ;
#29624=CARTESIAN_POINT ( 'NONE',  ( 97.38187162881654046, -40.64678755884852279, 202.6327681330539860 ) ) ;
#29625=CARTESIAN_POINT ( 'NONE',  ( 179.1667039024474377, -28.27351298636771659, 313.9678068554149490 ) ) ;
#29627=CARTESIAN_POINT ( 'NONE',  ( 51.06670390244799762, -33.35206098992630075, -5.074374724088000832 ) ) ;
#29628=ORIENTED_EDGE ( 'NONE', *, *, #43515, .F. ) ;
#29630=AXIS2_PLACEMENT_3D ( 'NONE', #22764, #30014, #78183 ) ;
#29631=FACE_OUTER_BOUND ( 'NONE', #12234, .T. ) ;
#29633=ORIENTED_EDGE ( 'NONE', *, *, #55194, .T. ) ;
#29634=FACE_OUTER_BOUND ( 'NONE', #41993, .T. ) ;
#29636=CARTESIAN_POINT ( 'NONE',  ( 97.79819947057245599, -40.48432372764506226, 42.63278048571394407 ) ) ;
#29637=CARTESIAN_POINT ( 'NONE',  ( 115.7815527111783069, -39.19119195442627301, 143.0419436376009799 ) ) ;
#29638=CARTESIAN_POINT ( 'NONE',  ( 96.74139913992713957, -35.13602278645100796, 266.2041967044820581 ) ) ;
#29639=B_SPLINE_CURVE_WITH_KNOTS ( 'NONE', 3,
 ( #53152, #12308, #60896, #24596, #32284, #31394, #38221, #45901, #88181, #4146, #40001, #59091, #74081, #59982, #67259, #73632, #38659, #65914 ),
 .UNSPECIFIED., .F., .F.,
 ( 4, 2, 2, 2, 2, 2, 2, 2, 4 ),
 ( 0.5000457028255199665, 0.5625399899723300123, 0.6250342771191399471, 0.6875285642659499930, 0.7500228514127600388, 0.8125171385595699736, 0.8750114257063800194, 0.9375057128531900652, 1.000000000000000000 ),
 .UNSPECIFIED. ) ;
#29642=EDGE_LOOP ( 'NONE', ( #59907, #2497, #16997, #24530 ) ) ;
#29643=FACE_OUTER_BOUND ( 'NONE', #85193, .T. ) ;
#29644=CARTESIAN_POINT ( 'NONE',  ( 172.5664832912729878, -27.57844715994070484, 18.92562527591200094 ) ) ;
#29646=CARTESIAN_POINT ( 'NONE',  ( 116.5734795788845020, -32.34496456428597355, 104.1699109901969535 ) ) ;
#29648=ORIENTED_EDGE ( 'NONE', *, *, #44685, .F. ) ;
#29650=CARTESIAN_POINT ( 'NONE',  ( 105.6320445689042486, -47.05559920284586184, 257.4670538473393435 ) ) ;
#29652=DIRECTION ( 'NONE',  ( 1.000000000000000000, 4.299999999999999979E-14, 1.000000000000000078E-15 ) ) ;
#29653=VECTOR ( 'NONE', #37181, 1000.000000000000000 ) ;
#29657=CARTESIAN_POINT ( 'NONE',  ( 172.5664832912728457, -18.82844715994071194, 201.9256252759118979 ) ) ;
#29659=CARTESIAN_POINT ( 'NONE',  ( 46.03715912545427358, -48.62818131006086020, 300.4678068554150059 ) ) ;
#29662=CYLINDRICAL_SURFACE ( 'NONE', #55667, 2.750000000000002665 ) ;
#29665=CARTESIAN_POINT ( 'NONE',  ( 107.0667039024467329, -19.36444715994092292, 196.2188068554170002 ) ) ;
#29666=DIRECTION ( 'NONE',  ( 1.000000000000000000, 6.508581945447490214E-14, 1.000000000000000078E-15 ) ) ;
#29667=DIRECTION ( 'NONE',  ( 0.000000000000000000, 0.000000000000000000, -1.000000000000000000 ) ) ;
#29668=VERTEX_POINT ( 'NONE', #68915 ) ;
#29670=CARTESIAN_POINT ( 'NONE',  ( 111.7490138926534797, -27.39026733005105640, 279.7070538473396937 ) ) ;
#29671=CARTESIAN_POINT ( 'NONE',  ( 108.3661019610163123, -47.70601195518164417, 158.6822919425779617 ) ) ;
#29672=CARTESIAN_POINT ( 'NONE',  ( 112.3603056216204550, -28.17164194844215430, 285.6356252759109680 ) ) ;
#29674=DIRECTION ( 'NONE',  ( -1.000000000000000000, 0.000000000000000000, 0.000000000000000000 ) ) ;
#29675=CARTESIAN_POINT ( 'NONE',  ( 116.8171253540862722, -34.15292439824600024, 140.0314580866620418 ) ) ;
#29676=EDGE_CURVE ( 'NONE', #11556, #79496, #55216, .T. ) ;
#29677=ORIENTED_EDGE ( 'NONE', *, *, #10608, .T. ) ;
#29678=EDGE_CURVE ( 'NONE', #39780, #5447, #66841, .T. ) ;
#29679=CYLINDRICAL_SURFACE ( 'NONE', #81017, 9.999999999999998224 ) ;
#29680=ORIENTED_EDGE ( 'NONE', *, *, #3979, .F. ) ;
#29681=CARTESIAN_POINT ( 'NONE',  ( 96.76615086495803553, -37.93025403122315709, 82.43086337114895912 ) ) ;
#29682=EDGE_CURVE ( 'NONE', #5757, #24119, #37873, .T. ) ;
#29684=ORIENTED_EDGE ( 'NONE', *, *, #27932, .T. ) ;
#29686=CARTESIAN_POINT ( 'NONE',  ( 117.3910620576582318, -35.19077923515893502, 214.9441967044829767 ) ) ;
#29687=CARTESIAN_POINT ( 'NONE',  ( 182.6664832912729821, 12.92155284005730387, 358.9756252759109998 ) ) ;
#29688=CARTESIAN_POINT ( 'NONE',  ( 110.8542634740689294, -45.98432270134635047, 147.8856073499956096 ) ) ;
#29689=CARTESIAN_POINT ( 'NONE',  ( 97.31582641009998724, -39.30593163064425966, 151.5319995835646694 ) ) ;
#29690=LINE ( 'NONE', #85128, #10782 ) ;
#29693=FACE_BOUND ( 'NONE', #86224, .T. ) ;
#29694=CARTESIAN_POINT ( 'NONE',  ( 98.38046330306050891, -41.69534231700428251, 96.73979469042932067 ) ) ;
#29695=CARTESIAN_POINT ( 'NONE',  ( 116.5944731948638804, -42.45914096480947819, 128.3956252759109873 ) ) ;
#29698=EDGE_CURVE ( 'NONE', #36849, #53830, #49797, .T. ) ;
#29700=CARTESIAN_POINT ( 'NONE',  ( 107.2828545668587878, -27.33638008851531609, 71.47777378208797927 ) ) ;
#29702=CARTESIAN_POINT ( 'NONE',  ( 83.56670390244799762, -36.72944715994108122, 229.5838068554169524 ) ) ;
#29703=CARTESIAN_POINT ( 'NONE',  ( 115.3120223323505940, -44.18753462406601074, 229.2413395616249545 ) ) ;
#29704=CARTESIAN_POINT ( 'NONE',  ( 108.3334481699632192, -46.73485934377682582, 37.67729194854296537 ) ) ;
#29706=CARTESIAN_POINT ( 'NONE',  ( 104.4905885192464865, -26.97863551867121146, 55.28004222319953698 ) ) ;
#29708=CARTESIAN_POINT ( 'NONE',  ( 134.0664832912740110, -46.72944715994100306, 4.925625275910997303 ) ) ;
#29709=CARTESIAN_POINT ( 'NONE',  ( 168.0371591254545365, -48.62818131005519007, 193.9678068554149775 ) ) ;
#29710=LINE ( 'NONE', #22910, #69566 ) ;
#29713=CARTESIAN_POINT ( 'NONE',  ( 108.6454077996538530, -25.81962716842089378, 149.9737205140059473 ) ) ;
#29714=VERTEX_POINT ( 'NONE', #83007 ) ;
#29716=ADVANCED_FACE ( 'NONE', ( #20762 ), #763, .F. ) ;
#29718=FACE_BOUND ( 'NONE', #42206, .T. ) ;
#29720=CARTESIAN_POINT ( 'NONE',  ( 104.4885766460745486, -26.97918181991462916, 130.2815734883101868 ) ) ;
#29721=CARTESIAN_POINT ( 'NONE',  ( 105.7149892088140319, -46.72379639561137310, 103.4689199191626869 ) ) ;
#29722=CARTESIAN_POINT ( 'NONE',  ( 109.9085748933103162, -45.56225229135190347, 205.6423760838769681 ) ) ;
#29724=CIRCLE ( 'NONE', #9421, 12.99999999999999822 ) ;
#29725=VECTOR ( 'NONE', #60834, 999.9999999999998863 ) ;
#29727=AXIS2_PLACEMENT_3D ( 'NONE', #25666, #12949, #53342 ) ;
#29728=AXIS2_PLACEMENT_3D ( 'NONE', #52258, #12762, #26378 ) ;
#29729=CARTESIAN_POINT ( 'NONE',  ( 117.5811103608870383, -33.32038496654947579, 134.0880062282919880 ) ) ;
#29733=VERTEX_POINT ( 'NONE', #9825 ) ;
#29735=EDGE_CURVE ( 'NONE', #59978, #27885, #45107, .T. ) ;
#29740=LINE ( 'NONE', #57879, #69588 ) ;
#29742=CARTESIAN_POINT ( 'NONE',  ( 131.5325842222575261, -35.66080143920349599, 7.039723185229046720 ) ) ;
#29744=CARTESIAN_POINT ( 'NONE',  ( 102.0014872285204035, -30.29305903553749602, 13.42523322673394581 ) ) ;
#29745=FACE_BOUND ( 'NONE', #66684, .T. ) ;
#29746=ORIENTED_EDGE ( 'NONE', *, *, #56713, .T. ) ;
#29747=EDGE_CURVE ( 'NONE', #35180, #58643, #24992, .T. ) ;
#29748=CARTESIAN_POINT ( 'NONE',  ( 113.0350491764517216, -43.12594021296303737, 9.635625275910943088 ) ) ;
#29750=ORIENTED_EDGE ( 'NONE', *, *, #84160, .T. ) ;
#29752=CARTESIAN_POINT ( 'NONE',  ( 110.8557683604797290, -45.98370673585618817, 112.8857367299098229 ) ) ;
#29753=ORIENTED_EDGE ( 'NONE', *, *, #26915, .T. ) ;
#29754=ORIENTED_EDGE ( 'NONE', *, *, #31874, .F. ) ;
#29756=CARTESIAN_POINT ( 'NONE',  ( 101.6136182267745056, -30.15507309768812050, 40.04956268521897300 ) ) ;
#29757=CARTESIAN_POINT ( 'NONE',  ( 103.8004457107024194, -26.80577029241926112, 165.3299109901969643 ) ) ;
#29758=CARTESIAN_POINT ( 'NONE',  ( 108.2741602056595411, -26.36093993100598354, 129.9841967044819739 ) ) ;
#29759=DIRECTION ( 'NONE',  ( -1.000000000000000000, -4.299999999999999979E-14, -1.000000000000000078E-15 ) ) ;
#29760=CARTESIAN_POINT ( 'NONE',  ( 96.68218458626328982, -35.80812861978466799, 227.2556252759109725 ) ) ;
#29761=CARTESIAN_POINT ( 'NONE',  ( 113.1784580317933120, -44.75174589757562416, 99.09546334846962168 ) ) ;
#29762=CARTESIAN_POINT ( 'NONE',  ( 100.9537377020563582, -28.70775746239330317, 126.5940524488469379 ) ) ;
#29765=ORIENTED_EDGE ( 'NONE', *, *, #11536, .F. ) ;
#29767=VECTOR ( 'NONE', #56548, 1000.000000000000000 ) ;
#29768=CARTESIAN_POINT ( 'NONE',  ( 102.6649408499558689, -27.23033719207987602, 180.4213395616249898 ) ) ;
#29770=CARTESIAN_POINT ( 'NONE',  ( 103.0496837167155491, -26.43166057102584077, 170.3603871806729444 ) ) ;
#29771=DIRECTION ( 'NONE',  ( 1.000000000000000000, 4.299999999999999979E-14, 1.000000000000000078E-15 ) ) ;
#29773=CARTESIAN_POINT ( 'NONE',  ( 136.1807380203761682, -34.97076862298531097, 7.459445689450600270 ) ) ;
#29774=PLANE ( 'NONE',  #49999 ) ;
#29775=DIRECTION ( 'NONE',  ( 0.000000000000000000, 0.000000000000000000, 1.000000000000000000 ) ) ;
#29776=CARTESIAN_POINT ( 'NONE',  ( 97.90460831411941456, -40.73749365022396063, 56.65424410226409435 ) ) ;
#29777=CARTESIAN_POINT ( 'NONE',  ( 112.4005920293389948, -46.38403708128146974, 248.9661014663869878 ) ) ;
#29778=DIRECTION ( 'NONE',  ( -1.000000000000000000, -2.999999999999999839E-15, -1.000000000000000078E-15 ) ) ;
#29781=DIRECTION ( 'NONE',  ( -1.000000000000000000, 0.000000000000000000, 0.000000000000000000 ) ) ;
#29783=FACE_OUTER_BOUND ( 'NONE', #3258, .T. ) ;
#29784=CARTESIAN_POINT ( 'NONE',  ( 99.99848706593783731, -40.87057048248247071, 195.5838068554172651 ) ) ;
#29785=ORIENTED_EDGE ( 'NONE', *, *, #45748, .T. ) ;
#29786=DIRECTION ( 'NONE',  ( 0.000000000000000000, 0.000000000000000000, -1.000000000000000000 ) ) ;
#29787=CARTESIAN_POINT ( 'NONE',  ( 99.40582560697848180, -27.65448416857716651, 150.6356252759109680 ) ) ;
#29788=CARTESIAN_POINT ( 'NONE',  ( 97.62238793418175931, -32.23162594710754547, 71.97276813305397525 ) ) ;
#29789=CARTESIAN_POINT ( 'NONE',  ( 109.6164515631795524, -26.53946793531281756, 195.8813395616249977 ) ) ;
#29790=DIRECTION ( 'NONE',  ( -0.7071067812158990940, -0.7071067811571960515, 0.000000000000000000 ) ) ;
#29791=LINE ( 'NONE', #77950, #2545 ) ;
#29794=DIRECTION ( 'NONE',  ( 0.000000000000000000, 0.000000000000000000, 1.000000000000000000 ) ) ;
#29796=ORIENTED_EDGE ( 'NONE', *, *, #30022, .T. ) ;
#29798=VECTOR ( 'NONE', #44305, 1000.000000000000000 ) ;
#29799=AXIS2_PLACEMENT_3D ( 'NONE', #75500, #55013, #68238 ) ;
#29800=CIRCLE ( 'NONE', #76201, 2.517500000000000071 ) ;
#29801=VECTOR ( 'NONE', #63593, 1000.000000000000000 ) ;
#29805=EDGE_LOOP ( 'NONE', ( #84764, #42024, #17612, #34619 ) ) ;
#29807=EDGE_CURVE ( 'NONE', #87649, #56977, #65664, .T. ) ;
#29808=DIRECTION ( 'NONE',  ( -2.999999999999999839E-15, 1.000000000000000000, -2.999999999999999900E-30 ) ) ;
#29809=VERTEX_POINT ( 'NONE', #64346 ) ;
#29810=CARTESIAN_POINT ( 'NONE',  ( 107.9437834512411314, -25.73425880284256095, 111.0251490854349754 ) ) ;
#29811=DIRECTION ( 'NONE',  ( -2.999999999999999839E-15, 1.000000000000000000, -2.999999999999999900E-30 ) ) ;
#29812=AXIS2_PLACEMENT_3D ( 'NONE', #42463, #23845, #79708 ) ;
#29815=DIRECTION ( 'NONE',  ( 0.000000000000000000, -1.000000000000000000, 0.000000000000000000 ) ) ;
#29816=CARTESIAN_POINT ( 'NONE',  ( 97.69287098190314111, -33.93680905855605801, 31.09562527591097592 ) ) ;
#29817=ORIENTED_EDGE ( 'NONE', *, *, #15423, .T. ) ;
#29819=ORIENTED_EDGE ( 'NONE', *, *, #85526, .T. ) ;
#29822=DIRECTION ( 'NONE',  ( 0.7071067811578790607, 0.7071067812152160847, 0.000000000000000000 ) ) ;
#29823=CARTESIAN_POINT ( 'NONE',  ( 107.0664832912739968, -36.72944715994100306, 287.6356252759109680 ) ) ;
#29824=CARTESIAN_POINT ( 'NONE',  ( 97.81169962758427516, -40.51743340529665005, 76.63548575323150658 ) ) ;
#29825=AXIS2_PLACEMENT_3D ( 'NONE', #22402, #14242, #63279 ) ;
#29828=CARTESIAN_POINT ( 'NONE',  ( 105.8001462888458519, -26.72394952473684882, 51.17876692797100446 ) ) ;
#29829=DIRECTION ( 'NONE',  ( -1.000000000000000078E-15, 1.000000000000000083E-30, 1.000000000000000000 ) ) ;
#29831=CARTESIAN_POINT ( 'NONE',  ( 104.6539710028518897, -47.49251396406771164, 27.38895860924395009 ) ) ;
#29833=VERTEX_POINT ( 'NONE', #4345 ) ;
#29834=CARTESIAN_POINT ( 'NONE',  ( 107.0664832912739541, -22.72944715994095688, 315.1356252759112522 ) ) ;
#29836=CARTESIAN_POINT ( 'NONE',  ( 108.6369934722860506, -45.24028864696019525, 125.5518998934009574 ) ) ;
#29839=CIRCLE ( 'NONE', #83452, 7.500000000000007105 ) ;
#29840=CARTESIAN_POINT ( 'NONE',  ( 97.75849014177104834, -40.38515380072060168, 96.62427964741705466 ) ) ;
#29841=CARTESIAN_POINT ( 'NONE',  ( 48.16670390244701139, -26.71338133339251542, 342.9256252759119548 ) ) ;
#29842=ORIENTED_EDGE ( 'NONE', *, *, #10196, .F. ) ;
#29843=EDGE_LOOP ( 'NONE', ( #39143, #30620, #86115, #1402 ) ) ;
#29848=CARTESIAN_POINT ( 'NONE',  ( 115.9244277637092040, -39.86207309682762912, 174.9996785439919904 ) ) ;
#29850=EDGE_CURVE ( 'NONE', #1345, #87676, #53843, .T. ) ;
#29851=CARTESIAN_POINT ( 'NONE',  ( 95.46382812221506242, -34.19949780945433560, 102.1556252759109640 ) ) ;
#29852=CARTESIAN_POINT ( 'NONE',  ( 113.2363792478179789, -44.61460182729985036, 18.10486178924557521 ) ) ;
#29854=EDGE_LOOP ( 'NONE', ( #35908, #7582, #60853, #17200 ) ) ;
#29855=VECTOR ( 'NONE', #39064, 1000.000000000000000 ) ;
#29856=VECTOR ( 'NONE', #81885, 1000.000000000000000 ) ;
#29858=VERTEX_POINT ( 'NONE', #11143 ) ;
#29859=VERTEX_POINT ( 'NONE', #59730 ) ;
#29860=CARTESIAN_POINT ( 'NONE',  ( 103.0873890296785333, -43.88832256772609952, 184.9909475124489688 ) ) ;
#29861=CARTESIAN_POINT ( 'NONE',  ( 110.3789737648050107, -47.29935009229100729, 52.80610146638697699 ) ) ;
#29862=EDGE_LOOP ( 'NONE', ( #1755, #71593 ) ) ;
#29863=CARTESIAN_POINT ( 'NONE',  ( 109.6066175024219973, -25.17973177368032012, 29.90419670448196854 ) ) ;
#29864=CARTESIAN_POINT ( 'NONE',  ( 114.9815172128508465, -29.91112648151817410, 180.3927681330539770 ) ) ;
#29867=CARTESIAN_POINT ( 'NONE',  ( 113.0769238478409449, -28.21140209294909695, 125.5870538473399591 ) ) ;
#29870=VECTOR ( 'NONE', #17404, 1000.000000000000000 ) ;
#29872=EDGE_CURVE ( 'NONE', #77063, #34249, #52882, .T. ) ;
#29875=ORIENTED_EDGE ( 'NONE', *, *, #51693, .F. ) ;
#29876=AXIS2_PLACEMENT_3D ( 'NONE', #50452, #78199, #51336 ) ;
#29881=CARTESIAN_POINT ( 'NONE',  ( 98.64717563880898865, -43.89145428829765194, 76.89943479971999807 ) ) ;
#29882=CARTESIAN_POINT ( 'NONE',  ( 48.86082318535700608, -35.55794170701751256, -5.074374724088000832 ) ) ;
#29883=VECTOR ( 'NONE', #70916, 1000.000000000000000 ) ;
#29884=PLANE ( 'NONE',  #59407 ) ;
#29885=DIRECTION ( 'NONE',  ( 0.000000000000000000, -1.000000000000000000, 0.000000000000000000 ) ) ;
#29886=CARTESIAN_POINT ( 'NONE',  ( 116.4365193811697310, -32.28633913640743458, 64.19086337114998742 ) ) ;
#29887=LINE ( 'NONE', #63495, #53595 ) ;
#29888=CARTESIAN_POINT ( 'NONE',  ( 118.8928063919343145, -36.92768728534039013, 149.8127681330539644 ) ) ;
#29891=VERTEX_POINT ( 'NONE', #32474 ) ;
#29896=CARTESIAN_POINT ( 'NONE',  ( 111.4357194830650002, -47.79916136671457849, 172.8756252759109771 ) ) ;
#29897=EDGE_LOOP ( 'NONE', ( #3106, #25952, #19715, #31012 ) ) ;
#29898=LINE ( 'NONE', #77596, #26258 ) ;
#29899=CARTESIAN_POINT ( 'NONE',  ( 108.0160737019250377, -24.89219542061752577, 261.0127681330534415 ) ) ;
#29900=CARTESIAN_POINT ( 'NONE',  ( 95.98963492482539550, -41.07853246264400582, 92.62419670448296927 ) ) ;
#29901=CARTESIAN_POINT ( 'NONE',  ( 128.5492039024480562, -51.22944715994093912, 207.5838068554170377 ) ) ;
#29902=CARTESIAN_POINT ( 'NONE',  ( 97.07201034874346135, -35.37904553719489797, 192.2188556906257304 ) ) ;
#29903=DIRECTION ( 'NONE',  ( 6.524622321627019585E-16, 3.741823817616790462E-31, 1.000000000000000000 ) ) ;
#29905=ADVANCED_FACE ( 'NONE', ( #11610 ), #60174, .T. ) ;
#29906=VERTEX_POINT ( 'NONE', #26567 ) ;
#29908=ORIENTED_EDGE ( 'NONE', *, *, #64493, .T. ) ;
#29911=DIRECTION ( 'NONE',  ( 4.299999999999999979E-14, -1.000000000000000000, 4.400000000000000367E-29 ) ) ;
#29912=CARTESIAN_POINT ( 'NONE',  ( 95.29510253380274776, -38.09663793710245017, 232.4184824187679794 ) ) ;
#29913=DIRECTION ( 'NONE',  ( -4.237773401492740281E-14, 1.000000000000000000, 0.000000000000000000 ) ) ;
#29914=CARTESIAN_POINT ( 'NONE',  ( 132.8230071953894083, -34.27587548316717658, 1.868342134762299045 ) ) ;
#29915=EDGE_CURVE ( 'NONE', #89702, #80585, #79973, .T. ) ;
#29916=DIRECTION ( 'NONE',  ( -6.831565154159360295E-14, 1.000000000000000000, 0.000000000000000000 ) ) ;
#29918=AXIS2_PLACEMENT_3D ( 'NONE', #66919, #65580, #32381 ) ;
#29920=CARTESIAN_POINT ( 'NONE',  ( 99.96564438395634511, -44.39263518965486099, 46.98133956162592284 ) ) ;
#29921=ORIENTED_EDGE ( 'NONE', *, *, #15796, .T. ) ;
#29922=ORIENTED_EDGE ( 'NONE', *, *, #4195, .T. ) ;
#29925=EDGE_CURVE ( 'NONE', #30966, #29159, #43689, .T. ) ;
#29926=VECTOR ( 'NONE', #3728, 1000.000000000000000 ) ;
#29930=FACE_OUTER_BOUND ( 'NONE', #76889, .T. ) ;
#29931=CARTESIAN_POINT ( 'NONE',  ( 110.6561457788924230, -27.59554888373227755, 265.7784824187677941 ) ) ;
#29934=CARTESIAN_POINT ( 'NONE',  ( 116.0091996907507195, -30.12340400999218559, 105.3327681330529515 ) ) ;
#29935=CARTESIAN_POINT ( 'NONE',  ( 107.0664832912739968, -36.72944715994100306, 287.6356252759109680 ) ) ;
#29937=FACE_OUTER_BOUND ( 'NONE', #66337, .T. ) ;
#29939=VERTEX_POINT ( 'NONE', #34272 ) ;
#29940=CIRCLE ( 'NONE', #67593, 11.57110091390439699 ) ;
#29942=CARTESIAN_POINT ( 'NONE',  ( 99.56565989216673529, -33.50937434423423156, 13.82237608387698558 ) ) ;
#29943=FACE_OUTER_BOUND ( 'NONE', #72908, .T. ) ;
#29944=AXIS2_PLACEMENT_3D ( 'NONE', #40832, #22552, #8013 ) ;
#29946=CARTESIAN_POINT ( 'NONE',  ( 116.8171726708769285, -34.15311105152028404, 195.0314804765609722 ) ) ;
#29947=ORIENTED_EDGE ( 'NONE', *, *, #52171, .T. ) ;
#29949=FACE_OUTER_BOUND ( 'NONE', #63664, .T. ) ;
#29950=ORIENTED_EDGE ( 'NONE', *, *, #84604, .T. ) ;
#29951=CARTESIAN_POINT ( 'NONE',  ( 102.9709959788349636, -46.31662683568885086, 92.25562527591097250 ) ) ;
#29952=ORIENTED_EDGE ( 'NONE', *, *, #52908, .T. ) ;
#29953=CARTESIAN_POINT ( 'NONE',  ( 109.9248237270229680, -44.80917438794489271, 37.26956268521996662 ) ) ;
#29954=CARTESIAN_POINT ( 'NONE',  ( 115.0390926746001981, -42.79681148600482032, 89.30794038968477366 ) ) ;
#29955=CARTESIAN_POINT ( 'NONE',  ( 112.4269750522866502, -44.91043508143939533, 178.0384824187689503 ) ) ;
#29959=CARTESIAN_POINT ( 'NONE',  ( 115.6911734784272170, -30.73338764459478867, 275.3099109901965562 ) ) ;
#29960=ORIENTED_EDGE ( 'NONE', *, *, #14103, .T. ) ;
#29961=CARTESIAN_POINT ( 'NONE',  ( 48.85858412958099706, -30.08671355700241179, -5.074374724088000832 ) ) ;
#29962=VERTEX_POINT ( 'NONE', #89711 ) ;
#29963=CARTESIAN_POINT ( 'NONE',  ( 100.8606736390591720, -45.92946726319084405, 148.0918157521009562 ) ) ;
#29967=EDGE_LOOP ( 'NONE', ( #15581, #39132, #62171, #83310 ) ) ;
#29969=LINE ( 'NONE', #72197, #39102 ) ;
#29970=CARTESIAN_POINT ( 'NONE',  ( 114.3351522754913674, -30.13549343754558407, 209.4127681330539872 ) ) ;
#29973=DIRECTION ( 'NONE',  ( 0.000000000000000000, 0.000000000000000000, -1.000000000000000000 ) ) ;
#29974=CARTESIAN_POINT ( 'NONE',  ( 111.3231501057927346, -27.21297328954094041, 20.74133956162494030 ) ) ;
#29975=LINE ( 'NONE', #76777, #68232 ) ;
#29976=ORIENTED_EDGE ( 'NONE', *, *, #32785, .F. ) ;
#29977=CARTESIAN_POINT ( 'NONE',  ( 103.2784589858348596, -27.47467144708731368, 171.3856301094683374 ) ) ;
#29979=DIRECTION ( 'NONE',  ( 0.000000000000000000, 0.000000000000000000, 1.000000000000000000 ) ) ;
#29980=EDGE_LOOP ( 'NONE', ( #54068, #54386, #20590, #14941 ) ) ;
#29983=EDGE_CURVE ( 'NONE', #40161, #34521, #13394, .T. ) ;
#29984=VECTOR ( 'NONE', #30545, 1000.000000000000000 ) ;
#29985=CARTESIAN_POINT ( 'NONE',  ( 168.0371591254546217, -48.62818131005519007, 129.9678068554150059 ) ) ;
#29988=CARTESIAN_POINT ( 'NONE',  ( 110.4916936757735471, -26.90617889774101812, 209.8099109901969541 ) ) ;
#29990=CIRCLE ( 'NONE', #80756, 2.500000000000002220 ) ;
#29991=CARTESIAN_POINT ( 'NONE',  ( 75.31670390244798341, -57.40094715994099772, 35.51780685541480409 ) ) ;
#29992=DIRECTION ( 'NONE',  ( -4.237773401492740281E-14, 1.000000000000000000, 0.000000000000000000 ) ) ;
#29993=CARTESIAN_POINT ( 'NONE',  ( 115.0883484252707376, -39.66301350383546520, 217.9695626852199837 ) ) ;
#29994=DIRECTION ( 'NONE',  ( 5.512527431108029424E-15, -1.000000000000000000, 0.000000000000000000 ) ) ;
#29995=CARTESIAN_POINT ( 'NONE',  ( 100.4929927897290582, -27.87207479535962662, 31.59657765686396758 ) ) ;
#29997=CARTESIAN_POINT ( 'NONE',  ( 100.2700262342886219, -46.49863182355969116, 87.09276813305393716 ) ) ;
#29998=ORIENTED_EDGE ( 'NONE', *, *, #22105, .F. ) ;
#29999=CARTESIAN_POINT ( 'NONE',  ( 131.4052890608957682, -19.42303004212037010, 6.877070700250059510 ) ) ;
#30002=CARTESIAN_POINT ( 'NONE',  ( 103.2798918628733134, -27.47408509851724290, 276.3855069386696073 ) ) ;
#30004=LINE ( 'NONE', #1405, #24425 ) ;
#30005=VERTEX_POINT ( 'NONE', #7473 ) ;
#30006=CARTESIAN_POINT ( 'NONE',  ( 63.03715912545639100, -24.42818131006026761, 180.4678068554151196 ) ) ;
#30009=EDGE_LOOP ( 'NONE', ( #44242, #18210, #74258, #12917 ) ) ;
#30011=CARTESIAN_POINT ( 'NONE',  ( 103.3545649297684577, -47.16578287771347533, 102.3165776568629752 ) ) ;
#30013=DIRECTION ( 'NONE',  ( -0.7071067811571960515, 0.7071067812158990940, 0.000000000000000000 ) ) ;
#30014=DIRECTION ( 'NONE',  ( -0.000000000000000000, -0.000000000000000000, 1.000000000000000000 ) ) ;
#30015=ORIENTED_EDGE ( 'NONE', *, *, #73789, .F. ) ;
#30018=LINE ( 'NONE', #70914, #34429 ) ;
#30021=CARTESIAN_POINT ( 'NONE',  ( 41.56648329127398966, -18.82844715994071194, 18.92562527591200094 ) ) ;
#30022=EDGE_CURVE ( 'NONE', #26639, #8253, #39350, .T. ) ;
#30023=FACE_OUTER_BOUND ( 'NONE', #62339, .T. ) ;
#30024=CARTESIAN_POINT ( 'NONE',  ( 107.0664832912739968, -36.72944715994100306, 287.6356252759109680 ) ) ;
#30027=PLANE ( 'NONE',  #36066 ) ;
#30028=CARTESIAN_POINT ( 'NONE',  ( 118.1473594538625349, -37.63838399483782382, 184.7613395616249647 ) ) ;
#30030=DIRECTION ( 'NONE',  ( 0.000000000000000000, 1.000000000000000000, 0.000000000000000000 ) ) ;
#30031=EDGE_LOOP ( 'NONE', ( #25612, #58624, #32394, #78148 ) ) ;
#30032=CARTESIAN_POINT ( 'NONE',  ( 97.72045521349410535, -39.61305637792672485, 17.56419670448195092 ) ) ;
#30034=CARTESIAN_POINT ( 'NONE',  ( 110.8549148032106615, -45.98405610977419400, 52.88566334576604788 ) ) ;
#30035=CARTESIAN_POINT ( 'NONE',  ( 104.4067564067896399, -46.45769496072055915, 12.36492216824909463 ) ) ;
#30039=CARTESIAN_POINT ( 'NONE',  ( 117.4008144674645280, -32.62901037329574905, 249.1270538473399654 ) ) ;
#30041=ORIENTED_EDGE ( 'NONE', *, *, #19874, .F. ) ;
#30042=CARTESIAN_POINT ( 'NONE',  ( 109.0147404159584568, -27.53810233378435157, 181.3539642582779550 ) ) ;
#30045=VECTOR ( 'NONE', #27253, 1000.000000000000000 ) ;
#30046=CARTESIAN_POINT ( 'NONE',  ( 97.81060075337646254, -38.34349919808700236, 42.88348806780201272 ) ) ;
#30047=AXIS2_PLACEMENT_3D ( 'NONE', #69380, #6697, #56628 ) ;
#30049=CARTESIAN_POINT ( 'NONE',  ( 84.06648329127399677, -18.82844715994099971, 17.92562527591199739 ) ) ;
#30051=ORIENTED_EDGE ( 'NONE', *, *, #38318, .F. ) ;
#30052=CARTESIAN_POINT ( 'NONE',  ( 167.2371591254543262, -47.82818131005522844, 249.9678068554149775 ) ) ;
#30053=DIRECTION ( 'NONE',  ( 0.000000000000000000, 1.000000000000000000, 0.000000000000000000 ) ) ;
#30054=CARTESIAN_POINT ( 'NONE',  ( 112.6519946835718855, -45.50616226388166297, 263.0270538473394595 ) ) ;
#30056=EDGE_LOOP ( 'NONE', ( #72946, #11934 ) ) ;
#30057=ORIENTED_EDGE ( 'NONE', *, *, #17243, .F. ) ;
#30058=FACE_OUTER_BOUND ( 'NONE', #23657, .T. ) ;
#30060=DIRECTION ( 'NONE',  ( 0.000000000000000000, 0.000000000000000000, 1.000000000000000000 ) ) ;
#30062=CARTESIAN_POINT ( 'NONE',  ( 123.0664832912757163, -36.72944715993921960, -4.074374724089013355 ) ) ;
#30063=VECTOR ( 'NONE', #3172, 1000.000000000000000 ) ;
#30064=ADVANCED_FACE ( 'NONE', ( #27022 ), #62427, .F. ) ;
#30065=CARTESIAN_POINT ( 'NONE',  ( 117.3951115944450123, -37.65585020919950665, 29.74324432352998215 ) ) ;
#30068=CARTESIAN_POINT ( 'NONE',  ( 112.7653987728015323, -27.20474975302890996, 50.65943479972101215 ) ) ;
#30070=EDGE_CURVE ( 'NONE', #82153, #76973, #30669, .T. ) ;
#30071=CARTESIAN_POINT ( 'NONE',  ( 100.1774089044720881, -45.37350532423673144, 272.0289586092443415 ) ) ;
#30072=EDGE_LOOP ( 'NONE', ( #89429, #37900, #80135, #2989 ) ) ;
#30073=CARTESIAN_POINT ( 'NONE',  ( 82.59704509974100972, -17.65293374834238094, 2.807537076564926348 ) ) ;
#30075=DIRECTION ( 'NONE',  ( -0.7071067811868619879, -0.7071067811862330466, -7.071067811868925614E-16 ) ) ;
#30076=CARTESIAN_POINT ( 'NONE',  ( 111.9804352529405804, -29.60526291441071578, 87.42618560768700320 ) ) ;
#30077=CARTESIAN_POINT ( 'NONE',  ( 96.83718905160354495, -34.60841009949970726, 212.1641967044819808 ) ) ;
#30081=ORIENTED_EDGE ( 'NONE', *, *, #74802, .F. ) ;
#30082=AXIS2_PLACEMENT_3D ( 'NONE', #43848, #51108, #22099 ) ;
#30083=ORIENTED_EDGE ( 'NONE', *, *, #75777, .F. ) ;
#30084=EDGE_CURVE ( 'NONE', #10149, #50389, #75614, .T. ) ;
#30087=ORIENTED_EDGE ( 'NONE', *, *, #32838, .F. ) ;
#30088=CARTESIAN_POINT ( 'NONE',  ( 116.3153332067577850, -32.94059133099460723, 170.1356252759109680 ) ) ;
#30089=CARTESIAN_POINT ( 'NONE',  ( 97.06382365635857923, -37.34195890833274234, 42.37516235093055883 ) ) ;
#30090=CARTESIAN_POINT ( 'NONE',  ( 115.5032561769494066, -38.06248691838574416, 113.1238483995059596 ) ) ;
#30091=CARTESIAN_POINT ( 'NONE',  ( 104.8365363718904888, -26.48661066032647327, 260.2470538473397710 ) ) ;
#30095=VERTEX_POINT ( 'NONE', #62871 ) ;
#30096=CARTESIAN_POINT ( 'NONE',  ( 41.56648329127399677, -18.82844715994099971, 78.92562527591199739 ) ) ;
#30098=CARTESIAN_POINT ( 'NONE',  ( 104.4073484937606935, -46.45786862655047145, 32.36494955462968903 ) ) ;
#30099=CARTESIAN_POINT ( 'NONE',  ( 46.48091746482051434, -49.32844715994088602, 129.9678068554150911 ) ) ;
#30100=AXIS2_PLACEMENT_3D ( 'NONE', #77271, #7777, #77725 ) ;
#30101=CARTESIAN_POINT ( 'NONE',  ( 41.56648329127398966, -27.82844715994070484, 15.92562527591200094 ) ) ;
#30102=ORIENTED_EDGE ( 'NONE', *, *, #88734, .F. ) ;
#30104=CARTESIAN_POINT ( 'NONE',  ( 97.55979742750555772, -43.80499729575070234, 261.8356252759109566 ) ) ;
#30105=CARTESIAN_POINT ( 'NONE',  ( 114.8518103909616315, -43.72813715869710904, 34.24419670448197905 ) ) ;
#30107=CARTESIAN_POINT ( 'NONE',  ( 104.4081006533185274, -46.45808913802587625, 118.3647919419379662 ) ) ;
#30108=LINE ( 'NONE', #78727, #5655 ) ;
#30109=CARTESIAN_POINT ( 'NONE',  ( 181.5667039024459939, -18.82844715994099971, 342.9256252759109884 ) ) ;
#30110=DIRECTION ( 'NONE',  ( 4.194175870806139918E-14, -1.000000000000000000, 0.000000000000000000 ) ) ;
#30111=DIRECTION ( 'NONE',  ( 0.000000000000000000, 0.000000000000000000, -1.000000000000000000 ) ) ;
#30113=CARTESIAN_POINT ( 'NONE',  ( 168.5667039024485803, -48.82844715993516616, 180.4678068554150059 ) ) ;
#30114=ADVANCED_FACE ( 'NONE', ( #20215 ), #7916, .F. ) ;
#30115=CARTESIAN_POINT ( 'NONE',  ( 98.30754688952644926, -41.72890701560834970, 161.7395981821620978 ) ) ;
#30116=CIRCLE ( 'NONE', #80902, 0.5000000000000004441 ) ;
#30117=DIRECTION ( 'NONE',  ( -0.9254794337955620787, -0.3787978585227822492, 0.000000000000000000 ) ) ;
#30118=CARTESIAN_POINT ( 'NONE',  ( 81.80795390244803400, -42.97311385574014508, 207.5838068554169809 ) ) ;
#30119=CARTESIAN_POINT ( 'NONE',  ( 118.3649377238561300, -33.07154184081399961, 284.0756252759109657 ) ) ;
#30120=CARTESIAN_POINT ( 'NONE',  ( 98.16828830165673025, -31.29763223543249850, 166.8899109901969950 ) ) ;
#30121=CARTESIAN_POINT ( 'NONE',  ( 97.46669833601751520, -32.60829619471579122, 12.00419670448293985 ) ) ;
#30125=CARTESIAN_POINT ( 'NONE',  ( 115.0372575073645578, -42.90846256548200444, 48.30229194269750792 ) ) ;
#30126=CARTESIAN_POINT ( 'NONE',  ( 82.45999417309988644, -35.37149686611228816, 2.653088969726210777 ) ) ;
#30127=AXIS2_PLACEMENT_3D ( 'NONE', #42292, #7349, #63203 ) ;
#30128=ORIENTED_EDGE ( 'NONE', *, *, #12101, .T. ) ;
#30129=FACE_OUTER_BOUND ( 'NONE', #18519, .T. ) ;
#30130=ORIENTED_EDGE ( 'NONE', *, *, #51238, .F. ) ;
#30131=CARTESIAN_POINT ( 'NONE',  ( 112.3909220325769382, -27.83061929752864572, 50.65943479972001739 ) ) ;
#30133=DIRECTION ( 'NONE',  ( 0.9068632946707805287, -0.4214249218767882610, 9.061988307341536250E-16 ) ) ;
#30134=EDGE_LOOP ( 'NONE', ( #56142, #68771, #35181, #50845, #60922, #4651, #48775, #15969 ) ) ;
#30135=DIRECTION ( 'NONE',  ( 1.000000000000000000, 4.194175870806139918E-14, 0.000000000000000000 ) ) ;
#30136=CARTESIAN_POINT ( 'NONE',  ( 101.9951592035502586, -45.85337710724431304, 183.1727681330539781 ) ) ;
#30137=PLANE ( 'NONE',  #36673 ) ;
#30138=CARTESIAN_POINT ( 'NONE',  ( 97.81362463995230883, -40.52215243649990128, 146.6360314391660893 ) ) ;
#30143=CARTESIAN_POINT ( 'NONE',  ( 110.8532826261943569, -45.98472416447314259, 97.88552295559415484 ) ) ;
#30144=CARTESIAN_POINT ( 'NONE',  ( 108.8662857618680562, -46.94215964495590043, 122.7032443235309671 ) ) ;
#30145=VERTEX_POINT ( 'NONE', #15186 ) ;
#30148=CARTESIAN_POINT ( 'NONE',  ( 106.2249424221556922, -46.76750045321607985, 108.9415833058969554 ) ) ;
#30149=CARTESIAN_POINT ( 'NONE',  ( 76.06670390244796920, -26.72944715994109899, 239.5838068554169809 ) ) ;
#30150=CARTESIAN_POINT ( 'NONE',  ( 98.06605190618653012, -40.64173669134672906, 227.6527681330529731 ) ) ;
#30151=PLANE ( 'NONE',  #89781 ) ;
#30152=FACE_OUTER_BOUND ( 'NONE', #2247, .T. ) ;
#30153=DIRECTION ( 'NONE',  ( -0.04216478779797398074, 0.9991106698809455455, 0.000000000000000000 ) ) ;
#30154=DIRECTION ( 'NONE',  ( 0.000000000000000000, 0.000000000000000000, -1.000000000000000000 ) ) ;
#30155=CARTESIAN_POINT ( 'NONE',  ( 73.06670390244801183, -48.82844715994099971, 250.9178068554160461 ) ) ;
#30157=CARTESIAN_POINT ( 'NONE',  ( 108.3633857348901586, -47.68307073960303910, 162.6822919425769669 ) ) ;
#30159=VERTEX_POINT ( 'NONE', #6141 ) ;
#30160=ORIENTED_EDGE ( 'NONE', *, *, #38299, .F. ) ;
#30163=VECTOR ( 'NONE', #21384, 1000.000000000000000 ) ;
#30164=LINE ( 'NONE', #51046, #27279 ) ;
#30165=CARTESIAN_POINT ( 'NONE',  ( 98.04124286399094501, -41.04127998252142362, 102.6811413373515762 ) ) ;
#30166=CARTESIAN_POINT ( 'NONE',  ( 114.9947780803761503, -40.19975936245594283, 206.3042808457819604 ) ) ;
#30167=AXIS2_PLACEMENT_3D ( 'NONE', #1760, #57143, #84889 ) ;
#30168=CIRCLE ( 'NONE', #60552, 5.600000000000000533 ) ;
#30170=ADVANCED_FACE ( 'NONE', ( #47885 ), #75627, .F. ) ;
#30171=CARTESIAN_POINT ( 'NONE',  ( 98.55109871784688380, -44.97133477160940629, 191.9384824187679612 ) ) ;
#30173=EDGE_LOOP ( 'NONE', ( #45106, #57723, #70424, #43023, #89412, #2830, #57872, #86262, #44013, #72971, #55765, #8730, #84306, #69304, #11747, #82140 ) ) ;
#30175=ORIENTED_EDGE ( 'NONE', *, *, #24672, .T. ) ;
#30182=CARTESIAN_POINT ( 'NONE',  ( 108.8902037297786762, -46.63625027785658972, 274.1530118773256390 ) ) ;
#30185=ORIENTED_EDGE ( 'NONE', *, *, #63218, .T. ) ;
#30186=CIRCLE ( 'NONE', #80971, 2.116999999999980009 ) ;
#30187=CIRCLE ( 'NONE', #4047, 2.500000000000002220 ) ;
#30188=CARTESIAN_POINT ( 'NONE',  ( 115.8167425921599971, -40.08859881155650129, 9.635625275910941312 ) ) ;
#30191=ORIENTED_EDGE ( 'NONE', *, *, #16223, .F. ) ;
#30192=VECTOR ( 'NONE', #22127, 1000.000000000000000 ) ;
#30194=CARTESIAN_POINT ( 'NONE',  ( 110.8546553593343589, -45.98416230330774823, 112.8856410521173501 ) ) ;
#30195=VERTEX_POINT ( 'NONE', #23363 ) ;
#30198=CARTESIAN_POINT ( 'NONE',  ( 111.2046685188893775, -28.67413054290084062, 19.13337220902994318 ) ) ;
#30200=CARTESIAN_POINT ( 'NONE',  ( 117.8235219141173218, -34.08718286818967158, 164.0061014663869798 ) ) ;
#30201=CARTESIAN_POINT ( 'NONE',  ( 103.4759237351580623, -46.49349013887667326, 142.2956252759109645 ) ) ;
#30202=CARTESIAN_POINT ( 'NONE',  ( 188.5667039024479834, -62.87844715994099687, 137.2178068554150059 ) ) ;
#30203=CARTESIAN_POINT ( 'NONE',  ( 97.01652928432748979, -33.95800134492240119, 247.1127681330539758 ) ) ;
#30205=DIRECTION ( 'NONE',  ( 0.7071067811868677611, 0.7071067811862271624, 7.071067811868671206E-16 ) ) ;
#30208=ORIENTED_EDGE ( 'NONE', *, *, #54049, .F. ) ;
#30209=EDGE_CURVE ( 'NONE', #44005, #6482, #46521, .T. ) ;
#30210=EDGE_LOOP ( 'NONE', ( #7302, #11227, #5005, #86755 ) ) ;
#30211=VECTOR ( 'NONE', #81015, 1000.000000000000000 ) ;
#30212=AXIS2_PLACEMENT_3D ( 'NONE', #33820, #40630, #32020 ) ;
#30214=CARTESIAN_POINT ( 'NONE',  ( 113.7790015168560558, -44.76367177190390834, 193.1299109901969757 ) ) ;
#30216=CARTESIAN_POINT ( 'NONE',  ( 100.8863770005861795, -45.89136241369948976, 152.0918157521009562 ) ) ;
#30217=CARTESIAN_POINT ( 'NONE',  ( 136.8164832912739826, -18.72944715994099951, -5.074374724088999145 ) ) ;
#30220=DIRECTION ( 'NONE',  ( 1.000000000000000078E-15, -1.000000000000000083E-30, -1.000000000000000000 ) ) ;
#30223=CARTESIAN_POINT ( 'NONE',  ( 103.0988156209413518, -47.86972635628415418, 248.3041967044829619 ) ) ;
#30224=CARTESIAN_POINT ( 'NONE',  ( 176.7738106835694225, -48.62134037881071436, 249.9678068554149775 ) ) ;
#30225=DIRECTION ( 'NONE',  ( 0.000000000000000000, -1.000000000000000000, 0.000000000000000000 ) ) ;
#30226=CARTESIAN_POINT ( 'NONE',  ( 108.4139696804897852, -26.73458958342939340, 270.9688129685129638 ) ) ;
#30227=DIRECTION ( 'NONE',  ( -1.346944695195362088E-15, 1.000000000000000000, -3.469446951953620425E-31 ) ) ;
#30228=CARTESIAN_POINT ( 'NONE',  ( 97.07207205457036991, -35.37844123025803356, 257.2189586117278850 ) ) ;
#30229=EDGE_CURVE ( 'NONE', #7741, #30095, #17416, .T. ) ;
#30230=CYLINDRICAL_SURFACE ( 'NONE', #66604, 9.999999999999998224 ) ;
#30231=CARTESIAN_POINT ( 'NONE',  ( 111.7894810538943347, -43.25978944192451792, 195.5838068554170377 ) ) ;
#30233=LINE ( 'NONE', #24310, #64012 ) ;
#30234=CARTESIAN_POINT ( 'NONE',  ( 107.9200767535970584, -47.17740107552570805, 177.6413395616249886 ) ) ;
#30235=CARTESIAN_POINT ( 'NONE',  ( 97.28846512631339749, -33.11380776793520653, 62.04419670448196911 ) ) ;
#30236=CARTESIAN_POINT ( 'NONE',  ( 97.72358123494467463, -41.53030082902068898, 192.7041967044819728 ) ) ;
#30238=CARTESIAN_POINT ( 'NONE',  ( 167.6524903400753601, -49.32844715993521589, 300.4678068554149490 ) ) ;
#30239=DIRECTION ( 'NONE',  ( 0.000000000000000000, 0.000000000000000000, -1.000000000000000000 ) ) ;
#30240=FACE_OUTER_BOUND ( 'NONE', #50476, .T. ) ;
#30242=DIRECTION ( 'NONE',  ( 0.000000000000000000, 1.000000000000000000, 0.000000000000000000 ) ) ;
#30244=CARTESIAN_POINT ( 'NONE',  ( 105.8015779202953013, -26.72375086159097890, 65.17860495093832185 ) ) ;
#30245=CIRCLE ( 'NONE', #44671, 2.116999999999993776 ) ;
#30246=AXIS2_PLACEMENT_3D ( 'NONE', #23647, #59019, #85878 ) ;
#30248=VERTEX_POINT ( 'NONE', #31037 ) ;
#30249=CARTESIAN_POINT ( 'NONE',  ( 99.26324148224303201, -33.25589724784042289, 100.4152769709339736 ) ) ;
#30250=EDGE_CURVE ( 'NONE', #87811, #78226, #1696, .T. ) ;
#30251=VECTOR ( 'NONE', #78781, 1000.000000000000000 ) ;
#30254=CARTESIAN_POINT ( 'NONE',  ( 97.28692064948108964, -31.62807703868918807, 86.93181575210095957 ) ) ;
#30257=ADVANCED_FACE ( 'NONE', ( #30599, #51901 ), #24235, .F. ) ;
#30258=DIRECTION ( 'NONE',  ( -0.9068632946707755327, 0.4214249218767993077, 0.000000000000000000 ) ) ;
#30259=DIRECTION ( 'NONE',  ( 1.000000000000000000, -3.885780586188044357E-13, 0.000000000000000000 ) ) ;
#30260=EDGE_CURVE ( 'NONE', #34521, #51959, #75675, .T. ) ;
#30261=CIRCLE ( 'NONE', #15741, 3.600000000000000089 ) ;
#30262=CARTESIAN_POINT ( 'NONE',  ( 115.1412022171004850, -43.23618977845876543, 43.27467289495995573 ) ) ;
#30264=VERTEX_POINT ( 'NONE', #1564 ) ;
#30266=LINE ( 'NONE', #72492, #21029 ) ;
#30268=CARTESIAN_POINT ( 'NONE',  ( 102.0670549655111330, -27.97049805627439412, 116.4897919420885017 ) ) ;
#30271=CARTESIAN_POINT ( 'NONE',  ( 97.53180040003341844, -39.74881746577888464, 52.57028483553885678 ) ) ;
#30272=VECTOR ( 'NONE', #30318, 1000.000000000000000 ) ;
#30273=DIRECTION ( 'NONE',  ( 1.000000000000000000, 0.000000000000000000, 0.000000000000000000 ) ) ;
#30275=CARTESIAN_POINT ( 'NONE',  ( 100.9539191370901960, -46.85292318231938680, 52.14419670448194921 ) ) ;
#30276=ORIENTED_EDGE ( 'NONE', *, *, #38118, .F. ) ;
#30277=CARTESIAN_POINT ( 'NONE',  ( 112.1393459024198478, -28.01282294203041801, 269.6564585851592142 ) ) ;
#30279=CARTESIAN_POINT ( 'NONE',  ( 100.7929862627584754, -41.95179922106267156, 114.6966617981629639 ) ) ;
#30280=CARTESIAN_POINT ( 'NONE',  ( 107.0664832912739257, -52.42944715994095617, 311.6356252759109680 ) ) ;
#30284=CARTESIAN_POINT ( 'NONE',  ( 97.86670452396658959, -40.64952357659477400, 136.6473464318451647 ) ) ;
#30287=CARTESIAN_POINT ( 'NONE',  ( 108.5815432132388878, -45.46059095889125246, 164.1444404487539828 ) ) ;
#30290=CARTESIAN_POINT ( 'NONE',  ( 98.43831584450654759, -42.68208710540699258, 122.8070538473389490 ) ) ;
#30291=CARTESIAN_POINT ( 'NONE',  ( 109.7248659736901999, -27.00080519511008248, 119.8647919382667055 ) ) ;
#30292=CARTESIAN_POINT ( 'NONE',  ( 117.0509866428105710, -35.93349926821310447, 18.88982133577855649 ) ) ;
#30293=CIRCLE ( 'NONE', #25949, 5.599999999999994316 ) ;
#30295=CIRCLE ( 'NONE', #2757, 2.117000000000000881 ) ;
#30297=ORIENTED_EDGE ( 'NONE', *, *, #76346, .F. ) ;
#30298=EDGE_LOOP ( 'NONE', ( #37450, #32656, #64873, #79556 ) ) ;
#30300=CARTESIAN_POINT ( 'NONE',  ( 100.3081386793954408, -31.32336695771306623, 193.5957094172099744 ) ) ;
#30303=CARTESIAN_POINT ( 'NONE',  ( 96.89953391513134306, -32.33301889150666142, 61.01372051400599616 ) ) ;
#30305=CARTESIAN_POINT ( 'NONE',  ( 117.4658636684177679, -37.01502254527063940, 43.80419670448293346 ) ) ;
#30306=CARTESIAN_POINT ( 'NONE',  ( 117.0378900095125942, -33.61363155034663208, 170.0670538473399631 ) ) ;
#30309=CARTESIAN_POINT ( 'NONE',  ( 103.1746689306972939, -27.05803214298817849, 126.3813395616259783 ) ) ;
#30310=DIRECTION ( 'NONE',  ( 0.000000000000000000, 0.000000000000000000, -1.000000000000000000 ) ) ;
#30313=DIRECTION ( 'NONE',  ( 0.0001713722456127401463, -0.9999999853157766072, -1.713722456137401502E-19 ) ) ;
#30314=EDGE_CURVE ( 'NONE', #55131, #2012, #17854, .T. ) ;
#30315=ADVANCED_FACE ( 'NONE', ( #11038 ), #53233, .T. ) ;
#30316=EDGE_LOOP ( 'NONE', ( #58151, #906, #27204, #71785 ) ) ;
#30318=DIRECTION ( 'NONE',  ( 0.000000000000000000, 0.000000000000000000, 1.000000000000000000 ) ) ;
#30319=ORIENTED_EDGE ( 'NONE', *, *, #65275, .F. ) ;
#30320=VERTEX_POINT ( 'NONE', #82677 ) ;
#30322=FACE_OUTER_BOUND ( 'NONE', #47545, .T. ) ;
#30323=LINE ( 'NONE', #3944, #69644 ) ;
#30324=CARTESIAN_POINT ( 'NONE',  ( 96.33825113647944249, -41.76388066030261115, 61.67562527591097421 ) ) ;
#30329=CARTESIAN_POINT ( 'NONE',  ( 100.8863495415024119, -28.40209871822978371, 35.59657765686397113 ) ) ;
#30331=CARTESIAN_POINT ( 'NONE',  ( 108.6454077996538246, -25.81962716842098970, 145.9737205140069420 ) ) ;
#30334=ORIENTED_EDGE ( 'NONE', *, *, #28781, .F. ) ;
#30338=PLANE ( 'NONE',  #80686 ) ;
#30341=CARTESIAN_POINT ( 'NONE',  ( 110.0646822317013118, -26.04189894992025955, 219.8708633711489711 ) ) ;
#30342=ORIENTED_EDGE ( 'NONE', *, *, #31926, .T. ) ;
#30344=CARTESIAN_POINT ( 'NONE',  ( 115.7943364950945977, -30.98820711043258669, 250.2899109901966028 ) ) ;
#30345=CARTESIAN_POINT ( 'NONE',  ( 102.5393486652204160, -27.29027178147674348, 91.43276813305395478 ) ) ;
#30347=CARTESIAN_POINT ( 'NONE',  ( 113.2430583326422493, -28.75680677547383723, 190.5522713588539148 ) ) ;
#30348=VECTOR ( 'NONE', #46989, 1000.000000000000000 ) ;
#30351=VERTEX_POINT ( 'NONE', #66442 ) ;
#30352=EDGE_LOOP ( 'NONE', ( #21350, #53792, #28973, #28454 ) ) ;
#30356=CARTESIAN_POINT ( 'NONE',  ( 118.1075207852818068, -36.21034067742461815, 264.8518157521014587 ) ) ;
#30359=EDGE_CURVE ( 'NONE', #7162, #67833, #4229, .T. ) ;
#30360=AXIS2_PLACEMENT_3D ( 'NONE', #43614, #37724, #51765 ) ;
#30364=FACE_OUTER_BOUND ( 'NONE', #74019, .T. ) ;
#30365=CARTESIAN_POINT ( 'NONE',  ( 107.5482541545970605, -45.77270802984816811, 197.0533722090289643 ) ) ;
#30367=VERTEX_POINT ( 'NONE', #31922 ) ;
#30369=CIRCLE ( 'NONE', #49206, 3.000000000000002665 ) ;
#30370=ORIENTED_EDGE ( 'NONE', *, *, #32590, .F. ) ;
#30371=CARTESIAN_POINT ( 'NONE',  ( 110.8561819789184284, -45.98353734325511510, 182.8857722960176204 ) ) ;
#30372=CARTESIAN_POINT ( 'NONE',  ( 106.2788006184939888, -47.06957971430141185, 263.5280062282914741 ) ) ;
#30375=CARTESIAN_POINT ( 'NONE',  ( 109.6422150510572635, -46.48028739024776002, 27.78139385761759428 ) ) ;
#30376=ORIENTED_EDGE ( 'NONE', *, *, #1151, .T. ) ;
#30377=CARTESIAN_POINT ( 'NONE',  ( 77.52387074035010528, -35.68172011937328136, 2.822018711113899236 ) ) ;
#30378=VERTEX_POINT ( 'NONE', #27235 ) ;
#30379=CARTESIAN_POINT ( 'NONE',  ( 168.0371591254543944, -48.62818131005519007, 237.4678068554150059 ) ) ;
#30380=CARTESIAN_POINT ( 'NONE',  ( 98.69396380956492010, -33.82637249272325164, 282.4930118773256709 ) ) ;
#30382=DIRECTION ( 'NONE',  ( 1.000000000000000078E-15, -1.000000000000000083E-30, -1.000000000000000000 ) ) ;
#30383=DIRECTION ( 'NONE',  ( -4.299999999999999979E-14, 1.000000000000000000, -4.400000000000000367E-29 ) ) ;
#30384=AXIS2_PLACEMENT_3D ( 'NONE', #75788, #88969, #64841 ) ;
#30385=FACE_OUTER_BOUND ( 'NONE', #17307, .T. ) ;
#30387=DIRECTION ( 'NONE',  ( 1.000000000000000078E-15, -1.000000000000000083E-30, -1.000000000000000000 ) ) ;
#30388=CARTESIAN_POINT ( 'NONE',  ( 51.06648329127400388, -18.82844715994099971, 333.4006252759120343 ) ) ;
#30389=ORIENTED_EDGE ( 'NONE', *, *, #17702, .T. ) ;
#30390=CARTESIAN_POINT ( 'NONE',  ( 107.3210346550871179, -25.67891364084480799, 75.04610146638695767 ) ) ;
#30392=CARTESIAN_POINT ( 'NONE',  ( 98.68252487213293023, -38.50746385042646125, 30.91527697093399141 ) ) ;
#30394=CARTESIAN_POINT ( 'NONE',  ( 115.8258230018156354, -33.33084548093709287, 90.54063092494496345 ) ) ;
#30395=LINE ( 'NONE', #2252, #50586 ) ;
#30396=CARTESIAN_POINT ( 'NONE',  ( 172.5664832912729878, -18.82844715994071194, 15.92562527591207022 ) ) ;
#30399=EDGE_CURVE ( 'NONE', #43566, #4960, #59618, .T. ) ;
#30400=CARTESIAN_POINT ( 'NONE',  ( 106.2234015700748699, -47.79681864418333959, 263.5280062282922131 ) ) ;
#30402=ORIENTED_EDGE ( 'NONE', *, *, #38046, .F. ) ;
#30403=FACE_OUTER_BOUND ( 'NONE', #30591, .T. ) ;
#30404=ORIENTED_EDGE ( 'NONE', *, *, #70513, .F. ) ;
#30405=CARTESIAN_POINT ( 'NONE',  ( 117.6248412043677121, -33.30620651169719082, 130.0880062282919880 ) ) ;
#30406=CARTESIAN_POINT ( 'NONE',  ( 79.11888855177762991, -21.31186128672829128, 1.764000668898225044 ) ) ;
#30409=EDGE_CURVE ( 'NONE', #33706, #65644, #58284, .T. ) ;
#30410=EDGE_CURVE ( 'NONE', #17392, #59373, #11494, .T. ) ;
#30411=DIRECTION ( 'NONE',  ( 1.000000000000000078E-15, -1.000000000000000083E-30, -1.000000000000000000 ) ) ;
#30412=VECTOR ( 'NONE', #62762, 1000.000000000000000 ) ;
#30413=EDGE_CURVE ( 'NONE', #11261, #88962, #52410, .T. ) ;
#30414=DIRECTION ( 'NONE',  ( 1.071939472051879986E-15, 0.000000000000000000, 1.000000000000000000 ) ) ;
#30415=CARTESIAN_POINT ( 'NONE',  ( 116.5663773505005310, -40.88766770462213884, 208.4861014663879644 ) ) ;
#30416=CARTESIAN_POINT ( 'NONE',  ( 172.5664832912740110, -36.32844715994070839, 138.9256252759119832 ) ) ;
#30419=CARTESIAN_POINT ( 'NONE',  ( 96.65901483881968659, -33.00673566691533978, 22.06514908543494258 ) ) ;
#30421=ORIENTED_EDGE ( 'NONE', *, *, #54154, .T. ) ;
#30422=CARTESIAN_POINT ( 'NONE',  ( 115.7815775597082109, -31.78852007784938039, 170.2368360151835702 ) ) ;
#30423=AXIS2_PLACEMENT_3D ( 'NONE', #59262, #16608, #58376 ) ;
#30424=CARTESIAN_POINT ( 'NONE',  ( 163.0667039024469034, -32.29483332967940612, 117.4678068554150485 ) ) ;
#30426=VECTOR ( 'NONE', #75791, 1000.000000000000000 ) ;
#30427=AXIS2_PLACEMENT_3D ( 'NONE', #10179, #36995, #64701 ) ;
#30428=EDGE_CURVE ( 'NONE', #44647, #59006, #68411, .T. ) ;
#30429=CARTESIAN_POINT ( 'NONE',  ( 81.20961857873741963, -21.23068377182416455, 1.829869271363169458 ) ) ;
#30430=CARTESIAN_POINT ( 'NONE',  ( 180.1667039024460166, -26.71338133339240528, -5.074374724088000832 ) ) ;
#30431=CARTESIAN_POINT ( 'NONE',  ( 99.76842024043810397, -29.31547782932919688, 225.6956252759109702 ) ) ;
#30433=FACE_BOUND ( 'NONE', #20400, .T. ) ;
#30434=CARTESIAN_POINT ( 'NONE',  ( 63.06670390244641311, -24.92844715994017335, 180.4678068554151196 ) ) ;
#30436=CARTESIAN_POINT ( 'NONE',  ( 104.8198721574821803, -27.95645401395800533, 244.7105150661719790 ) ) ;
#30438=CARTESIAN_POINT ( 'NONE',  ( 103.4847015977353379, -25.45917443855082496, 51.32133956162493149 ) ) ;
#30440=CARTESIAN_POINT ( 'NONE',  ( 108.2818241440822788, -26.29514120620494921, 129.9841967044819739 ) ) ;
#30441=ORIENTED_EDGE ( 'NONE', *, *, #41022, .T. ) ;
#30442=CARTESIAN_POINT ( 'NONE',  ( 131.8668787344577424, -20.38871026387126051, 7.389079501607389133 ) ) ;
#30443=ORIENTED_EDGE ( 'NONE', *, *, #33326, .F. ) ;
#30444=AXIS2_PLACEMENT_3D ( 'NONE', #58756, #79691, #88292 ) ;
#30445=CARTESIAN_POINT ( 'NONE',  ( 107.0664832912739968, -36.72944715994100306, -1.864374724089012947 ) ) ;
#30446=CARTESIAN_POINT ( 'NONE',  ( 103.7389900727278729, -27.29752428252023577, 276.3463639899791815 ) ) ;
#30449=CARTESIAN_POINT ( 'NONE',  ( 62.03715912545833078, -47.82818131006021645, 313.9678068554150059 ) ) ;
#30450=ORIENTED_EDGE ( 'NONE', *, *, #29747, .T. ) ;
#30451=CARTESIAN_POINT ( 'NONE',  ( 130.5667039024479834, -36.72944715994093912, 239.5838068554170377 ) ) ;
#30454=CARTESIAN_POINT ( 'NONE',  ( 116.3259296754763028, -32.93870509136930025, 260.1356252759109680 ) ) ;
#30456=CARTESIAN_POINT ( 'NONE',  ( 116.6952228212742995, -32.58508497927773817, 79.14991099019697174 ) ) ;
#30458=FACE_OUTER_BOUND ( 'NONE', #21155, .T. ) ;
#30459=CARTESIAN_POINT ( 'NONE',  ( 108.3334480745109545, -46.73485935675521574, 142.6772919409591509 ) ) ;
#30460=VERTEX_POINT ( 'NONE', #15421 ) ;
#30461=AXIS2_PLACEMENT_3D ( 'NONE', #71119, #2068, #85205 ) ;
#30462=DIRECTION ( 'NONE',  ( 8.673617379884035472E-16, 1.000000000000000000, 0.000000000000000000 ) ) ;
#30463=DIRECTION ( 'NONE',  ( 0.000000000000000000, 0.000000000000000000, -1.000000000000000000 ) ) ;
#30465=CARTESIAN_POINT ( 'NONE',  ( 184.5667039024480118, -67.87844715994100397, 300.9178068554150514 ) ) ;
#30468=CARTESIAN_POINT ( 'NONE',  ( 25.56670390244797275, -62.87844715994099687, 254.4678068554150343 ) ) ;
#30469=AXIS2_PLACEMENT_3D ( 'NONE', #47226, #53579, #53123 ) ;
#30470=ORIENTED_EDGE ( 'NONE', *, *, #75755, .T. ) ;
#30471=PLANE ( 'NONE',  #88276 ) ;
#30472=CARTESIAN_POINT ( 'NONE',  ( 113.8941270090216733, -29.67983328691853018, 170.4641967044819637 ) ) ;
#30473=LINE ( 'NONE', #72708, #66025 ) ;
#30476=CARTESIAN_POINT ( 'NONE',  ( 105.4283309587863613, -27.08694620864308789, 11.20991099019597037 ) ) ;
#30477=LINE ( 'NONE', #57270, #35290 ) ;
#30478=DIRECTION ( 'NONE',  ( 0.000000000000000000, 0.000000000000000000, 1.000000000000000000 ) ) ;
#30479=CARTESIAN_POINT ( 'NONE',  ( 167.2371591254542693, -47.82818131005522844, 300.4678068554149490 ) ) ;
#30480=AXIS2_PLACEMENT_3D ( 'NONE', #49992, #63190, #7781 ) ;
#30481=ORIENTED_EDGE ( 'NONE', *, *, #69276, .T. ) ;
#30484=CARTESIAN_POINT ( 'NONE',  ( 114.8736367985563334, -30.83777597042981711, 219.3413395616259720 ) ) ;
#30487=CARTESIAN_POINT ( 'NONE',  ( 115.3361691346596558, -39.99662111280561305, 189.9587261630399553 ) ) ;
#30488=AXIS2_PLACEMENT_3D ( 'NONE', #14232, #35101, #76904 ) ;
#30489=EDGE_CURVE ( 'NONE', #28975, #22460, #10442, .T. ) ;
#30490=CARTESIAN_POINT ( 'NONE',  ( 182.3467384525650061, -29.62846900982231446, -5.074374724088000832 ) ) ;
#30491=CARTESIAN_POINT ( 'NONE',  ( 106.6003420031022415, -27.34545878416701115, 41.55967854399195005 ) ) ;
#30493=DIRECTION ( 'NONE',  ( 0.000000000000000000, 0.000000000000000000, -1.000000000000000000 ) ) ;
#30494=CARTESIAN_POINT ( 'NONE',  ( 88.17226027475679473, -58.72944715994100306, 239.5838068554174924 ) ) ;
#30495=ORIENTED_EDGE ( 'NONE', *, *, #89050, .F. ) ;
#30496=CARTESIAN_POINT ( 'NONE',  ( 62.03715912545828814, -47.82818131006021645, 249.9678068554150343 ) ) ;
#30497=CARTESIAN_POINT ( 'NONE',  ( 48.86082318535700608, -35.55794170701751256, -5.074374724088000832 ) ) ;
#30498=CARTESIAN_POINT ( 'NONE',  ( 96.29057984255072711, -34.37493501460198075, 256.1432443235300980 ) ) ;
#30503=CIRCLE ( 'NONE', #79867, 5.599999999999994316 ) ;
#30504=CYLINDRICAL_SURFACE ( 'NONE', #31613, 2.030000000001807248 ) ;
#30505=CARTESIAN_POINT ( 'NONE',  ( 134.0664832912739826, -8.729447159941003065, 4.925625275910997303 ) ) ;
#30506=CARTESIAN_POINT ( 'NONE',  ( 115.0831197249979851, -29.02584261466837390, 35.43562527591098643 ) ) ;
#30508=ORIENTED_EDGE ( 'NONE', *, *, #50935, .F. ) ;
#30509=CARTESIAN_POINT ( 'NONE',  ( 101.9391980234526187, -27.60234874203171884, 56.48419670448296159 ) ) ;
#30510=LINE ( 'NONE', #16438, #35174 ) ;
#30511=CARTESIAN_POINT ( 'NONE',  ( 114.4151681834755294, -27.43228005255051016, 274.5441967044824878 ) ) ;
#30513=ORIENTED_EDGE ( 'NONE', *, *, #26841, .T. ) ;
#30514=AXIS2_PLACEMENT_3D ( 'NONE', #69736, #54724, #70632 ) ;
#30516=CARTESIAN_POINT ( 'NONE',  ( 41.56648329127398966, -18.82844715994071194, 138.9256252759119832 ) ) ;
#30517=CARTESIAN_POINT ( 'NONE',  ( 53.56670390244743629, -48.82844715994058049, 180.4678068554151196 ) ) ;
#30518=CYLINDRICAL_SURFACE ( 'NONE', #74094, 9.999999999999998224 ) ;
#30519=CARTESIAN_POINT ( 'NONE',  ( 112.9396172237807860, -42.43812354398048114, 96.03094751244795191 ) ) ;
#30520=CARTESIAN_POINT ( 'NONE',  ( 116.8155376854491720, -40.58108761943747567, 189.5270538473389479 ) ) ;
#30523=VERTEX_POINT ( 'NONE', #65342 ) ;
#30524=EDGE_CURVE ( 'NONE', #74810, #40280, #87135, .T. ) ;
#30525=DIRECTION ( 'NONE',  ( -9.868649107779159826E-16, 0.000000000000000000, 1.000000000000000000 ) ) ;
#30526=AXIS2_PLACEMENT_3D ( 'NONE', #43095, #70839, #78105 ) ;
#30530=FACE_OUTER_BOUND ( 'NONE', #55712, .T. ) ;
#30531=EDGE_LOOP ( 'NONE', ( #56476, #4043, #86079, #46963 ) ) ;
#30532=VERTEX_POINT ( 'NONE', #86687 ) ;
#30534=CARTESIAN_POINT ( 'NONE',  ( 103.2798274406795116, -27.47411150201141439, 41.38551241025358962 ) ) ;
#30536=CARTESIAN_POINT ( 'NONE',  ( 98.02237212078092909, -37.19498283172546849, 120.8019436376009708 ) ) ;
#30537=CARTESIAN_POINT ( 'NONE',  ( 117.5135424720979103, -36.80237478700602338, 263.8213395616250523 ) ) ;
#30538=AXIS2_PLACEMENT_3D ( 'NONE', #35171, #49700, #29277 ) ;
#30539=CARTESIAN_POINT ( 'NONE',  ( 107.0664832912739399, -36.72944715994095333, 247.7440089327910755 ) ) ;
#30540=VERTEX_POINT ( 'NONE', #38963 ) ;
#30542=CARTESIAN_POINT ( 'NONE',  ( 97.06383274664968042, -37.34207438287794645, 137.3751712589593126 ) ) ;
#30545=DIRECTION ( 'NONE',  ( -0.7071067811875165754, -0.7071067811855784591, -7.071067811875470201E-16 ) ) ;
#30548=DIRECTION ( 'NONE',  ( -2.999999999999999839E-15, 1.000000000000000000, -2.999999999999999900E-30 ) ) ;
#30551=CARTESIAN_POINT ( 'NONE',  ( 117.4908834113230682, -35.85893649831510999, 253.8927681330538348 ) ) ;
#30552=CARTESIAN_POINT ( 'NONE',  ( 115.6469432611725665, -28.48403513818922761, 35.43562527591098643 ) ) ;
#30554=FACE_OUTER_BOUND ( 'NONE', #32265, .T. ) ;
#30555=DIRECTION ( 'NONE',  ( 5.512527431108029424E-15, -1.000000000000000000, 0.000000000000000000 ) ) ;
#30556=FACE_OUTER_BOUND ( 'NONE', #71589, .T. ) ;
#30557=CARTESIAN_POINT ( 'NONE',  ( 152.0368932755770288, -23.42844715993588522, 313.9678068554149490 ) ) ;
#30558=LINE ( 'NONE', #79173, #9105 ) ;
#30559=CARTESIAN_POINT ( 'NONE',  ( 131.7606268095730684, -38.22815166920154439, 7.286367513305490817 ) ) ;
#30561=CARTESIAN_POINT ( 'NONE',  ( 112.1393456294539419, -28.01282277365494977, 10.65645861034278852 ) ) ;
#30562=CARTESIAN_POINT ( 'NONE',  ( 105.7157591367752758, -46.72390112185112088, 162.4687997112716289 ) ) ;
#30563=CARTESIAN_POINT ( 'NONE',  ( 116.3212776292293995, -32.94146857471267253, 120.1356252759109537 ) ) ;
#30564=CARTESIAN_POINT ( 'NONE',  ( 96.86726761138238828, -30.64586122335317953, 280.8984824187682534 ) ) ;
#30565=CARTESIAN_POINT ( 'NONE',  ( 112.4860951546057919, -26.19083136796355404, 165.6984824187679521 ) ) ;
#30566=CARTESIAN_POINT ( 'NONE',  ( 99.27755186283980038, -43.74455535675208040, 52.90991099019698396 ) ) ;
#30567=PLANE ( 'NONE',  #72567 ) ;
#30568=DIRECTION ( 'NONE',  ( -4.237773401492740281E-14, 1.000000000000000000, 0.000000000000000000 ) ) ;
#30570=CARTESIAN_POINT ( 'NONE',  ( 82.81644824798257787, -36.55833207211471603, 3.101428811465905433 ) ) ;
#30572=ORIENTED_EDGE ( 'NONE', *, *, #42633, .T. ) ;
#30574=VERTEX_POINT ( 'NONE', #50815 ) ;
#30575=AXIS2_PLACEMENT_3D ( 'NONE', #36890, #30525, #65044 ) ;
#30576=CARTESIAN_POINT ( 'NONE',  ( 114.5308976578478166, -43.10096916487045604, 59.26419670448196086 ) ) ;
#30577=FACE_OUTER_BOUND ( 'NONE', #66701, .T. ) ;
#30579=VECTOR ( 'NONE', #46961, 1000.000000000000000 ) ;
#30580=CARTESIAN_POINT ( 'NONE',  ( 97.81169418859235520, -40.51741816698509524, 47.63568902202231925 ) ) ;
#30581=CARTESIAN_POINT ( 'NONE',  ( 97.07914014679033698, -41.41098531455288168, 207.6632443235299661 ) ) ;
#30582=DIRECTION ( 'NONE',  ( 0.000000000000000000, 0.000000000000000000, -1.000000000000000000 ) ) ;
#30583=LINE ( 'NONE', #78758, #37090 ) ;
#30585=CARTESIAN_POINT ( 'NONE',  ( 97.07207205650352932, -35.37844121661813546, 47.21895861061143052 ) ) ;
#30586=PLANE ( 'NONE',  #89743 ) ;
#30587=CARTESIAN_POINT ( 'NONE',  ( 97.81201254632964037, -40.51821635194160365, 96.63569287326528467 ) ) ;
#30588=CARTESIAN_POINT ( 'NONE',  ( 116.2961327041338535, -39.96626766897450977, 133.5584824187689605 ) ) ;
#30590=CIRCLE ( 'NONE', #48002, 1.000000000000000888 ) ;
#30591=EDGE_LOOP ( 'NONE', ( #85701, #14656, #56131, #69960 ) ) ;
#30592=CARTESIAN_POINT ( 'NONE',  ( 103.9179606659962616, -45.58175368509670733, 98.74824997256392578 ) ) ;
#30594=EDGE_CURVE ( 'NONE', #85915, #23208, #73037, .T. ) ;
#30595=FACE_OUTER_BOUND ( 'NONE', #7651, .T. ) ;
#30596=CARTESIAN_POINT ( 'NONE',  ( 117.1144258088630039, -31.97015794161414703, 210.1784824187679703 ) ) ;
#30597=FACE_OUTER_BOUND ( 'NONE', #49878, .T. ) ;
#30599=FACE_BOUND ( 'NONE', #85532, .T. ) ;
#30604=CARTESIAN_POINT ( 'NONE',  ( 103.0581626738561880, -26.45339789934162411, 170.3603871806729444 ) ) ;
#30605=ORIENTED_EDGE ( 'NONE', *, *, #10224, .T. ) ;
#30612=DIRECTION ( 'NONE',  ( -4.237773401492740281E-14, 1.000000000000000000, 0.000000000000000000 ) ) ;
#30613=CARTESIAN_POINT ( 'NONE',  ( 109.4041143893713297, -28.39659615353044231, 217.6890427505439902 ) ) ;
#30614=AXIS2_PLACEMENT_3D ( 'NONE', #86200, #66176, #31214 ) ;
#30615=CARTESIAN_POINT ( 'NONE',  ( 41.56648329127398966, -27.57844715994070484, 15.92562527591200094 ) ) ;
#30616=CARTESIAN_POINT ( 'NONE',  ( 109.8560245667294311, -26.68427469084152293, 174.8613395616249591 ) ) ;
#30617=CYLINDRICAL_SURFACE ( 'NONE', #48885, 2.117000000000000881 ) ;
#30620=ORIENTED_EDGE ( 'NONE', *, *, #25206, .T. ) ;
#30621=ORIENTED_EDGE ( 'NONE', *, *, #34710, .T. ) ;
#30622=VECTOR ( 'NONE', #70296, 1000.000000000000000 ) ;
#30626=DIRECTION ( 'NONE',  ( 0.000000000000000000, 0.000000000000000000, -1.000000000000000000 ) ) ;
#30628=CARTESIAN_POINT ( 'NONE',  ( 99.56565989216673529, -33.50937434423423156, 13.82237608387698558 ) ) ;
#30630=VERTEX_POINT ( 'NONE', #4003 ) ;
#30632=CARTESIAN_POINT ( 'NONE',  ( 115.2616190319047433, -40.84650019411598976, 9.635625275910943088 ) ) ;
#30633=CYLINDRICAL_SURFACE ( 'NONE', #31441, 3.250000000000002665 ) ;
#30635=VERTEX_POINT ( 'NONE', #31704 ) ;
#30636=CARTESIAN_POINT ( 'NONE',  ( 115.9332344144704194, -41.42518548927348121, 113.4390407645330185 ) ) ;
#30637=EDGE_LOOP ( 'NONE', ( #53789, #21667, #12885, #3541, #37514 ) ) ;
#30638=ORIENTED_EDGE ( 'NONE', *, *, #70515, .F. ) ;
#30639=ADVANCED_FACE ( 'NONE', ( #17201 ), #22001, .T. ) ;
#30640=CARTESIAN_POINT ( 'NONE',  ( 98.28161005395152472, -38.92874716189901818, 15.95622935188595370 ) ) ;
#30641=CARTESIAN_POINT ( 'NONE',  ( 96.62784866533952766, -37.15519789137512419, 161.3584824187679487 ) ) ;
#30643=CARTESIAN_POINT ( 'NONE',  ( 95.80265872640100611, -40.33145541733363615, 131.5727681330539554 ) ) ;
#30644=EDGE_CURVE ( 'NONE', #2462, #67095, #72614, .T. ) ;
#30646=CARTESIAN_POINT ( 'NONE',  ( 116.2186307022408727, -41.79497087860992366, 259.4241967044825969 ) ) ;
#30647=LINE ( 'NONE', #58343, #9379 ) ;
#30650=ORIENTED_EDGE ( 'NONE', *, *, #33959, .T. ) ;
#30651=ORIENTED_EDGE ( 'NONE', *, *, #22798, .T. ) ;
#30654=CARTESIAN_POINT ( 'NONE',  ( 106.9746081534954669, -47.19836424831742505, 187.5699109901969734 ) ) ;
#30656=CARTESIAN_POINT ( 'NONE',  ( 108.2778356434855027, -47.71639565607667066, 157.6518157521019532 ) ) ;
#30659=DIRECTION ( 'NONE',  ( 0.000000000000000000, 0.000000000000000000, -1.000000000000000000 ) ) ;
#30660=CARTESIAN_POINT ( 'NONE',  ( 41.56670390244804025, -42.82844715994103524, 300.4678068554150059 ) ) ;
#30661=CARTESIAN_POINT ( 'NONE',  ( 107.0664832912739968, -36.72944715994100306, 287.6356252759109680 ) ) ;
#30662=CARTESIAN_POINT ( 'NONE',  ( 106.8369185487093063, -47.13021470646864941, 268.5584824187679374 ) ) ;
#30663=CARTESIAN_POINT ( 'NONE',  ( 85.58420390244799592, -43.72944715994107412, 231.5838068554169524 ) ) ;
#30667=CARTESIAN_POINT ( 'NONE',  ( 97.81171235735017433, -40.51746255502365557, 257.6350867217079212 ) ) ;
#30668=FACE_OUTER_BOUND ( 'NONE', #46190, .T. ) ;
#30669=CIRCLE ( 'NONE', #10373, 2.750000000000002665 ) ;
#30670=CARTESIAN_POINT ( 'NONE',  ( 114.3253520721945620, -31.31565170232914497, 195.5838068554167819 ) ) ;
#30671=ORIENTED_EDGE ( 'NONE', *, *, #1637, .F. ) ;
#30673=CARTESIAN_POINT ( 'NONE',  ( 118.9025049541195358, -37.70032671045152028, 188.7613395616259595 ) ) ;
#30674=CARTESIAN_POINT ( 'NONE',  ( 106.9273518165185948, -26.26990724610170247, 56.08705384733997334 ) ) ;
#30675=CARTESIAN_POINT ( 'NONE',  ( 96.73312529990856490, -40.78150971882554643, 242.6118157521009664 ) ) ;
#30677=DIRECTION ( 'NONE',  ( 0.7071067811864886199, 0.7071067811866064146, 7.071067811864879743E-16 ) ) ;
#30678=DIRECTION ( 'NONE',  ( 0.000000000000000000, 0.000000000000000000, -1.000000000000000000 ) ) ;
#30679=CARTESIAN_POINT ( 'NONE',  ( 116.9190213240937197, -38.53463890124888280, 39.68201433323524441 ) ) ;
#30680=CARTESIAN_POINT ( 'NONE',  ( 167.2371591254542693, -47.82818131005522844, 300.4678068554149490 ) ) ;
#30681=LINE ( 'NONE', #4320, #74581 ) ;
#30682=ORIENTED_EDGE ( 'NONE', *, *, #56157, .F. ) ;
#30683=DIRECTION ( 'NONE',  ( -1.000000000000000000, -3.999999999999999995E-14, 4.193851878741028267E-47 ) ) ;
#30685=ORIENTED_EDGE ( 'NONE', *, *, #13705, .T. ) ;
#30688=CARTESIAN_POINT ( 'NONE',  ( 100.0140161817732860, -31.91085406740108610, 120.2724198280769912 ) ) ;
#30689=CARTESIAN_POINT ( 'NONE',  ( 160.7738106836351051, -48.62134037874900372, 129.9678068554149775 ) ) ;
#30690=ORIENTED_EDGE ( 'NONE', *, *, #11856, .T. ) ;
#30691=CARTESIAN_POINT ( 'NONE',  ( 108.0321269276242049, -25.74166508409292220, 105.9946728949589811 ) ) ;
#30693=AXIS2_PLACEMENT_3D ( 'NONE', #6639, #67513, #34335 ) ;
#30695=CARTESIAN_POINT ( 'NONE',  ( 80.06648329127402519, -36.72944715994107412, -5.074374724089057764 ) ) ;
#30696=CARTESIAN_POINT ( 'NONE',  ( 103.0217603569634690, -26.37318327779222216, 20.37276813305394185 ) ) ;
#30697=ORIENTED_EDGE ( 'NONE', *, *, #52266, .T. ) ;
#30699=ORIENTED_EDGE ( 'NONE', *, *, #34177, .T. ) ;
#30701=ADVANCED_FACE ( 'NONE', ( #66673 ), #4459, .F. ) ;
#30702=LINE ( 'NONE', #44314, #70375 ) ;
#30703=DIRECTION ( 'NONE',  ( 1.000000000000000078E-15, 1.000000000000000083E-30, -1.000000000000000000 ) ) ;
#30704=CARTESIAN_POINT ( 'NONE',  ( 162.5667039024470171, -33.35206098992711077, -5.074374724088000832 ) ) ;
#30705=DIRECTION ( 'NONE',  ( 1.907762142705490052E-15, 7.167082501179359715E-16, -1.000000000000000000 ) ) ;
#30706=DIRECTION ( 'NONE',  ( 0.000000000000000000, 0.000000000000000000, -1.000000000000000000 ) ) ;
#30707=CARTESIAN_POINT ( 'NONE',  ( 97.31300249461010310, -38.96030167564788371, 52.50535227464659727 ) ) ;
#30708=CARTESIAN_POINT ( 'NONE',  ( 177.4809174648213741, -49.32844715993478957, 300.4678068554149490 ) ) ;
#30709=CIRCLE ( 'NONE', #40864, 2.500000000000002220 ) ;
#30711=CARTESIAN_POINT ( 'NONE',  ( 117.4658636684177679, -37.01502254527063940, 43.80419670448293346 ) ) ;
#30718=CARTESIAN_POINT ( 'NONE',  ( 115.1291642039608547, -38.00337907228554712, 111.5195189410199674 ) ) ;
#30719=VECTOR ( 'NONE', #59225, 1000.000000000000000 ) ;
#30724=ORIENTED_EDGE ( 'NONE', *, *, #8757, .T. ) ;
#30726=ORIENTED_EDGE ( 'NONE', *, *, #24940, .F. ) ;
#30730=CARTESIAN_POINT ( 'NONE',  ( 115.3457950989190408, -42.46736495413998824, 159.7758690201829666 ) ) ;
#30732=CARTESIAN_POINT ( 'NONE',  ( 117.7257289732168744, -39.74036323029751117, 139.6194347997199827 ) ) ;
#30733=CARTESIAN_POINT ( 'NONE',  ( 97.33784135113081959, -34.07106438717736552, 121.1147919308765353 ) ) ;
#30734=CARTESIAN_POINT ( 'NONE',  ( 109.6423256655219660, -46.48025961810147066, 17.78142711047368962 ) ) ;
#30735=ORIENTED_EDGE ( 'NONE', *, *, #1891, .T. ) ;
#30736=VECTOR ( 'NONE', #72635, 1000.000000000000000 ) ;
#30737=ORIENTED_EDGE ( 'NONE', *, *, #63632, .F. ) ;
#30738=VERTEX_POINT ( 'NONE', #5812 ) ;
#30740=EDGE_CURVE ( 'NONE', #944, #41003, #54813, .T. ) ;
#30741=CARTESIAN_POINT ( 'NONE',  ( 115.5869623526398016, -35.21209367091628906, 196.7728522743529425 ) ) ;
#30742=CARTESIAN_POINT ( 'NONE',  ( 103.5913855974186362, -46.58186107657011377, 57.30705384733997221 ) ) ;
#30743=ORIENTED_EDGE ( 'NONE', *, *, #25207, .T. ) ;
#30744=CARTESIAN_POINT ( 'NONE',  ( 96.73636544059188225, -37.96124694896867169, 41.42133956162496844 ) ) ;
#30745=CARTESIAN_POINT ( 'NONE',  ( 113.1756163759788620, -44.75386896731635744, 253.0940677049611338 ) ) ;
#30746=EDGE_CURVE ( 'NONE', #40826, #68446, #81674, .T. ) ;
#30747=PLANE ( 'NONE',  #84370 ) ;
#30749=CARTESIAN_POINT ( 'NONE',  ( 96.67093460706618657, -35.94617138369610387, 142.2670538473399517 ) ) ;
#30750=AXIS2_PLACEMENT_3D ( 'NONE', #64190, #1061, #15142 ) ;
#30751=CARTESIAN_POINT ( 'NONE',  ( 64.67079002020506096, -0.9301828534102468682, 361.9756252759101471 ) ) ;
#30752=EDGE_CURVE ( 'NONE', #63918, #58668, #33940, .T. ) ;
#30753=EDGE_LOOP ( 'NONE', ( #63916, #49194, #54267, #52783 ) ) ;
#30756=ADVANCED_FACE ( 'NONE', ( #88025 ), #19424, .T. ) ;
#30757=EDGE_LOOP ( 'NONE', ( #86248, #51833, #54820, #25228 ) ) ;
#30758=LINE ( 'NONE', #51181, #89802 ) ;
#30761=FACE_OUTER_BOUND ( 'NONE', #18730, .T. ) ;
#30762=CARTESIAN_POINT ( 'NONE',  ( 97.03967865257850178, -35.94463544949734057, 132.2646067221455155 ) ) ;
#30763=CARTESIAN_POINT ( 'NONE',  ( 117.4547340842499210, -37.95832963484174627, 53.73276813305394484 ) ) ;
#30765=CARTESIAN_POINT ( 'NONE',  ( 41.56648329127398966, -27.82844715994070484, 14.17562527591199917 ) ) ;
#30767=CARTESIAN_POINT ( 'NONE',  ( 115.6651410650259066, -32.06827565682259262, 69.22133956162596746 ) ) ;
#30768=DIRECTION ( 'NONE',  ( 1.000000000000000078E-15, -1.000000000000000000, 0.000000000000000000 ) ) ;
#30769=CARTESIAN_POINT ( 'NONE',  ( 109.6005296801413067, -26.60309369064642127, 195.8813395616249977 ) ) ;
#30770=DIRECTION ( 'NONE',  ( 1.000000000000000078E-15, -1.000000000000000083E-30, -1.000000000000000000 ) ) ;
#30772=EDGE_LOOP ( 'NONE', ( #28444, #27469, #55156, #37104 ) ) ;
#30773=CARTESIAN_POINT ( 'NONE',  ( 63.03715912545730760, -24.42818131006027826, 300.4678068554150627 ) ) ;
#30775=CARTESIAN_POINT ( 'NONE',  ( 87.06648329127403940, -54.72944906728955061, -5.074374724089050659 ) ) ;
#30776=CARTESIAN_POINT ( 'NONE',  ( 182.0374245136172249, -23.42844715993459559, 300.4678068554149490 ) ) ;
#30777=CARTESIAN_POINT ( 'NONE',  ( 96.60014388984734524, -36.47963607454698831, 196.3070538473399438 ) ) ;
#30778=ORIENTED_EDGE ( 'NONE', *, *, #75743, .T. ) ;
#30779=FACE_OUTER_BOUND ( 'NONE', #61541, .T. ) ;
#30780=CARTESIAN_POINT ( 'NONE',  ( 100.1243021666677606, -44.53607127582347402, 262.9984824187678782 ) ) ;
#30781=CARTESIAN_POINT ( 'NONE',  ( 97.89440201276070752, -31.60978508062128967, 106.9213395616259703 ) ) ;
#30782=CARTESIAN_POINT ( 'NONE',  ( 100.9565521831709987, -28.70555570752797792, 251.5995088816804355 ) ) ;
#30786=CARTESIAN_POINT ( 'NONE',  ( 98.30751334827748167, -41.72882313198851278, 262.7398596741535357 ) ) ;
#30790=ORIENTED_EDGE ( 'NONE', *, *, #65300, .F. ) ;
#30791=VERTEX_POINT ( 'NONE', #74842 ) ;
#30792=EDGE_LOOP ( 'NONE', ( #43524, #11743 ) ) ;
#30793=CARTESIAN_POINT ( 'NONE',  ( 138.8167039024479834, -67.87844715994100397, 86.31780685541500020 ) ) ;
#30794=CARTESIAN_POINT ( 'NONE',  ( 110.8926193997603065, -26.99384161864454157, 265.7784824187680783 ) ) ;
#30795=DIRECTION ( 'NONE',  ( 1.000000000000000000, 4.163336342344333240E-14, 0.000000000000000000 ) ) ;
#30796=LINE ( 'NONE', #79415, #89052 ) ;
#30797=VECTOR ( 'NONE', #77989, 1000.000000000000000 ) ;
#30798=CARTESIAN_POINT ( 'NONE',  ( 172.5664832912740110, -36.32844715994070839, 203.6756252759119832 ) ) ;
#30801=CARTESIAN_POINT ( 'NONE',  ( 109.5825779133427460, -28.02991049533996204, 214.2628960185529365 ) ) ;
#30802=ORIENTED_EDGE ( 'NONE', *, *, #82576, .F. ) ;
#30803=VERTEX_POINT ( 'NONE', #47561 ) ;
#30804=ORIENTED_EDGE ( 'NONE', *, *, #77481, .T. ) ;
#30807=DIRECTION ( 'NONE',  ( 1.000000000000000000, 3.930900487435134677E-14, 0.000000000000000000 ) ) ;
#30809=ADVANCED_FACE ( 'NONE', ( #19879 ), #46662, .F. ) ;
#30810=CARTESIAN_POINT ( 'NONE',  ( 97.60228370342871074, -39.19771807616534431, 272.5299109901961856 ) ) ;
#30811=CIRCLE ( 'NONE', #9043, 2.999999999999933387 ) ;
#30812=LINE ( 'NONE', #2673, #73422 ) ;
#30813=ADVANCED_FACE ( 'NONE', ( #87577 ), #26679, .F. ) ;
#30816=EDGE_CURVE ( 'NONE', #51305, #5456, #73943, .T. ) ;
#30817=ORIENTED_EDGE ( 'NONE', *, *, #1404, .T. ) ;
#30818=ADVANCED_FACE ( 'NONE', ( #12170 ), #13068, .F. ) ;
#30819=CARTESIAN_POINT ( 'NONE',  ( 100.9530876688875480, -28.70826590416694302, 56.59407357525381599 ) ) ;
#30820=ORIENTED_EDGE ( 'NONE', *, *, #80306, .F. ) ;
#30822=CARTESIAN_POINT ( 'NONE',  ( 111.0211786934911231, -29.03130846684521060, 17.52904275054395455 ) ) ;
#30824=DIRECTION ( 'NONE',  ( 0.000000000000000000, 0.000000000000000000, 1.000000000000000000 ) ) ;
#30825=EDGE_CURVE ( 'NONE', #36562, #41877, #53913, .T. ) ;
#30826=CARTESIAN_POINT ( 'NONE',  ( 49.16670390244752298, -28.27351298637373489, 237.4678068554150059 ) ) ;
#30828=ORIENTED_EDGE ( 'NONE', *, *, #69213, .F. ) ;
#30829=CARTESIAN_POINT ( 'NONE',  ( 172.5664832912740110, -36.32844715994070839, 314.1756252759120116 ) ) ;
#30830=CARTESIAN_POINT ( 'NONE',  ( 25.56670390244797275, -65.37844715994100397, 137.2178068554150059 ) ) ;
#30831=VECTOR ( 'NONE', #76262, 1000.000000000000000 ) ;
#30832=EDGE_CURVE ( 'NONE', #24378, #22610, #75736, .T. ) ;
#30834=CARTESIAN_POINT ( 'NONE',  ( 108.9852622695951112, -46.97665739950247143, 82.72419670448194040 ) ) ;
#30836=CARTESIAN_POINT ( 'NONE',  ( 105.1568233002730182, -45.58189704936153674, 31.84194363760095570 ) ) ;
#30837=EDGE_CURVE ( 'NONE', #37713, #34867, #48441, .T. ) ;
#30839=CARTESIAN_POINT ( 'NONE',  ( 97.94737569220006890, -41.00876738043628222, 58.10729759161198160 ) ) ;
#30840=CARTESIAN_POINT ( 'NONE',  ( 29.56670390244797630, -67.87844715994100397, 310.9178068554150514 ) ) ;
#30843=CARTESIAN_POINT ( 'NONE',  ( 100.3971814656068915, -28.68844771884695888, 36.62705384733894221 ) ) ;
#30844=FACE_OUTER_BOUND ( 'NONE', #73830, .T. ) ;
#30845=EDGE_LOOP ( 'NONE', ( #63794, #41112, #79944, #89730 ) ) ;
#30846=VECTOR ( 'NONE', #51820, 999.9999999999998863 ) ;
#30847=DIRECTION ( 'NONE',  ( 1.000000000000000000, 0.000000000000000000, -7.043400939473319300E-33 ) ) ;
#30849=CARTESIAN_POINT ( 'NONE',  ( 95.26251351713513316, -38.28569616102737427, 147.4299109901969871 ) ) ;
#30851=VERTEX_POINT ( 'NONE', #28472 ) ;
#30853=DIRECTION ( 'NONE',  ( -1.000000000000000078E-15, 0.000000000000000000, -1.000000000000000000 ) ) ;
#30854=CARTESIAN_POINT ( 'NONE',  ( 71.06648329127399677, -18.82844715994099971, 226.9256252759120116 ) ) ;
#30855=CARTESIAN_POINT ( 'NONE',  ( 115.9419818307744663, -40.91744192719425399, 228.4756252759109714 ) ) ;
#30859=CARTESIAN_POINT ( 'NONE',  ( 167.6524903400755875, -49.32844715993520879, 180.4678068554150059 ) ) ;
#30860=CARTESIAN_POINT ( 'NONE',  ( 118.0020517745808633, -38.33796275862062686, 69.72229194257801055 ) ) ;
#30862=CARTESIAN_POINT ( 'NONE',  ( 163.2569089553709034, -33.54226604284439617, 193.9678068554149775 ) ) ;
#30863=EDGE_CURVE ( 'NONE', #60356, #36108, #87341, .T. ) ;
#30864=VERTEX_POINT ( 'NONE', #77535 ) ;
#30865=CARTESIAN_POINT ( 'NONE',  ( 103.2894945095962242, -27.47016022250103973, 171.3846815306852704 ) ) ;
#30866=ADVANCED_FACE ( 'NONE', ( #28938 ), #77093, .F. ) ;
#30869=VECTOR ( 'NONE', #76900, 1000.000000000000000 ) ;
#30870=FACE_OUTER_BOUND ( 'NONE', #66168, .T. ) ;
#30872=CARTESIAN_POINT ( 'NONE',  ( 117.4525030917818782, -36.13006561810994555, 228.8727681330539667 ) ) ;
#30875=CYLINDRICAL_SURFACE ( 'NONE', #86772, 2.517500000000005844 ) ;
#30876=CARTESIAN_POINT ( 'NONE',  ( 98.63267121701338169, -35.20533560836722131, 240.6067055423629597 ) ) ;
#30878=DIRECTION ( 'NONE',  ( -0.7071067811864671926, -0.7071067811866279529, -6.612322855854137577E-17 ) ) ;
#30879=CARTESIAN_POINT ( 'NONE',  ( 118.0525141433397636, -37.71481444994962118, 29.74324432352998215 ) ) ;
#30881=CARTESIAN_POINT ( 'NONE',  ( 108.3247603638532865, -47.12287801086134920, 117.6727681330539639 ) ) ;
#30882=ORIENTED_EDGE ( 'NONE', *, *, #21789, .T. ) ;
#30883=DIRECTION ( 'NONE',  ( 1.000000000000000000, 4.237773401492740281E-14, 0.000000000000000000 ) ) ;
#30884=ORIENTED_EDGE ( 'NONE', *, *, #49803, .F. ) ;
#30886=CARTESIAN_POINT ( 'NONE',  ( 108.4174892303373241, -26.73503592435250198, 65.96895861098096248 ) ) ;
#30888=ORIENTED_EDGE ( 'NONE', *, *, #50705, .F. ) ;
#30889=FACE_OUTER_BOUND ( 'NONE', #40373, .T. ) ;
#30890=ORIENTED_EDGE ( 'NONE', *, *, #13091, .T. ) ;
#30892=DIRECTION ( 'NONE',  ( -4.237773401492740281E-14, 1.000000000000000000, 0.000000000000000000 ) ) ;
#30893=DIRECTION ( 'NONE',  ( 0.000000000000000000, -1.000000000000000000, 0.000000000000000000 ) ) ;
#30894=VERTEX_POINT ( 'NONE', #42098 ) ;
#30895=CARTESIAN_POINT ( 'NONE',  ( 117.1278252906914048, -39.54294340788323581, 98.60991099019594230 ) ) ;
#30897=DIRECTION ( 'NONE',  ( 0.000000000000000000, 0.000000000000000000, 1.000000000000000000 ) ) ;
#30898=CARTESIAN_POINT ( 'NONE',  ( 41.56648329127398966, -27.82844715994070484, 138.9256252759119832 ) ) ;
#30899=CARTESIAN_POINT ( 'NONE',  ( 109.6430121121371570, -46.48008674026510079, 142.7814586077414276 ) ) ;
#30900=ORIENTED_EDGE ( 'NONE', *, *, #9625, .T. ) ;
#30901=AXIS2_PLACEMENT_3D ( 'NONE', #87448, #52867, #60156 ) ;
#30902=DIRECTION ( 'NONE',  ( -4.237773401492740281E-14, 1.000000000000000000, 0.000000000000000000 ) ) ;
#30904=DIRECTION ( 'NONE',  ( -0.7071067811865671127, -0.7071067811865279218, -7.071067811865664660E-16 ) ) ;
#30906=DIRECTION ( 'NONE',  ( 0.000000000000000000, 0.000000000000000000, 1.000000000000000000 ) ) ;
#30908=ORIENTED_EDGE ( 'NONE', *, *, #50819, .F. ) ;
#30909=ADVANCED_FACE ( 'NONE', ( #55264, #14872 ), #69375, .F. ) ;
#30910=CARTESIAN_POINT ( 'NONE',  ( 115.0372575601887917, -42.90846249503305643, 34.30229194963032313 ) ) ;
#30911=EDGE_CURVE ( 'NONE', #14111, #38840, #42378, .T. ) ;
#30912=CARTESIAN_POINT ( 'NONE',  ( 108.2857792741417597, -47.02760743735399984, 158.6822919425769669 ) ) ;
#30913=DIRECTION ( 'NONE',  ( -4.237773401492740281E-14, 1.000000000000000000, 0.000000000000000000 ) ) ;
#30915=ADVANCED_FACE ( 'NONE', ( #15314 ), #83013, .T. ) ;
#30916=CARTESIAN_POINT ( 'NONE',  ( 100.2135729606528685, -43.75450166055420453, 17.96133956162493206 ) ) ;
#30925=CARTESIAN_POINT ( 'NONE',  ( 102.2066036383193222, -44.77047292137198298, 198.5634880678019272 ) ) ;
#30926=EDGE_CURVE ( 'NONE', #68369, #88451, #76636, .T. ) ;
#30928=FACE_OUTER_BOUND ( 'NONE', #29854, .T. ) ;
#30929=CARTESIAN_POINT ( 'NONE',  ( 100.3180865808431719, -43.26669944020724756, 38.38253568684996253 ) ) ;
#30931=AXIS2_PLACEMENT_3D ( 'NONE', #57782, #70532, #57324 ) ;
#30933=VECTOR ( 'NONE', #45340, 1000.000000000000000 ) ;
#30934=CARTESIAN_POINT ( 'NONE',  ( 104.4899544582702049, -26.97880758309926819, 80.28145860873343054 ) ) ;
#30935=DIRECTION ( 'NONE',  ( 1.000000000000000000, 4.299999999999999979E-14, 1.000000000000000078E-15 ) ) ;
#30936=ORIENTED_EDGE ( 'NONE', *, *, #76983, .F. ) ;
#30938=DIRECTION ( 'NONE',  ( 1.000000000000000078E-15, -1.000000000000000083E-30, -1.000000000000000000 ) ) ;
#30939=VERTEX_POINT ( 'NONE', #36195 ) ;
#30940=CARTESIAN_POINT ( 'NONE',  ( 103.0988156209413233, -47.86972635628425365, 252.3041967044823366 ) ) ;
#30943=EDGE_CURVE ( 'NONE', #6162, #73924, #64132, .T. ) ;
#30944=DIRECTION ( 'NONE',  ( 4.299999999999999979E-14, -1.000000000000000000, 0.000000000000000000 ) ) ;
#30946=CARTESIAN_POINT ( 'NONE',  ( 107.0664832912739968, -18.82844715994099971, 168.9256252759119832 ) ) ;
#30948=CARTESIAN_POINT ( 'NONE',  ( 113.0503328260151079, -46.07776482166018184, 214.0175300378159591 ) ) ;
#30950=ORIENTED_EDGE ( 'NONE', *, *, #79250, .T. ) ;
#30951=CARTESIAN_POINT ( 'NONE',  ( 115.9284861604400731, -31.15648700444841879, 30.27276813305396175 ) ) ;
#30953=CIRCLE ( 'NONE', #72957, 4.875000000000017764 ) ;
#30954=CARTESIAN_POINT ( 'NONE',  ( 110.9930863310008959, -46.38701419431276207, 282.8841967044824628 ) ) ;
#30955=ORIENTED_EDGE ( 'NONE', *, *, #72717, .F. ) ;
#30957=CARTESIAN_POINT ( 'NONE',  ( 78.24498361944210956, -38.78962918509265023, 7.677444906553891890 ) ) ;
#30958=CARTESIAN_POINT ( 'NONE',  ( 101.9938210835711203, -45.44620686955099131, 18.15674971878247490 ) ) ;
#30960=CARTESIAN_POINT ( 'NONE',  ( 115.1349747707284479, -33.59889284931170295, 91.92713798863898944 ) ) ;
#30961=CARTESIAN_POINT ( 'NONE',  ( 107.6557286256638264, -47.79009794008123890, 193.6308633711489620 ) ) ;
#30962=DIRECTION ( 'NONE',  ( 1.000000000000000000, 0.000000000000000000, 0.000000000000000000 ) ) ;
#30964=EDGE_CURVE ( 'NONE', #70690, #19753, #72872, .T. ) ;
#30966=VERTEX_POINT ( 'NONE', #43885 ) ;
#30967=EDGE_LOOP ( 'NONE', ( #9058, #23414, #8870, #83259 ) ) ;
#30969=DIRECTION ( 'NONE',  ( 1.042073847087816516E-15, 1.000000000000000000, 0.000000000000000000 ) ) ;
#30971=ORIENTED_EDGE ( 'NONE', *, *, #73537, .T. ) ;
#30972=PLANE ( 'NONE',  #87478 ) ;
#30974=CARTESIAN_POINT ( 'NONE',  ( 103.2961519303028552, -27.46744216278922579, 41.38410912957840537 ) ) ;
#30975=CARTESIAN_POINT ( 'NONE',  ( 103.1631342820178929, -29.09950819311272951, 119.8752769709339816 ) ) ;
#30976=CARTESIAN_POINT ( 'NONE',  ( 107.6091449839925929, -48.61785814739364042, 42.61276813305398292 ) ) ;
#30978=ORIENTED_EDGE ( 'NONE', *, *, #3130, .T. ) ;
#30980=DIRECTION ( 'NONE',  ( 1.000000000000000000, -5.337610695313248426E-16, 0.000000000000000000 ) ) ;
#30981=ORIENTED_EDGE ( 'NONE', *, *, #14644, .T. ) ;
#30983=CARTESIAN_POINT ( 'NONE',  ( 105.7145878461457187, -46.72372356240133939, 32.46910694999912295 ) ) ;
#30984=PLANE ( 'NONE',  #67830 ) ;
#30985=CIRCLE ( 'NONE', #65796, 2.750000000000002665 ) ;
#30987=CARTESIAN_POINT ( 'NONE',  ( 172.5664832912728457, -27.82844715994070484, 201.9256252759119832 ) ) ;
#30988=ORIENTED_EDGE ( 'NONE', *, *, #39118, .F. ) ;
#30989=CARTESIAN_POINT ( 'NONE',  ( 101.0865414634836696, -45.26919196907830667, 282.0899109901967563 ) ) ;
#30990=CARTESIAN_POINT ( 'NONE',  ( 104.6388127410885005, -47.56014030727299513, 23.38895860924494841 ) ) ;
#30992=LINE ( 'NONE', #50985, #53183 ) ;
#30993=DIRECTION ( 'NONE',  ( 0.7071067811865483499, 0.7071067811865466846, 7.071067811865491110E-16 ) ) ;
#30996=DIRECTION ( 'NONE',  ( 0.000000000000000000, 0.000000000000000000, -1.000000000000000000 ) ) ;
#30997=CARTESIAN_POINT ( 'NONE',  ( 131.4241199117880114, -37.49143581486269738, 6.902478035881958185 ) ) ;
#30998=CARTESIAN_POINT ( 'NONE',  ( 156.5667039024485803, -48.82844715993568485, 137.2178068554149775 ) ) ;
#31000=FACE_OUTER_BOUND ( 'NONE', #29843, .T. ) ;
#31001=CARTESIAN_POINT ( 'NONE',  ( 105.3130012014428445, -26.40811315510063295, 15.20991099019697401 ) ) ;
#31002=CARTESIAN_POINT ( 'NONE',  ( 101.9845378472182773, -45.87248622144053911, 183.1727681330539781 ) ) ;
#31003=CARTESIAN_POINT ( 'NONE',  ( 118.7569292017688696, -34.64240976163905827, 44.96705384733895272 ) ) ;
#31004=FACE_BOUND ( 'NONE', #67677, .T. ) ;
#31005=CARTESIAN_POINT ( 'NONE',  ( 108.3334480975946974, -46.73485935361659926, 47.67729194278742000 ) ) ;
#31006=CARTESIAN_POINT ( 'NONE',  ( 80.25489464535191075, -33.97944715994105991, 1.625625275910944634 ) ) ;
#31007=AXIS2_PLACEMENT_3D ( 'NONE', #34503, #62213, #83130 ) ;
#31008=CIRCLE ( 'NONE', #33862, 3.250000000000002665 ) ;
#31009=ORIENTED_EDGE ( 'NONE', *, *, #38150, .F. ) ;
#31010=EDGE_CURVE ( 'NONE', #89279, #81541, #9836, .T. ) ;
#31011=CARTESIAN_POINT ( 'NONE',  ( 113.2454987153061694, -28.75867295907008270, 185.5522919408021494 ) ) ;
#31012=ORIENTED_EDGE ( 'NONE', *, *, #82221, .T. ) ;
#31014=CARTESIAN_POINT ( 'NONE',  ( 106.6854394624702849, -26.95610377642496758, 81.10705384733896040 ) ) ;
#31015=FACE_OUTER_BOUND ( 'NONE', #58086, .T. ) ;
#31020=CARTESIAN_POINT ( 'NONE',  ( 113.1426608820137716, -26.58408993604434301, 200.6470538473399756 ) ) ;
#31022=CARTESIAN_POINT ( 'NONE',  ( 110.8542472415531250, -45.98432934487685486, 147.8856059545649941 ) ) ;
#31027=CARTESIAN_POINT ( 'NONE',  ( 117.0956141847452869, -37.54243412410453118, 98.76173397921864705 ) ) ;
#31028=CARTESIAN_POINT ( 'NONE',  ( 98.40655050692420502, -32.18313002855524729, 135.9413395616259947 ) ) ;
#31029=ORIENTED_EDGE ( 'NONE', *, *, #64625, .F. ) ;
#31031=CARTESIAN_POINT ( 'NONE',  ( 106.7212481586559392, -27.87455634666363835, 81.53872616303998200 ) ) ;
#31032=ADVANCED_FACE ( 'NONE', ( #3459, #85705 ), #23031, .F. ) ;
#31033=FACE_OUTER_BOUND ( 'NONE', #13276, .T. ) ;
#31034=CARTESIAN_POINT ( 'NONE',  ( 109.7813264909552231, -47.51098736074720108, 238.7727681330529776 ) ) ;
#31035=CARTESIAN_POINT ( 'NONE',  ( 172.5664832912729878, -27.57844715994070484, 75.92562527591199739 ) ) ;
#31037=CARTESIAN_POINT ( 'NONE',  ( 49.21213752015889042, -29.73316016639542880, 117.4678068554150485 ) ) ;
#31039=CARTESIAN_POINT ( 'NONE',  ( 21.03715912545739641, -47.82818131006197149, 180.4678068554150911 ) ) ;
#31040=CARTESIAN_POINT ( 'NONE',  ( 80.06648329127399677, 0.2215528400590013880, 7.443125275912000127 ) ) ;
#31042=LINE ( 'NONE', #59181, #85044 ) ;
#31043=CARTESIAN_POINT ( 'NONE',  ( 113.5515132932711566, -44.90922781482916548, 168.1099109901969939 ) ) ;
#31044=ORIENTED_EDGE ( 'NONE', *, *, #61673, .T. ) ;
#31045=EDGE_LOOP ( 'NONE', ( #45838, #47815, #58833, #50448 ) ) ;
#31047=CARTESIAN_POINT ( 'NONE',  ( 98.34985896447652465, -31.65658472180727401, 151.9064586012064808 ) ) ;
#31048=CARTESIAN_POINT ( 'NONE',  ( 194.5667039024482108, -40.82844715993405060, 180.4678068554150343 ) ) ;
#31049=CARTESIAN_POINT ( 'NONE',  ( 97.92310363649473004, -40.78041284545158618, 102.6583543547307329 ) ) ;
#31050=CARTESIAN_POINT ( 'NONE',  ( 101.9936049672545550, -45.44606238681409138, 268.1564571553904557 ) ) ;
#31052=CARTESIAN_POINT ( 'NONE',  ( 117.2917222856570447, -34.52255020207628888, 183.9956252759109532 ) ) ;
#31053=CARTESIAN_POINT ( 'NONE',  ( 63.56670390244796920, -40.82844715994016127, 300.4678068554150627 ) ) ;
#31054=ORIENTED_EDGE ( 'NONE', *, *, #46931, .T. ) ;
#31057=CARTESIAN_POINT ( 'NONE',  ( 114.1612546374381907, -43.81239283379284899, 64.20290172889339431 ) ) ;
#31058=CARTESIAN_POINT ( 'NONE',  ( 51.56670390244760682, -32.29483332968564469, 313.9678068554150059 ) ) ;
#31060=CARTESIAN_POINT ( 'NONE',  ( 101.1777422249941338, -43.35145646725580804, 263.4301547344683740 ) ) ;
#31062=ORIENTED_EDGE ( 'NONE', *, *, #58382, .T. ) ;
#31063=ADVANCED_FACE ( 'NONE', ( #66116 ), #8952, .T. ) ;
#31064=CARTESIAN_POINT ( 'NONE',  ( 116.2888956068410522, -39.44798389054702170, 9.635625275910941312 ) ) ;
#31068=CIRCLE ( 'NONE', #23832, 15.99999999999999822 ) ;
#31069=CIRCLE ( 'NONE', #24025, 3.250000000000002665 ) ;
#31070=CARTESIAN_POINT ( 'NONE',  ( 113.6434775417805554, -44.29062971714213148, 113.1460879784515896 ) ) ;
#31071=AXIS2_PLACEMENT_3D ( 'NONE', #2824, #18554, #47585 ) ;
#31072=ORIENTED_EDGE ( 'NONE', *, *, #74640, .F. ) ;
#31073=ORIENTED_EDGE ( 'NONE', *, *, #5444, .F. ) ;
#31075=CIRCLE ( 'NONE', #73089, 2.517500000000000071 ) ;
#31076=CARTESIAN_POINT ( 'NONE',  ( 106.6898958108015307, -27.68119582636871456, 39.52003887569599527 ) ) ;
#31077=VECTOR ( 'NONE', #67967, 1000.000000000000000 ) ;
#31078=CARTESIAN_POINT ( 'NONE',  ( 112.2159804458396479, -45.81949903116512246, 212.9870538473389558 ) ) ;
#31079=CARTESIAN_POINT ( 'NONE',  ( 107.6517678568360594, -47.10594642807022581, 152.6213395616249500 ) ) ;
#31081=CARTESIAN_POINT ( 'NONE',  ( 95.23138046818854718, -37.33356364299761054, 267.3670538473395482 ) ) ;
#31084=VERTEX_POINT ( 'NONE', #72511 ) ;
#31085=EDGE_LOOP ( 'NONE', ( #63550, #87615, #83282, #28153, #71511 ) ) ;
#31087=CARTESIAN_POINT ( 'NONE',  ( 97.36106687025375095, -40.65520290104787904, 206.6327681330539860 ) ) ;
#31088=ORIENTED_EDGE ( 'NONE', *, *, #10674, .F. ) ;
#31089=CARTESIAN_POINT ( 'NONE',  ( 113.5652313304969567, -44.92653082429684730, 168.1099109901969939 ) ) ;
#31090=CARTESIAN_POINT ( 'NONE',  ( 112.1380301846104146, -28.01206920713002191, 264.6564718616416485 ) ) ;
#31091=FACE_BOUND ( 'NONE', #66150, .T. ) ;
#31092=CARTESIAN_POINT ( 'NONE',  ( 83.56670559755357885, -33.43837296219067667, 249.5838068554176630 ) ) ;
#31096=CARTESIAN_POINT ( 'NONE',  ( 96.93559702949583823, -34.21358363697174099, 272.1327681330538439 ) ) ;
#31098=DIRECTION ( 'NONE',  ( -0.0001713722456133526934, 0.9999999853157766072, 0.000000000000000000 ) ) ;
#31099=DIRECTION ( 'NONE',  ( 1.000000000000000078E-15, 0.000000000000000000, 1.000000000000000000 ) ) ;
#31102=FACE_OUTER_BOUND ( 'NONE', #82043, .T. ) ;
#31103=CARTESIAN_POINT ( 'NONE',  ( 111.2166545661128652, -43.61238145012286083, 195.5838068554168672 ) ) ;
#31105=CARTESIAN_POINT ( 'NONE',  ( 84.06648329127399677, -18.82844715994099971, 17.92562527591199739 ) ) ;
#31106=CARTESIAN_POINT ( 'NONE',  ( 117.4484615961127218, -30.96329225543088270, 179.2299109901959753 ) ) ;
#31107=CARTESIAN_POINT ( 'NONE',  ( 109.9110140596799425, -46.79572638734455126, 68.79562527591099297 ) ) ;
#31108=CARTESIAN_POINT ( 'NONE',  ( 116.9665165100108908, -41.74809644303882550, 244.4651490854349731 ) ) ;
#31110=CARTESIAN_POINT ( 'NONE',  ( 41.56670390244695312, -36.32844715994109208, 129.9678068554150911 ) ) ;
#31114=DIRECTION ( 'NONE',  ( -0.000000000000000000, 1.000000000000000000, 0.000000000000000000 ) ) ;
#31117=( BOUNDED_CURVE ( )  B_SPLINE_CURVE ( 3, ( #37732, #51771, #9575, #23230 ),
 .UNSPECIFIED., .F., .T. ) 
 B_SPLINE_CURVE_WITH_KNOTS ( ( 4, 4 ),
 ( 1.570796326780094843, 3.141592653577910621 ),
 .UNSPECIFIED. ) 
 CURVE ( )  GEOMETRIC_REPRESENTATION_ITEM ( )  RATIONAL_B_SPLINE_CURVE ( ( 1.000000000000000000, 0.8047378541236769323, 0.8047378541236769323, 1.000000000000000000 ) ) 
 REPRESENTATION_ITEM ( '' )  );
#31119=EDGE_LOOP ( 'NONE', ( #38496, #25442, #48878, #68007 ) ) ;
#31120=VERTEX_POINT ( 'NONE', #23916 ) ;
#31122=CARTESIAN_POINT ( 'NONE',  ( 103.7110576214454341, -44.58420688232069296, 91.67813411379100330 ) ) ;
#31124=ORIENTED_EDGE ( 'NONE', *, *, #30489, .T. ) ;
#31126=CARTESIAN_POINT ( 'NONE',  ( 104.2200364793041700, -25.25138339198311144, 86.26991099019699050 ) ) ;
#31128=EDGE_CURVE ( 'NONE', #62792, #26105, #4801, .T. ) ;
#31130=CARTESIAN_POINT ( 'NONE',  ( 41.56648329127499153, -32.07844715994070839, 134.1756252759119832 ) ) ;
#31132=CARTESIAN_POINT ( 'NONE',  ( 101.7353989658528661, -28.52926574610319932, 25.53562527591096654 ) ) ;
#31134=ORIENTED_EDGE ( 'NONE', *, *, #66383, .F. ) ;
#31135=ORIENTED_EDGE ( 'NONE', *, *, #60949, .T. ) ;
#31136=CYLINDRICAL_SURFACE ( 'NONE', #87750, 2.500000000000002220 ) ;
#31137=CIRCLE ( 'NONE', #81930, 16.00000000000090239 ) ;
#31138=CARTESIAN_POINT ( 'NONE',  ( 107.0664832912748068, -36.72944715993923381, -4.074374724089028454 ) ) ;
#31139=CARTESIAN_POINT ( 'NONE',  ( 98.34985891665434110, -31.65658480256832519, 116.9064586086046376 ) ) ;
#31144=EDGE_CURVE ( 'NONE', #42921, #34489, #27869, .T. ) ;
#31145=VECTOR ( 'NONE', #73777, 1000.000000000000000 ) ;
#31146=CARTESIAN_POINT ( 'NONE',  ( 41.56648329127398966, -27.82844715994070484, 315.9256252759120116 ) ) ;
#31149=CARTESIAN_POINT ( 'NONE',  ( 101.1541078795467996, -28.12664281037970682, 50.55562527591095545 ) ) ;
#31151=EDGE_LOOP ( 'NONE', ( #78104, #24665, #29684, #11069, #64776 ) ) ;
#31155=CARTESIAN_POINT ( 'NONE',  ( 111.9717725103620722, -43.25385221418022752, 140.9080903695919460 ) ) ;
#31156=AXIS2_PLACEMENT_3D ( 'NONE', #88759, #74230, #82401 ) ;
#31159=EDGE_LOOP ( 'NONE', ( #56171, #24391, #64437, #31608 ) ) ;
#31161=VERTEX_POINT ( 'NONE', #33396 ) ;
#31162=ORIENTED_EDGE ( 'NONE', *, *, #45145, .T. ) ;
#31163=LINE ( 'NONE', #46568, #20190 ) ;
#31164=CARTESIAN_POINT ( 'NONE',  ( 117.1060311394199402, -37.55296641157723769, 185.1930118773259437 ) ) ;
#31165=CARTESIAN_POINT ( 'NONE',  ( 135.9998166246059839, 12.92155284005730387, 355.9756252759109998 ) ) ;
#31167=CARTESIAN_POINT ( 'NONE',  ( 107.0664832912739399, -36.72944715994095333, 311.6356252759109680 ) ) ;
#31168=CARTESIAN_POINT ( 'NONE',  ( 99.50480724682302025, -43.30587341447913019, 16.89607863635162488 ) ) ;
#31169=ORIENTED_EDGE ( 'NONE', *, *, #38012, .T. ) ;
#31170=CIRCLE ( 'NONE', #71794, 3.250000000000002665 ) ;
#31171=ORIENTED_EDGE ( 'NONE', *, *, #5909, .T. ) ;
#31172=ORIENTED_EDGE ( 'NONE', *, *, #25584, .T. ) ;
#31174=CARTESIAN_POINT ( 'NONE',  ( 102.6495774910181780, -44.17201850306531696, 204.9804713219729706 ) ) ;
#31175=CARTESIAN_POINT ( 'NONE',  ( 96.90545716317438973, -39.15842060370329847, 56.51276813305394597 ) ) ;
#31176=CARTESIAN_POINT ( 'NONE',  ( 115.6551466294303623, -43.65033472170377138, 43.27467289495795200 ) ) ;
#31177=DIRECTION ( 'NONE',  ( 9.351236661543306751E-17, -3.725950533538267725E-29, -1.000000000000000000 ) ) ;
#31178=FACE_BOUND ( 'NONE', #80996, .T. ) ;
#31180=CARTESIAN_POINT ( 'NONE',  ( 114.1750726078950890, -45.19361863149571690, 144.1203871806729637 ) ) ;
#31181=DIRECTION ( 'NONE',  ( 1.000000000000000078E-15, 0.000000000000000000, 1.000000000000000000 ) ) ;
#31182=VERTEX_POINT ( 'NONE', #61097 ) ;
#31185=DIRECTION ( 'NONE',  ( 0.7071067811862258301, -0.7071067811868692043, 7.071067811862265655E-16 ) ) ;
#31187=EDGE_LOOP ( 'NONE', ( #15008, #46776, #74650, #4362 ) ) ;
#31188=CIRCLE ( 'NONE', #80556, 1.000000000000000888 ) ;
#31189=DIRECTION ( 'NONE',  ( 0.000000000000000000, -1.000000000000000000, 0.000000000000000000 ) ) ;
#31190=EDGE_CURVE ( 'NONE', #3872, #37614, #26142, .T. ) ;
#31191=AXIS2_PLACEMENT_3D ( 'NONE', #66305, #43630, #31793 ) ;
#31193=DIRECTION ( 'NONE',  ( 0.000000000000000000, 0.000000000000000000, 1.000000000000000000 ) ) ;
#31194=CARTESIAN_POINT ( 'NONE',  ( 109.6430426817424433, -46.83134659365198615, 47.77562527591094721 ) ) ;
#31197=CARTESIAN_POINT ( 'NONE',  ( 25.56670390244797275, -48.82844715994099971, 173.2178068554149775 ) ) ;
#31199=CARTESIAN_POINT ( 'NONE',  ( 104.9021620152489191, -46.26774620671726268, 72.39848241876894974 ) ) ;
#31201=CARTESIAN_POINT ( 'NONE',  ( 117.3921119255896599, -35.46056622170122807, 189.9241967044829664 ) ) ;
#31202=CARTESIAN_POINT ( 'NONE',  ( 48.86082318535585500, -35.55794170701788204, 193.9678068554150911 ) ) ;
#31204=ORIENTED_EDGE ( 'NONE', *, *, #86122, .F. ) ;
#31205=PLANE ( 'NONE',  #77351 ) ;
#31208=CARTESIAN_POINT ( 'NONE',  ( 97.75871328428027596, -40.38572213467175231, 136.6247029066429377 ) ) ;
#31209=VECTOR ( 'NONE', #16287, 1000.000000000000000 ) ;
#31211=CARTESIAN_POINT ( 'NONE',  ( 172.5664832912740110, -18.82844715994099971, 198.9256252759119832 ) ) ;
#31212=CARTESIAN_POINT ( 'NONE',  ( 96.07878916947804271, -35.15354693665655361, 226.2251490854349640 ) ) ;
#31213=EDGE_LOOP ( 'NONE', ( #86268, #68583, #44777, #75892 ) ) ;
#31214=DIRECTION ( 'NONE',  ( 0.000000000000000000, 0.000000000000000000, -1.000000000000000000 ) ) ;
#31215=CARTESIAN_POINT ( 'NONE',  ( 111.1359251431956210, -27.10775802199072970, 240.7584824187679544 ) ) ;
#31216=CARTESIAN_POINT ( 'NONE',  ( 111.8139374584311554, -25.81739915606283375, 130.7499109901969518 ) ) ;
#31218=CARTESIAN_POINT ( 'NONE',  ( 82.81519967300334883, -36.82419990104791196, 6.751707299519725147 ) ) ;
#31219=CIRCLE ( 'NONE', #48573, 3.250000000000002665 ) ;
#31221=DIRECTION ( 'NONE',  ( 3.999999999999999995E-14, -1.000000000000000000, 4.100000000000000342E-29 ) ) ;
#31222=ORIENTED_EDGE ( 'NONE', *, *, #76871, .T. ) ;
#31224=ORIENTED_EDGE ( 'NONE', *, *, #9184, .F. ) ;
#31225=EDGE_LOOP ( 'NONE', ( #57342, #3206, #59125, #88114 ) ) ;
#31227=CARTESIAN_POINT ( 'NONE',  ( 99.04406184532244595, -42.84125762267669302, 71.84395860752657370 ) ) ;
#31228=CARTESIAN_POINT ( 'NONE',  ( 99.33320739591177073, -28.83195234130426243, 266.7051490854347549 ) ) ;
#31229=CARTESIAN_POINT ( 'NONE',  ( 188.5667039024479834, -48.82844715994099971, 259.9678068554150059 ) ) ;
#31230=CARTESIAN_POINT ( 'NONE',  ( 131.3834856945509841, -36.12003772029553517, 3.004064388422954313 ) ) ;
#31231=ADVANCED_FACE ( 'NONE', ( #61533 ), #12965, .F. ) ;
#31232=CARTESIAN_POINT ( 'NONE',  ( 97.81169150544869240, -40.51741169384158781, 71.63577594787710723 ) ) ;
#31234=CARTESIAN_POINT ( 'NONE',  ( 102.3821975904229333, -44.47993990548584975, 201.5543245899819738 ) ) ;
#31235=ORIENTED_EDGE ( 'NONE', *, *, #33941, .F. ) ;
#31236=ORIENTED_EDGE ( 'NONE', *, *, #60728, .F. ) ;
#31237=AXIS2_PLACEMENT_3D ( 'NONE', #65268, #80252, #86612 ) ;
#31238=VERTEX_POINT ( 'NONE', #25231 ) ;
#31239=CARTESIAN_POINT ( 'NONE',  ( 31.78666935232950408, -29.62846900982343001, 313.9678068554150059 ) ) ;
#31241=CARTESIAN_POINT ( 'NONE',  ( 57.56670390244732260, -42.82844715994040996, 175.7178068554150911 ) ) ;
#31242=DIRECTION ( 'NONE',  ( 0.7071067811866377228, -0.7071067811864573116, 0.000000000000000000 ) ) ;
#31243=CARTESIAN_POINT ( 'NONE',  ( 114.3297541623348224, -29.74979092151301074, 35.86729759161094933 ) ) ;
#31245=ADVANCED_FACE ( 'NONE', ( #87475 ), #4356, .T. ) ;
#31246=CARTESIAN_POINT ( 'NONE',  ( 116.3212776292296127, -32.94146857471318413, 249.5838068554167535 ) ) ;
#31248=DIRECTION ( 'NONE',  ( 0.9999999853157766072, 0.0001713722456143218888, 0.000000000000000000 ) ) ;
#31250=CARTESIAN_POINT ( 'NONE',  ( 97.12559044764091709, -37.99707808599399783, 57.42728215261879399 ) ) ;
#31251=ORIENTED_EDGE ( 'NONE', *, *, #30863, .T. ) ;
#31253=CARTESIAN_POINT ( 'NONE',  ( 116.6500553765360451, -33.62673909641207359, 280.5072975916113478 ) ) ;
#31257=CARTESIAN_POINT ( 'NONE',  ( 136.7925547069177128, -18.36732994130890262, 6.785344856282517156 ) ) ;
#31259=DIRECTION ( 'NONE',  ( 0.000000000000000000, 1.000000000000000000, 0.000000000000000000 ) ) ;
#31260=DIRECTION ( 'NONE',  ( 0.7071067811868696484, 0.7071067811862253860, 7.071067811869001541E-16 ) ) ;
#31263=DIRECTION ( 'NONE',  ( 0.000000000000000000, 0.000000000000000000, 1.000000000000000000 ) ) ;
#31265=VERTEX_POINT ( 'NONE', #46105 ) ;
#31266=CARTESIAN_POINT ( 'NONE',  ( 99.05404782812107101, -43.39937282746017644, 116.8784824187679732 ) ) ;
#31267=ORIENTED_EDGE ( 'NONE', *, *, #54579, .T. ) ;
#31268=CARTESIAN_POINT ( 'NONE',  ( 98.58513254605244924, -37.74079342042374918, 40.84384839950494239 ) ) ;
#31271=CARTESIAN_POINT ( 'NONE',  ( 109.4844142153598057, -45.28606679814626546, 69.22729759161194352 ) ) ;
#31272=CARTESIAN_POINT ( 'NONE',  ( 112.0649019730212643, -45.48895927759898683, 13.98970061351897343 ) ) ;
#31273=DIRECTION ( 'NONE',  ( 1.000000000000000000, 0.000000000000000000, 9.868649107779159826E-16 ) ) ;
#31275=AXIS2_PLACEMENT_3D ( 'NONE', #42625, #13161, #14051 ) ;
#31276=CARTESIAN_POINT ( 'NONE',  ( 114.8356066511136504, -43.71357066064707197, 34.24419670448197905 ) ) ;
#31279=DIRECTION ( 'NONE',  ( -0.7071067811864671926, -0.7071067811866279529, 2.899137802865059124E-29 ) ) ;
#31281=DIRECTION ( 'NONE',  ( 0.7071067811868710917, -0.7071067811862240537, 0.000000000000000000 ) ) ;
#31283=VECTOR ( 'NONE', #63187, 1000.000000000000000 ) ;
#31284=ORIENTED_EDGE ( 'NONE', *, *, #55580, .T. ) ;
#31286=CYLINDRICAL_SURFACE ( 'NONE', #17407, 3.299999999999997158 ) ;
#31287=CARTESIAN_POINT ( 'NONE',  ( 117.3720538532507618, -35.57445771113444977, 233.9032443235299752 ) ) ;
#31290=CARTESIAN_POINT ( 'NONE',  ( 107.6068523407233926, -48.56763185392661342, 38.61276813305397582 ) ) ;
#31291=CARTESIAN_POINT ( 'NONE',  ( 97.81825285133052716, -40.53342921643464081, 42.63700214333596250 ) ) ;
#31293=CARTESIAN_POINT ( 'NONE',  ( 97.80396622205201140, -40.49851628999532949, 172.6339998519910637 ) ) ;
#31295=ORIENTED_EDGE ( 'NONE', *, *, #32765, .F. ) ;
#31298=CYLINDRICAL_SURFACE ( 'NONE', #81779, 1.000000000002049694 ) ;
#31299=CARTESIAN_POINT ( 'NONE',  ( 111.1189502094635202, -27.14789314160929479, 244.7584824187679544 ) ) ;
#31300=AXIS2_PLACEMENT_3D ( 'NONE', #39329, #87048, #67477 ) ;
#31304=CARTESIAN_POINT ( 'NONE',  ( 98.30761769748181678, -41.72907704524488537, 91.73956018709316140 ) ) ;
#31305=CARTESIAN_POINT ( 'NONE',  ( 114.8253727231603136, -41.39981172478538696, 277.8057531614101663 ) ) ;
#31307=CARTESIAN_POINT ( 'NONE',  ( 117.5733473178507467, -42.15660255127702527, 89.44705384733997278 ) ) ;
#31309=CARTESIAN_POINT ( 'NONE',  ( 99.65330034922125435, -46.03930839343899351, 122.0413395616249659 ) ) ;
#31310=VERTEX_POINT ( 'NONE', #20226 ) ;
#31311=CARTESIAN_POINT ( 'NONE',  ( 132.2129280580766135, -20.76093376057972861, 7.655955902696334192 ) ) ;
#31316=CYLINDRICAL_SURFACE ( 'NONE', #61580, 3.000000000000002665 ) ;
#31317=ORIENTED_EDGE ( 'NONE', *, *, #61869, .T. ) ;
#31321=CARTESIAN_POINT ( 'NONE',  ( 107.9493508131109962, -25.66448314884807047, 115.0251490854349612 ) ) ;
#31322=ORIENTED_EDGE ( 'NONE', *, *, #51347, .T. ) ;
#31323=DIRECTION ( 'NONE',  ( 0.7071067812158990940, 0.7071067811571960515, 0.000000000000000000 ) ) ;
#31328=ORIENTED_EDGE ( 'NONE', *, *, #61982, .F. ) ;
#31329=CARTESIAN_POINT ( 'NONE',  ( 116.6186327310674500, -29.67321183330947321, 109.3327681330539605 ) ) ;
#31331=AXIS2_PLACEMENT_3D ( 'NONE', #97, #55024, #69589 ) ;
#31332=( NAMED_UNIT ( * ) SI_UNIT ( $, .STERADIAN. ) SOLID_ANGLE_UNIT ( ) );
#31333=CIRCLE ( 'NONE', #82132, 13.49999999999999822 ) ;
#31334=ADVANCED_FACE ( 'NONE', ( #28365 ), #61986, .T. ) ;
#31336=CARTESIAN_POINT ( 'NONE',  ( 137.8897065959775716, -5.906223855237799469, 14.67562527591100263 ) ) ;
#31337=DIRECTION ( 'NONE',  ( 0.000000000000000000, 0.000000000000000000, 1.000000000000000000 ) ) ;
#31339=ORIENTED_EDGE ( 'NONE', *, *, #43528, .T. ) ;
#31341=FACE_OUTER_BOUND ( 'NONE', #88202, .T. ) ;
#31344=CARTESIAN_POINT ( 'NONE',  ( 40.31648329127400388, 12.92155284005802507, 349.2756252759108406 ) ) ;
#31346=DIRECTION ( 'NONE',  ( 0.000000000000000000, 0.000000000000000000, -1.000000000000000000 ) ) ;
#31349=ORIENTED_EDGE ( 'NONE', *, *, #45748, .F. ) ;
#31351=DIRECTION ( 'NONE',  ( 0.000000000000000000, 1.000000000000000000, 0.000000000000000000 ) ) ;
#31352=CARTESIAN_POINT ( 'NONE',  ( 96.59955023297828802, -32.98040794253982000, 172.0527681330529788 ) ) ;
#31355=EDGE_CURVE ( 'NONE', #87708, #16685, #11996, .T. ) ;
#31356=CARTESIAN_POINT ( 'NONE',  ( 97.95204982468537480, -33.09064556074058316, 37.02419670448192335 ) ) ;
#31357=CARTESIAN_POINT ( 'NONE',  ( 97.81362140459485488, -40.52214454336083094, 51.63603076018934956 ) ) ;
#31359=DIRECTION ( 'NONE',  ( 1.000000000000000000, 4.237773401492740281E-14, 0.000000000000000000 ) ) ;
#31360=EDGE_CURVE ( 'NONE', #68501, #28780, #67100, .T. ) ;
#31361=ORIENTED_EDGE ( 'NONE', *, *, #23271, .T. ) ;
#31366=CARTESIAN_POINT ( 'NONE',  ( 116.3165111044169038, -35.08217335353153743, 195.3863452106589875 ) ) ;
#31367=CARTESIAN_POINT ( 'NONE',  ( 182.3467384525650061, -36.02818131005800950, -5.074374724088000832 ) ) ;
#31369=CARTESIAN_POINT ( 'NONE',  ( 151.0371591254575208, -24.42818131005592264, 180.4678068554149775 ) ) ;
#31371=ORIENTED_EDGE ( 'NONE', *, *, #37585, .F. ) ;
#31373=CARTESIAN_POINT ( 'NONE',  ( 151.0371591254575208, -24.42818131005592264, 193.9678068554149775 ) ) ;
#31374=ORIENTED_EDGE ( 'NONE', *, *, #89162, .F. ) ;
#31375=CARTESIAN_POINT ( 'NONE',  ( 111.5990003564989905, -46.09347164638234062, 247.9356252759109509 ) ) ;
#31378=CARTESIAN_POINT ( 'NONE',  ( 117.0608945233188507, -38.08045312314173003, 83.71895860905850384 ) ) ;
#31383=CARTESIAN_POINT ( 'NONE',  ( 114.1542194384027908, -29.02509929289194801, 195.4841967044819739 ) ) ;
#31385=VERTEX_POINT ( 'NONE', #55149 ) ;
#31386=AXIS2_PLACEMENT_3D ( 'NONE', #67977, #6208, #28426 ) ;
#31387=CARTESIAN_POINT ( 'NONE',  ( 107.1959371850970086, -26.26158102413311468, 31.06705384733893283 ) ) ;
#31388=VECTOR ( 'NONE', #12061, 1000.000000000000000 ) ;
#31390=CARTESIAN_POINT ( 'NONE',  ( 111.8641478345923019, -46.02505481121716002, 272.9556252759110180 ) ) ;
#31392=CARTESIAN_POINT ( 'NONE',  ( 81.48703104220281546, -16.36767655967523893, 1.942446731261492143 ) ) ;
#31393=CARTESIAN_POINT ( 'NONE',  ( 112.0670051061717771, -45.48779079837375861, 18.99044305992054760 ) ) ;
#31394=CARTESIAN_POINT ( 'NONE',  ( 104.4067584314151134, -46.45769567148069967, 152.3653096109091791 ) ) ;
#31395=CARTESIAN_POINT ( 'NONE',  ( 99.83919217201646745, -32.93524248800951426, 133.7595189410199623 ) ) ;
#31396=CARTESIAN_POINT ( 'NONE',  ( 112.4229354917722787, -46.42447813297522430, 248.9661014663869878 ) ) ;
#31397=CARTESIAN_POINT ( 'NONE',  ( 80.06648329127399677, 0.2215528400590013880, 296.1531252759119752 ) ) ;
#31398=ORIENTED_EDGE ( 'NONE', *, *, #37695, .T. ) ;
#31399=CARTESIAN_POINT ( 'NONE',  ( 135.4847699230674323, -39.08750326150417465, 1.944748881531143336 ) ) ;
#31400=VERTEX_POINT ( 'NONE', #84257 ) ;
#31401=ORIENTED_EDGE ( 'NONE', *, *, #13757, .T. ) ;
#31402=DIRECTION ( 'NONE',  ( 5.512527431108029424E-15, -1.000000000000000000, 0.000000000000000000 ) ) ;
#31405=CYLINDRICAL_SURFACE ( 'NONE', #67167, 0.9999999999999731326 ) ;
#31406=DIRECTION ( 'NONE',  ( 1.000000000000000078E-15, -1.000000000000000000, 0.000000000000000000 ) ) ;
#31408=LINE ( 'NONE', #24610, #18480 ) ;
#31409=CARTESIAN_POINT ( 'NONE',  ( 111.2069583914694419, -45.51165039160690640, 137.3495626852199507 ) ) ;
#31410=CARTESIAN_POINT ( 'NONE',  ( 104.7257947241298979, -47.57997989614905521, 32.41943479972098174 ) ) ;
#31412=EDGE_CURVE ( 'NONE', #53911, #85068, #68816, .T. ) ;
#31413=CARTESIAN_POINT ( 'NONE',  ( 176.7738106836355314, -48.62134037874481152, 180.4678068554150059 ) ) ;
#31416=ADVANCED_FACE ( 'NONE', ( #69263 ), #43882, .T. ) ;
#31417=CARTESIAN_POINT ( 'NONE',  ( 90.44969454456408187, -50.04645651782490745, 239.5838068554174356 ) ) ;
#31419=DIRECTION ( 'NONE',  ( 1.000000000000000000, 0.000000000000000000, 0.000000000000000000 ) ) ;
#31426=CARTESIAN_POINT ( 'NONE',  ( 105.3166869522846838, -26.42980843014500181, 15.20991099019697401 ) ) ;
#31427=CARTESIAN_POINT ( 'NONE',  ( 102.7372881883638058, -25.64480981559214712, 16.37276813305293999 ) ) ;
#31428=EDGE_CURVE ( 'NONE', #18839, #8744, #14308, .T. ) ;
#31430=DIRECTION ( 'NONE',  ( 0.000000000000000000, 1.000000000000000000, 1.914177628664063178E-15 ) ) ;
#31431=DIRECTION ( 'NONE',  ( 0.000000000000000000, 0.000000000000000000, -1.000000000000000000 ) ) ;
#31432=LINE ( 'NONE', #59132, #19329 ) ;
#31433=FACE_OUTER_BOUND ( 'NONE', #46690, .T. ) ;
#31434=CARTESIAN_POINT ( 'NONE',  ( 51.34673845256598668, -36.02818131005800950, -5.074374724088000832 ) ) ;
#31436=EDGE_CURVE ( 'NONE', #5064, #65413, #35172, .T. ) ;
#31438=CARTESIAN_POINT ( 'NONE',  ( 96.95731234646120811, -39.36592712812080208, 276.5299109901967540 ) ) ;
#31439=CARTESIAN_POINT ( 'NONE',  ( 96.13817600250692408, -35.07231702426307152, 217.1946728949589840 ) ) ;
#31440=CARTESIAN_POINT ( 'NONE',  ( 105.9861696881796860, -26.33857706295247070, 46.15848241876796720 ) ) ;
#31441=AXIS2_PLACEMENT_3D ( 'NONE', #50163, #51065, #9745 ) ;
#31443=DIRECTION ( 'NONE',  ( -1.000000000000000078E-15, 1.000000000000000083E-30, 1.000000000000000000 ) ) ;
#31444=FACE_OUTER_BOUND ( 'NONE', #44311, .T. ) ;
#31445=EDGE_CURVE ( 'NONE', #61667, #53177, #18213, .T. ) ;
#31447=CIRCLE ( 'NONE', #43056, 3.300000000000000711 ) ;
#31448=ORIENTED_EDGE ( 'NONE', *, *, #46902, .F. ) ;
#31451=CARTESIAN_POINT ( 'NONE',  ( 110.2470682213182300, -46.59973918892927003, 53.83657765686300678 ) ) ;
#31455=CARTESIAN_POINT ( 'NONE',  ( 109.6005296801413067, -26.60309369064642127, 195.8813395616249977 ) ) ;
#31456=CARTESIAN_POINT ( 'NONE',  ( 99.08905494682572623, -42.79484345344285146, 252.8444919503191102 ) ) ;
#31457=FACE_OUTER_BOUND ( 'NONE', #48596, .T. ) ;
#31458=LINE ( 'NONE', #78759, #84988 ) ;
#31459=EDGE_CURVE ( 'NONE', #72895, #36690, #71957, .T. ) ;
#31460=CARTESIAN_POINT ( 'NONE',  ( 131.5565945955644622, -37.85370728022187592, 2.783021134851944911 ) ) ;
#31462=CIRCLE ( 'NONE', #32957, 2.124999999999998224 ) ;
#31464=CARTESIAN_POINT ( 'NONE',  ( 102.3899016914588458, -28.13915478247111679, 145.4727681330539610 ) ) ;
#31465=ORIENTED_EDGE ( 'NONE', *, *, #6394, .F. ) ;
#31467=CARTESIAN_POINT ( 'NONE',  ( 108.9267623252842441, -45.42435897675616019, 104.1758690201829722 ) ) ;
#31468=CLOSED_SHELL ( 'NONE', ( #89553, #33121, #71545, #20756 ) ) ;
#31469=LINE ( 'NONE', #59613, #87815 ) ;
#31470=CARTESIAN_POINT ( 'NONE',  ( 112.6571330189592430, -45.46348522128858605, 214.0175300378159591 ) ) ;
#31471=DIRECTION ( 'NONE',  ( 1.000000000000000078E-15, 0.000000000000000000, -1.000000000000000000 ) ) ;
#31476=CARTESIAN_POINT ( 'NONE',  ( 181.5667039024459939, -18.82844715994099971, -5.074374724088000832 ) ) ;
#31478=CARTESIAN_POINT ( 'NONE',  ( 117.4355769707883468, -40.49052663852281597, 173.5375300378159693 ) ) ;
#31480=ORIENTED_EDGE ( 'NONE', *, *, #26490, .T. ) ;
#31482=CARTESIAN_POINT ( 'NONE',  ( 77.38348569455060044, -18.12003772028603876, 3.004064388423441478 ) ) ;
#31483=CARTESIAN_POINT ( 'NONE',  ( 101.9936209266849119, -45.44607153056026760, 78.15645860795193300 ) ) ;
#31484=CARTESIAN_POINT ( 'NONE',  ( 184.5667039024483245, -48.82844715993448403, 300.4678068554149490 ) ) ;
#31485=VECTOR ( 'NONE', #5828, 1000.000000000000000 ) ;
#31486=VECTOR ( 'NONE', #39488, 1000.000000000000000 ) ;
#31487=EDGE_CURVE ( 'NONE', #78352, #45673, #42444, .T. ) ;
#31488=CARTESIAN_POINT ( 'NONE',  ( 113.1782861458026730, -44.75187455886691623, 269.0939578440578543 ) ) ;
#31489=CARTESIAN_POINT ( 'NONE',  ( 96.04647588134957914, -35.87007288833441976, 191.2765776568629690 ) ) ;
#31491=ORIENTED_EDGE ( 'NONE', *, *, #81916, .F. ) ;
#31492=ORIENTED_EDGE ( 'NONE', *, *, #19410, .T. ) ;
#31493=ORIENTED_EDGE ( 'NONE', *, *, #86270, .F. ) ;
#31494=CARTESIAN_POINT ( 'NONE',  ( 97.82290962912863108, -40.54474197294914717, 62.63844076402585870 ) ) ;
#31495=CARTESIAN_POINT ( 'NONE',  ( 165.6738106836030227, -28.98061976758901892, -5.074374724088000832 ) ) ;
#31497=CARTESIAN_POINT ( 'NONE',  ( 98.43690990026183840, -34.58641363334965035, 272.5644404487542829 ) ) ;
#31498=DIRECTION ( 'NONE',  ( 0.000000000000000000, 0.000000000000000000, -1.000000000000000000 ) ) ;
#31500=VECTOR ( 'NONE', #5660, 1000.000000000000000 ) ;
#31502=CARTESIAN_POINT ( 'NONE',  ( 165.9667039024452038, -28.27351298637401200, 342.9256252759109884 ) ) ;
#31503=ADVANCED_FACE ( 'NONE', ( #65130 ), #51477, .F. ) ;
#31507=VECTOR ( 'NONE', #56805, 1000.000000000000000 ) ;
#31508=AXIS2_PLACEMENT_3D ( 'NONE', #12632, #33063, #60764 ) ;
#31511=ORIENTED_EDGE ( 'NONE', *, *, #70196, .F. ) ;
#31513=CARTESIAN_POINT ( 'NONE',  ( 99.09507348882337396, -30.55127953124758378, 156.8021594390647238 ) ) ;
#31516=CARTESIAN_POINT ( 'NONE',  ( 111.1942201901869680, -30.05669425270436790, 287.4538046553057029 ) ) ;
#31517=CARTESIAN_POINT ( 'NONE',  ( 118.9025049541195358, -37.70032671045152028, 188.7613395616259595 ) ) ;
#31518=EDGE_CURVE ( 'NONE', #15446, #52251, #3797, .T. ) ;
#31519=CARTESIAN_POINT ( 'NONE',  ( 97.44537786355540732, -42.12371753947140007, 181.7451490854349743 ) ) ;
#31520=CYLINDRICAL_SURFACE ( 'NONE', #69891, 2.517500000000005844 ) ;
#31521=CARTESIAN_POINT ( 'NONE',  ( 118.1075207852818068, -36.21034067742461815, 264.8518157521014587 ) ) ;
#31522=LINE ( 'NONE', #37016, #61734 ) ;
#31523=DIRECTION ( 'NONE',  ( 0.000000000000000000, 0.000000000000000000, -1.000000000000000000 ) ) ;
#31524=ORIENTED_EDGE ( 'NONE', *, *, #87252, .T. ) ;
#31526=ADVANCED_FACE ( 'NONE', ( #77877 ), #64687, .F. ) ;
#31527=EDGE_LOOP ( 'NONE', ( #20752, #21781 ) ) ;
#31530=VECTOR ( 'NONE', #74173, 1000.000000000000000 ) ;
#31532=CARTESIAN_POINT ( 'NONE',  ( 130.3998166246070127, 12.92155284005802685, 336.5756252759110225 ) ) ;
#31533=CARTESIAN_POINT ( 'NONE',  ( 95.24515967180828113, -38.10243856675759133, 236.4184824187679510 ) ) ;
#31534=EDGE_LOOP ( 'NONE', ( #53944, #62478, #82674, #78997 ) ) ;
#31535=CARTESIAN_POINT ( 'NONE',  ( 117.1261863205049423, -33.86823216992616636, 149.0470538473389581 ) ) ;
#31536=DIRECTION ( 'NONE',  ( -0.7071067811865849873, 0.7071067811865101582, 0.000000000000000000 ) ) ;
#31542=CARTESIAN_POINT ( 'NONE',  ( 116.5166575185068467, -42.41785904284974862, 274.3832443235299365 ) ) ;
#31545=EDGE_CURVE ( 'NONE', #82808, #45317, #39538, .T. ) ;
#31546=DIRECTION ( 'NONE',  ( 0.7071067811865157093, 0.7071067811865794361, 7.071067811865148942E-16 ) ) ;
#31548=CARTESIAN_POINT ( 'NONE',  ( 123.6837132603318707, -18.85368780205705619, 218.8274735512161158 ) ) ;
#31550=CARTESIAN_POINT ( 'NONE',  ( 98.79997750155241931, -33.98483017033598941, 195.5838068554174356 ) ) ;
#31552=DIRECTION ( 'NONE',  ( 2.900000000000000265E-14, -2.000000000000000155E-15, 1.000000000000000000 ) ) ;
#31553=CARTESIAN_POINT ( 'NONE',  ( 98.41658590534017037, -29.81029140585139814, 195.7775300378159784 ) ) ;
#31554=CARTESIAN_POINT ( 'NONE',  ( 99.05421528594702352, -43.39923342774125814, 112.8784824187679732 ) ) ;
#31555=CARTESIAN_POINT ( 'NONE',  ( 99.05265045910354615, -29.93853425193624318, 211.7670538473399517 ) ) ;
#31556=DIRECTION ( 'NONE',  ( 5.512527431108029424E-15, -1.000000000000000000, 0.000000000000000000 ) ) ;
#31557=DIRECTION ( 'NONE',  ( 1.000000000000000078E-15, -1.000000000000000083E-30, -1.000000000000000000 ) ) ;
#31558=DIRECTION ( 'NONE',  ( -1.000000000000000078E-15, 1.000000000000000083E-30, 1.000000000000000000 ) ) ;
#31559=CARTESIAN_POINT ( 'NONE',  ( 107.8235642108959382, -46.74791189189382834, 38.63593913708626815 ) ) ;
#31562=CIRCLE ( 'NONE', #4006, 0.5000000000000004441 ) ;
#31563=CARTESIAN_POINT ( 'NONE',  ( 98.35024246080324417, -31.65587940141233148, 65.90773501403860735 ) ) ;
#31564=ORIENTED_EDGE ( 'NONE', *, *, #77303, .F. ) ;
#31566=CARTESIAN_POINT ( 'NONE',  ( 115.9223471279375843, -38.62321220144315248, 108.0933722090289564 ) ) ;
#31569=CARTESIAN_POINT ( 'NONE',  ( 98.16825066461163374, -43.24752039522706326, 102.8175300378159847 ) ) ;
#31570=LINE ( 'NONE', #88800, #74402 ) ;
#31571=CARTESIAN_POINT ( 'NONE',  ( 77.33253953643593093, -18.38432368373347359, 6.774690158159028641 ) ) ;
#31572=CARTESIAN_POINT ( 'NONE',  ( 97.31584370704455011, -39.30597596449835862, 177.5314586064030209 ) ) ;
#31573=AXIS2_PLACEMENT_3D ( 'NONE', #86169, #87060, #58878 ) ;
#31575=CARTESIAN_POINT ( 'NONE',  ( 97.46604185887800043, -38.76544784714115366, 31.49276813305495892 ) ) ;
#31576=ORIENTED_EDGE ( 'NONE', *, *, #60162, .T. ) ;
#31579=VECTOR ( 'NONE', #37168, 1000.000000000000000 ) ;
#31582=CARTESIAN_POINT ( 'NONE',  ( 111.5019814087853405, -26.53443175268790100, 130.7499109901969518 ) ) ;
#31583=CARTESIAN_POINT ( 'NONE',  ( 164.7830935719574939, -29.99615139351707782, 237.4678068554150059 ) ) ;
#31584=DIRECTION ( 'NONE',  ( 2.900000000000000265E-14, -2.000000000000000155E-15, 1.000000000000000000 ) ) ;
#31586=B_SPLINE_CURVE_WITH_KNOTS ( 'NONE', 3,
 ( #6474, #33737, #60074, #13300, #46889, #61873, #4693, #40989, #89607, #27365, #82355, #33290, #54144, #75072, #32374, #25572, #68708, #47791 ),
 .UNSPECIFIED., .F., .F.,
 ( 4, 2, 2, 2, 2, 2, 2, 2, 4 ),
 ( 0.000000000000000000, 0.06250874477208767654, 0.1250174895441753531, 0.1875262343162630296, 0.2500349790883507062, 0.3125437238604384382, 0.3750524686325260593, 0.4375612134046134027, 0.5000699581767007462 ),
 .UNSPECIFIED. ) ;
#31587=LINE ( 'NONE', #38849, #25698 ) ;
#31588=VECTOR ( 'NONE', #7149, 1000.000000000000000 ) ;
#31590=DIRECTION ( 'NONE',  ( -4.237773401492740281E-14, 1.000000000000000000, 0.000000000000000000 ) ) ;
#31591=CARTESIAN_POINT ( 'NONE',  ( 116.2124334422530865, -31.77159869865914388, 69.22133956162495849 ) ) ;
#31592=ORIENTED_EDGE ( 'NONE', *, *, #61363, .F. ) ;
#31596=DIRECTION ( 'NONE',  ( 0.000000000000000000, -1.000000000000000000, 0.000000000000000000 ) ) ;
#31597=AXIS2_PLACEMENT_3D ( 'NONE', #59062, #23259, #66332 ) ;
#31600=CARTESIAN_POINT ( 'NONE',  ( 112.9083776113003665, -30.34675141079074834, 152.2928522743529527 ) ) ;
#31601=VECTOR ( 'NONE', #43191, 1000.000000000000000 ) ;
#31603=DIRECTION ( 'NONE',  ( 0.000000000000000000, 0.000000000000000000, 1.000000000000000000 ) ) ;
#31604=ORIENTED_EDGE ( 'NONE', *, *, #83743, .T. ) ;
#31607=VERTEX_POINT ( 'NONE', #88275 ) ;
#31608=ORIENTED_EDGE ( 'NONE', *, *, #33842, .F. ) ;
#31609=CARTESIAN_POINT ( 'NONE',  ( 34.67381068360400320, -28.98061976758901892, -5.074374724088000832 ) ) ;
#31611=CARTESIAN_POINT ( 'NONE',  ( 106.5710281304903901, -26.66837221057895846, 191.5472975916109704 ) ) ;
#31612=FACE_OUTER_BOUND ( 'NONE', #33158, .T. ) ;
#31613=AXIS2_PLACEMENT_3D ( 'NONE', #50485, #30060, #16432 ) ;
#31614=CARTESIAN_POINT ( 'NONE',  ( 115.0889047326819536, -30.61763669310897029, 119.3439586080126276 ) ) ;
#31615=VECTOR ( 'NONE', #20184, 1000.000000000000000 ) ;
#31616=DIRECTION ( 'NONE',  ( 0.000000000000000000, 1.000000000000000000, 0.000000000000000000 ) ) ;
#31618=ORIENTED_EDGE ( 'NONE', *, *, #73381, .F. ) ;
#31621=ADVANCED_FACE ( 'NONE', ( #33291 ), #11960, .F. ) ;
#31622=CARTESIAN_POINT ( 'NONE',  ( 105.0207293620135118, -28.82725652202227096, 198.0966617981629554 ) ) ;
#31623=CARTESIAN_POINT ( 'NONE',  ( 97.91311022844104173, -31.62022761154550210, 110.9213395616259703 ) ) ;
#31624=EDGE_CURVE ( 'NONE', #25804, #3896, #35186, .T. ) ;
#31625=CARTESIAN_POINT ( 'NONE',  ( 112.8057071037347754, -27.31004523576145360, 49.62895860924498947 ) ) ;
#31628=DIRECTION ( 'NONE',  ( 0.000000000000000000, 0.000000000000000000, 1.000000000000000000 ) ) ;
#31629=EDGE_CURVE ( 'NONE', #54188, #77895, #87808, .T. ) ;
#31630=CARTESIAN_POINT ( 'NONE',  ( 117.3100215237039805, -34.79230872694400034, 154.9756252759109714 ) ) ;
#31632=VERTEX_POINT ( 'NONE', #52788 ) ;
#31633=DIRECTION ( 'NONE',  ( 1.000000000000000000, 0.000000000000000000, 0.000000000000000000 ) ) ;
#31634=VERTEX_POINT ( 'NONE', #24686 ) ;
#31637=CARTESIAN_POINT ( 'NONE',  ( 41.56648329127399677, -9.303447159940999356, 138.9256252759119832 ) ) ;
#31640=CYLINDRICAL_SURFACE ( 'NONE', #6899, 0.5000000000000129896 ) ;
#31645=CARTESIAN_POINT ( 'NONE',  ( 113.9010889189769955, -29.38240039765346978, 130.4802758126486140 ) ) ;
#31646=CARTESIAN_POINT ( 'NONE',  ( 114.3532617768494504, -44.18530993788802874, 73.19276813305397411 ) ) ;
#31647=DIRECTION ( 'NONE',  ( 1.000000000000000078E-15, -1.000000000000000000, 0.000000000000000000 ) ) ;
#31648=CARTESIAN_POINT ( 'NONE',  ( 25.56670390244797275, -62.87844715994099687, 175.9678068554150059 ) ) ;
#31650=CARTESIAN_POINT ( 'NONE',  ( 101.3216544293209864, -28.81361639883581205, 75.57562527591093726 ) ) ;
#31651=DIRECTION ( 'NONE',  ( 1.639958061481212836E-42, -4.100000000000000342E-29, -1.000000000000000000 ) ) ;
#31652=CARTESIAN_POINT ( 'NONE',  ( 114.3286968523003253, -29.23113535793739359, 170.4641967044829585 ) ) ;
#31653=DIRECTION ( 'NONE',  ( 4.299999999999999979E-14, -1.000000000000000000, 4.400000000000000367E-29 ) ) ;
#31654=DIRECTION ( 'NONE',  ( -0.7071067811865165975, -0.7071067811865784369, -7.071067811865470403E-16 ) ) ;
#31656=ORIENTED_EDGE ( 'NONE', *, *, #33079, .F. ) ;
#31658=AXIS2_PLACEMENT_3D ( 'NONE', #66003, #58312, #86039 ) ;
#31659=DIRECTION ( 'NONE',  ( 4.299999999999999979E-14, -1.000000000000000000, 0.000000000000000000 ) ) ;
#31662=CARTESIAN_POINT ( 'NONE',  ( 107.0664832912739968, -14.47844715994100007, 151.4256252759119832 ) ) ;
#31663=CARTESIAN_POINT ( 'NONE',  ( 118.8398422492546018, -38.46634565031615693, 223.7099109901969598 ) ) ;
#31664=EDGE_LOOP ( 'NONE', ( #15041, #71355, #74745, #19465, #66147 ) ) ;
#31665=LINE ( 'NONE', #18477, #62517 ) ;
#31666=CARTESIAN_POINT ( 'NONE',  ( 99.38090234834324121, -28.75341736348360655, 261.6746728949589169 ) ) ;
#31667=CARTESIAN_POINT ( 'NONE',  ( 99.65376319600918009, -46.03872712633670972, 118.0413395616259606 ) ) ;
#31668=CIRCLE ( 'NONE', #21500, 15.69999999999999929 ) ;
#31669=CARTESIAN_POINT ( 'NONE',  ( 41.56648329127399677, 0.2215528400590013880, 136.8086252759119645 ) ) ;
#31670=VECTOR ( 'NONE', #12232, 1000.000000000000000 ) ;
#31673=CARTESIAN_POINT ( 'NONE',  ( 115.0366562237703647, -42.90922531116172678, 264.3024214611318143 ) ) ;
#31675=ORIENTED_EDGE ( 'NONE', *, *, #44259, .T. ) ;
#31678=VERTEX_POINT ( 'NONE', #25573 ) ;
#31679=DIRECTION ( 'NONE',  ( -1.000000000000000000, -4.299999999999999979E-14, -1.000000000000000078E-15 ) ) ;
#31680=CARTESIAN_POINT ( 'NONE',  ( 112.3382693683599314, -28.20726497302192826, 285.6356252759109680 ) ) ;
#31682=CARTESIAN_POINT ( 'NONE',  ( 131.5238707403503042, -35.68172011937276267, 2.822018711113692735 ) ) ;
#31685=CIRCLE ( 'NONE', #28787, 2.517500000000005844 ) ;
#31686=EDGE_CURVE ( 'NONE', #11064, #55190, #60075, .T. ) ;
#31687=CARTESIAN_POINT ( 'NONE',  ( 98.11275290507195734, -35.37173493080541675, 220.6171817328389864 ) ) ;
#31689=AXIS2_PLACEMENT_3D ( 'NONE', #38116, #18111, #32180 ) ;
#31690=ORIENTED_EDGE ( 'NONE', *, *, #45450, .T. ) ;
#31691=ORIENTED_EDGE ( 'NONE', *, *, #25801, .T. ) ;
#31693=CARTESIAN_POINT ( 'NONE',  ( 99.08980160023928363, -42.79582177768785556, 181.8439945534138076 ) ) ;
#31694=EDGE_CURVE ( 'NONE', #1382, #14442, #40547, .T. ) ;
#31696=CARTESIAN_POINT ( 'NONE',  ( 101.4671292710339117, -29.18466352532158226, 32.02824997256392692 ) ) ;
#31698=DIRECTION ( 'NONE',  ( 0.000000000000000000, 0.000000000000000000, -1.000000000000000000 ) ) ;
#31699=FACE_BOUND ( 'NONE', #50873, .T. ) ;
#31700=EDGE_LOOP ( 'NONE', ( #89056, #45200, #10619, #74754 ) ) ;
#31702=CARTESIAN_POINT ( 'NONE',  ( 103.2764230263689598, -27.47550512461969774, 56.38580517588684415 ) ) ;
#31703=ORIENTED_EDGE ( 'NONE', *, *, #22526, .T. ) ;
#31704=CARTESIAN_POINT ( 'NONE',  ( 116.3136297247243078, -32.94478793390952376, 255.1356252759109395 ) ) ;
#31705=CARTESIAN_POINT ( 'NONE',  ( 109.6406350139562136, -27.81487066565610888, 62.67094751244894724 ) ) ;
#31707=AXIS2_PLACEMENT_3D ( 'NONE', #53134, #25467, #10502 ) ;
#31708=EDGE_CURVE ( 'NONE', #58445, #79084, #37560, .T. ) ;
#31709=CARTESIAN_POINT ( 'NONE',  ( 107.0664832912739968, -18.82844715994099971, 168.9256252759119832 ) ) ;
#31712=EDGE_LOOP ( 'NONE', ( #81430, #31284, #69996, #77432 ) ) ;
#31713=DIRECTION ( 'NONE',  ( 0.000000000000000000, 0.000000000000000000, 1.000000000000000000 ) ) ;
#31714=AXIS2_PLACEMENT_3D ( 'NONE', #71299, #17220, #57641 ) ;
#31715=FACE_OUTER_BOUND ( 'NONE', #24871, .T. ) ;
#31717=CARTESIAN_POINT ( 'NONE',  ( 95.48778530930356112, -34.20472165425801592, 106.1556252759109640 ) ) ;
#31719=CARTESIAN_POINT ( 'NONE',  ( 99.71754419879584930, -32.37637629707774778, 85.32384839950596245 ) ) ;
#31720=AXIS2_PLACEMENT_3D ( 'NONE', #34154, #48219, #23137 ) ;
#31722=CARTESIAN_POINT ( 'NONE',  ( 100.6361971157895283, -42.82696290926312344, 78.36158330589692866 ) ) ;
#31723=CARTESIAN_POINT ( 'NONE',  ( 135.7780479399592366, -20.88970947302825110, 2.099345637358482453 ) ) ;
#31727=CARTESIAN_POINT ( 'NONE',  ( 118.1061288724552725, -37.63024191249119355, 34.77372051400695341 ) ) ;
#31731=ORIENTED_EDGE ( 'NONE', *, *, #77509, .F. ) ;
#31733=ORIENTED_EDGE ( 'NONE', *, *, #31128, .T. ) ;
#31734=ORIENTED_EDGE ( 'NONE', *, *, #32927, .F. ) ;
#31736=AXIS2_PLACEMENT_3D ( 'NONE', #26715, #54400, #89869 ) ;
#31738=ORIENTED_EDGE ( 'NONE', *, *, #15350, .T. ) ;
#31739=CARTESIAN_POINT ( 'NONE',  ( 99.40370404213540212, -29.74227323812493751, 230.7261014663879735 ) ) ;
#31740=CARTESIAN_POINT ( 'NONE',  ( 97.27692878956830214, -38.81776010764613005, 126.4931294640330179 ) ) ;
#31741=CARTESIAN_POINT ( 'NONE',  ( 116.3231543710223121, -32.93883412237410369, 190.1356252759109680 ) ) ;
#31743=CARTESIAN_POINT ( 'NONE',  ( 96.19318211390864803, -38.71572558720041712, 47.48229194257797303 ) ) ;
#31744=CARTESIAN_POINT ( 'NONE',  ( 97.81533971292206786, -40.52633391481636949, 42.63639178031785093 ) ) ;
#31745=ORIENTED_EDGE ( 'NONE', *, *, #48131, .T. ) ;
#31746=CARTESIAN_POINT ( 'NONE',  ( 97.12556571727343169, -37.99690723059678277, 172.4272692053028493 ) ) ;
#31747=DIRECTION ( 'NONE',  ( 0.000000000000000000, 0.000000000000000000, 1.000000000000000000 ) ) ;
#31749=ORIENTED_EDGE ( 'NONE', *, *, #68202, .T. ) ;
#31751=CARTESIAN_POINT ( 'NONE',  ( 115.0352363965828886, -42.91102566678780050, 114.3029152670657709 ) ) ;
#31752=CARTESIAN_POINT ( 'NONE',  ( 101.6619702986602505, -45.61876124157287649, 247.1413395616249602 ) ) ;
#31753=CARTESIAN_POINT ( 'NONE',  ( 191.6377717143134589, -67.87844715994100397, 307.9888746672805269 ) ) ;
#31755=CARTESIAN_POINT ( 'NONE',  ( 78.15700282949474342, -38.71057579844610075, 2.232988688759218743 ) ) ;
#31756=CARTESIAN_POINT ( 'NONE',  ( 110.0705912124663968, -28.18614534367760172, 254.2419436376007695 ) ) ;
#31757=CARTESIAN_POINT ( 'NONE',  ( 142.0664832912740394, -45.72944715994099596, -4.824374724088994704 ) ) ;
#31758=CARTESIAN_POINT ( 'NONE',  ( 103.8480726019013645, -46.65951555449685628, 78.32705384733995402 ) ) ;
#31760=CARTESIAN_POINT ( 'NONE',  ( 97.79690410337100559, -31.86307605613059835, 135.9413395616259947 ) ) ;
#31761=VERTEX_POINT ( 'NONE', #45542 ) ;
#31762=CARTESIAN_POINT ( 'NONE',  ( 151.0371591254573218, -24.95799193692592866, 300.4678068554149490 ) ) ;
#31764=EDGE_LOOP ( 'NONE', ( #54887, #59871, #80485, #15572 ) ) ;
#31766=LINE ( 'NONE', #59462, #76934 ) ;
#31767=ADVANCED_FACE ( 'NONE', ( #59631 ), #46210, .F. ) ;
#31772=CARTESIAN_POINT ( 'NONE',  ( 95.97680135624298714, -37.21094296235740018, 116.3489586092439652 ) ) ;
#31775=CARTESIAN_POINT ( 'NONE',  ( 80.06648329127399677, 0.2215528400590013880, 2.408125275911999097 ) ) ;
#31778=ORIENTED_EDGE ( 'NONE', *, *, #53700, .F. ) ;
#31780=CARTESIAN_POINT ( 'NONE',  ( 114.0011561472229289, -28.09198494482817310, 119.5261014663869474 ) ) ;
#31782=DIRECTION ( 'NONE',  ( 0.000000000000000000, 1.000000000000000000, 0.000000000000000000 ) ) ;
#31783=LINE ( 'NONE', #53540, #640 ) ;
#31784=ORIENTED_EDGE ( 'NONE', *, *, #3455, .T. ) ;
#31786=ORIENTED_EDGE ( 'NONE', *, *, #81713, .T. ) ;
#31787=DIRECTION ( 'NONE',  ( 1.000000000000000078E-15, -1.000000000000000083E-30, -1.000000000000000000 ) ) ;
#31788=CARTESIAN_POINT ( 'NONE',  ( 172.5664832912729878, -27.57844715994070484, 21.92562527591199739 ) ) ;
#31793=DIRECTION ( 'NONE',  ( 1.000000000000000000, 0.000000000000000000, 0.000000000000000000 ) ) ;
#31796=CYLINDRICAL_SURFACE ( 'NONE', #15777, 2.117000000000007987 ) ;
#31798=CARTESIAN_POINT ( 'NONE',  ( 101.0349934672011614, -27.38958028709088310, 216.5327681330529686 ) ) ;
#31799=AXIS2_PLACEMENT_3D ( 'NONE', #24948, #4055, #18125 ) ;
#31800=CARTESIAN_POINT ( 'NONE',  ( 34.67381068360361951, -28.98061976759042224, 117.4678068554150485 ) ) ;
#31801=ORIENTED_EDGE ( 'NONE', *, *, #147, .T. ) ;
#31802=CARTESIAN_POINT ( 'NONE',  ( 99.23822674327652749, -42.59304969680523101, 62.83848241876793850 ) ) ;
#31803=DIRECTION ( 'NONE',  ( 0.000000000000000000, 1.000000000000000000, 0.000000000000000000 ) ) ;
#31804=CARTESIAN_POINT ( 'NONE',  ( 98.30745885735822753, -41.72869143677799997, 11.73981054624496245 ) ) ;
#31805=LINE ( 'NONE', #68125, #75030 ) ;
#31808=ORIENTED_EDGE ( 'NONE', *, *, #40382, .F. ) ;
#31810=VECTOR ( 'NONE', #7028, 1000.000000000000000 ) ;
#31811=CARTESIAN_POINT ( 'NONE',  ( 98.31652346514815122, -35.14820314722400241, 237.6158690201829415 ) ) ;
#31812=CARTESIAN_POINT ( 'NONE',  ( 193.0371591254582881, -47.82818131005411999, 300.4678068554149490 ) ) ;
#31813=EDGE_CURVE ( 'NONE', #43969, #25661, #35510, .T. ) ;
#31816=CARTESIAN_POINT ( 'NONE',  ( 82.27374021058591325, -38.37320971852818019, 2.471387388685636566 ) ) ;
#31817=VERTEX_POINT ( 'NONE', #6475 ) ;
#31818=CARTESIAN_POINT ( 'NONE',  ( 76.06670390244796920, -14.72944715994109899, 199.5838068554169524 ) ) ;
#31821=CARTESIAN_POINT ( 'NONE',  ( 117.4080659314679025, -35.59792815749687378, 278.9127681330539872 ) ) ;
#31828=CARTESIAN_POINT ( 'NONE',  ( 71.25614885437424562, -84.12815644128085069, 396.9756252759102040 ) ) ;
#31829=DIRECTION ( 'NONE',  ( -0.000000000000000000, 1.000000000000000000, 0.000000000000000000 ) ) ;
#31830=DIRECTION ( 'NONE',  ( -8.252657816380299978E-16, 0.000000000000000000, -1.000000000000000000 ) ) ;
#31831=CARTESIAN_POINT ( 'NONE',  ( 113.0470503471827044, -45.36488765107162635, 199.0584824187679374 ) ) ;
#31835=ORIENTED_EDGE ( 'NONE', *, *, #38184, .F. ) ;
#31836=CARTESIAN_POINT ( 'NONE',  ( 115.2412948192700952, -44.23743989039658686, 74.22324432352993995 ) ) ;
#31838=ADVANCED_FACE ( 'NONE', ( #1010 ), #75971, .F. ) ;
#31843=CARTESIAN_POINT ( 'NONE',  ( 80.06648281188265059, -39.47944715903999224, 8.225259175037734849 ) ) ;
#31844=DIRECTION ( 'NONE',  ( -1.000000000000000078E-15, -1.000000000000000083E-30, 1.000000000000000000 ) ) ;
#31845=PLANE ( 'NONE',  #85725 ) ;
#31847=CARTESIAN_POINT ( 'NONE',  ( 98.42339386660059120, -37.17434067858062008, 119.1976141791149786 ) ) ;
#31848=CARTESIAN_POINT ( 'NONE',  ( 105.1068790668079203, -26.46800427226792962, 231.2270538473399597 ) ) ;
#31849=DIRECTION ( 'NONE',  ( 0.000000000000000000, 0.000000000000000000, 1.000000000000000000 ) ) ;
#31850=ORIENTED_EDGE ( 'NONE', *, *, #64143, .T. ) ;
#31852=CARTESIAN_POINT ( 'NONE',  ( 135.2096185787368086, -39.23068377182440969, 1.829869271362987604 ) ) ;
#31853=ORIENTED_EDGE ( 'NONE', *, *, #8436, .F. ) ;
#31855=CARTESIAN_POINT ( 'NONE',  ( 87.06648329127402519, -54.72944906728955061, 14.67562527591094934 ) ) ;
#31856=VECTOR ( 'NONE', #82387, 1000.000000000000000 ) ;
#31857=ORIENTED_EDGE ( 'NONE', *, *, #82115, .F. ) ;
#31858=VERTEX_POINT ( 'NONE', #551 ) ;
#31859=CARTESIAN_POINT ( 'NONE',  ( 116.7179538190731733, -33.91062837146667164, 10.05229194257760916 ) ) ;
#31862=AXIS2_PLACEMENT_3D ( 'NONE', #28512, #41685, #82171 ) ;
#31863=CARTESIAN_POINT ( 'NONE',  ( 108.3628298334300268, -27.77214277553820665, 149.3962293518869444 ) ) ;
#31864=CARTESIAN_POINT ( 'NONE',  ( 101.5858402103170590, -47.29319095008832363, 17.19562527591095247 ) ) ;
#31865=ADVANCED_FACE ( 'NONE', ( #40990 ), #24462, .F. ) ;
#31871=FACE_OUTER_BOUND ( 'NONE', #67388, .T. ) ;
#31872=VERTEX_POINT ( 'NONE', #7820 ) ;
#31874=EDGE_CURVE ( 'NONE', #62791, #44500, #88345, .T. ) ;
#31875=CARTESIAN_POINT ( 'NONE',  ( 100.8871230453359686, -44.69993579328431821, 32.05247736852121676 ) ) ;
#31876=DIRECTION ( 'NONE',  ( 0.000000000000000000, 1.000000000000000000, 0.000000000000000000 ) ) ;
#31877=VECTOR ( 'NONE', #65120, 1000.000000000000000 ) ;
#31878=DIRECTION ( 'NONE',  ( 0.000000000000000000, 0.000000000000000000, 1.000000000000000000 ) ) ;
#31880=CARTESIAN_POINT ( 'NONE',  ( 111.0547186471684995, -47.06334559972322751, 17.85753003781598380 ) ) ;
#31881=CARTESIAN_POINT ( 'NONE',  ( 112.2026027939200361, -27.56657145192123082, 30.66991099019694644 ) ) ;
#31883=CARTESIAN_POINT ( 'NONE',  ( 131.0667039024480118, -61.87844715994100397, 234.8338068554150198 ) ) ;
#31884=LINE ( 'NONE', #82305, #83032 ) ;
#31886=DIRECTION ( 'NONE',  ( 0.7071067811989671936, 0.7071067811741279519, -2.899137802813809155E-29 ) ) ;
#31889=CARTESIAN_POINT ( 'NONE',  ( 182.5667039024476708, -32.29483332967956954, 237.4678068554150059 ) ) ;
#31890=AXIS2_PLACEMENT_3D ( 'NONE', #19723, #20185, #27429 ) ;
#31891=CARTESIAN_POINT ( 'NONE',  ( 104.4797840155964082, -46.91084102236943920, 47.37848241876796607 ) ) ;
#31892=CARTESIAN_POINT ( 'NONE',  ( 97.05822270422260090, -41.42079030513556859, 207.6632443235299661 ) ) ;
#31893=CARTESIAN_POINT ( 'NONE',  ( 97.78987344453990715, -29.31549002224505429, 41.78991099019596334 ) ) ;
#31894=CARTESIAN_POINT ( 'NONE',  ( 107.0664832912750057, -36.72944715993903486, 0.7256252759109708128 ) ) ;
#31895=DIRECTION ( 'NONE',  ( -0.7071067811864666375, -0.7071067811866283970, -7.071067811864659848E-16 ) ) ;
#31896=DIRECTION ( 'NONE',  ( 0.000000000000000000, 0.000000000000000000, 1.000000000000000000 ) ) ;
#31900=VERTEX_POINT ( 'NONE', #69155 ) ;
#31901=CARTESIAN_POINT ( 'NONE',  ( 109.9668656698224538, -46.07028316908876775, 93.81562527591097478 ) ) ;
#31902=CIRCLE ( 'NONE', #23260, 2.517500000000005844 ) ;
#31904=ORIENTED_EDGE ( 'NONE', *, *, #56218, .F. ) ;
#31905=LINE ( 'NONE', #54450, #83351 ) ;
#31906=CARTESIAN_POINT ( 'NONE',  ( 96.83034234600431489, -40.83861266248838007, 247.6422919425769749 ) ) ;
#31908=DIRECTION ( 'NONE',  ( 1.000000000000000078E-15, 0.000000000000000000, 1.000000000000000000 ) ) ;
#31909=LINE ( 'NONE', #16513, #13832 ) ;
#31910=CARTESIAN_POINT ( 'NONE',  ( 48.16670390244701139, -28.27351298637280408, -5.074374724088000832 ) ) ;
#31913=CARTESIAN_POINT ( 'NONE',  ( 104.7173522264389334, -47.59653351925024367, 182.4070538473399665 ) ) ;
#31916=CARTESIAN_POINT ( 'NONE',  ( 98.97073112826979013, -33.12568863208839076, 97.42444044875497866 ) ) ;
#31917=DIRECTION ( 'NONE',  ( 0.000000000000000000, 0.000000000000000000, 1.000000000000000000 ) ) ;
#31919=CARTESIAN_POINT ( 'NONE',  ( 97.41213207386813622, -40.51524797426102253, 242.6118157521009664 ) ) ;
#31920=CARTESIAN_POINT ( 'NONE',  ( 172.5664832912740110, -36.32844715994070839, 198.9256252759119832 ) ) ;
#31921=CARTESIAN_POINT ( 'NONE',  ( 107.0664832912750057, -36.72944715993903486, 3.024967495036150922 ) ) ;
#31922=CARTESIAN_POINT ( 'NONE',  ( 182.4202572930269923, -31.94127993907680718, 193.9678068554150059 ) ) ;
#31923=EDGE_CURVE ( 'NONE', #43506, #76954, #76414, .T. ) ;
#31926=EDGE_CURVE ( 'NONE', #57874, #62557, #13741, .T. ) ;
#31927=CARTESIAN_POINT ( 'NONE',  ( 51.06648329127400388, 19.62155284005901024, 330.1506252759110680 ) ) ;
#31928=CARTESIAN_POINT ( 'NONE',  ( 172.5664832912740110, -32.07844715994070839, 18.92562527591200094 ) ) ;
#31929=CARTESIAN_POINT ( 'NONE',  ( 123.6837132603319418, -53.34645651782485487, 239.5838068554170377 ) ) ;
#31930=CARTESIAN_POINT ( 'NONE',  ( 117.1759530674219860, -34.27439392744687296, 209.0156252759109634 ) ) ;
#31935=CARTESIAN_POINT ( 'NONE',  ( 63.03715912545643363, -24.42818131006026761, 129.9678068554150911 ) ) ;
#31938=DIRECTION ( 'NONE',  ( 0.000000000000000000, 0.000000000000000000, 1.000000000000000000 ) ) ;
#31940=ADVANCED_FACE ( 'NONE', ( #83689 ), #7377, .F. ) ;
#31941=VERTEX_POINT ( 'NONE', #16433 ) ;
#31942=DIRECTION ( 'NONE',  ( -0.7071067811865433539, -0.7071067811865516806, -7.071067811865440820E-16 ) ) ;
#31943=EDGE_CURVE ( 'NONE', #70423, #55559, #81088, .T. ) ;
#31944=CARTESIAN_POINT ( 'NONE',  ( 102.8439234467419965, -46.26134197790700853, 177.2441967044819648 ) ) ;
#31945=FACE_OUTER_BOUND ( 'NONE', #36454, .T. ) ;
#31946=ORIENTED_EDGE ( 'NONE', *, *, #11171, .F. ) ;
#31947=ORIENTED_EDGE ( 'NONE', *, *, #18224, .T. ) ;
#31950=CARTESIAN_POINT ( 'NONE',  ( 97.83437608159194099, -40.57245513861558095, 62.64082807836916800 ) ) ;
#31951=PLANE ( 'NONE',  #8652 ) ;
#31952=CARTESIAN_POINT ( 'NONE',  ( 97.86671988816787859, -40.64955957847482182, 166.6470179981232036 ) ) ;
#31953=EDGE_CURVE ( 'NONE', #31900, #19378, #29165, .T. ) ;
#31954=CARTESIAN_POINT ( 'NONE',  ( 102.4274780401303531, -29.97946060242000144, 48.37380465530593909 ) ) ;
#31956=CARTESIAN_POINT ( 'NONE',  ( 164.9667039024477333, -28.27351298636832055, 117.4678068554150485 ) ) ;
#31958=CARTESIAN_POINT ( 'NONE',  ( 163.0664832912739826, 25.62155284005901379, 327.8006252759110453 ) ) ;
#31959=CARTESIAN_POINT ( 'NONE',  ( 82.79255470691722962, -18.36732994130672836, 6.785344856283117565 ) ) ;
#31961=AXIS2_PLACEMENT_3D ( 'NONE', #27752, #33673, #55434 ) ;
#31964=ORIENTED_EDGE ( 'NONE', *, *, #62386, .T. ) ;
#31965=VERTEX_POINT ( 'NONE', #79564 ) ;
#31967=CARTESIAN_POINT ( 'NONE',  ( 99.32879058785749748, -33.04431300321336806, 75.39527697093394920 ) ) ;
#31968=CARTESIAN_POINT ( 'NONE',  ( 117.9717084303226500, -34.78741065070708061, 198.9546728949589749 ) ) ;
#31969=CARTESIAN_POINT ( 'NONE',  ( 117.0473132972741865, -39.66401662079137225, 183.5984824187679578 ) ) ;
#31970=LINE ( 'NONE', #46025, #44687 ) ;
#31971=CARTESIAN_POINT ( 'NONE',  ( 114.4150145978633049, -27.43247436093422920, 270.5441967044823741 ) ) ;
#31973=DIRECTION ( 'NONE',  ( 0.000000000000000000, 1.000000000000000000, 0.000000000000000000 ) ) ;
#31974=EDGE_LOOP ( 'NONE', ( #86393, #57121, #73854, #42192 ) ) ;
#31976=VERTEX_POINT ( 'NONE', #2360 ) ;
#31977=EDGE_CURVE ( 'NONE', #33306, #40190, #85040, .T. ) ;
#31978=CARTESIAN_POINT ( 'NONE',  ( 175.4414832912740110, 12.92155284005802685, 335.5992267699913327 ) ) ;
#31979=CARTESIAN_POINT ( 'NONE',  ( 117.8217860357262481, -31.63511105064214490, 214.1784824187679419 ) ) ;
#31980=ORIENTED_EDGE ( 'NONE', *, *, #74084, .T. ) ;
#31981=CARTESIAN_POINT ( 'NONE',  ( 96.19116125691978425, -32.02117184027007113, 211.0013395616249738 ) ) ;
#31982=LINE ( 'NONE', #60122, #44248 ) ;
#31984=CARTESIAN_POINT ( 'NONE',  ( 41.56670390244777735, -36.32844715994104234, 300.4678068554150059 ) ) ;
#31985=DIRECTION ( 'NONE',  ( -0.7071067811875165754, -0.7071067811855784591, -7.071067811875158601E-16 ) ) ;
#31986=CARTESIAN_POINT ( 'NONE',  ( 97.89674744388518945, -40.44469223237895505, 277.6356252759110248 ) ) ;
#31987=FACE_OUTER_BOUND ( 'NONE', #84219, .T. ) ;
#31988=CARTESIAN_POINT ( 'NONE',  ( 111.8540205700168713, -46.00543295620330753, 268.9556252759110180 ) ) ;
#31989=DIRECTION ( 'NONE',  ( 0.000000000000000000, 1.000000000000000000, 0.000000000000000000 ) ) ;
#31990=CARTESIAN_POINT ( 'NONE',  ( 141.8897065959774011, -45.55267046464435055, 14.92562527591100618 ) ) ;
#31991=CIRCLE ( 'NONE', #10220, 2.749999999999974687 ) ;
#31993=LINE ( 'NONE', #32430, #52916 ) ;
#31995=FACE_OUTER_BOUND ( 'NONE', #3640, .T. ) ;
#31996=CARTESIAN_POINT ( 'NONE',  ( 162.9033555647770015, -33.89581943344391135, 117.4678068554150485 ) ) ;
#31997=EDGE_LOOP ( 'NONE', ( #27606, #11530, #34127, #54942 ) ) ;
#31998=CARTESIAN_POINT ( 'NONE',  ( 136.5037707043289288, -20.00325133682047252, 7.150416387933974605 ) ) ;
#31999=CARTESIAN_POINT ( 'NONE',  ( 99.27200920372420967, -29.77297264586844960, 190.7470538473399415 ) ) ;
#32000=CARTESIAN_POINT ( 'NONE',  ( 107.3339483091110225, -26.30778942656879948, 116.0556252759109555 ) ) ;
#32001=CARTESIAN_POINT ( 'NONE',  ( 116.8983464293968524, -40.32492306460803633, 214.5470538473389581 ) ) ;
#32003=DIRECTION ( 'NONE',  ( 1.000000000000000000, 0.000000000000000000, 0.000000000000000000 ) ) ;
#32007=DIRECTION ( 'NONE',  ( -0.7071067811865774377, 0.7071067811865175967, -7.071067811865782003E-16 ) ) ;
#32008=LINE ( 'NONE', #60941, #6375 ) ;
#32009=CARTESIAN_POINT ( 'NONE',  ( 131.3325395364357462, -19.07457063614894821, 3.076560393663102300 ) ) ;
#32010=VERTEX_POINT ( 'NONE', #78683 ) ;
#32011=ORIENTED_EDGE ( 'NONE', *, *, #65276, .F. ) ;
#32012=CARTESIAN_POINT ( 'NONE',  ( 99.80400324059088746, -42.13953531443270606, 111.2705150661719671 ) ) ;
#32014=ORIENTED_EDGE ( 'NONE', *, *, #46396, .F. ) ;
#32015=CARTESIAN_POINT ( 'NONE',  ( 114.1602155298369325, -45.17592836263234091, 144.1203871806729637 ) ) ;
#32016=CARTESIAN_POINT ( 'NONE',  ( 142.8830277309892836, -77.57998310118428265, 542.9756252759101471 ) ) ;
#32018=CARTESIAN_POINT ( 'NONE',  ( 165.9667039024459996, -28.27351298637401200, -5.074374724088000832 ) ) ;
#32019=AXIS2_PLACEMENT_3D ( 'NONE', #47535, #82551, #26211 ) ;
#32020=DIRECTION ( 'NONE',  ( 1.000000000000000000, -3.885780586187990841E-13, 0.000000000000000000 ) ) ;
#32021=CARTESIAN_POINT ( 'NONE',  ( 45.76696975232822950, -48.62818131005971622, 129.9678068554150911 ) ) ;
#32022=CARTESIAN_POINT ( 'NONE',  ( 110.1509004715571791, -26.04776408289588474, 64.85276813305395649 ) ) ;
#32024=EDGE_CURVE ( 'NONE', #36849, #17132, #64136, .T. ) ;
#32025=ORIENTED_EDGE ( 'NONE', *, *, #7060, .T. ) ;
#32026=ORIENTED_EDGE ( 'NONE', *, *, #69975, .T. ) ;
#32028=CARTESIAN_POINT ( 'NONE',  ( 113.4245949246307532, -29.25360672088989489, 135.5156252759109634 ) ) ;
#32029=DIRECTION ( 'NONE',  ( 0.000000000000000000, 0.000000000000000000, -1.000000000000000000 ) ) ;
#32032=DIRECTION ( 'NONE',  ( 0.7071067811861728725, -0.7071067811869222730, 0.000000000000000000 ) ) ;
#32033=EDGE_CURVE ( 'NONE', #41944, #7841, #30295, .T. ) ;
#32035=LINE ( 'NONE', #59291, #11372 ) ;
#32036=ADVANCED_FACE ( 'NONE', ( #57756, #9610, #50939, #44109, #71847, #50030 ), #58635, .F. ) ;
#32038=DIRECTION ( 'NONE',  ( 1.000000000000000000, 0.000000000000000000, 0.000000000000000000 ) ) ;
#32039=CARTESIAN_POINT ( 'NONE',  ( 115.5559444348971851, -42.74257571503951425, 53.33562527591095659 ) ) ;
#32040=ORIENTED_EDGE ( 'NONE', *, *, #16357, .T. ) ;
#32042=ORIENTED_EDGE ( 'NONE', *, *, #12263, .T. ) ;
#32043=EDGE_CURVE ( 'NONE', #61450, #20221, #1911, .T. ) ;
#32047=CARTESIAN_POINT ( 'NONE',  ( 108.4620505914581798, -44.77196653648033475, 165.5309475124489609 ) ) ;
#32050=VECTOR ( 'NONE', #20136, 1000.000000000000000 ) ;
#32053=ORIENTED_EDGE ( 'NONE', *, *, #19436, .T. ) ;
#32054=LINE ( 'NONE', #3467, #36638 ) ;
#32055=VECTOR ( 'NONE', #47305, 1000.000000000000114 ) ;
#32057=ORIENTED_EDGE ( 'NONE', *, *, #15240, .T. ) ;
#32059=EDGE_CURVE ( 'NONE', #85061, #86269, #51815, .T. ) ;
#32060=CARTESIAN_POINT ( 'NONE',  ( 116.3165111044169038, -35.08217335353153743, 195.3863452106589875 ) ) ;
#32061=DIRECTION ( 'NONE',  ( -0.9242245927363031965, -0.3818493186865919986, 0.000000000000000000 ) ) ;
#32062=CIRCLE ( 'NONE', #7441, 2.550000000000006040 ) ;
#32063=CARTESIAN_POINT ( 'NONE',  ( 144.8545562996767444, -1.932463243632626781, 361.9756252759100335 ) ) ;
#32065=ORIENTED_EDGE ( 'NONE', *, *, #16990, .F. ) ;
#32066=ORIENTED_EDGE ( 'NONE', *, *, #12787, .T. ) ;
#32067=CIRCLE ( 'NONE', #78537, 2.500000000000002220 ) ;
#32068=ORIENTED_EDGE ( 'NONE', *, *, #49469, .F. ) ;
#32070=CARTESIAN_POINT ( 'NONE',  ( 114.6839398542181101, -39.73893943580953447, 191.3452332267339671 ) ) ;
#32071=CARTESIAN_POINT ( 'NONE',  ( 98.31770816264274515, -42.43955203770550355, 101.7870538473399620 ) ) ;
#32072=CARTESIAN_POINT ( 'NONE',  ( 113.4020503763144632, -27.70036014686454351, 84.57753003781698453 ) ) ;
#32073=CARTESIAN_POINT ( 'NONE',  ( 34.27482367531369789, -30.08671355700341010, 117.4678068554150485 ) ) ;
#32076=CARTESIAN_POINT ( 'NONE',  ( 98.00710227423795118, -30.39686567179408172, 156.8289586092439549 ) ) ;
#32077=PLANE ( 'NONE',  #1588 ) ;
#32079=CARTESIAN_POINT ( 'NONE',  ( 19.56670390244796920, -67.87844715994100397, 10.91780685541479734 ) ) ;
#32080=ORIENTED_EDGE ( 'NONE', *, *, #32732, .F. ) ;
#32082=CARTESIAN_POINT ( 'NONE',  ( 167.2371591254544967, -47.82818131005522133, 193.9678068554149775 ) ) ;
#32085=ORIENTED_EDGE ( 'NONE', *, *, #44960, .F. ) ;
#32087=DIRECTION ( 'NONE',  ( 1.000000000000000078E-15, 1.000000000000000083E-30, -1.000000000000000000 ) ) ;
#32088=ORIENTED_EDGE ( 'NONE', *, *, #15204, .T. ) ;
#32089=CARTESIAN_POINT ( 'NONE',  ( 105.1805947621287345, -26.88300331097110885, 131.2268115755357201 ) ) ;
#32090=CARTESIAN_POINT ( 'NONE',  ( 108.9852622695951112, -46.97665739950247143, 82.72419670448194040 ) ) ;
#32092=DIRECTION ( 'NONE',  ( 0.8571673007021115565, -0.5150380749100554878, 7.521945815882500121E-16 ) ) ;
#32093=DIRECTION ( 'NONE',  ( -0.9254794337955620787, -0.3787978585227822492, 0.000000000000000000 ) ) ;
#32094=CARTESIAN_POINT ( 'NONE',  ( 98.84777479348167617, -29.24180311599940651, 80.73848241876795839 ) ) ;
#32095=CARTESIAN_POINT ( 'NONE',  ( 108.6716496925947126, -26.45072611336629720, 185.9527681330539792 ) ) ;
#32096=LINE ( 'NONE', #16700, #40791 ) ;
#32097=PLANE ( 'NONE',  #49661 ) ;
#32099=VECTOR ( 'NONE', #37705, 1000.000000000000000 ) ;
#32100=DIRECTION ( 'NONE',  ( 0.000000000000000000, 0.000000000000000000, 1.000000000000000000 ) ) ;
#32106=CARTESIAN_POINT ( 'NONE',  ( 96.47340144944560336, -31.30584922022854144, 245.9499109901969689 ) ) ;
#32108=CARTESIAN_POINT ( 'NONE',  ( 112.1392620572132870, -28.01277122371624273, 144.6564663131155726 ) ) ;
#32109=CARTESIAN_POINT ( 'NONE',  ( 100.0093689611455687, -28.97871315454919028, 281.6641967044822650 ) ) ;
#32110=CARTESIAN_POINT ( 'NONE',  ( 95.62763156918455820, -33.44862719079586810, 137.1041967044819501 ) ) ;
#32114=CARTESIAN_POINT ( 'NONE',  ( 116.3251085584666527, -32.94148239642360210, 265.1356252759109680 ) ) ;
#32117=ORIENTED_EDGE ( 'NONE', *, *, #66609, .T. ) ;
#32118=ORIENTED_EDGE ( 'NONE', *, *, #57691, .T. ) ;
#32120=ORIENTED_EDGE ( 'NONE', *, *, #40278, .T. ) ;
#32122=CARTESIAN_POINT ( 'NONE',  ( 99.77739493559407435, -44.20163642594127396, 17.96133956162493206 ) ) ;
#32125=B_SPLINE_CURVE_WITH_KNOTS ( 'NONE', 3,
 ( #71618, #42536, #35733, #21682, #30277, #1234, #85703, #64351, #9383, #2578, #64792, #78445, #77986, #57520, #56162, #28937, #23029, #63448 ),
 .UNSPECIFIED., .F., .F.,
 ( 4, 2, 2, 2, 2, 2, 2, 2, 4 ),
 ( 0.000000000000000000, 0.06249999710979182305, 0.1249999942195836461, 0.1874999913293754761, 0.2499999884391672922, 0.3124999855489591361, 0.3749999826587509522, 0.4374999797685427683, 0.4999999768783345844 ),
 .UNSPECIFIED. ) ;
#32126=LINE ( 'NONE', #46186, #58388 ) ;
#32128=CARTESIAN_POINT ( 'NONE',  ( 99.57203460073428403, -40.82693060065560076, 221.1467055423629517 ) ) ;
#32129=ORIENTED_EDGE ( 'NONE', *, *, #45866, .T. ) ;
#32130=ORIENTED_EDGE ( 'NONE', *, *, #44649, .T. ) ;
#32131=ORIENTED_EDGE ( 'NONE', *, *, #55792, .F. ) ;
#32132=CIRCLE ( 'NONE', #82932, 4.874999999999990230 ) ;
#32133=PLANE ( 'NONE',  #15202 ) ;
#32134=CARTESIAN_POINT ( 'NONE',  ( 172.5664832912729878, -27.82844715994070484, 18.92562527591200094 ) ) ;
#32135=CARTESIAN_POINT ( 'NONE',  ( 172.5664832912740110, 0.2215528400590013880, 258.9256252759120116 ) ) ;
#32136=ADVANCED_FACE ( 'NONE', ( #74065 ), #25924, .F. ) ;
#32137=CARTESIAN_POINT ( 'NONE',  ( 105.0852382675896024, -45.91373775275845759, 28.85110711542093753 ) ) ;
#32138=EDGE_CURVE ( 'NONE', #81368, #84820, #54898, .T. ) ;
#32140=EDGE_CURVE ( 'NONE', #39757, #10951, #70906, .T. ) ;
#32141=LINE ( 'NONE', #58944, #76704 ) ;
#32142=CARTESIAN_POINT ( 'NONE',  ( 116.8310051202518309, -36.16593252570070405, 228.8727681330539667 ) ) ;
#32143=DIRECTION ( 'NONE',  ( 4.299999999999999979E-14, -1.000000000000000000, 4.400000000000000367E-29 ) ) ;
#32144=VECTOR ( 'NONE', #11722, 1000.000000000000000 ) ;
#32145=ORIENTED_EDGE ( 'NONE', *, *, #30911, .T. ) ;
#32147=CARTESIAN_POINT ( 'NONE',  ( 106.0828347753605811, -26.76541559764442724, 56.15474603281727184 ) ) ;
#32149=CARTESIAN_POINT ( 'NONE',  ( 99.12283442819817481, -33.29442637601800214, 58.83189989340093007 ) ) ;
#32150=CIRCLE ( 'NONE', #82952, 2.999999999999999112 ) ;
#32154=VECTOR ( 'NONE', #30883, 1000.000000000000000 ) ;
#32156=ORIENTED_EDGE ( 'NONE', *, *, #70009, .T. ) ;
#32157=CARTESIAN_POINT ( 'NONE',  ( 114.0075790447407087, -33.88846322102013175, 9.635625275910941312 ) ) ;
#32158=LINE ( 'NONE', #10386, #54187 ) ;
#32159=ORIENTED_EDGE ( 'NONE', *, *, #66374, .T. ) ;
#32160=CARTESIAN_POINT ( 'NONE',  ( 109.2550203967672928, -46.95863148777297624, 107.7441967044829880 ) ) ;
#32161=ORIENTED_EDGE ( 'NONE', *, *, #19060, .F. ) ;
#32162=CARTESIAN_POINT ( 'NONE',  ( 113.5850730991778619, -42.29362625859309333, 62.68670554236294379 ) ) ;
#32164=DIRECTION ( 'NONE',  ( -1.000000000000000078E-15, 1.000000000000000083E-30, 1.000000000000000000 ) ) ;
#32165=CARTESIAN_POINT ( 'NONE',  ( 111.9059958850653800, -29.27014106345288624, 66.05015473446795227 ) ) ;
#32167=CARTESIAN_POINT ( 'NONE',  ( 182.0667039024480118, -32.29483332968430886, -5.074374724088000832 ) ) ;
#32168=CARTESIAN_POINT ( 'NONE',  ( 115.6290845971308414, -28.50119646097363812, 35.43562527591098643 ) ) ;
#32169=DIRECTION ( 'NONE',  ( 1.907762142705490052E-15, 7.167082501179359715E-16, -1.000000000000000000 ) ) ;
#32170=ORIENTED_EDGE ( 'NONE', *, *, #78573, .T. ) ;
#32171=CARTESIAN_POINT ( 'NONE',  ( 101.9935452999619798, -45.44602508736877411, 257.1563564671954509 ) ) ;
#32172=VERTEX_POINT ( 'NONE', #32727 ) ;
#32174=ORIENTED_EDGE ( 'NONE', *, *, #80976, .F. ) ;
#32177=EDGE_LOOP ( 'NONE', ( #25963, #47139, #23830, #18437 ) ) ;
#32178=CARTESIAN_POINT ( 'NONE',  ( 115.4995704134666994, -41.68388727776413560, 238.4041967044829562 ) ) ;
#32179=DIRECTION ( 'NONE',  ( -1.000000000000000000, 0.000000000000000000, 0.000000000000000000 ) ) ;
#32180=DIRECTION ( 'NONE',  ( -0.1811243269279065315, 0.9834602067165264527, 0.000000000000000000 ) ) ;
#32181=CARTESIAN_POINT ( 'NONE',  ( 95.34914990350537778, -34.95780559393485731, 67.20705384733894050 ) ) ;
#32184=FACE_OUTER_BOUND ( 'NONE', #69158, .T. ) ;
#32189=AXIS2_PLACEMENT_3D ( 'NONE', #17896, #58773, #45577 ) ;
#32190=CARTESIAN_POINT ( 'NONE',  ( 107.0667039024479834, -54.72944715994100306, 239.5838068554169809 ) ) ;
#32192=CARTESIAN_POINT ( 'NONE',  ( 112.0635997081393640, -45.48968496527341188, 113.9904082404935366 ) ) ;
#32193=CARTESIAN_POINT ( 'NONE',  ( 98.05565822401619869, -44.38798742045811707, 226.8870538473399563 ) ) ;
#32195=EDGE_CURVE ( 'NONE', #43151, #39354, #74516, .T. ) ;
#32196=CARTESIAN_POINT ( 'NONE',  ( 97.81168895331838087, -40.51742574516882200, 287.6356252759109680 ) ) ;
#32197=CARTESIAN_POINT ( 'NONE',  ( 194.0667039024475571, -24.92844715993407334, 129.9678068554150343 ) ) ;
#32198=CARTESIAN_POINT ( 'NONE',  ( 98.66229053285113082, -40.10320091580625501, 251.0648007804577730 ) ) ;
#32199=DIRECTION ( 'NONE',  ( 1.000000000000000078E-15, -1.000000000000000083E-30, -1.000000000000000000 ) ) ;
#32200=CARTESIAN_POINT ( 'NONE',  ( 100.9560042165379770, -28.30978499293933126, 71.57562527591099411 ) ) ;
#32202=CARTESIAN_POINT ( 'NONE',  ( 95.97680135624298714, -37.21094296235740018, 116.3489586092439652 ) ) ;
#32203=ORIENTED_EDGE ( 'NONE', *, *, #50181, .T. ) ;
#32205=ORIENTED_EDGE ( 'NONE', *, *, #13198, .T. ) ;
#32206=CARTESIAN_POINT ( 'NONE',  ( 90.06648329127389729, -36.72944715993924802, 14.92562527591095289 ) ) ;
#32207=DIRECTION ( 'NONE',  ( 1.000000000000000000, -1.000000000000000078E-15, 0.000000000000000000 ) ) ;
#32208=CARTESIAN_POINT ( 'NONE',  ( 41.56648329127398966, -27.57844715994070484, 198.9256252759119832 ) ) ;
#32209=ORIENTED_EDGE ( 'NONE', *, *, #40970, .T. ) ;
#32212=CARTESIAN_POINT ( 'NONE',  ( 108.5441999379606983, -26.36493947475176114, 104.9641967044819779 ) ) ;
#32214=LINE ( 'NONE', #58576, #82769 ) ;
#32216=AXIS2_PLACEMENT_3D ( 'NONE', #30793, #11234, #46181 ) ;
#32217=CARTESIAN_POINT ( 'NONE',  ( 31.78666935232898894, -29.62846900982320264, -5.074374724088000832 ) ) ;
#32218=ORIENTED_EDGE ( 'NONE', *, *, #37098, .T. ) ;
#32221=CARTESIAN_POINT ( 'NONE',  ( 113.9315101381565682, -28.03652776953382286, 124.5565776568629559 ) ) ;
#32223=CARTESIAN_POINT ( 'NONE',  ( 95.60734603896362671, -36.72944715994100306, 277.6356252759110248 ) ) ;
#32224=DIRECTION ( 'NONE',  ( 9.912705577010326536E-16, 1.000000000000000000, 0.000000000000000000 ) ) ;
#32225=VERTEX_POINT ( 'NONE', #60879 ) ;
#32226=VECTOR ( 'NONE', #31654, 1000.000000000000000 ) ;
#32228=CARTESIAN_POINT ( 'NONE',  ( 51.03742451361238608, -23.42844715994066362, 237.4678068554150059 ) ) ;
#32229=DIRECTION ( 'NONE',  ( 0.000000000000000000, 0.000000000000000000, 1.000000000000000000 ) ) ;
#32230=DIRECTION ( 'NONE',  ( 0.7071067811743789733, -0.7071067811987160612, 0.000000000000000000 ) ) ;
#32232=CARTESIAN_POINT ( 'NONE',  ( 138.0667039024480403, -58.72944715994091069, 239.5838068554170377 ) ) ;
#32233=DIRECTION ( 'NONE',  ( -0.7071067811864671926, -0.7071067811866279529, -7.071067811864664779E-16 ) ) ;
#32234=FACE_OUTER_BOUND ( 'NONE', #38497, .T. ) ;
#32237=CARTESIAN_POINT ( 'NONE',  ( 117.0608945280935274, -38.08045307652025713, 34.71895861277068462 ) ) ;
#32238=CARTESIAN_POINT ( 'NONE',  ( 97.48942487598456808, -34.74365074496814998, 212.1641967044819808 ) ) ;
#32239=ADVANCED_FACE ( 'NONE', ( #67701 ), #5485, .T. ) ;
#32240=CARTESIAN_POINT ( 'NONE',  ( 63.56670390244824631, -47.82844715994016127, 300.4678068554150627 ) ) ;
#32242=CARTESIAN_POINT ( 'NONE',  ( 112.4079628628857250, -28.49644221148697198, 65.61848241876694487 ) ) ;
#32247=LINE ( 'NONE', #87673, #59052 ) ;
#32248=ORIENTED_EDGE ( 'NONE', *, *, #35430, .T. ) ;
#32249=CARTESIAN_POINT ( 'NONE',  ( 83.06670390244796920, -58.72944715994098885, 231.5838068554150198 ) ) ;
#32250=EDGE_CURVE ( 'NONE', #56062, #39918, #52688, .T. ) ;
#32253=CARTESIAN_POINT ( 'NONE',  ( 115.8610455727973090, -35.41879699190349129, 215.3758690201829609 ) ) ;
#32255=LINE ( 'NONE', #31812, #22670 ) ;
#32256=CYLINDRICAL_SURFACE ( 'NONE', #16023, 11.45913725231036118 ) ;
#32258=EDGE_CURVE ( 'NONE', #50690, #9081, #88166, .T. ) ;
#32259=CARTESIAN_POINT ( 'NONE',  ( 82.63685198412170507, -37.70758306363496359, 2.855952960430489185 ) ) ;
#32262=CARTESIAN_POINT ( 'NONE',  ( 97.33721762003443700, -34.07359039618388863, 37.11469305630519244 ) ) ;
#32263=EDGE_LOOP ( 'NONE', ( #57800, #68104 ) ) ;
#32264=CARTESIAN_POINT ( 'NONE',  ( 109.6119907475197550, -25.15530020966791369, 29.90419670448196854 ) ) ;
#32265=EDGE_LOOP ( 'NONE', ( #12530, #41007, #63958, #89075 ) ) ;
#32266=VERTEX_POINT ( 'NONE', #80010 ) ;
#32267=CARTESIAN_POINT ( 'NONE',  ( 101.0114332956932088, -30.54581597779692359, 268.5233284648295466 ) ) ;
#32271=DIRECTION ( 'NONE',  ( 0.000000000000000000, -1.000000000000000000, 0.000000000000000000 ) ) ;
#32273=CARTESIAN_POINT ( 'NONE',  ( 113.1808386317757282, -26.52034477659904610, 200.6470538473399756 ) ) ;
#32275=EDGE_LOOP ( 'NONE', ( #52109, #41105 ) ) ;
#32276=CARTESIAN_POINT ( 'NONE',  ( 98.26973918885833825, -28.71518450514261289, 76.73848241876795839 ) ) ;
#32277=DIRECTION ( 'NONE',  ( 0.000000000000000000, -1.000000000000000000, 0.000000000000000000 ) ) ;
#32279=ORIENTED_EDGE ( 'NONE', *, *, #84548, .F. ) ;
#32280=ORIENTED_EDGE ( 'NONE', *, *, #13705, .F. ) ;
#32282=CYLINDRICAL_SURFACE ( 'NONE', #36142, 2.749999999999974687 ) ;
#32283=DIRECTION ( 'NONE',  ( 1.000000000000000000, 8.163404592831600092E-16, 1.020425574103949962E-15 ) ) ;
#32284=CARTESIAN_POINT ( 'NONE',  ( 101.9927640441988501, -45.44554309988366469, 152.1569868649772843 ) ) ;
#32285=CARTESIAN_POINT ( 'NONE',  ( 100.3248355287147291, -41.38056247698398238, 124.6252332267339682 ) ) ;
#32286=CARTESIAN_POINT ( 'NONE',  ( 106.3003414554210764, -47.14819399153626023, 218.5184824187679453 ) ) ;
#32288=EDGE_LOOP ( 'NONE', ( #71499, #45854 ) ) ;
#32290=CARTESIAN_POINT ( 'NONE',  ( 136.6880318146010325, -37.56139158948385415, 2.921136715971366371 ) ) ;
#32291=EDGE_CURVE ( 'NONE', #62792, #33465, #39037, .T. ) ;
#32292=ORIENTED_EDGE ( 'NONE', *, *, #60623, .F. ) ;
#32293=ORIENTED_EDGE ( 'NONE', *, *, #2526, .T. ) ;
#32295=ORIENTED_EDGE ( 'NONE', *, *, #55906, .T. ) ;
#32296=ORIENTED_EDGE ( 'NONE', *, *, #65804, .F. ) ;
#32297=CARTESIAN_POINT ( 'NONE',  ( 98.30773656818189465, -41.72926007762017520, 167.7402057210307191 ) ) ;
#32298=LINE ( 'NONE', #33213, #68925 ) ;
#32299=EDGE_CURVE ( 'NONE', #40647, #5575, #82580, .T. ) ;
#32300=CARTESIAN_POINT ( 'NONE',  ( 51.42025729302798709, -31.94127993907680718, 237.4678068554150059 ) ) ;
#32301=CARTESIAN_POINT ( 'NONE',  ( 98.54925023078828872, -36.08769725913535353, 145.6895626852199541 ) ) ;
#32302=CARTESIAN_POINT ( 'NONE',  ( 100.4512773062034370, -27.81586575833916442, 35.59657765686397113 ) ) ;
#32308=DIRECTION ( 'NONE',  ( -0.7071067811865774377, 0.7071067811865175967, -7.071067811865470403E-16 ) ) ;
#32313=VECTOR ( 'NONE', #26811, 1000.000000000000000 ) ;
#32314=DIRECTION ( 'NONE',  ( -1.000000000000000000, 0.000000000000000000, -0.000000000000000000 ) ) ;
#32315=ORIENTED_EDGE ( 'NONE', *, *, #79629, .T. ) ;
#32316=EDGE_CURVE ( 'NONE', #78335, #70136, #76306, .T. ) ;
#32317=CARTESIAN_POINT ( 'NONE',  ( 112.2083724274664291, -26.91728527761779333, 14.68038718067299442 ) ) ;
#32318=CARTESIAN_POINT ( 'NONE',  ( 103.9444121564427235, -47.38074615057520589, 58.33753003781600199 ) ) ;
#32322=DIRECTION ( 'NONE',  ( 4.299999999999999979E-14, -1.000000000000000000, 4.128053709984630540E-29 ) ) ;
#32323=DIRECTION ( 'NONE',  ( 9.912705577010326536E-16, 1.000000000000000000, 0.000000000000000000 ) ) ;
#32324=DIRECTION ( 'NONE',  ( -4.237773401492740281E-14, 1.000000000000000000, 0.000000000000000000 ) ) ;
#32325=DIRECTION ( 'NONE',  ( 1.000000000000000078E-15, -1.000000000000000083E-30, -1.000000000000000000 ) ) ;
#32328=ORIENTED_EDGE ( 'NONE', *, *, #76370, .T. ) ;
#32329=CARTESIAN_POINT ( 'NONE',  ( 96.13137017992535505, -38.63632546489608188, 46.45181575210094138 ) ) ;
#32330=CARTESIAN_POINT ( 'NONE',  ( 99.75313521292756036, -29.29995004827394212, 221.6956252759109702 ) ) ;
#32331=CARTESIAN_POINT ( 'NONE',  ( 112.9754938005188478, -28.11429459860147873, 40.59848241876795782 ) ) ;
#32332=CARTESIAN_POINT ( 'NONE',  ( 97.81304204170952232, -40.52073163124537558, 171.6361819576471532 ) ) ;
#32333=DIRECTION ( 'NONE',  ( 0.000000000000000000, 0.000000000000000000, 1.000000000000000000 ) ) ;
#32336=VECTOR ( 'NONE', #4163, 1000.000000000000000 ) ;
#32338=DIRECTION ( 'NONE',  ( 1.000000000000000000, 0.000000000000000000, 0.000000000000000000 ) ) ;
#32339=VERTEX_POINT ( 'NONE', #55384 ) ;
#32340=CARTESIAN_POINT ( 'NONE',  ( 97.28369645613172167, -37.51102008256656717, 97.38991099019594344 ) ) ;
#32342=ORIENTED_EDGE ( 'NONE', *, *, #81101, .T. ) ;
#32343=CARTESIAN_POINT ( 'NONE',  ( 113.0874441278155160, -45.97130050132138024, 219.0480062282919960 ) ) ;
#32348=CARTESIAN_POINT ( 'NONE',  ( 105.7995184788125016, -26.72403496690349911, 46.17729194326120989 ) ) ;
#32351=CARTESIAN_POINT ( 'NONE',  ( 113.2095242374420252, -45.08419629851117350, 183.0689586092449588 ) ) ;
#32353=ORIENTED_EDGE ( 'NONE', *, *, #40976, .T. ) ;
#32354=CARTESIAN_POINT ( 'NONE',  ( 99.22037001696983793, -32.61037140242165577, 132.3730118773259790 ) ) ;
#32355=FACE_OUTER_BOUND ( 'NONE', #21237, .T. ) ;
#32356=CARTESIAN_POINT ( 'NONE',  ( 106.2788006184939888, -47.06957971430141185, 263.5280062282914741 ) ) ;
#32357=DIRECTION ( 'NONE',  ( 1.000000000000000000, 0.000000000000000000, 0.000000000000000000 ) ) ;
#32358=VECTOR ( 'NONE', #9574, 1000.000000000000000 ) ;
#32359=DIRECTION ( 'NONE',  ( 0.7071067812164788524, -0.7071067811566160710, 0.000000000000000000 ) ) ;
#32360=DIRECTION ( 'NONE',  ( 0.000000000000000000, 1.000000000000000000, 0.000000000000000000 ) ) ;
#32362=EDGE_CURVE ( 'NONE', #42340, #68948, #33270, .T. ) ;
#32363=DIRECTION ( 'NONE',  ( -0.9254794337955620787, -0.3787978585227822492, 0.000000000000000000 ) ) ;
#32364=VECTOR ( 'NONE', #88244, 1000.000000000000000 ) ;
#32365=DIRECTION ( 'NONE',  ( 0.000000000000000000, 0.000000000000000000, 1.000000000000000000 ) ) ;
#32366=CARTESIAN_POINT ( 'NONE',  ( 25.56670390244797275, -62.87844715994099687, 170.4678068554149775 ) ) ;
#32367=ADVANCED_FACE ( 'NONE', ( #69498 ), #41763, .F. ) ;
#32368=CARTESIAN_POINT ( 'NONE',  ( 95.93334478249045105, -32.74178691125829488, 176.0527681330539735 ) ) ;
#32369=CARTESIAN_POINT ( 'NONE',  ( 107.0664832912739968, -36.72944715994100306, 9.635625275910941312 ) ) ;
#32370=VERTEX_POINT ( 'NONE', #26805 ) ;
#32371=VERTEX_POINT ( 'NONE', #49020 ) ;
#32373=CARTESIAN_POINT ( 'NONE',  ( 79.68958420874194815, -15.97944715994105813, 1.625625275910942413 ) ) ;
#32374=CARTESIAN_POINT ( 'NONE',  ( 97.07209078958956638, -35.37825800277666133, 186.2194405451776902 ) ) ;
#32376=CONICAL_SURFACE ( 'NONE', #46893, 1.258749999999999369, 1.029744258676650093 ) ;
#32377=CARTESIAN_POINT ( 'NONE',  ( 109.7212179059393407, -26.99983407561881066, 94.86509365950415429 ) ) ;
#32378=ORIENTED_EDGE ( 'NONE', *, *, #67452, .F. ) ;
#32380=CARTESIAN_POINT ( 'NONE',  ( 103.7231215738078163, -26.19374500585225363, 205.3089586092439731 ) ) ;
#32381=DIRECTION ( 'NONE',  ( 0.000000000000000000, 0.000000000000000000, -1.000000000000000000 ) ) ;
#32382=ORIENTED_EDGE ( 'NONE', *, *, #55324, .F. ) ;
#32383=ORIENTED_EDGE ( 'NONE', *, *, #37865, .F. ) ;
#32385=DIRECTION ( 'NONE',  ( 1.000000000000000000, 4.299999999999999979E-14, 1.000000000000000078E-15 ) ) ;
#32386=CARTESIAN_POINT ( 'NONE',  ( 98.15098341961036965, -41.26162459717305353, 166.7007383883326952 ) ) ;
#32387=CARTESIAN_POINT ( 'NONE',  ( 112.5662596640460720, -44.20262526656594559, 30.89951894101994156 ) ) ;
#32388=CARTESIAN_POINT ( 'NONE',  ( 116.9247085916874909, -40.18670803819183845, 129.5584824187679658 ) ) ;
#32390=ORIENTED_EDGE ( 'NONE', *, *, #30740, .F. ) ;
#32391=DIRECTION ( 'NONE',  ( -4.237773401492740281E-14, 1.000000000000000000, 0.000000000000000000 ) ) ;
#32392=CARTESIAN_POINT ( 'NONE',  ( 82.51738923907551282, -17.48112160756095790, 7.135585143040647615 ) ) ;
#32393=ORIENTED_EDGE ( 'NONE', *, *, #55195, .F. ) ;
#32394=ORIENTED_EDGE ( 'NONE', *, *, #43139, .T. ) ;
#32398=VERTEX_POINT ( 'NONE', #47685 ) ;
#32400=CIRCLE ( 'NONE', #12136, 2.500000000000002220 ) ;
#32401=ADVANCED_FACE ( 'NONE', ( #48570 ), #34515, .T. ) ;
#32402=CARTESIAN_POINT ( 'NONE',  ( 106.8818968526635160, -46.43699862984655624, 76.98384839950495007 ) ) ;
#32403=CARTESIAN_POINT ( 'NONE',  ( 103.2955449146038376, -26.98642977692344758, 215.3699109901969848 ) ) ;
#32404=CARTESIAN_POINT ( 'NONE',  ( 97.40233316251681117, -42.04621543282991780, 176.7146728949589658 ) ) ;
#32405=CARTESIAN_POINT ( 'NONE',  ( 98.17490182338630689, -41.30874685505506960, 21.70468755961504925 ) ) ;
#32406=CARTESIAN_POINT ( 'NONE',  ( 97.09625384711495144, -33.75906160244647936, 27.09562527591097236 ) ) ;
#32408=DIRECTION ( 'NONE',  ( -0.9242245927363026414, -0.3818493186865932754, 0.000000000000000000 ) ) ;
#32409=ORIENTED_EDGE ( 'NONE', *, *, #79264, .F. ) ;
#32412=CARTESIAN_POINT ( 'NONE',  ( 116.5668037432639608, -41.21227053747742985, 228.4756252759109714 ) ) ;
#32413=AXIS2_PLACEMENT_3D ( 'NONE', #58085, #78561, #78108 ) ;
#32414=VERTEX_POINT ( 'NONE', #7713 ) ;
#32416=CARTESIAN_POINT ( 'NONE',  ( 117.4139541310910175, -35.45788210829842058, 193.9241967044829664 ) ) ;
#32418=AXIS2_PLACEMENT_3D ( 'NONE', #52100, #9916, #43963 ) ;
#32419=LINE ( 'NONE', #47838, #92 ) ;
#32420=PLANE ( 'NONE',  #14509 ) ;
#32421=LINE ( 'NONE', #38800, #38398 ) ;
#32422=EDGE_CURVE ( 'NONE', #50547, #79315, #30369, .T. ) ;
#32423=CARTESIAN_POINT ( 'NONE',  ( 113.4284485525086836, -31.82768681777509201, 277.6356252759110248 ) ) ;
#32425=CARTESIAN_POINT ( 'NONE',  ( 168.5667039024485803, -48.82844715993516616, 180.4678068554150059 ) ) ;
#32427=LINE ( 'NONE', #47395, #9280 ) ;
#32428=EDGE_CURVE ( 'NONE', #31120, #33618, #68024, .T. ) ;
#32430=CARTESIAN_POINT ( 'NONE',  ( 73.06670390244801183, -58.72944715994110254, 310.9178068554150514 ) ) ;
#32431=LINE ( 'NONE', #31548, #992 ) ;
#32432=ADVANCED_FACE ( 'NONE', ( #54932 ), #12748, .T. ) ;
#32433=CARTESIAN_POINT ( 'NONE',  ( 116.3212776292294279, -32.94146857471271517, 75.13562527591093954 ) ) ;
#32434=PLANE ( 'NONE',  #18187 ) ;
#32435=ORIENTED_EDGE ( 'NONE', *, *, #16381, .T. ) ;
#32437=FACE_OUTER_BOUND ( 'NONE', #40705, .T. ) ;
#32438=CARTESIAN_POINT ( 'NONE',  ( 103.8128537583787363, -48.15082670742215498, 217.3556252759109668 ) ) ;
#32439=CARTESIAN_POINT ( 'NONE',  ( 103.3624612311685809, -47.14358183654965018, 98.31657765686297523 ) ) ;
#32440=CARTESIAN_POINT ( 'NONE',  ( 106.2987435450237541, -47.16992394167115776, 218.5184824187679453 ) ) ;
#32441=DIRECTION ( 'NONE',  ( 0.000000000000000000, 0.000000000000000000, 1.000000000000000000 ) ) ;
#32442=DIRECTION ( 'NONE',  ( 0.000000000000000000, 0.000000000000000000, 1.000000000000000000 ) ) ;
#32443=DIRECTION ( 'NONE',  ( -4.237773401492740281E-14, 1.000000000000000000, 0.000000000000000000 ) ) ;
#32444=CARTESIAN_POINT ( 'NONE',  ( 100.6688401597533868, -44.50955353575831452, 38.02898386382569385 ) ) ;
#32446=EDGE_CURVE ( 'NONE', #22553, #77150, #47710, .T. ) ;
#32447=AXIS2_PLACEMENT_3D ( 'NONE', #59645, #18324, #38763 ) ;
#32449=EDGE_CURVE ( 'NONE', #29859, #46563, #28597, .T. ) ;
#32450=EDGE_CURVE ( 'NONE', #42888, #88057, #75860, .T. ) ;
#32451=VERTEX_POINT ( 'NONE', #69046 ) ;
#32453=CARTESIAN_POINT ( 'NONE',  ( 103.8778598771455677, -28.80550795996352420, 129.8038483995049432 ) ) ;
#32455=ORIENTED_EDGE ( 'NONE', *, *, #37422, .T. ) ;
#32456=CARTESIAN_POINT ( 'NONE',  ( 97.81375517989221180, -40.51659548082960072, 91.63516306087667829 ) ) ;
#32457=CARTESIAN_POINT ( 'NONE',  ( 108.5866130067098254, -47.05677245125736619, 138.6927681330539883 ) ) ;
#32458=ADVANCED_FACE ( 'NONE', ( #6812 ), #56286, .T. ) ;
#32459=FACE_OUTER_BOUND ( 'NONE', #77269, .T. ) ;
#32460=ADVANCED_FACE ( 'NONE', ( #84030 ), #27708, .F. ) ;
#32461=CARTESIAN_POINT ( 'NONE',  ( 77.31648329127399677, -18.72944715994106346, 6.749768910606400496 ) ) ;
#32464=CARTESIAN_POINT ( 'NONE',  ( 110.1676348244934616, -46.62498374987622896, 52.80610146638697699 ) ) ;
#32465=ORIENTED_EDGE ( 'NONE', *, *, #14214, .T. ) ;
#32466=ORIENTED_EDGE ( 'NONE', *, *, #14633, .F. ) ;
#32467=VERTEX_POINT ( 'NONE', #38424 ) ;
#32470=CARTESIAN_POINT ( 'NONE',  ( 111.1483613326457629, -47.07112276671751516, 168.8756252759109486 ) ) ;
#32471=FACE_OUTER_BOUND ( 'NONE', #59827, .T. ) ;
#32472=CIRCLE ( 'NONE', #576, 10.00000000000000711 ) ;
#32474=CARTESIAN_POINT ( 'NONE',  ( 176.5667039024412759, -48.82844715994099971, 180.4678068554150343 ) ) ;
#32475=DIRECTION ( 'NONE',  ( -1.000000000000000000, 8.775353200852647323E-16, 0.000000000000000000 ) ) ;
#32476=ADVANCED_FACE ( 'NONE', ( #78121 ), #26013, .T. ) ;
#32478=CARTESIAN_POINT ( 'NONE',  ( 105.7152543472329427, -46.72382459542755839, 178.4689408536116275 ) ) ;
#32479=CARTESIAN_POINT ( 'NONE',  ( 115.1902516771093445, -44.19056033372790893, 78.22324432352995416 ) ) ;
#32480=ORIENTED_EDGE ( 'NONE', *, *, #36048, .F. ) ;
#32481=EDGE_LOOP ( 'NONE', ( #4487, #52811, #13706, #85275 ) ) ;
#32483=DIRECTION ( 'NONE',  ( 1.000000000000000078E-15, -1.000000000000000083E-30, -1.000000000000000000 ) ) ;
#32485=ADVANCED_FACE ( 'NONE', ( #84935 ), #15439, .T. ) ;
#32486=DIRECTION ( 'NONE',  ( -1.000000000000000000, 1.122464679914735423E-15, 0.000000000000000000 ) ) ;
#32487=CARTESIAN_POINT ( 'NONE',  ( 112.8963470814680932, -31.01156847455079912, 147.2623760838769726 ) ) ;
#32488=VECTOR ( 'NONE', #71412, 1000.000000000000000 ) ;
#32490=AXIS2_PLACEMENT_3D ( 'NONE', #38905, #80715, #58894 ) ;
#32491=CARTESIAN_POINT ( 'NONE',  ( 177.0664832912730162, 12.92155284005730387, 355.9756252759109998 ) ) ;
#32492=VERTEX_POINT ( 'NONE', #3914 ) ;
#32494=CARTESIAN_POINT ( 'NONE',  ( 162.7866693523280048, -29.62846900982320264, -5.074374724088000832 ) ) ;
#32495=AXIS2_PLACEMENT_3D ( 'NONE', #30661, #51529, #79279 ) ;
#32496=EDGE_LOOP ( 'NONE', ( #57761, #65260 ) ) ;
#32497=ORIENTED_EDGE ( 'NONE', *, *, #16921, .T. ) ;
#32499=B_SPLINE_CURVE_WITH_KNOTS ( 'NONE', 3,
 ( #81402, #19151, #19587, #69990, #20506, #34557, #76801, #494, #54083, #48172, #20048, #54528, #27299, #75905, #82292, #89542, #35449, #83182 ),
 .UNSPECIFIED., .F., .F.,
 ( 4, 2, 2, 2, 2, 2, 2, 2, 4 ),
 ( 0.5000035245575573661, 0.5625030839878626399, 0.6250026434181680246, 0.6875022028484734093, 0.7500017622787786831, 0.8125013217090839568, 0.8750008811393893415, 0.9375004405696947263, 1.000000000000000000 ),
 .UNSPECIFIED. ) ;
#32500=CARTESIAN_POINT ( 'NONE',  ( 109.6042693146342515, -27.68311267370638618, 216.3025356868499500 ) ) ;
#32502=FACE_OUTER_BOUND ( 'NONE', #10402, .T. ) ;
#32503=DIRECTION ( 'NONE',  ( 0.7071067811864697461, 0.7071067811866252883, 7.071067811864691403E-16 ) ) ;
#32506=ORIENTED_EDGE ( 'NONE', *, *, #39402, .T. ) ;
#32507=ORIENTED_EDGE ( 'NONE', *, *, #70071, .T. ) ;
#32508=CARTESIAN_POINT ( 'NONE',  ( 104.8109701446277171, -28.85573464981227687, 223.1166617981629656 ) ) ;
#32509=CARTESIAN_POINT ( 'NONE',  ( 117.6177984774595870, -42.17956309877360610, 93.44705384733897802 ) ) ;
#32510=CARTESIAN_POINT ( 'NONE',  ( 115.0059970501927182, -43.50650750775904640, 63.26419670448196797 ) ) ;
#32511=CARTESIAN_POINT ( 'NONE',  ( 115.7810385730902709, -41.80580201647777017, 253.4065349762460357 ) ) ;
#32513=CARTESIAN_POINT ( 'NONE',  ( 172.5664832912740110, -32.07844715994070839, 258.9256252759120116 ) ) ;
#32514=CARTESIAN_POINT ( 'NONE',  ( 114.3439067968150624, -29.21543093042305728, 170.4641967044829585 ) ) ;
#32515=DIRECTION ( 'NONE',  ( 0.000000000000000000, 0.000000000000000000, -1.000000000000000000 ) ) ;
#32517=CARTESIAN_POINT ( 'NONE',  ( 51.23005224011598102, -33.89581943344511217, -5.074374724088000832 ) ) ;
#32519=ORIENTED_EDGE ( 'NONE', *, *, #13198, .F. ) ;
#32520=CARTESIAN_POINT ( 'NONE',  ( 49.35031423293579422, -29.99615139352249926, 193.9678068554150911 ) ) ;
#32524=DIRECTION ( 'NONE',  ( 1.000000000000000000, 1.000000000000000078E-15, 1.000000000000000078E-15 ) ) ;
#32525=EDGE_LOOP ( 'NONE', ( #48662, #24801, #32690, #51406 ) ) ;
#32526=CARTESIAN_POINT ( 'NONE',  ( 117.0608945229253095, -38.08045312698342144, 178.7189586088083217 ) ) ;
#32527=CARTESIAN_POINT ( 'NONE',  ( 118.8429430416104680, -35.40450127974935413, 83.91562527591095488 ) ) ;
#32529=CIRCLE ( 'NONE', #18075, 2.750000000000002665 ) ;
#32530=ADVANCED_FACE ( 'NONE', ( #70392 ), #52474, .T. ) ;
#32531=CARTESIAN_POINT ( 'NONE',  ( 118.7735074478422348, -37.73348171986721411, 298.1356252759109680 ) ) ;
#32532=CARTESIAN_POINT ( 'NONE',  ( 180.1667039024476651, -28.27351298636767041, 193.9678068554150059 ) ) ;
#32534=CARTESIAN_POINT ( 'NONE',  ( 25.56670390244797275, -48.82844715994099971, 257.2178068554150059 ) ) ;
#32535=CARTESIAN_POINT ( 'NONE',  ( 97.81196631179071233, -40.51810333633504513, 56.63526628290931342 ) ) ;
#32536=CARTESIAN_POINT ( 'NONE',  ( 98.68348088377354088, -30.50934295487602199, 176.8184824187679567 ) ) ;
#32539=VERTEX_POINT ( 'NONE', #49923 ) ;
#32540=CYLINDRICAL_SURFACE ( 'NONE', #13548, 2.500000000000002220 ) ;
#32541=EDGE_CURVE ( 'NONE', #48061, #47812, #59311, .T. ) ;
#32542=CARTESIAN_POINT ( 'NONE',  ( 182.5667039024469886, -33.35206098992650681, 342.9256252759109884 ) ) ;
#32543=LINE ( 'NONE', #52521, #89445 ) ;
#32545=DIRECTION ( 'NONE',  ( 1.054009200593500181E-15, 1.000000000000000000, 0.000000000000000000 ) ) ;
#32546=CARTESIAN_POINT ( 'NONE',  ( 100.6291634319263864, -44.98581313249158598, 232.0499109901969632 ) ) ;
#32549=CARTESIAN_POINT ( 'NONE',  ( 104.4897453729551984, -26.97886022956733143, 145.2814755117790355 ) ) ;
#32550=CARTESIAN_POINT ( 'NONE',  ( 116.1583077856502086, -43.02023234939740348, 9.356577656862985037 ) ) ;
#32551=CARTESIAN_POINT ( 'NONE',  ( 96.65590158217011663, -37.83070472558634378, 122.4099109901969626 ) ) ;
#32552=DIRECTION ( 'NONE',  ( 0.000000000000000000, 0.000000000000000000, -1.000000000000000000 ) ) ;
#32556=ORIENTED_EDGE ( 'NONE', *, *, #81762, .T. ) ;
#32558=AXIS2_PLACEMENT_3D ( 'NONE', #42071, #71599, #2557 ) ;
#32560=AXIS2_PLACEMENT_3D ( 'NONE', #83476, #55727, #14445 ) ;
#32561=AXIS2_PLACEMENT_3D ( 'NONE', #78389, #30220, #28417 ) ;
#32563=EDGE_LOOP ( 'NONE', ( #72670, #88090, #41557 ) ) ;
#32566=CIRCLE ( 'NONE', #35482, 0.5000000000000004441 ) ;
#32568=CARTESIAN_POINT ( 'NONE',  ( 104.4081006448918174, -46.45808913579163857, 72.36479194125030290 ) ) ;
#32569=CARTESIAN_POINT ( 'NONE',  ( 109.6376038899290393, -46.81002275840752702, 43.77562527591094721 ) ) ;
#32570=CARTESIAN_POINT ( 'NONE',  ( 25.56670390244797275, -62.87844715994099687, 257.2178068554150059 ) ) ;
#32575=CARTESIAN_POINT ( 'NONE',  ( 100.3258375188005402, -30.68160747159130963, 235.1790864947439559 ) ) ;
#32577=EDGE_CURVE ( 'NONE', #35335, #30635, #36769, .T. ) ;
#32578=ORIENTED_EDGE ( 'NONE', *, *, #58909, .T. ) ;
#32580=PLANE ( 'NONE',  #58679 ) ;
#32581=CARTESIAN_POINT ( 'NONE',  ( 113.2149055592938964, -44.63128427178952506, 183.1027008292588505 ) ) ;
#32583=CYLINDRICAL_SURFACE ( 'NONE', #2584, 5.599999999999994316 ) ;
#32584=CARTESIAN_POINT ( 'NONE',  ( 110.7632188227358512, -44.78316835090528514, 24.35015473446894418 ) ) ;
#32587=CARTESIAN_POINT ( 'NONE',  ( 114.5610390845466355, -30.44493693613343765, 269.3813395616256798 ) ) ;
#32588=CARTESIAN_POINT ( 'NONE',  ( 63.06670390244645574, -24.92844715994017335, 129.9678068554150911 ) ) ;
#32589=ORIENTED_EDGE ( 'NONE', *, *, #2662, .T. ) ;
#32590=EDGE_CURVE ( 'NONE', #30367, #82586, #31163, .T. ) ;
#32591=CARTESIAN_POINT ( 'NONE',  ( 103.7678503744106138, -27.28725441292130682, 56.34392717193131972 ) ) ;
#32592=EDGE_CURVE ( 'NONE', #39230, #87811, #74746, .T. ) ;
#32593=DIRECTION ( 'NONE',  ( 0.000000000000000000, 1.000000000000000000, 0.000000000000000000 ) ) ;
#32594=CARTESIAN_POINT ( 'NONE',  ( 99.15069935661746570, -33.23069170325895527, 53.80142370292495713 ) ) ;
#32595=VECTOR ( 'NONE', #55556, 1000.000000000000000 ) ;
#32596=CARTESIAN_POINT ( 'NONE',  ( 135.3633572498686988, -16.30134337669370836, 7.962481652676212107 ) ) ;
#32598=DIRECTION ( 'NONE',  ( 1.067522139062650671E-15, 1.000000000000000000, 0.000000000000000000 ) ) ;
#32600=VERTEX_POINT ( 'NONE', #12978 ) ;
#32602=DIRECTION ( 'NONE',  ( -0.7071067811864671926, -0.7071067811866279529, -7.071067811864664779E-16 ) ) ;
#32603=ORIENTED_EDGE ( 'NONE', *, *, #84015, .T. ) ;
#32604=CARTESIAN_POINT ( 'NONE',  ( 112.8018845221357367, -47.09986945403115044, 102.9784824187679817 ) ) ;
#32606=CARTESIAN_POINT ( 'NONE',  ( 104.4240671743138478, -44.88234475468695450, 81.74956268521998481 ) ) ;
#32607=DIRECTION ( 'NONE',  ( -0.7071067811856560636, -0.7071067811874389708, 0.000000000000000000 ) ) ;
#32608=CARTESIAN_POINT ( 'NONE',  ( 103.0662520580798116, -44.63681263099613972, 123.6358690201829802 ) ) ;
#32610=DIRECTION ( 'NONE',  ( 1.000000000000000000, 0.000000000000000000, 0.000000000000000000 ) ) ;
#32612=CARTESIAN_POINT ( 'NONE',  ( 106.5169537372109545, -25.66675205370546919, 41.12800622829193742 ) ) ;
#32613=FACE_OUTER_BOUND ( 'NONE', #34757, .T. ) ;
#32615=EDGE_CURVE ( 'NONE', #46455, #42342, #4812, .T. ) ;
#32617=VECTOR ( 'NONE', #25208, 1000.000000000000114 ) ;
#32618=ORIENTED_EDGE ( 'NONE', *, *, #15375, .F. ) ;
#32619=PLANE ( 'NONE',  #83188 ) ;
#32624=VERTEX_POINT ( 'NONE', #40666 ) ;
#32625=AXIS2_PLACEMENT_3D ( 'NONE', #2088, #56121, #42059 ) ;
#32629=CARTESIAN_POINT ( 'NONE',  ( 116.2779988688840547, -41.49250982992363390, 243.4346728949589647 ) ) ;
#32632=CARTESIAN_POINT ( 'NONE',  ( 116.7448692891101985, -32.85500114480387168, 50.12991099019698282 ) ) ;
#32635=CARTESIAN_POINT ( 'NONE',  ( 115.0891255709548773, -30.61791286384668354, 114.3446839461548024 ) ) ;
#32637=VECTOR ( 'NONE', #1086, 1000.000000000000000 ) ;
#32639=ORIENTED_EDGE ( 'NONE', *, *, #10510, .T. ) ;
#32640=LINE ( 'NONE', #11307, #88024 ) ;
#32641=DIRECTION ( 'NONE',  ( 1.000000000000000000, 3.999999999999999995E-14, 1.000000000000000078E-15 ) ) ;
#32642=CARTESIAN_POINT ( 'NONE',  ( 96.55902551080266960, -40.08462249002853639, 281.5603871806728762 ) ) ;
#32643=CARTESIAN_POINT ( 'NONE',  ( 172.5664832912740110, 0.2215528400590013880, 18.92562527591200094 ) ) ;
#32644=AXIS2_PLACEMENT_3D ( 'NONE', #44715, #65616, #17035 ) ;
#32646=CARTESIAN_POINT ( 'NONE',  ( 46.83715912545339677, -47.82818131006086304, 180.4678068554150911 ) ) ;
#32647=CARTESIAN_POINT ( 'NONE',  ( 19.56648329127400032, -18.82844715994099971, -5.074374724088000832 ) ) ;
#32648=EDGE_CURVE ( 'NONE', #72716, #69535, #24585, .T. ) ;
#32649=CARTESIAN_POINT ( 'NONE',  ( 105.4627246288800109, -27.81649992262058646, 274.6286103042674540 ) ) ;
#32651=CARTESIAN_POINT ( 'NONE',  ( 113.4461594614341209, -46.68675298423766407, 64.02991099019695298 ) ) ;
#32653=CARTESIAN_POINT ( 'NONE',  ( 114.5437501075917481, -29.39581020157643110, 149.4441967044819819 ) ) ;
#32656=ORIENTED_EDGE ( 'NONE', *, *, #7946, .F. ) ;
#32660=CARTESIAN_POINT ( 'NONE',  ( 107.0664832912750057, -36.72944715993903486, 6.826283056785790393 ) ) ;
#32661=ORIENTED_EDGE ( 'NONE', *, *, #16473, .T. ) ;
#32663=EDGE_CURVE ( 'NONE', #35560, #2509, #61109, .T. ) ;
#32664=CARTESIAN_POINT ( 'NONE',  ( 112.1415033342358640, -47.49387789398046067, 137.9270538473389820 ) ) ;
#32665=EDGE_LOOP ( 'NONE', ( #31690, #70338 ) ) ;
#32669=CARTESIAN_POINT ( 'NONE',  ( 41.56648329127399677, 0.2215528400590013880, 201.0426252759120018 ) ) ;
#32671=DIRECTION ( 'NONE',  ( 0.000000000000000000, 0.000000000000000000, -1.000000000000000000 ) ) ;
#32674=CARTESIAN_POINT ( 'NONE',  ( 102.3831517106511484, -26.69142711411281255, 135.4118157521009493 ) ) ;
#32676=AXIS2_PLACEMENT_3D ( 'NONE', #80615, #18364, #72890 ) ;
#32677=FACE_OUTER_BOUND ( 'NONE', #89291, .T. ) ;
#32678=CYLINDRICAL_SURFACE ( 'NONE', #38376, 0.9999999999992039701 ) ;
#32682=DIRECTION ( 'NONE',  ( 0.000000000000000000, 0.000000000000000000, -1.000000000000000000 ) ) ;
#32683=CARTESIAN_POINT ( 'NONE',  ( 101.6985779264912821, -28.22415967511243906, 250.5243335900576653 ) ) ;
#32686=CARTESIAN_POINT ( 'NONE',  ( 97.07206558903125426, -35.37850437031580242, 106.2189636383757687 ) ) ;
#32687=CARTESIAN_POINT ( 'NONE',  ( 165.3359832912740046, -36.32844715994100682, 193.9678068554150059 ) ) ;
#32689=AXIS2_PLACEMENT_3D ( 'NONE', #59276, #4331, #66092 ) ;
#32690=ORIENTED_EDGE ( 'NONE', *, *, #32615, .T. ) ;
#32692=VECTOR ( 'NONE', #61852, 1000.000000000000000 ) ;
#32694=CARTESIAN_POINT ( 'NONE',  ( 172.5664832912728457, -27.82844715994070484, 81.92562527591199739 ) ) ;
#32695=CARTESIAN_POINT ( 'NONE',  ( 96.86352172870826394, -32.31225822881506815, 207.0013395616249738 ) ) ;
#32698=VECTOR ( 'NONE', #54215, 1000.000000000000000 ) ;
#32699=CARTESIAN_POINT ( 'NONE',  ( 107.8187922529720026, -26.97765417004757538, 66.01562527591097762 ) ) ;
#32700=CARTESIAN_POINT ( 'NONE',  ( 61.56670390244727287, -23.42844715994043980, 300.4678068554150627 ) ) ;
#32701=CARTESIAN_POINT ( 'NONE',  ( 188.5667039024479834, -62.87844715994099687, 257.2178068554150059 ) ) ;
#32703=DIRECTION ( 'NONE',  ( -0.000000000000000000, -0.000000000000000000, 1.000000000000000000 ) ) ;
#32705=ORIENTED_EDGE ( 'NONE', *, *, #42984, .F. ) ;
#32707=AXIS2_PLACEMENT_3D ( 'NONE', #48534, #7243, #8135 ) ;
#32708=CARTESIAN_POINT ( 'NONE',  ( 115.9133815579708937, -36.21888896485111076, 225.3044404487539794 ) ) ;
#32711=B_SPLINE_CURVE_WITH_KNOTS ( 'NONE', 3,
 ( #62806, #69188, #26961, #82388, #145, #54181, #27844, #7851, #19695, #35551, #6961, #34209, #55522, #42351, #49168, #62363, #75999, #20152 ),
 .UNSPECIFIED., .F., .F.,
 ( 4, 2, 2, 2, 2, 2, 2, 2, 4 ),
 ( 0.000000000000000000, 0.06249945059766286864, 0.1249989011953257373, 0.1874983517929885990, 0.2499978023906514746, 0.3124972529883143224, 0.3749967035859771980, 0.4374961541836400736, 0.4999956047813029492 ),
 .UNSPECIFIED. ) ;
#32712=DIRECTION ( 'NONE',  ( 1.639958061481212836E-42, -4.100000000000000342E-29, -1.000000000000000000 ) ) ;
#32713=CARTESIAN_POINT ( 'NONE',  ( 82.80053463576300032, -37.07423037057513682, 3.076719480831281217 ) ) ;
#32714=ORIENTED_EDGE ( 'NONE', *, *, #27640, .F. ) ;
#32715=DIRECTION ( 'NONE',  ( 2.900000000000000265E-14, -2.000000000000000155E-15, 1.000000000000000000 ) ) ;
#32716=CARTESIAN_POINT ( 'NONE',  ( 116.3137647483393806, -32.94861263809731611, 185.1356252759109680 ) ) ;
#32717=ORIENTED_EDGE ( 'NONE', *, *, #10741, .F. ) ;
#32718=CARTESIAN_POINT ( 'NONE',  ( 104.2408938701987040, -46.76453939261368475, 22.35848241876792031 ) ) ;
#32720=AXIS2_PLACEMENT_3D ( 'NONE', #87931, #45230, #32061 ) ;
#32721=ORIENTED_EDGE ( 'NONE', *, *, #25593, .F. ) ;
#32722=CARTESIAN_POINT ( 'NONE',  ( 101.0613286755868359, -30.49734935201787422, 263.4928522743534813 ) ) ;
#32724=CARTESIAN_POINT ( 'NONE',  ( 116.6769215743980936, -34.91203320259893417, 158.9756252759109714 ) ) ;
#32726=DIRECTION ( 'NONE',  ( 0.000000000000000000, 0.000000000000000000, 1.000000000000000000 ) ) ;
#32727=CARTESIAN_POINT ( 'NONE',  ( 92.82872956494375671, -30.11307588647346023, 0.4256252759109567241 ) ) ;
#32729=CARTESIAN_POINT ( 'NONE',  ( 99.05265045910354615, -29.93853425193624318, 211.7670538473399517 ) ) ;
#32732=EDGE_CURVE ( 'NONE', #87803, #53062, #11549, .T. ) ;
#32733=CARTESIAN_POINT ( 'NONE',  ( 107.3220933465437810, -25.63295393647281628, 71.04610146638795243 ) ) ;
#32734=DIRECTION ( 'NONE',  ( 1.000000000000000078E-15, -1.000000000000000000, 0.000000000000000000 ) ) ;
#32736=ORIENTED_EDGE ( 'NONE', *, *, #19493, .T. ) ;
#32737=ORIENTED_EDGE ( 'NONE', *, *, #60747, .F. ) ;
#32739=DIRECTION ( 'NONE',  ( 0.000000000000000000, 0.000000000000000000, 1.000000000000000000 ) ) ;
#32742=CARTESIAN_POINT ( 'NONE',  ( 97.86260780209082100, -37.94289672904660193, 149.2480903695909547 ) ) ;
#32743=CARTESIAN_POINT ( 'NONE',  ( 110.8246185410185944, -26.31015614812341141, 245.7889586092439629 ) ) ;
#32746=ORIENTED_EDGE ( 'NONE', *, *, #61227, .T. ) ;
#32750=VERTEX_POINT ( 'NONE', #70169 ) ;
#32751=AXIS2_PLACEMENT_3D ( 'NONE', #42293, #83661, #64112 ) ;
#32752=LINE ( 'NONE', #45029, #57538 ) ;
#32753=CIRCLE ( 'NONE', #40013, 3.300000000000000711 ) ;
#32756=DIRECTION ( 'NONE',  ( 0.000000000000000000, 0.000000000000000000, -1.000000000000000000 ) ) ;
#32761=CARTESIAN_POINT ( 'NONE',  ( 103.7755263489600281, -28.29248842296361133, 169.7828960185539415 ) ) ;
#32762=CARTESIAN_POINT ( 'NONE',  ( 111.4338919110110311, -46.24429912893436523, 27.91848241876792969 ) ) ;
#32764=ORIENTED_EDGE ( 'NONE', *, *, #24759, .T. ) ;
#32765=EDGE_CURVE ( 'NONE', #32906, #2876, #55161, .T. ) ;
#32767=ADVANCED_FACE ( 'NONE', ( #82922 ), #28844, .T. ) ;
#32768=ORIENTED_EDGE ( 'NONE', *, *, #21898, .F. ) ;
#32769=CARTESIAN_POINT ( 'NONE',  ( 97.81169138727440782, -40.51741131469341184, 51.63568823874075520 ) ) ;
#32770=EDGE_CURVE ( 'NONE', #36953, #62140, #15214, .T. ) ;
#32771=ORIENTED_EDGE ( 'NONE', *, *, #78051, .F. ) ;
#32772=FACE_OUTER_BOUND ( 'NONE', #31712, .T. ) ;
#32774=CARTESIAN_POINT ( 'NONE',  ( 110.8532532929841636, -45.98473607795947515, 132.8855204752115924 ) ) ;
#32775=AXIS2_PLACEMENT_3D ( 'NONE', #72156, #49896, #36289 ) ;
#32776=DIRECTION ( 'NONE',  ( -2.999999999999999839E-15, 1.000000000000000000, -2.999999999999999900E-30 ) ) ;
#32778=CARTESIAN_POINT ( 'NONE',  ( 105.4174756516424054, -47.04580008967651850, 37.44991099019695469 ) ) ;
#32779=CARTESIAN_POINT ( 'NONE',  ( 96.88468944541251915, -39.16338508605922186, 52.51276813305394597 ) ) ;
#32781=DIRECTION ( 'NONE',  ( 0.9068632946707807507, -0.4214249218767880945, 8.673617379884035472E-16 ) ) ;
#32783=CARTESIAN_POINT ( 'NONE',  ( 41.56648329127399677, -9.303447159940999356, 16.80862527591200006 ) ) ;
#32784=CYLINDRICAL_SURFACE ( 'NONE', #23812, 4.749999999999976907 ) ;
#32785=EDGE_CURVE ( 'NONE', #11728, #64364, #76994, .T. ) ;
#32786=CARTESIAN_POINT ( 'NONE',  ( 51.06670390244683944, -33.35206098992668444, 117.4678068554150485 ) ) ;
#32787=DIRECTION ( 'NONE',  ( 1.000000000000000078E-15, 1.000000000000000083E-30, -1.000000000000000000 ) ) ;
#32789=CARTESIAN_POINT ( 'NONE',  ( 105.4140021367065003, -47.06753073853725056, 37.44991099019695469 ) ) ;
#32790=CARTESIAN_POINT ( 'NONE',  ( 98.37977233551227130, -29.89460749427659181, 196.8080062282919869 ) ) ;
#32791=CARTESIAN_POINT ( 'NONE',  ( 111.0909104302412373, -25.55688089738240976, 95.80133956162495679 ) ) ;
#32792=CARTESIAN_POINT ( 'NONE',  ( 194.0371591254574923, -24.42818131005417115, 193.9678068554150343 ) ) ;
#32793=LINE ( 'NONE', #4647, #45564 ) ;
#32794=LINE ( 'NONE', #25988, #11781 ) ;
#32795=VECTOR ( 'NONE', #2253, 1000.000000000000000 ) ;
#32796=CARTESIAN_POINT ( 'NONE',  ( 105.7995185434065775, -26.72403495956872277, 186.1772919381388647 ) ) ;
#32797=ORIENTED_EDGE ( 'NONE', *, *, #78936, .F. ) ;
#32798=CARTESIAN_POINT ( 'NONE',  ( 104.2906771502716055, -46.10805769451163627, 103.3470538473389411 ) ) ;
#32801=CARTESIAN_POINT ( 'NONE',  ( 107.2488531970940073, -24.90511003128411360, 226.0641967044829812 ) ) ;
#32803=CARTESIAN_POINT ( 'NONE',  ( 112.4064011319317729, -45.19864057730971751, 148.0241013645836290 ) ) ;
#32804=CARTESIAN_POINT ( 'NONE',  ( 97.81169817874256012, -40.51742791483425776, 82.63555527327814332 ) ) ;
#32805=CARTESIAN_POINT ( 'NONE',  ( 165.3359832912749710, -36.32844715993532247, 193.9678068554149775 ) ) ;
#32806=CARTESIAN_POINT ( 'NONE',  ( 133.1188885517794347, -39.31186128672820956, 1.764000668897718560 ) ) ;
#32807=DIRECTION ( 'NONE',  ( 1.387778780781444492E-15, 0.000000000000000000, -1.000000000000000000 ) ) ;
#32808=CARTESIAN_POINT ( 'NONE',  ( 102.3610132369663148, -45.97051510703457922, 172.2137205140069511 ) ) ;
#32810=EDGE_LOOP ( 'NONE', ( #62464, #77386, #63761, #62153 ) ) ;
#32811=EDGE_CURVE ( 'NONE', #81580, #46354, #72514, .T. ) ;
#32813=CARTESIAN_POINT ( 'NONE',  ( 103.0939887460847189, -28.21499987170311385, 131.8434880678019567 ) ) ;
#32814=VECTOR ( 'NONE', #72566, 1000.000000000000000 ) ;
#32815=CARTESIAN_POINT ( 'NONE',  ( 21.03715912545829170, -47.82818131006186491, 249.9678068554150059 ) ) ;
#32817=CARTESIAN_POINT ( 'NONE',  ( 113.9608400058609874, -28.00707201209563024, 270.5441967044819194 ) ) ;
#32820=DIRECTION ( 'NONE',  ( -0.9988791501868375944, -0.04215501712985142424, 0.02152667770008048417 ) ) ;
#32823=DIRECTION ( 'NONE',  ( -0.7071067811861110330, -0.7071067811869841124, 0.000000000000000000 ) ) ;
#32827=CARTESIAN_POINT ( 'NONE',  ( 101.3611157396114066, -46.16939438856412181, 202.1318157521019430 ) ) ;
#32828=CARTESIAN_POINT ( 'NONE',  ( 123.6837132603318992, -20.11243780205710507, 239.5838068554165545 ) ) ;
#32829=ORIENTED_EDGE ( 'NONE', *, *, #60839, .T. ) ;
#32830=ORIENTED_EDGE ( 'NONE', *, *, #36741, .T. ) ;
#32832=CARTESIAN_POINT ( 'NONE',  ( 81.19091742810981316, -21.23916151080281622, 8.028235474618183432 ) ) ;
#32833=DIRECTION ( 'NONE',  ( 0.000000000000000000, 1.000000000000000000, 0.000000000000000000 ) ) ;
#32836=CARTESIAN_POINT ( 'NONE',  ( 107.0664832912739968, -36.72944715994100306, 9.635625275910941312 ) ) ;
#32838=EDGE_CURVE ( 'NONE', #64390, #52978, #27931, .T. ) ;
#32840=VECTOR ( 'NONE', #88351, 1000.000000000000000 ) ;
#32841=CARTESIAN_POINT ( 'NONE',  ( 106.3019233867144351, -47.12668134090281313, 222.5184824187679453 ) ) ;
#32842=CARTESIAN_POINT ( 'NONE',  ( 135.2096432771673733, -39.23067567606470618, 8.021372095560604265 ) ) ;
#32845=DIRECTION ( 'NONE',  ( 0.7071067811865473507, 0.7071067811865476838, 0.000000000000000000 ) ) ;
#32846=CARTESIAN_POINT ( 'NONE',  ( 104.4076216956003407, -46.45794926476974496, 167.3648273245584051 ) ) ;
#32847=CARTESIAN_POINT ( 'NONE',  ( 100.8629568432159260, -42.03472619363567730, 29.70809036959193250 ) ) ;
#32848=CARTESIAN_POINT ( 'NONE',  ( 114.0008668920709738, -28.09234522576677762, 115.5261014663869474 ) ) ;
#32850=EDGE_LOOP ( 'NONE', ( #88577, #71216, #2349, #33540 ) ) ;
#32851=CIRCLE ( 'NONE', #87991, 17.00000000000090239 ) ;
#32853=CARTESIAN_POINT ( 'NONE',  ( 82.78382032693684778, -18.30343833343667015, 6.798133076500889160 ) ) ;
#32854=ORIENTED_EDGE ( 'NONE', *, *, #39075, .T. ) ;
#32856=LINE ( 'NONE', #26496, #24164 ) ;
#32858=VERTEX_POINT ( 'NONE', #8860 ) ;
#32859=CARTESIAN_POINT ( 'NONE',  ( 125.9611475301391721, -14.72944715994100484, 239.5838068554164977 ) ) ;
#32860=CARTESIAN_POINT ( 'NONE',  ( 102.2122376447956213, -29.66627497393060509, 49.97813411379098625 ) ) ;
#32861=CARTESIAN_POINT ( 'NONE',  ( 109.6112504147204163, -26.56025234872169349, 199.8813395616249977 ) ) ;
#32862=CARTESIAN_POINT ( 'NONE',  ( 103.0581626738561880, -26.45339789934162411, 170.3603871806729444 ) ) ;
#32863=DIRECTION ( 'NONE',  ( -4.237773401492740281E-14, 1.000000000000000000, 0.000000000000000000 ) ) ;
#32864=CARTESIAN_POINT ( 'NONE',  ( 96.71096103112840581, -32.93116260832598385, 17.03467289495896964 ) ) ;
#32866=EDGE_CURVE ( 'NONE', #4156, #15222, #53597, .T. ) ;
#32867=CARTESIAN_POINT ( 'NONE',  ( 119.5435152932140426, -31.57448135767196362, 293.1356252759106837 ) ) ;
#32869=ORIENTED_EDGE ( 'NONE', *, *, #84715, .F. ) ;
#32870=VECTOR ( 'NONE', #53268, 1000.000000000000000 ) ;
#32872=VECTOR ( 'NONE', #57020, 1000.000000000000000 ) ;
#32873=CARTESIAN_POINT ( 'NONE',  ( 96.63812674735558517, -35.80421970836195555, 231.2556252759109725 ) ) ;
#32876=CARTESIAN_POINT ( 'NONE',  ( 117.2277029493381377, -41.08016003417893103, 213.5165776568629781 ) ) ;
#32877=CARTESIAN_POINT ( 'NONE',  ( 97.33784128341626740, -34.07106462853889894, 36.11479195067344250 ) ) ;
#32879=AXIS2_PLACEMENT_3D ( 'NONE', #88930, #82135, #11268 ) ;
#32880=CARTESIAN_POINT ( 'NONE',  ( 100.8870258581724357, -44.69987146937267397, 23.05224687894370206 ) ) ;
#32882=CARTESIAN_POINT ( 'NONE',  ( 103.1392712078617961, -29.55585189219027953, 277.6356252759111953 ) ) ;
#32883=DIRECTION ( 'NONE',  ( -4.237773401492740281E-14, 1.000000000000000000, 0.000000000000000000 ) ) ;
#32885=PLANE ( 'NONE',  #51152 ) ;
#32890=DIRECTION ( 'NONE',  ( 0.000000000000000000, 0.000000000000000000, 1.000000000000000000 ) ) ;
#32893=EDGE_LOOP ( 'NONE', ( #9783, #67208, #54434, #79804 ) ) ;
#32895=CARTESIAN_POINT ( 'NONE',  ( 117.4964429983690337, -36.12752982774328103, 228.8727681330539667 ) ) ;
#32896=CARTESIAN_POINT ( 'NONE',  ( 117.2094703596446550, -39.28701360234872197, 119.6299109901969615 ) ) ;
#32897=CARTESIAN_POINT ( 'NONE',  ( 99.34942397265413661, -29.65555323683921074, 271.7356252759109907 ) ) ;
#32898=LINE ( 'NONE', #81532, #31500 ) ;
#32900=AXIS2_PLACEMENT_3D ( 'NONE', #79930, #38560, #38126 ) ;
#32901=DIRECTION ( 'NONE',  ( -3.999999999999999995E-14, 1.000000000000000000, -4.100000000000000342E-29 ) ) ;
#32902=CARTESIAN_POINT ( 'NONE',  ( 71.25416588882602298, -72.55705569728901594, 542.9756252759101471 ) ) ;
#32904=CARTESIAN_POINT ( 'NONE',  ( 133.8780722764207098, -21.47944715994101017, 1.625625275910997036 ) ) ;
#32906=VERTEX_POINT ( 'NONE', #83814 ) ;
#32908=CARTESIAN_POINT ( 'NONE',  ( 115.3871705984363984, -41.73312485046139386, 127.8181341137909470 ) ) ;
#32909=CARTESIAN_POINT ( 'NONE',  ( 116.3212776292296127, -32.94146857471318413, 287.6356252759109680 ) ) ;
#32912=CARTESIAN_POINT ( 'NONE',  ( 102.6254653968536417, -46.82603978519634325, 128.2346728949589760 ) ) ;
#32914=DIRECTION ( 'NONE',  ( -0.7071067811865171526, -0.7071067811865779928, -7.071067811865164719E-16 ) ) ;
#32917=CARTESIAN_POINT ( 'NONE',  ( 97.55373691267104164, -39.00345059616621768, 56.51276813305494784 ) ) ;
#32918=ORIENTED_EDGE ( 'NONE', *, *, #77339, .T. ) ;
#32919=VERTEX_POINT ( 'NONE', #21588 ) ;
#32921=ORIENTED_EDGE ( 'NONE', *, *, #59603, .F. ) ;
#32922=CARTESIAN_POINT ( 'NONE',  ( 89.24325807922211595, -56.55267046464445002, 14.92562527591095289 ) ) ;
#32923=CARTESIAN_POINT ( 'NONE',  ( 116.4077482568849007, -39.73851878533132975, 154.5784824187679476 ) ) ;
#32925=FACE_OUTER_BOUND ( 'NONE', #29208, .T. ) ;
#32927=EDGE_CURVE ( 'NONE', #41091, #21703, #84273, .T. ) ;
#32928=DIRECTION ( 'NONE',  ( 0.000000000000000000, 0.000000000000000000, 1.000000000000000000 ) ) ;
#32929=LINE ( 'NONE', #13398, #65147 ) ;
#32930=CARTESIAN_POINT ( 'NONE',  ( 117.0608155050156256, -38.08101054489313242, 179.7189142246099891 ) ) ;
#32931=CARTESIAN_POINT ( 'NONE',  ( 96.67837842349533162, -37.29153504031420141, 76.36991099019697060 ) ) ;
#32933=ORIENTED_EDGE ( 'NONE', *, *, #68368, .T. ) ;
#32938=CARTESIAN_POINT ( 'NONE',  ( 108.0149359080884324, -45.33189881898218232, 155.4699951314959776 ) ) ;
#32940=CIRCLE ( 'NONE', #25754, 2.550000000000006040 ) ;
#32941=EDGE_CURVE ( 'NONE', #76097, #27698, #17330, .T. ) ;
#32942=CIRCLE ( 'NONE', #67770, 2.517500000000005844 ) ;
#32947=DIRECTION ( 'NONE',  ( 1.000000000000000000, 4.163336342344333240E-14, 0.000000000000000000 ) ) ;
#32948=ORIENTED_EDGE ( 'NONE', *, *, #77471, .F. ) ;
#32951=CARTESIAN_POINT ( 'NONE',  ( 77.43081253121032148, -19.51428458727107440, 6.911392308671570284 ) ) ;
#32952=EDGE_CURVE ( 'NONE', #15112, #7607, #5791, .T. ) ;
#32953=CARTESIAN_POINT ( 'NONE',  ( 115.7036244402283529, -40.42759782077664710, 209.9482499725639855 ) ) ;
#32956=CARTESIAN_POINT ( 'NONE',  ( 177.0371591254545365, -48.62818131005479927, 193.9678068554150059 ) ) ;
#32957=AXIS2_PLACEMENT_3D ( 'NONE', #10697, #32475, #24346 ) ;
#32958=AXIS2_PLACEMENT_3D ( 'NONE', #38899, #3494, #18457 ) ;
#32959=DIRECTION ( 'NONE',  ( 1.000000000000000000, 3.999999999999999995E-14, 1.000000000000000078E-15 ) ) ;
#32962=VERTEX_POINT ( 'NONE', #44233 ) ;
#32963=ORIENTED_EDGE ( 'NONE', *, *, #59277, .F. ) ;
#32965=EDGE_LOOP ( 'NONE', ( #57150, #50687, #29406, #73940 ) ) ;
#32967=EDGE_CURVE ( 'NONE', #56235, #71705, #29740, .T. ) ;
#32968=CARTESIAN_POINT ( 'NONE',  ( 113.9479352111735295, -42.95371825284467349, 231.0595189410199453 ) ) ;
#32969=CARTESIAN_POINT ( 'NONE',  ( 113.3280054804099137, -28.32220607287434078, 104.5670538473399347 ) ) ;
#32970=CARTESIAN_POINT ( 'NONE',  ( 115.1498815335951491, -43.27828968249936992, 88.28419670448195689 ) ) ;
#32971=CARTESIAN_POINT ( 'NONE',  ( 106.8071438116306382, -44.97946765276041958, 249.5838068554170093 ) ) ;
#32972=CARTESIAN_POINT ( 'NONE',  ( 133.4132809338111940, -16.05633243510671804, 8.161687850939825850 ) ) ;
#32973=CARTESIAN_POINT ( 'NONE',  ( 107.6934652253138722, -25.28725624216507484, 321.0207719853553385 ) ) ;
#32974=CARTESIAN_POINT ( 'NONE',  ( 97.76247233159546113, -41.51031662465626937, 192.7041967044819728 ) ) ;
#32976=CARTESIAN_POINT ( 'NONE',  ( 59.68306514483415270, -72.55903866283681225, 396.9756252759102040 ) ) ;
#32978=LINE ( 'NONE', #32079, #45235 ) ;
#32979=EDGE_LOOP ( 'NONE', ( #87957, #2386, #31134, #20284 ) ) ;
#32980=VERTEX_POINT ( 'NONE', #78354 ) ;
#32981=CARTESIAN_POINT ( 'NONE',  ( 161.4809174648183330, -48.32844715993547879, 300.4678068554149490 ) ) ;
#32982=VERTEX_POINT ( 'NONE', #23391 ) ;
#32983=CARTESIAN_POINT ( 'NONE',  ( 97.81170238817014706, -40.51743819009087844, 137.6355114220584994 ) ) ;
#32984=CARTESIAN_POINT ( 'NONE',  ( 115.0863374808427011, -30.61430893546196330, 90.34429048859003331 ) ) ;
#32985=CARTESIAN_POINT ( 'NONE',  ( 109.2550203967672928, -46.95863148777297624, 107.7441967044829880 ) ) ;
#32987=DIRECTION ( 'NONE',  ( 0.000000000000000000, 0.000000000000000000, 1.000000000000000000 ) ) ;
#32988=DIRECTION ( 'NONE',  ( 0.000000000000000000, 0.000000000000000000, 1.000000000000000000 ) ) ;
#32989=CARTESIAN_POINT ( 'NONE',  ( 116.3135867418571650, -32.94878190598771539, 189.1356252759109680 ) ) ;
#32990=DIRECTION ( 'NONE',  ( -0.9254794337955620787, -0.3787978585227822492, 0.000000000000000000 ) ) ;
#32991=CARTESIAN_POINT ( 'NONE',  ( 110.6887065042382545, -47.98678726807230532, 203.8241967044819489 ) ) ;
#32992=CARTESIAN_POINT ( 'NONE',  ( 46.48091746482041486, -48.32844715994088602, 180.4678068554150911 ) ) ;
#32993=LINE ( 'NONE', #54307, #4681 ) ;
#32994=EDGE_LOOP ( 'NONE', ( #37750, #66824, #61543, #24136 ) ) ;
#32995=CARTESIAN_POINT ( 'NONE',  ( 182.5667039024476708, -33.35206098992057377, 313.9678068554149490 ) ) ;
#32996=EDGE_CURVE ( 'NONE', #41877, #32414, #52108, .T. ) ;
#32998=EDGE_CURVE ( 'NONE', #53561, #56608, #78795, .T. ) ;
#32999=CARTESIAN_POINT ( 'NONE',  ( 97.39155240945729020, -39.27951294533326632, 136.5318526297954520 ) ) ;
#33000=EDGE_CURVE ( 'NONE', #40888, #70942, #16999, .T. ) ;
#33001=FACE_OUTER_BOUND ( 'NONE', #39349, .T. ) ;
#33002=CARTESIAN_POINT ( 'NONE',  ( 110.7486471836621860, -26.25784018214204707, 254.8194347997204545 ) ) ;
#33004=CARTESIAN_POINT ( 'NONE',  ( 114.2795876152497243, -29.76195770723571954, 194.4373016625220032 ) ) ;
#33005=CARTESIAN_POINT ( 'NONE',  ( 100.1631548973110739, -45.39139052332982516, 268.0289586092443415 ) ) ;
#33006=CARTESIAN_POINT ( 'NONE',  ( 117.6520138419322734, -33.39117794972031561, 125.0575300378149706 ) ) ;
#33008=AXIS2_PLACEMENT_3D ( 'NONE', #20932, #13227, #48604 ) ;
#33011=CARTESIAN_POINT ( 'NONE',  ( 134.0664832912739826, -9.029447159941003775, 1.625625275910997480 ) ) ;
#33013=CARTESIAN_POINT ( 'NONE',  ( 105.7995185409999692, -26.72403495984207922, 190.1772919383297449 ) ) ;
#33015=EDGE_LOOP ( 'NONE', ( #38486, #28493, #34999, #76310 ) ) ;
#33018=EDGE_LOOP ( 'NONE', ( #3092, #35890 ) ) ;
#33019=ORIENTED_EDGE ( 'NONE', *, *, #68253, .F. ) ;
#33020=AXIS2_PLACEMENT_3D ( 'NONE', #62991, #772, #28470 ) ;
#33023=CARTESIAN_POINT ( 'NONE',  ( 111.0379167980822928, -47.01981040405694756, 13.85753003781498016 ) ) ;
#33027=VECTOR ( 'NONE', #86030, 1000.000000000000000 ) ;
#33028=LINE ( 'NONE', #66192, #67076 ) ;
#33029=CARTESIAN_POINT ( 'NONE',  ( 137.8167039024479834, -50.82844715994100682, 250.9178068554160461 ) ) ;
#33031=CARTESIAN_POINT ( 'NONE',  ( 114.8821461825539245, -40.17495804977037466, 252.9181341137911545 ) ) ;
#33033=ORIENTED_EDGE ( 'NONE', *, *, #52911, .F. ) ;
#33036=LINE ( 'NONE', #60729, #2170 ) ;
#33037=DIRECTION ( 'NONE',  ( -0.7071067811866279529, 0.7071067811864671926, -7.071067811866286874E-16 ) ) ;
#33038=DIRECTION ( 'NONE',  ( -0.9825752044165969590, -0.1858654558159821002, 0.000000000000000000 ) ) ;
#33040=CARTESIAN_POINT ( 'NONE',  ( 115.0635112019030686, -32.91162553226137533, 15.61301187732594364 ) ) ;
#33042=DIRECTION ( 'NONE',  ( 1.067522139062650671E-15, 1.000000000000000000, 0.000000000000000000 ) ) ;
#33043=CARTESIAN_POINT ( 'NONE',  ( 97.18779033502694631, -39.88384928074078317, 281.5603871806734446 ) ) ;
#33044=LINE ( 'NONE', #59396, #38519 ) ;
#33045=ORIENTED_EDGE ( 'NONE', *, *, #15375, .T. ) ;
#33048=CARTESIAN_POINT ( 'NONE',  ( 109.6546009468767693, -44.98793201169110034, 50.62428084578196774 ) ) ;
#33049=VECTOR ( 'NONE', #7734, 1000.000000000000000 ) ;
#33052=DIRECTION ( 'NONE',  ( 0.000000000000000000, 0.000000000000000000, -1.000000000000000000 ) ) ;
#33053=DIRECTION ( 'NONE',  ( 0.000000000000000000, 0.000000000000000000, 1.000000000000000000 ) ) ;
#33055=DIRECTION ( 'NONE',  ( -4.237773401492740281E-14, 1.000000000000000000, 0.000000000000000000 ) ) ;
#33059=CARTESIAN_POINT ( 'NONE',  ( 109.5085389712880612, -46.86470218963918200, 132.7641967044819751 ) ) ;
#33061=CARTESIAN_POINT ( 'NONE',  ( 105.1764056618614944, -45.05913732685939976, 71.82099125664798578 ) ) ;
#33063=DIRECTION ( 'NONE',  ( 0.7071067811868710917, -0.7071067811862240537, 0.000000000000000000 ) ) ;
#33064=CARTESIAN_POINT ( 'NONE',  ( 99.30241108408027628, -32.39570601076609080, 107.3530118773259545 ) ) ;
#33065=ADVANCED_FACE ( 'NONE', ( #72415 ), #71531, .F. ) ;
#33066=CARTESIAN_POINT ( 'NONE',  ( 177.0664832912730162, 12.92155284005730387, 355.9756252759109998 ) ) ;
#33067=VECTOR ( 'NONE', #40913, 1000.000000000000000 ) ;
#33069=CARTESIAN_POINT ( 'NONE',  ( 114.3683386633632324, -44.20073667237542026, 69.19276813305397411 ) ) ;
#33071=ADVANCED_FACE ( 'NONE', ( #38320 ), #66018, .T. ) ;
#33072=DIRECTION ( 'NONE',  ( 0.000000000000000000, 0.000000000000000000, 1.000000000000000000 ) ) ;
#33075=VECTOR ( 'NONE', #34456, 1000.000000000000000 ) ;
#33078=ORIENTED_EDGE ( 'NONE', *, *, #44757, .T. ) ;
#33079=EDGE_CURVE ( 'NONE', #31182, #23292, #5607, .T. ) ;
#33080=VECTOR ( 'NONE', #13299, 1000.000000000000000 ) ;
#33082=EDGE_LOOP ( 'NONE', ( #71146, #80394, #86699, #15282, #80602, #13639, #48047, #25771, #40688, #11045, #37509, #72174 ) ) ;
#33083=CARTESIAN_POINT ( 'NONE',  ( 112.1541913332956710, -45.76570811864968391, 257.9965776568639626 ) ) ;
#33084=CARTESIAN_POINT ( 'NONE',  ( 97.72691728231733066, -42.68408598780226271, 137.7661014663869992 ) ) ;
#33085=CARTESIAN_POINT ( 'NONE',  ( 19.56648329127303043, -81.37844715994266664, 342.9256252759109884 ) ) ;
#33086=CARTESIAN_POINT ( 'NONE',  ( 117.0603735531381346, -38.08412411259971009, 129.7186663005400078 ) ) ;
#33087=CARTESIAN_POINT ( 'NONE',  ( 111.0825168487035626, -25.58018305758348632, 95.80133956162495679 ) ) ;
#33089=CARTESIAN_POINT ( 'NONE',  ( 192.5667039024472444, -23.42844715993414084, 300.4678068554149490 ) ) ;
#33090=ORIENTED_EDGE ( 'NONE', *, *, #85425, .T. ) ;
#33091=CIRCLE ( 'NONE', #72268, 15.69999999999999574 ) ;
#33092=CARTESIAN_POINT ( 'NONE',  ( 156.5667039024485803, -48.82844715993568485, 139.7178068554149775 ) ) ;
#33095=DIRECTION ( 'NONE',  ( -0.7071067811865279218, 0.7071067811865670016, -6.612322855859973915E-17 ) ) ;
#33096=ORIENTED_EDGE ( 'NONE', *, *, #46486, .T. ) ;
#33097=DIRECTION ( 'NONE',  ( 5.512527431108029424E-15, -1.000000000000000000, 0.000000000000000000 ) ) ;
#33099=CARTESIAN_POINT ( 'NONE',  ( 116.1995025514324169, -41.78438384397603045, 263.4241967044824833 ) ) ;
#33100=CARTESIAN_POINT ( 'NONE',  ( 107.0664832912739399, -36.72944715994096754, 300.2406250056037038 ) ) ;
#33101=CARTESIAN_POINT ( 'NONE',  ( 182.5667039024480118, -32.29483332968450782, 342.9256252759119548 ) ) ;
#33102=CARTESIAN_POINT ( 'NONE',  ( 79.41328093381464726, -39.40256188477533073, 1.689562700881423130 ) ) ;
#33103=CARTESIAN_POINT ( 'NONE',  ( 111.6523633261645188, -43.93540552976629243, 262.4495626852196892 ) ) ;
#33104=DIRECTION ( 'NONE',  ( 2.900000000000000265E-14, -2.000000000000000155E-15, 1.000000000000000000 ) ) ;
#33105=CARTESIAN_POINT ( 'NONE',  ( 107.2318599658364207, -25.70055450771780059, 76.07657765686298035 ) ) ;
#33106=LINE ( 'NONE', #62600, #146 ) ;
#33107=CARTESIAN_POINT ( 'NONE',  ( 118.9678564412739092, -36.92894532057803758, 153.8127681330539644 ) ) ;
#33108=ORIENTED_EDGE ( 'NONE', *, *, #11254, .T. ) ;
#33109=DIRECTION ( 'NONE',  ( -0.7071067812163274180, 0.7071067811567677275, -6.612322856138636565E-17 ) ) ;
#33111=VECTOR ( 'NONE', #81270, 1000.000000000000000 ) ;
#33112=FACE_OUTER_BOUND ( 'NONE', #43153, .T. ) ;
#33116=EDGE_CURVE ( 'NONE', #48698, #77063, #28942, .T. ) ;
#33117=CARTESIAN_POINT ( 'NONE',  ( 112.1419149229391650, -28.01429753427307290, 60.65653136556989722 ) ) ;
#33118=CARTESIAN_POINT ( 'NONE',  ( 97.75494523667518365, -42.77206137223026161, 146.7965776568629508 ) ) ;
#33119=ORIENTED_EDGE ( 'NONE', *, *, #84511, .T. ) ;
#33120=DIRECTION ( 'NONE',  ( 0.000000000000000000, -1.000000000000000000, 0.000000000000000000 ) ) ;
#33121=ADVANCED_FACE ( 'NONE', ( #75082 ), #87823, .T. ) ;
#33123=VECTOR ( 'NONE', #68153, 1000.000000000000114 ) ;
#33124=CARTESIAN_POINT ( 'NONE',  ( 97.81170255947417047, -40.51743869465033754, 117.6354096206635518 ) ) ;
#33126=CARTESIAN_POINT ( 'NONE',  ( 100.8874678944084593, -44.70022138268650735, 77.05229194355962363 ) ) ;
#33127=EDGE_LOOP ( 'NONE', ( #87776, #40819, #54455, #73643 ) ) ;
#33129=PLANE ( 'NONE',  #35586 ) ;
#33130=PLANE ( 'NONE',  #63080 ) ;
#33132=ORIENTED_EDGE ( 'NONE', *, *, #27978, .T. ) ;
#33135=CARTESIAN_POINT ( 'NONE',  ( 49.35211078756547209, -35.65087443492560482, 342.9256252759109884 ) ) ;
#33136=DIRECTION ( 'NONE',  ( -1.000000000000000000, -2.999999999999999839E-15, -1.000000000000000078E-15 ) ) ;
#33137=AXIS2_PLACEMENT_3D ( 'NONE', #30660, #37920, #57912 ) ;
#33138=CARTESIAN_POINT ( 'NONE',  ( 31.56670390244800828, -32.29483332968611364, -5.074374724088000832 ) ) ;
#33140=CARTESIAN_POINT ( 'NONE',  ( 31.56670390244679325, -32.29483332968652576, 117.4678068554150485 ) ) ;
#33141=AXIS2_PLACEMENT_3D ( 'NONE', #10031, #37738, #65436 ) ;
#33143=ORIENTED_EDGE ( 'NONE', *, *, #31708, .F. ) ;
#33145=CARTESIAN_POINT ( 'NONE',  ( 97.99937763885738207, -40.39701179870334613, 202.6327681330529629 ) ) ;
#33146=FACE_BOUND ( 'NONE', #47919, .T. ) ;
#33147=ORIENTED_EDGE ( 'NONE', *, *, #53773, .T. ) ;
#33148=AXIS2_PLACEMENT_3D ( 'NONE', #51055, #77887, #78351 ) ;
#33149=CARTESIAN_POINT ( 'NONE',  ( 116.1466984671187248, -33.09446055034466383, 50.12991099019598096 ) ) ;
#33150=CARTESIAN_POINT ( 'NONE',  ( 107.0664832912739399, -36.72944715994095333, 311.3356252759109566 ) ) ;
#33151=CYLINDRICAL_SURFACE ( 'NONE', #80505, 0.2500000000000002220 ) ;
#33153=CARTESIAN_POINT ( 'NONE',  ( 194.0371591254575208, -24.89890238294407254, 180.4678068554150343 ) ) ;
#33157=ORIENTED_EDGE ( 'NONE', *, *, #3738, .T. ) ;
#33158=EDGE_LOOP ( 'NONE', ( #13523, #61738, #82822, #72805 ) ) ;
#33160=CARTESIAN_POINT ( 'NONE',  ( 98.65401097786960349, -39.51487139837627893, 238.0130118773259653 ) ) ;
#33162=DIRECTION ( 'NONE',  ( 1.000000000000000000, 0.000000000000000000, 0.000000000000000000 ) ) ;
#33163=EDGE_CURVE ( 'NONE', #19112, #66320, #18323, .T. ) ;
#33165=CARTESIAN_POINT ( 'NONE',  ( 97.81169409577289287, -40.51741657705139232, 81.63570706759205109 ) ) ;
#33166=VECTOR ( 'NONE', #10312, 1000.000000000000000 ) ;
#33167=CARTESIAN_POINT ( 'NONE',  ( 97.81452210549078075, -40.51628237377364883, 52.63520911028864901 ) ) ;
#33169=CARTESIAN_POINT ( 'NONE',  ( 179.4595971212720258, -26.00627455219131789, -5.074374724088000832 ) ) ;
#33170=EDGE_CURVE ( 'NONE', #69198, #77789, #81029, .T. ) ;
#33172=ORIENTED_EDGE ( 'NONE', *, *, #33571, .T. ) ;
#33173=CARTESIAN_POINT ( 'NONE',  ( 112.1975415602056216, -26.93795424888832812, 14.68038718067299442 ) ) ;
#33174=ORIENTED_EDGE ( 'NONE', *, *, #80979, .F. ) ;
#33176=CARTESIAN_POINT ( 'NONE',  ( 113.4754094548699186, -31.62960856676687982, 242.1795189410199782 ) ) ;
#33177=ADVANCED_FACE ( 'NONE', ( #68278 ), #31951, .T. ) ;
#33178=CARTESIAN_POINT ( 'NONE',  ( 98.51953950620406886, -30.85675296092858844, 165.8594347997209582 ) ) ;
#33184=CARTESIAN_POINT ( 'NONE',  ( 99.50795136241276850, -29.43516104912357179, 246.7156252759109520 ) ) ;
#33188=CARTESIAN_POINT ( 'NONE',  ( 112.5370353716610055, -27.80386372334747236, 90.63848241876793566 ) ) ;
#33190=ORIENTED_EDGE ( 'NONE', *, *, #1720, .F. ) ;
#33192=ORIENTED_EDGE ( 'NONE', *, *, #22466, .T. ) ;
#33193=ADVANCED_FACE ( 'NONE', ( #89166 ), #40101, .T. ) ;
#33194=DIRECTION ( 'NONE',  ( 4.194175870806139918E-14, -1.000000000000000000, 0.000000000000000000 ) ) ;
#33195=FACE_OUTER_BOUND ( 'NONE', #14195, .T. ) ;
#33196=CARTESIAN_POINT ( 'NONE',  ( 34.96670390244699433, -26.71338133339301635, 237.4678068554150059 ) ) ;
#33197=CARTESIAN_POINT ( 'NONE',  ( 108.2592170473780300, -44.83253820548913637, 140.5109475124479559 ) ) ;
#33198=CARTESIAN_POINT ( 'NONE',  ( 109.3416101119966442, -26.53331765884353644, 220.9013395616249795 ) ) ;
#33199=EDGE_CURVE ( 'NONE', #35463, #77666, #33301, .T. ) ;
#33200=DIRECTION ( 'NONE',  ( 1.000000000000000000, 3.999999999999999995E-14, 1.000000000000000078E-15 ) ) ;
#33203=AXIS2_PLACEMENT_3D ( 'NONE', #38355, #66055, #3846 ) ;
#33204=CARTESIAN_POINT ( 'NONE',  ( 136.6235172543038061, -37.74149216370406634, 2.839569540204782250 ) ) ;
#33207=VECTOR ( 'NONE', #77077, 1000.000000000000000 ) ;
#33208=VECTOR ( 'NONE', #23276, 1000.000000000000000 ) ;
#33209=DIRECTION ( 'NONE',  ( -3.360405532702990443E-14, 1.000000000000000000, 0.000000000000000000 ) ) ;
#33212=DIRECTION ( 'NONE',  ( -4.299999999999999979E-14, 1.000000000000000000, 0.000000000000000000 ) ) ;
#33213=CARTESIAN_POINT ( 'NONE',  ( 183.6524903400785433, -48.32844715993451956, 180.4678068554150343 ) ) ;
#33214=PLANE ( 'NONE',  #84436 ) ;
#33215=DIRECTION ( 'NONE',  ( 0.000000000000000000, 0.000000000000000000, 1.000000000000000000 ) ) ;
#33216=CARTESIAN_POINT ( 'NONE',  ( 97.43556672503765981, -37.99919831760565359, 150.8524198280769895 ) ) ;
#33217=CARTESIAN_POINT ( 'NONE',  ( 116.4271464750313498, -31.96187137292554681, 44.20133956162491984 ) ) ;
#33218=PLANE ( 'NONE',  #52362 ) ;
#33219=VERTEX_POINT ( 'NONE', #26935 ) ;
#33220=VECTOR ( 'NONE', #29618, 1000.000000000000000 ) ;
#33222=ORIENTED_EDGE ( 'NONE', *, *, #873, .T. ) ;
#33224=LINE ( 'NONE', #87297, #15675 ) ;
#33226=CARTESIAN_POINT ( 'NONE',  ( 41.56648329127499153, -36.32844715994070839, 314.1756252759120116 ) ) ;
#33229=EDGE_CURVE ( 'NONE', #7923, #71348, #54602, .T. ) ;
#33230=CARTESIAN_POINT ( 'NONE',  ( 115.1270644249241997, -42.70333644879877255, 133.3187822923470378 ) ) ;
#33231=CARTESIAN_POINT ( 'NONE',  ( 177.4809174648216299, -49.32844715993478246, 129.9678068554150059 ) ) ;
#33233=CARTESIAN_POINT ( 'NONE',  ( 112.3383795496262820, -28.20708685789894687, 289.6356252759109680 ) ) ;
#33234=CARTESIAN_POINT ( 'NONE',  ( 100.9155127638074703, -46.91653085812070856, 48.14419670448194211 ) ) ;
#33235=CARTESIAN_POINT ( 'NONE',  ( 97.81168839172025287, -40.51739946886939947, 131.6358419732753475 ) ) ;
#33236=DIRECTION ( 'NONE',  ( 0.000000000000000000, 1.000000000000000000, 0.000000000000000000 ) ) ;
#33237=CARTESIAN_POINT ( 'NONE',  ( 116.3212776292299253, -32.94146857471393730, 145.1356252759109680 ) ) ;
#33238=CARTESIAN_POINT ( 'NONE',  ( 107.0664832912730020, -27.87844715994269862, 361.9756252759109998 ) ) ;
#33240=B_SPLINE_CURVE_WITH_KNOTS ( 'NONE', 3,
 ( #43466, #36683, #57552, #85294, #48471, #76214, #41671, #62583, #7184, #34872, #358, #83483, #48927, #76670, #38013, #37572, #72541, #79369 ),
 .UNSPECIFIED., .F., .F.,
 ( 4, 2, 2, 2, 2, 2, 2, 2, 4 ),
 ( 0.5000000006881730741, 0.5625000006021514398, 0.6250000005161298056, 0.6875000004301081713, 0.7500000003440865370, 0.8125000002580649028, 0.8750000001720432685, 0.9375000000860216343, 1.000000000000000000 ),
 .UNSPECIFIED. ) ;
#33245=CARTESIAN_POINT ( 'NONE',  ( 97.76994516709639527, -29.29956314839395048, 45.78991099019697231 ) ) ;
#33246=CARTESIAN_POINT ( 'NONE',  ( 96.05470400087912708, -37.92356717231275098, 77.40038718067299328 ) ) ;
#33247=CARTESIAN_POINT ( 'NONE',  ( 97.86672871672134022, -40.64958041416993240, 171.6472150801397163 ) ) ;
#33249=CYLINDRICAL_SURFACE ( 'NONE', #50927, 0.5000000000000004441 ) ;
#33250=VECTOR ( 'NONE', #22020, 1000.000000000000114 ) ;
#33251=EDGE_CURVE ( 'NONE', #10387, #26370, #38762, .T. ) ;
#33253=ORIENTED_EDGE ( 'NONE', *, *, #64704, .F. ) ;
#33254=CARTESIAN_POINT ( 'NONE',  ( 116.3624975636023322, -33.68846805112529808, 85.07848241876692441 ) ) ;
#33255=LINE ( 'NONE', #88685, #25380 ) ;
#33256=EDGE_LOOP ( 'NONE', ( #30421, #8095 ) ) ;
#33257=CARTESIAN_POINT ( 'NONE',  ( 98.05565822401628395, -44.38798742045805312, 222.8870538473399563 ) ) ;
#33258=CARTESIAN_POINT ( 'NONE',  ( 104.4070333491352471, -46.45780296964726119, 253.3665111305816140 ) ) ;
#33259=CYLINDRICAL_SURFACE ( 'NONE', #23222, 3.299999999999997158 ) ;
#33261=CARTESIAN_POINT ( 'NONE',  ( 104.4899544425265532, -26.97880758706315873, 46.28145860999622130 ) ) ;
#33262=AXIS2_PLACEMENT_3D ( 'NONE', #77718, #14137, #35012 ) ;
#33263=CARTESIAN_POINT ( 'NONE',  ( 73.06670390244801183, -48.82844715994099971, 250.9178068554160461 ) ) ;
#33264=CARTESIAN_POINT ( 'NONE',  ( 41.56648329127399677, 0.2215528400590013880, 18.92562527591200094 ) ) ;
#33265=CARTESIAN_POINT ( 'NONE',  ( 118.1851208724672233, -36.91582462397655462, 153.8127681330539644 ) ) ;
#33267=EDGE_LOOP ( 'NONE', ( #37896, #15743, #32130, #31786, #9963 ) ) ;
#33268=AXIS2_PLACEMENT_3D ( 'NONE', #62598, #33104, #88534 ) ;
#33269=CARTESIAN_POINT ( 'NONE',  ( 107.8137748826309377, -27.36365403737595159, 111.4568214011349738 ) ) ;
#33270=CIRCLE ( 'NONE', #50641, 0.5000000000000004441 ) ;
#33271=DIRECTION ( 'NONE',  ( -0.9999999853157766072, -0.0001713722456126752025, 0.000000000000000000 ) ) ;
#33272=CARTESIAN_POINT ( 'NONE',  ( 106.1957191385480854, -47.06291487533366080, 258.4975300378154088 ) ) ;
#33273=FACE_OUTER_BOUND ( 'NONE', #25596, .T. ) ;
#33275=ADVANCED_FACE ( 'NONE', ( #53710 ), #66465, .T. ) ;
#33276=EDGE_CURVE ( 'NONE', #1529, #68029, #82001, .T. ) ;
#33278=CIRCLE ( 'NONE', #20253, 0.5000000000000129896 ) ;
#33279=CYLINDRICAL_SURFACE ( 'NONE', #73962, 2.750000000000002665 ) ;
#33280=ADVANCED_FACE ( 'NONE', ( #560, #68718 ), #42330, .T. ) ;
#33282=CARTESIAN_POINT ( 'NONE',  ( 113.0097079652340568, -45.31096836313454190, 203.0584824187679374 ) ) ;
#33284=ORIENTED_EDGE ( 'NONE', *, *, #78133, .F. ) ;
#33285=ORIENTED_EDGE ( 'NONE', *, *, #51013, .F. ) ;
#33286=EDGE_CURVE ( 'NONE', #53618, #33391, #49143, .T. ) ;
#33287=DIRECTION ( 'NONE',  ( -3.418174336900117128E-15, -1.000000000000000000, 0.000000000000000000 ) ) ;
#33289=AXIS2_PLACEMENT_3D ( 'NONE', #25183, #66516, #58798 ) ;
#33290=CARTESIAN_POINT ( 'NONE',  ( 99.09593196240410862, -30.55013448537800258, 185.8027427927754047 ) ) ;
#33291=FACE_OUTER_BOUND ( 'NONE', #51178, .T. ) ;
#33292=DIRECTION ( 'NONE',  ( 0.000000000000000000, 0.000000000000000000, 1.000000000000000000 ) ) ;
#33294=CYLINDRICAL_SURFACE ( 'NONE', #20484, 9.999999999999998224 ) ;
#33295=CARTESIAN_POINT ( 'NONE',  ( 103.3034881226635946, -27.00695273605797908, 215.3699109901969848 ) ) ;
#33296=CARTESIAN_POINT ( 'NONE',  ( 51.03742451361726751, -23.42844715994066362, 300.4678068554150059 ) ) ;
#33298=ADVANCED_FACE ( 'NONE', ( #28726 ), #89618, .T. ) ;
#33300=CARTESIAN_POINT ( 'NONE',  ( 126.8164832912740394, -54.62589567669621005, -5.074374724089010691 ) ) ;
#33301=LINE ( 'NONE', #60998, #50710 ) ;
#33303=CARTESIAN_POINT ( 'NONE',  ( 101.9087497524793804, -29.77971984236790703, 33.41475703625796001 ) ) ;
#33304=CARTESIAN_POINT ( 'NONE',  ( 114.7420861883949215, -43.81622209775510157, 119.2327681330539804 ) ) ;
#33306=VERTEX_POINT ( 'NONE', #27375 ) ;
#33307=FACE_OUTER_BOUND ( 'NONE', #6593, .T. ) ;
#33308=VECTOR ( 'NONE', #65459, 1000.000000000000000 ) ;
#33309=CARTESIAN_POINT ( 'NONE',  ( 82.26522136039946531, -17.07517613920460420, 7.387586420634624673 ) ) ;
#33310=ORIENTED_EDGE ( 'NONE', *, *, #80984, .T. ) ;
#33314=ORIENTED_EDGE ( 'NONE', *, *, #77635, .T. ) ;
#33315=DIRECTION ( 'NONE',  ( -1.000000000000000000, -8.163404592831600092E-16, -1.020425574103949962E-15 ) ) ;
#33316=CARTESIAN_POINT ( 'NONE',  ( 107.2750367832685043, -27.67576416532946126, 74.46861030426799744 ) ) ;
#33317=CARTESIAN_POINT ( 'NONE',  ( 103.9326413674837539, -26.76323430032771000, 250.3184824187677577 ) ) ;
#33319=CARTESIAN_POINT ( 'NONE',  ( 98.27975524859421341, -42.29919363830190804, 186.7756252759109543 ) ) ;
#33320=CARTESIAN_POINT ( 'NONE',  ( 180.2121375201600131, -29.73316016639650172, -5.074374724088000832 ) ) ;
#33321=CARTESIAN_POINT ( 'NONE',  ( 104.2468583329775811, -46.74335657891433726, 18.35848241876792031 ) ) ;
#33322=FACE_OUTER_BOUND ( 'NONE', #16263, .T. ) ;
#33323=DIRECTION ( 'NONE',  ( -8.568612280633850929E-05, 0.4999999926578935772, -0.8660254037844357100 ) ) ;
#33324=AXIS2_PLACEMENT_3D ( 'NONE', #66527, #72902, #30678 ) ;
#33325=EDGE_LOOP ( 'NONE', ( #42955, #19224, #39099, #3991 ) ) ;
#33326=EDGE_CURVE ( 'NONE', #84820, #28975, #41436, .T. ) ;
#33327=VECTOR ( 'NONE', #79832, 1000.000000000000000 ) ;
#33328=AXIS2_PLACEMENT_3D ( 'NONE', #28379, #42890, #70624 ) ;
#33330=CARTESIAN_POINT ( 'NONE',  ( 110.2694181837619141, -26.72479813065621812, 234.8299109901969643 ) ) ;
#33332=CARTESIAN_POINT ( 'NONE',  ( 115.0397999656063917, -29.07403674218411638, 189.4232443235299570 ) ) ;
#33333=FACE_OUTER_BOUND ( 'NONE', #50523, .T. ) ;
#33335=CARTESIAN_POINT ( 'NONE',  ( 108.3326240688572994, -46.73495791008426892, 23.67722514622035490 ) ) ;
#33336=DIRECTION ( 'NONE',  ( -0.7071067811865779928, 0.7071067811865171526, -7.071067811865786933E-16 ) ) ;
#33337=CARTESIAN_POINT ( 'NONE',  ( 114.8103026587852042, -34.36884736280054398, 277.6356252759111953 ) ) ;
#33338=CYLINDRICAL_SURFACE ( 'NONE', #42733, 0.4999999999999932832 ) ;
#33339=CARTESIAN_POINT ( 'NONE',  ( 98.04139480429049058, -41.04159787523226299, 172.6811693813438637 ) ) ;
#33341=CARTESIAN_POINT ( 'NONE',  ( 134.0664832912740110, -46.72944715994100306, 10.72562527591099801 ) ) ;
#33343=DIRECTION ( 'NONE',  ( 1.000000000000000078E-15, 1.000000000000000083E-30, -1.000000000000000000 ) ) ;
#33344=CARTESIAN_POINT ( 'NONE',  ( 41.56648329127499153, -32.07844715994070839, 198.9256252759119832 ) ) ;
#33345=PLANE ( 'NONE',  #69544 ) ;
#33346=CARTESIAN_POINT ( 'NONE',  ( 101.1158614047228070, -28.69863163947533735, 195.5838086201111992 ) ) ;
#33348=CARTESIAN_POINT ( 'NONE',  ( 136.7703230406665398, -19.23127003359448395, 6.817519769821157816 ) ) ;
#33349=CARTESIAN_POINT ( 'NONE',  ( 117.2491520020922451, -41.08934384016853869, 213.5165776568629781 ) ) ;
#33350=CARTESIAN_POINT ( 'NONE',  ( 117.1064219673475719, -39.53695830471063744, 94.60991099019693706 ) ) ;
#33351=CARTESIAN_POINT ( 'NONE',  ( 117.4730440113279855, -35.59081861377887179, 274.9127681330539872 ) ) ;
#33352=CARTESIAN_POINT ( 'NONE',  ( 107.0664832912739399, -48.18858441225130917, 309.2406250056037038 ) ) ;
#33353=AXIS2_PLACEMENT_3D ( 'NONE', #44464, #26159, #53829 ) ;
#33354=FACE_OUTER_BOUND ( 'NONE', #12484, .T. ) ;
#33355=DIRECTION ( 'NONE',  ( 0.000000000000000000, 0.000000000000000000, 1.000000000000000000 ) ) ;
#33356=DIRECTION ( 'NONE',  ( -4.237773401492740281E-14, 1.000000000000000000, 0.000000000000000000 ) ) ;
#33357=CARTESIAN_POINT ( 'NONE',  ( 48.45959712127249475, -26.00627455219082407, 117.4678068554150485 ) ) ;
#33358=CARTESIAN_POINT ( 'NONE',  ( 29.56670390244828184, -48.82844715994152551, 300.4678068554150059 ) ) ;
#33360=ORIENTED_EDGE ( 'NONE', *, *, #31360, .F. ) ;
#33363=CARTESIAN_POINT ( 'NONE',  ( 98.01111206384085506, -36.61009632703314765, 155.7505150661719995 ) ) ;
#33366=CARTESIAN_POINT ( 'NONE',  ( 188.5667039024479834, -48.82844715994099971, 254.4678068554150343 ) ) ;
#33367=CARTESIAN_POINT ( 'NONE',  ( 102.0922439024871551, -27.59239485085799970, 141.4727681330539895 ) ) ;
#33368=DIRECTION ( 'NONE',  ( 0.000000000000000000, 0.000000000000000000, 1.000000000000000000 ) ) ;
#33369=DIRECTION ( 'NONE',  ( -1.000000000000000000, -4.299999999999999979E-14, -1.000000000000000078E-15 ) ) ;
#33372=CARTESIAN_POINT ( 'NONE',  ( 110.2470682213182869, -46.59973918892936240, 57.83657765686300678 ) ) ;
#33374=VECTOR ( 'NONE', #79106, 1000.000000000000000 ) ;
#33375=ORIENTED_EDGE ( 'NONE', *, *, #52235, .T. ) ;
#33376=VERTEX_POINT ( 'NONE', #34637 ) ;
#33378=CARTESIAN_POINT ( 'NONE',  ( 98.71823956546970180, -31.63334453281608916, 166.8899109901959719 ) ) ;
#33382=ADVANCED_FACE ( 'NONE', ( #61887 ), #55054, .F. ) ;
#33383=DIRECTION ( 'NONE',  ( -1.000000000000000000, -8.843517682682131024E-16, -1.000000000000000078E-15 ) ) ;
#33386=CARTESIAN_POINT ( 'NONE',  ( 109.6427116155909545, -46.48016239540778827, 178.7814341963612605 ) ) ;
#33387=CARTESIAN_POINT ( 'NONE',  ( 98.87507392487043489, -43.19978241230797522, 91.85848241876892928 ) ) ;
#33388=EDGE_LOOP ( 'NONE', ( #10245, #80473, #16317, #18217, #58243 ) ) ;
#33389=EDGE_CURVE ( 'NONE', #79084, #2549, #15100, .T. ) ;
#33391=VERTEX_POINT ( 'NONE', #48693 ) ;
#33392=VECTOR ( 'NONE', #14714, 1000.000000000000114 ) ;
#33394=CYLINDRICAL_SURFACE ( 'NONE', #27058, 9.999999999999998224 ) ;
#33396=CARTESIAN_POINT ( 'NONE',  ( 53.56670390244786262, -48.82844715994099971, 180.4678068554151196 ) ) ;
#33397=CARTESIAN_POINT ( 'NONE',  ( 109.2506105747909828, -28.86437792779224409, 172.6795189410199498 ) ) ;
#33398=VECTOR ( 'NONE', #10102, 1000.000000000000000 ) ;
#33400=ORIENTED_EDGE ( 'NONE', *, *, #40284, .F. ) ;
#33402=VERTEX_POINT ( 'NONE', #13311 ) ;
#33403=EDGE_CURVE ( 'NONE', #32600, #4876, #70517, .T. ) ;
#33404=VECTOR ( 'NONE', #37231, 1000.000000000000000 ) ;
#33405=LINE ( 'NONE', #68382, #68519 ) ;
#33406=FACE_OUTER_BOUND ( 'NONE', #82802, .T. ) ;
#33407=VERTEX_POINT ( 'NONE', #123 ) ;
#33409=EDGE_CURVE ( 'NONE', #79637, #68056, #6502, .T. ) ;
#33410=CARTESIAN_POINT ( 'NONE',  ( 41.56648329127398966, -27.82844715994070484, 258.9256252759120116 ) ) ;
#33411=CARTESIAN_POINT ( 'NONE',  ( 112.1951879357659152, -44.60173489647391420, 219.4796785439919802 ) ) ;
#33415=ORIENTED_EDGE ( 'NONE', *, *, #32362, .T. ) ;
#33417=CARTESIAN_POINT ( 'NONE',  ( 141.8664832912739939, -71.52944715994085811, 361.9756252759100335 ) ) ;
#33420=VECTOR ( 'NONE', #64473, 1000.000000000000114 ) ;
#33421=CARTESIAN_POINT ( 'NONE',  ( 110.2461554203946292, -29.21150786992351911, 242.5766617981629452 ) ) ;
#33422=CARTESIAN_POINT ( 'NONE',  ( 98.13060510664840308, -43.27509626496242134, 106.8175300378159704 ) ) ;
#33423=CARTESIAN_POINT ( 'NONE',  ( 117.9019101119220068, -41.46671778014666643, 58.49848241876792798 ) ) ;
#33424=CARTESIAN_POINT ( 'NONE',  ( 115.9130035588905798, -40.24476411946300658, 249.5838068554177482 ) ) ;
#33425=CARTESIAN_POINT ( 'NONE',  ( 132.1570028294955819, -16.74831852143706712, 7.618261863063341188 ) ) ;
#33426=CARTESIAN_POINT ( 'NONE',  ( 107.4813127257300636, -25.27694550238891580, 320.8178638332907440 ) ) ;
#33427=CARTESIAN_POINT ( 'NONE',  ( 97.05822270422260090, -41.42079030513556859, 207.6632443235299661 ) ) ;
#33430=CARTESIAN_POINT ( 'NONE',  ( 19.56648329127400032, -18.82844715994099971, -5.074374724088000832 ) ) ;
#33431=ORIENTED_EDGE ( 'NONE', *, *, #24447, .F. ) ;
#33433=DIRECTION ( 'NONE',  ( -1.000000000000000000, -4.299999999999999979E-14, -1.000000000000000078E-15 ) ) ;
#33434=VECTOR ( 'NONE', #11729, 1000.000000000000000 ) ;
#33437=CARTESIAN_POINT ( 'NONE',  ( 112.1361961822399707, -28.01101909465306150, 90.65674523166063636 ) ) ;
#33438=CARTESIAN_POINT ( 'NONE',  ( 113.3148160382734773, -28.33991531616941728, 104.5670538473399347 ) ) ;
#33439=CARTESIAN_POINT ( 'NONE',  ( 109.7287940957687908, -27.00184760396491868, 254.8647456037904533 ) ) ;
#33440=EDGE_CURVE ( 'NONE', #38972, #5327, #55500, .T. ) ;
#33441=CARTESIAN_POINT ( 'NONE',  ( 88.24325903289653183, -55.55267141831875222, -4.824374724089048883 ) ) ;
#33442=LINE ( 'NONE', #13012, #52752 ) ;
#33445=CARTESIAN_POINT ( 'NONE',  ( 97.07914014679033698, -41.41098531455288168, 207.6632443235299661 ) ) ;
#33446=CARTESIAN_POINT ( 'NONE',  ( 177.0371591254543375, -48.62818131005480637, 300.4678068554149490 ) ) ;
#33447=CARTESIAN_POINT ( 'NONE',  ( 165.9667039024476765, -26.71338133338628040, 117.4678068554150485 ) ) ;
#33448=ORIENTED_EDGE ( 'NONE', *, *, #54174, .F. ) ;
#33449=CARTESIAN_POINT ( 'NONE',  ( 163.0959832912772356, -23.42844715993520310, 193.9678068554149775 ) ) ;
#33452=AXIS2_PLACEMENT_3D ( 'NONE', #68112, #74478, #32233 ) ;
#33453=CARTESIAN_POINT ( 'NONE',  ( 37.36643805256671413, -48.62818131006120836, 300.4678068554150059 ) ) ;
#33454=CARTESIAN_POINT ( 'NONE',  ( 99.50747941120199869, -29.43470559729854230, 250.7156252759109520 ) ) ;
#33456=FACE_OUTER_BOUND ( 'NONE', #35313, .T. ) ;
#33457=CARTESIAN_POINT ( 'NONE',  ( 96.68927247633037325, -32.92320750051204215, 17.03467289495896964 ) ) ;
#33458=CARTESIAN_POINT ( 'NONE',  ( 102.8960693947464051, -27.08911147246314499, 151.4013395616249511 ) ) ;
#33459=PLANE ( 'NONE',  #40329 ) ;
#33460=CARTESIAN_POINT ( 'NONE',  ( 102.0672082652289419, -27.97040743572448562, 101.4897538293649006 ) ) ;
#33463=CARTESIAN_POINT ( 'NONE',  ( 100.9546728717598540, -28.70702568209258843, 190.5939586032972670 ) ) ;
#33464=LINE ( 'NONE', #5774, #75587 ) ;
#33465=VERTEX_POINT ( 'NONE', #56412 ) ;
#33467=EDGE_CURVE ( 'NONE', #82508, #65069, #67447, .T. ) ;
#33468=VERTEX_POINT ( 'NONE', #1479 ) ;
#33469=ORIENTED_EDGE ( 'NONE', *, *, #56729, .T. ) ;
#33471=ORIENTED_EDGE ( 'NONE', *, *, #3195, .T. ) ;
#33472=PLANE ( 'NONE',  #53785 ) ;
#33473=CARTESIAN_POINT ( 'NONE',  ( 104.7405551043178633, -47.51155644559842273, 28.41943479971997988 ) ) ;
#33474=DIRECTION ( 'NONE',  ( 0.000000000000000000, 0.000000000000000000, -1.000000000000000000 ) ) ;
#33478=CARTESIAN_POINT ( 'NONE',  ( 114.2672205647202048, -43.24251175450689288, 232.6638483995059801 ) ) ;
#33480=ORIENTED_EDGE ( 'NONE', *, *, #26740, .F. ) ;
#33485=CARTESIAN_POINT ( 'NONE',  ( 63.06670390244645574, -24.92844715994017335, 129.9678068554150911 ) ) ;
#33486=CARTESIAN_POINT ( 'NONE',  ( 179.1667039024460166, -28.27351298637280408, -5.074374724088000832 ) ) ;
#33487=CARTESIAN_POINT ( 'NONE',  ( 111.8905564713631549, -28.66688903671830246, 51.09110711541997318 ) ) ;
#33488=AXIS2_PLACEMENT_3D ( 'NONE', #85063, #37339, #56873 ) ;
#33489=DIRECTION ( 'NONE',  ( 0.000000000000000000, 0.000000000000000000, -1.000000000000000000 ) ) ;
#33492=CARTESIAN_POINT ( 'NONE',  ( 116.0161715043950466, -40.67488961668907166, 253.4956252759109532 ) ) ;
#33494=EDGE_CURVE ( 'NONE', #30523, #62685, #36447, .T. ) ;
#33495=CYLINDRICAL_SURFACE ( 'NONE', #55950, 2.500000000000002220 ) ;
#33497=CARTESIAN_POINT ( 'NONE',  ( 162.7131505118539962, -33.70561438052111214, -5.074374724088000832 ) ) ;
#33500=CARTESIAN_POINT ( 'NONE',  ( 99.41042786952979782, -33.89845062227509231, 63.86237608387695985 ) ) ;
#33504=DIRECTION ( 'NONE',  ( -0.9999999853157766072, -0.0001713722456134502174, 0.000000000000000000 ) ) ;
#33505=VERTEX_POINT ( 'NONE', #78246 ) ;
#33508=EDGE_LOOP ( 'NONE', ( #51210, #11731, #84301, #3883, #59650, #67365 ) ) ;
#33509=CARTESIAN_POINT ( 'NONE',  ( 99.42196222650996162, -27.67359991961172128, 150.6356252759109680 ) ) ;
#33512=CARTESIAN_POINT ( 'NONE',  ( 104.7294611837924094, -27.30559681290521112, 89.69241982807696445 ) ) ;
#33514=LINE ( 'NONE', #61215, #15591 ) ;
#33515=CARTESIAN_POINT ( 'NONE',  ( 100.0737993132363783, -29.47871783549896918, 112.1187261630399661 ) ) ;
#33516=CYLINDRICAL_SURFACE ( 'NONE', #1098, 2.500000000000002220 ) ;
#33517=EDGE_CURVE ( 'NONE', #73231, #37163, #23478, .T. ) ;
#33518=CARTESIAN_POINT ( 'NONE',  ( 63.06670390244732971, -24.92844715994017690, 300.4678068554150627 ) ) ;
#33519=CARTESIAN_POINT ( 'NONE',  ( 110.4636787236150184, -47.27194539037950705, 53.83657765686300678 ) ) ;
#33522=CARTESIAN_POINT ( 'NONE',  ( 182.2738106836200132, -23.19206098993950604, 342.9256252759119548 ) ) ;
#33523=VERTEX_POINT ( 'NONE', #77781 ) ;
#33525=ORIENTED_EDGE ( 'NONE', *, *, #4141, .F. ) ;
#33526=EDGE_LOOP ( 'NONE', ( #68614, #24269, #29070, #8535 ) ) ;
#33527=VECTOR ( 'NONE', #47275, 999.9999999999998863 ) ;
#33529=EDGE_LOOP ( 'NONE', ( #5129, #31835 ) ) ;
#33530=CARTESIAN_POINT ( 'NONE',  ( 106.1957191385480570, -47.06291487533376028, 262.4975300378164320 ) ) ;
#33531=CARTESIAN_POINT ( 'NONE',  ( 105.7176149122623485, -24.93101994221251516, 156.1670538473399574 ) ) ;
#33533=DIRECTION ( 'NONE',  ( 0.000000000000000000, 0.000000000000000000, 1.000000000000000000 ) ) ;
#33534=CARTESIAN_POINT ( 'NONE',  ( 117.3534687869931048, -38.62661931536851512, 84.68133956162593279 ) ) ;
#33538=DIRECTION ( 'NONE',  ( -1.000000000000000000, -6.814610998690690172E-14, -1.000000000000000078E-15 ) ) ;
#33539=CARTESIAN_POINT ( 'NONE',  ( 117.0718120722267628, -35.46179131731675227, 159.9271957950691956 ) ) ;
#33540=ORIENTED_EDGE ( 'NONE', *, *, #72266, .F. ) ;
#33542=FACE_OUTER_BOUND ( 'NONE', #53977, .T. ) ;
#33543=CARTESIAN_POINT ( 'NONE',  ( 105.1131368864170241, -25.87365329830167937, 275.2061014663871674 ) ) ;
#33544=LINE ( 'NONE', #28065, #88160 ) ;
#33546=CARTESIAN_POINT ( 'NONE',  ( 116.3137647483393806, -32.94861263809731611, 185.1356252759109680 ) ) ;
#33547=CARTESIAN_POINT ( 'NONE',  ( 105.0359719168109933, -28.43277227512634298, 284.6895626852196415 ) ) ;
#33548=PLANE ( 'NONE',  #34756 ) ;
#33549=CARTESIAN_POINT ( 'NONE',  ( 102.6254653968536417, -46.82603978519634325, 128.2346728949589760 ) ) ;
#33550=PLANE ( 'NONE',  #19014 ) ;
#33551=CARTESIAN_POINT ( 'NONE',  ( 108.2829496674670224, -47.76277978039057359, 157.6518157521019532 ) ) ;
#33552=VERTEX_POINT ( 'NONE', #71421 ) ;
#33556=VECTOR ( 'NONE', #36397, 1000.000000000000000 ) ;
#33557=CARTESIAN_POINT ( 'NONE',  ( 188.5667039024479834, -62.87844715994099687, 293.2178068554150627 ) ) ;
#33558=CARTESIAN_POINT ( 'NONE',  ( 136.7325000480765311, -36.03188439719874481, 2.979900720422823390 ) ) ;
#33559=ORIENTED_EDGE ( 'NONE', *, *, #6422, .T. ) ;
#33561=CARTESIAN_POINT ( 'NONE',  ( 99.06758658495417080, -45.54097539030503583, 156.9899109901969609 ) ) ;
#33566=VECTOR ( 'NONE', #1858, 1000.000000000000000 ) ;
#33567=FACE_OUTER_BOUND ( 'NONE', #68813, .T. ) ;
#33568=DIRECTION ( 'NONE',  ( 1.000000000000000000, 4.299999999999999979E-14, 1.000000000000000078E-15 ) ) ;
#33569=ORIENTED_EDGE ( 'NONE', *, *, #38191, .F. ) ;
#33570=AXIS2_PLACEMENT_3D ( 'NONE', #46586, #24825, #52490 ) ;
#33571=EDGE_CURVE ( 'NONE', #82307, #71390, #15558, .T. ) ;
#33575=EDGE_CURVE ( 'NONE', #31161, #20465, #57768, .T. ) ;
#33577=DIRECTION ( 'NONE',  ( -2.900000000000000265E-14, 2.000000000000000155E-15, -1.000000000000000000 ) ) ;
#33578=CARTESIAN_POINT ( 'NONE',  ( 105.7386178790360418, -26.75993881439924138, 250.1823171237273584 ) ) ;
#33579=PLANE ( 'NONE',  #43973 ) ;
#33580=CYLINDRICAL_SURFACE ( 'NONE', #29944, 3.000000000000002665 ) ;
#33581=ADVANCED_FACE ( 'NONE', ( #50950 ), #71859, .T. ) ;
#33583=ADVANCED_FACE ( 'NONE', ( #59537 ), #74530, .F. ) ;
#33584=CARTESIAN_POINT ( 'NONE',  ( 108.4172366116780637, -26.73500384902263960, 104.9689787242619019 ) ) ;
#33586=CARTESIAN_POINT ( 'NONE',  ( 105.7993493439852699, -26.72405417386548265, 180.1773053279698331 ) ) ;
#33588=EDGE_CURVE ( 'NONE', #50227, #57751, #53099, .T. ) ;
#33589=ORIENTED_EDGE ( 'NONE', *, *, #78526, .T. ) ;
#33590=DIRECTION ( 'NONE',  ( -0.000000000000000000, 1.000000000000000000, 0.000000000000000000 ) ) ;
#33591=DIRECTION ( 'NONE',  ( 0.000000000000000000, 0.000000000000000000, 1.000000000000000000 ) ) ;
#33592=ADVANCED_FACE ( 'NONE', ( #67715 ), #73631, .T. ) ;
#33593=CARTESIAN_POINT ( 'NONE',  ( 106.5196382177907140, -25.62481104856566105, 191.1156252759109861 ) ) ;
#33596=ORIENTED_EDGE ( 'NONE', *, *, #35121, .T. ) ;
#33597=CARTESIAN_POINT ( 'NONE',  ( 102.0112516875887678, -27.67497761899955933, 101.4937205140059575 ) ) ;
#33598=EDGE_CURVE ( 'NONE', #18234, #76080, #88623, .T. ) ;
#33599=CARTESIAN_POINT ( 'NONE',  ( 32.06670390244668312, -32.29483332968541731, 237.4678068554150059 ) ) ;
#33600=CARTESIAN_POINT ( 'NONE',  ( 116.3265979651016409, -32.94445627519164077, 14.13562527591094664 ) ) ;
#33603=DIRECTION ( 'NONE',  ( 0.000000000000000000, 0.000000000000000000, 1.000000000000000000 ) ) ;
#33606=ORIENTED_EDGE ( 'NONE', *, *, #45028, .F. ) ;
#33607=ORIENTED_EDGE ( 'NONE', *, *, #39096, .T. ) ;
#33608=CARTESIAN_POINT ( 'NONE',  ( 107.2218274976867463, -26.65737820016106951, 226.4958690201829654 ) ) ;
#33609=CARTESIAN_POINT ( 'NONE',  ( 99.50484159579329457, -43.30592805723910033, 52.89564321832823879 ) ) ;
#33611=CARTESIAN_POINT ( 'NONE',  ( 117.0718954875924851, -35.46248236815851840, 154.9272919416320065 ) ) ;
#33613=VECTOR ( 'NONE', #23224, 1000.000000000000000 ) ;
#33617=DIRECTION ( 'NONE',  ( 0.000000000000000000, -1.000000000000000000, 0.000000000000000000 ) ) ;
#33618=VERTEX_POINT ( 'NONE', #19560 ) ;
#33619=CARTESIAN_POINT ( 'NONE',  ( 100.5975332644244844, -28.50897509465477597, 15.60705384733995871 ) ) ;
#33620=ORIENTED_EDGE ( 'NONE', *, *, #42716, .F. ) ;
#33621=ADVANCED_FACE ( 'NONE', ( #33195 ), #5501, .F. ) ;
#33622=CARTESIAN_POINT ( 'NONE',  ( 102.8259602516037177, -43.70423678882019658, 244.9595189410199794 ) ) ;
#33624=DIRECTION ( 'NONE',  ( -0.000000000000000000, -0.000000000000000000, 1.000000000000000000 ) ) ;
#33625=CARTESIAN_POINT ( 'NONE',  ( 117.0460787713799817, -39.54838250520750620, 143.6194347997209775 ) ) ;
#33627=CYLINDRICAL_SURFACE ( 'NONE', #63600, 9.999999999999998224 ) ;
#33628=CARTESIAN_POINT ( 'NONE',  ( 34.67381068360400320, -28.98061976758901892, -5.074374724088000832 ) ) ;
#33629=EDGE_CURVE ( 'NONE', #51052, #8294, #34041, .T. ) ;
#33632=CARTESIAN_POINT ( 'NONE',  ( 100.7237713325202861, -45.83809708005067307, 233.0803871806729717 ) ) ;
#33634=VERTEX_POINT ( 'NONE', #40451 ) ;
#33636=CARTESIAN_POINT ( 'NONE',  ( 98.55462967347544634, -43.85305904914448405, 67.86895860924497015 ) ) ;
#33637=CARTESIAN_POINT ( 'NONE',  ( 25.56670390244797275, -48.82844715994099971, 257.2178068554150059 ) ) ;
#33638=ORIENTED_EDGE ( 'NONE', *, *, #6719, .F. ) ;
#33641=CARTESIAN_POINT ( 'NONE',  ( 97.33768314765580953, -34.07170803572739715, 161.1146346061390204 ) ) ;
#33644=FACE_OUTER_BOUND ( 'NONE', #58650, .T. ) ;
#33645=CARTESIAN_POINT ( 'NONE',  ( 115.4711811475381467, -34.66499115051416169, 161.8242808457819706 ) ) ;
#33646=CARTESIAN_POINT ( 'NONE',  ( 96.74182981399745529, -35.13608925046722220, 262.2041967044821149 ) ) ;
#33647=VECTOR ( 'NONE', #53361, 1000.000000000000000 ) ;
#33649=ORIENTED_EDGE ( 'NONE', *, *, #59260, .F. ) ;
#33650=CARTESIAN_POINT ( 'NONE',  ( 162.7131505118539962, -33.70561438052110503, 342.9256252759109884 ) ) ;
#33651=LINE ( 'NONE', #20030, #56300 ) ;
#33652=ORIENTED_EDGE ( 'NONE', *, *, #74809, .F. ) ;
#33653=CIRCLE ( 'NONE', #4608, 0.9999999999999800160 ) ;
#33654=ORIENTED_EDGE ( 'NONE', *, *, #24979, .F. ) ;
#33656=PLANE ( 'NONE',  #5353 ) ;
#33657=ORIENTED_EDGE ( 'NONE', *, *, #306, .T. ) ;
#33658=VERTEX_POINT ( 'NONE', #61333 ) ;
#33660=DIRECTION ( 'NONE',  ( 1.000000000000000000, 4.163336342344333240E-14, 0.000000000000000000 ) ) ;
#33662=CARTESIAN_POINT ( 'NONE',  ( 100.1253875378072848, -39.57043109886186727, 9.635625275910941312 ) ) ;
#33663=CARTESIAN_POINT ( 'NONE',  ( 113.1794296094924874, -30.05060732774411036, 153.8971817328389875 ) ) ;
#33665=CARTESIAN_POINT ( 'NONE',  ( 97.76994516709639527, -29.29956314839395048, 45.78991099019697231 ) ) ;
#33666=CARTESIAN_POINT ( 'NONE',  ( 162.7131505118553321, -33.70561438051485936, 193.9678068554149775 ) ) ;
#33667=ORIENTED_EDGE ( 'NONE', *, *, #41864, .F. ) ;
#33669=AXIS2_PLACEMENT_3D ( 'NONE', #48731, #42818, #6979 ) ;
#33671=FACE_OUTER_BOUND ( 'NONE', #79051, .T. ) ;
#33672=ORIENTED_EDGE ( 'NONE', *, *, #73310, .T. ) ;
#33673=DIRECTION ( 'NONE',  ( 0.000000000000000000, 0.000000000000000000, 1.000000000000000000 ) ) ;
#33675=CARTESIAN_POINT ( 'NONE',  ( 108.3322807220838655, -46.73499201940651204, 132.6772426970024128 ) ) ;
#33676=CARTESIAN_POINT ( 'NONE',  ( 45.77381068356854144, -48.62134037881681081, 129.9678068554150911 ) ) ;
#33677=EDGE_LOOP ( 'NONE', ( #17873, #26054 ) ) ;
#33678=CARTESIAN_POINT ( 'NONE',  ( 112.9757402841042904, -28.11393523324086985, 44.59848241876795782 ) ) ;
#33679=CARTESIAN_POINT ( 'NONE',  ( 116.7149026195978792, -32.57661448200846621, 75.14991099019697174 ) ) ;
#33683=CARTESIAN_POINT ( 'NONE',  ( 86.06670390244796920, -50.82844715994100682, 10.91780685541499807 ) ) ;
#33685=ADVANCED_FACE ( 'NONE', ( #68171 ), #87711, .F. ) ;
#33686=CARTESIAN_POINT ( 'NONE',  ( 132.0298243561156539, -16.87939921900816387, 2.327894594454689603 ) ) ;
#33687=VERTEX_POINT ( 'NONE', #39554 ) ;
#33690=DIRECTION ( 'NONE',  ( 0.000000000000000000, 0.000000000000000000, -1.000000000000000000 ) ) ;
#33691=PLANE ( 'NONE',  #39753 ) ;
#33692=EDGE_CURVE ( 'NONE', #40190, #71887, #64547, .T. ) ;
#33693=ORIENTED_EDGE ( 'NONE', *, *, #28549, .T. ) ;
#33694=CARTESIAN_POINT ( 'NONE',  ( 96.63486483157898022, -37.29388950852173679, 72.36991099019596163 ) ) ;
#33695=VECTOR ( 'NONE', #27105, 1000.000000000000114 ) ;
#33696=CARTESIAN_POINT ( 'NONE',  ( 194.5664832912739826, 15.62155284005900491, 323.8756252759109202 ) ) ;
#33697=DIRECTION ( 'NONE',  ( 4.194175870806139918E-14, -1.000000000000000000, 0.000000000000000000 ) ) ;
#33698=DIRECTION ( 'NONE',  ( 0.000000000000000000, 0.000000000000000000, -1.000000000000000000 ) ) ;
#33699=ADVANCED_FACE ( 'NONE', ( #59981 ), #25038, .T. ) ;
#33700=AXIS2_PLACEMENT_3D ( 'NONE', #39758, #67471, #38869 ) ;
#33701=CARTESIAN_POINT ( 'NONE',  ( 36.65249034007445772, -49.32844715994130524, 180.4678068554150911 ) ) ;
#33702=ORIENTED_EDGE ( 'NONE', *, *, #86017, .F. ) ;
#33704=CARTESIAN_POINT ( 'NONE',  ( 109.6029845306728134, -46.78454271877401283, 88.78514908543394313 ) ) ;
#33706=VERTEX_POINT ( 'NONE', #60436 ) ;
#33707=CARTESIAN_POINT ( 'NONE',  ( 115.6772654923306902, -42.56752007954064965, 269.3527681330536439 ) ) ;
#33711=DIRECTION ( 'NONE',  ( 0.000000000000000000, 0.000000000000000000, -1.000000000000000000 ) ) ;
#33714=DIRECTION ( 'NONE',  ( 1.000000000000000000, 4.101809204280141026E-14, 0.000000000000000000 ) ) ;
#33715=DIRECTION ( 'NONE',  ( 1.000000000000000078E-15, -1.000000000000000083E-30, -1.000000000000000000 ) ) ;
#33716=CARTESIAN_POINT ( 'NONE',  ( 98.71823956546961654, -31.63334453281603587, 170.8899109901969950 ) ) ;
#33718=ORIENTED_EDGE ( 'NONE', *, *, #27640, .T. ) ;
#33720=CARTESIAN_POINT ( 'NONE',  ( 100.2558307937446074, -42.39895253252459639, 113.3101547344679574 ) ) ;
#33721=CIRCLE ( 'NONE', #71479, 2.500000000000002220 ) ;
#33722=CARTESIAN_POINT ( 'NONE',  ( 194.5664832912729878, 15.62155284005731204, 361.9756252759109998 ) ) ;
#33723=CARTESIAN_POINT ( 'NONE',  ( 110.5064767540468011, -26.94654216138288660, 250.8194347997200850 ) ) ;
#33724=DIRECTION ( 'NONE',  ( 1.000000000000000000, 4.299999999999999979E-14, 1.000000000000000078E-15 ) ) ;
#33726=VECTOR ( 'NONE', #47052, 1000.000000000000000 ) ;
#33730=CARTESIAN_POINT ( 'NONE',  ( 194.5664832912729878, 25.62155284005700295, 361.9756252759109998 ) ) ;
#33731=CARTESIAN_POINT ( 'NONE',  ( 98.56907362037662779, -44.95393718666142746, 191.9384824187679612 ) ) ;
#33732=FACE_OUTER_BOUND ( 'NONE', #36806, .T. ) ;
#33734=ORIENTED_EDGE ( 'NONE', *, *, #38012, .F. ) ;
#33736=CARTESIAN_POINT ( 'NONE',  ( 80.44329752326743233, -21.47944369576872603, 8.225625303283912615 ) ) ;
#33737=CARTESIAN_POINT ( 'NONE',  ( 115.8259672271617120, -31.73094390465656289, 184.2401262212665642 ) ) ;
#33738=DIRECTION ( 'NONE',  ( -1.000000000000000078E-15, 1.000000000000000083E-30, 1.000000000000000000 ) ) ;
#33740=DIRECTION ( 'NONE',  ( 0.000000000000000000, 1.000000000000000000, 0.000000000000000000 ) ) ;
#33741=ORIENTED_EDGE ( 'NONE', *, *, #47725, .T. ) ;
#33742=CARTESIAN_POINT ( 'NONE',  ( 101.9929316774952497, -45.44564633532985454, 62.15639494301799317 ) ) ;
#33743=CARTESIAN_POINT ( 'NONE',  ( 102.2371489609593880, -45.96874152625851906, 212.1927681330539599 ) ) ;
#33744=ORIENTED_EDGE ( 'NONE', *, *, #7693, .F. ) ;
#33749=CARTESIAN_POINT ( 'NONE',  ( 107.4895849179006575, -45.99858499349326735, 40.43094751244896656 ) ) ;
#33750=CARTESIAN_POINT ( 'NONE',  ( 114.5431187036783740, -28.56067750227894564, 150.4746728949579619 ) ) ;
#33751=CARTESIAN_POINT ( 'NONE',  ( 41.56648329127399677, 0.2215528400590013880, 256.8086252759120498 ) ) ;
#33753=EDGE_CURVE ( 'NONE', #78550, #49825, #39880, .T. ) ;
#33755=CARTESIAN_POINT ( 'NONE',  ( 104.1327126252334665, -46.37477890040964468, 67.34360547614434722 ) ) ;
#33758=EDGE_CURVE ( 'NONE', #34233, #26191, #82263, .T. ) ;
#33759=CARTESIAN_POINT ( 'NONE',  ( 97.81168895331838087, -40.51742574516882200, 287.6356252759109680 ) ) ;
#33760=ORIENTED_EDGE ( 'NONE', *, *, #87447, .T. ) ;
#33763=CARTESIAN_POINT ( 'NONE',  ( 113.5850730991778619, -42.29362625859309333, 62.68670554236294379 ) ) ;
#33764=CARTESIAN_POINT ( 'NONE',  ( 96.75080816152406271, -34.86525579675927844, 241.1841967044819626 ) ) ;
#33765=CARTESIAN_POINT ( 'NONE',  ( 97.42226921825827901, -40.63044708855872500, 206.6327681330539860 ) ) ;
#33766=CARTESIAN_POINT ( 'NONE',  ( 162.8913605087226415, -31.76306994223245539, 237.4678068554150059 ) ) ;
#33767=CARTESIAN_POINT ( 'NONE',  ( 117.4903696573863385, -37.28369426754698424, 14.78419670448294454 ) ) ;
#33769=CARTESIAN_POINT ( 'NONE',  ( 131.0667039024480403, -42.97311385573999587, 207.5838068554170377 ) ) ;
#33771=CARTESIAN_POINT ( 'NONE',  ( 110.8343066518040416, -26.26926122352943338, 99.80133956162498521 ) ) ;
#33772=VECTOR ( 'NONE', #70778, 1000.000000000000000 ) ;
#33773=CARTESIAN_POINT ( 'NONE',  ( 103.9442172157761917, -47.38141121271982570, 62.33753003781600199 ) ) ;
#33774=CARTESIAN_POINT ( 'NONE',  ( 106.1344186357298867, -47.79037565197016590, 262.4975300378158067 ) ) ;
#33775=EDGE_LOOP ( 'NONE', ( #2907, #29785, #66610, #75197 ) ) ;
#33776=CARTESIAN_POINT ( 'NONE',  ( 97.09604340039788895, -41.50117806558871791, 216.6937205140059461 ) ) ;
#33777=DIRECTION ( 'NONE',  ( 1.000000000000000078E-15, -1.000000000000000083E-30, -1.000000000000000000 ) ) ;
#33779=CARTESIAN_POINT ( 'NONE',  ( 115.7825283181106926, -41.80329352439114388, 24.40636741810707733 ) ) ;
#33780=CARTESIAN_POINT ( 'NONE',  ( 113.5891433990094157, -44.41776597164441398, 29.13712086416463976 ) ) ;
#33781=ADVANCED_FACE ( 'NONE', ( #20021 ), #21364, .T. ) ;
#33782=CARTESIAN_POINT ( 'NONE',  ( 111.5783628878732401, -44.33946045148141479, 277.6356252759111953 ) ) ;
#33784=CARTESIAN_POINT ( 'NONE',  ( 117.0608881454332675, -38.08051539367706084, 174.7189536622046546 ) ) ;
#33786=CARTESIAN_POINT ( 'NONE',  ( 106.5656518807525117, -24.23945688555024702, 323.2548426863285727 ) ) ;
#33788=FACE_OUTER_BOUND ( 'NONE', #54666, .T. ) ;
#33789=EDGE_CURVE ( 'NONE', #62770, #22460, #82067, .T. ) ;
#33791=CARTESIAN_POINT ( 'NONE',  ( 109.7166342287432315, -26.99862646155922263, 39.86461898627592149 ) ) ;
#33792=CARTESIAN_POINT ( 'NONE',  ( 100.9546728209955688, -28.70702572003537512, 76.59395860829201297 ) ) ;
#33793=FACE_OUTER_BOUND ( 'NONE', #4823, .T. ) ;
#33797=CARTESIAN_POINT ( 'NONE',  ( 97.45268567403179816, -40.90835349962023315, 231.6527681330539679 ) ) ;
#33798=CARTESIAN_POINT ( 'NONE',  ( 109.5084879329568679, -46.86449036543412205, 128.7641967044819751 ) ) ;
#33799=CARTESIAN_POINT ( 'NONE',  ( 100.2197142693901668, -28.81018370247272742, 256.6441967044821695 ) ) ;
#33800=CARTESIAN_POINT ( 'NONE',  ( 113.2454987156834108, -28.75867295938290624, 154.5522919407626716 ) ) ;
#33803=DIRECTION ( 'NONE',  ( 1.907762142705490052E-15, 7.167082501179359715E-16, -1.000000000000000000 ) ) ;
#33804=LINE ( 'NONE', #33357, #20409 ) ;
#33805=CARTESIAN_POINT ( 'NONE',  ( 132.1570028294930523, -20.71057579844040930, 2.232988688760512375 ) ) ;
#33806=EDGE_CURVE ( 'NONE', #52459, #71638, #49038, .T. ) ;
#33810=EDGE_CURVE ( 'NONE', #59070, #51539, #13207, .T. ) ;
#33811=CARTESIAN_POINT ( 'NONE',  ( 105.6324958909751075, -46.33196107771311745, 146.8809912566479738 ) ) ;
#33815=CARTESIAN_POINT ( 'NONE',  ( 115.8253432708642094, -31.72986461983916939, 89.23953976385652709 ) ) ;
#33816=CARTESIAN_POINT ( 'NONE',  ( 116.8835868046512587, -40.17228670562622739, 129.5584824187679658 ) ) ;
#33817=LINE ( 'NONE', #631, #48244 ) ;
#33818=B_SPLINE_CURVE_WITH_KNOTS ( 'NONE', 3,
 ( #43423, #63438, #62982, #35272, #760, #1224, #28928, #28461, #21673, #49347, #77078, #22126, #6680, #15304, #42971, #34378, #62086, #29824 ),
 .UNSPECIFIED., .F., .F.,
 ( 4, 2, 2, 2, 2, 2, 2, 2, 4 ),
 ( 0.000000000000000000, 0.06250000002945982347, 0.1250000000589196469, 0.1875000000883794704, 0.2500000001178392939, 0.3125000001472991173, 0.3750000001767589408, 0.4375000002062187643, 0.5000000002356785878 ),
 .UNSPECIFIED. ) ;
#33820=CARTESIAN_POINT ( 'NONE',  ( 51.06670390244899238, -32.29483332968430886, 342.9256252759119548 ) ) ;
#33821=LINE ( 'NONE', #88359, #4840 ) ;
#33822=CARTESIAN_POINT ( 'NONE',  ( 96.07333748454163924, -35.06730156692549372, 71.20705384733993526 ) ) ;
#33823=ORIENTED_EDGE ( 'NONE', *, *, #15858, .F. ) ;
#33824=ORIENTED_EDGE ( 'NONE', *, *, #4259, .T. ) ;
#33825=EDGE_LOOP ( 'NONE', ( #69288, #33192, #61622, #40114, #58972, #58919 ) ) ;
#33826=VECTOR ( 'NONE', #18392, 999.9999999999998863 ) ;
#33827=LINE ( 'NONE', #67001, #34174 ) ;
#33828=CARTESIAN_POINT ( 'NONE',  ( 102.0969121991173125, -45.15362633196975395, 158.1527681330539963 ) ) ;
#33829=DIRECTION ( 'NONE',  ( -0.7071067812160279908, 0.7071067811570671546, -6.612322856135836109E-17 ) ) ;
#33830=CARTESIAN_POINT ( 'NONE',  ( 107.0664832912739968, -36.72944715994100306, 287.6356252759109680 ) ) ;
#33832=CARTESIAN_POINT ( 'NONE',  ( 168.3664380525668491, -48.62818131005517586, 129.9678068554150059 ) ) ;
#33834=CARTESIAN_POINT ( 'NONE',  ( 123.6837132603319560, -53.34645651782485487, 229.5838068554170093 ) ) ;
#33835=CARTESIAN_POINT ( 'NONE',  ( 109.7644292386350457, -47.42453529627131559, 92.78514908543495210 ) ) ;
#33836=ORIENTED_EDGE ( 'NONE', *, *, #5420, .T. ) ;
#33838=ORIENTED_EDGE ( 'NONE', *, *, #28361, .T. ) ;
#33839=CARTESIAN_POINT ( 'NONE',  ( 25.56670390244734747, -42.82844715994178131, 139.7178068554150627 ) ) ;
#33840=DIRECTION ( 'NONE',  ( 0.000000000000000000, 0.000000000000000000, -1.000000000000000000 ) ) ;
#33842=EDGE_CURVE ( 'NONE', #43699, #79942, #55847, .T. ) ;
#33843=CARTESIAN_POINT ( 'NONE',  ( 99.78156907347540994, -40.47280301881529851, 194.5223760838769920 ) ) ;
#33845=AXIS2_PLACEMENT_3D ( 'NONE', #89636, #84171, #9203 ) ;
#33847=ORIENTED_EDGE ( 'NONE', *, *, #11179, .F. ) ;
#33850=PLANE ( 'NONE',  #67091 ) ;
#33853=ORIENTED_EDGE ( 'NONE', *, *, #7241, .F. ) ;
#33854=CARTESIAN_POINT ( 'NONE',  ( 77.76062680957342366, -20.22815166920278429, 7.286367513305838095 ) ) ;
#33855=CARTESIAN_POINT ( 'NONE',  ( 115.1079044709731676, -40.52387399376650734, 224.9072975916109840 ) ) ;
#33856=LINE ( 'NONE', #28384, #79880 ) ;
#33858=EDGE_LOOP ( 'NONE', ( #20033, #64483, #44105, #52212 ) ) ;
#33859=ORIENTED_EDGE ( 'NONE', *, *, #26501, .F. ) ;
#33860=EDGE_CURVE ( 'NONE', #31965, #76782, #83597, .T. ) ;
#33861=DIRECTION ( 'NONE',  ( 2.900000000000000265E-14, -2.000000000000000155E-15, 1.000000000000000000 ) ) ;
#33862=AXIS2_PLACEMENT_3D ( 'NONE', #38060, #50789, #17619 ) ;
#33865=CARTESIAN_POINT ( 'NONE',  ( 111.2517653011026226, -44.30469234039772886, 250.7842808457816375 ) ) ;
#33866=VECTOR ( 'NONE', #16849, 1000.000000000000000 ) ;
#33867=CARTESIAN_POINT ( 'NONE',  ( 95.65096329713743728, -33.45531905120653704, 141.1041967044829732 ) ) ;
#33868=CARTESIAN_POINT ( 'NONE',  ( 103.9639062230918825, -47.31423993612443724, 62.33753003781600199 ) ) ;
#33869=CARTESIAN_POINT ( 'NONE',  ( 105.3771735659821616, -28.36731242524880159, 249.5838068554170661 ) ) ;
#33870=DIRECTION ( 'NONE',  ( 0.000000000000000000, 1.000000000000000000, 0.000000000000000000 ) ) ;
#33871=CARTESIAN_POINT ( 'NONE',  ( 108.0719115850922236, -25.31448365300273551, 321.8079557531246451 ) ) ;
#33872=CARTESIAN_POINT ( 'NONE',  ( 96.74313874428034410, -35.27650366090898615, 177.2156252759109805 ) ) ;
#33875=DIRECTION ( 'NONE',  ( 0.000000000000000000, 0.000000000000000000, 1.000000000000000000 ) ) ;
#33877=ORIENTED_EDGE ( 'NONE', *, *, #70721, .T. ) ;
#33878=DIRECTION ( 'NONE',  ( 0.000000000000000000, 0.000000000000000000, 1.000000000000000000 ) ) ;
#33880=AXIS2_PLACEMENT_3D ( 'NONE', #2925, #22936, #78796 ) ;
#33882=CARTESIAN_POINT ( 'NONE',  ( 97.22546204445637841, -31.69621874537715556, 95.96229194257799122 ) ) ;
#33884=CARTESIAN_POINT ( 'NONE',  ( 136.5887892044395926, -35.63370978841413006, 7.053538376721769865 ) ) ;
#33885=DIRECTION ( 'NONE',  ( 1.000000000000000078E-15, -1.000000000000000083E-30, -1.000000000000000000 ) ) ;
#33886=DIRECTION ( 'NONE',  ( 1.000000000000000078E-15, -1.000000000000000083E-30, -1.000000000000000000 ) ) ;
#33887=DIRECTION ( 'NONE',  ( 1.000000000000000078E-15, 1.000000000000000083E-30, -1.000000000000000000 ) ) ;
#33888=CARTESIAN_POINT ( 'NONE',  ( 106.3035372762157493, -47.10473409126645805, 218.5184824187679453 ) ) ;
#33890=EDGE_CURVE ( 'NONE', #12535, #3336, #23, .T. ) ;
#33893=LINE ( 'NONE', #18927, #39668 ) ;
#33896=EDGE_CURVE ( 'NONE', #62011, #49381, #66079, .T. ) ;
#33898=DIRECTION ( 'NONE',  ( 0.000000000000000000, 0.000000000000000000, -1.000000000000000000 ) ) ;
#33899=CARTESIAN_POINT ( 'NONE',  ( 96.73248008985177648, -40.78176272772311250, 246.6118157521009664 ) ) ;
#33900=ORIENTED_EDGE ( 'NONE', *, *, #88928, .T. ) ;
#33902=CARTESIAN_POINT ( 'NONE',  ( 119.0814029968458811, -31.76540601701525901, 292.6356252759106837 ) ) ;
#33903=CARTESIAN_POINT ( 'NONE',  ( 100.2329966457367334, -45.44659500335379221, 273.0594347997205773 ) ) ;
#33904=CARTESIAN_POINT ( 'NONE',  ( 98.05313438099307177, -42.12366292992533801, 157.7556252759109725 ) ) ;
#33905=CARTESIAN_POINT ( 'NONE',  ( 104.4899543326152127, -26.97880761473700417, 31.28145861894176960 ) ) ;
#33906=FACE_OUTER_BOUND ( 'NONE', #58369, .T. ) ;
#33908=DIRECTION ( 'NONE',  ( -1.000000000000000000, -4.299999999999999979E-14, -1.000000000000000078E-15 ) ) ;
#33909=CARTESIAN_POINT ( 'NONE',  ( 115.0889047299720431, -30.61763668903771674, 189.3439586083947290 ) ) ;
#33917=VERTEX_POINT ( 'NONE', #78589 ) ;
#33919=CARTESIAN_POINT ( 'NONE',  ( 101.3960830062750631, -28.00733582429768376, 21.53562527591096298 ) ) ;
#33922=CARTESIAN_POINT ( 'NONE',  ( 20.56670390244743984, -48.82844715994200158, 180.4678068554150911 ) ) ;
#33923=CARTESIAN_POINT ( 'NONE',  ( 110.3936857311090023, -28.86269079874493571, 244.1809912566479568 ) ) ;
#33924=ORIENTED_EDGE ( 'NONE', *, *, #78426, .F. ) ;
#33925=ORIENTED_EDGE ( 'NONE', *, *, #78216, .F. ) ;
#33926=ORIENTED_EDGE ( 'NONE', *, *, #25159, .T. ) ;
#33928=CARTESIAN_POINT ( 'NONE',  ( 133.5842039024480528, -51.22944715994092491, 231.5838068554170093 ) ) ;
#33929=VECTOR ( 'NONE', #58223, 1000.000000000000000 ) ;
#33930=CARTESIAN_POINT ( 'NONE',  ( 108.3335946874162374, -46.73484295057657789, 102.6771468619035517 ) ) ;
#33932=LINE ( 'NONE', #41630, #46033 ) ;
#33934=AXIS2_PLACEMENT_3D ( 'NONE', #78878, #30705, #65662 ) ;
#33935=CARTESIAN_POINT ( 'NONE',  ( 172.5664832912729878, -27.82844715994070484, 255.9256252759120116 ) ) ;
#33936=CARTESIAN_POINT ( 'NONE',  ( 116.8470136369842720, -36.79772195930841150, 263.8213395616257912 ) ) ;
#33937=DIRECTION ( 'NONE',  ( 0.000000000000000000, 0.000000000000000000, -1.000000000000000000 ) ) ;
#33940=LINE ( 'NONE', #20337, #82949 ) ;
#33941=EDGE_CURVE ( 'NONE', #81819, #50094, #48622, .T. ) ;
#33942=CARTESIAN_POINT ( 'NONE',  ( 115.1095529034481331, -33.53414494269306800, 96.95761417911496949 ) ) ;
#33943=ADVANCED_FACE ( 'NONE', ( #77675 ), #44467, .F. ) ;
#33945=CARTESIAN_POINT ( 'NONE',  ( 104.4899544499527053, -26.97880758519347211, 45.28145860940914957 ) ) ;
#33946=ORIENTED_EDGE ( 'NONE', *, *, #54154, .F. ) ;
#33947=CARTESIAN_POINT ( 'NONE',  ( 77.85525873416803222, -35.08426237656984625, 7.378668740741173515 ) ) ;
#33949=CARTESIAN_POINT ( 'NONE',  ( 107.6530059321349455, -47.12789624220987150, 152.6213395616249500 ) ) ;
#33951=CARTESIAN_POINT ( 'NONE',  ( 109.6430121650047909, -46.48008672573308786, 68.78145861206645861 ) ) ;
#33952=CARTESIAN_POINT ( 'NONE',  ( 112.9486100676287208, -29.40298074535265727, 115.9577737820869601 ) ) ;
#33953=DIRECTION ( 'NONE',  ( 1.000000000000000078E-15, -1.000000000000000083E-30, -1.000000000000000000 ) ) ;
#33954=CARTESIAN_POINT ( 'NONE',  ( 150.5667039024485234, -47.82844715993594065, 180.4678068554149775 ) ) ;
#33955=CARTESIAN_POINT ( 'NONE',  ( 116.1426067713721437, -29.07136428874337142, 70.38419670448192278 ) ) ;
#33956=AXIS2_PLACEMENT_3D ( 'NONE', #56592, #63877, #88556 ) ;
#33959=EDGE_CURVE ( 'NONE', #69055, #11886, #79022, .T. ) ;
#33960=DIRECTION ( 'NONE',  ( 4.299999999999999979E-14, -1.000000000000000000, 4.400000000000000367E-29 ) ) ;
#33961=VECTOR ( 'NONE', #6856, 1000.000000000000000 ) ;
#33963=VERTEX_POINT ( 'NONE', #36784 ) ;
#33964=DIRECTION ( 'NONE',  ( 0.000000000000000000, -1.000000000000000000, 0.000000000000000000 ) ) ;
#33965=VERTEX_POINT ( 'NONE', #71757 ) ;
#33966=CARTESIAN_POINT ( 'NONE',  ( 112.1213531720970309, -45.14146623880455422, 238.0070538473399324 ) ) ;
#33967=CARTESIAN_POINT ( 'NONE',  ( 98.07189402449054683, -42.11243585264244160, 157.7556252759109725 ) ) ;
#33969=CARTESIAN_POINT ( 'NONE',  ( 97.07207206070478378, -35.37844118697538676, 142.2189586082815822 ) ) ;
#33970=CARTESIAN_POINT ( 'NONE',  ( 103.3624612311685809, -47.14358183654965018, 98.31657765686297523 ) ) ;
#33972=ORIENTED_EDGE ( 'NONE', *, *, #76668, .T. ) ;
#33976=ORIENTED_EDGE ( 'NONE', *, *, #63864, .F. ) ;
#33977=CARTESIAN_POINT ( 'NONE',  ( 123.6837132603318565, -20.11243780205705534, 229.5838068554170093 ) ) ;
#33979=CIRCLE ( 'NONE', #3525, 2.117000000000000881 ) ;
#33980=CARTESIAN_POINT ( 'NONE',  ( 176.7738106835050758, -48.62134037887501847, 300.4678068554149490 ) ) ;
#33981=CARTESIAN_POINT ( 'NONE',  ( 97.79211192542227593, -40.52543860420435351, 11.63562527591094309 ) ) ;
#33983=CIRCLE ( 'NONE', #73146, 2.500000000000002220 ) ;
#33984=CARTESIAN_POINT ( 'NONE',  ( 154.4532655810166091, -72.54279768053238797, 542.9756252759101471 ) ) ;
#33985=CARTESIAN_POINT ( 'NONE',  ( 113.1806887538930795, -44.75007787370592638, 93.09499265662630307 ) ) ;
#33986=CARTESIAN_POINT ( 'NONE',  ( 110.6828660728576637, -28.42687563832788200, 284.1600388756959887 ) ) ;
#33988=CARTESIAN_POINT ( 'NONE',  ( 98.16825066461163374, -43.24752039522706326, 102.8175300378159847 ) ) ;
#33989=CARTESIAN_POINT ( 'NONE',  ( 142.8679068202682458, 10.65431904611001634, 396.9756252759102040 ) ) ;
#33990=CARTESIAN_POINT ( 'NONE',  ( 105.7147172347987407, -24.90567422487873017, 160.1670538473389627 ) ) ;
#33995=VECTOR ( 'NONE', #43755, 1000.000000000000000 ) ;
#33996=FACE_BOUND ( 'NONE', #51786, .T. ) ;
#33997=DIRECTION ( 'NONE',  ( -1.000000000000000000, -1.000000000000000078E-15, -1.000000000000000078E-15 ) ) ;
#33998=EDGE_CURVE ( 'NONE', #88268, #76542, #85407, .T. ) ;
#33999=EDGE_LOOP ( 'NONE', ( #79968, #75068, #84505, #31493, #29753, #56640 ) ) ;
#34001=CARTESIAN_POINT ( 'NONE',  ( 97.96866571142417968, -30.36999819975766357, 160.8289586092449497 ) ) ;
#34002=EDGE_LOOP ( 'NONE', ( #7051, #26374, #4835, #61303, #61711, #68831, #9600, #89405 ) ) ;
#34003=DIRECTION ( 'NONE',  ( 0.000000000000000000, 0.000000000000000000, 1.000000000000000000 ) ) ;
#34009=ORIENTED_EDGE ( 'NONE', *, *, #77471, .T. ) ;
#34011=EDGE_CURVE ( 'NONE', #58534, #1672, #57325, .T. ) ;
#34013=CARTESIAN_POINT ( 'NONE',  ( 51.34673845256598668, -36.02818131005800950, -5.074374724088000832 ) ) ;
#34014=CARTESIAN_POINT ( 'NONE',  ( 111.9958537464713970, -27.96271286943853696, 249.6692924242317417 ) ) ;
#34017=DIRECTION ( 'NONE',  ( -4.299999999999999979E-14, 1.000000000000000000, -4.400000000000000367E-29 ) ) ;
#34020=EDGE_LOOP ( 'NONE', ( #57766, #80262, #77792, #88453 ) ) ;
#34021=CIRCLE ( 'NONE', #79056, 4.749999999999976907 ) ;
#34023=DIRECTION ( 'NONE',  ( 0.000000000000000000, 0.000000000000000000, -1.000000000000000000 ) ) ;
#34025=DIRECTION ( 'NONE',  ( 0.000000000000000000, 0.000000000000000000, 1.000000000000000000 ) ) ;
#34026=CARTESIAN_POINT ( 'NONE',  ( 101.2327472597882263, -44.62129728587211730, 253.0699109901961492 ) ) ;
#34028=CARTESIAN_POINT ( 'NONE',  ( 100.7170190823677132, -45.85612711270987774, 83.09276813305294240 ) ) ;
#34030=CARTESIAN_POINT ( 'NONE',  ( 103.4635681255033433, -27.40063510583546957, 21.36976600060490838 ) ) ;
#34031=ORIENTED_EDGE ( 'NONE', *, *, #16010, .T. ) ;
#34032=CARTESIAN_POINT ( 'NONE',  ( 76.06670390244796920, -26.72944715994109899, 239.5838068554169809 ) ) ;
#34034=VERTEX_POINT ( 'NONE', #16786 ) ;
#34036=CARTESIAN_POINT ( 'NONE',  ( 105.4026065362546802, -27.48239143091520020, 271.6377737820876632 ) ) ;
#34037=LINE ( 'NONE', #62656, #9617 ) ;
#34039=AXIS2_PLACEMENT_3D ( 'NONE', #16737, #4889, #79428 ) ;
#34041=CIRCLE ( 'NONE', #29728, 2.517499999999998739 ) ;
#34042=CARTESIAN_POINT ( 'NONE',  ( 97.31584371262773914, -39.30597598611567633, 81.53145860817606660 ) ) ;
#34044=AXIS2_PLACEMENT_3D ( 'NONE', #50538, #57806, #2856 ) ;
#34045=ORIENTED_EDGE ( 'NONE', *, *, #55087, .T. ) ;
#34048=FACE_OUTER_BOUND ( 'NONE', #58288, .T. ) ;
#34050=CARTESIAN_POINT ( 'NONE',  ( 115.0227918137121037, -43.52084328818016701, 63.26419670448196797 ) ) ;
#34051=ORIENTED_EDGE ( 'NONE', *, *, #24492, .T. ) ;
#34052=CARTESIAN_POINT ( 'NONE',  ( 98.59685088459899305, -34.95005064942726136, 258.9918998934010119 ) ) ;
#34053=FACE_BOUND ( 'NONE', #10363, .T. ) ;
#34054=CARTESIAN_POINT ( 'NONE',  ( 108.2857792741417882, -47.02760743735412063, 162.6822919425779617 ) ) ;
#34056=DIRECTION ( 'NONE',  ( -4.237773401492740281E-14, 1.000000000000000000, 0.000000000000000000 ) ) ;
#34059=CARTESIAN_POINT ( 'NONE',  ( 111.1444126100616927, -27.08769046218140986, 240.7584824187679544 ) ) ;
#34062=EDGE_LOOP ( 'NONE', ( #29137, #21853, #16142, #59762 ) ) ;
#34063=CARTESIAN_POINT ( 'NONE',  ( 107.9492956907162267, -25.66517399690753720, 111.0251490854349754 ) ) ;
#34067=VERTEX_POINT ( 'NONE', #43126 ) ;
#34071=DIRECTION ( 'NONE',  ( 4.299999999999999979E-14, -1.000000000000000000, 4.400000000000000367E-29 ) ) ;
#34072=DIRECTION ( 'NONE',  ( 0.7071067811868710917, -0.7071067811862240537, 0.000000000000000000 ) ) ;
#34074=CARTESIAN_POINT ( 'NONE',  ( 104.5146602464430714, -28.97587216416100375, 163.1480903695919551 ) ) ;
#34075=CARTESIAN_POINT ( 'NONE',  ( 106.2251562910655309, -47.77378392694726017, 263.5280062282920994 ) ) ;
#34081=CARTESIAN_POINT ( 'NONE',  ( 29.56670390244797630, -67.87844715994100397, 300.9178068554150514 ) ) ;
#34084=ADVANCED_FACE ( 'NONE', ( #56762 ), #22268, .T. ) ;
#34085=AXIS2_PLACEMENT_3D ( 'NONE', #87437, #39712, #26996 ) ;
#34086=LINE ( 'NONE', #82278, #19878 ) ;
#34087=ORIENTED_EDGE ( 'NONE', *, *, #72053, .T. ) ;
#34089=DIRECTION ( 'NONE',  ( 0.8571673007021091140, -8.250245410175212261E-16, 0.5150380749100597066 ) ) ;
#34092=ADVANCED_FACE ( 'NONE', ( #31699, #58945, #86683 ), #4900, .F. ) ;
#34093=CARTESIAN_POINT ( 'NONE',  ( 142.0664832912740394, -56.72944715994099596, -4.824374724088994704 ) ) ;
#34094=DIRECTION ( 'NONE',  ( 0.000000000000000000, 0.000000000000000000, 1.000000000000000000 ) ) ;
#34095=CARTESIAN_POINT ( 'NONE',  ( 109.8786884439187759, -28.66423582349726118, 209.2324198280769849 ) ) ;
#34096=CARTESIAN_POINT ( 'NONE',  ( 96.88405369895032493, -39.16353706000892032, 56.51276813305394597 ) ) ;
#34097=ORIENTED_EDGE ( 'NONE', *, *, #52196, .T. ) ;
#34098=DIRECTION ( 'NONE',  ( 3.999999999999999995E-14, -1.000000000000000000, 4.100000000000000342E-29 ) ) ;
#34099=ORIENTED_EDGE ( 'NONE', *, *, #52082, .F. ) ;
#34101=EDGE_CURVE ( 'NONE', #55129, #46554, #45750, .T. ) ;
#34102=ORIENTED_EDGE ( 'NONE', *, *, #25891, .F. ) ;
#34105=DIRECTION ( 'NONE',  ( -0.000000000000000000, -0.000000000000000000, -1.000000000000000000 ) ) ;
#34107=CARTESIAN_POINT ( 'NONE',  ( 116.3743287984549966, -40.51183142128556369, 133.5190709745654658 ) ) ;
#34109=CIRCLE ( 'NONE', #15278, 0.9999999999999731326 ) ;
#34111=CARTESIAN_POINT ( 'NONE',  ( 97.78948648769619467, -29.31518076255846239, 45.78991099019697231 ) ) ;
#34116=CARTESIAN_POINT ( 'NONE',  ( 75.31670390244798341, -57.40094715994099772, 60.91780685541480267 ) ) ;
#34119=CARTESIAN_POINT ( 'NONE',  ( 131.3834856945508989, -18.12003772029462922, 3.004064388422935661 ) ) ;
#34122=CARTESIAN_POINT ( 'NONE',  ( 107.0664832912739968, 25.62155284005901379, 333.4006252759110112 ) ) ;
#34123=ADVANCED_FACE ( 'NONE', ( #73033 ), #39850, .F. ) ;
#34124=EDGE_CURVE ( 'NONE', #27744, #79856, #33044, .T. ) ;
#34126=FACE_OUTER_BOUND ( 'NONE', #53602, .T. ) ;
#34127=ORIENTED_EDGE ( 'NONE', *, *, #21925, .T. ) ;
#34128=CARTESIAN_POINT ( 'NONE',  ( 98.84076182955313072, -43.22688528923472262, 87.85848241876792031 ) ) ;
#34131=LINE ( 'NONE', #5096, #6438 ) ;
#34132=CARTESIAN_POINT ( 'NONE',  ( 188.5667039024479834, -58.35344715994099829, 257.2178068554150059 ) ) ;
#34134=VECTOR ( 'NONE', #48725, 1000.000000000000000 ) ;
#34137=CARTESIAN_POINT ( 'NONE',  ( 112.7054497023526238, -28.73785826246146158, 125.5870538473389502 ) ) ;
#34140=CARTESIAN_POINT ( 'NONE',  ( 96.91023542590100703, -30.67149048741791262, 276.8984824187680829 ) ) ;
#34141=CARTESIAN_POINT ( 'NONE',  ( 83.56670559755329464, -33.43837296219065536, 239.5838068554176914 ) ) ;
#34143=LINE ( 'NONE', #75047, #52940 ) ;
#34144=DIRECTION ( 'NONE',  ( 1.000000000000000000, 4.299999999999999979E-14, 1.000000000000000078E-15 ) ) ;
#34147=CARTESIAN_POINT ( 'NONE',  ( 109.4488926988246646, -27.20905326525207357, 199.8813395616259925 ) ) ;
#34148=ORIENTED_EDGE ( 'NONE', *, *, #10421, .T. ) ;
#34149=ORIENTED_EDGE ( 'NONE', *, *, #38305, .T. ) ;
#34150=VECTOR ( 'NONE', #4164, 1000.000000000000114 ) ;
#34151=CARTESIAN_POINT ( 'NONE',  ( 98.17580767689473475, -36.86367352702462341, 132.7701547344679511 ) ) ;
#34153=CARTESIAN_POINT ( 'NONE',  ( 98.57375871705461634, -34.19924797442281772, 27.52729759161093170 ) ) ;
#34154=CARTESIAN_POINT ( 'NONE',  ( 107.0664832912739968, -36.72944715994100306, 293.2242906452868851 ) ) ;
#34155=VECTOR ( 'NONE', #12015, 1000.000000000000114 ) ;
#34158=DIRECTION ( 'NONE',  ( -1.000000000000000000, -4.299999999999999979E-14, -1.000000000000000078E-15 ) ) ;
#34160=CARTESIAN_POINT ( 'NONE',  ( 51.06648329127400388, -8.350947159940998787, 335.9181252759120184 ) ) ;
#34161=CARTESIAN_POINT ( 'NONE',  ( 115.3705510513157861, -30.46277945167181045, 219.3413395616249773 ) ) ;
#34162=DIRECTION ( 'NONE',  ( 0.000000000000000000, 0.000000000000000000, 1.000000000000000000 ) ) ;
#34164=ORIENTED_EDGE ( 'NONE', *, *, #3428, .F. ) ;
#34166=CARTESIAN_POINT ( 'NONE',  ( 77.51853161617800936, -17.69475198630787105, 2.828485944707570088 ) ) ;
#34167=CARTESIAN_POINT ( 'NONE',  ( 19.56648329127303043, -81.37844715994266664, 342.9256252759109884 ) ) ;
#34172=VECTOR ( 'NONE', #22893, 1000.000000000000000 ) ;
#34173=CARTESIAN_POINT ( 'NONE',  ( 97.75353936551157119, -40.54122631656009190, 7.635625275910939536 ) ) ;
#34174=VECTOR ( 'NONE', #89706, 1000.000000000000114 ) ;
#34176=CARTESIAN_POINT ( 'NONE',  ( 95.40772882630993479, -38.85404833720006224, 201.4699109901969791 ) ) ;
#34177=EDGE_CURVE ( 'NONE', #2296, #67030, #16755, .T. ) ;
#34183=CARTESIAN_POINT ( 'NONE',  ( 110.8572222768187174, -45.98311135449077369, 167.8858617136263263 ) ) ;
#34184=CARTESIAN_POINT ( 'NONE',  ( 106.7484768184134083, -28.57294068349449034, 82.92523322673494590 ) ) ;
#34185=CARTESIAN_POINT ( 'NONE',  ( 95.54549022710490647, -39.60850420455695087, 162.5213395616259788 ) ) ;
#34186=AXIS2_PLACEMENT_3D ( 'NONE', #36517, #193, #62414 ) ;
#34187=EDGE_CURVE ( 'NONE', #20192, #44506, #60291, .T. ) ;
#34190=EDGE_CURVE ( 'NONE', #48357, #32010, #80322, .T. ) ;
#34191=AXIS2_PLACEMENT_3D ( 'NONE', #56715, #3112, #17192 ) ;
#34193=CARTESIAN_POINT ( 'NONE',  ( 97.82591666500863425, -40.55218698018725831, 66.63908578027370311 ) ) ;
#34194=ORIENTED_EDGE ( 'NONE', *, *, #5196, .F. ) ;
#34198=ORIENTED_EDGE ( 'NONE', *, *, #45349, .F. ) ;
#34202=EDGE_CURVE ( 'NONE', #3477, #48525, #25783, .T. ) ;
#34203=CARTESIAN_POINT ( 'NONE',  ( 98.64819939953339656, -38.17465580927972724, 90.88384839950496996 ) ) ;
#34204=CARTESIAN_POINT ( 'NONE',  ( 116.9057501799638601, -41.81710558299434410, 243.4346728949589647 ) ) ;
#34205=CARTESIAN_POINT ( 'NONE',  ( 98.55548742614587354, -30.74683778668241985, 205.8384824187679669 ) ) ;
#34206=DIRECTION ( 'NONE',  ( 1.000000000000000078E-15, 0.000000000000000000, -1.000000000000000000 ) ) ;
#34207=CARTESIAN_POINT ( 'NONE',  ( 96.36668125800727580, -39.40815171121896299, 12.53372051400597442 ) ) ;
#34208=DIRECTION ( 'NONE',  ( 0.000000000000000000, 0.000000000000000000, -1.000000000000000000 ) ) ;
#34209=CARTESIAN_POINT ( 'NONE',  ( 105.7137777181048079, -46.72360065728855716, 93.46882327081740982 ) ) ;
#34210=ADVANCED_FACE ( 'NONE', ( #47103 ), #795, .T. ) ;
#34211=ORIENTED_EDGE ( 'NONE', *, *, #38604, .F. ) ;
#34212=ADVANCED_FACE ( 'NONE', ( #79884 ), #39411, .T. ) ;
#34213=CARTESIAN_POINT ( 'NONE',  ( 109.7352083718000415, -46.17358189742688523, 72.79562527591099297 ) ) ;
#34214=CARTESIAN_POINT ( 'NONE',  ( 111.9494872540039694, -27.46861899264377982, 59.68991099019693536 ) ) ;
#34215=CARTESIAN_POINT ( 'NONE',  ( 117.5348925983358583, -35.85526142194976273, 253.8927681330537780 ) ) ;
#34216=VERTEX_POINT ( 'NONE', #38958 ) ;
#34217=CARTESIAN_POINT ( 'NONE',  ( 110.0520778049922939, -26.08682939676148038, 219.8708633711489711 ) ) ;
#34218=FACE_OUTER_BOUND ( 'NONE', #31151, .T. ) ;
#34219=VECTOR ( 'NONE', #81590, 1000.000000000000000 ) ;
#34220=CARTESIAN_POINT ( 'NONE',  ( 134.0664832912739826, -18.72944715994100306, -5.074374724089001809 ) ) ;
#34222=CARTESIAN_POINT ( 'NONE',  ( 102.3066985797795354, -45.62759501947567031, 28.18602549569725824 ) ) ;
#34223=CARTESIAN_POINT ( 'NONE',  ( 102.7374329129088295, -29.76594532732805476, 277.6356252759111953 ) ) ;
#34224=CARTESIAN_POINT ( 'NONE',  ( 172.5664832912740110, -32.07844715994070839, 314.1756252759120116 ) ) ;
#34225=FACE_OUTER_BOUND ( 'NONE', #58932, .T. ) ;
#34226=LINE ( 'NONE', #60584, #65677 ) ;
#34228=CARTESIAN_POINT ( 'NONE',  ( 188.5667039024479834, -58.35344715994099829, 290.4678068554150627 ) ) ;
#34229=CARTESIAN_POINT ( 'NONE',  ( 112.1310993758104928, -28.00810349215226580, 39.65633506902878480 ) ) ;
#34230=CARTESIAN_POINT ( 'NONE',  ( 115.8254323922487856, -31.73001882956195985, 75.23979194250962621 ) ) ;
#34231=EDGE_CURVE ( 'NONE', #60225, #65413, #66669, .T. ) ;
#34232=DIRECTION ( 'NONE',  ( 0.000000000000000000, 0.000000000000000000, 1.000000000000000000 ) ) ;
#34233=VERTEX_POINT ( 'NONE', #87572 ) ;
#34234=FACE_OUTER_BOUND ( 'NONE', #43403, .T. ) ;
#34235=CARTESIAN_POINT ( 'NONE',  ( 116.9463234969885974, -41.73785994705047386, 248.4651490854349731 ) ) ;
#34236=CARTESIAN_POINT ( 'NONE',  ( 117.2380278806138278, -39.01742120631563893, 144.6499109901969859 ) ) ;
#34237=CARTESIAN_POINT ( 'NONE',  ( 96.49300521333343283, -40.10570368261699059, 277.5603871806730467 ) ) ;
#34239=AXIS2_PLACEMENT_3D ( 'NONE', #73734, #38757, #53706 ) ;
#34240=DIRECTION ( 'NONE',  ( -6.493183223601999383E-14, 1.000000000000000000, -6.593183223602000791E-29 ) ) ;
#34242=DIRECTION ( 'NONE',  ( -1.175184669632759901E-16, 1.000000000000000000, 2.000000000000003705E-15 ) ) ;
#34243=LINE ( 'NONE', #74254, #84226 ) ;
#34244=CARTESIAN_POINT ( 'NONE',  ( 142.8838050580813785, -82.11588141944041297, 542.9756252759101471 ) ) ;
#34246=AXIS2_PLACEMENT_3D ( 'NONE', #65442, #10039, #59047 ) ;
#34249=VERTEX_POINT ( 'NONE', #54353 ) ;
#34252=CARTESIAN_POINT ( 'NONE',  ( 97.73346832622766556, -34.05261013000342274, 140.5267055423629756 ) ) ;
#34253=DIRECTION ( 'NONE',  ( 1.000000000000000000, 0.000000000000000000, 0.000000000000000000 ) ) ;
#34254=ORIENTED_EDGE ( 'NONE', *, *, #48976, .T. ) ;
#34256=CARTESIAN_POINT ( 'NONE',  ( 117.0473132972741013, -39.66401662079133672, 179.5984824187679294 ) ) ;
#34258=LINE ( 'NONE', #81550, #19675 ) ;
#34262=CARTESIAN_POINT ( 'NONE',  ( 109.5220866130624984, -46.80460460589471694, 87.75467289495897205 ) ) ;
#34263=ORIENTED_EDGE ( 'NONE', *, *, #19561, .F. ) ;
#34264=VERTEX_POINT ( 'NONE', #28468 ) ;
#34265=ORIENTED_EDGE ( 'NONE', *, *, #61698, .F. ) ;
#34266=EDGE_CURVE ( 'NONE', #58704, #11027, #28346, .T. ) ;
#34268=CARTESIAN_POINT ( 'NONE',  ( 99.59366209610200826, -44.96145431533973635, 152.9899109901959946 ) ) ;
#34269=PLANE ( 'NONE',  #14305 ) ;
#34270=CIRCLE ( 'NONE', #67668, 5.600000000000000533 ) ;
#34272=CARTESIAN_POINT ( 'NONE',  ( 90.44969454456439450, -50.04645651782492166, 249.5838068554174640 ) ) ;
#34274=CARTESIAN_POINT ( 'NONE',  ( 34.96670390244699433, -26.71338133339301635, -5.074374724088000832 ) ) ;
#34276=CARTESIAN_POINT ( 'NONE',  ( 104.1140010245780445, -46.70499295924816607, 107.3470538473389411 ) ) ;
#34278=ORIENTED_EDGE ( 'NONE', *, *, #14718, .F. ) ;
#34283=CARTESIAN_POINT ( 'NONE',  ( 99.51751092519847930, -40.96193357599213414, 179.5633284648289703 ) ) ;
#34286=EDGE_CURVE ( 'NONE', #5714, #12855, #13508, .T. ) ;
#34287=CARTESIAN_POINT ( 'NONE',  ( 172.5664832912740110, 0.2215528400590013880, 201.0426252759120018 ) ) ;
#34289=EDGE_LOOP ( 'NONE', ( #13930, #83060, #72411, #58336 ) ) ;
#34291=EDGE_CURVE ( 'NONE', #43353, #78013, #47269, .T. ) ;
#34292=CARTESIAN_POINT ( 'NONE',  ( 107.0664832912739968, 19.62155284005901024, 339.0006252759110339 ) ) ;
#34293=EDGE_LOOP ( 'NONE', ( #47136, #32065, #84884, #83078 ) ) ;
#34295=CARTESIAN_POINT ( 'NONE',  ( 97.81168895331838087, -40.51742574516882200, 287.6356252759109680 ) ) ;
#34296=CARTESIAN_POINT ( 'NONE',  ( 97.88747888210261294, -34.72385408216754143, 252.5749166392305938 ) ) ;
#34299=CIRCLE ( 'NONE', #69132, 13.49999999999999822 ) ;
#34305=AXIS2_PLACEMENT_3D ( 'NONE', #76588, #27533, #55211 ) ;
#34306=CIRCLE ( 'NONE', #85113, 4.750000000000004441 ) ;
#34308=ORIENTED_EDGE ( 'NONE', *, *, #69193, .F. ) ;
#34311=CARTESIAN_POINT ( 'NONE',  ( 114.7541070161690158, -40.70454043057743121, 241.2528522743529606 ) ) ;
#34312=CARTESIAN_POINT ( 'NONE',  ( 117.1474210844629766, -33.86219250605441999, 149.0470538473389581 ) ) ;
#34313=CARTESIAN_POINT ( 'NONE',  ( 113.3016265961370408, -28.35762455946448668, 104.5670538473399347 ) ) ;
#34314=CARTESIAN_POINT ( 'NONE',  ( 109.9155554066019391, -44.68685817540732330, 249.5838068554167819 ) ) ;
#34315=CARTESIAN_POINT ( 'NONE',  ( 132.3573525511381774, -16.57277629269280794, 7.749696248599565962 ) ) ;
#34316=CARTESIAN_POINT ( 'NONE',  ( 112.7801043229996338, -45.44936815460292934, 174.0384824187679556 ) ) ;
#34317=DIRECTION ( 'NONE',  ( 1.000000000000000000, 4.163336342344333240E-14, 0.000000000000000000 ) ) ;
#34320=ORIENTED_EDGE ( 'NONE', *, *, #71358, .T. ) ;
#34323=DIRECTION ( 'NONE',  ( -0.7071067812159675947, -0.7071067811571274397, -7.071067812159669175E-16 ) ) ;
#34324=AXIS2_PLACEMENT_3D ( 'NONE', #75095, #62794, #12883 ) ;
#34325=ORIENTED_EDGE ( 'NONE', *, *, #45922, .T. ) ;
#34326=DIRECTION ( 'NONE',  ( 1.000000000000000000, 4.163336342344333240E-14, 0.000000000000000000 ) ) ;
#34327=CLOSED_SHELL ( 'NONE', ( #23058, #70736, #46128, #75833 ) ) ;
#34328=CARTESIAN_POINT ( 'NONE',  ( 102.3022244709477775, -27.41667396567568815, 120.4527681330539792 ) ) ;
#34329=CARTESIAN_POINT ( 'NONE',  ( 115.0921084478398058, -30.62179353620878430, 254.3439423599735392 ) ) ;
#34331=DIRECTION ( 'NONE',  ( 1.000000000000000000, 2.999999999999999839E-15, 1.000000000000000078E-15 ) ) ;
#34334=CARTESIAN_POINT ( 'NONE',  ( 113.0129699484215564, -46.01939436189636012, 214.0175300378159591 ) ) ;
#34335=DIRECTION ( 'NONE',  ( 0.000000000000000000, 1.000000000000000000, 0.000000000000000000 ) ) ;
#34336=CARTESIAN_POINT ( 'NONE',  ( 163.0959832912770082, -23.42844715993521021, 313.9678068554149490 ) ) ;
#34337=ORIENTED_EDGE ( 'NONE', *, *, #60873, .T. ) ;
#34338=CARTESIAN_POINT ( 'NONE',  ( 142.8698897858160706, -0.9167816978817300289, 394.9756252759102040 ) ) ;
#34341=LINE ( 'NONE', #12119, #47664 ) ;
#34342=CARTESIAN_POINT ( 'NONE',  ( 96.84578370412310733, -30.63304659132085206, 280.8984824187681397 ) ) ;
#34344=FACE_OUTER_BOUND ( 'NONE', #31664, .T. ) ;
#34345=CARTESIAN_POINT ( 'NONE',  ( 98.82253044624914651, -28.18127440817969287, 115.6870538473389587 ) ) ;
#34346=CARTESIAN_POINT ( 'NONE',  ( 99.06589935993768847, -44.35602157064030848, 32.92038718067297509 ) ) ;
#34347=CARTESIAN_POINT ( 'NONE',  ( 111.4354466870268539, -47.79847022207366081, 168.8756252759109486 ) ) ;
#34349=ADVANCED_FACE ( 'NONE', ( #89369, #83012 ), #62989, .F. ) ;
#34350=CARTESIAN_POINT ( 'NONE',  ( 104.4901659694147895, -26.97874889091799488, 101.2814670705812432 ) ) ;
#34351=CARTESIAN_POINT ( 'NONE',  ( 19.56670390244744695, -47.82844715994204421, 129.9678068554150627 ) ) ;
#34353=DIRECTION ( 'NONE',  ( -1.000000000000000078E-15, 1.000000000000000083E-30, 1.000000000000000000 ) ) ;
#34354=PLANE ( 'NONE',  #10482 ) ;
#34355=ORIENTED_EDGE ( 'NONE', *, *, #58382, .F. ) ;
#34356=AXIS2_PLACEMENT_3D ( 'NONE', #53531, #74463, #12237 ) ;
#34358=ORIENTED_EDGE ( 'NONE', *, *, #44746, .F. ) ;
#34361=CARTESIAN_POINT ( 'NONE',  ( 96.21590750669005843, -38.71157422997261932, 47.48229194257797303 ) ) ;
#34362=DIRECTION ( 'NONE',  ( 4.299999999999999979E-14, -1.000000000000000000, 4.400000000000000367E-29 ) ) ;
#34363=CARTESIAN_POINT ( 'NONE',  ( 116.3183510266638336, -32.94967450325654568, 119.1356252759109537 ) ) ;
#34364=EDGE_CURVE ( 'NONE', #73742, #84106, #34384, .T. ) ;
#34365=CARTESIAN_POINT ( 'NONE',  ( 102.6652156630552355, -27.23093027504711117, 176.4213395616249898 ) ) ;
#34366=CIRCLE ( 'NONE', #25679, 0.5000000000000004441 ) ;
#34367=DIRECTION ( 'NONE',  ( 1.000000000000000078E-15, 1.000000000000000083E-30, -1.000000000000000000 ) ) ;
#34368=AXIS2_PLACEMENT_3D ( 'NONE', #32701, #19076, #25002 ) ;
#34369=CARTESIAN_POINT ( 'NONE',  ( 110.9231077663976066, -44.92578233336853799, 287.3371817328388147 ) ) ;
#34370=ORIENTED_EDGE ( 'NONE', *, *, #16874, .T. ) ;
#34373=EDGE_CURVE ( 'NONE', #6566, #61739, #5806, .T. ) ;
#34377=CARTESIAN_POINT ( 'NONE',  ( 117.0887403345581390, -37.65561820057894948, 183.7527465225524566 ) ) ;
#34378=CARTESIAN_POINT ( 'NONE',  ( 97.06107109887885542, -37.99641197720560370, 76.42729194365786327 ) ) ;
#34379=CARTESIAN_POINT ( 'NONE',  ( 115.8228748906893770, -31.72559827117937203, 274.2397737358683116 ) ) ;
#34380=CARTESIAN_POINT ( 'NONE',  ( 94.12733899296569007, -42.07533762155324553, 293.6369201390379544 ) ) ;
#34381=DIRECTION ( 'NONE',  ( 1.000000000000000000, 4.510281037539788691E-14, 0.000000000000000000 ) ) ;
#34382=DIRECTION ( 'NONE',  ( 0.000000000000000000, 0.000000000000000000, 1.000000000000000000 ) ) ;
#34383=CARTESIAN_POINT ( 'NONE',  ( 110.6561457788925793, -27.59554888373224557, 269.7784824187687605 ) ) ;
#34384=LINE ( 'NONE', #76177, #41432 ) ;
#34387=AXIS2_PLACEMENT_3D ( 'NONE', #69254, #7025, #21110 ) ;
#34388=B_SPLINE_CURVE_WITH_KNOTS ( 'NONE', 3,
 ( #20553, #62314, #55026, #75954, #13727, #69141, #34610, #29036, #1784, #49902, #77632, #43083, #31250, #58947, #88023, #3117, #67122, #37641, #30819, #86685, #53460, #31702, #65339, #80324, #38511, #38078, #59398, #51688, #79435, #66671, #87132, #24901, #81230, #32591, #86236, #65770, #58510, #32147, #11720, #24013, #52565, #73484, #18976, #17199, #46661, #18069, #79886, #11260 ),
 .UNSPECIFIED., .F., .F.,
 ( 4, 2, 1, 1, 1, 1, 1, 2, 2, 2, 2, 2, 2, 2, 1, 1, 1, 1, 1, 1, 1, 2, 2, 2, 2, 2, 2, 2, 2, 4 ),
 ( 0.5000149529902581103, 0.5002590863139874111, 0.5005032196377168230, 0.5009914862851752027, 0.5019680195800924061, 0.5039210861699265909, 0.5078272193495947384, 0.5156394857089309225, 0.5312640184276032906, 0.5625130838649480269, 0.6250112147396373885, 0.6875093456143268611, 0.7500074764890162227, 0.7500685098199482148, 0.7501295431508803180, 0.7502516098127460786, 0.7504957431364880360, 0.7509840097839701745, 0.7519605430789346734, 0.7539136096688627831, 0.7578197428487252196, 0.7656320092084450968, 0.7812565419278810763, 0.8125056073667551448, 0.8437546728056293244, 0.8750037382445035039, 0.9062528036833776834, 0.9375018691222517520, 0.9687509345611258205, 1.000000000000000000 ),
 .UNSPECIFIED. ) ;
#34391=CARTESIAN_POINT ( 'NONE',  ( 104.1662843248667230, -44.88357317080683373, 100.1347570362589892 ) ) ;
#34392=AXIS2_PLACEMENT_3D ( 'NONE', #84137, #7371, #42314 ) ;
#34394=ADVANCED_FACE ( 'NONE', ( #21222 ), #69821, .T. ) ;
#34395=CARTESIAN_POINT ( 'NONE',  ( 188.5667039024483529, -42.82844715993430640, 137.2178068554150059 ) ) ;
#34397=CARTESIAN_POINT ( 'NONE',  ( 79.00802158143936538, -34.19118199975294914, 8.051357469096430464 ) ) ;
#34398=ADVANCED_FACE ( 'NONE', ( #75734 ), #33495, .F. ) ;
#34400=CARTESIAN_POINT ( 'NONE',  ( 114.5276809309653459, -28.57754439525472989, 154.4746728949589851 ) ) ;
#34404=CARTESIAN_POINT ( 'NONE',  ( 113.5773531717103282, -42.74084067657960162, 119.6644404487539646 ) ) ;
#34407=PLANE ( 'NONE',  #26620 ) ;
#34408=CARTESIAN_POINT ( 'NONE',  ( 115.5915050065794247, -42.76776344903117888, 49.33562527591095659 ) ) ;
#34410=ORIENTED_EDGE ( 'NONE', *, *, #51200, .T. ) ;
#34411=ADVANCED_FACE ( 'NONE', ( #59179 ), #16976, .F. ) ;
#34412=CARTESIAN_POINT ( 'NONE',  ( 133.6498166246059895, 12.92155284005730387, 355.9756252759109998 ) ) ;
#34413=ORIENTED_EDGE ( 'NONE', *, *, #82118, .F. ) ;
#34416=CARTESIAN_POINT ( 'NONE',  ( 83.73314995793998605, 12.92155284005730387, 358.9756252759109998 ) ) ;
#34417=EDGE_LOOP ( 'NONE', ( #23793, #62355 ) ) ;
#34418=CARTESIAN_POINT ( 'NONE',  ( 105.2300248619626757, -26.52326248392216357, 275.2061014663877927 ) ) ;
#34419=CARTESIAN_POINT ( 'NONE',  ( 108.3688181871424945, -47.72895317076035582, 158.6822919425779617 ) ) ;
#34420=DIRECTION ( 'NONE',  ( 4.554376769437570034E-14, -1.000000000000000000, 0.000000000000000000 ) ) ;
#34421=CARTESIAN_POINT ( 'NONE',  ( 116.3212776292297406, -32.94146857471347545, 140.1356252759109680 ) ) ;
#34422=CARTESIAN_POINT ( 'NONE',  ( 117.3712488531672165, -32.73122415481606851, 90.10895860924395606 ) ) ;
#34424=ORIENTED_EDGE ( 'NONE', *, *, #20573, .T. ) ;
#34425=PLANE ( 'NONE',  #64141 ) ;
#34426=CIRCLE ( 'NONE', #54768, 2.500000000000002220 ) ;
#34427=CARTESIAN_POINT ( 'NONE',  ( 117.0609834333835977, -38.07982572155707146, 159.7188531337575910 ) ) ;
#34429=VECTOR ( 'NONE', #7333, 1000.000000000000000 ) ;
#34432=PLANE ( 'NONE',  #24642 ) ;
#34433=CARTESIAN_POINT ( 'NONE',  ( 96.99990081654250673, -39.35482002063354656, 276.5299109901967540 ) ) ;
#34436=CARTESIAN_POINT ( 'NONE',  ( 123.6837132603318423, -17.59493780205705704, 229.5838068554170093 ) ) ;
#34437=CARTESIAN_POINT ( 'NONE',  ( 41.56670390244695312, -36.32844715994109208, 129.9678068554150911 ) ) ;
#34438=CARTESIAN_POINT ( 'NONE',  ( 103.2261711710990824, -45.64430683061108596, 286.6752769709340782 ) ) ;
#34439=CARTESIAN_POINT ( 'NONE',  ( 97.86195078277592074, -32.64092898360054562, 100.9941899314778198 ) ) ;
#34440=CARTESIAN_POINT ( 'NONE',  ( 117.3423061886548027, -38.35306328171702717, 109.7013395616249767 ) ) ;
#34442=CARTESIAN_POINT ( 'NONE',  ( 117.5314631938956182, -40.43040369381473198, 178.5680062282919778 ) ) ;
#34446=FACE_BOUND ( 'NONE', #52255, .T. ) ;
#34449=VECTOR ( 'NONE', #27626, 1000.000000000000000 ) ;
#34451=CARTESIAN_POINT ( 'NONE',  ( 108.2818241440822788, -26.29514120620494921, 129.9841967044819739 ) ) ;
#34452=ORIENTED_EDGE ( 'NONE', *, *, #84057, .F. ) ;
#34454=CARTESIAN_POINT ( 'NONE',  ( 113.0378785334839193, -46.05830800173890793, 214.0175300378159591 ) ) ;
#34456=DIRECTION ( 'NONE',  ( 3.999999999999999995E-14, -1.000000000000000000, 4.100000000000000342E-29 ) ) ;
#34459=DIRECTION ( 'NONE',  ( -0.7071067811865779928, 0.7071067811865171526, -7.071067811865785947E-16 ) ) ;
#34460=CARTESIAN_POINT ( 'NONE',  ( 164.9212702847350158, -29.73316016639540749, -5.074374724088000832 ) ) ;
#34461=ORIENTED_EDGE ( 'NONE', *, *, #37491, .F. ) ;
#34462=CIRCLE ( 'NONE', #43201, 0.4999999999999933387 ) ;
#34467=ORIENTED_EDGE ( 'NONE', *, *, #48728, .T. ) ;
#34468=DIRECTION ( 'NONE',  ( 0.000000000000000000, 0.000000000000000000, 1.000000000000000000 ) ) ;
#34469=CARTESIAN_POINT ( 'NONE',  ( 118.7901020289055225, -38.45900758189035429, 219.7099109901969882 ) ) ;
#34472=CARTESIAN_POINT ( 'NONE',  ( 163.0667039024470171, -32.29483332968611364, -5.074374724088000832 ) ) ;
#34474=CARTESIAN_POINT ( 'NONE',  ( 21.56670390244609692, -23.42844715994195326, 129.9678068554150627 ) ) ;
#34475=ORIENTED_EDGE ( 'NONE', *, *, #80153, .F. ) ;
#34476=AXIS2_PLACEMENT_3D ( 'NONE', #61335, #89062, #76321 ) ;
#34477=VERTEX_POINT ( 'NONE', #31927 ) ;
#34478=EDGE_CURVE ( 'NONE', #26191, #33658, #70264, .T. ) ;
#34479=DIRECTION ( 'NONE',  ( -0.7071067811864671926, -0.7071067811866279529, -7.071067811864976379E-16 ) ) ;
#34480=DIRECTION ( 'NONE',  ( -1.000000000000000078E-15, 0.000000000000000000, 1.000000000000000000 ) ) ;
#34481=CARTESIAN_POINT ( 'NONE',  ( 97.32398421004042177, -35.86507053846868587, 227.2556252759109725 ) ) ;
#34483=CARTESIAN_POINT ( 'NONE',  ( 101.3216544293210291, -28.81361639883588310, 71.57562527591099411 ) ) ;
#34485=CARTESIAN_POINT ( 'NONE',  ( 104.5953338484273161, -27.03378288979946475, 21.27505383609677381 ) ) ;
#34489=VERTEX_POINT ( 'NONE', #86031 ) ;
#34490=ORIENTED_EDGE ( 'NONE', *, *, #55304, .F. ) ;
#34491=DIRECTION ( 'NONE',  ( -6.831565154159360295E-14, 1.000000000000000000, 0.000000000000000000 ) ) ;
#34492=CARTESIAN_POINT ( 'NONE',  ( 113.3129409812876389, -28.82675956000495887, 270.9758690201826425 ) ) ;
#34493=AXIS2_PLACEMENT_3D ( 'NONE', #16281, #9028, #24437 ) ;
#34494=FACE_BOUND ( 'NONE', #44349, .T. ) ;
#34495=CIRCLE ( 'NONE', #72191, 15.99999999999999822 ) ;
#34497=FACE_OUTER_BOUND ( 'NONE', #73097, .T. ) ;
#34501=LINE ( 'NONE', #42643, #1486 ) ;
#34502=CIRCLE ( 'NONE', #38850, 2.030000000000003801 ) ;
#34503=CARTESIAN_POINT ( 'NONE',  ( 162.7866693523297670, -36.02818131005322755, 313.9678068554149490 ) ) ;
#34504=VERTEX_POINT ( 'NONE', #65565 ) ;
#34505=CARTESIAN_POINT ( 'NONE',  ( 110.3541591212943445, -25.34385655279935534, 64.85276813305395649 ) ) ;
#34508=CARTESIAN_POINT ( 'NONE',  ( 115.6248209149117940, -37.18450138507482450, 18.20670554236297889 ) ) ;
#34509=VECTOR ( 'NONE', #30878, 1000.000000000000000 ) ;
#34510=CARTESIAN_POINT ( 'NONE',  ( 113.1795509746323773, -44.75092164323887545, 128.0941733130784428 ) ) ;
#34511=CARTESIAN_POINT ( 'NONE',  ( 98.82386243697609984, -31.40279086140550291, 145.8699109901969848 ) ) ;
#34512=DIRECTION ( 'NONE',  ( 1.000000000000000000, 0.000000000000000000, 0.000000000000000000 ) ) ;
#34513=EDGE_CURVE ( 'NONE', #33658, #64390, #48689, .T. ) ;
#34514=DIRECTION ( 'NONE',  ( 1.000000000000000078E-15, -1.000000000000000083E-30, -1.000000000000000000 ) ) ;
#34515=PLANE ( 'NONE',  #18744 ) ;
#34518=CARTESIAN_POINT ( 'NONE',  ( 109.9722659835539389, -48.26927123350142779, 238.7727681330539724 ) ) ;
#34520=AXIS2_PLACEMENT_3D ( 'NONE', #10695, #45207, #37082 ) ;
#34521=VERTEX_POINT ( 'NONE', #31040 ) ;
#34522=VERTEX_POINT ( 'NONE', #8035 ) ;
#34523=CARTESIAN_POINT ( 'NONE',  ( 114.0511858335762270, -28.93156859308855644, 110.4956252759109816 ) ) ;
#34524=CARTESIAN_POINT ( 'NONE',  ( 33.81648329127399677, 12.92155284005802685, 349.2756252759108406 ) ) ;
#34525=ORIENTED_EDGE ( 'NONE', *, *, #74313, .F. ) ;
#34526=EDGE_LOOP ( 'NONE', ( #31349, #63131, #1464, #28924 ) ) ;
#34532=DIRECTION ( 'NONE',  ( 1.387778780781444492E-15, 0.000000000000000000, -1.000000000000000000 ) ) ;
#34533=ADVANCED_FACE ( 'NONE', ( #22135 ), #58730, .T. ) ;
#34535=LINE ( 'NONE', #28162, #54815 ) ;
#34536=CARTESIAN_POINT ( 'NONE',  ( 105.1059768409772062, -45.79875505096494237, 180.2252332267349857 ) ) ;
#34537=CARTESIAN_POINT ( 'NONE',  ( 111.0012107362514939, -46.40699640104500645, 278.8841967044824059 ) ) ;
#34538=CARTESIAN_POINT ( 'NONE',  ( 109.6412602768308489, -46.48053052121719730, 58.78131275420368951 ) ) ;
#34542=DIRECTION ( 'NONE',  ( -4.237773401492740281E-14, 1.000000000000000000, 0.000000000000000000 ) ) ;
#34545=ORIENTED_EDGE ( 'NONE', *, *, #15848, .T. ) ;
#34547=LINE ( 'NONE', #13224, #87546 ) ;
#34548=CARTESIAN_POINT ( 'NONE',  ( 107.0664832912739399, -36.72944715994095333, 302.6356252759109680 ) ) ;
#34549=LINE ( 'NONE', #39, #47745 ) ;
#34550=CARTESIAN_POINT ( 'NONE',  ( 165.3359832912748004, -36.32844715993531537, 237.4678068554150059 ) ) ;
#34551=CARTESIAN_POINT ( 'NONE',  ( 114.6728154972408475, -42.76387655025251888, 197.7152769709339566 ) ) ;
#34552=CARTESIAN_POINT ( 'NONE',  ( 110.4709766755849643, -47.29459308529762041, 57.83657765686300678 ) ) ;
#34557=CARTESIAN_POINT ( 'NONE',  ( 98.34958594530606035, -31.65707425139662590, 261.9065036680587468 ) ) ;
#34559=CARTESIAN_POINT ( 'NONE',  ( 36.74138383868079671, -48.33240602328870494, 180.4678068554150911 ) ) ;
#34561=CARTESIAN_POINT ( 'NONE',  ( 171.4664832912730219, 12.92155284005730387, 358.9756252759109998 ) ) ;
#34562=B_SPLINE_CURVE_WITH_KNOTS ( 'NONE', 3,
 ( #79481, #38121, #31293, #2724, #3600, #79029, #24059, #64939, #37233, #2275, #17241, #31746, #44920, #37685, #72206, #9532, #72651, #66252, #79926, #29977, #9980, #17680, #45359, #44474, #59442, #73080, #16794, #30865, #10417, #23189, #50857, #65813, #10859, #38557, #86727, #3166, #78595, #16348, #51728, #78145, #58986, #65385, #58551, #44026, #86280, #24500, #30422, #51281, #71764 ),
 .UNSPECIFIED., .F., .F.,
 ( 4, 2, 1, 1, 1, 1, 2, 2, 2, 2, 2, 2, 2, 1, 1, 1, 1, 1, 1, 1, 2, 2, 2, 2, 2, 2, 2, 2, 2, 4 ),
 ( 0.5000301082837493860, 0.5005183601311320452, 0.5010066119785148153, 0.5019831156732802446, 0.5039361230628114363, 0.5078421378418741527, 0.5156541673999998077, 0.5312782265162505624, 0.5625263447487519608, 0.6250225812137547576, 0.6875188176787576655, 0.7500150541437604623, 0.7500760856246835306, 0.7501371171056067100, 0.7502591800674560663, 0.7505033059911569993, 0.7509915578385393253, 0.7519680615332882123, 0.7539210689227870965, 0.7578270837017879735, 0.7656391132597950566, 0.7812631723758085567, 0.8125112906078360009, 0.8437594088398633341, 0.8750075270718906673, 0.9062556453039180004, 0.9375037635359453336, 0.9687518817679727778, 0.9843759408839864999, 1.000000000000000000 ),
 .UNSPECIFIED. ) ;
#34563=AXIS2_PLACEMENT_3D ( 'NONE', #85562, #35589, #78748 ) ;
#34564=CARTESIAN_POINT ( 'NONE',  ( 180.1667039024460166, -28.27351298637340093, -5.074374724088000832 ) ) ;
#34565=VERTEX_POINT ( 'NONE', #81893 ) ;
#34567=CARTESIAN_POINT ( 'NONE',  ( 115.0395865772315034, -43.53517906860128051, 63.26419670448196797 ) ) ;
#34568=( BOUNDED_CURVE ( )  B_SPLINE_CURVE ( 3, ( #46847, #21873, #7340, #8236 ),
 .UNSPECIFIED., .F., .T. ) 
 B_SPLINE_CURVE_WITH_KNOTS ( ( 4, 4 ),
 ( 1.570796326793646225, 3.141592653589124318 ),
 .UNSPECIFIED. ) 
 CURVE ( )  GEOMETRIC_REPRESENTATION_ITEM ( )  RATIONAL_B_SPLINE_CURVE ( ( 1.000000000000000000, 0.8047378541242278249, 0.8047378541242278249, 1.000000000000000000 ) ) 
 REPRESENTATION_ITEM ( '' )  );
#34571=ADVANCED_FACE ( 'NONE', ( #68256 ), #89145, .T. ) ;
#34573=CARTESIAN_POINT ( 'NONE',  ( 131.3325396840767496, -18.38436945697832670, 3.076560175367930139 ) ) ;
#34576=DIRECTION ( 'NONE',  ( 0.000000000000000000, 0.000000000000000000, -1.000000000000000000 ) ) ;
#34577=VECTOR ( 'NONE', #33829, 1000.000000000000114 ) ;
#34580=VERTEX_POINT ( 'NONE', #25561 ) ;
#34581=CARTESIAN_POINT ( 'NONE',  ( 103.2709630098024576, -47.13517786649186547, 93.28610146638693834 ) ) ;
#34585=CARTESIAN_POINT ( 'NONE',  ( 116.3191307872214821, -32.94748812527954840, 115.1356252759109822 ) ) ;
#34588=EDGE_LOOP ( 'NONE', ( #63414, #81806, #33652, #66237 ) ) ;
#34589=CARTESIAN_POINT ( 'NONE',  ( 103.1701080265564912, -27.72257962874998327, 151.4013395616249511 ) ) ;
#34591=DIRECTION ( 'NONE',  ( 0.000000000000000000, 0.000000000000000000, -1.000000000000000000 ) ) ;
#34592=ORIENTED_EDGE ( 'NONE', *, *, #21954, .T. ) ;
#34593=CARTESIAN_POINT ( 'NONE',  ( 100.8614382317055345, -45.12360235833653377, 253.0699109901968882 ) ) ;
#34594=CYLINDRICAL_SURFACE ( 'NONE', #75902, 11.57110091390437034 ) ;
#34595=B_SPLINE_CURVE_WITH_KNOTS ( 'NONE', 3,
 ( #48046, #19464, #33539, #34427, #74882, #41230, #88524, #19916, #6284, #76218, #75781, #74433, #83059, #81714, #13546, #68066, #12657, #21260 ),
 .UNSPECIFIED., .F., .F.,
 ( 4, 2, 2, 2, 2, 2, 2, 2, 4 ),
 ( 0.000000000000000000, 0.06250388370504290914, 0.1250077674100858183, 0.1875116511151287413, 0.2500155348201716365, 0.3125194185252145318, 0.3750233022302574826, 0.4375271859353003778, 0.5000310696403432731 ),
 .UNSPECIFIED. ) ;
#34603=CARTESIAN_POINT ( 'NONE',  ( 110.2867295656602664, -27.49400189596543242, 209.8099109901969541 ) ) ;
#34605=ORIENTED_EDGE ( 'NONE', *, *, #27032, .T. ) ;
#34607=CARTESIAN_POINT ( 'NONE',  ( 97.29374130088892514, -39.17162219779756782, 162.9530118773259630 ) ) ;
#34609=CARTESIAN_POINT ( 'NONE',  ( 111.2075884809769803, -27.22220029719803591, 280.7375300378151337 ) ) ;
#34610=CARTESIAN_POINT ( 'NONE',  ( 97.75828504134041452, -40.38463153286905793, 57.62423291007743131 ) ) ;
#34613=DIRECTION ( 'NONE',  ( 1.000000000000000000, -9.073094938289460781E-13, 0.000000000000000000 ) ) ;
#34614=CARTESIAN_POINT ( 'NONE',  ( 134.0664832912740110, 0.2215528400590013880, 308.6356252759119911 ) ) ;
#34615=CARTESIAN_POINT ( 'NONE',  ( 63.03715912545640521, -24.89890238295017255, 180.4678068554151196 ) ) ;
#34616=DIRECTION ( 'NONE',  ( -1.000000000000000078E-15, 1.000000000000000083E-30, 1.000000000000000000 ) ) ;
#34617=CARTESIAN_POINT ( 'NONE',  ( 100.8363305107023251, -45.83159080358284854, 242.1108633711489517 ) ) ;
#34618=CARTESIAN_POINT ( 'NONE',  ( 48.79742451362098166, -36.32844715994040996, -5.074374724088000832 ) ) ;
#34619=ORIENTED_EDGE ( 'NONE', *, *, #75743, .F. ) ;
#34620=EDGE_CURVE ( 'NONE', #46082, #65478, #5212, .T. ) ;
#34622=AXIS2_PLACEMENT_3D ( 'NONE', #61146, #68423, #48386 ) ;
#34623=CARTESIAN_POINT ( 'NONE',  ( 115.7831076660190206, -41.80230951752221813, 88.40645860859268623 ) ) ;
#34625=CARTESIAN_POINT ( 'NONE',  ( 105.7159130685152206, -46.72393690838458724, 123.4674154773381503 ) ) ;
#34627=AXIS2_PLACEMENT_3D ( 'NONE', #23672, #51334, #16843 ) ;
#34628=LINE ( 'NONE', #54595, #10774 ) ;
#34629=VECTOR ( 'NONE', #27366, 1000.000000000000000 ) ;
#34631=CARTESIAN_POINT ( 'NONE',  ( 116.7674666963954309, -31.33607907186020824, 25.24229194257798881 ) ) ;
#34632=CARTESIAN_POINT ( 'NONE',  ( 108.0141129856239957, -24.91663700320364327, 265.0127681330535552 ) ) ;
#34633=ORIENTED_EDGE ( 'NONE', *, *, #64456, .F. ) ;
#34636=DIRECTION ( 'NONE',  ( 0.000000000000000000, -1.000000000000000000, 0.000000000000000000 ) ) ;
#34637=CARTESIAN_POINT ( 'NONE',  ( 46.03715912545432332, -48.62818131006086020, 249.9678068554150343 ) ) ;
#34639=CARTESIAN_POINT ( 'NONE',  ( 110.8538671553213817, -45.98448489464616529, 167.8855732625641224 ) ) ;
#34641=CARTESIAN_POINT ( 'NONE',  ( 100.4744175226576886, -42.33708426910433076, 74.71761417911493197 ) ) ;
#34642=CARTESIAN_POINT ( 'NONE',  ( 114.4782738979392747, -28.49838154746453256, 155.5051490854349652 ) ) ;
#34645=ADVANCED_FACE ( 'NONE', ( #67335 ), #5124, .T. ) ;
#34646=VECTOR ( 'NONE', #65729, 1000.000000000000000 ) ;
#34647=DIRECTION ( 'NONE',  ( 0.000000000000000000, 0.000000000000000000, -1.000000000000000000 ) ) ;
#34649=ORIENTED_EDGE ( 'NONE', *, *, #59314, .T. ) ;
#34654=VECTOR ( 'NONE', #39466, 1000.000000000000000 ) ;
#34655=CARTESIAN_POINT ( 'NONE',  ( 107.8593070027901746, -27.70813345913228076, 109.4171817328389551 ) ) ;
#34656=CARTESIAN_POINT ( 'NONE',  ( 100.7367085078155640, -45.81951824476916357, 237.0803871806729717 ) ) ;
#34657=CARTESIAN_POINT ( 'NONE',  ( 114.7977927517518566, -29.71579763117545880, 209.4127681330539872 ) ) ;
#34658=CARTESIAN_POINT ( 'NONE',  ( 107.1951288810177090, -26.32694189238808491, 31.06705384733893283 ) ) ;
#34659=CARTESIAN_POINT ( 'NONE',  ( 152.0368932755770288, -23.42844715993588522, 313.9678068554149490 ) ) ;
#34661=ORIENTED_EDGE ( 'NONE', *, *, #70576, .F. ) ;
#34663=CARTESIAN_POINT ( 'NONE',  ( 113.4935171807054246, -28.59114140144088623, 124.5565776568639507 ) ) ;
#34664=CARTESIAN_POINT ( 'NONE',  ( 107.2329094490511068, -25.63056496568808029, 80.07657765686299456 ) ) ;
#34665=CARTESIAN_POINT ( 'NONE',  ( 117.5355484441921163, -36.80252840376058288, 263.8213395616250523 ) ) ;
#34666=ORIENTED_EDGE ( 'NONE', *, *, #85515, .T. ) ;
#34667=CARTESIAN_POINT ( 'NONE',  ( 118.0511761103140316, -35.49834556997346624, 233.9032443235299752 ) ) ;
#34668=CARTESIAN_POINT ( 'NONE',  ( 19.56670390244796920, -67.87844715994100397, 10.91780685541479734 ) ) ;
#34669=CARTESIAN_POINT ( 'NONE',  ( 98.15082878629252150, -41.26132049930647128, 22.70069694779929037 ) ) ;
#34672=DIRECTION ( 'NONE',  ( 0.7071067811864661934, 0.7071067811866289521, 7.071067811864654918E-16 ) ) ;
#34674=DIRECTION ( 'NONE',  ( 1.094868876412250136E-15, 0.000000000000000000, 1.000000000000000000 ) ) ;
#34675=DIRECTION ( 'NONE',  ( 0.000000000000000000, 0.000000000000000000, 1.000000000000000000 ) ) ;
#34676=DIRECTION ( 'NONE',  ( 1.000000000000000078E-15, 1.000000000000000083E-30, -1.000000000000000000 ) ) ;
#34677=DIRECTION ( 'NONE',  ( -0.0001211784769727627432, 0.7071067708032326982, -0.7071067811865484609 ) ) ;
#34678=CARTESIAN_POINT ( 'NONE',  ( 151.5667039024483813, -48.82844715993591223, 249.9678068554149490 ) ) ;
#34679=CARTESIAN_POINT ( 'NONE',  ( 97.81171236172070849, -40.51746256574213589, 261.6350867226296941 ) ) ;
#34681=CIRCLE ( 'NONE', #72375, 2.517499999999998739 ) ;
#34683=CARTESIAN_POINT ( 'NONE',  ( 115.0717820980658814, -30.01665675799653599, 269.3813395616251682 ) ) ;
#34684=CARTESIAN_POINT ( 'NONE',  ( 96.69923704014651378, -37.82612059164544860, 122.4099109901969626 ) ) ;
#34685=CARTESIAN_POINT ( 'NONE',  ( 105.6260786687505657, -47.09854616955767881, 253.4670538473393719 ) ) ;
#34687=DIRECTION ( 'NONE',  ( 1.000000000000000000, 0.000000000000000000, 0.000000000000000000 ) ) ;
#34690=LINE ( 'NONE', #179, #32595 ) ;
#34691=CIRCLE ( 'NONE', #85496, 2.750000000000002665 ) ;
#34693=EDGE_CURVE ( 'NONE', #78030, #52268, #31333, .T. ) ;
#34696=DIRECTION ( 'NONE',  ( 1.000000000000000000, 6.145690160522480771E-16, 0.000000000000000000 ) ) ;
#34697=VERTEX_POINT ( 'NONE', #45986 ) ;
#34698=CARTESIAN_POINT ( 'NONE',  ( 113.5990078486005217, -30.45738264864434441, 188.8457531614099594 ) ) ;
#34699=VECTOR ( 'NONE', #55401, 1000.000000000000000 ) ;
#34700=EDGE_CURVE ( 'NONE', #18701, #3477, #40080, .T. ) ;
#34701=CARTESIAN_POINT ( 'NONE',  ( 104.4059374613178335, -46.45745470167850044, 187.3651553329266335 ) ) ;
#34703=CARTESIAN_POINT ( 'NONE',  ( 160.7738106836360146, -48.62134037874781001, 300.4678068554149490 ) ) ;
#34704=CARTESIAN_POINT ( 'NONE',  ( 103.0581626738562306, -26.45339789934171293, 166.3603871806729444 ) ) ;
#34705=DIRECTION ( 'NONE',  ( -1.000000000000000078E-15, 1.000000000000000083E-30, 1.000000000000000000 ) ) ;
#34706=CIRCLE ( 'NONE', #11500, 1.000000000000000888 ) ;
#34709=EDGE_CURVE ( 'NONE', #40401, #64957, #5584, .T. ) ;
#34710=EDGE_CURVE ( 'NONE', #78458, #53618, #83934, .T. ) ;
#34712=FACE_OUTER_BOUND ( 'NONE', #42013, .T. ) ;
#34713=AXIS2_PLACEMENT_3D ( 'NONE', #87423, #78840, #65629 ) ;
#34714=CARTESIAN_POINT ( 'NONE',  ( 97.83387747045368599, -32.00739517038274329, 95.96229194257799122 ) ) ;
#34715=ORIENTED_EDGE ( 'NONE', *, *, #57682, .F. ) ;
#34716=ORIENTED_EDGE ( 'NONE', *, *, #68142, .T. ) ;
#34717=VERTEX_POINT ( 'NONE', #18299 ) ;
#34719=FACE_OUTER_BOUND ( 'NONE', #85021, .T. ) ;
#34720=CARTESIAN_POINT ( 'NONE',  ( 112.6540662323891837, -44.79745133516134104, 199.0584824187679374 ) ) ;
#34723=EDGE_CURVE ( 'NONE', #17392, #78195, #15408, .T. ) ;
#34726=FACE_OUTER_BOUND ( 'NONE', #67157, .T. ) ;
#34727=LINE ( 'NONE', #8376, #71000 ) ;
#34728=DIRECTION ( 'NONE',  ( 1.000000000000000000, 0.000000000000000000, 0.000000000000000000 ) ) ;
#34729=CARTESIAN_POINT ( 'NONE',  ( 96.04673288144547882, -37.20790665022158805, 116.3489586092439652 ) ) ;
#34732=EDGE_CURVE ( 'NONE', #2851, #60793, #56390, .T. ) ;
#34733=ORIENTED_EDGE ( 'NONE', *, *, #13138, .F. ) ;
#34736=DIRECTION ( 'NONE',  ( 0.000000000000000000, 0.000000000000000000, 1.000000000000000000 ) ) ;
#34737=CARTESIAN_POINT ( 'NONE',  ( 104.3071780974205183, -29.01783752938878180, 188.1680903695909706 ) ) ;
#34738=AXIS2_PLACEMENT_3D ( 'NONE', #14638, #1458, #70043 ) ;
#34739=LINE ( 'NONE', #28835, #50884 ) ;
#34740=CARTESIAN_POINT ( 'NONE',  ( 116.3115597373110290, -32.94279827685361539, 270.1356252759109680 ) ) ;
#34741=ORIENTED_EDGE ( 'NONE', *, *, #22130, .F. ) ;
#34742=VERTEX_POINT ( 'NONE', #1898 ) ;
#34743=ORIENTED_EDGE ( 'NONE', *, *, #60276, .T. ) ;
#34744=AXIS2_PLACEMENT_3D ( 'NONE', #54578, #66893, #6463 ) ;
#34745=CARTESIAN_POINT ( 'NONE',  ( 136.8164832912739826, -18.72944715994099951, 3.101481641215532825 ) ) ;
#34746=ORIENTED_EDGE ( 'NONE', *, *, #29925, .F. ) ;
#34750=CARTESIAN_POINT ( 'NONE',  ( 105.4042388664825722, -28.02512512522124410, 231.6587261630399439 ) ) ;
#34753=EDGE_CURVE ( 'NONE', #69198, #29300, #28414, .T. ) ;
#34754=DIRECTION ( 'NONE',  ( 0.000000000000000000, 1.000000000000000000, 0.000000000000000000 ) ) ;
#34756=AXIS2_PLACEMENT_3D ( 'NONE', #34888, #88972, #81281 ) ;
#34757=EDGE_LOOP ( 'NONE', ( #24334, #40413, #43853, #28810 ) ) ;
#34758=VECTOR ( 'NONE', #15666, 999.9999999999998863 ) ;
#34759=ORIENTED_EDGE ( 'NONE', *, *, #79443, .F. ) ;
#34760=CYLINDRICAL_SURFACE ( 'NONE', #46355, 10.04999999999999361 ) ;
#34762=ORIENTED_EDGE ( 'NONE', *, *, #23972, .T. ) ;
#34763=CARTESIAN_POINT ( 'NONE',  ( 114.1709767417603132, -32.67596046159766132, 287.0566617981627360 ) ) ;
#34764=AXIS2_PLACEMENT_3D ( 'NONE', #37892, #26047, #19233 ) ;
#34765=CARTESIAN_POINT ( 'NONE',  ( 117.7261736041901372, -39.74048882516440528, 143.6194347997209775 ) ) ;
#34766=CARTESIAN_POINT ( 'NONE',  ( 97.24623519876071498, -31.70684325556592853, 95.96229194257799122 ) ) ;
#34767=CARTESIAN_POINT ( 'NONE',  ( 102.2827366117606402, -43.22316888111082989, 249.5838068554171798 ) ) ;
#34768=CARTESIAN_POINT ( 'NONE',  ( 132.8008218761672765, -16.28157759252032122, 7.978179524061537187 ) ) ;
#34769=( GEOMETRIC_REPRESENTATION_CONTEXT ( 3 ) GLOBAL_UNCERTAINTY_ASSIGNED_CONTEXT ( ( #49630 ) ) GLOBAL_UNIT_ASSIGNED_CONTEXT ( ( #38593, #86763, #50888 ) ) REPRESENTATION_CONTEXT ( 'NONE', 'WORKASPACE' ) );
#34770=CARTESIAN_POINT ( 'NONE',  ( 96.67410449796260252, -35.53789531767939991, 202.2356252759109623 ) ) ;
#34771=DIRECTION ( 'NONE',  ( -1.000000000000000000, 0.000000000000000000, 0.000000000000000000 ) ) ;
#34772=LINE ( 'NONE', #56553, #74128 ) ;
#34773=VERTEX_POINT ( 'NONE', #49571 ) ;
#34775=ORIENTED_EDGE ( 'NONE', *, *, #34961, .F. ) ;
#34779=CARTESIAN_POINT ( 'NONE',  ( 106.5069774953447990, -26.72368516806847794, 136.1209971908085663 ) ) ;
#34780=CARTESIAN_POINT ( 'NONE',  ( 98.83989573471103540, -28.19928051380002287, 115.6870538473389587 ) ) ;
#34782=CARTESIAN_POINT ( 'NONE',  ( 179.8585841295808052, -30.08671355699668126, 117.4678068554150627 ) ) ;
#34783=DIRECTION ( 'NONE',  ( -0.7071067811865671127, -0.7071067811865279218, -7.071067811865664660E-16 ) ) ;
#34784=DIRECTION ( 'NONE',  ( -1.000000000000000000, 0.000000000000000000, 0.000000000000000000 ) ) ;
#34785=CARTESIAN_POINT ( 'NONE',  ( 115.8503464879663198, -41.61300288441327666, 58.42257506363554853 ) ) ;
#34786=CARTESIAN_POINT ( 'NONE',  ( 97.49318720818088480, -40.89074837367928694, 227.6527681330539679 ) ) ;
#34790=AXIS2_PLACEMENT_3D ( 'NONE', #15806, #2624, #63950 ) ;
#34791=CARTESIAN_POINT ( 'NONE',  ( 33.78309357196401663, -29.99615139349950965, -5.074374724088000832 ) ) ;
#34793=DIRECTION ( 'NONE',  ( 1.000000000000000078E-15, -1.000000000000000083E-30, -1.000000000000000000 ) ) ;
#34794=LINE ( 'NONE', #62047, #62200 ) ;
#34795=CARTESIAN_POINT ( 'NONE',  ( 96.71965009938165281, -35.13266635363193302, 266.2041967044820581 ) ) ;
#34796=ORIENTED_EDGE ( 'NONE', *, *, #23576, .T. ) ;
#34797=DIRECTION ( 'NONE',  ( 1.000000000000000078E-15, 1.000000000000000083E-30, -1.000000000000000000 ) ) ;
#34798=CARTESIAN_POINT ( 'NONE',  ( 114.3594209402202182, -29.19941241435835266, 174.4641967044819637 ) ) ;
#34799=CARTESIAN_POINT ( 'NONE',  ( 106.6068465219953794, -25.68577410589699994, 36.09753003781596448 ) ) ;
#34800=CARTESIAN_POINT ( 'NONE',  ( 117.5007279078441655, -40.51415819784174488, 169.5375300378159693 ) ) ;
#34801=CARTESIAN_POINT ( 'NONE',  ( 116.3214877775586018, -32.94188667902410117, 30.13562527591096085 ) ) ;
#34802=CARTESIAN_POINT ( 'NONE',  ( 98.34990339064583509, -31.65650299388843436, 101.9063771684363360 ) ) ;
#34803=DIRECTION ( 'NONE',  ( 0.000000000000000000, 0.000000000000000000, 1.000000000000000000 ) ) ;
#34804=DIRECTION ( 'NONE',  ( 1.000000000000000078E-15, -1.000000000000000083E-30, -1.000000000000000000 ) ) ;
#34806=LINE ( 'NONE', #14385, #45286 ) ;
#34809=EDGE_CURVE ( 'NONE', #56684, #84817, #70493, .T. ) ;
#34810=ORIENTED_EDGE ( 'NONE', *, *, #81525, .T. ) ;
#34812=VERTEX_POINT ( 'NONE', #69145 ) ;
#34813=CIRCLE ( 'NONE', #85608, 2.116999999999993776 ) ;
#34815=ORIENTED_EDGE ( 'NONE', *, *, #55714, .T. ) ;
#34816=CARTESIAN_POINT ( 'NONE',  ( 97.79189512308838061, -32.01662636557821173, 46.95276813305393659 ) ) ;
#34817=LINE ( 'NONE', #69799, #81802 ) ;
#34821=CARTESIAN_POINT ( 'NONE',  ( 95.52146136750830863, -39.61450893497475079, 162.5213395616259788 ) ) ;
#34822=DIRECTION ( 'NONE',  ( 0.000000000000000000, 0.000000000000000000, 1.000000000000000000 ) ) ;
#34823=CARTESIAN_POINT ( 'NONE',  ( 115.5964019700117973, -42.63146254436634308, 13.35657765686398868 ) ) ;
#34824=ORIENTED_EDGE ( 'NONE', *, *, #16990, .T. ) ;
#34825=EDGE_LOOP ( 'NONE', ( #20513, #14840, #1419, #49707 ) ) ;
#34826=VECTOR ( 'NONE', #51407, 1000.000000000000000 ) ;
#34827=EDGE_LOOP ( 'NONE', ( #51781, #14580 ) ) ;
#34828=EDGE_CURVE ( 'NONE', #46354, #81580, #64733, .T. ) ;
#34832=CARTESIAN_POINT ( 'NONE',  ( 51.06648329127400388, 19.62155284005901024, 327.8006252759110453 ) ) ;
#34840=CARTESIAN_POINT ( 'NONE',  ( 118.1852327621007532, -40.75705396371412803, 23.54991099019593292 ) ) ;
#34841=DIRECTION ( 'NONE',  ( 1.000000000000000078E-15, -1.000000000000000083E-30, -1.000000000000000000 ) ) ;
#34843=EDGE_LOOP ( 'NONE', ( #88186, #83262, #2340 ) ) ;
#34845=CARTESIAN_POINT ( 'NONE',  ( 41.56648329127398966, -27.82844715994070484, 258.9256252759120116 ) ) ;
#34846=CARTESIAN_POINT ( 'NONE',  ( 104.8330862573783122, -27.72345643971313578, 88.08809036959192440 ) ) ;
#34847=B_SPLINE_CURVE_WITH_KNOTS ( 'NONE', 3,
 ( #77994, #4695, #37097, #53250, #57071, #32377, #74182, #25575, #10275, #23484, #51151, #37545, #36655, #29391, #60077, #39203, #17101, #64356, #58415, #2133, #11962, #87810, #29840, #3018, #72067, #23920, #2585, #57529, #84815, #64801 ),
 .UNSPECIFIED., .F., .F.,
 ( 4, 2, 2, 2, 2, 2, 2, 2, 2, 2, 1, 1, 1, 1, 1, 1, 2, 4 ),
 ( 0.000000000000000000, 0.06250180752313003185, 0.1250036150462600637, 0.1875054225693900956, 0.2500072300925201274, 0.3125090376156501315, 0.3750108451387801911, 0.4375126526619102507, 0.4687635564234753915, 0.4843890083042580175, 0.4922017342446494137, 0.4961080972148451118, 0.4980612786999429331, 0.4990378694424920103, 0.4995261648137667154, 0.4997703124994041790, 0.4998923863422226610, 0.5000144601850410320 ),
 .UNSPECIFIED. ) ;
#34849=CARTESIAN_POINT ( 'NONE',  ( 97.33784131013395324, -34.07106453330637663, 46.11479194286231120 ) ) ;
#34852=CARTESIAN_POINT ( 'NONE',  ( 78.42773927739702344, -34.51875925605449424, 7.791169830173473976 ) ) ;
#34854=CARTESIAN_POINT ( 'NONE',  ( 97.95630822081318456, -30.46975087157407458, 165.8594347997199634 ) ) ;
#34855=EDGE_LOOP ( 'NONE', ( #87346, #83839 ) ) ;
#34856=CARTESIAN_POINT ( 'NONE',  ( 116.7951252747353408, -39.38782977664463658, 69.61479194366307865 ) ) ;
#34857=CARTESIAN_POINT ( 'NONE',  ( 103.5362709388849254, -28.56900242483978047, 151.8330118773259585 ) ) ;
#34860=CARTESIAN_POINT ( 'NONE',  ( 99.03746950336261534, -43.41317339962571253, 112.8784824187679732 ) ) ;
#34861=CARTESIAN_POINT ( 'NONE',  ( 142.8690268918515471, 4.118420757222291506, 542.9756252759101471 ) ) ;
#34862=ORIENTED_EDGE ( 'NONE', *, *, #28995, .T. ) ;
#34863=CARTESIAN_POINT ( 'NONE',  ( 162.7131505118679797, -31.94127993907790852, 117.4678068554150485 ) ) ;
#34864=EDGE_LOOP ( 'NONE', ( #53381, #41420, #19733, #77073 ) ) ;
#34865=VERTEX_POINT ( 'NONE', #83678 ) ;
#34866=FACE_BOUND ( 'NONE', #29146, .T. ) ;
#34867=VERTEX_POINT ( 'NONE', #21451 ) ;
#34868=CARTESIAN_POINT ( 'NONE',  ( 104.7413500955949672, -27.22895272701804359, 285.2670538473402075 ) ) ;
#34869=CARTESIAN_POINT ( 'NONE',  ( 99.40614514399899804, -27.65486269830070398, 146.6356252759109395 ) ) ;
#34870=CARTESIAN_POINT ( 'NONE',  ( 104.4899544585065030, -26.97880758303967852, 141.2814586087148427 ) ) ;
#34871=CARTESIAN_POINT ( 'NONE',  ( 96.03574380810476896, -41.06042880536169548, 92.62419670448296927 ) ) ;
#34872=CARTESIAN_POINT ( 'NONE',  ( 112.0659116397137325, -45.48839625046556989, 262.9897919441546605 ) ) ;
#34873=ORIENTED_EDGE ( 'NONE', *, *, #10513, .F. ) ;
#34877=FACE_OUTER_BOUND ( 'NONE', #14386, .T. ) ;
#34878=ORIENTED_EDGE ( 'NONE', *, *, #40290, .T. ) ;
#34879=VECTOR ( 'NONE', #14130, 1000.000000000000000 ) ;
#34883=CARTESIAN_POINT ( 'NONE',  ( 104.7356349775885320, -47.53436426244870461, 32.41943479972098174 ) ) ;
#34886=CARTESIAN_POINT ( 'NONE',  ( 109.6452928465588741, -46.47951212188701220, 92.78246786428896087 ) ) ;
#34887=CARTESIAN_POINT ( 'NONE',  ( 98.07879527422882404, -32.87106628761745952, 16.00419670448294340 ) ) ;
#34888=CARTESIAN_POINT ( 'NONE',  ( 143.0664832912740110, -18.82844715994099971, 284.9256252759119548 ) ) ;
#34889=CARTESIAN_POINT ( 'NONE',  ( 104.9672558511366276, -25.09151557957609668, 121.2184824187679766 ) ) ;
#34891=DIRECTION ( 'NONE',  ( -2.900000000000000265E-14, 2.000000000000000155E-15, -1.000000000000000000 ) ) ;
#34892=ORIENTED_EDGE ( 'NONE', *, *, #36332, .T. ) ;
#34894=CARTESIAN_POINT ( 'NONE',  ( 34.67381068360400320, -28.98061976758901892, -5.074374724088000832 ) ) ;
#34895=FACE_BOUND ( 'NONE', #17625, .T. ) ;
#34897=ORIENTED_EDGE ( 'NONE', *, *, #82944, .T. ) ;
#34898=CARTESIAN_POINT ( 'NONE',  ( 116.3279290549545806, -32.94269076977911226, 60.13562527591098927 ) ) ;
#34899=CARTESIAN_POINT ( 'NONE',  ( 95.99995219064309993, -35.86644482699779246, 191.2765776568629690 ) ) ;
#34901=CARTESIAN_POINT ( 'NONE',  ( 41.56648329127398966, -18.82844715994071194, 315.9256252759120684 ) ) ;
#34902=CARTESIAN_POINT ( 'NONE',  ( 107.2496171063691577, -24.85558036374148472, 226.0641967044829812 ) ) ;
#34905=CARTESIAN_POINT ( 'NONE',  ( 172.5664832912740110, -9.303447159940999356, 196.8086252759119645 ) ) ;
#34907=VERTEX_POINT ( 'NONE', #44544 ) ;
#34909=VERTEX_POINT ( 'NONE', #79104 ) ;
#34914=EDGE_CURVE ( 'NONE', #20800, #69845, #85482, .T. ) ;
#34917=CARTESIAN_POINT ( 'NONE',  ( 98.94264532560653436, -30.19601435972772308, 236.7870538473399336 ) ) ;
#34920=ADVANCED_FACE ( 'NONE', ( #44993 ), #43660, .F. ) ;
#34921=CARTESIAN_POINT ( 'NONE',  ( 86.06670390244796920, -50.82844715994100682, 310.9178068554150514 ) ) ;
#34922=DIRECTION ( 'NONE',  ( -4.237773401492740281E-14, 1.000000000000000000, 0.000000000000000000 ) ) ;
#34923=DIRECTION ( 'NONE',  ( 1.000000000000000078E-15, 1.000000000000000083E-30, -1.000000000000000000 ) ) ;
#34925=CARTESIAN_POINT ( 'NONE',  ( 115.7470646134707266, -43.61006842878475709, 48.30514908543492680 ) ) ;
#34927=ORIENTED_EDGE ( 'NONE', *, *, #22516, .T. ) ;
#34929=CARTESIAN_POINT ( 'NONE',  ( 97.80474605953816081, -40.50046288348590195, 17.63384904215703131 ) ) ;
#34930=CARTESIAN_POINT ( 'NONE',  ( 109.7813264909552231, -47.51098736074720108, 238.7727681330529776 ) ) ;
#34931=EDGE_CURVE ( 'NONE', #86212, #14684, #44098, .T. ) ;
#34932=DIRECTION ( 'NONE',  ( 0.000000000000000000, 0.000000000000000000, -1.000000000000000000 ) ) ;
#34933=CARTESIAN_POINT ( 'NONE',  ( 98.20607846729137691, -32.50961293922097894, 71.97276813305397525 ) ) ;
#34935=CARTESIAN_POINT ( 'NONE',  ( 97.06383915561490028, -37.34216361049876554, 22.37517802614766183 ) ) ;
#34937=VERTEX_POINT ( 'NONE', #45430 ) ;
#34938=CARTESIAN_POINT ( 'NONE',  ( 180.2121375201600131, -29.73316016639650172, -5.074374724088000832 ) ) ;
#34939=ORIENTED_EDGE ( 'NONE', *, *, #83020, .F. ) ;
#34940=ORIENTED_EDGE ( 'NONE', *, *, #29390, .F. ) ;
#34942=CARTESIAN_POINT ( 'NONE',  ( 113.8567361903355675, -31.03552547285496388, 265.8130118773257777 ) ) ;
#34944=CARTESIAN_POINT ( 'NONE',  ( 113.2450767973898280, -28.75835022255681750, 139.5523338186963827 ) ) ;
#34946=VECTOR ( 'NONE', #63837, 1000.000000000000000 ) ;
#34948=EDGE_LOOP ( 'NONE', ( #19318, #83116, #3660, #80228 ) ) ;
#34949=DIRECTION ( 'NONE',  ( -1.000000000000000000, -3.999999999999999995E-14, -1.000000000000000078E-15 ) ) ;
#34951=VERTEX_POINT ( 'NONE', #50475 ) ;
#34952=CARTESIAN_POINT ( 'NONE',  ( 97.35142178662984236, -32.85085377626895564, 41.02419670448193045 ) ) ;
#34953=ORIENTED_EDGE ( 'NONE', *, *, #1443, .T. ) ;
#34954=CARTESIAN_POINT ( 'NONE',  ( 110.3271547037548004, -45.17815799167961899, 17.28003887569495944 ) ) ;
#34955=VECTOR ( 'NONE', #71228, 1000.000000000000000 ) ;
#34957=CARTESIAN_POINT ( 'NONE',  ( 101.5632356570520756, -44.81509498605974784, 197.1013395616259913 ) ) ;
#34959=CARTESIAN_POINT ( 'NONE',  ( 29.77381068363392913, -48.62134037875510018, 180.4678068554150911 ) ) ;
#34960=DIRECTION ( 'NONE',  ( 0.000000000000000000, 1.000000000000000000, 0.000000000000000000 ) ) ;
#34961=EDGE_CURVE ( 'NONE', #7607, #3590, #8202, .T. ) ;
#34962=DIRECTION ( 'NONE',  ( 0.000000000000000000, 0.000000000000000000, -1.000000000000000000 ) ) ;
#34963=CARTESIAN_POINT ( 'NONE',  ( 97.43303641489029587, -40.91689460032421266, 227.6527681330539679 ) ) ;
#34964=CARTESIAN_POINT ( 'NONE',  ( 144.8545562996767444, -1.932463243632626781, 361.9756252759100335 ) ) ;
#34965=ORIENTED_EDGE ( 'NONE', *, *, #52266, .F. ) ;
#34966=CARTESIAN_POINT ( 'NONE',  ( 136.7282109818851552, -37.44060378570205216, 6.877169033949778409 ) ) ;
#34968=CARTESIAN_POINT ( 'NONE',  ( 102.3408129182306823, -46.07080783562200565, 123.2041967044829818 ) ) ;
#34970=VERTEX_POINT ( 'NONE', #86801 ) ;
#34974=CARTESIAN_POINT ( 'NONE',  ( 109.6430120328528233, -46.48008676205834178, 122.7814586012382847 ) ) ;
#34975=CARTESIAN_POINT ( 'NONE',  ( 112.1393497837960638, -28.01282533620751636, 265.6564582266507841 ) ) ;
#34977=DIRECTION ( 'NONE',  ( 4.299999999999999979E-14, -1.000000000000000000, 4.400000000000000367E-29 ) ) ;
#34978=CARTESIAN_POINT ( 'NONE',  ( 29.77381068363392913, -48.62134037875510018, 180.4678068554150911 ) ) ;
#34979=CARTESIAN_POINT ( 'NONE',  ( 103.9214495108435017, -28.66658863671924706, 168.1785665600669688 ) ) ;
#34980=CARTESIAN_POINT ( 'NONE',  ( 111.4896171341011666, -26.57472070863446589, 280.7375300378156453 ) ) ;
#34982=ORIENTED_EDGE ( 'NONE', *, *, #71960, .T. ) ;
#34984=FACE_OUTER_BOUND ( 'NONE', #72599, .T. ) ;
#34985=AXIS2_PLACEMENT_3D ( 'NONE', #45544, #31942, #79229 ) ;
#34987=ORIENTED_EDGE ( 'NONE', *, *, #15452, .F. ) ;
#34988=CIRCLE ( 'NONE', #68395, 0.5000000000000016653 ) ;
#34989=ADVANCED_FACE ( 'NONE', ( #37308 ), #3240, .T. ) ;
#34990=CARTESIAN_POINT ( 'NONE',  ( 57.56670390244829605, -48.82844715994039575, 295.7178068554150627 ) ) ;
#34992=FACE_OUTER_BOUND ( 'NONE', #55413, .T. ) ;
#34993=FACE_OUTER_BOUND ( 'NONE', #78093, .T. ) ;
#34994=LINE ( 'NONE', #48163, #30163 ) ;
#34995=CARTESIAN_POINT ( 'NONE',  ( 98.55184737119530780, -35.75319039346454986, 205.6581341137909646 ) ) ;
#34996=CARTESIAN_POINT ( 'NONE',  ( 97.58231912995226764, -32.21254287871169453, 75.97276813305397525 ) ) ;
#34997=ORIENTED_EDGE ( 'NONE', *, *, #20251, .F. ) ;
#34998=DIRECTION ( 'NONE',  ( -0.7071067811869841124, 0.7071067811861110330, 0.000000000000000000 ) ) ;
#34999=ORIENTED_EDGE ( 'NONE', *, *, #89482, .T. ) ;
#35000=CARTESIAN_POINT ( 'NONE',  ( 131.0667039024480118, -67.87844715994100397, 225.9838068554150254 ) ) ;
#35003=CARTESIAN_POINT ( 'NONE',  ( 87.06648329127315833, -54.72944906728996273, 14.82207188531695863 ) ) ;
#35004=ORIENTED_EDGE ( 'NONE', *, *, #79906, .F. ) ;
#35005=CARTESIAN_POINT ( 'NONE',  ( 29.56670390244797630, -67.87844715994100397, 300.9178068554150514 ) ) ;
#35007=CARTESIAN_POINT ( 'NONE',  ( 73.10937651008708826, -8.833000550533901318, -5.074374724088975164 ) ) ;
#35009=LINE ( 'NONE', #62722, #20546 ) ;
#35010=ORIENTED_EDGE ( 'NONE', *, *, #52118, .F. ) ;
#35011=CARTESIAN_POINT ( 'NONE',  ( 99.11053040751089327, -44.43647348971805400, 41.95086337114900488 ) ) ;
#35012=DIRECTION ( 'NONE',  ( 0.000000000000000000, 0.000000000000000000, -1.000000000000000000 ) ) ;
#35014=LINE ( 'NONE', #77720, #20647 ) ;
#35015=CARTESIAN_POINT ( 'NONE',  ( 132.8830524875716605, -16.24700279812585180, 1.845048209623397995 ) ) ;
#35017=ADVANCED_FACE ( 'NONE', ( #24129 ), #51358, .T. ) ;
#35018=AXIS2_PLACEMENT_3D ( 'NONE', #63615, #84074, #23639 ) ;
#35020=DIRECTION ( 'NONE',  ( 0.7071067811865784369, -0.7071067811865165975, 7.071067811865791864E-16 ) ) ;
#35022=CIRCLE ( 'NONE', #72770, 3.249999999999975131 ) ;
#35025=ORIENTED_EDGE ( 'NONE', *, *, #80768, .T. ) ;
#35026=CARTESIAN_POINT ( 'NONE',  ( 102.6068629045982021, -46.86833229348674479, 128.2346728949589760 ) ) ;
#35027=EDGE_CURVE ( 'NONE', #86462, #87604, #50255, .T. ) ;
#35029=DIRECTION ( 'NONE',  ( 0.7071067811866516006, -0.7071067811864434338, 0.000000000000000000 ) ) ;
#35031=FACE_BOUND ( 'NONE', #57506, .T. ) ;
#35032=CARTESIAN_POINT ( 'NONE',  ( 97.25364341294459791, -36.87759583893578963, 132.3384824187679669 ) ) ;
#35034=DIRECTION ( 'NONE',  ( -4.554376769437570034E-14, 1.000000000000000000, 0.000000000000000000 ) ) ;
#35036=VECTOR ( 'NONE', #76601, 1000.000000000000000 ) ;
#35037=CARTESIAN_POINT ( 'NONE',  ( 100.1532602078033278, -44.50350736857013345, 262.9984824187678782 ) ) ;
#35039=DIRECTION ( 'NONE',  ( 1.000000000000000078E-15, 1.000000000000000083E-30, -1.000000000000000000 ) ) ;
#35044=CARTESIAN_POINT ( 'NONE',  ( 108.5755967597531821, -27.06580334247533770, 189.9527681330539792 ) ) ;
#35045=VERTEX_POINT ( 'NONE', #30494 ) ;
#35046=CIRCLE ( 'NONE', #85855, 1.000000000000003775 ) ;
#35048=CARTESIAN_POINT ( 'NONE',  ( 103.3408556358882890, -28.68905057859731755, 176.8530118773259687 ) ) ;
#35049=CIRCLE ( 'NONE', #36568, 5.599999999999994316 ) ;
#35051=CARTESIAN_POINT ( 'NONE',  ( 100.8575770528253628, -43.09432028306430595, 18.39301187732595011 ) ) ;
#35053=CARTESIAN_POINT ( 'NONE',  ( 85.53617444537002257, -18.82844715994099971, 342.9256252759119548 ) ) ;
#35056=LINE ( 'NONE', #76406, #66198 ) ;
#35057=CARTESIAN_POINT ( 'NONE',  ( 109.3321198358312074, -26.57584895156206173, 224.9013395616249511 ) ) ;
#35058=CARTESIAN_POINT ( 'NONE',  ( 97.39153615373059836, -39.27944949574720113, 171.5316118837727686 ) ) ;
#35059=ORIENTED_EDGE ( 'NONE', *, *, #57276, .T. ) ;
#35060=ORIENTED_EDGE ( 'NONE', *, *, #9289, .F. ) ;
#35061=AXIS2_PLACEMENT_3D ( 'NONE', #70601, #8373, #63787 ) ;
#35063=CARTESIAN_POINT ( 'NONE',  ( 33.96670390244699433, -26.71338133339301635, -5.074374724088000832 ) ) ;
#35066=AXIS2_PLACEMENT_3D ( 'NONE', #69000, #13583, #26319 ) ;
#35067=LINE ( 'NONE', #43223, #32488 ) ;
#35068=ORIENTED_EDGE ( 'NONE', *, *, #40845, .F. ) ;
#35069=VECTOR ( 'NONE', #44004, 1000.000000000000000 ) ;
#35072=CARTESIAN_POINT ( 'NONE',  ( 115.3236443966936235, -45.23002221789283084, 268.1899109901965517 ) ) ;
#35074=AXIS2_PLACEMENT_3D ( 'NONE', #22631, #63957, #1735 ) ;
#35075=CARTESIAN_POINT ( 'NONE',  ( 77.68755387133397505, -38.11069332323667425, 7.213126773494069610 ) ) ;
#35077=CARTESIAN_POINT ( 'NONE',  ( 113.2492417207108417, -44.60456355013358376, 168.1061584034887915 ) ) ;
#35079=CARTESIAN_POINT ( 'NONE',  ( 98.96126485936372319, -37.90763323093077020, 64.25951894101994810 ) ) ;
#35080=CARTESIAN_POINT ( 'NONE',  ( 97.65507918845807467, -41.26406199109977280, 167.6841967044829573 ) ) ;
#35085=EDGE_LOOP ( 'NONE', ( #5687, #53813, #83782, #21538 ) ) ;
#35086=VERTEX_POINT ( 'NONE', #80892 ) ;
#35088=DIRECTION ( 'NONE',  ( 0.000000000000000000, 0.000000000000000000, -1.000000000000000000 ) ) ;
#35089=( BOUNDED_CURVE ( )  B_SPLINE_CURVE ( 3, ( #39919, #81738, #19488, #47171 ),
 .UNSPECIFIED., .F., .F. ) 
 B_SPLINE_CURVE_WITH_KNOTS ( ( 4, 4 ),
 ( 1.570796326787725850, 3.141592653584011519 ),
 .UNSPECIFIED. ) 
 CURVE ( )  GEOMETRIC_REPRESENTATION_ITEM ( )  RATIONAL_B_SPLINE_CURVE ( ( 1.000000000000000000, 0.8047378541240375327, 0.8047378541240375327, 1.000000000000000000 ) ) 
 REPRESENTATION_ITEM ( '' )  );
#35091=ORIENTED_EDGE ( 'NONE', *, *, #4865, .T. ) ;
#35092=CARTESIAN_POINT ( 'NONE',  ( 36.74138383868084645, -48.33240602328870494, 129.9678068554150911 ) ) ;
#35093=CARTESIAN_POINT ( 'NONE',  ( 112.2681825743621431, -29.31628353742046755, 84.00003887569602057 ) ) ;
#35094=CARTESIAN_POINT ( 'NONE',  ( 107.2496247454619152, -24.85508506706595000, 230.0641967044819580 ) ) ;
#35095=CARTESIAN_POINT ( 'NONE',  ( 113.0097079652340568, -45.31096836313454190, 203.0584824187679374 ) ) ;
#35096=CARTESIAN_POINT ( 'NONE',  ( 110.3472192523918238, -25.36789009815987228, 60.85276813305395649 ) ) ;
#35097=LINE ( 'NONE', #69637, #87602 ) ;
#35098=LINE ( 'NONE', #21041, #30869 ) ;
#35099=EDGE_CURVE ( 'NONE', #37640, #23174, #39528, .T. ) ;
#35101=DIRECTION ( 'NONE',  ( 0.000000000000000000, 0.000000000000000000, 1.000000000000000000 ) ) ;
#35102=LINE ( 'NONE', #28287, #57969 ) ;
#35103=DIRECTION ( 'NONE',  ( 0.000000000000000000, 0.000000000000000000, -1.000000000000000000 ) ) ;
#35105=CARTESIAN_POINT ( 'NONE',  ( 97.28626111821314737, -36.62605694204433604, 111.3184824187689657 ) ) ;
#35106=CARTESIAN_POINT ( 'NONE',  ( 100.9172270114722494, -28.25635367234391992, 75.57562527591093726 ) ) ;
#35107=CARTESIAN_POINT ( 'NONE',  ( 106.2233489284451338, -47.79750968570053971, 267.5280062282920994 ) ) ;
#35110=CARTESIAN_POINT ( 'NONE',  ( 97.47293644110631305, -40.89955093664978136, 231.6527681330539679 ) ) ;
#35111=CARTESIAN_POINT ( 'NONE',  ( 97.31584374709767360, -39.30597611958086190, 36.53145861904452829 ) ) ;
#35113=CARTESIAN_POINT ( 'NONE',  ( 46.83715912545429205, -47.82818131006082751, 249.9678068554150343 ) ) ;
#35116=FACE_OUTER_BOUND ( 'NONE', #24393, .T. ) ;
#35120=DIRECTION ( 'NONE',  ( 0.000000000000000000, 0.000000000000000000, 1.000000000000000000 ) ) ;
#35121=EDGE_CURVE ( 'NONE', #11288, #8413, #77841, .T. ) ;
#35122=DIRECTION ( 'NONE',  ( 1.000000000000000078E-15, -1.000000000000000000, 0.000000000000000000 ) ) ;
#35123=DIRECTION ( 'NONE',  ( 0.000000000000000000, 1.000000000000000000, 0.000000000000000000 ) ) ;
#35126=CARTESIAN_POINT ( 'NONE',  ( 99.38058175836560793, -28.75308465796231516, 265.6746728949588032 ) ) ;
#35127=CARTESIAN_POINT ( 'NONE',  ( 114.2533759015650787, -44.28132150547345702, 154.1813395616249807 ) ) ;
#35128=CARTESIAN_POINT ( 'NONE',  ( 111.0545523236672807, -47.06291463499678684, 13.85753003781498016 ) ) ;
#35129=CARTESIAN_POINT ( 'NONE',  ( 107.0664832912739968, -18.82844715994099971, 168.9256252759119832 ) ) ;
#35131=CARTESIAN_POINT ( 'NONE',  ( 82.73027604518235023, -36.02416100035765112, 6.874390491354032129 ) ) ;
#35132=CARTESIAN_POINT ( 'NONE',  ( 97.81489200343717982, -40.52525142474216580, 137.6362986401610158 ) ) ;
#35135=VERTEX_POINT ( 'NONE', #18643 ) ;
#35136=DIRECTION ( 'NONE',  ( 0.000000000000000000, 0.000000000000000000, -1.000000000000000000 ) ) ;
#35139=CARTESIAN_POINT ( 'NONE',  ( 99.64399296875224366, -31.54106566633107533, 160.2514674471249521 ) ) ;
#35141=CARTESIAN_POINT ( 'NONE',  ( 177.4809174648215730, -49.32844715993478246, 180.4678068554150059 ) ) ;
#35142=ORIENTED_EDGE ( 'NONE', *, *, #64773, .F. ) ;
#35143=CARTESIAN_POINT ( 'NONE',  ( 107.0664832912739968, -36.72944715994100306, 287.6356252759109680 ) ) ;
#35144=CARTESIAN_POINT ( 'NONE',  ( 101.7806060443209049, -45.68981339355057969, 158.1527681330539963 ) ) ;
#35147=CARTESIAN_POINT ( 'NONE',  ( 57.56670390244747892, -48.82844715994040286, 134.7178068554150911 ) ) ;
#35148=CARTESIAN_POINT ( 'NONE',  ( 51.56670390244699576, -22.48495420874030515, 342.9256252759109884 ) ) ;
#35150=CYLINDRICAL_SURFACE ( 'NONE', #78855, 18.00000000000000000 ) ;
#35151=CARTESIAN_POINT ( 'NONE',  ( 98.65123886609826798, -31.74476095556097377, 85.90133956162593165 ) ) ;
#35152=EDGE_LOOP ( 'NONE', ( #60545, #72505, #42566, #52058 ) ) ;
#35153=ORIENTED_EDGE ( 'NONE', *, *, #79778, .F. ) ;
#35155=CARTESIAN_POINT ( 'NONE',  ( 115.5880482615279163, -32.77224410791782816, 55.59205949637296840 ) ) ;
#35156=DIRECTION ( 'NONE',  ( 1.000000000000000078E-15, 1.000000000000000083E-30, -1.000000000000000000 ) ) ;
#35157=CARTESIAN_POINT ( 'NONE',  ( 116.4500618263485592, -39.48841239489304655, 179.5984824187679294 ) ) ;
#35158=DIRECTION ( 'NONE',  ( -1.000000000000000000, 0.000000000000000000, 0.000000000000000000 ) ) ;
#35160=DIRECTION ( 'NONE',  ( 0.000000000000000000, 0.000000000000000000, -1.000000000000000000 ) ) ;
#35161=LINE ( 'NONE', #76513, #51814 ) ;
#35165=CARTESIAN_POINT ( 'NONE',  ( 116.7751801856528147, -32.99181816784836485, 139.1184824187679396 ) ) ;
#35167=ORIENTED_EDGE ( 'NONE', *, *, #67321, .T. ) ;
#35168=ORIENTED_EDGE ( 'NONE', *, *, #67460, .F. ) ;
#35171=CARTESIAN_POINT ( 'NONE',  ( 41.56648329127398966, -27.82844715994070484, 78.92562527591199739 ) ) ;
#35172=LINE ( 'NONE', #62883, #4731 ) ;
#35173=CARTESIAN_POINT ( 'NONE',  ( 111.7296936849409406, -43.46273440104761221, 200.8766617981629565 ) ) ;
#35174=VECTOR ( 'NONE', #3261, 1000.000000000000000 ) ;
#35175=DIRECTION ( 'NONE',  ( 0.000000000000000000, 0.000000000000000000, 1.000000000000000000 ) ) ;
#35177=ADVANCED_FACE ( 'NONE', ( #25911 ), #19532, .T. ) ;
#35180=VERTEX_POINT ( 'NONE', #33167 ) ;
#35181=ORIENTED_EDGE ( 'NONE', *, *, #38118, .T. ) ;
#35182=PLANE ( 'NONE',  #33148 ) ;
#35184=ORIENTED_EDGE ( 'NONE', *, *, #32449, .T. ) ;
#35185=CARTESIAN_POINT ( 'NONE',  ( 79.31518617682141326, -21.40257939794846109, 8.160477455077044695 ) ) ;
#35186=CIRCLE ( 'NONE', #23621, 2.999999999999929834 ) ;
#35187=CARTESIAN_POINT ( 'NONE',  ( 114.4699299399979395, -31.85941057575024971, 250.7215833058968997 ) ) ;
#35192=ORIENTED_EDGE ( 'NONE', *, *, #41464, .F. ) ;
#35193=EDGE_LOOP ( 'NONE', ( #11474, #70125 ) ) ;
#35194=AXIS2_PLACEMENT_3D ( 'NONE', #5173, #31973, #39680 ) ;
#35195=ADVANCED_FACE ( 'NONE', ( #53576 ), #85114, .F. ) ;
#35196=CARTESIAN_POINT ( 'NONE',  ( 106.6019379103756535, -25.27972995136449441, 322.9014499992877631 ) ) ;
#35197=ORIENTED_EDGE ( 'NONE', *, *, #32446, .T. ) ;
#35198=ORIENTED_EDGE ( 'NONE', *, *, #74531, .T. ) ;
#35199=EDGE_CURVE ( 'NONE', #36669, #9938, #51680, .T. ) ;
#35200=VECTOR ( 'NONE', #89213, 1000.000000000000000 ) ;
#35201=CARTESIAN_POINT ( 'NONE',  ( 101.0613286755868359, -30.49734935201787422, 263.4928522743534813 ) ) ;
#35202=EDGE_CURVE ( 'NONE', #43121, #5764, #47673, .T. ) ;
#35203=CARTESIAN_POINT ( 'NONE',  ( 96.58491273044850800, -36.88769195468244533, 136.3384824187679385 ) ) ;
#35204=CARTESIAN_POINT ( 'NONE',  ( 107.3333893024683903, -26.32957087652219741, 120.0556252759109555 ) ) ;
#35205=CARTESIAN_POINT ( 'NONE',  ( 41.56648329127398966, -18.82844715994071194, 135.9256252759120684 ) ) ;
#35206=DIRECTION ( 'NONE',  ( 0.000000000000000000, 0.000000000000000000, -1.000000000000000000 ) ) ;
#35207=CARTESIAN_POINT ( 'NONE',  ( 96.12521010412353917, -35.16020481777900386, 222.2251490854349640 ) ) ;
#35209=CARTESIAN_POINT ( 'NONE',  ( 168.3664380525666218, -48.62818131005488453, 249.9678068554149775 ) ) ;
#35212=EDGE_CURVE ( 'NONE', #18895, #25576, #6860, .T. ) ;
#35213=VERTEX_POINT ( 'NONE', #42641 ) ;
#35216=CARTESIAN_POINT ( 'NONE',  ( 89.06648329127401098, -18.82844715994099971, 323.8756252759120002 ) ) ;
#35217=EDGE_CURVE ( 'NONE', #5997, #20800, #27694, .T. ) ;
#35218=ADVANCED_FACE ( 'NONE', ( #28126 ), #57528, .F. ) ;
#35219=LINE ( 'NONE', #7973, #14233 ) ;
#35220=ORIENTED_EDGE ( 'NONE', *, *, #63054, .F. ) ;
#35221=CARTESIAN_POINT ( 'NONE',  ( 117.5811103608870383, -33.32038496654947579, 134.0880062282919880 ) ) ;
#35222=CARTESIAN_POINT ( 'NONE',  ( 184.3595971212625386, -48.62134037874549364, 180.4678068554150343 ) ) ;
#35225=DIRECTION ( 'NONE',  ( -4.554376769437570034E-14, 1.000000000000000000, 0.000000000000000000 ) ) ;
#35227=LINE ( 'NONE', #62491, #606 ) ;
#35228=CARTESIAN_POINT ( 'NONE',  ( 118.0844448206163833, -36.21142561920247971, 264.8518157521014587 ) ) ;
#35231=EDGE_LOOP ( 'NONE', ( #33667, #83473, #77449, #24802 ) ) ;
#35233=CARTESIAN_POINT ( 'NONE',  ( 188.5667039024481255, -42.82844715993431350, 254.7178068554150059 ) ) ;
#35234=DIRECTION ( 'NONE',  ( 1.000000000000000000, 4.443626637970152463E-14, 0.000000000000000000 ) ) ;
#35235=ADVANCED_FACE ( 'NONE', ( #56271 ), #20443, .T. ) ;
#35236=FACE_BOUND ( 'NONE', #61569, .T. ) ;
#35237=CARTESIAN_POINT ( 'NONE',  ( 116.5766284862631466, -42.45395780223795157, 278.3832443235297660 ) ) ;
#35240=CARTESIAN_POINT ( 'NONE',  ( 108.2803926554762626, -47.73958771823362213, 157.6518157521019532 ) ) ;
#35241=CARTESIAN_POINT ( 'NONE',  ( 99.14357900773808296, -43.50514455292471894, 27.88991099019694175 ) ) ;
#35242=CARTESIAN_POINT ( 'NONE',  ( 114.2047867640113594, -45.22899916922247598, 144.1203871806729637 ) ) ;
#35244=CARTESIAN_POINT ( 'NONE',  ( 97.12553229912508357, -37.99667850842347860, 102.4272513145173491 ) ) ;
#35246=CARTESIAN_POINT ( 'NONE',  ( 125.9611475301391721, -58.72944715994100306, 239.5838068554164124 ) ) ;
#35247=CARTESIAN_POINT ( 'NONE',  ( 115.8254323922932940, -31.73001882967317044, 69.23979194249955071 ) ) ;
#35251=CARTESIAN_POINT ( 'NONE',  ( 194.0371591254572934, -24.42818131005407878, 300.4678068554149490 ) ) ;
#35257=CARTESIAN_POINT ( 'NONE',  ( 117.4328057974122714, -37.95573561897357706, 49.73276813305393773 ) ) ;
#35259=ADVANCED_FACE ( 'NONE', ( #3562 ), #72618, .F. ) ;
#35260=CARTESIAN_POINT ( 'NONE',  ( 36.65249034007530327, -49.32844715994124130, 300.4678068554150059 ) ) ;
#35261=CARTESIAN_POINT ( 'NONE',  ( 96.69998679698829847, -35.27043030541812385, 177.2156252759109805 ) ) ;
#35262=EDGE_CURVE ( 'NONE', #62736, #58734, #15870, .T. ) ;
#35263=CARTESIAN_POINT ( 'NONE',  ( 110.6828660728576637, -28.42687563832788200, 284.1600388756959887 ) ) ;
#35267=AXIS2_PLACEMENT_3D ( 'NONE', #89887, #27639, #76236 ) ;
#35269=DIRECTION ( 'NONE',  ( 9.030537910253610117E-13, -1.000000000000000000, 9.040537910253610592E-28 ) ) ;
#35270=CARTESIAN_POINT ( 'NONE',  ( 48.45959712129000252, -28.98061976758940617, -5.074374724088000832 ) ) ;
#35272=CARTESIAN_POINT ( 'NONE',  ( 113.2454986961229935, -28.75867294318174316, 74.55229194277401916 ) ) ;
#35276=CARTESIAN_POINT ( 'NONE',  ( 116.3219235766278672, -32.94275373074044211, 34.13562527591096085 ) ) ;
#35278=CARTESIAN_POINT ( 'NONE',  ( 113.3428377330624954, -29.55695056567750711, 289.5032443235305664 ) ) ;
#35279=DIRECTION ( 'NONE',  ( -0.7071067811571960515, 0.7071067812158990940, 0.000000000000000000 ) ) ;
#35280=ORIENTED_EDGE ( 'NONE', *, *, #88611, .T. ) ;
#35281=FACE_OUTER_BOUND ( 'NONE', #16403, .T. ) ;
#35282=DIRECTION ( 'NONE',  ( 0.000000000000000000, -1.000000000000000000, 0.000000000000000000 ) ) ;
#35283=CARTESIAN_POINT ( 'NONE',  ( 109.1158479366964684, -45.13783758831200998, 85.57285227435401964 ) ) ;
#35289=CARTESIAN_POINT ( 'NONE',  ( 77.45242755740702023, -35.85322059724175858, 6.943211687812227417 ) ) ;
#35290=VECTOR ( 'NONE', #2781, 1000.000000000000000 ) ;
#35292=EDGE_LOOP ( 'NONE', ( #7481, #88635, #28492, #89784 ) ) ;
#35293=CARTESIAN_POINT ( 'NONE',  ( 113.4085779730985166, -29.80024602262787425, 150.9063452106589693 ) ) ;
#35294=DIRECTION ( 'NONE',  ( 0.000000000000000000, 0.000000000000000000, 1.000000000000000000 ) ) ;
#35295=CARTESIAN_POINT ( 'NONE',  ( 117.3927859964040437, -32.72286779764937847, 90.10895860924395606 ) ) ;
#35296=CIRCLE ( 'NONE', #19366, 2.116999999999993776 ) ;
#35297=CARTESIAN_POINT ( 'NONE',  ( 109.6430121127644952, -46.48008674009260233, 83.78145860778620602 ) ) ;
#35300=ORIENTED_EDGE ( 'NONE', *, *, #18209, .T. ) ;
#35301=ORIENTED_EDGE ( 'NONE', *, *, #70202, .T. ) ;
#35302=EDGE_CURVE ( 'NONE', #60117, #45, #64457, .T. ) ;
#35303=EDGE_CURVE ( 'NONE', #64498, #25149, #58956, .T. ) ;
#35305=CARTESIAN_POINT ( 'NONE',  ( 22.49563609058250435, -48.82844715994099971, 13.84673904354932361 ) ) ;
#35306=EDGE_LOOP ( 'NONE', ( #54141, #43369, #6346, #28230 ) ) ;
#35307=CARTESIAN_POINT ( 'NONE',  ( 115.1244435679684699, -31.12738977229718884, 279.3099109901971815 ) ) ;
#35308=CARTESIAN_POINT ( 'NONE',  ( 117.9712535577395869, -34.78749165583555225, 194.9546728949589749 ) ) ;
#35309=DIRECTION ( 'NONE',  ( 0.000000000000000000, 1.000000000000000000, 0.000000000000000000 ) ) ;
#35311=CARTESIAN_POINT ( 'NONE',  ( 116.7955140328789412, -32.98399009599280873, 135.1184824187679396 ) ) ;
#35312=CARTESIAN_POINT ( 'NONE',  ( 33.96670390244699433, -26.71338133339301635, -5.074374724088000832 ) ) ;
#35313=EDGE_LOOP ( 'NONE', ( #36570, #55621, #36881, #71674 ) ) ;
#35315=EDGE_CURVE ( 'NONE', #71030, #70034, #64017, .T. ) ;
#35316=ADVANCED_FACE ( 'NONE', ( #30385 ), #58516, .T. ) ;
#35317=CARTESIAN_POINT ( 'NONE',  ( 51.06648329127400388, 19.62155284005901024, 333.4006252759110112 ) ) ;
#35318=VERTEX_POINT ( 'NONE', #3127 ) ;
#35320=VECTOR ( 'NONE', #31099, 1000.000000000000000 ) ;
#35321=CARTESIAN_POINT ( 'NONE',  ( 41.56648329127381203, -18.82844715994071194, 201.9256252759118979 ) ) ;
#35323=LINE ( 'NONE', #71220, #27569 ) ;
#35324=CARTESIAN_POINT ( 'NONE',  ( 100.4790876285538275, -27.85333844968608830, 35.59657765686397113 ) ) ;
#35326=CIRCLE ( 'NONE', #70160, 4.875000000000017764 ) ;
#35327=ADVANCED_FACE ( 'NONE', ( #79892 ), #24024, .T. ) ;
#35329=DIRECTION ( 'NONE',  ( 0.7071067811873671394, 0.7071067811857280061, 6.612322855862553737E-17 ) ) ;
#35330=CARTESIAN_POINT ( 'NONE',  ( 112.5471327968798221, -30.46552556802231138, 288.9257531614101708 ) ) ;
#35331=CARTESIAN_POINT ( 'NONE',  ( 100.9543307028228583, -28.70728144113564539, 110.5939921354201374 ) ) ;
#35332=CARTESIAN_POINT ( 'NONE',  ( 96.04673288144557830, -37.20790665022158805, 112.3489586092449599 ) ) ;
#35335=VERTEX_POINT ( 'NONE', #1793 ) ;
#35337=FACE_BOUND ( 'NONE', #42964, .T. ) ;
#35338=FACE_OUTER_BOUND ( 'NONE', #67739, .T. ) ;
#35339=ORIENTED_EDGE ( 'NONE', *, *, #36654, .T. ) ;
#35340=ADVANCED_FACE ( 'NONE', ( #24466 ), #2240, .F. ) ;
#35341=CARTESIAN_POINT ( 'NONE',  ( 92.82872956494375671, -30.11307588647346023, 9.425625275910956447 ) ) ;
#35342=CARTESIAN_POINT ( 'NONE',  ( 95.86269369446621624, -32.71648115089089259, 176.0527681330539735 ) ) ;
#35343=ORIENTED_EDGE ( 'NONE', *, *, #57648, .T. ) ;
#35344=DIRECTION ( 'NONE',  ( 0.9825752044328148749, 0.1858654557302456822, 0.000000000000000000 ) ) ;
#35345=CARTESIAN_POINT ( 'NONE',  ( 113.1126646695910409, -46.01001268607183903, 219.0480062282919960 ) ) ;
#35346=CARTESIAN_POINT ( 'NONE',  ( 104.4799455178094405, -46.91020534057368963, 43.37848241876896083 ) ) ;
#35349=ADVANCED_FACE ( 'NONE', ( #78991 ), #16312, .T. ) ;
#35350=CARTESIAN_POINT ( 'NONE',  ( 90.44969454456416713, -53.34645651782494724, 218.8274735512160589 ) ) ;
#35352=B_SPLINE_CURVE_WITH_KNOTS ( 'NONE', 3,
 ( #50446, #50899, #60385, #4989, #47191, #26327, #80410, #33586, #67206, #82210, #87221, #61284, #19966, #54443, #74931, #53553, #81321, #67665, #52653, #68564, #89007, #19065, #59932, #47645, #75380, #18161, #25427, #26761, #45845 ),
 .UNSPECIFIED., .F., .F.,
 ( 4, 2, 2, 2, 2, 2, 2, 2, 2, 2, 1, 1, 1, 1, 1, 2, 4 ),
 ( 0.000000000000000000, 0.06250186238324358101, 0.1250037247664871620, 0.1875055871497307569, 0.2500074495329743240, 0.3125093119162178912, 0.3750111742994615138, 0.4375130366827050810, 0.4687639678743268368, 0.4843894334701378535, 0.4922021662680436394, 0.4961085326669965601, 0.4980617158664727984, 0.4990383074662109175, 0.4995266032660801714, 0.4997707511660147706, 0.5000148990659494252 ),
 .UNSPECIFIED. ) ;
#35353=CONICAL_SURFACE ( 'NONE', #86142, 1.624999999999987566, 1.029744258676650093 ) ;
#35354=AXIS2_PLACEMENT_3D ( 'NONE', #7672, #41273, #1761 ) ;
#35356=ORIENTED_EDGE ( 'NONE', *, *, #35217, .F. ) ;
#35357=VECTOR ( 'NONE', #53451, 1000.000000000000000 ) ;
#35359=CARTESIAN_POINT ( 'NONE',  ( 49.16670390244738797, -26.71338133339273924, 313.9678068554150059 ) ) ;
#35360=CARTESIAN_POINT ( 'NONE',  ( 113.7992560408602145, -26.97729936261201900, 235.5956252759109759 ) ) ;
#35362=CARTESIAN_POINT ( 'NONE',  ( 31.56670390244800828, -33.35206098992711077, 313.9678068554150059 ) ) ;
#35363=EDGE_CURVE ( 'NONE', #42590, #33552, #77904, .T. ) ;
#35364=DIRECTION ( 'NONE',  ( 0.000000000000000000, -1.000000000000000000, 0.000000000000000000 ) ) ;
#35365=CARTESIAN_POINT ( 'NONE',  ( 107.0664832912739399, -36.72944715994095333, 294.6356252759106837 ) ) ;
#35366=EDGE_CURVE ( 'NONE', #32980, #54776, #48021, .T. ) ;
#35367=LINE ( 'NONE', #14949, #41381 ) ;
#35368=CARTESIAN_POINT ( 'NONE',  ( 109.6173639926175269, -25.13086864565549661, 29.90419670448196854 ) ) ;
#35373=CARTESIAN_POINT ( 'NONE',  ( 116.8464009251321301, -35.91275531464980730, 249.8927681330532664 ) ) ;
#35375=CARTESIAN_POINT ( 'NONE',  ( 117.1895451461016648, -38.97942580829903392, 99.64038718067195077 ) ) ;
#35377=CARTESIAN_POINT ( 'NONE',  ( 116.3162594664470788, -32.94075446336835000, 20.13562527591095019 ) ) ;
#35378=EDGE_LOOP ( 'NONE', ( #33638, #30208, #4732, #51242 ) ) ;
#35381=ORIENTED_EDGE ( 'NONE', *, *, #51621, .T. ) ;
#35383=CARTESIAN_POINT ( 'NONE',  ( 101.2707639275114815, -30.02587231748817231, 257.0758690201828927 ) ) ;
#35384=CIRCLE ( 'NONE', #57104, 0.4999999999999982236 ) ;
#35385=EDGE_CURVE ( 'NONE', #26589, #64680, #12176, .T. ) ;
#35386=CARTESIAN_POINT ( 'NONE',  ( 104.4081005726111187, -46.45808911662692964, 192.3647919353561804 ) ) ;
#35387=DIRECTION ( 'NONE',  ( 0.000000000000000000, 0.000000000000000000, -1.000000000000000000 ) ) ;
#35389=CARTESIAN_POINT ( 'NONE',  ( 104.4899544645860061, -26.97880758150905223, 85.28145860822031921 ) ) ;
#35395=CARTESIAN_POINT ( 'NONE',  ( 100.9409889914183225, -46.87433776650586736, 52.14419670448194921 ) ) ;
#35396=EDGE_LOOP ( 'NONE', ( #37706, #28869, #47646, #23829 ) ) ;
#35397=CARTESIAN_POINT ( 'NONE',  ( 98.90470121413369498, -39.24767091914073802, 20.98670554236298358 ) ) ;
#35399=CARTESIAN_POINT ( 'NONE',  ( 109.2982854457139581, -26.60236246699145113, 179.8918157521019339 ) ) ;
#35402=DIRECTION ( 'NONE',  ( 0.000000000000000000, 0.000000000000000000, 1.000000000000000000 ) ) ;
#35403=LINE ( 'NONE', #77215, #62466 ) ;
#35405=CARTESIAN_POINT ( 'NONE',  ( 111.8841015539045713, -46.06371569386821818, 268.9556252759110180 ) ) ;
#35406=CARTESIAN_POINT ( 'NONE',  ( 101.5000928429637526, -45.09554281357727490, 117.1111000679451735 ) ) ;
#35407=ORIENTED_EDGE ( 'NONE', *, *, #50231, .T. ) ;
#35408=CARTESIAN_POINT ( 'NONE',  ( 136.4532669483771485, -38.09809895854112227, 7.205238605741180358 ) ) ;
#35410=ORIENTED_EDGE ( 'NONE', *, *, #61194, .F. ) ;
#35411=CARTESIAN_POINT ( 'NONE',  ( 106.0723295733845362, -48.58789440604735432, 108.5099109901969712 ) ) ;
#35412=DIRECTION ( 'NONE',  ( 0.000000000000000000, 1.000000000000000000, 0.000000000000000000 ) ) ;
#35416=ORIENTED_EDGE ( 'NONE', *, *, #558, .T. ) ;
#35417=EDGE_CURVE ( 'NONE', #79159, #22206, #5818, .T. ) ;
#35418=EDGE_CURVE ( 'NONE', #35754, #60336, #72066, .T. ) ;
#35419=VERTEX_POINT ( 'NONE', #12625 ) ;
#35420=DIRECTION ( 'NONE',  ( 0.9999999853157766072, 0.0001713722456134972175, 0.000000000000000000 ) ) ;
#35421=EDGE_CURVE ( 'NONE', #25045, #59341, #76401, .T. ) ;
#35422=CARTESIAN_POINT ( 'NONE',  ( 97.06106854294668551, -37.99639079834587108, 267.4272902591680463 ) ) ;
#35423=CARTESIAN_POINT ( 'NONE',  ( 69.67078994678415427, -0.9293259921821603875, 540.9756252759101471 ) ) ;
#35424=DIRECTION ( 'NONE',  ( 0.000000000000000000, -1.000000000000000000, 0.000000000000000000 ) ) ;
#35426=CARTESIAN_POINT ( 'NONE',  ( 110.9006160922534150, -26.97349402997008383, 265.7784824187680783 ) ) ;
#35430=EDGE_CURVE ( 'NONE', #88399, #24119, #46213, .T. ) ;
#35431=CARTESIAN_POINT ( 'NONE',  ( 116.3212776292271258, -32.94146857470711609, 44.13562527591097506 ) ) ;
#35433=ORIENTED_EDGE ( 'NONE', *, *, #15046, .T. ) ;
#35434=EDGE_CURVE ( 'NONE', #3872, #54700, #53145, .T. ) ;
#35435=CARTESIAN_POINT ( 'NONE',  ( 82.27374021058859910, -20.37320971852071594, 2.471387388688038644 ) ) ;
#35437=CARTESIAN_POINT ( 'NONE',  ( 108.4174480110805661, -26.73502967738932767, 14.96896184951245345 ) ) ;
#35438=CARTESIAN_POINT ( 'NONE',  ( 143.0664832912740110, -18.82844715994099971, 17.92562527591199739 ) ) ;
#35439=LINE ( 'NONE', #82285, #46080 ) ;
#35441=CARTESIAN_POINT ( 'NONE',  ( 104.3272728202184538, -28.09756461201434874, 204.7314674471249702 ) ) ;
#35443=CARTESIAN_POINT ( 'NONE',  ( 107.6054179116733707, -26.23843464447702090, 95.03562527591097364 ) ) ;
#35445=DIRECTION ( 'NONE',  ( 1.000000000000000000, 1.765660420430506939E-15, 0.000000000000000000 ) ) ;
#35449=CARTESIAN_POINT ( 'NONE',  ( 115.8245126124521391, -31.72842839644282620, 260.2397945930957803 ) ) ;
#35453=CARTESIAN_POINT ( 'NONE',  ( 108.3350409249663926, -46.73467830386606181, 273.6769742538326682 ) ) ;
#35454=VECTOR ( 'NONE', #53085, 1000.000000000000000 ) ;
#35457=CARTESIAN_POINT ( 'NONE',  ( 118.1065893711158594, -37.63027948749972751, 38.77372051400595865 ) ) ;
#35459=CYLINDRICAL_SURFACE ( 'NONE', #24577, 2.117000000000000881 ) ;
#35460=DIRECTION ( 'NONE',  ( 0.7071067811865779928, -0.7071067811865171526, 7.071067811865786933E-16 ) ) ;
#35462=CARTESIAN_POINT ( 'NONE',  ( 132.3549177285000269, -16.56918551487757085, 2.099346190920966748 ) ) ;
#35463=VERTEX_POINT ( 'NONE', #46670 ) ;
#35465=FACE_OUTER_BOUND ( 'NONE', #85146, .T. ) ;
#35467=CARTESIAN_POINT ( 'NONE',  ( 113.8705839548662908, -44.65670854160515546, 104.1413395616249744 ) ) ;
#35469=LINE ( 'NONE', #55899, #63034 ) ;
#35470=EDGE_CURVE ( 'NONE', #86726, #10270, #73493, .T. ) ;
#35473=VERTEX_POINT ( 'NONE', #63454 ) ;
#35474=VECTOR ( 'NONE', #57255, 1000.000000000000000 ) ;
#35475=VECTOR ( 'NONE', #14506, 1000.000000000000000 ) ;
#35478=CARTESIAN_POINT ( 'NONE',  ( 114.2526777242400726, -43.36435822665418982, 119.2327681330529714 ) ) ;
#35480=ORIENTED_EDGE ( 'NONE', *, *, #77095, .T. ) ;
#35482=AXIS2_PLACEMENT_3D ( 'NONE', #62750, #84571, #63659 ) ;
#35483=CARTESIAN_POINT ( 'NONE',  ( 118.3173389373706925, -33.08695204176930105, 280.0756252759109657 ) ) ;
#35484=CARTESIAN_POINT ( 'NONE',  ( 98.15039990372359568, -41.26047703464855232, 252.7008027240838999 ) ) ;
#35485=PLANE ( 'NONE',  #86732 ) ;
#35490=CARTESIAN_POINT ( 'NONE',  ( 96.12852455334814294, -38.72269610271991525, 201.4699109901969791 ) ) ;
#35491=VERTEX_POINT ( 'NONE', #21232 ) ;
#35492=ORIENTED_EDGE ( 'NONE', *, *, #38684, .F. ) ;
#35493=CARTESIAN_POINT ( 'NONE',  ( 100.5685618138929271, -29.03188392736010570, 147.0672975916109806 ) ) ;
#35494=ADVANCED_FACE ( 'NONE', ( #1240 ), #7603, .T. ) ;
#35496=CARTESIAN_POINT ( 'NONE',  ( 115.8371248229627639, -37.99598801341877419, 25.14444044875396855 ) ) ;
#35498=AXIS2_PLACEMENT_3D ( 'NONE', #72443, #59239, #72002 ) ;
#35499=DIRECTION ( 'NONE',  ( 0.7071067811575898476, -0.7071067812155052978, 0.000000000000000000 ) ) ;
#35501=DIRECTION ( 'NONE',  ( 0.1858654558203329255, -0.9825752044157738396, 0.000000000000000000 ) ) ;
#35503=CARTESIAN_POINT ( 'NONE',  ( 105.1150531980676277, -26.51080800785435443, 235.2270538473399313 ) ) ;
#35505=ORIENTED_EDGE ( 'NONE', *, *, #82944, .F. ) ;
#35506=ORIENTED_EDGE ( 'NONE', *, *, #7673, .T. ) ;
#35508=CARTESIAN_POINT ( 'NONE',  ( 82.76352869194700190, -19.26660482608858160, 6.827192804310135976 ) ) ;
#35509=CARTESIAN_POINT ( 'NONE',  ( 97.81262911421374895, -40.51702269960655656, 122.6351715870756323 ) ) ;
#35510=LINE ( 'NONE', #14649, #34629 ) ;
#35512=CARTESIAN_POINT ( 'NONE',  ( 104.6499073705539473, -46.24122592705968771, 43.37848241876795896 ) ) ;
#35514=ORIENTED_EDGE ( 'NONE', *, *, #87438, .T. ) ;
#35515=CARTESIAN_POINT ( 'NONE',  ( 96.29945253806019423, -39.42498279898523350, 12.53372051400597442 ) ) ;
#35516=CARTESIAN_POINT ( 'NONE',  ( 180.1667039024474377, -28.27351298636767396, 313.9678068554149490 ) ) ;
#35517=AXIS2_PLACEMENT_3D ( 'NONE', #69772, #42486, #29339 ) ;
#35518=CARTESIAN_POINT ( 'NONE',  ( 116.0552987087602048, -42.01037774571695849, 238.4041967044829562 ) ) ;
#35519=ADVANCED_FACE ( 'NONE', ( #14877 ), #76640, .T. ) ;
#35521=ADVANCED_FACE ( 'NONE', ( #41201 ), #62997, .T. ) ;
#35522=CARTESIAN_POINT ( 'NONE',  ( 77.41433294703958268, -37.45719076514816948, 6.889371645759243989 ) ) ;
#35525=CARTESIAN_POINT ( 'NONE',  ( 116.3159136950847170, -32.94903743517052419, 150.1356252759109680 ) ) ;
#35526=CARTESIAN_POINT ( 'NONE',  ( 107.6943352634791182, -28.59092592337147209, 67.83380465530596837 ) ) ;
#35527=CARTESIAN_POINT ( 'NONE',  ( 117.0439256081559165, -39.94344854842797332, 154.5784824187679476 ) ) ;
#35529=ORIENTED_EDGE ( 'NONE', *, *, #3959, .T. ) ;
#35530=EDGE_CURVE ( 'NONE', #38211, #43566, #82258, .T. ) ;
#35531=CARTESIAN_POINT ( 'NONE',  ( 34.33598329127499227, -36.32844715994100682, -5.074374724088000832 ) ) ;
#35534=VECTOR ( 'NONE', #38387, 1000.000000000000114 ) ;
#35535=AXIS2_PLACEMENT_3D ( 'NONE', #11242, #46641, #26217 ) ;
#35536=CARTESIAN_POINT ( 'NONE',  ( 167.6524903400755306, -48.32844715993520879, 180.4678068554150059 ) ) ;
#35537=CIRCLE ( 'NONE', #64546, 2.517500000000005844 ) ;
#35543=EDGE_CURVE ( 'NONE', #65069, #82508, #31447, .T. ) ;
#35544=CARTESIAN_POINT ( 'NONE',  ( 104.0317209996959065, -45.26190801010356779, 101.7390864947439724 ) ) ;
#35546=CARTESIAN_POINT ( 'NONE',  ( 99.38058175836560793, -28.75308465796231516, 265.6746728949588032 ) ) ;
#35547=CARTESIAN_POINT ( 'NONE',  ( 101.4371718687637838, -46.21494532752030437, 207.1622919425779514 ) ) ;
#35551=CARTESIAN_POINT ( 'NONE',  ( 109.6407213914652345, -46.48066322255345284, 93.78127252070859754 ) ) ;
#35552=ORIENTED_EDGE ( 'NONE', *, *, #69111, .T. ) ;
#35553=CARTESIAN_POINT ( 'NONE',  ( 131.0667039024480687, -58.72944715994092491, 231.5838068554170093 ) ) ;
#35554=CARTESIAN_POINT ( 'NONE',  ( 156.5667039024480971, -42.82844715993568485, 290.7178068554149490 ) ) ;
#35555=CARTESIAN_POINT ( 'NONE',  ( 142.8679068202682458, 10.65431904611001634, 542.9756252759101471 ) ) ;
#35557=CARTESIAN_POINT ( 'NONE',  ( 98.98846131648976154, -42.30253745798197684, 126.8070538473399580 ) ) ;
#35558=CARTESIAN_POINT ( 'NONE',  ( 96.04102276344947597, -38.01478905114413465, 86.43086337114897333 ) ) ;
#35559=CARTESIAN_POINT ( 'NONE',  ( 118.7030916724021665, -39.22306760090339139, 258.6584824187677896 ) ) ;
#35560=VERTEX_POINT ( 'NONE', #6254 ) ;
#35561=CARTESIAN_POINT ( 'NONE',  ( 115.8553914792215380, -44.67901184617146981, 233.2413395616259493 ) ) ;
#35562=FACE_OUTER_BOUND ( 'NONE', #82704, .T. ) ;
#35564=CARTESIAN_POINT ( 'NONE',  ( 130.5667039024480118, -36.72944715994093912, 218.0711402470151370 ) ) ;
#35566=CARTESIAN_POINT ( 'NONE',  ( 107.8173249548519692, -46.71069529603006032, 277.6356222035115024 ) ) ;
#35567=DIRECTION ( 'NONE',  ( 1.000000000000000078E-15, -1.000000000000000083E-30, -1.000000000000000000 ) ) ;
#35568=CARTESIAN_POINT ( 'NONE',  ( 105.1200014541032601, -25.43661125475656704, 321.6731097870184044 ) ) ;
#35570=DIRECTION ( 'NONE',  ( 0.000000000000000000, 0.000000000000000000, -1.000000000000000000 ) ) ;
#35571=DIRECTION ( 'NONE',  ( 0.000000000000000000, 0.000000000000000000, 1.000000000000000000 ) ) ;
#35577=CARTESIAN_POINT ( 'NONE',  ( 109.9954698844069156, -26.70111721404902383, 259.8499109901965767 ) ) ;
#35578=CARTESIAN_POINT ( 'NONE',  ( 102.3604841619309411, -46.03192315517718214, 123.2041967044829818 ) ) ;
#35579=CARTESIAN_POINT ( 'NONE',  ( 112.1278237076712543, -26.87713336146359211, 15.71086337114896381 ) ) ;
#35580=PLANE ( 'NONE',  #24374 ) ;
#35583=EDGE_CURVE ( 'NONE', #37091, #87995, #21021, .T. ) ;
#35584=CARTESIAN_POINT ( 'NONE',  ( 98.15094550295600584, -41.26155033938827188, 137.7007176044859307 ) ) ;
#35586=AXIS2_PLACEMENT_3D ( 'NONE', #80400, #60373, #88112 ) ;
#35587=ADVANCED_FACE ( 'NONE', ( #77099 ), #20779, .F. ) ;
#35589=DIRECTION ( 'NONE',  ( -0.000000000000000000, 1.000000000000000000, 0.000000000000000000 ) ) ;
#35590=ORIENTED_EDGE ( 'NONE', *, *, #58591, .T. ) ;
#35591=B_SPLINE_CURVE_WITH_KNOTS ( 'NONE', 3,
 ( #71464, #50541, #37371, #65077, #1522, #36028, #50990, #30997, #86430, #9227, #78283, #16488, #79174, #58257, #79617, #9662, #23758, #2859, #30559, #17374, #85987, #8789, #16934, #70558, #8330, #63742, #56911, #50088, #77822, #15600, #25978, #73673, #52297, #11455, #10996, #81418, #38696, #80060 ),
 .UNSPECIFIED., .F., .F.,
 ( 4, 2, 2, 1, 2, 2, 2, 2, 1, 1, 2, 2, 2, 1, 2, 2, 1, 2, 1, 2, 2, 4 ),
 ( 0.000000000000000000, 0.04166793602361257287, 0.05208492002951500832, 0.05729341203246553910, 0.05989765803394084265, 0.06250190403541615314, 0.08333587204722690822, 0.1041698400590376355, 0.1145868240649424580, 0.1197953160678960766, 0.1223995620693742042, 0.1250038080708523180, 0.1666717440944873729, 0.1770887281003949987, 0.1822972201033483952, 0.1875057121063017640, 0.2083396801181268687, 0.2291736481299520012, 0.2395906321358649282, 0.2447991241388212946, 0.2500076161417776888, 0.3333434881890902091 ),
 .UNSPECIFIED. ) ;
#35592=B_SPLINE_CURVE_WITH_KNOTS ( 'NONE', 3,
 ( #27860, #62825, #36026, #55538, #56452, #83292, #55993, #21971, #83739, #21516, #49186, #35568, #49637, #63739, #29222, #56909, #84645, #22409, #65518, #79615, #16932, #79172, #38693, #51423, #45055, #65953, #44610, #16045 ),
 .UNSPECIFIED., .F., .F.,
 ( 4, 2, 2, 2, 2, 2, 2, 2, 2, 2, 2, 2, 2, 4 ),
 ( 0.000000000000000000, 0.0002934189718615978055, 0.0005868379437231956109, 0.0008802569155847934706, 0.001173675887446391222, 0.001760513831169494784, 0.002347351774892598129, 0.002640770746754149152, 0.002934189718615699740, 0.003521027662338802652, 0.003814446634200298163, 0.004107865606061793240, 0.004401284577923288317, 0.004694703549784783395 ),
 .UNSPECIFIED. ) ;
#35593=CARTESIAN_POINT ( 'NONE',  ( 99.16725398249624845, -41.15831232534042528, 181.1676579233149482 ) ) ;
#35597=CARTESIAN_POINT ( 'NONE',  ( 97.69433714244412670, -41.24514667321082584, 167.6841967044829573 ) ) ;
#35598=CARTESIAN_POINT ( 'NONE',  ( 115.0351528678677226, -42.91113197315783623, 149.3027457930269861 ) ) ;
#35600=CARTESIAN_POINT ( 'NONE',  ( 114.8717157601983132, -30.43847619068483468, 85.36600443824613649 ) ) ;
#35602=CARTESIAN_POINT ( 'NONE',  ( 31.56670390244700641, -22.48495420874110806, -5.074374724088000832 ) ) ;
#35603=CARTESIAN_POINT ( 'NONE',  ( 116.7039036015866031, -32.90075090702271865, 99.13943479972198247 ) ) ;
#35604=ORIENTED_EDGE ( 'NONE', *, *, #81399, .F. ) ;
#35608=CARTESIAN_POINT ( 'NONE',  ( 102.0296606431220994, -28.79805742369273958, 61.94634521065894717 ) ) ;
#35611=CYLINDRICAL_SURFACE ( 'NONE', #48621, 2.517499999999998739 ) ;
#35612=CARTESIAN_POINT ( 'NONE',  ( 114.3351522754912963, -30.13549343754564092, 205.4127681330539872 ) ) ;
#35613=DIRECTION ( 'NONE',  ( -1.000000000000000000, 0.000000000000000000, 0.000000000000000000 ) ) ;
#35614=VECTOR ( 'NONE', #61775, 1000.000000000000000 ) ;
#35616=CARTESIAN_POINT ( 'NONE',  ( 141.8664832912729992, -1.929447159941394263, 342.9256252759109316 ) ) ;
#35619=CARTESIAN_POINT ( 'NONE',  ( 142.8821648370248170, -72.54478064608022692, 542.9756252759101471 ) ) ;
#35621=CARTESIAN_POINT ( 'NONE',  ( 102.3122812202564376, -27.43633205498510108, 120.4527681330539792 ) ) ;
#35623=EDGE_LOOP ( 'NONE', ( #67040, #85913, #40967, #56173, #1996 ) ) ;
#35624=ORIENTED_EDGE ( 'NONE', *, *, #38941, .T. ) ;
#35626=ORIENTED_CLOSED_SHELL ( 'NONE', *, #60448, .F. );
#35628=DIRECTION ( 'NONE',  ( -0.7071067811866279529, 0.7071067811864671926, -7.071067811865978232E-16 ) ) ;
#35629=CARTESIAN_POINT ( 'NONE',  ( 116.8171344286183029, -34.15294656915441607, 105.0314561802934321 ) ) ;
#35630=AXIS2_PLACEMENT_3D ( 'NONE', #58173, #58603, #37286 ) ;
#35631=CARTESIAN_POINT ( 'NONE',  ( 103.2852591291245830, -43.96353797031052579, 210.0109475124489506 ) ) ;
#35632=B_SPLINE_CURVE_WITH_KNOTS ( 'NONE', 3,
 ( #50478, #38198, #43664, #65894, #29156, #56840, #84586, #9165, #36862, #22349, #52679, #73156, #12285, #80895, #67691, #32262, #80439, #38634, #67235, #18195, #45433, #10932, #59515, #45874, #54025, #60410, #88154, #59066, #3679 ),
 .UNSPECIFIED., .F., .F.,
 ( 4, 2, 1, 1, 1, 1, 1, 2, 2, 2, 2, 2, 2, 2, 2, 2, 4 ),
 ( 0.5000592588468526500, 0.5003033705368687967, 0.5005474822268849433, 0.5010357056069173476, 0.5020121523669820451, 0.5039650458871114402, 0.5078708329273705635, 0.5156824070078886990, 0.5313055551689245259, 0.5625518514909964018, 0.6250444441351398206, 0.6875370367792832393, 0.7500296294234265471, 0.8125222220675698548, 0.8750148147117132735, 0.9375074073558566923, 1.000000000000000000 ),
 .UNSPECIFIED. ) ;
#35633=DIRECTION ( 'NONE',  ( -0.9963424814100679816, 0.08544974978095716545, 0.000000000000000000 ) ) ;
#35635=DIRECTION ( 'NONE',  ( -3.999999999999999995E-14, 1.000000000000000000, -4.100000000000000342E-29 ) ) ;
#35637=VERTEX_POINT ( 'NONE', #54817 ) ;
#35639=DIRECTION ( 'NONE',  ( 0.000000000000000000, 0.000000000000000000, 1.000000000000000000 ) ) ;
#35640=ORIENTED_EDGE ( 'NONE', *, *, #42514, .T. ) ;
#35641=ORIENTED_EDGE ( 'NONE', *, *, #61973, .F. ) ;
#35642=CARTESIAN_POINT ( 'NONE',  ( 78.34779240611281637, -20.87777042261386740, 7.743969477059374107 ) ) ;
#35643=EDGE_CURVE ( 'NONE', #71592, #88986, #20341, .T. ) ;
#35644=CARTESIAN_POINT ( 'NONE',  ( 114.7070687854681807, -41.21829243659817621, 234.8358690201829404 ) ) ;
#35645=CARTESIAN_POINT ( 'NONE',  ( 172.5664832912729878, -27.82844715994070484, 198.9256252759119832 ) ) ;
#35646=ORIENTED_EDGE ( 'NONE', *, *, #5615, .F. ) ;
#35650=ORIENTED_EDGE ( 'NONE', *, *, #40374, .F. ) ;
#35652=DIRECTION ( 'NONE',  ( 0.7071067811865671127, 0.7071067811865279218, 7.071067811865664660E-16 ) ) ;
#35654=ORIENTED_EDGE ( 'NONE', *, *, #39952, .T. ) ;
#35655=EDGE_CURVE ( 'NONE', #58384, #35419, #75748, .T. ) ;
#35656=CARTESIAN_POINT ( 'NONE',  ( 114.4813385407417741, -41.19272473522806166, 276.2014237029247852 ) ) ;
#35657=CARTESIAN_POINT ( 'NONE',  ( 105.3125257651413307, -48.47460025707392361, 147.4584824187679715 ) ) ;
#35658=CARTESIAN_POINT ( 'NONE',  ( 109.2504006710444315, -46.93703897017543625, 107.7441967044829880 ) ) ;
#35659=CARTESIAN_POINT ( 'NONE',  ( 116.1386594504526357, -39.99393533005606827, 249.5838068554177482 ) ) ;
#35661=DIRECTION ( 'NONE',  ( 0.000000000000000000, 0.000000000000000000, 1.000000000000000000 ) ) ;
#35662=CARTESIAN_POINT ( 'NONE',  ( 115.5173804941753133, -29.60510038635626273, 220.3718157521019521 ) ) ;
#35663=DIRECTION ( 'NONE',  ( 0.000000000000000000, 0.000000000000000000, 1.000000000000000000 ) ) ;
#35667=EDGE_LOOP ( 'NONE', ( #49450, #85341, #67039 ) ) ;
#35670=VECTOR ( 'NONE', #60983, 1000.000000000000000 ) ;
#35671=DIRECTION ( 'NONE',  ( -0.7071067811865789920, 0.7071067811865159314, 0.000000000000000000 ) ) ;
#35672=AXIS2_PLACEMENT_3D ( 'NONE', #46307, #81331, #48098 ) ;
#35673=ORIENTED_EDGE ( 'NONE', *, *, #10674, .T. ) ;
#35674=AXIS2_PLACEMENT_3D ( 'NONE', #15073, #28232, #43202 ) ;
#35675=CARTESIAN_POINT ( 'NONE',  ( 117.6792309033718027, -39.81954026856703877, 138.5889586092439743 ) ) ;
#35676=CARTESIAN_POINT ( 'NONE',  ( 97.07216983056154902, -35.37748917612672273, 256.2188997677546922 ) ) ;
#35677=VECTOR ( 'NONE', #34158, 1000.000000000000000 ) ;
#35679=FACE_OUTER_BOUND ( 'NONE', #14398, .T. ) ;
#35682=CARTESIAN_POINT ( 'NONE',  ( 111.1189502094634776, -27.14789314160936229, 240.7584824187679544 ) ) ;
#35684=CARTESIAN_POINT ( 'NONE',  ( 33.92127028473468187, -29.73316016639587644, 117.4678068554150485 ) ) ;
#35685=CARTESIAN_POINT ( 'NONE',  ( 29.56648329127298069, 15.62155284005731204, 361.9756252759109998 ) ) ;
#35687=CARTESIAN_POINT ( 'NONE',  ( 108.4174892396751630, -26.73503592576763666, 255.9689586102375642 ) ) ;
#35689=CARTESIAN_POINT ( 'NONE',  ( 116.6223143332234997, -42.37736834728454483, 283.4137205140060018 ) ) ;
#35690=ORIENTED_EDGE ( 'NONE', *, *, #68724, .T. ) ;
#35692=CARTESIAN_POINT ( 'NONE',  ( 103.0412047595748959, -26.40992324271003966, 170.3603871806729444 ) ) ;
#35693=CARTESIAN_POINT ( 'NONE',  ( 104.6489182489307552, -47.51505607846939938, 23.38895860924494841 ) ) ;
#35694=CARTESIAN_POINT ( 'NONE',  ( 115.0109179074633374, -28.97809521412381883, 190.4537205140059655 ) ) ;
#35695=CARTESIAN_POINT ( 'NONE',  ( 99.09570896555410968, -30.55043189343225052, 31.80229195668304953 ) ) ;
#35697=VECTOR ( 'NONE', #85800, 999.9999999999998863 ) ;
#35700=CARTESIAN_POINT ( 'NONE',  ( 49.35031423293201414, -29.99615139349890569, 237.4678068554150059 ) ) ;
#35701=DIRECTION ( 'NONE',  ( 0.000000000000000000, 0.000000000000000000, -1.000000000000000000 ) ) ;
#35708=CARTESIAN_POINT ( 'NONE',  ( 154.4532655810166091, -72.54279768053238797, 540.9756252759101471 ) ) ;
#35709=EDGE_LOOP ( 'NONE', ( #76148, #81839, #82583, #72857 ) ) ;
#35710=CARTESIAN_POINT ( 'NONE',  ( 103.9639062230919251, -47.31423993612432355, 58.33753003781600199 ) ) ;
#35711=CARTESIAN_POINT ( 'NONE',  ( 37.36643805256586859, -48.62818131006087441, 180.4678068554150911 ) ) ;
#35712=DIRECTION ( 'NONE',  ( 0.000000000000000000, 0.000000000000000000, -1.000000000000000000 ) ) ;
#35713=CARTESIAN_POINT ( 'NONE',  ( 99.97865438147567829, -27.17048309217152990, 181.5841967044829630 ) ) ;
#35714=CARTESIAN_POINT ( 'NONE',  ( 114.8626455990942361, -41.33732585285711991, 282.8362293518863453 ) ) ;
#35715=EDGE_LOOP ( 'NONE', ( #65657, #8891, #60620, #73844 ) ) ;
#35716=ORIENTED_EDGE ( 'NONE', *, *, #14734, .T. ) ;
#35717=ORIENTED_EDGE ( 'NONE', *, *, #53043, .T. ) ;
#35718=ADVANCED_FACE ( 'NONE', ( #78893 ), #73536, .F. ) ;
#35720=CARTESIAN_POINT ( 'NONE',  ( 99.04406186213515184, -42.84125764447927054, 106.8439586097051688 ) ) ;
#35722=CARTESIAN_POINT ( 'NONE',  ( 72.26949937496598864, -71.54137415153812185, 361.9756252759101471 ) ) ;
#35725=DIRECTION ( 'NONE',  ( 1.000000000000000000, 0.000000000000000000, 0.000000000000000000 ) ) ;
#35728=CARTESIAN_POINT ( 'NONE',  ( 115.8731522275743941, -31.19128430790902584, 34.27276813305396530 ) ) ;
#35730=EDGE_CURVE ( 'NONE', #45118, #9390, #50257, .T. ) ;
#35732=EDGE_CURVE ( 'NONE', #45, #89358, #65245, .T. ) ;
#35733=CARTESIAN_POINT ( 'NONE',  ( 115.0889047923113964, -30.61763678268615863, 269.3439585996102892 ) ) ;
#35734=DIRECTION ( 'NONE',  ( -4.237773401492740281E-14, 1.000000000000000000, 0.000000000000000000 ) ) ;
#35735=CARTESIAN_POINT ( 'NONE',  ( 115.1210532203963766, -38.21490719095142197, 86.49951894101998562 ) ) ;
#35736=VECTOR ( 'NONE', #30938, 1000.000000000000000 ) ;
#35738=AXIS2_PLACEMENT_3D ( 'NONE', #59063, #58193, #24568 ) ;
#35743=ORIENTED_EDGE ( 'NONE', *, *, #48753, .T. ) ;
#35745=ORIENTED_EDGE ( 'NONE', *, *, #32362, .F. ) ;
#35746=ORIENTED_EDGE ( 'NONE', *, *, #23257, .F. ) ;
#35747=ADVANCED_FACE ( 'NONE', ( #42988 ), #64358, .T. ) ;
#35748=CARTESIAN_POINT ( 'NONE',  ( 115.7737780547358710, -35.08282516751891933, 155.4072975916109556 ) ) ;
#35751=CARTESIAN_POINT ( 'NONE',  ( 116.9955931624231624, -33.48136526131695234, 85.07848241876791917 ) ) ;
#35752=CARTESIAN_POINT ( 'NONE',  ( 59.67079009362632291, -0.9310397146383332379, 542.9756252759101471 ) ) ;
#35753=VERTEX_POINT ( 'NONE', #1690 ) ;
#35754=VERTEX_POINT ( 'NONE', #43439 ) ;
#35757=FACE_OUTER_BOUND ( 'NONE', #19105, .T. ) ;
#35758=VERTEX_POINT ( 'NONE', #16213 ) ;
#35759=CARTESIAN_POINT ( 'NONE',  ( 105.3240584539683766, -26.47319898023375728, 15.20991099019697401 ) ) ;
#35760=CARTESIAN_POINT ( 'NONE',  ( 116.6808514842340259, -40.81615526105927927, 164.5070538473399608 ) ) ;
#35761=EDGE_CURVE ( 'NONE', #23447, #2591, #29990, .T. ) ;
#35762=FACE_BOUND ( 'NONE', #69585, .T. ) ;
#35764=CARTESIAN_POINT ( 'NONE',  ( 108.0341493669268260, -25.71865232712709215, 105.9946728949589811 ) ) ;
#35765=CARTESIAN_POINT ( 'NONE',  ( 194.0667039024475571, -24.92844715993407334, 129.9678068554150343 ) ) ;
#35766=ADVANCED_FACE ( 'NONE', ( #16652 ), #71183, .T. ) ;
#35769=EDGE_CURVE ( 'NONE', #33407, #24965, #36200, .T. ) ;
#35770=ORIENTED_EDGE ( 'NONE', *, *, #24475, .T. ) ;
#35771=CARTESIAN_POINT ( 'NONE',  ( 117.0610774055309093, -38.07918021125614416, 134.7195873375643203 ) ) ;
#35773=ORIENTED_EDGE ( 'NONE', *, *, #32250, .T. ) ;
#35776=CARTESIAN_POINT ( 'NONE',  ( 111.4155313275575168, -46.20429869645016652, 27.91848241876792969 ) ) ;
#35778=CARTESIAN_POINT ( 'NONE',  ( 71.25416588882602298, -72.55705569728901594, 540.9756252759101471 ) ) ;
#35780=CARTESIAN_POINT ( 'NONE',  ( 114.3402351757609665, -43.26825200597438226, 38.24419670448392594 ) ) ;
#35781=LINE ( 'NONE', #1280, #78297 ) ;
#35782=CARTESIAN_POINT ( 'NONE',  ( 117.2167691715782070, -39.01263929987993606, 144.6499109901969859 ) ) ;
#35783=CARTESIAN_POINT ( 'NONE',  ( 34.27482367531500529, -30.08671355700301575, -5.074374724088000832 ) ) ;
#35789=ORIENTED_EDGE ( 'NONE', *, *, #63004, .T. ) ;
#35791=CARTESIAN_POINT ( 'NONE',  ( 99.25559070964938257, -29.75831933708737864, 190.7470538473399415 ) ) ;
#35793=DIRECTION ( 'NONE',  ( 1.000000000000000000, 4.299999999999999979E-14, 1.000000000000000078E-15 ) ) ;
#35794=CARTESIAN_POINT ( 'NONE',  ( 100.6429626219512983, -44.96811459249982335, 228.0499109901969348 ) ) ;
#35795=CARTESIAN_POINT ( 'NONE',  ( 112.5370353716610055, -27.80386372334747236, 90.63848241876793566 ) ) ;
#35796=VECTOR ( 'NONE', #75761, 999.9999999999998863 ) ;
#35798=CARTESIAN_POINT ( 'NONE',  ( 57.56670390244735103, -48.82844715994040286, 139.7178068554150911 ) ) ;
#35799=CARTESIAN_POINT ( 'NONE',  ( 176.7669697523278955, -48.62818131005232658, 249.9678068554149775 ) ) ;
#35802=AXIS2_PLACEMENT_3D ( 'NONE', #88715, #6047, #40543 ) ;
#35804=AXIS2_PLACEMENT_3D ( 'NONE', #85818, #38086, #84921 ) ;
#35805=B_SPLINE_CURVE_WITH_KNOTS ( 'NONE', 3,
 ( #43051, #10343, #67087, #80732, #52089, #66180, #18942, #24863, #59806, #38477, #11224, #3970, #86651, #79849, #72576, #87097, #52531, #3518, #10770, #24427, #53877, #73006, #58914, #18482, #80293, #17607, #38929, #81192, #87540, #45287, #73449, #25300, #31218, #38049, #46625 ),
 .UNSPECIFIED., .F., .F.,
 ( 4, 2, 2, 1, 1, 2, 2, 2, 2, 2, 2, 1, 1, 2, 2, 2, 1, 1, 1, 2, 4 ),
 ( 0.3333434881890895429, 0.4166701562234092493, 0.4218780729755542414, 0.4270859897276991779, 0.4375018232319922706, 0.4583334902405750699, 0.4999968242577399469, 0.5208284912663228017, 0.5416601582749056565, 0.5624918252834885113, 0.5650957836595601469, 0.5676997420356317825, 0.5729076587877761639, 0.5833234922920649268, 0.6249868263092226428, 0.6275907846852966099, 0.6301947430613705770, 0.6354026598135189552, 0.6458184933178172660, 0.6562343268221155768, 0.6666501603264138875 ),
 .UNSPECIFIED. ) ;
#35806=ORIENTED_EDGE ( 'NONE', *, *, #75488, .F. ) ;
#35809=DIRECTION ( 'NONE',  ( 1.000000000000000078E-15, -1.000000000000000083E-30, -1.000000000000000000 ) ) ;
#35810=CARTESIAN_POINT ( 'NONE',  ( 113.2200137887798235, -45.14470412949270184, 224.0784824187679476 ) ) ;
#35811=CARTESIAN_POINT ( 'NONE',  ( 41.56648329127399677, -18.82844715994099971, 198.9256252759119832 ) ) ;
#35812=CARTESIAN_POINT ( 'NONE',  ( 180.1667039024460166, -28.27351298637340093, 342.9256252759119548 ) ) ;
#35816=AXIS2_PLACEMENT_3D ( 'NONE', #57675, #42684, #23196 ) ;
#35817=CARTESIAN_POINT ( 'NONE',  ( 117.5344697633125577, -37.28603910398157240, 18.78419670448294809 ) ) ;
#35818=ORIENTED_EDGE ( 'NONE', *, *, #19603, .T. ) ;
#35819=ORIENTED_EDGE ( 'NONE', *, *, #29915, .T. ) ;
#35820=CLOSED_SHELL ( 'NONE', ( #54060, #59708, #77498, #75862 ) ) ;
#35822=CARTESIAN_POINT ( 'NONE',  ( 97.06380509542137247, -37.34170171876225908, 17.37620855293377886 ) ) ;
#35823=EDGE_CURVE ( 'NONE', #67197, #2317, #44787, .T. ) ;
#35824=CARTESIAN_POINT ( 'NONE',  ( 110.0587659310071302, -27.38278898179171605, 230.8299109901959412 ) ) ;
#35825=DIRECTION ( 'NONE',  ( 1.000000000000000078E-15, -1.000000000000000000, 0.000000000000000000 ) ) ;
#35827=CARTESIAN_POINT ( 'NONE',  ( 116.3126599349420900, -33.43976754494801185, 110.0984824187669631 ) ) ;
#35830=EDGE_CURVE ( 'NONE', #33306, #15468, #24274, .T. ) ;
#35832=CARTESIAN_POINT ( 'NONE',  ( 162.7131505118547352, -33.70561438051439040, 237.4678068554150059 ) ) ;
#35833=EDGE_CURVE ( 'NONE', #2950, #44520, #9389, .T. ) ;
#35834=ORIENTED_EDGE ( 'NONE', *, *, #58310, .T. ) ;
#35835=ORIENTED_EDGE ( 'NONE', *, *, #36390, .T. ) ;
#35837=CARTESIAN_POINT ( 'NONE',  ( 105.1749981762835802, -28.04127050161159218, 256.6787261630399826 ) ) ;
#35838=CIRCLE ( 'NONE', #5372, 2.517499999999998739 ) ;
#35839=EDGE_CURVE ( 'NONE', #70760, #82741, #17544, .T. ) ;
#35840=CARTESIAN_POINT ( 'NONE',  ( 108.3334480201780963, -46.73485936414270725, 192.6772919366305246 ) ) ;
#35843=CARTESIAN_POINT ( 'NONE',  ( 97.81169818311565223, -40.51742792548894556, 86.63555527419073599 ) ) ;
#35845=ORIENTED_EDGE ( 'NONE', *, *, #67614, .T. ) ;
#35846=CARTESIAN_POINT ( 'NONE',  ( 105.7809510460201210, -24.27257308096163868, 321.6188579224977389 ) ) ;
#35847=LINE ( 'NONE', #15430, #57134 ) ;
#35849=CARTESIAN_POINT ( 'NONE',  ( 96.95653860995706452, -32.26087848594701057, 55.98324432352897162 ) ) ;
#35851=CARTESIAN_POINT ( 'NONE',  ( 99.21763626795888058, -33.35996782468227195, 15.42670554236297242 ) ) ;
#35854=CARTESIAN_POINT ( 'NONE',  ( 102.3610132369663148, -45.97051510703457922, 172.2137205140069511 ) ) ;
#35856=VECTOR ( 'NONE', #10665, 1000.000000000000000 ) ;
#35857=CARTESIAN_POINT ( 'NONE',  ( 131.0667039024480403, -43.72944715994093201, 207.5838068554170377 ) ) ;
#35859=AXIS2_PLACEMENT_3D ( 'NONE', #66319, #73591, #52663 ) ;
#35860=CARTESIAN_POINT ( 'NONE',  ( 177.0371591254543659, -48.62818131005480637, 249.9678068554149775 ) ) ;
#35861=CARTESIAN_POINT ( 'NONE',  ( 105.1596118751612323, -47.03031267540156080, 8.429910990196965770 ) ) ;
#35862=DIRECTION ( 'NONE',  ( 1.000000000000000078E-15, 0.000000000000000000, 1.000000000000000000 ) ) ;
#35864=CARTESIAN_POINT ( 'NONE',  ( 136.5037707043280477, -38.00325133682356693, 7.150416387934964035 ) ) ;
#35865=VECTOR ( 'NONE', #64092, 1000.000000000000000 ) ;
#35867=CARTESIAN_POINT ( 'NONE',  ( 117.2518684062627727, -39.29770432102194633, 119.6299109901969615 ) ) ;
#35870=AXIS2_PLACEMENT_3D ( 'NONE', #3908, #31603, #81130 ) ;
#35872=ORIENTED_EDGE ( 'NONE', *, *, #3731, .T. ) ;
#35873=ORIENTED_EDGE ( 'NONE', *, *, #43037, .F. ) ;
#35874=CARTESIAN_POINT ( 'NONE',  ( 98.30753410070099108, -41.72887533559486428, 121.7397919284131547 ) ) ;
#35875=DIRECTION ( 'NONE',  ( -1.000000000000000000, -4.163336342344333240E-14, 0.000000000000000000 ) ) ;
#35877=CARTESIAN_POINT ( 'NONE',  ( 107.0664832912739257, -50.36908288530316469, 302.6356252759109680 ) ) ;
#35878=DIRECTION ( 'NONE',  ( 1.000000000000000078E-15, 1.000000000000000083E-30, -1.000000000000000000 ) ) ;
#35879=CARTESIAN_POINT ( 'NONE',  ( 112.1172674779030558, -26.89768192312349271, 15.71086337114896381 ) ) ;
#35880=LINE ( 'NONE', #63597, #75494 ) ;
#35881=EDGE_CURVE ( 'NONE', #37766, #5375, #84474, .T. ) ;
#35885=VECTOR ( 'NONE', #4346, 1000.000000000000000 ) ;
#35889=EDGE_LOOP ( 'NONE', ( #47, #59639, #38898, #56327 ) ) ;
#35890=ORIENTED_EDGE ( 'NONE', *, *, #42995, .T. ) ;
#35893=PLANE ( 'NONE',  #16480 ) ;
#35895=DIRECTION ( 'NONE',  ( 0.000000000000000000, 1.000000000000000000, 0.000000000000000000 ) ) ;
#35896=DIRECTION ( 'NONE',  ( 1.000000000000000078E-15, -1.000000000000000083E-30, -1.000000000000000000 ) ) ;
#35898=CARTESIAN_POINT ( 'NONE',  ( 99.16725398249624845, -41.15831232534042528, 181.1676579233149482 ) ) ;
#35899=CARTESIAN_POINT ( 'NONE',  ( 41.56648329127499153, -32.07844715994070839, 138.9256252759119832 ) ) ;
#35900=CARTESIAN_POINT ( 'NONE',  ( 124.9629318080292251, -56.47944715994101728, 14.92562527591098842 ) ) ;
#35901=CARTESIAN_POINT ( 'NONE',  ( 98.05881815954255387, -31.39384645160161469, 85.90133956162493689 ) ) ;
#35903=CARTESIAN_POINT ( 'NONE',  ( 90.44969454456408187, -16.81243780205710436, 239.5838068554175209 ) ) ;
#35904=VERTEX_POINT ( 'NONE', #25236 ) ;
#35905=CARTESIAN_POINT ( 'NONE',  ( 121.3042370176062548, -43.34581843340460239, 9.425625275910984868 ) ) ;
#35907=CARTESIAN_POINT ( 'NONE',  ( 102.0668449664933064, -27.97061517841426692, 50.48981082298863754 ) ) ;
#35908=ORIENTED_EDGE ( 'NONE', *, *, #1323, .F. ) ;
#35909=PLANE ( 'NONE',  #79909 ) ;
#35911=CIRCLE ( 'NONE', #79440, 5.600000000000000533 ) ;
#35912=CARTESIAN_POINT ( 'NONE',  ( 188.5667039024485518, -48.82844715993430640, 173.2178068554150059 ) ) ;
#35913=ORIENTED_EDGE ( 'NONE', *, *, #76000, .F. ) ;
#35914=CARTESIAN_POINT ( 'NONE',  ( 116.1429853652930149, -29.07104484579759784, 74.38419670448293175 ) ) ;
#35915=CARTESIAN_POINT ( 'NONE',  ( 115.0884034490740362, -30.61698329126820894, 164.3440238799496456 ) ) ;
#35918=CARTESIAN_POINT ( 'NONE',  ( 115.7831076650244881, -41.80230951930585093, 143.4064586084350879 ) ) ;
#35919=ORIENTED_EDGE ( 'NONE', *, *, #12101, .F. ) ;
#35921=CYLINDRICAL_SURFACE ( 'NONE', #28025, 2.750000000000002665 ) ;
#35922=DIRECTION ( 'NONE',  ( 1.639958061481212836E-42, -4.100000000000000342E-29, -1.000000000000000000 ) ) ;
#35923=CARTESIAN_POINT ( 'NONE',  ( 117.8979321085648877, -39.04567734339117635, 104.6708633711489824 ) ) ;
#35924=CIRCLE ( 'NONE', #61985, 2.517500000000005844 ) ;
#35925=DIRECTION ( 'NONE',  ( 1.000000000000000000, 4.299999999999999979E-14, 1.000000000000000078E-15 ) ) ;
#35926=DIRECTION ( 'NONE',  ( 1.000000000000000000, 4.163336342344333240E-14, 0.000000000000000000 ) ) ;
#35931=AXIS2_PLACEMENT_3D ( 'NONE', #20510, #82296, #20053 ) ;
#35933=ADVANCED_FACE ( 'NONE', ( #11626 ), #87480, .F. ) ;
#35934=DIRECTION ( 'NONE',  ( 9.912705577010326536E-16, 1.000000000000000000, 0.000000000000000000 ) ) ;
#35935=EDGE_CURVE ( 'NONE', #28327, #85809, #17014, .T. ) ;
#35936=CARTESIAN_POINT ( 'NONE',  ( 96.47668441219811086, -40.11591174724600251, 127.5727681330529606 ) ) ;
#35937=DIRECTION ( 'NONE',  ( 5.512527431108029424E-15, -1.000000000000000000, 0.000000000000000000 ) ) ;
#35938=ORIENTED_EDGE ( 'NONE', *, *, #82036, .F. ) ;
#35939=AXIS2_PLACEMENT_3D ( 'NONE', #59739, #33840, #87916 ) ;
#35940=EDGE_CURVE ( 'NONE', #57034, #78275, #54708, .T. ) ;
#35941=CARTESIAN_POINT ( 'NONE',  ( 100.8863495415024829, -28.40209871822986543, 31.59657765686296926 ) ) ;
#35943=CARTESIAN_POINT ( 'NONE',  ( 143.0664832912740110, -18.82844715994099971, 284.9256252759119548 ) ) ;
#35944=CARTESIAN_POINT ( 'NONE',  ( 123.6837132603321692, -50.04645651782492166, 249.5838068554164693 ) ) ;
#35945=CARTESIAN_POINT ( 'NONE',  ( 107.0664832912739257, -50.22944715994096043, 315.6356252759111953 ) ) ;
#35946=AXIS2_PLACEMENT_3D ( 'NONE', #29540, #84529, #78158 ) ;
#35947=ADVANCED_FACE ( 'NONE', ( #12070 ), #25687, .F. ) ;
#35948=FACE_OUTER_BOUND ( 'NONE', #33999, .T. ) ;
#35949=CARTESIAN_POINT ( 'NONE',  ( 97.33793063222405806, -34.07070140586845497, 31.11498729261382934 ) ) ;
#35951=CARTESIAN_POINT ( 'NONE',  ( 97.17009264939167679, -31.66255117090383564, 245.9499109901979637 ) ) ;
#35952=ORIENTED_EDGE ( 'NONE', *, *, #80356, .F. ) ;
#35953=VERTEX_POINT ( 'NONE', #66119 ) ;
#35954=CARTESIAN_POINT ( 'NONE',  ( 113.1640969444738971, -43.88191609279036243, 149.5825356868499512 ) ) ;
#35958=CARTESIAN_POINT ( 'NONE',  ( 101.5678104218880549, -29.74196420480149072, 12.03872616303996956 ) ) ;
#35961=LINE ( 'NONE', #62764, #83819 ) ;
#35963=CARTESIAN_POINT ( 'NONE',  ( 107.0664832912739968, -36.72944715994100306, 9.635625275910941312 ) ) ;
#35965=CARTESIAN_POINT ( 'NONE',  ( 110.4916936757735471, -26.90617889774101812, 209.8099109901969541 ) ) ;
#35966=DIRECTION ( 'NONE',  ( -1.000000000000000000, -4.237773401492740281E-14, 0.000000000000000000 ) ) ;
#35967=VERTEX_POINT ( 'NONE', #4806 ) ;
#35968=ORIENTED_EDGE ( 'NONE', *, *, #67811, .T. ) ;
#35970=CARTESIAN_POINT ( 'NONE',  ( 116.8171228669754242, -34.15291832173085140, 89.03145860915122967 ) ) ;
#35972=DIRECTION ( 'NONE',  ( 0.7071067811865046071, 0.7071067811865904273, 7.071067811865039488E-16 ) ) ;
#35974=CIRCLE ( 'NONE', #86758, 2.117000000000007987 ) ;
#35976=CARTESIAN_POINT ( 'NONE',  ( 110.8778723966665751, -46.37372517157803742, 18.88800622829095488 ) ) ;
#35977=CYLINDRICAL_SURFACE ( 'NONE', #13700, 0.4999999999999994449 ) ;
#35978=VERTEX_POINT ( 'NONE', #47005 ) ;
#35979=CARTESIAN_POINT ( 'NONE',  ( 104.6388127410885005, -47.56014030727299513, 23.38895860924494841 ) ) ;
#35982=CARTESIAN_POINT ( 'NONE',  ( 105.6320445689042486, -47.05559920284586184, 257.4670538473393435 ) ) ;
#35983=ORIENTED_EDGE ( 'NONE', *, *, #39717, .T. ) ;
#35984=FACE_OUTER_BOUND ( 'NONE', #29, .T. ) ;
#35986=FACE_OUTER_BOUND ( 'NONE', #3884, .T. ) ;
#35987=CARTESIAN_POINT ( 'NONE',  ( 115.6288848908637732, -37.98889302744424867, 71.54047132197199232 ) ) ;
#35988=CARTESIAN_POINT ( 'NONE',  ( 96.65238424151439744, -35.53540495314400260, 202.2356252759109623 ) ) ;
#35989=DIRECTION ( 'NONE',  ( 1.000000000000000078E-15, 0.000000000000000000, 1.000000000000000000 ) ) ;
#35990=ORIENTED_EDGE ( 'NONE', *, *, #50746, .F. ) ;
#35991=VECTOR ( 'NONE', #74891, 1000.000000000000000 ) ;
#35993=CARTESIAN_POINT ( 'NONE',  ( 182.0374245136174522, -23.42844715993458848, 193.9678068554150343 ) ) ;
#35995=EDGE_LOOP ( 'NONE', ( #60367, #21296, #51004, #81914 ) ) ;
#36001=CARTESIAN_POINT ( 'NONE',  ( 107.9191913915661871, -25.30201086838711788, 321.3423205873733082 ) ) ;
#36002=CARTESIAN_POINT ( 'NONE',  ( 104.7294611837924094, -27.30559681290521112, 89.69241982807696445 ) ) ;
#36003=CARTESIAN_POINT ( 'NONE',  ( 111.7836659179374408, -46.75466717335095268, 287.9146728949587555 ) ) ;
#36006=CARTESIAN_POINT ( 'NONE',  ( 138.8167039024479834, -57.40094715994099772, 33.40080685541480676 ) ) ;
#36008=EDGE_CURVE ( 'NONE', #49936, #72873, #52468, .T. ) ;
#36010=CARTESIAN_POINT ( 'NONE',  ( 188.5667039024479834, -58.35344715994099829, 175.9678068554150059 ) ) ;
#36015=CARTESIAN_POINT ( 'NONE',  ( 113.5587197313314505, -28.64306037466250743, 119.5261014663879564 ) ) ;
#36016=EDGE_CURVE ( 'NONE', #29733, #66334, #38740, .T. ) ;
#36017=CARTESIAN_POINT ( 'NONE',  ( 95.43890296797121664, -34.19406290021405681, 106.1556252759109640 ) ) ;
#36018=CARTESIAN_POINT ( 'NONE',  ( 111.4991187713021219, -26.55290587224241960, 284.7375300378155316 ) ) ;
#36020=CARTESIAN_POINT ( 'NONE',  ( 113.7993967570077700, -26.97709554098909024, 239.5956252759109759 ) ) ;
#36024=CARTESIAN_POINT ( 'NONE',  ( 108.0925365931996680, -46.37966058722595619, 277.6356252759107406 ) ) ;
#36025=CARTESIAN_POINT ( 'NONE',  ( 63.06670390244799052, -40.32844715994017548, 249.9678068554150343 ) ) ;
#36026=CARTESIAN_POINT ( 'NONE',  ( 106.3547972878507579, -25.29203239850954787, 320.5499541688668614 ) ) ;
#36028=CARTESIAN_POINT ( 'NONE',  ( 131.4052890608956545, -37.42303004212691775, 6.877070700249918289 ) ) ;
#36029=AXIS2_PLACEMENT_3D ( 'NONE', #63147, #85854, #50860 ) ;
#36031=DIRECTION ( 'NONE',  ( -0.000000000000000000, -0.000000000000000000, 1.000000000000000000 ) ) ;
#36033=LINE ( 'NONE', #55999, #70406 ) ;
#36034=ORIENTED_EDGE ( 'NONE', *, *, #45880, .F. ) ;
#36035=PLANE ( 'NONE',  #36526 ) ;
#36036=CARTESIAN_POINT ( 'NONE',  ( 112.4231589263966526, -46.42488254349225940, 252.9661014663871015 ) ) ;
#36037=CARTESIAN_POINT ( 'NONE',  ( 116.6607991934174322, -40.80763178269008762, 164.5070538473399608 ) ) ;
#36038=CARTESIAN_POINT ( 'NONE',  ( 114.1052656684236979, -46.29384956339717405, 29.08133956162595268 ) ) ;
#36041=CARTESIAN_POINT ( 'NONE',  ( 172.5667039024480687, -36.32844715993499563, 129.9678068554150059 ) ) ;
#36043=CARTESIAN_POINT ( 'NONE',  ( 99.50482035239026857, -43.30589195511487333, 137.8960310260671633 ) ) ;
#36044=ORIENTED_EDGE ( 'NONE', *, *, #24812, .T. ) ;
#36046=CARTESIAN_POINT ( 'NONE',  ( 172.5664832912729878, -27.82844715994070484, 138.9256252759119832 ) ) ;
#36048=EDGE_CURVE ( 'NONE', #60674, #54334, #47459, .T. ) ;
#36049=CARTESIAN_POINT ( 'NONE',  ( 112.3908963168805712, -43.44530362507355647, 167.5324198280769963 ) ) ;
#36050=FACE_OUTER_BOUND ( 'NONE', #40584, .T. ) ;
#36051=ORIENTED_EDGE ( 'NONE', *, *, #15576, .F. ) ;
#36054=CARTESIAN_POINT ( 'NONE',  ( 95.33621695423336462, -38.27597901479983733, 147.4299109901969871 ) ) ;
#36055=CARTESIAN_POINT ( 'NONE',  ( 135.3756687995053483, -12.91806617559082504, 361.9756252759100335 ) ) ;
#36056=DIRECTION ( 'NONE',  ( 0.000000000000000000, 0.000000000000000000, 1.000000000000000000 ) ) ;
#36057=CARTESIAN_POINT ( 'NONE',  ( 104.5015244207571357, -26.97598608851367530, 86.28151539219055621 ) ) ;
#36059=CARTESIAN_POINT ( 'NONE',  ( 61.56670390244730839, -23.42844715994043980, 249.9678068554150343 ) ) ;
#36061=DIRECTION ( 'NONE',  ( 0.000000000000000000, 1.000000000000000000, 0.000000000000000000 ) ) ;
#36062=CARTESIAN_POINT ( 'NONE',  ( 116.4859054502389881, -39.36344060769046393, 98.60991099019695127 ) ) ;
#36063=VERTEX_POINT ( 'NONE', #7045 ) ;
#36064=ORIENTED_EDGE ( 'NONE', *, *, #84263, .T. ) ;
#36065=VERTEX_POINT ( 'NONE', #27924 ) ;
#36066=AXIS2_PLACEMENT_3D ( 'NONE', #70926, #8699, #36400 ) ;
#36067=CARTESIAN_POINT ( 'NONE',  ( 99.03873739112161445, -32.90617299384241790, 72.40444044875393104 ) ) ;
#36068=AXIS2_PLACEMENT_3D ( 'NONE', #49130, #70503, #89155 ) ;
#36070=CARTESIAN_POINT ( 'NONE',  ( 97.31640351007386869, -35.61153895465465524, 202.2356252759109623 ) ) ;
#36072=CARTESIAN_POINT ( 'NONE',  ( 99.09600433706673073, -30.55004372760710041, 55.80090408730614371 ) ) ;
#36073=CARTESIAN_POINT ( 'NONE',  ( 105.7995095144211462, -26.72403595622594707, 111.1776164158398643 ) ) ;
#36074=EDGE_CURVE ( 'NONE', #62004, #65745, #76078, .T. ) ;
#36075=DIRECTION ( 'NONE',  ( -0.9254794337955620787, -0.3787978585227822492, 0.000000000000000000 ) ) ;
#36076=CIRCLE ( 'NONE', #75244, 1.000000000000000888 ) ;
#36077=DIRECTION ( 'NONE',  ( -1.000000000000000000, -4.299999999999999979E-14, -1.000000000000000078E-15 ) ) ;
#36079=CARTESIAN_POINT ( 'NONE',  ( 108.2741602056595411, -26.36093993100598354, 129.9841967044819739 ) ) ;
#36080=VERTEX_POINT ( 'NONE', #34740 ) ;
#36081=ORIENTED_EDGE ( 'NONE', *, *, #40872, .T. ) ;
#36083=AXIS2_PLACEMENT_3D ( 'NONE', #53684, #68694, #39627 ) ;
#36087=CARTESIAN_POINT ( 'NONE',  ( 22.49563609058249725, -67.87844715994100397, 307.9888746672805269 ) ) ;
#36089=CARTESIAN_POINT ( 'NONE',  ( 115.4521610479674081, -32.75750308622325946, 211.9966617981629611 ) ) ;
#36092=ORIENTED_EDGE ( 'NONE', *, *, #6909, .T. ) ;
#36093=ORIENTED_EDGE ( 'NONE', *, *, #69440, .F. ) ;
#36098=VERTEX_POINT ( 'NONE', #69722 ) ;
#36099=CARTESIAN_POINT ( 'NONE',  ( 163.0959832912772924, -23.42844715993538074, 237.4678068554150059 ) ) ;
#36101=CARTESIAN_POINT ( 'NONE',  ( 109.7775653660112596, -28.26114369521987868, 231.2615833058969770 ) ) ;
#36102=CARTESIAN_POINT ( 'NONE',  ( 98.30753348724731211, -41.72887427465273191, 271.7397918317862491 ) ) ;
#36103=ORIENTED_EDGE ( 'NONE', *, *, #87758, .F. ) ;
#36105=CARTESIAN_POINT ( 'NONE',  ( 101.7541625622157540, -42.82727082765900661, 9.635625275910939536 ) ) ;
#36107=DIRECTION ( 'NONE',  ( 1.027984282060330356E-15, 1.000000000000000000, 0.000000000000000000 ) ) ;
#36108=VERTEX_POINT ( 'NONE', #88830 ) ;
#36112=VERTEX_POINT ( 'NONE', #666 ) ;
#36113=EDGE_CURVE ( 'NONE', #51823, #8449, #1057, .T. ) ;
#36114=CARTESIAN_POINT ( 'NONE',  ( 115.2289877667042930, -36.78642703073501252, 261.6395189410197872 ) ) ;
#36115=CARTESIAN_POINT ( 'NONE',  ( 117.0383059485392607, -33.61350157978694142, 174.0670538473389399 ) ) ;
#36116=CARTESIAN_POINT ( 'NONE',  ( 111.0741232671659304, -25.60348521778444209, 99.80133956162498521 ) ) ;
#36117=CARTESIAN_POINT ( 'NONE',  ( 37.03715912545425937, -48.62818131006122258, 313.9678068554150059 ) ) ;
#36118=LINE ( 'NONE', #84292, #39461 ) ;
#36119=CARTESIAN_POINT ( 'NONE',  ( 104.3244243092125032, -26.02173531178284804, 241.2880062282919482 ) ) ;
#36121=DIRECTION ( 'NONE',  ( -1.000000000000000000, 0.000000000000000000, 0.000000000000000000 ) ) ;
#36125=VECTOR ( 'NONE', #53642, 1000.000000000000000 ) ;
#36127=VECTOR ( 'NONE', #54901, 1000.000000000000000 ) ;
#36128=AXIS2_PLACEMENT_3D ( 'NONE', #83581, #21345, #62222 ) ;
#36129=EDGE_CURVE ( 'NONE', #18171, #36809, #70709, .T. ) ;
#36130=CARTESIAN_POINT ( 'NONE',  ( 103.5274535807004384, -26.83869072616077744, 190.3499109901969746 ) ) ;
#36131=ORIENTED_EDGE ( 'NONE', *, *, #4895, .F. ) ;
#36132=CARTESIAN_POINT ( 'NONE',  ( 109.2014631304945027, -26.52509060526352869, 139.9127681330539872 ) ) ;
#36135=CARTESIAN_POINT ( 'NONE',  ( 182.2738106836200132, -23.19206098993950604, -5.074374724088000832 ) ) ;
#36136=CARTESIAN_POINT ( 'NONE',  ( 74.38348329127296665, -71.52944715994141234, 361.9756252759109998 ) ) ;
#36138=CARTESIAN_POINT ( 'NONE',  ( 100.8614382317055345, -45.12360235833653377, 253.0699109901968882 ) ) ;
#36141=DIRECTION ( 'NONE',  ( -1.000000000000000078E-15, 1.000000000000000000, 0.000000000000000000 ) ) ;
#36142=AXIS2_PLACEMENT_3D ( 'NONE', #81808, #13206, #20020 ) ;
#36143=CARTESIAN_POINT ( 'NONE',  ( 177.8371591254545194, -47.82818131005477369, 180.4678068554150343 ) ) ;
#36147=CARTESIAN_POINT ( 'NONE',  ( 100.1093887754828984, -44.55284168805902567, 266.9984824187678782 ) ) ;
#36149=CARTESIAN_POINT ( 'NONE',  ( 134.0664832912740110, -36.72944715994100306, -5.074374724089001809 ) ) ;
#36150=CARTESIAN_POINT ( 'NONE',  ( 117.0544076763083297, -30.30483159375883062, 144.2813395616249750 ) ) ;
#36151=CARTESIAN_POINT ( 'NONE',  ( 96.17756896972203151, -38.62826926382330583, 42.45181575210199298 ) ) ;
#36152=CARTESIAN_POINT ( 'NONE',  ( 107.6569575903311318, -47.81316668278100224, 193.6308633711489620 ) ) ;
#36155=DIRECTION ( 'NONE',  ( 0.000000000000000000, 1.000000000000000000, 0.000000000000000000 ) ) ;
#36158=LINE ( 'NONE', #15723, #8946 ) ;
#36161=FACE_OUTER_BOUND ( 'NONE', #6157, .T. ) ;
#36163=VERTEX_POINT ( 'NONE', #34287 ) ;
#36165=AXIS2_PLACEMENT_3D ( 'NONE', #58128, #36353, #23631 ) ;
#36169=CARTESIAN_POINT ( 'NONE',  ( 99.31004196827758790, -43.71529311364903947, 52.90991099019698396 ) ) ;
#36170=DIRECTION ( 'NONE',  ( 0.000000000000000000, 0.000000000000000000, 1.000000000000000000 ) ) ;
#36172=LINE ( 'NONE', #57044, #60227 ) ;
#36173=CARTESIAN_POINT ( 'NONE',  ( 104.5521338839504608, -48.36083399734661725, 178.4070538473399665 ) ) ;
#36175=CARTESIAN_POINT ( 'NONE',  ( 114.5003125304781122, -32.48770244606883040, 288.6609912566482308 ) ) ;
#36177=AXIS2_PLACEMENT_3D ( 'NONE', #35619, #41974, #50133 ) ;
#36178=EDGE_LOOP ( 'NONE', ( #51229, #33222, #62000, #33702 ) ) ;
#36181=CARTESIAN_POINT ( 'NONE',  ( 131.0667039024480687, -58.72944715994092491, 231.5838068554170093 ) ) ;
#36182=CARTESIAN_POINT ( 'NONE',  ( 181.8884939055940038, -32.11662333284530746, -5.074374724088000832 ) ) ;
#36183=CARTESIAN_POINT ( 'NONE',  ( 100.9544197307436093, -28.70722375064775278, 161.5939840054776653 ) ) ;
#36185=DIRECTION ( 'NONE',  ( 0.000000000000000000, -1.000000000000000000, 0.000000000000000000 ) ) ;
#36187=ADVANCED_FACE ( 'NONE', ( #63347 ), #70616, .T. ) ;
#36190=EDGE_CURVE ( 'NONE', #7721, #2591, #23383, .T. ) ;
#36191=CARTESIAN_POINT ( 'NONE',  ( 114.8031991714177451, -43.68443766454706889, 38.24419670448192221 ) ) ;
#36193=VECTOR ( 'NONE', #21862, 1000.000000000000000 ) ;
#36195=CARTESIAN_POINT ( 'NONE',  ( 114.1400169897070924, -40.01656155057797548, 9.425625275910977763 ) ) ;
#36196=CARTESIAN_POINT ( 'NONE',  ( 100.1260263088618103, -41.89964850235647020, 109.6661856076859607 ) ) ;
#36197=CIRCLE ( 'NONE', #52107, 2.749999999999974687 ) ;
#36199=FACE_OUTER_BOUND ( 'NONE', #16176, .T. ) ;
#36200=LINE ( 'NONE', #29841, #86590 ) ;
#36201=ORIENTED_EDGE ( 'NONE', *, *, #23070, .T. ) ;
#36202=ORIENTED_EDGE ( 'NONE', *, *, #12697, .T. ) ;
#36203=CARTESIAN_POINT ( 'NONE',  ( 98.15098810655345574, -41.26163425357335512, 136.7008391909870113 ) ) ;
#36204=ORIENTED_EDGE ( 'NONE', *, *, #10565, .T. ) ;
#36205=ORIENTED_EDGE ( 'NONE', *, *, #15570, .T. ) ;
#36207=CARTESIAN_POINT ( 'NONE',  ( 103.0939887460847189, -28.21499987170311385, 131.8434880678019567 ) ) ;
#36209=AXIS2_PLACEMENT_3D ( 'NONE', #33417, #30853, #58110 ) ;
#36210=CARTESIAN_POINT ( 'NONE',  ( 96.00057345886969529, -37.20991081664785582, 112.3489586092449599 ) ) ;
#36212=CARTESIAN_POINT ( 'NONE',  ( 112.0733969452682004, -45.39207061711373825, 17.99352580270544522 ) ) ;
#36213=ORIENTED_EDGE ( 'NONE', *, *, #4599, .F. ) ;
#36214=CIRCLE ( 'NONE', #43455, 2.517500000000000071 ) ;
#36217=EDGE_CURVE ( 'NONE', #2787, #66733, #64693, .T. ) ;
#36219=CARTESIAN_POINT ( 'NONE',  ( 96.69274360309970007, -38.23738870492909570, 66.44133956162495735 ) ) ;
#36220=ORIENTED_EDGE ( 'NONE', *, *, #79231, .F. ) ;
#36221=CARTESIAN_POINT ( 'NONE',  ( 105.1675567143510079, -46.98732170830152910, 12.42991099019596923 ) ) ;
#36222=CARTESIAN_POINT ( 'NONE',  ( 97.36185206511996171, -42.06848625969246314, 172.7146728949589942 ) ) ;
#36224=CYLINDRICAL_SURFACE ( 'NONE', #38768, 4.750000000000004441 ) ;
#36225=CARTESIAN_POINT ( 'NONE',  ( 108.5897967589408495, -47.07840195076833112, 138.6927681330539883 ) ) ;
#36227=ORIENTED_EDGE ( 'NONE', *, *, #54677, .T. ) ;
#36228=CARTESIAN_POINT ( 'NONE',  ( 168.5667039024483529, -48.82844715993517326, 300.4678068554149490 ) ) ;
#36231=CARTESIAN_POINT ( 'NONE',  ( 97.92324688886398576, -40.78073627936089451, 132.6587986620884863 ) ) ;
#36232=VERTEX_POINT ( 'NONE', #56971 ) ;
#36233=CIRCLE ( 'NONE', #41986, 29.00000000000000000 ) ;
#36234=ORIENTED_EDGE ( 'NONE', *, *, #61861, .F. ) ;
#36236=EDGE_CURVE ( 'NONE', #70138, #51366, #16546, .T. ) ;
#36237=DIRECTION ( 'NONE',  ( 0.000000000000000000, 0.000000000000000000, -1.000000000000000000 ) ) ;
#36238=CARTESIAN_POINT ( 'NONE',  ( 105.3203727031265373, -26.45150370518939198, 15.20991099019697401 ) ) ;
#36240=DIRECTION ( 'NONE',  ( -1.000000000000000000, -4.163336342344333240E-14, 0.000000000000000000 ) ) ;
#36242=CARTESIAN_POINT ( 'NONE',  ( 99.61812512063040970, -43.94476044465314857, 41.95086337115000674 ) ) ;
#36243=CARTESIAN_POINT ( 'NONE',  ( 34.96670390244699433, -28.27351298637401200, -5.074374724088000832 ) ) ;
#36244=CARTESIAN_POINT ( 'NONE',  ( 97.85535806214043930, -31.89376338832687097, 131.9413395616259947 ) ) ;
#36247=ORIENTED_EDGE ( 'NONE', *, *, #4165, .T. ) ;
#36249=AXIS2_PLACEMENT_3D ( 'NONE', #13284, #67794, #73715 ) ;
#36250=DIRECTION ( 'NONE',  ( -0.4214249218767880945, -0.9068632946707806397, -4.214249218767889924E-16 ) ) ;
#36252=ORIENTED_EDGE ( 'NONE', *, *, #35839, .F. ) ;
#36254=ADVANCED_FACE ( 'NONE', ( #44224 ), #71965, .F. ) ;
#36255=CARTESIAN_POINT ( 'NONE',  ( 87.06648329127402519, -54.72944906728955061, 14.92562527591094934 ) ) ;
#36256=CARTESIAN_POINT ( 'NONE',  ( 102.6649408499558689, -27.23033719207987602, 180.4213395616249898 ) ) ;
#36258=LINE ( 'NONE', #21284, #69789 ) ;
#36259=CARTESIAN_POINT ( 'NONE',  ( 118.8146046005060015, -38.46262239392275717, 219.7099109901969882 ) ) ;
#36260=CARTESIAN_POINT ( 'NONE',  ( 113.4418579183357849, -27.64362872000679516, 80.57753003781597556 ) ) ;
#36263=DIRECTION ( 'NONE',  ( 0.7071067811869841124, -0.7071067811861110330, 0.000000000000000000 ) ) ;
#36264=ORIENTED_EDGE ( 'NONE', *, *, #40858, .T. ) ;
#36268=VERTEX_POINT ( 'NONE', #29286 ) ;
#36271=DIRECTION ( 'NONE',  ( 1.000000000000000000, -5.337610695313248426E-16, 0.000000000000000000 ) ) ;
#36272=CARTESIAN_POINT ( 'NONE',  ( 112.4893506266177070, -46.36098340020668473, 253.9965776568634510 ) ) ;
#36273=CARTESIAN_POINT ( 'NONE',  ( 34.96670390244738513, -26.71338133339315490, 313.9678068554150059 ) ) ;
#36274=CARTESIAN_POINT ( 'NONE',  ( 136.4174407532304940, -17.29868422071827183, 2.608896314067475242 ) ) ;
#36277=VECTOR ( 'NONE', #78614, 1000.000000000000000 ) ;
#36281=CARTESIAN_POINT ( 'NONE',  ( 118.0989925035467252, -37.71898322177068508, 33.74324432352998571 ) ) ;
#36282=ORIENTED_EDGE ( 'NONE', *, *, #58108, .F. ) ;
#36283=VERTEX_POINT ( 'NONE', #1584 ) ;
#36284=ORIENTED_EDGE ( 'NONE', *, *, #41980, .F. ) ;
#36285=LINE ( 'NONE', #22671, #73210 ) ;
#36287=CARTESIAN_POINT ( 'NONE',  ( 115.4101910119109533, -30.57141770992062035, 255.3203871806724123 ) ) ;
#36288=AXIS2_PLACEMENT_3D ( 'NONE', #73321, #72444, #37918 ) ;
#36289=DIRECTION ( 'NONE',  ( 1.000000000000000000, 4.299999999999999979E-14, 1.000000000000000078E-15 ) ) ;
#36290=EDGE_CURVE ( 'NONE', #78258, #56977, #88080, .T. ) ;
#36291=CARTESIAN_POINT ( 'NONE',  ( 96.47668441219811086, -40.11591174724600251, 127.5727681330529606 ) ) ;
#36292=ADVANCED_FACE ( 'NONE', ( #2475 ), #30617, .F. ) ;
#36293=EDGE_CURVE ( 'NONE', #86673, #57650, #23816, .T. ) ;
#36294=FACE_OUTER_BOUND ( 'NONE', #43085, .T. ) ;
#36297=CARTESIAN_POINT ( 'NONE',  ( 77.80861903141534697, -35.15582774928859067, 2.518078172607126408 ) ) ;
#36298=EDGE_CURVE ( 'NONE', #4135, #22294, #60490, .T. ) ;
#36300=ORIENTED_EDGE ( 'NONE', *, *, #21734, .F. ) ;
#36301=AXIS2_PLACEMENT_3D ( 'NONE', #82239, #437, #54475 ) ;
#36303=CARTESIAN_POINT ( 'NONE',  ( 101.0802515965118573, -30.15484820110618358, 282.0958690201827039 ) ) ;
#36304=DIRECTION ( 'NONE',  ( 0.000000000000000000, 0.000000000000000000, -1.000000000000000000 ) ) ;
#36305=CARTESIAN_POINT ( 'NONE',  ( 108.4174892614935004, -26.73503592907457005, 84.96895860849961934 ) ) ;
#36306=DIRECTION ( 'NONE',  ( 0.000000000000000000, 1.000000000000000000, 0.000000000000000000 ) ) ;
#36307=EDGE_LOOP ( 'NONE', ( #45398, #72943, #24001 ) ) ;
#36308=AXIS2_PLACEMENT_3D ( 'NONE', #60750, #81234, #59847 ) ;
#36309=CARTESIAN_POINT ( 'NONE',  ( 19.56648329127303043, -71.37844715994266664, 342.9256252759109884 ) ) ;
#36311=EDGE_LOOP ( 'NONE', ( #34892, #43070 ) ) ;
#36312=CARTESIAN_POINT ( 'NONE',  ( 104.7595363604009435, -46.89630637601933927, 72.39848241876795498 ) ) ;
#36313=ORIENTED_EDGE ( 'NONE', *, *, #69379, .F. ) ;
#36314=CARTESIAN_POINT ( 'NONE',  ( 102.5950791370611768, -45.34791940167762192, 16.61813411379198158 ) ) ;
#36316=LINE ( 'NONE', #76751, #25619 ) ;
#36317=CARTESIAN_POINT ( 'NONE',  ( 104.7173522264389334, -47.59653351925024367, 182.4070538473399665 ) ) ;
#36318=DIRECTION ( 'NONE',  ( 0.000000000000000000, 0.000000000000000000, -1.000000000000000000 ) ) ;
#36319=DIRECTION ( 'NONE',  ( -2.999999999999999839E-15, 1.000000000000000000, -2.999999999999999900E-30 ) ) ;
#36322=CARTESIAN_POINT ( 'NONE',  ( 116.6217178149748008, -42.37701578139068204, 279.4137205140061724 ) ) ;
#36326=DIRECTION ( 'NONE',  ( -1.000000000000000078E-15, 0.000000000000000000, -1.000000000000000000 ) ) ;
#36327=ORIENTED_EDGE ( 'NONE', *, *, #32450, .F. ) ;
#36328=CARTESIAN_POINT ( 'NONE',  ( 97.70743813507087339, -42.69650533217181021, 137.7661014663869992 ) ) ;
#36330=ORIENTED_EDGE ( 'NONE', *, *, #7082, .T. ) ;
#36331=ORIENTED_EDGE ( 'NONE', *, *, #48971, .F. ) ;
#36332=EDGE_CURVE ( 'NONE', #22610, #24378, #32942, .T. ) ;
#36333=ORIENTED_EDGE ( 'NONE', *, *, #3684, .F. ) ;
#36334=CIRCLE ( 'NONE', #53729, 0.5000000000000004441 ) ;
#36336=CARTESIAN_POINT ( 'NONE',  ( 97.31583813429813290, -39.30595438711576151, 267.5314568493160436 ) ) ;
#36337=DIRECTION ( 'NONE',  ( -1.175184669632759901E-16, 1.000000000000000000, 2.000000000000003705E-15 ) ) ;
#36338=DIRECTION ( 'NONE',  ( 1.000000000000000000, 0.000000000000000000, 0.000000000000000000 ) ) ;
#36339=DIRECTION ( 'NONE',  ( -1.000000000000000000, -4.299999999999999979E-14, -1.000000000000000078E-15 ) ) ;
#36340=CARTESIAN_POINT ( 'NONE',  ( 113.7700232194324883, -29.06831460768450626, 285.5032443235299979 ) ) ;
#36341=LINE ( 'NONE', #57666, #72585 ) ;
#36342=EDGE_LOOP ( 'NONE', ( #18800, #76051, #44238, #14331 ) ) ;
#36345=DIRECTION ( 'NONE',  ( 0.7071067811566161820, 0.7071067812164789634, 0.000000000000000000 ) ) ;
#36348=CARTESIAN_POINT ( 'NONE',  ( 80.81785596311139841, -21.40256188477534138, 1.690787648075373850 ) ) ;
#36349=EDGE_CURVE ( 'NONE', #31634, #61394, #7935, .T. ) ;
#36352=ADVANCED_FACE ( 'NONE', ( #22036 ), #57452, .F. ) ;
#36353=DIRECTION ( 'NONE',  ( -4.237773401492740281E-14, 1.000000000000000000, 0.000000000000000000 ) ) ;
#36356=CARTESIAN_POINT ( 'NONE',  ( 113.9432952986174854, -30.83689873488770061, 228.8248007804579629 ) ) ;
#36357=DIRECTION ( 'NONE',  ( 0.000000000000000000, 0.000000000000000000, -1.000000000000000000 ) ) ;
#36359=CARTESIAN_POINT ( 'NONE',  ( 113.5334051825838202, -28.49624685289517245, 79.54705384733995288 ) ) ;
#36361=DIRECTION ( 'NONE',  ( 0.000000000000000000, 0.000000000000000000, 1.000000000000000000 ) ) ;
#36362=ORIENTED_EDGE ( 'NONE', *, *, #34513, .F. ) ;
#36363=ADVANCED_FACE ( 'NONE', ( #31945 ), #3363, .T. ) ;
#36365=CARTESIAN_POINT ( 'NONE',  ( 97.81219807385008380, -40.51719912245609123, 147.6362401243850115 ) ) ;
#36366=DIRECTION ( 'NONE',  ( -4.237773401492740281E-14, 1.000000000000000000, 0.000000000000000000 ) ) ;
#36368=EDGE_CURVE ( 'NONE', #65418, #78803, #52358, .T. ) ;
#36370=DIRECTION ( 'NONE',  ( 9.351236661543306751E-17, -3.725950533538267725E-29, -1.000000000000000000 ) ) ;
#36371=ORIENTED_EDGE ( 'NONE', *, *, #56729, .F. ) ;
#36373=CARTESIAN_POINT ( 'NONE',  ( 104.4091780781909335, -46.45840484912275059, 273.3644384837980965 ) ) ;
#36374=VECTOR ( 'NONE', #33055, 1000.000000000000000 ) ;
#36376=DIRECTION ( 'NONE',  ( 0.7071067811865473507, 0.7071067811865476838, 0.000000000000000000 ) ) ;
#36377=EDGE_CURVE ( 'NONE', #20562, #60619, #53255, .T. ) ;
#36378=ORIENTED_EDGE ( 'NONE', *, *, #11997, .F. ) ;
#36379=CARTESIAN_POINT ( 'NONE',  ( 97.60225484043094468, -32.22203741027808377, 75.97276813305397525 ) ) ;
#36382=CARTESIAN_POINT ( 'NONE',  ( 193.0371591254575208, -23.42818131005411075, 117.4678068554150627 ) ) ;
#36386=EDGE_CURVE ( 'NONE', #3581, #32750, #72409, .T. ) ;
#36387=CARTESIAN_POINT ( 'NONE',  ( 108.5609052613744012, -26.81332519519535040, 120.9559658802212567 ) ) ;
#36388=CARTESIAN_POINT ( 'NONE',  ( 149.4409906032288404, -0.9156555935619370423, 361.9756252759100335 ) ) ;
#36390=EDGE_CURVE ( 'NONE', #54558, #35318, #4699, .T. ) ;
#36392=AXIS2_PLACEMENT_3D ( 'NONE', #71370, #23232, #9136 ) ;
#36394=CARTESIAN_POINT ( 'NONE',  ( 101.4892552882362793, -27.89588691190665060, 106.5241967044819944 ) ) ;
#36396=DIRECTION ( 'NONE',  ( 0.000000000000000000, 0.000000000000000000, -1.000000000000000000 ) ) ;
#36397=DIRECTION ( 'NONE',  ( -2.999999999999999839E-15, 1.000000000000000000, -2.999999999999999900E-30 ) ) ;
#36398=AXIS2_PLACEMENT_3D ( 'NONE', #45826, #10005, #60361 ) ;
#36400=DIRECTION ( 'NONE',  ( -1.000000000000000078E-15, 1.000000000000000083E-30, 1.000000000000000000 ) ) ;
#36401=CARTESIAN_POINT ( 'NONE',  ( 117.1372161989436904, -34.25576096370540569, 160.0061014663869798 ) ) ;
#36405=ADVANCED_FACE ( 'NONE', ( #66459 ), #86488, .F. ) ;
#36406=CARTESIAN_POINT ( 'NONE',  ( 99.56037394151449860, -43.88466257697679396, 32.92038718067297509 ) ) ;
#36408=CARTESIAN_POINT ( 'NONE',  ( 80.06648329127401098, -41.22944715994105280, 4.925625275910944012 ) ) ;
#36410=ADVANCED_FACE ( 'NONE', ( #25133 ), #18770, .T. ) ;
#36411=CYLINDRICAL_SURFACE ( 'NONE', #89191, 2.517500000000005844 ) ;
#36412=AXIS2_PLACEMENT_3D ( 'NONE', #36701, #69872, #37145 ) ;
#36413=EDGE_CURVE ( 'NONE', #62685, #76826, #17435, .T. ) ;
#36414=PLANE ( 'NONE',  #25491 ) ;
#36416=CARTESIAN_POINT ( 'NONE',  ( 110.5849939505706772, -26.97450646431652643, 249.7889586092449576 ) ) ;
#36417=ORIENTED_EDGE ( 'NONE', *, *, #22350, .F. ) ;
#36418=ORIENTED_EDGE ( 'NONE', *, *, #23450, .F. ) ;
#36419=CARTESIAN_POINT ( 'NONE',  ( 102.8032110495234264, -45.10208326393837552, 168.6453928297069353 ) ) ;
#36421=CARTESIAN_POINT ( 'NONE',  ( 98.44769980935930676, -38.78975051229773641, 52.94444044875496047 ) ) ;
#36423=VECTOR ( 'NONE', #6066, 1000.000000000000000 ) ;
#36424=DIRECTION ( 'NONE',  ( 0.000000000000000000, 0.000000000000000000, 1.000000000000000000 ) ) ;
#36426=VECTOR ( 'NONE', #76824, 1000.000000000000000 ) ;
#36427=LINE ( 'NONE', #84585, #76887 ) ;
#36428=CYLINDRICAL_SURFACE ( 'NONE', #11084, 0.4999999999999982236 ) ;
#36429=CARTESIAN_POINT ( 'NONE',  ( 103.9458437887065827, -26.80522050874817808, 250.3184824187678714 ) ) ;
#36430=CARTESIAN_POINT ( 'NONE',  ( 97.12563415398577149, -37.99750651866536089, 171.4272510260306603 ) ) ;
#36431=ORIENTED_EDGE ( 'NONE', *, *, #4992, .F. ) ;
#36432=ORIENTED_EDGE ( 'NONE', *, *, #58489, .T. ) ;
#36435=DIRECTION ( 'NONE',  ( -1.000000000000000078E-15, 1.000000000000000083E-30, 1.000000000000000000 ) ) ;
#36437=CIRCLE ( 'NONE', #81380, 2.517500000000005844 ) ;
#36438=CARTESIAN_POINT ( 'NONE',  ( 97.46604185887804306, -38.76544784714101155, 27.49276813305395706 ) ) ;
#36440=VERTEX_POINT ( 'NONE', #45116 ) ;
#36442=CARTESIAN_POINT ( 'NONE',  ( 110.8100519147795922, -46.50588177123592715, 58.86705384733998159 ) ) ;
#36443=CARTESIAN_POINT ( 'NONE',  ( 21.03689327557613709, -23.42844715994197813, 193.9678068554150627 ) ) ;
#36444=CARTESIAN_POINT ( 'NONE',  ( 117.4908834113230682, -35.85893649831510999, 253.8927681330538348 ) ) ;
#36445=EDGE_LOOP ( 'NONE', ( #43343, #4169, #42708, #15098 ) ) ;
#36447=LINE ( 'NONE', #44572, #47134 ) ;
#36448=DIRECTION ( 'NONE',  ( 1.000000000000000078E-15, -1.000000000000000083E-30, -1.000000000000000000 ) ) ;
#36449=CARTESIAN_POINT ( 'NONE',  ( 111.5571307036148312, -44.84917726517733882, 100.7966617981629582 ) ) ;
#36450=CARTESIAN_POINT ( 'NONE',  ( 99.27233432241882838, -29.77326281039884037, 186.7470538473389752 ) ) ;
#36451=DIRECTION ( 'NONE',  ( 1.000000000000000000, 0.000000000000000000, -0.000000000000000000 ) ) ;
#36453=FACE_OUTER_BOUND ( 'NONE', #19586, .T. ) ;
#36454=EDGE_LOOP ( 'NONE', ( #29648, #7882, #47193, #56181 ) ) ;
#36457=CYLINDRICAL_SURFACE ( 'NONE', #87960, 1.000000000000000888 ) ;
#36458=VERTEX_POINT ( 'NONE', #10606 ) ;
#36462=EDGE_CURVE ( 'NONE', #17437, #28847, #70118, .T. ) ;
#36463=CARTESIAN_POINT ( 'NONE',  ( 108.4152994148071514, -26.73475809017443794, 24.96913296066860255 ) ) ;
#36464=CARTESIAN_POINT ( 'NONE',  ( 113.3421067344362996, -42.52364098839497331, 122.6552769709339827 ) ) ;
#36465=CARTESIAN_POINT ( 'NONE',  ( 110.9007760261032871, -26.97308707819648887, 269.7784824187680783 ) ) ;
#36467=PLANE ( 'NONE',  #67293 ) ;
#36470=EDGE_CURVE ( 'NONE', #34937, #37435, #50185, .T. ) ;
#36472=CARTESIAN_POINT ( 'NONE',  ( 25.56670390244797275, -67.87844715994100397, 257.2178068554150059 ) ) ;
#36473=CARTESIAN_POINT ( 'NONE',  ( 83.06670390244796920, -61.87844715994100397, 207.5838068554149913 ) ) ;
#36475=EDGE_CURVE ( 'NONE', #32010, #8825, #12526, .T. ) ;
#36476=CARTESIAN_POINT ( 'NONE',  ( 99.65330034922125435, -46.03930839343899351, 122.0413395616249659 ) ) ;
#36477=CARTESIAN_POINT ( 'NONE',  ( 80.54920390244805617, -43.72944715994108833, 207.5838068554169809 ) ) ;
#36479=CARTESIAN_POINT ( 'NONE',  ( 111.8641478345923019, -46.02505481121716002, 272.9556252759110180 ) ) ;
#36480=CARTESIAN_POINT ( 'NONE',  ( 98.38769172161842391, -42.09058819985752109, 7.768006228291934434 ) ) ;
#36481=DIRECTION ( 'NONE',  ( 0.000000000000000000, 0.000000000000000000, -1.000000000000000000 ) ) ;
#36483=EDGE_CURVE ( 'NONE', #76542, #42554, #63297, .T. ) ;
#36485=DIRECTION ( 'NONE',  ( 0.000000000000000000, 0.000000000000000000, -1.000000000000000000 ) ) ;
#36488=FACE_OUTER_BOUND ( 'NONE', #45909, .T. ) ;
#36489=AXIS2_PLACEMENT_3D ( 'NONE', #46628, #60709, #47068 ) ;
#36491=DIRECTION ( 'NONE',  ( 4.299999999999999979E-14, -1.000000000000000000, 0.000000000000000000 ) ) ;
#36492=DIRECTION ( 'NONE',  ( 0.7071067811866279529, -0.7071067811864671926, 7.071067811866286874E-16 ) ) ;
#36494=PLANE ( 'NONE',  #74738 ) ;
#36497=CARTESIAN_POINT ( 'NONE',  ( 104.6386611584700432, -47.56081657070318158, 27.38895860924395009 ) ) ;
#36498=CARTESIAN_POINT ( 'NONE',  ( 117.8006386470660658, -34.09280371250640940, 160.0061014663869798 ) ) ;
#36499=CARTESIAN_POINT ( 'NONE',  ( 96.81221355789537597, -38.90410760351644370, 27.49276813305395706 ) ) ;
#36500=AXIS2_PLACEMENT_3D ( 'NONE', #34564, #83631, #81845 ) ;
#36501=LINE ( 'NONE', #42387, #52224 ) ;
#36502=CARTESIAN_POINT ( 'NONE',  ( 107.0664832912739541, -36.72944715994095333, 305.0306255462182321 ) ) ;
#36503=DIRECTION ( 'NONE',  ( 1.054009200593500181E-15, 1.000000000000000000, 0.000000000000000000 ) ) ;
#36505=VECTOR ( 'NONE', #49944, 1000.000000000000000 ) ;
#36509=CARTESIAN_POINT ( 'NONE',  ( 104.2296407737279935, -46.70397019442127373, 63.36800622829197494 ) ) ;
#36511=ORIENTED_EDGE ( 'NONE', *, *, #60787, .F. ) ;
#36512=DIRECTION ( 'NONE',  ( 1.000000000000000000, 4.299999999999999979E-14, 1.000000000000000078E-15 ) ) ;
#36513=CARTESIAN_POINT ( 'NONE',  ( 100.0229104548316883, -27.23016881827670943, 181.5841967044829630 ) ) ;
#36515=CARTESIAN_POINT ( 'NONE',  ( 110.8543535328673073, -45.98428584226713411, 147.8856150920996413 ) ) ;
#36517=CARTESIAN_POINT ( 'NONE',  ( 177.8371591254545478, -47.82818131005477369, 129.9678068554150059 ) ) ;
#36518=AXIS2_PLACEMENT_3D ( 'NONE', #59401, #52568, #85810 ) ;
#36519=ADVANCED_FACE ( 'NONE', ( #43114 ), #70859, .T. ) ;
#36521=CARTESIAN_POINT ( 'NONE',  ( 114.7254303483478992, -43.19231997828638470, 98.26877717035283410 ) ) ;
#36522=EDGE_CURVE ( 'NONE', #70069, #36736, #62228, .T. ) ;
#36523=CARTESIAN_POINT ( 'NONE',  ( 117.0231039428183522, -39.62849705588583760, 138.5889586092449690 ) ) ;
#36524=EDGE_LOOP ( 'NONE', ( #76373, #59409, #20739, #46567 ) ) ;
#36525=ORIENTED_EDGE ( 'NONE', *, *, #72051, .T. ) ;
#36526=AXIS2_PLACEMENT_3D ( 'NONE', #6988, #69216, #1530 ) ;
#36527=CARTESIAN_POINT ( 'NONE',  ( 104.1188366437555288, -45.08645965563772506, 53.73872616303998484 ) ) ;
#36528=LINE ( 'NONE', #14292, #67501 ) ;
#36529=CARTESIAN_POINT ( 'NONE',  ( 98.48461633480667388, -41.42146110206439147, 217.7241967044819546 ) ) ;
#36531=DIRECTION ( 'NONE',  ( 1.000000000000000078E-15, 1.000000000000000083E-30, -1.000000000000000000 ) ) ;
#36533=AXIS2_PLACEMENT_3D ( 'NONE', #68977, #61255, #82629 ) ;
#36534=LINE ( 'NONE', #57400, #5484 ) ;
#36535=DIRECTION ( 'NONE',  ( -0.7071067811856560636, -0.7071067811874389708, 0.000000000000000000 ) ) ;
#36537=CARTESIAN_POINT ( 'NONE',  ( 97.59110611908489830, -31.08311649095515250, 130.9108633711489915 ) ) ;
#36539=EDGE_LOOP ( 'NONE', ( #5989, #11638, #39936, #10740 ) ) ;
#36540=VECTOR ( 'NONE', #29778, 1000.000000000000000 ) ;
#36541=EDGE_LOOP ( 'NONE', ( #16083, #76418, #15817, #17466 ) ) ;
#36542=EDGE_CURVE ( 'NONE', #19234, #86883, #64035, .T. ) ;
#36544=CARTESIAN_POINT ( 'NONE',  ( 97.12560902511589234, -37.99725552183497967, 131.4273394659764449 ) ) ;
#36545=DIRECTION ( 'NONE',  ( 0.000000000000000000, 0.000000000000000000, -1.000000000000000000 ) ) ;
#36546=CARTESIAN_POINT ( 'NONE',  ( 109.7539934464052465, -29.02185251678796618, 207.6280903695909501 ) ) ;
#36547=EDGE_CURVE ( 'NONE', #61434, #39757, #84942, .T. ) ;
#36548=FACE_OUTER_BOUND ( 'NONE', #60193, .T. ) ;
#36549=CARTESIAN_POINT ( 'NONE',  ( 103.4683284843053883, -46.51414440030927011, 142.2956252759109645 ) ) ;
#36550=CARTESIAN_POINT ( 'NONE',  ( 83.73314995794051185, 12.92155284005802685, 335.5992267699911054 ) ) ;
#36551=EDGE_LOOP ( 'NONE', ( #78747, #83980, #34265, #61151 ) ) ;
#36553=ORIENTED_EDGE ( 'NONE', *, *, #10406, .F. ) ;
#36554=AXIS2_PLACEMENT_3D ( 'NONE', #49767, #7562, #83875 ) ;
#36555=LINE ( 'NONE', #76991, #79597 ) ;
#36557=ORIENTED_EDGE ( 'NONE', *, *, #43012, .T. ) ;
#36558=DIRECTION ( 'NONE',  ( -6.193183223602000661E-14, 1.000000000000000000, -6.293183223602000206E-29 ) ) ;
#36559=CARTESIAN_POINT ( 'NONE',  ( 131.5565945955609095, -35.60518703966645404, 7.068229416965921885 ) ) ;
#36560=CARTESIAN_POINT ( 'NONE',  ( 116.0742395100671871, -34.51300936444170020, 11.83666179816295028 ) ) ;
#36562=VERTEX_POINT ( 'NONE', #7720 ) ;
#36564=CARTESIAN_POINT ( 'NONE',  ( 115.8237480606924379, -40.07876769136255035, 9.635625275910941312 ) ) ;
#36565=CARTESIAN_POINT ( 'NONE',  ( 152.4409905591762424, -0.9151414768250908383, 542.9756252759101471 ) ) ;
#36566=ORIENTED_EDGE ( 'NONE', *, *, #63331, .T. ) ;
#36567=VERTEX_POINT ( 'NONE', #48577 ) ;
#36568=AXIS2_PLACEMENT_3D ( 'NONE', #47483, #248, #40684 ) ;
#36569=CARTESIAN_POINT ( 'NONE',  ( 101.9936682836478639, -45.44610077275940085, 112.1565371792481329 ) ) ;
#36570=ORIENTED_EDGE ( 'NONE', *, *, #43633, .F. ) ;
#36571=ORIENTED_EDGE ( 'NONE', *, *, #61756, .T. ) ;
#36572=EDGE_CURVE ( 'NONE', #89295, #2919, #15399, .T. ) ;
#36573=EDGE_CURVE ( 'NONE', #51954, #45647, #83587, .T. ) ;
#36574=CARTESIAN_POINT ( 'NONE',  ( 112.8202834993214481, -29.45004372636961065, 272.3623760838771091 ) ) ;
#36575=CARTESIAN_POINT ( 'NONE',  ( 117.3318588842742685, -34.78817910010258174, 158.9756252759109714 ) ) ;
#36577=CARTESIAN_POINT ( 'NONE',  ( 117.5589153096732105, -33.32758106675089493, 134.0880062282919880 ) ) ;
#36580=CARTESIAN_POINT ( 'NONE',  ( 113.2200137887798235, -45.14470412949270184, 224.0784824187679476 ) ) ;
#36581=CARTESIAN_POINT ( 'NONE',  ( 116.3185177584062444, -32.94221225046054968, 100.1356252759109680 ) ) ;
#36585=EDGE_LOOP ( 'NONE', ( #16193, #83299 ) ) ;
#36587=ORIENTED_EDGE ( 'NONE', *, *, #13757, .F. ) ;
#36589=ADVANCED_FACE ( 'NONE', ( #30403 ), #17227, .T. ) ;
#36590=AXIS2_PLACEMENT_3D ( 'NONE', #25834, #46245, #19017 ) ;
#36591=CARTESIAN_POINT ( 'NONE',  ( 103.6240789207236475, -26.17659276989511596, 210.3394347997209763 ) ) ;
#36592=ORIENTED_EDGE ( 'NONE', *, *, #33860, .F. ) ;
#36593=CARTESIAN_POINT ( 'NONE',  ( 114.5123156819773698, -29.42664080734638787, 149.4441967044819819 ) ) ;
#36594=CARTESIAN_POINT ( 'NONE',  ( 100.9565531848881079, -28.70555496000909912, 255.5938937405331615 ) ) ;
#36595=CARTESIAN_POINT ( 'NONE',  ( 134.8062005078064090, -34.05355276379778218, 8.162233076793905084 ) ) ;
#36598=DIRECTION ( 'NONE',  ( 0.000000000000000000, 0.000000000000000000, -1.000000000000000000 ) ) ;
#36599=CARTESIAN_POINT ( 'NONE',  ( 103.9458437887066111, -26.80522050874827755, 246.3184824187679567 ) ) ;
#36600=CARTESIAN_POINT ( 'NONE',  ( 116.3130905035090876, -32.93898513502411163, 35.13562527591096796 ) ) ;
#36602=EDGE_CURVE ( 'NONE', #11834, #85625, #50840, .T. ) ;
#36603=CIRCLE ( 'NONE', #87354, 2.117000000000007987 ) ;
#36605=FACE_OUTER_BOUND ( 'NONE', #4270, .T. ) ;
#36607=AXIS2_PLACEMENT_3D ( 'NONE', #3741, #24192, #43723 ) ;
#36608=FACE_OUTER_BOUND ( 'NONE', #59947, .T. ) ;
#36609=CARTESIAN_POINT ( 'NONE',  ( 103.6824468220397080, -44.03050751637072580, 195.5838068554171230 ) ) ;
#36612=CARTESIAN_POINT ( 'NONE',  ( 116.6812525300504291, -40.81632573062672265, 168.5070538473399608 ) ) ;
#36613=CARTESIAN_POINT ( 'NONE',  ( 96.79170515468972269, -38.49336940632627346, 87.46133956162493917 ) ) ;
#36614=CARTESIAN_POINT ( 'NONE',  ( 108.6817352505430705, -26.38614300430984372, 185.9527681330539792 ) ) ;
#36615=LINE ( 'NONE', #2085, #72317 ) ;
#36616=CARTESIAN_POINT ( 'NONE',  ( 51.56670390244799762, -33.35206098992650681, 313.9678068554150059 ) ) ;
#36617=LINE ( 'NONE', #28437, #53587 ) ;
#36618=FACE_OUTER_BOUND ( 'NONE', #82921, .T. ) ;
#36619=B_SPLINE_CURVE_WITH_KNOTS ( 'NONE', 3,
 ( #13967, #40764, #88932, #13519, #7161, #68487, #42107, #69832, #34397, #41203, #76188, #68930, #34852, #6256, #19431, #26686, #47567, #33947, #7606, #48448, #41647, #12627, #27592, #40314, #27147, #62558, #35289, #89841, #61645, #55271, #63001 ),
 .UNSPECIFIED., .F., .F.,
 ( 4, 2, 2, 1, 2, 2, 2, 2, 2, 2, 2, 1, 1, 2, 2, 2, 4 ),
 ( 0.000000000000000000, 0.1249999999999550360, 0.1874999999999277245, 0.2187499999999183153, 0.2343749999999145128, 0.2499999999999106826, 0.3749999999999218958, 0.4374999999999263367, 0.4999999999999307221, 0.6249999999999393818, 0.6874999999999438227, 0.7187499999999441558, 0.7343749999999424904, 0.7421874999999451550, 0.7499999999999479305, 0.8749999999999739098, 1.000000000000000000 ),
 .UNSPECIFIED. ) ;
#36622=ORIENTED_EDGE ( 'NONE', *, *, #40010, .F. ) ;
#36623=CARTESIAN_POINT ( 'NONE',  ( 97.07208351798986712, -35.37818212751453473, 66.21999532449092385 ) ) ;
#36624=ORIENTED_EDGE ( 'NONE', *, *, #15576, .T. ) ;
#36626=CARTESIAN_POINT ( 'NONE',  ( 107.0664832912739968, -36.72944715994100306, 287.6356252759109680 ) ) ;
#36629=CARTESIAN_POINT ( 'NONE',  ( 117.3423061886548027, -38.35306328171702717, 109.7013395616249767 ) ) ;
#36630=CARTESIAN_POINT ( 'NONE',  ( 131.0667039024480687, -51.22944715994093201, 207.5838068554170377 ) ) ;
#36632=CARTESIAN_POINT ( 'NONE',  ( 98.34985892603175728, -31.65658478673192278, 176.9064586071441170 ) ) ;
#36633=EDGE_CURVE ( 'NONE', #18008, #52712, #86710, .T. ) ;
#36634=CARTESIAN_POINT ( 'NONE',  ( 115.8929839771518573, -32.51563103440816604, 19.18133956162593279 ) ) ;
#36635=ORIENTED_EDGE ( 'NONE', *, *, #87123, .T. ) ;
#36638=VECTOR ( 'NONE', #25239, 1000.000000000000000 ) ;
#36639=CYLINDRICAL_SURFACE ( 'NONE', #28272, 6.571100913904396101 ) ;
#36640=CARTESIAN_POINT ( 'NONE',  ( 193.5667039024485803, -48.82844715993409324, 180.4678068554150343 ) ) ;
#36641=DIRECTION ( 'NONE',  ( 0.000000000000000000, 0.000000000000000000, -1.000000000000000000 ) ) ;
#36642=CARTESIAN_POINT ( 'NONE',  ( 176.5667039024410769, -48.82844715994099971, 300.4678068554149490 ) ) ;
#36644=DIRECTION ( 'NONE',  ( -1.000000000000000078E-15, 0.000000000000000000, -1.000000000000000000 ) ) ;
#36647=CARTESIAN_POINT ( 'NONE',  ( 116.7496603916997202, -31.44741115753626204, 24.21181575210196257 ) ) ;
#36651=CARTESIAN_POINT ( 'NONE',  ( 71.24189083761808661, -0.9290567490904538817, 542.9756252759101471 ) ) ;
#36652=CARTESIAN_POINT ( 'NONE',  ( 112.3828903148906306, -42.92343960232698663, 105.9595189410199652 ) ) ;
#36654=EDGE_CURVE ( 'NONE', #88172, #59914, #44007, .T. ) ;
#36655=CARTESIAN_POINT ( 'NONE',  ( 98.34892672930283197, -31.65823485578066965, 95.90661232045958684 ) ) ;
#36656=AXIS2_PLACEMENT_3D ( 'NONE', #23323, #30996, #80059 ) ;
#36657=DIRECTION ( 'NONE',  ( 0.000000000000000000, 0.000000000000000000, 1.000000000000000000 ) ) ;
#36659=VERTEX_POINT ( 'NONE', #23607 ) ;
#36660=DIRECTION ( 'NONE',  ( 0.7071067811575828532, -0.7071067812155121812, 0.000000000000000000 ) ) ;
#36661=ORIENTED_EDGE ( 'NONE', *, *, #79338, .F. ) ;
#36662=EDGE_LOOP ( 'NONE', ( #44008, #23056, #41151, #53818 ) ) ;
#36663=CARTESIAN_POINT ( 'NONE',  ( 113.0289363901617889, -43.32575541760495241, 129.5930118773259778 ) ) ;
#36664=CARTESIAN_POINT ( 'NONE',  ( 49.16670390244701139, -26.71338133339240528, -5.074374724088000832 ) ) ;
#36665=CARTESIAN_POINT ( 'NONE',  ( 107.6042626387647090, -26.26092342527675072, 91.03562527591097364 ) ) ;
#36666=B_SPLINE_CURVE_WITH_KNOTS ( 'NONE', 3,
 ( #82282, #89533, #75894, #41793, #21381, #27737, #35437, #55864, #14574, #13663, #63154, #41348, #49055, #27289, #42249, #61349, #935, #20493, #54964, #6847, #55420, #83172, #13225, #20930, #69978, #7745, #76337, #69530 ),
 .UNSPECIFIED., .F., .F.,
 ( 4, 2, 2, 2, 2, 2, 2, 2, 2, 2, 1, 1, 1, 1, 2, 4 ),
 ( 0.000000000000000000, 0.06250189622662993827, 0.1250037924532598765, 0.1875056886798898148, 0.2500075849065197531, 0.3125094811331496913, 0.3750113773597796296, 0.4375132735864095679, 0.4687642216997245370, 0.4843896957563820771, 0.4922024327847105973, 0.4961088012988748019, 0.4980619855559567100, 0.4990385776844978305, 0.4995268737487682520, 0.5000151698130386180 ),
 .UNSPECIFIED. ) ;
#36667=CARTESIAN_POINT ( 'NONE',  ( 110.8549796485604020, -45.98402957564880467, 17.88566890375461327 ) ) ;
#36668=VERTEX_POINT ( 'NONE', #44457 ) ;
#36669=VERTEX_POINT ( 'NONE', #24487 ) ;
#36670=ORIENTED_EDGE ( 'NONE', *, *, #5457, .T. ) ;
#36672=CARTESIAN_POINT ( 'NONE',  ( 112.1934831763302896, -30.37778608165438854, 162.3538046553059644 ) ) ;
#36673=AXIS2_PLACEMENT_3D ( 'NONE', #84673, #22437, #9689 ) ;
#36674=CARTESIAN_POINT ( 'NONE',  ( 116.7655018478977951, -32.84674153052576884, 54.12991099019698282 ) ) ;
#36677=CARTESIAN_POINT ( 'NONE',  ( 105.9906760191434358, -26.38192068051316141, 50.15848241876796720 ) ) ;
#36678=CARTESIAN_POINT ( 'NONE',  ( 102.9585648456520772, -26.44303807861259870, 171.3908633711489813 ) ) ;
#36679=FACE_OUTER_BOUND ( 'NONE', #70979, .T. ) ;
#36682=CARTESIAN_POINT ( 'NONE',  ( 106.0764678730365063, -48.53853201145131635, 108.5099109901969712 ) ) ;
#36683=CARTESIAN_POINT ( 'NONE',  ( 98.30753421155790761, -41.72887552731712901, 261.7397919458750835 ) ) ;
#36684=ORIENTED_EDGE ( 'NONE', *, *, #69295, .T. ) ;
#36685=DIRECTION ( 'NONE',  ( 1.000000000000000000, 0.000000000000000000, 0.000000000000000000 ) ) ;
#36686=ADVANCED_FACE ( 'NONE', ( #17667 ), #85393, .F. ) ;
#36687=ORIENTED_EDGE ( 'NONE', *, *, #12157, .F. ) ;
#36690=VERTEX_POINT ( 'NONE', #73064 ) ;
#36691=VECTOR ( 'NONE', #85396, 1000.000000000000000 ) ;
#36694=CARTESIAN_POINT ( 'NONE',  ( 107.1954010100577364, -26.30493706674213428, 35.06705384733893283 ) ) ;
#36697=CARTESIAN_POINT ( 'NONE',  ( 21.56670390244604718, -23.42844715994195326, 180.4678068554150911 ) ) ;
#36698=CARTESIAN_POINT ( 'NONE',  ( 116.8124865092211451, -37.88235468918158944, 53.73276813305394484 ) ) ;
#36699=FACE_OUTER_BOUND ( 'NONE', #13146, .T. ) ;
#36700=CARTESIAN_POINT ( 'NONE',  ( 95.59354794629810215, -39.59649474372135813, 162.5213395616259788 ) ) ;
#36701=CARTESIAN_POINT ( 'NONE',  ( 25.56670390244828894, -48.82844715994168183, 293.2178068554150059 ) ) ;
#36702=DIRECTION ( 'NONE',  ( 0.000000000000000000, 0.000000000000000000, -1.000000000000000000 ) ) ;
#36706=FACE_OUTER_BOUND ( 'NONE', #19088, .T. ) ;
#36709=DIRECTION ( 'NONE',  ( -4.299999999999999979E-14, 1.000000000000000000, -4.400000000000000367E-29 ) ) ;
#36710=CARTESIAN_POINT ( 'NONE',  ( 108.8564100269821608, -47.04462182233018552, 167.7127681330539701 ) ) ;
#36713=CARTESIAN_POINT ( 'NONE',  ( 99.52368306943544951, -29.45034277662237443, 246.7156252759109520 ) ) ;
#36714=CARTESIAN_POINT ( 'NONE',  ( 96.59565658895887452, -37.56598942197172164, 97.38991099019594344 ) ) ;
#36715=CARTESIAN_POINT ( 'NONE',  ( 97.06097963517905214, -37.99593394772350052, 252.4290318010866656 ) ) ;
#36717=CARTESIAN_POINT ( 'NONE',  ( 105.7973883670204600, -26.72432487108696009, 191.1772404832683208 ) ) ;
#36718=CARTESIAN_POINT ( 'NONE',  ( 112.0659116283640060, -45.48839625712076185, 77.98979194311773711 ) ) ;
#36719=EDGE_LOOP ( 'NONE', ( #14112, #56539, #35835, #12960 ) ) ;
#36721=AXIS2_PLACEMENT_3D ( 'NONE', #13325, #5624, #54620 ) ;
#36723=EDGE_LOOP ( 'NONE', ( #72364, #40929, #13, #80440 ) ) ;
#36725=ORIENTED_EDGE ( 'NONE', *, *, #16230, .F. ) ;
#36726=CARTESIAN_POINT ( 'NONE',  ( 49.16670390244701139, -26.71338133339240528, -5.074374724088000832 ) ) ;
#36727=CARTESIAN_POINT ( 'NONE',  ( 98.83931482081872844, -29.34787013040062931, 231.7565776568629587 ) ) ;
#36728=FACE_OUTER_BOUND ( 'NONE', #61920, .T. ) ;
#36730=DIRECTION ( 'NONE',  ( 0.000000000000000000, 0.000000000000000000, -1.000000000000000000 ) ) ;
#36731=DIRECTION ( 'NONE',  ( 1.000000000000000078E-15, -1.000000000000000083E-30, -1.000000000000000000 ) ) ;
#36732=LINE ( 'NONE', #86222, #31209 ) ;
#36733=ADVANCED_FACE ( 'NONE', ( #37217 ), #2258, .T. ) ;
#36734=CARTESIAN_POINT ( 'NONE',  ( 96.69266203715996255, -37.96645829736812061, 41.42133956162496844 ) ) ;
#36736=VERTEX_POINT ( 'NONE', #22708 ) ;
#36737=ORIENTED_EDGE ( 'NONE', *, *, #9289, .T. ) ;
#36738=CARTESIAN_POINT ( 'NONE',  ( 107.0664832912739257, -49.89611382660765315, 357.5272416190308604 ) ) ;
#36739=CIRCLE ( 'NONE', #13514, 10.00000000000000355 ) ;
#36741=EDGE_CURVE ( 'NONE', #10572, #73470, #64921, .T. ) ;
#36742=CARTESIAN_POINT ( 'NONE',  ( 102.6690082227317475, -46.93785447722112281, 283.2527681330534506 ) ) ;
#36744=AXIS2_PLACEMENT_3D ( 'NONE', #28222, #54560, #83659 ) ;
#36745=CARTESIAN_POINT ( 'NONE',  ( 116.5825849560771417, -39.12894369053751120, 119.6299109901959525 ) ) ;
#36747=ORIENTED_EDGE ( 'NONE', *, *, #7241, .T. ) ;
#36748=CARTESIAN_POINT ( 'NONE',  ( 51.42025729302798709, -31.94127993907680718, 313.9678068554150059 ) ) ;
#36749=CARTESIAN_POINT ( 'NONE',  ( 77.66889017809432971, -35.37024878622109725, 2.654395752959056498 ) ) ;
#36752=CARTESIAN_POINT ( 'NONE',  ( 102.0014872285204035, -30.29305903553749602, 13.42523322673394581 ) ) ;
#36753=EDGE_CURVE ( 'NONE', #89702, #82107, #85835, .T. ) ;
#36755=DIRECTION ( 'NONE',  ( -4.237773401492740281E-14, 1.000000000000000000, 0.000000000000000000 ) ) ;
#36756=CARTESIAN_POINT ( 'NONE',  ( 116.3263622980238097, -32.93962144782776846, 195.1356252759109680 ) ) ;
#36757=ORIENTED_EDGE ( 'NONE', *, *, #47214, .T. ) ;
#36759=DIRECTION ( 'NONE',  ( 1.000000000000000000, 4.510281037539819615E-14, 0.000000000000000000 ) ) ;
#36760=ORIENTED_EDGE ( 'NONE', *, *, #30746, .T. ) ;
#36761=CARTESIAN_POINT ( 'NONE',  ( 103.8412645720801493, -46.68052101597508852, 82.32705384733995402 ) ) ;
#36763=CARTESIAN_POINT ( 'NONE',  ( 98.75426529987753099, -33.13504840779251737, 60.43622935188691514 ) ) ;
#36764=EDGE_CURVE ( 'NONE', #74855, #8105, #65366, .T. ) ;
#36766=CARTESIAN_POINT ( 'NONE',  ( 117.1170091337237551, -34.17489915221370467, 169.0365776568639831 ) ) ;
#36768=DIRECTION ( 'NONE',  ( 1.000000000000000078E-15, 1.000000000000000083E-30, -1.000000000000000000 ) ) ;
#36769=LINE ( 'NONE', #1807, #1318 ) ;
#36770=DIRECTION ( 'NONE',  ( 4.299999999999999979E-14, -1.000000000000000000, 4.400000000000000367E-29 ) ) ;
#36771=CARTESIAN_POINT ( 'NONE',  ( 108.0180542234412684, -24.86750695335871697, 261.0127681330534415 ) ) ;
#36772=B_SPLINE_CURVE_WITH_KNOTS ( 'NONE', 3,
 ( #77292, #16410, #58181, #85471, #86348, #44086, #71821, #78206, #85911, #3227, #15967, #23683, #9590, #35949, #79092, #43648, #65447, #42741 ),
 .UNSPECIFIED., .F., .F.,
 ( 4, 2, 2, 2, 2, 2, 2, 2, 4 ),
 ( 0.000000000000000000, 0.06250441113620554268, 0.1250088222724110854, 0.1875132334086166419, 0.2500176445448221707, 0.3125220556810276995, 0.3750264668172332838, 0.4375308779534388126, 0.5000352890896443414 ),
 .UNSPECIFIED. ) ;
#36773=ORIENTED_EDGE ( 'NONE', *, *, #27471, .F. ) ;
#36776=CARTESIAN_POINT ( 'NONE',  ( 114.2047867640113594, -45.22899916922247598, 144.1203871806729637 ) ) ;
#36779=ORIENTED_EDGE ( 'NONE', *, *, #49156, .F. ) ;
#36780=ORIENTED_EDGE ( 'NONE', *, *, #80153, .T. ) ;
#36782=CARTESIAN_POINT ( 'NONE',  ( 41.56648329127398966, -27.82844715994070484, 318.9256252759120116 ) ) ;
#36783=DIRECTION ( 'NONE',  ( 1.000000000000000000, -6.938893903907232322E-15, -2.775557561562892929E-14 ) ) ;
#36784=CARTESIAN_POINT ( 'NONE',  ( 97.81168921572486852, -40.51740600946125426, 16.63579259794490284 ) ) ;
#36785=DIRECTION ( 'NONE',  ( 0.000000000000000000, 1.000000000000000000, 0.000000000000000000 ) ) ;
#36786=DIRECTION ( 'NONE',  ( 0.000000000000000000, -1.000000000000000000, 0.000000000000000000 ) ) ;
#36787=EDGE_CURVE ( 'NONE', #72226, #82610, #52591, .T. ) ;
#36788=CARTESIAN_POINT ( 'NONE',  ( 116.7699407904022451, -31.43634848722146202, 20.21181575210195902 ) ) ;
#36789=DIRECTION ( 'NONE',  ( 1.907762142705490052E-15, 7.167082501179359715E-16, -1.000000000000000000 ) ) ;
#36790=ORIENTED_EDGE ( 'NONE', *, *, #79689, .F. ) ;
#36797=FACE_OUTER_BOUND ( 'NONE', #84845, .T. ) ;
#36799=FACE_OUTER_BOUND ( 'NONE', #685, .T. ) ;
#36801=CARTESIAN_POINT ( 'NONE',  ( 100.4104977919876802, -31.37650509455747283, 240.2095626852199928 ) ) ;
#36802=CARTESIAN_POINT ( 'NONE',  ( 142.0664832912740394, -56.47944715994099596, 14.67562527591100441 ) ) ;
#36803=CARTESIAN_POINT ( 'NONE',  ( 101.9712125536871383, -27.65933791914800111, 56.48419670448296159 ) ) ;
#36805=CARTESIAN_POINT ( 'NONE',  ( 104.0952645214482430, -46.76829794407347407, 107.3470538473389411 ) ) ;
#36806=EDGE_LOOP ( 'NONE', ( #3071, #27581, #9905, #74823, #68727 ) ) ;
#36808=EDGE_CURVE ( 'NONE', #41573, #83210, #21225, .T. ) ;
#36809=VERTEX_POINT ( 'NONE', #88507 ) ;
#36811=DIRECTION ( 'NONE',  ( 0.000000000000000000, 0.000000000000000000, -1.000000000000000000 ) ) ;
#36812=ADVANCED_FACE ( 'NONE', ( #53488 ), #83605, .F. ) ;
#36813=CARTESIAN_POINT ( 'NONE',  ( 104.6390307648651117, -27.02259228910022415, 276.2714668963693043 ) ) ;
#36814=EDGE_LOOP ( 'NONE', ( #45026, #49275, #50769, #38731, #27004, #40293 ) ) ;
#36815=CARTESIAN_POINT ( 'NONE',  ( 107.0664832912750057, -36.72944715993903486, 9.125625275910969947 ) ) ;
#36816=ORIENTED_EDGE ( 'NONE', *, *, #349, .T. ) ;
#36818=CARTESIAN_POINT ( 'NONE',  ( 188.5667039024483529, -48.82844715993431350, 290.7178068554150059 ) ) ;
#36819=VECTOR ( 'NONE', #52585, 1000.000000000000000 ) ;
#36820=DIRECTION ( 'NONE',  ( -8.673617379884035472E-16, -1.000000000000000000, 0.000000000000000000 ) ) ;
#36822=CARTESIAN_POINT ( 'NONE',  ( 111.0910783018720025, -25.55641485417826431, 99.80133956162498521 ) ) ;
#36824=CARTESIAN_POINT ( 'NONE',  ( 97.81167943543778165, -40.51737693692245301, 166.6360185166829808 ) ) ;
#36825=CARTESIAN_POINT ( 'NONE',  ( 51.06670390244760682, -32.29483332968566600, 313.9678068554150059 ) ) ;
#36828=CARTESIAN_POINT ( 'NONE',  ( 63.06670390244711655, -40.32844715994016838, 129.9678068554150911 ) ) ;
#36829=DIRECTION ( 'NONE',  ( 0.000000000000000000, 0.000000000000000000, -1.000000000000000000 ) ) ;
#36831=DIRECTION ( 'NONE',  ( 0.000000000000000000, 1.000000000000000000, 0.000000000000000000 ) ) ;
#36833=CARTESIAN_POINT ( 'NONE',  ( 87.06648329127402519, -54.72944906728955061, 14.67562527591094934 ) ) ;
#36834=AXIS2_PLACEMENT_3D ( 'NONE', #33238, #26427, #53193 ) ;
#36835=ORIENTED_EDGE ( 'NONE', *, *, #64868, .T. ) ;
#36838=EDGE_CURVE ( 'NONE', #49620, #86172, #79266, .T. ) ;
#36839=CARTESIAN_POINT ( 'NONE',  ( 105.8036208730406003, -25.68330614324009886, 156.1670538473389627 ) ) ;
#36842=CARTESIAN_POINT ( 'NONE',  ( 115.3963619165045458, -41.85549553236474196, 14.38705384733895976 ) ) ;
#36847=CARTESIAN_POINT ( 'NONE',  ( 100.2051353121704835, -29.75912871662441361, 225.6956252759109702 ) ) ;
#36848=ORIENTED_EDGE ( 'NONE', *, *, #85198, .T. ) ;
#36849=VERTEX_POINT ( 'NONE', #66697 ) ;
#36850=CARTESIAN_POINT ( 'NONE',  ( 116.3029726692365813, -35.00788115540211010, 200.4168214011349676 ) ) ;
#36851=VECTOR ( 'NONE', #51699, 1000.000000000000000 ) ;
#36852=DIRECTION ( 'NONE',  ( 1.000000000000000078E-15, 0.000000000000000000, 1.000000000000000000 ) ) ;
#36853=EDGE_CURVE ( 'NONE', #75906, #1995, #81867, .T. ) ;
#36854=CARTESIAN_POINT ( 'NONE',  ( 112.0788320361856307, -29.42159941445254390, 41.03015473446897232 ) ) ;
#36855=AXIS2_PLACEMENT_3D ( 'NONE', #76207, #77115, #70289 ) ;
#36858=ADVANCED_FACE ( 'NONE', ( #68500 ), #11744, .T. ) ;
#36861=DIRECTION ( 'NONE',  ( 1.000000000000000078E-15, -1.000000000000000083E-30, -1.000000000000000000 ) ) ;
#36862=CARTESIAN_POINT ( 'NONE',  ( 97.60794579242353564, -39.98258380600313444, 37.58978887728247287 ) ) ;
#36863=CARTESIAN_POINT ( 'NONE',  ( 106.1402962346845982, -47.72062544595571154, 262.4975300378158636 ) ) ;
#36865=ORIENTED_EDGE ( 'NONE', *, *, #46691, .T. ) ;
#36866=VERTEX_POINT ( 'NONE', #81253 ) ;
#36868=EDGE_CURVE ( 'NONE', #29421, #26390, #24205, .T. ) ;
#36869=CYLINDRICAL_SURFACE ( 'NONE', #21293, 2.030000000001310312 ) ;
#36870=DIRECTION ( 'NONE',  ( -1.000000000000000078E-15, 1.000000000000000083E-30, 1.000000000000000000 ) ) ;
#36871=CARTESIAN_POINT ( 'NONE',  ( 141.8664832912729992, -1.929447159941394263, 352.4506252759079530 ) ) ;
#36873=ADVANCED_FACE ( 'NONE', ( #67145 ), #68048, .F. ) ;
#36874=CARTESIAN_POINT ( 'NONE',  ( 109.4837483930865289, -46.20680252518636166, 43.77562527591094721 ) ) ;
#36877=CARTESIAN_POINT ( 'NONE',  ( 115.7648065088891371, -43.62413145733483333, 44.30514908543492680 ) ) ;
#36878=DIRECTION ( 'NONE',  ( -1.000000000000000078E-15, 1.000000000000000083E-30, 1.000000000000000000 ) ) ;
#36880=CARTESIAN_POINT ( 'NONE',  ( 96.32141381413643444, -39.41948438522342713, 16.53372051400597798 ) ) ;
#36881=ORIENTED_EDGE ( 'NONE', *, *, #53258, .F. ) ;
#36882=DIRECTION ( 'NONE',  ( 0.000000000000000000, 0.000000000000000000, -1.000000000000000000 ) ) ;
#36886=CARTESIAN_POINT ( 'NONE',  ( 107.8241526860280430, -28.10814435038363968, 107.8128522743529771 ) ) ;
#36887=CARTESIAN_POINT ( 'NONE',  ( 101.3372171518963398, -46.20893634704900421, 198.1318157521009482 ) ) ;
#36889=ORIENTED_EDGE ( 'NONE', *, *, #57852, .T. ) ;
#36890=CARTESIAN_POINT ( 'NONE',  ( 71.06648329127399677, -18.82844715994099971, 323.8756252759120002 ) ) ;
#36894=CARTESIAN_POINT ( 'NONE',  ( 131.0667039024480118, -61.87844715994100397, 237.1838068554150141 ) ) ;
#36895=VERTEX_POINT ( 'NONE', #67597 ) ;
#36896=ORIENTED_EDGE ( 'NONE', *, *, #20683, .T. ) ;
#36899=CARTESIAN_POINT ( 'NONE',  ( 112.7653361951733473, -30.36711996764882571, 113.9181341137909556 ) ) ;
#36900=CARTESIAN_POINT ( 'NONE',  ( 115.6735817710496264, -30.74561775548394849, 279.3099109901964994 ) ) ;
#36901=ADVANCED_FACE ( 'NONE', ( #22155 ), #77548, .T. ) ;
#36902=EDGE_CURVE ( 'NONE', #62685, #86125, #28042, .T. ) ;
#36904=VERTEX_POINT ( 'NONE', #13976 ) ;
#36906=VERTEX_POINT ( 'NONE', #89851 ) ;
#36908=EDGE_CURVE ( 'NONE', #82784, #73516, #83466, .T. ) ;
#36909=DIRECTION ( 'NONE',  ( 1.000000000000000000, -5.337610695313248426E-16, 0.000000000000000000 ) ) ;
#36910=CARTESIAN_POINT ( 'NONE',  ( 194.0371591254574923, -24.42818131005417115, 193.9678068554150343 ) ) ;
#36911=CARTESIAN_POINT ( 'NONE',  ( 161.4809174648183614, -49.32844715993547879, 300.4678068554149490 ) ) ;
#36912=AXIS2_PLACEMENT_3D ( 'NONE', #9840, #78449, #85708 ) ;
#36913=ORIENTED_EDGE ( 'NONE', *, *, #10669, .F. ) ;
#36915=CARTESIAN_POINT ( 'NONE',  ( 116.6059430675273063, -40.93488859202243901, 253.4956252759109532 ) ) ;
#36916=VECTOR ( 'NONE', #39600, 1000.000000000000000 ) ;
#36917=FACE_OUTER_BOUND ( 'NONE', #55603, .T. ) ;
#36921=DIRECTION ( 'NONE',  ( 1.000000000000000078E-15, -1.000000000000000000, 0.000000000000000000 ) ) ;
#36924=DIRECTION ( 'NONE',  ( 4.299999999999999979E-14, -1.000000000000000000, 4.400000000000000367E-29 ) ) ;
#36925=DIRECTION ( 'NONE',  ( -0.7071067811864687469, -0.7071067811866262875, -7.071067811864681542E-16 ) ) ;
#36927=AXIS2_PLACEMENT_3D ( 'NONE', #51513, #50633, #45579 ) ;
#36928=CARTESIAN_POINT ( 'NONE',  ( 97.07207205096092650, -35.37844125572550524, 12.21895861363828040 ) ) ;
#36930=FACE_OUTER_BOUND ( 'NONE', #37344, .T. ) ;
#36932=CARTESIAN_POINT ( 'NONE',  ( 96.61485869678695337, -32.99094118449985302, 26.06514908543494613 ) ) ;
#36933=CARTESIAN_POINT ( 'NONE',  ( 118.8773263846236148, -37.69826137473897631, 184.7613395616249647 ) ) ;
#36934=CARTESIAN_POINT ( 'NONE',  ( 104.5778203770529586, -26.56076746289640411, 281.2670538473396959 ) ) ;
#36935=CARTESIAN_POINT ( 'NONE',  ( 168.0371591254546217, -48.62818131005518296, 117.4678068554150485 ) ) ;
#36936=DIRECTION ( 'NONE',  ( 0.000000000000000000, -1.000000000000000000, 0.000000000000000000 ) ) ;
#36937=CARTESIAN_POINT ( 'NONE',  ( 82.59704509974031339, -35.65293374834178053, 2.807537076564044387 ) ) ;
#36939=LINE ( 'NONE', #43291, #79526 ) ;
#36940=ORIENTED_EDGE ( 'NONE', *, *, #16230, .T. ) ;
#36941=CARTESIAN_POINT ( 'NONE',  ( 99.96923091713372855, -43.45941328387849723, 77.92991099019597812 ) ) ;
#36943=VERTEX_POINT ( 'NONE', #21243 ) ;
#36945=CARTESIAN_POINT ( 'NONE',  ( 98.56907362037671305, -44.95393718666134930, 187.9384824187679612 ) ) ;
#36948=CARTESIAN_POINT ( 'NONE',  ( 104.4904853333757586, -26.97866173706016824, 150.2818345845702765 ) ) ;
#36950=DIRECTION ( 'NONE',  ( 0.000000000000000000, 0.000000000000000000, -1.000000000000000000 ) ) ;
#36951=CARTESIAN_POINT ( 'NONE',  ( 97.81554761001611098, -40.52684041789147074, 96.63643476469849247 ) ) ;
#36952=CARTESIAN_POINT ( 'NONE',  ( 116.1942131220466621, -33.21547736372279758, 139.1184824187689628 ) ) ;
#36953=VERTEX_POINT ( 'NONE', #7613 ) ;
#36955=CARTESIAN_POINT ( 'NONE',  ( 102.3355707743008765, -29.23633396390525618, 106.9558690201829734 ) ) ;
#36957=EDGE_CURVE ( 'NONE', #73636, #37760, #62568, .T. ) ;
#36958=CARTESIAN_POINT ( 'NONE',  ( 110.0587659310071302, -27.38278898179171605, 230.8299109901959412 ) ) ;
#36959=CARTESIAN_POINT ( 'NONE',  ( 107.0664832912740252, -46.47944715994103149, -4.824374724089029343 ) ) ;
#36960=VECTOR ( 'NONE', #13022, 1000.000000000000000 ) ;
#36968=CARTESIAN_POINT ( 'NONE',  ( 107.6517678568360594, -47.10594642807022581, 152.6213395616249500 ) ) ;
#36969=VERTEX_POINT ( 'NONE', #34861 ) ;
#36970=ORIENTED_EDGE ( 'NONE', *, *, #2189, .F. ) ;
#36971=ORIENTED_EDGE ( 'NONE', *, *, #69580, .F. ) ;
#36974=CARTESIAN_POINT ( 'NONE',  ( 88.17226027475679473, -58.72944715994100306, 239.5838068554174924 ) ) ;
#36975=CARTESIAN_POINT ( 'NONE',  ( 77.31651910784952975, -18.55813574388988485, 3.101427645696272606 ) ) ;
#36976=CARTESIAN_POINT ( 'NONE',  ( 105.7154773167319206, -46.72385839048828160, 78.46895860815600088 ) ) ;
#36978=CARTESIAN_POINT ( 'NONE',  ( 102.1208986914200665, -43.83170863157916131, 234.8985665600679624 ) ) ;
#36979=EDGE_CURVE ( 'NONE', #31161, #58675, #1250, .T. ) ;
#36980=AXIS2_PLACEMENT_3D ( 'NONE', #88906, #54338, #82104 ) ;
#36981=AXIS2_PLACEMENT_3D ( 'NONE', #60383, #89006, #82209 ) ;
#36984=VECTOR ( 'NONE', #14202, 1000.000000000000000 ) ;
#36985=EDGE_CURVE ( 'NONE', #18226, #22928, #40127, .T. ) ;
#36986=CARTESIAN_POINT ( 'NONE',  ( 113.6143417880574020, -45.63476223351307226, 183.0689586092439640 ) ) ;
#36987=DIRECTION ( 'NONE',  ( 1.000000000000000078E-15, -1.000000000000000000, 0.000000000000000000 ) ) ;
#36989=ORIENTED_EDGE ( 'NONE', *, *, #28895, .F. ) ;
#36990=EDGE_LOOP ( 'NONE', ( #37774, #43059, #88511, #25251, #81271 ) ) ;
#36992=CARTESIAN_POINT ( 'NONE',  ( 31.89136050872298966, -31.76306994223740432, -5.074374724088000832 ) ) ;
#36994=ORIENTED_EDGE ( 'NONE', *, *, #8596, .T. ) ;
#36995=DIRECTION ( 'NONE',  ( 1.000000000000000078E-15, 0.000000000000000000, 1.000000000000000000 ) ) ;
#36998=CARTESIAN_POINT ( 'NONE',  ( 105.9698521113164844, -27.93594508925886188, 266.6072975916113705 ) ) ;
#36999=CARTESIAN_POINT ( 'NONE',  ( 113.1782932911942936, -44.75186896820116544, 273.0939585610741460 ) ) ;
#37001=CIRCLE ( 'NONE', #73290, 1.000000000000000888 ) ;
#37002=CARTESIAN_POINT ( 'NONE',  ( 106.3677493097285662, -44.90353489983662172, 9.635625275910937759 ) ) ;
#37003=EDGE_CURVE ( 'NONE', #27372, #29714, #83929, .T. ) ;
#37004=FACE_OUTER_BOUND ( 'NONE', #8869, .T. ) ;
#37006=ORIENTED_EDGE ( 'NONE', *, *, #18037, .F. ) ;
#37008=VERTEX_POINT ( 'NONE', #8514 ) ;
#37010=AXIS2_PLACEMENT_3D ( 'NONE', #34668, #18809, #26077 ) ;
#37011=CARTESIAN_POINT ( 'NONE',  ( 114.1180452634077369, -42.41171291218270767, 42.69718173283898466 ) ) ;
#37012=CARTESIAN_POINT ( 'NONE',  ( 97.40467406345878487, -42.14653896106843689, 181.7451490854349743 ) ) ;
#37013=CARTESIAN_POINT ( 'NONE',  ( 97.85535806214033983, -31.89376338832682123, 135.9413395616259947 ) ) ;
#37015=CARTESIAN_POINT ( 'NONE',  ( 100.7501737310821994, -45.80018108968007340, 233.0803871806729717 ) ) ;
#37016=CARTESIAN_POINT ( 'NONE',  ( 193.0371591254585724, -47.82818131005411999, 129.9678068554150343 ) ) ;
#37019=EDGE_LOOP ( 'NONE', ( #13722, #66904 ) ) ;
#37022=EDGE_CURVE ( 'NONE', #61208, #59170, #84129, .T. ) ;
#37023=CARTESIAN_POINT ( 'NONE',  ( 117.4576385420935338, -35.45251388149282690, 193.9241967044829664 ) ) ;
#37024=VERTEX_POINT ( 'NONE', #16663 ) ;
#37025=CARTESIAN_POINT ( 'NONE',  ( 112.4862084254573631, -26.19061110901967382, 169.6984824187679521 ) ) ;
#37026=DIRECTION ( 'NONE',  ( 1.000000000000000078E-15, -1.000000000000000083E-30, -1.000000000000000000 ) ) ;
#37027=AXIS2_PLACEMENT_3D ( 'NONE', #2527, #56109, #63858 ) ;
#37028=CARTESIAN_POINT ( 'NONE',  ( 135.2364670978292907, -34.23881677343971575, 8.012604158001305876 ) ) ;
#37031=DIRECTION ( 'NONE',  ( 1.000000000000000000, 1.780283607454400635E-15, 0.000000000000000000 ) ) ;
#37032=CARTESIAN_POINT ( 'NONE',  ( 104.3301552612371523, -26.04411461992211230, 241.2880062282919482 ) ) ;
#37033=DIRECTION ( 'NONE',  ( 0.000000000000000000, -1.000000000000000000, 0.000000000000000000 ) ) ;
#37035=LINE ( 'NONE', #86090, #46914 ) ;
#37037=B_SPLINE_CURVE_WITH_KNOTS ( 'NONE', 3,
 ( #62539, #63899, #70257, #56613, #13945, #27573, #77523, #315, #89821, #57056, #84802, #48887, #76625, #14407, #77977, #42082, #15750, #83902 ),
 .UNSPECIFIED., .F., .F.,
 ( 4, 2, 2, 2, 2, 2, 2, 2, 4 ),
 ( 0.000000000000000000, 0.06249209452423747091, 0.1249841890484749418, 0.1874762835727123989, 0.2499683780969498836, 0.3124604726211873684, 0.3749525671454247977, 0.4374446616696622825, 0.4999367561938997673 ),
 .UNSPECIFIED. ) ;
#37038=CARTESIAN_POINT ( 'NONE',  ( 115.0372575140148115, -42.90846255661264053, 259.3022919435708218 ) ) ;
#37040=CARTESIAN_POINT ( 'NONE',  ( 113.6372100165067422, -30.15837270650189339, 195.5838068554168103 ) ) ;
#37041=EDGE_LOOP ( 'NONE', ( #78052, #37576, #3542, #19825, #59633, #2651, #11691, #13387, #87065, #40304, #88189, #19295 ) ) ;
#37042=CARTESIAN_POINT ( 'NONE',  ( 136.7660003837314946, -19.25405382162758272, 6.823682607503624098 ) ) ;
#37043=CARTESIAN_POINT ( 'NONE',  ( 109.4503794976336764, -25.91221646008812840, 179.8918157521019339 ) ) ;
#37044=CARTESIAN_POINT ( 'NONE',  ( 113.5060836576900272, -28.53103057085638383, 75.54705384733995288 ) ) ;
#37045=CARTESIAN_POINT ( 'NONE',  ( 109.3680554845995232, -25.87125837001184081, 180.9222919425779708 ) ) ;
#37046=CARTESIAN_POINT ( 'NONE',  ( 163.0667039024470171, -32.29483332968611364, 342.9256252759119548 ) ) ;
#37047=CARTESIAN_POINT ( 'NONE',  ( 161.4809174648185603, -48.32844715993547169, 180.4678068554150059 ) ) ;
#37050=CARTESIAN_POINT ( 'NONE',  ( 182.5667039024459939, -22.48495420874030515, -5.074374724088000832 ) ) ;
#37051=CARTESIAN_POINT ( 'NONE',  ( 107.0664832912739968, -36.72944715994100306, 287.6356252759109680 ) ) ;
#37054=CARTESIAN_POINT ( 'NONE',  ( 80.06648329127398256, -9.029447159941060619, 4.925625275910944012 ) ) ;
#37057=VECTOR ( 'NONE', #31917, 1000.000000000000000 ) ;
#37059=ORIENTED_EDGE ( 'NONE', *, *, #50171, .T. ) ;
#37060=VERTEX_POINT ( 'NONE', #9854 ) ;
#37062=CARTESIAN_POINT ( 'NONE',  ( 112.6295607727957133, -43.21082823627408231, 107.5638483995059715 ) ) ;
#37065=CARTESIAN_POINT ( 'NONE',  ( 118.8180844208008722, -35.40729807334668777, 79.91562527591095488 ) ) ;
#37066=DIRECTION ( 'NONE',  ( 0.000000000000000000, 1.000000000000000000, 0.000000000000000000 ) ) ;
#37069=CARTESIAN_POINT ( 'NONE',  ( 115.0889047256920463, -30.61763668260735116, 175.3439586089972408 ) ) ;
#37071=CARTESIAN_POINT ( 'NONE',  ( 111.8651074766111861, -28.16866562884735004, 34.66991099019695355 ) ) ;
#37072=ORIENTED_EDGE ( 'NONE', *, *, #59216, .F. ) ;
#37073=EDGE_CURVE ( 'NONE', #33963, #68797, #22343, .T. ) ;
#37078=DIRECTION ( 'NONE',  ( 0.000000000000000000, 1.000000000000000000, 0.000000000000000000 ) ) ;
#37079=CARTESIAN_POINT ( 'NONE',  ( 112.1393456437007501, -28.01282278244291746, 115.6564586090561590 ) ) ;
#37081=TOROIDAL_SURFACE ( 'NONE', #86357, 15.84999999999999964, 0.1499999999999999944 ) ;
#37082=DIRECTION ( 'NONE',  ( -1.000000000000000000, -4.510281037539694659E-14, 0.000000000000000000 ) ) ;
#37087=EDGE_CURVE ( 'NONE', #9949, #5742, #59317, .T. ) ;
#37089=CARTESIAN_POINT ( 'NONE',  ( 109.9050689397999889, -46.77468768478704675, 72.79562527591099297 ) ) ;
#37090=VECTOR ( 'NONE', #58281, 1000.000000000000000 ) ;
#37091=VERTEX_POINT ( 'NONE', #59760 ) ;
#37094=CARTESIAN_POINT ( 'NONE',  ( 99.66770068389166681, -32.23957622922084454, 123.6985665600679738 ) ) ;
#37095=ADVANCED_FACE ( 'NONE', ( #46573 ), #74310, .F. ) ;
#37096=AXIS2_PLACEMENT_3D ( 'NONE', #80853, #46286, #39496 ) ;
#37097=CARTESIAN_POINT ( 'NONE',  ( 115.0860330880669551, -30.61390894146469677, 94.34433169324587709 ) ) ;
#37098=EDGE_CURVE ( 'NONE', #87386, #73279, #12081, .T. ) ;
#37099=CARTESIAN_POINT ( 'NONE',  ( 19.56670390244796920, -67.87844715994100397, 20.91780685541479912 ) ) ;
#37100=ORIENTED_EDGE ( 'NONE', *, *, #77867, .F. ) ;
#37102=CARTESIAN_POINT ( 'NONE',  ( 97.81942511135183338, -40.53627538877582026, 136.6376214459276639 ) ) ;
#37104=ORIENTED_EDGE ( 'NONE', *, *, #71880, .F. ) ;
#37105=EDGE_CURVE ( 'NONE', #19551, #29192, #51729, .T. ) ;
#37106=CARTESIAN_POINT ( 'NONE',  ( 103.6521623672117158, -27.97622271609356659, 166.7920594963739802 ) ) ;
#37107=DIRECTION ( 'NONE',  ( 1.025452301070035257E-14, -1.000000000000000000, 0.000000000000000000 ) ) ;
#37108=CARTESIAN_POINT ( 'NONE',  ( 109.5135917660753506, -46.88567278592853427, 128.7641967044819751 ) ) ;
#37110=CARTESIAN_POINT ( 'NONE',  ( 116.3521921512060686, -40.56741147027513250, 18.51432941078872929 ) ) ;
#37111=VECTOR ( 'NONE', #50810, 1000.000000000000000 ) ;
#37113=CIRCLE ( 'NONE', #8130, 0.9999999999999974465 ) ;
#37116=B_SPLINE_CURVE_WITH_KNOTS ( 'NONE', 3,
 ( #44378, #16696, #42578, #8543, #70314, #71667, #63951, #9430, #72107, #1278, #9881, #823, #28983, #29431, #24406, #65719, #72555, #12109 ),
 .UNSPECIFIED., .F., .F.,
 ( 4, 2, 2, 2, 2, 2, 2, 2, 4 ),
 ( 0.000000000000000000, 0.06249999997324977991, 0.1249999999464995598, 0.1874999999197493328, 0.2499999998929991196, 0.3124999998662488787, 0.3749999998394986656, 0.4374999998127484524, 0.4999999997859982392 ),
 .UNSPECIFIED. ) ;
#37117=ORIENTED_EDGE ( 'NONE', *, *, #51022, .F. ) ;
#37118=CARTESIAN_POINT ( 'NONE',  ( 97.93802767643609286, -38.39294625876189571, 199.2880903695909751 ) ) ;
#37119=CARTESIAN_POINT ( 'NONE',  ( 110.4638204314202881, -47.27238515144596676, 57.83657765686300678 ) ) ;
#37121=CARTESIAN_POINT ( 'NONE',  ( 104.6539710028518897, -47.49251396406771164, 27.38895860924395009 ) ) ;
#37122=CARTESIAN_POINT ( 'NONE',  ( 113.7646124051505154, -44.74644941934948861, 189.1299109901969757 ) ) ;
#37125=CARTESIAN_POINT ( 'NONE',  ( 116.9217636815068033, -33.22305568060546932, 110.0984824187679578 ) ) ;
#37126=DIRECTION ( 'NONE',  ( -1.000000000000000000, -4.299999999999999979E-14, -1.000000000000000078E-15 ) ) ;
#37128=LINE ( 'NONE', #17130, #69974 ) ;
#37130=DIRECTION ( 'NONE',  ( 0.000000000000000000, -1.000000000000000000, 0.000000000000000000 ) ) ;
#37131=ORIENTED_EDGE ( 'NONE', *, *, #51724, .F. ) ;
#37132=EDGE_CURVE ( 'NONE', #57830, #71968, #74963, .T. ) ;
#37133=CIRCLE ( 'NONE', #8144, 2.999999999999999112 ) ;
#37136=DIRECTION ( 'NONE',  ( 1.000000000000000000, 0.000000000000000000, 0.000000000000000000 ) ) ;
#37137=CARTESIAN_POINT ( 'NONE',  ( 117.0917326185583676, -32.07397045188266560, 59.16038718067295576 ) ) ;
#37141=DIRECTION ( 'NONE',  ( 0.000000000000000000, 0.000000000000000000, 1.000000000000000000 ) ) ;
#37142=CARTESIAN_POINT ( 'NONE',  ( 96.86520444330096780, -38.59296402346417665, 51.48229194257797303 ) ) ;
#37143=CARTESIAN_POINT ( 'NONE',  ( 97.33768507753748622, -34.07162146941007563, 111.1148373774395850 ) ) ;
#37144=CARTESIAN_POINT ( 'NONE',  ( 113.6008039948045649, -28.63430547549730676, 160.5356252759109736 ) ) ;
#37145=DIRECTION ( 'NONE',  ( 1.387778780781444492E-15, 0.000000000000000000, -1.000000000000000000 ) ) ;
#37146=PLANE ( 'NONE',  #77181 ) ;
#37148=CARTESIAN_POINT ( 'NONE',  ( 71.06648329127399677, -8.729447159940999512, 17.92562527591199739 ) ) ;
#37150=FACE_OUTER_BOUND ( 'NONE', #6789, .T. ) ;
#37151=CARTESIAN_POINT ( 'NONE',  ( 34.67381068362025331, -26.00627455219402506, 117.4678068554150485 ) ) ;
#37152=EDGE_CURVE ( 'NONE', #20562, #28735, #67038, .T. ) ;
#37153=CARTESIAN_POINT ( 'NONE',  ( 101.4014481618761181, -46.27514046166531614, 207.1622919425779514 ) ) ;
#37154=ORIENTED_EDGE ( 'NONE', *, *, #1423, .T. ) ;
#37156=CARTESIAN_POINT ( 'NONE',  ( 100.8102337077607871, -45.86971777371983450, 238.1108633711489517 ) ) ;
#37157=CARTESIAN_POINT ( 'NONE',  ( 109.7813809329710040, -47.49173451690833048, 88.78514908543493789 ) ) ;
#37163=VERTEX_POINT ( 'NONE', #18436 ) ;
#37164=ORIENTED_EDGE ( 'NONE', *, *, #82165, .F. ) ;
#37165=EDGE_LOOP ( 'NONE', ( #48817, #24572, #7768, #16813, #2478 ) ) ;
#37166=CARTESIAN_POINT ( 'NONE',  ( 29.56670390244797630, -67.87844715994100397, 20.91780685541479912 ) ) ;
#37167=CARTESIAN_POINT ( 'NONE',  ( 110.2773916389477478, -46.62487827714361543, 8.827053847339950465 ) ) ;
#37168=DIRECTION ( 'NONE',  ( 4.299999999999999979E-14, -1.000000000000000000, 0.000000000000000000 ) ) ;
#37170=CARTESIAN_POINT ( 'NONE',  ( 182.4202572930400379, -33.70561438051982606, 342.9256252759109884 ) ) ;
#37174=CARTESIAN_POINT ( 'NONE',  ( 98.10212974493634874, -35.44374275293071008, 225.6476579233149948 ) ) ;
#37175=ORIENTED_EDGE ( 'NONE', *, *, #29678, .F. ) ;
#37176=VERTEX_POINT ( 'NONE', #45668 ) ;
#37179=AXIS2_PLACEMENT_3D ( 'NONE', #89780, #61155, #20725 ) ;
#37181=DIRECTION ( 'NONE',  ( -1.000000000000000078E-15, 1.000000000000000083E-30, 1.000000000000000000 ) ) ;
#37183=FACE_OUTER_BOUND ( 'NONE', #83764, .T. ) ;
#37184=CARTESIAN_POINT ( 'NONE',  ( 97.83217745605955429, -40.05230289513912822, 262.6013395616248545 ) ) ;
#37186=DIRECTION ( 'NONE',  ( 0.000000000000000000, 0.000000000000000000, 1.000000000000000000 ) ) ;
#37187=CARTESIAN_POINT ( 'NONE',  ( 102.6819511611811180, -27.33185899950651887, 131.4118157521009778 ) ) ;
#37188=ADVANCED_FACE ( 'NONE', ( #23398 ), #22489, .T. ) ;
#37189=CARTESIAN_POINT ( 'NONE',  ( 87.06648329127403940, -54.72944906728955061, -4.824374724089049771 ) ) ;
#37191=ADVANCED_FACE ( 'NONE', ( #15220 ), #30633, .F. ) ;
#37192=CARTESIAN_POINT ( 'NONE',  ( 77.38348569455061465, -36.12003772029492410, 3.004064388423448584 ) ) ;
#37193=VERTEX_POINT ( 'NONE', #36565 ) ;
#37194=VECTOR ( 'NONE', #11420, 1000.000000000000000 ) ;
#37195=CARTESIAN_POINT ( 'NONE',  ( 41.56648329127399677, -9.303447159940999356, 201.0426252759120018 ) ) ;
#37196=CARTESIAN_POINT ( 'NONE',  ( 104.8541313898159757, -44.58662387026339502, 20.17666179816296435 ) ) ;
#37197=ADVANCED_FACE ( 'NONE', ( #86058 ), #2931, .F. ) ;
#37198=CARTESIAN_POINT ( 'NONE',  ( 136.8164806451551669, -18.72944715939129523, 6.749772901088581634 ) ) ;
#37199=AXIS2_PLACEMENT_3D ( 'NONE', #61063, #47869, #27003 ) ;
#37201=ADVANCED_FACE ( 'NONE', ( #37004 ), #3900, .F. ) ;
#37205=DIRECTION ( 'NONE',  ( 0.000000000000000000, 0.000000000000000000, -1.000000000000000000 ) ) ;
#37207=CARTESIAN_POINT ( 'NONE',  ( 118.8429430416104680, -35.40450127974935413, 83.91562527591095488 ) ) ;
#37209=CARTESIAN_POINT ( 'NONE',  ( 100.5114817196218411, -42.97801697403279775, 36.34289601855395091 ) ) ;
#37210=CARTESIAN_POINT ( 'NONE',  ( 109.2888275139916203, -46.51057382167308418, 88.75361627338941162 ) ) ;
#37211=CARTESIAN_POINT ( 'NONE',  ( 116.0163176773587708, -41.35234337494321721, 89.87872616303998541 ) ) ;
#37213=CARTESIAN_POINT ( 'NONE',  ( 130.5667039024480118, -34.21194715994094082, 239.5838068554170377 ) ) ;
#37214=CARTESIAN_POINT ( 'NONE',  ( 100.4515265478786574, -44.84261285976553779, 8.032768133053981074 ) ) ;
#37216=ORIENTED_EDGE ( 'NONE', *, *, #31686, .T. ) ;
#37217=FACE_OUTER_BOUND ( 'NONE', #56607, .T. ) ;
#37219=CARTESIAN_POINT ( 'NONE',  ( 99.39016829297771949, -27.63593621212785933, 146.6356252759109395 ) ) ;
#37222=ORIENTED_EDGE ( 'NONE', *, *, #13138, .T. ) ;
#37223=ORIENTED_EDGE ( 'NONE', *, *, #89391, .F. ) ;
#37224=FACE_OUTER_BOUND ( 'NONE', #82108, .T. ) ;
#37225=LINE ( 'NONE', #30854, #14492 ) ;
#37226=CARTESIAN_POINT ( 'NONE',  ( 98.91665286848242999, -30.31703347128389225, 200.8080062282919869 ) ) ;
#37227=DIRECTION ( 'NONE',  ( -2.900000000000000265E-14, 2.000000000000000155E-15, -1.000000000000000000 ) ) ;
#37229=CYLINDRICAL_SURFACE ( 'NONE', #89680, 2.517500000000005844 ) ;
#37230=CARTESIAN_POINT ( 'NONE',  ( 100.4653332305737905, -44.82571634032018437, 8.032768133053981074 ) ) ;
#37231=DIRECTION ( 'NONE',  ( -1.000000000000000000, -1.000000000000000078E-15, -1.000000000000000078E-15 ) ) ;
#37233=CARTESIAN_POINT ( 'NONE',  ( 97.53183428581748160, -39.74892342586570493, 172.5705140066459933 ) ) ;
#37235=LINE ( 'NONE', #84958, #46112 ) ;
#37236=ADVANCED_FACE ( 'NONE', ( #44241 ), #77898, .F. ) ;
#37238=VECTOR ( 'NONE', #77306, 1000.000000000000000 ) ;
#37239=CIRCLE ( 'NONE', #11156, 2.116999999999993776 ) ;
#37240=CARTESIAN_POINT ( 'NONE',  ( 81.48476992307091393, -21.08750326150235210, 1.944748881532749163 ) ) ;
#37242=CARTESIAN_POINT ( 'NONE',  ( 83.73314995793998605, 12.92155284005730387, 355.9756252759109998 ) ) ;
#37243=CARTESIAN_POINT ( 'NONE',  ( 97.49318720818078532, -40.89074837367932957, 231.6527681330539679 ) ) ;
#37245=VECTOR ( 'NONE', #86693, 999.9999999999998863 ) ;
#37246=EDGE_CURVE ( 'NONE', #21321, #27069, #80746, .T. ) ;
#37247=FACE_BOUND ( 'NONE', #5883, .T. ) ;
#37248=CYLINDRICAL_SURFACE ( 'NONE', #37426, 1.499999999999987788 ) ;
#37249=CARTESIAN_POINT ( 'NONE',  ( 113.7727705757230297, -31.39298644294678908, 243.7838483995059562 ) ) ;
#37251=CARTESIAN_POINT ( 'NONE',  ( 97.79189512308838061, -32.01662636557821173, 46.95276813305393659 ) ) ;
#37252=DIRECTION ( 'NONE',  ( 0.000000000000000000, 0.000000000000000000, -1.000000000000000000 ) ) ;
#37253=CARTESIAN_POINT ( 'NONE',  ( 101.4772741282170472, -27.87691040622789274, 110.5241967044819944 ) ) ;
#37254=ORIENTED_EDGE ( 'NONE', *, *, #66289, .F. ) ;
#37255=CARTESIAN_POINT ( 'NONE',  ( 131.7676426598729904, -20.23887630718033392, 7.293197373621852719 ) ) ;
#37257=LINE ( 'NONE', #85434, #11635 ) ;
#37258=DIRECTION ( 'NONE',  ( 0.000000000000000000, 0.000000000000000000, -1.000000000000000000 ) ) ;
#37260=DIRECTION ( 'NONE',  ( -1.000000000000000000, 0.000000000000000000, 0.000000000000000000 ) ) ;
#37262=DIRECTION ( 'NONE',  ( -0.000000000000000000, -0.000000000000000000, -1.000000000000000000 ) ) ;
#37263=CARTESIAN_POINT ( 'NONE',  ( 41.56648329127398966, -27.82844715994070484, 78.92562527591199739 ) ) ;
#37264=CIRCLE ( 'NONE', #42999, 2.517499999999998739 ) ;
#37265=CYLINDRICAL_SURFACE ( 'NONE', #19101, 3.299999999999997158 ) ;
#37269=CARTESIAN_POINT ( 'NONE',  ( 117.3606796971436523, -32.63983085838949449, 99.13943479972098771 ) ) ;
#37270=CARTESIAN_POINT ( 'NONE',  ( 87.06648329127403940, -54.72944906728955061, -4.824374724089049771 ) ) ;
#37271=DIRECTION ( 'NONE',  ( -0.7071067811865436870, 0.7071067811865513475, -7.071067811865430960E-16 ) ) ;
#37272=LINE ( 'NONE', #71361, #4990 ) ;
#37274=DIRECTION ( 'NONE',  ( 0.000000000000000000, 0.000000000000000000, -1.000000000000000000 ) ) ;
#37275=FACE_OUTER_BOUND ( 'NONE', #72193, .T. ) ;
#37277=DIRECTION ( 'NONE',  ( -1.000000000000000000, 0.000000000000000000, 0.000000000000000000 ) ) ;
#37278=CARTESIAN_POINT ( 'NONE',  ( 107.0664832912739968, -8.350947159940998787, 330.8831252759119934 ) ) ;
#37279=DIRECTION ( 'NONE',  ( 0.000000000000000000, 0.000000000000000000, 1.000000000000000000 ) ) ;
#37281=VERTEX_POINT ( 'NONE', #8412 ) ;
#37282=B_SPLINE_CURVE_WITH_KNOTS ( 'NONE', 3,
 ( #72661, #53056, #18126, #33102, #74442, #52614, #4508, #18575, #86738, #24509, #73991, #53511, #12218, #60343, #66724, #31755, #60799, #4056, #87625, #52173, #25389, #39906, #80376, #10869, #79935, #17691, #88532, #73091, #38567, #46255, #10428 ),
 .UNSPECIFIED., .F., .F.,
 ( 4, 2, 2, 1, 2, 2, 2, 2, 2, 2, 2, 1, 1, 2, 2, 2, 4 ),
 ( 0.000000000000000000, 0.1249999999999873990, 0.1874999999999810985, 0.2187499999999738542, 0.2343749999999741318, 0.2499999999999744094, 0.3749999999999857336, 0.4374999999999914513, 0.4999999999999972244, 0.6250000000000086597, 0.6875000000000128786, 0.7187500000000148770, 0.7343750000000159872, 0.7421875000000164313, 0.7500000000000168754, 0.8750000000000083267, 1.000000000000000000 ),
 .UNSPECIFIED. ) ;
#37283=DIRECTION ( 'NONE',  ( -6.831565154159360295E-14, 1.000000000000000000, 0.000000000000000000 ) ) ;
#37284=CARTESIAN_POINT ( 'NONE',  ( 104.0088209277215867, -27.43890701233904394, 161.3299109901969643 ) ) ;
#37286=DIRECTION ( 'NONE',  ( 1.000000000000000000, 0.000000000000000000, 1.261617073437676668E-15 ) ) ;
#37288=CARTESIAN_POINT ( 'NONE',  ( 113.6564618781686136, -45.68400828401183844, 29.08133956162495082 ) ) ;
#37289=FACE_OUTER_BOUND ( 'NONE', #43445, .T. ) ;
#37290=CARTESIAN_POINT ( 'NONE',  ( 98.38057243704078303, -41.69553627151279329, 51.73981168366587013 ) ) ;
#37291=EDGE_CURVE ( 'NONE', #9592, #48907, #34299, .T. ) ;
#37292=DIRECTION ( 'NONE',  ( 0.000000000000000000, 0.000000000000000000, -1.000000000000000000 ) ) ;
#37293=FACE_OUTER_BOUND ( 'NONE', #12243, .T. ) ;
#37294=EDGE_CURVE ( 'NONE', #8449, #51823, #45885, .T. ) ;
#37295=AXIS2_PLACEMENT_3D ( 'NONE', #37046, #2538, #58374 ) ;
#37296=VECTOR ( 'NONE', #70294, 1000.000000000000000 ) ;
#37297=CARTESIAN_POINT ( 'NONE',  ( 104.5747221139661320, -26.66317121150808944, 240.2575300378159682 ) ) ;
#37298=VERTEX_POINT ( 'NONE', #71094 ) ;
#37300=CARTESIAN_POINT ( 'NONE',  ( 115.8619398590553260, -35.64860379657582712, 190.3558690201829506 ) ) ;
#37302=AXIS2_PLACEMENT_3D ( 'NONE', #41313, #69042, #43103 ) ;
#37303=CARTESIAN_POINT ( 'NONE',  ( 114.9896934147946013, -32.69399539773264252, 40.63301187732598407 ) ) ;
#37306=DIRECTION ( 'NONE',  ( 0.9825752044328147639, 0.1858654557302462929, 0.000000000000000000 ) ) ;
#37307=EDGE_CURVE ( 'NONE', #7607, #63584, #64267, .T. ) ;
#37308=FACE_OUTER_BOUND ( 'NONE', #10460, .T. ) ;
#37309=EDGE_LOOP ( 'NONE', ( #17724, #73438 ) ) ;
#37311=FACE_OUTER_BOUND ( 'NONE', #38079, .T. ) ;
#37312=ADVANCED_FACE ( 'NONE', ( #2490, #45561 ), #66027, .T. ) ;
#37313=CARTESIAN_POINT ( 'NONE',  ( 101.6619702986602505, -45.61876124157287649, 247.1413395616249602 ) ) ;
#37315=VERTEX_POINT ( 'NONE', #74204 ) ;
#37316=CARTESIAN_POINT ( 'NONE',  ( 108.3334480867816296, -46.73485935508681166, 82.67729194192742170 ) ) ;
#37318=DIRECTION ( 'NONE',  ( 0.000000000000000000, 0.000000000000000000, -1.000000000000000000 ) ) ;
#37320=DIRECTION ( 'NONE',  ( 1.000000000000000078E-15, 1.000000000000000083E-30, -1.000000000000000000 ) ) ;
#37321=AXIS2_PLACEMENT_3D ( 'NONE', #61790, #89529, #54960 ) ;
#37322=CARTESIAN_POINT ( 'NONE',  ( 117.4022237771661281, -37.57280582802024327, 34.77372051400595865 ) ) ;
#37323=CARTESIAN_POINT ( 'NONE',  ( 90.44969454456422397, -56.64645651782490177, 239.5838068554174356 ) ) ;
#37326=CARTESIAN_POINT ( 'NONE',  ( 111.9491823805485922, -27.46919719833538309, 55.68991099019693536 ) ) ;
#37327=CARTESIAN_POINT ( 'NONE',  ( 72.31648329127399677, -9.833000550534366724, -5.074374724089063982 ) ) ;
#37328=CARTESIAN_POINT ( 'NONE',  ( 105.7763445623522500, -26.38427570067176831, 270.1756252759109884 ) ) ;
#37330=DIRECTION ( 'NONE',  ( 0.7071067811865692221, 0.7071067811865259234, 7.071067811865685367E-16 ) ) ;
#37332=CARTESIAN_POINT ( 'NONE',  ( 36.23715912545424089, -47.82818131006125384, 300.4678068554150059 ) ) ;
#37333=CARTESIAN_POINT ( 'NONE',  ( 98.90209562501077301, -37.38172185807169967, 99.20809036959194316 ) ) ;
#37334=CARTESIAN_POINT ( 'NONE',  ( 97.74302678327005367, -41.52030872683848628, 192.7041967044819728 ) ) ;
#37336=DIRECTION ( 'NONE',  ( 0.9963424814100688698, -0.08544974978094983797, 0.000000000000000000 ) ) ;
#37338=VECTOR ( 'NONE', #80791, 1000.000000000000000 ) ;
#37339=DIRECTION ( 'NONE',  ( 0.000000000000000000, 0.000000000000000000, -1.000000000000000000 ) ) ;
#37340=ORIENTED_EDGE ( 'NONE', *, *, #43316, .F. ) ;
#37342=EDGE_LOOP ( 'NONE', ( #85563, #21097, #5726, #40589 ) ) ;
#37343=DIRECTION ( 'NONE',  ( 2.900000000000000265E-14, -2.000000000000000155E-15, 1.000000000000000000 ) ) ;
#37344=EDGE_LOOP ( 'NONE', ( #45479, #88849, #62081, #67271 ) ) ;
#37345=ORIENTED_EDGE ( 'NONE', *, *, #10852, .T. ) ;
#37347=EDGE_CURVE ( 'NONE', #69712, #23413, #39665, .T. ) ;
#37348=CARTESIAN_POINT ( 'NONE',  ( 97.75828744068094522, -40.38463776613766498, 42.62423351867927579 ) ) ;
#37349=CARTESIAN_POINT ( 'NONE',  ( 112.6189512620115778, -30.20087909038965535, 138.9381341137909658 ) ) ;
#37350=CARTESIAN_POINT ( 'NONE',  ( 96.24499046374883449, -34.36497383161641039, 256.1432443235299843 ) ) ;
#37351=DIRECTION ( 'NONE',  ( 0.000000000000000000, 0.000000000000000000, -1.000000000000000000 ) ) ;
#37352=VERTEX_POINT ( 'NONE', #17884 ) ;
#37353=CARTESIAN_POINT ( 'NONE',  ( 103.2779182987110005, -27.47489285962728545, 136.3856765722742352 ) ) ;
#37356=CYLINDRICAL_SURFACE ( 'NONE', #66200, 9.999999999999998224 ) ;
#37357=DIRECTION ( 'NONE',  ( 0.000000000000000000, 0.000000000000000000, 1.000000000000000000 ) ) ;
#37361=VECTOR ( 'NONE', #55566, 999.9999999999998863 ) ;
#37362=EDGE_CURVE ( 'NONE', #30460, #49742, #66475, .T. ) ;
#37363=CARTESIAN_POINT ( 'NONE',  ( 106.8364329414440874, -47.15221585624544787, 272.5584824187680510 ) ) ;
#37364=CARTESIAN_POINT ( 'NONE',  ( 116.5137666388868780, -32.21926627522912412, 15.18133956162492915 ) ) ;
#37366=CARTESIAN_POINT ( 'NONE',  ( 116.3212776292293995, -32.94146857471267253, 120.1356252759109537 ) ) ;
#37368=CYLINDRICAL_SURFACE ( 'NONE', #34044, 0.4999999999999933387 ) ;
#37369=DIRECTION ( 'NONE',  ( 0.000000000000000000, 0.000000000000000000, 1.000000000000000000 ) ) ;
#37371=CARTESIAN_POINT ( 'NONE',  ( 131.3333327974764870, -37.08363404521318785, 6.775960187534245449 ) ) ;
#37372=CIRCLE ( 'NONE', #70779, 0.5000000000000004441 ) ;
#37373=FACE_OUTER_BOUND ( 'NONE', #3873, .T. ) ;
#37376=CARTESIAN_POINT ( 'NONE',  ( 141.0667039024479834, -48.82844715994099971, 310.9178068554150514 ) ) ;
#37379=CARTESIAN_POINT ( 'NONE',  ( 104.5828969173064849, -26.58150870143000688, 285.2670538473396391 ) ) ;
#37380=CARTESIAN_POINT ( 'NONE',  ( 101.9720301123653883, -46.53865341315756154, 163.1832443235299763 ) ) ;
#37381=CARTESIAN_POINT ( 'NONE',  ( 110.5624684038761814, -46.61161715960605534, 33.84705384733993583 ) ) ;
#37383=CIRCLE ( 'NONE', #32958, 11.45913725231036118 ) ;
#37384=CARTESIAN_POINT ( 'NONE',  ( 172.5667039024478413, -36.32844715993500273, 249.9678068554149775 ) ) ;
#37385=LINE ( 'NONE', #72797, #79151 ) ;
#37386=FACE_OUTER_BOUND ( 'NONE', #34293, .T. ) ;
#37388=EDGE_CURVE ( 'NONE', #48723, #54028, #26052, .T. ) ;
#37390=CARTESIAN_POINT ( 'NONE',  ( 188.5667039024480971, -42.82844715993431350, 293.2178068554150059 ) ) ;
#37392=CARTESIAN_POINT ( 'NONE',  ( 116.4719273984280790, -32.36179259691363796, 55.16038718067301261 ) ) ;
#37393=CARTESIAN_POINT ( 'NONE',  ( 116.3135867418571650, -32.94878190598771539, 189.1356252759109680 ) ) ;
#37396=CARTESIAN_POINT ( 'NONE',  ( 98.55548742614595881, -30.74683778668247669, 201.8384824187679385 ) ) ;
#37397=LINE ( 'NONE', #36055, #27974 ) ;
#37398=CYLINDRICAL_SURFACE ( 'NONE', #66676, 10.04999999999999361 ) ;
#37399=DIRECTION ( 'NONE',  ( 0.7071067811985215501, -0.7071067811745735954, 0.000000000000000000 ) ) ;
#37401=PLANE ( 'NONE',  #26940 ) ;
#37403=CARTESIAN_POINT ( 'NONE',  ( 112.5642669466485586, -45.09754247072631728, 98.03899555326725590 ) ) ;
#37404=CARTESIAN_POINT ( 'NONE',  ( 97.33998274022607688, -37.75834089694785689, 126.4099109901969626 ) ) ;
#37405=ORIENTED_EDGE ( 'NONE', *, *, #54042, .T. ) ;
#37407=CARTESIAN_POINT ( 'NONE',  ( 98.73617028912649118, -32.38405755445656808, 87.36348806780198117 ) ) ;
#37408=DIRECTION ( 'NONE',  ( -1.000000000000000000, -6.814610998690690172E-14, -1.000000000000000078E-15 ) ) ;
#37409=CARTESIAN_POINT ( 'NONE',  ( 114.9410966442421795, -29.98191058901456074, 225.4022919425769658 ) ) ;
#37410=CARTESIAN_POINT ( 'NONE',  ( 83.96770390244800808, -18.82844715994099971, 239.5838068554169809 ) ) ;
#37411=DIRECTION ( 'NONE',  ( 0.7071067811874389708, -0.7071067811856560636, 0.000000000000000000 ) ) ;
#37412=CARTESIAN_POINT ( 'NONE',  ( 106.5462518941686909, -24.40236651281373526, 322.0356252759110021 ) ) ;
#37413=B_SPLINE_CURVE_WITH_KNOTS ( 'NONE', 3,
 ( #53839, #27068, #54738, #67492, #81158, #88858, #46589, #81609, #80699, #73867 ),
 .UNSPECIFIED., .F., .F.,
 ( 4, 2, 2, 2, 4 ),
 ( 0.4999378446604081927, 0.5499671847885604370, 0.5999965249167127368, 0.6500258650448649256, 0.7000552051730172254 ),
 .UNSPECIFIED. ) ;
#37415=EDGE_CURVE ( 'NONE', #59219, #9306, #46108, .T. ) ;
#37419=CARTESIAN_POINT ( 'NONE',  ( 114.2383551682310525, -44.26553795382362466, 158.1813395616249807 ) ) ;
#37421=VERTEX_POINT ( 'NONE', #61896 ) ;
#37422=EDGE_CURVE ( 'NONE', #2509, #65246, #58048, .T. ) ;
#37423=CARTESIAN_POINT ( 'NONE',  ( 193.0371591254584018, -47.82818131005411999, 300.4678068554149490 ) ) ;
#37424=CARTESIAN_POINT ( 'NONE',  ( 77.48363092588481038, -17.78502016655210838, 2.871594975604033539 ) ) ;
#37425=ADVANCED_FACE ( 'NONE', ( #11369, #74942 ), #80875, .F. ) ;
#37426=AXIS2_PLACEMENT_3D ( 'NONE', #51292, #3177, #1390 ) ;
#37429=CARTESIAN_POINT ( 'NONE',  ( 114.9986391697397607, -34.80314782265816831, 206.8338046553059826 ) ) ;
#37430=AXIS2_PLACEMENT_3D ( 'NONE', #32570, #60270, #53437 ) ;
#37431=AXIS2_PLACEMENT_3D ( 'NONE', #30099, #52730, #58247 ) ;
#37433=CARTESIAN_POINT ( 'NONE',  ( 109.6058900474308757, -26.58167301968400764, 199.8813395616249977 ) ) ;
#37435=VERTEX_POINT ( 'NONE', #45859 ) ;
#37436=EDGE_LOOP ( 'NONE', ( #35060, #74487, #31480, #88100 ) ) ;
#37437=ORIENTED_EDGE ( 'NONE', *, *, #17484, .F. ) ;
#37439=CARTESIAN_POINT ( 'NONE',  ( 194.0371591254575492, -24.42818131005407167, 117.4678068554150627 ) ) ;
#37440=DIRECTION ( 'NONE',  ( -0.7071067811571960515, 0.7071067812158990940, 0.000000000000000000 ) ) ;
#37441=CARTESIAN_POINT ( 'NONE',  ( 131.7155263566292547, -35.29868341352990768, 7.242354772856963052 ) ) ;
#37442=CARTESIAN_POINT ( 'NONE',  ( 111.1445474647120051, -44.63080920614596181, 269.3872975916115706 ) ) ;
#37443=AXIS2_PLACEMENT_3D ( 'NONE', #38569, #65399, #87187 ) ;
#37444=LINE ( 'NONE', #23824, #17336 ) ;
#37446=AXIS2_PLACEMENT_3D ( 'NONE', #24023, #38085, #16756 ) ;
#37447=VECTOR ( 'NONE', #32524, 1000.000000000000000 ) ;
#37448=CARTESIAN_POINT ( 'NONE',  ( 102.4743188866377039, -43.40982696052134315, 9.635625275910939536 ) ) ;
#37450=ORIENTED_EDGE ( 'NONE', *, *, #36654, .F. ) ;
#37451=VERTEX_POINT ( 'NONE', #18632 ) ;
#37452=CARTESIAN_POINT ( 'NONE',  ( 116.7497567485386156, -34.15833269763940194, 114.0330597662738938 ) ) ;
#37453=VERTEX_POINT ( 'NONE', #33153 ) ;
#37454=ORIENTED_EDGE ( 'NONE', *, *, #89619, .F. ) ;
#37455=EDGE_CURVE ( 'NONE', #52482, #29231, #46759, .T. ) ;
#37456=AXIS2_PLACEMENT_3D ( 'NONE', #22373, #50050, #87278 ) ;
#37457=CARTESIAN_POINT ( 'NONE',  ( 109.1520131464112069, -27.24676858702523674, 29.32670554236194249 ) ) ;
#37458=CARTESIAN_POINT ( 'NONE',  ( 113.6281634912633223, -45.65356023013480780, 183.0689586092439640 ) ) ;
#37459=CARTESIAN_POINT ( 'NONE',  ( 117.1882713363357169, -39.28166824301213467, 123.6299109901969615 ) ) ;
#37461=CARTESIAN_POINT ( 'NONE',  ( 116.6057436952887372, -40.93480069938575383, 249.4956252759109532 ) ) ;
#37462=CARTESIAN_POINT ( 'NONE',  ( 117.0609360745339984, -38.08016024203720207, 99.71977895578028495 ) ) ;
#37463=CARTESIAN_POINT ( 'NONE',  ( 115.8240617383016797, -31.72764908460863609, 125.2400077891570902 ) ) ;
#37464=CARTESIAN_POINT ( 'NONE',  ( 141.8164832912739826, -9.833000550534297446, 14.92562527591100618 ) ) ;
#37466=EDGE_LOOP ( 'NONE', ( #56461, #14552, #8023, #23452 ) ) ;
#37467=AXIS2_PLACEMENT_3D ( 'NONE', #10062, #37318, #65022 ) ;
#37468=AXIS2_PLACEMENT_3D ( 'NONE', #30859, #80808, #17237 ) ;
#37469=CARTESIAN_POINT ( 'NONE',  ( 96.63001237737263693, -35.53283987767252228, 206.2356252759109623 ) ) ;
#37470=ORIENTED_EDGE ( 'NONE', *, *, #40901, .F. ) ;
#37471=ADVANCED_FACE ( 'NONE', ( #12720 ), #59943, .T. ) ;
#37472=CARTESIAN_POINT ( 'NONE',  ( 102.9670468844020235, -26.46427747797763175, 175.3908633711489813 ) ) ;
#37473=CARTESIAN_POINT ( 'NONE',  ( 106.5580495140764015, -24.23977772305836709, 322.9014499992877631 ) ) ;
#37476=EDGE_CURVE ( 'NONE', #76957, #72320, #60848, .T. ) ;
#37479=CARTESIAN_POINT ( 'NONE',  ( 96.91023542590100703, -30.67149048741791262, 276.8984824187680829 ) ) ;
#37480=DIRECTION ( 'NONE',  ( 0.000000000000000000, 0.000000000000000000, 1.000000000000000000 ) ) ;
#37482=CARTESIAN_POINT ( 'NONE',  ( 182.5667039024469886, -33.35206098992650681, -5.074374724088000832 ) ) ;
#37486=EDGE_CURVE ( 'NONE', #84622, #85514, #88071, .T. ) ;
#37487=DIRECTION ( 'NONE',  ( -4.237773401492740281E-14, 1.000000000000000000, 0.000000000000000000 ) ) ;
#37488=CARTESIAN_POINT ( 'NONE',  ( 108.7127106255978219, -44.55865754719168592, 195.5838068554167819 ) ) ;
#37489=EDGE_LOOP ( 'NONE', ( #87161, #33090 ) ) ;
#37490=CIRCLE ( 'NONE', #59254, 0.5000000000000004441 ) ;
#37491=EDGE_CURVE ( 'NONE', #81899, #57373, #31805, .T. ) ;
#37492=CARTESIAN_POINT ( 'NONE',  ( 135.1909174281126980, -21.23916151080255688, 8.028235474617199330 ) ) ;
#37493=CARTESIAN_POINT ( 'NONE',  ( 116.8159443494545826, -40.58124828358739222, 193.5270538473389479 ) ) ;
#37494=CARTESIAN_POINT ( 'NONE',  ( 117.0915230934440103, -32.07406775014006683, 55.16038718067301261 ) ) ;
#37495=CARTESIAN_POINT ( 'NONE',  ( 117.9780035659441495, -34.69567636304840619, 199.9851490854349549 ) ) ;
#37498=CARTESIAN_POINT ( 'NONE',  ( 165.9667039024473922, -26.71338133338714016, 313.9678068554149490 ) ) ;
#37500=DIRECTION ( 'NONE',  ( -0.7071067811567310901, 0.7071067812163639443, 0.000000000000000000 ) ) ;
#37501=CARTESIAN_POINT ( 'NONE',  ( 34.67381068360426610, -28.98061976759052527, 313.9678068554150059 ) ) ;
#37502=ORIENTED_EDGE ( 'NONE', *, *, #85077, .T. ) ;
#37503=EDGE_CURVE ( 'NONE', #16163, #42342, #85170, .T. ) ;
#37509=ORIENTED_EDGE ( 'NONE', *, *, #22979, .F. ) ;
#37511=CARTESIAN_POINT ( 'NONE',  ( 107.5061752250017264, -28.17031325930595642, 94.45813411379100444 ) ) ;
#37514=ORIENTED_EDGE ( 'NONE', *, *, #2277, .T. ) ;
#37515=CARTESIAN_POINT ( 'NONE',  ( 102.5676158828201778, -27.34920955258912301, 91.43276813305395478 ) ) ;
#37518=AXIS2_PLACEMENT_3D ( 'NONE', #89256, #40182, #26565 ) ;
#37521=AXIS2_PLACEMENT_3D ( 'NONE', #11786, #53525, #10882 ) ;
#37522=CARTESIAN_POINT ( 'NONE',  ( 97.30224646447496184, -33.23681714893609751, 26.06514908543594444 ) ) ;
#37524=ORIENTED_EDGE ( 'NONE', *, *, #84167, .F. ) ;
#37525=ORIENTED_EDGE ( 'NONE', *, *, #84078, .F. ) ;
#37526=DIRECTION ( 'NONE',  ( 0.000000000000000000, 0.000000000000000000, -1.000000000000000000 ) ) ;
#37527=LINE ( 'NONE', #86572, #43253 ) ;
#37530=CARTESIAN_POINT ( 'NONE',  ( 179.7974245136210527, -36.32844715993471141, 117.4678068554150627 ) ) ;
#37532=B_SPLINE_CURVE_WITH_KNOTS ( 'NONE', 3,
 ( #75017, #19164, #73670, #88664, #47741, #19604, #74568, #60936, #12808, #4636, #89103, #66856, #46838, #4188, #67296, #74125, #59575, #33237 ),
 .UNSPECIFIED., .F., .F.,
 ( 4, 2, 2, 2, 2, 2, 2, 2, 4 ),
 ( 0.4999597063510836659, 0.5624647430571981799, 0.6249697797633126939, 0.6874748164694273189, 0.7499798531755418329, 0.8124848898816563469, 0.8749899265877709720, 0.9374949632938854860, 1.000000000000000000 ),
 .UNSPECIFIED. ) ;
#37533=VECTOR ( 'NONE', #56196, 1000.000000000000000 ) ;
#37534=DIRECTION ( 'NONE',  ( 0.000000000000000000, 0.000000000000000000, 1.000000000000000000 ) ) ;
#37536=CARTESIAN_POINT ( 'NONE',  ( 96.20032699425225076, -38.62430069186631698, 46.45181575210094138 ) ) ;
#37541=EDGE_CURVE ( 'NONE', #12734, #45673, #48876, .T. ) ;
#37543=CARTESIAN_POINT ( 'NONE',  ( 105.4193742293517460, -27.59801994936882252, 123.0366617981629673 ) ) ;
#37544=VECTOR ( 'NONE', #51685, 1000.000000000000000 ) ;
#37545=CARTESIAN_POINT ( 'NONE',  ( 99.09444862205589288, -30.55209741447661287, 95.80246077065771715 ) ) ;
#37546=DIRECTION ( 'NONE',  ( -6.831565154159360295E-14, 1.000000000000000000, 0.000000000000000000 ) ) ;
#37548=ORIENTED_EDGE ( 'NONE', *, *, #15262, .T. ) ;
#37549=CARTESIAN_POINT ( 'NONE',  ( 100.8874983018639426, -44.70024987288356755, 137.0511845485476101 ) ) ;
#37550=ORIENTED_EDGE ( 'NONE', *, *, #1404, .F. ) ;
#37552=CARTESIAN_POINT ( 'NONE',  ( 115.5682375124590635, -39.22913789569613385, 180.0301547344689936 ) ) ;
#37553=VECTOR ( 'NONE', #44607, 1000.000000000000000 ) ;
#37555=CARTESIAN_POINT ( 'NONE',  ( 114.1899296859532171, -45.21130890035909999, 144.1203871806729637 ) ) ;
#37557=CARTESIAN_POINT ( 'NONE',  ( 97.81503796907703929, -40.52560807623309813, 16.63632852797828221 ) ) ;
#37558=VECTOR ( 'NONE', #40509, 1000.000000000000000 ) ;
#37559=ORIENTED_EDGE ( 'NONE', *, *, #43340, .T. ) ;
#37560=CIRCLE ( 'NONE', #62183, 1.000000000000000888 ) ;
#37563=CARTESIAN_POINT ( 'NONE',  ( 107.4574165340472263, -45.37514529517124373, 190.4185665600669779 ) ) ;
#37564=VECTOR ( 'NONE', #21928, 1000.000000000000000 ) ;
#37565=CARTESIAN_POINT ( 'NONE',  ( 111.9392231810069944, -27.48808525092397304, 59.68991099019693536 ) ) ;
#37566=EDGE_LOOP ( 'NONE', ( #8396, #49758, #20154, #54831 ) ) ;
#37567=CARTESIAN_POINT ( 'NONE',  ( 101.1541078795467996, -28.12664281037970682, 50.55562527591095545 ) ) ;
#37569=DIRECTION ( 'NONE',  ( 0.000000000000000000, 0.000000000000000000, 1.000000000000000000 ) ) ;
#37570=CARTESIAN_POINT ( 'NONE',  ( 107.7349035034188489, -25.28961927740925830, 323.0034242383203491 ) ) ;
#37571=CARTESIAN_POINT ( 'NONE',  ( 117.1259760753171548, -33.86829196857838298, 145.0470538473399529 ) ) ;
#37572=CARTESIAN_POINT ( 'NONE',  ( 117.0718954846165616, -35.46248235265727544, 263.9272919428643718 ) ) ;
#37576=ORIENTED_EDGE ( 'NONE', *, *, #45869, .F. ) ;
#37577=CIRCLE ( 'NONE', #57864, 2.117000000000007987 ) ;
#37578=DIRECTION ( 'NONE',  ( 0.000000000000000000, 0.000000000000000000, -1.000000000000000000 ) ) ;
#37580=ORIENTED_EDGE ( 'NONE', *, *, #84154, .T. ) ;
#37583=CARTESIAN_POINT ( 'NONE',  ( 115.0227918137121037, -43.52084328818016701, 63.26419670448196797 ) ) ;
#37584=DIRECTION ( 'NONE',  ( 4.194175870806139918E-14, -1.000000000000000000, 0.000000000000000000 ) ) ;
#37585=EDGE_CURVE ( 'NONE', #5375, #20111, #32247, .T. ) ;
#37589=CARTESIAN_POINT ( 'NONE',  ( 117.3137205126584348, -38.32096045344801638, 68.69181575210198787 ) ) ;
#37590=CARTESIAN_POINT ( 'NONE',  ( 182.3467384525658588, -36.02818131005238200, 237.4678068554150059 ) ) ;
#37591=CARTESIAN_POINT ( 'NONE',  ( 113.5515132932710713, -44.90922781482908732, 164.1099109901969655 ) ) ;
#37593=CARTESIAN_POINT ( 'NONE',  ( 177.0371591254545649, -48.62818131005479927, 180.4678068554150059 ) ) ;
#37595=CIRCLE ( 'NONE', #23092, 1.000000000000000888 ) ;
#37599=CYLINDRICAL_SURFACE ( 'NONE', #8197, 5.600000000000000533 ) ;
#37600=EDGE_CURVE ( 'NONE', #51011, #73231, #78491, .T. ) ;
#37601=DIRECTION ( 'NONE',  ( 0.000000000000000000, 1.000000000000000000, 0.000000000000000000 ) ) ;
#37602=CARTESIAN_POINT ( 'NONE',  ( 96.63001237737263693, -35.53283987767252228, 206.2356252759109623 ) ) ;
#37604=CARTESIAN_POINT ( 'NONE',  ( 97.12558495679242299, -37.99709113623088541, 146.4273255808599856 ) ) ;
#37605=CARTESIAN_POINT ( 'NONE',  ( 112.6753912189806073, -45.54292608213916793, 259.0270538473393458 ) ) ;
#37606=CARTESIAN_POINT ( 'NONE',  ( 100.2704505754038706, -46.49802187830721323, 83.09276813305294240 ) ) ;
#37607=CARTESIAN_POINT ( 'NONE',  ( 98.35067263469487386, -31.65512584675276386, 251.9111731073708143 ) ) ;
#37611=CARTESIAN_POINT ( 'NONE',  ( 99.04399605877385682, -42.84115830957615145, 262.8440304599521369 ) ) ;
#37612=EDGE_LOOP ( 'NONE', ( #55574, #4336, #45752, #76191 ) ) ;
#37614=VERTEX_POINT ( 'NONE', #54908 ) ;
#37616=VERTEX_POINT ( 'NONE', #48539 ) ;
#37617=ORIENTED_EDGE ( 'NONE', *, *, #64091, .F. ) ;
#37618=FACE_OUTER_BOUND ( 'NONE', #29207, .T. ) ;
#37619=CARTESIAN_POINT ( 'NONE',  ( 101.0866664386429647, -45.26901348810219616, 278.0899109901965858 ) ) ;
#37621=DIRECTION ( 'NONE',  ( 2.999999999999999839E-15, -1.000000000000000000, 2.999999999999999900E-30 ) ) ;
#37623=AXIS2_PLACEMENT_3D ( 'NONE', #56120, #21649, #57030 ) ;
#37626=CARTESIAN_POINT ( 'NONE',  ( 107.0664832912750057, -36.72944715993903486, 9.425625275910970657 ) ) ;
#37627=CARTESIAN_POINT ( 'NONE',  ( 111.2765704384832759, -44.16122339008717290, 212.4095626852199530 ) ) ;
#37631=AXIS2_PLACEMENT_3D ( 'NONE', #65903, #88610, #4585 ) ;
#37632=ORIENTED_EDGE ( 'NONE', *, *, #52901, .T. ) ;
#37633=FACE_BOUND ( 'NONE', #6514, .T. ) ;
#37634=CARTESIAN_POINT ( 'NONE',  ( 97.81361814658107789, -40.52213659492726805, 181.6360300764658291 ) ) ;
#37635=CARTESIAN_POINT ( 'NONE',  ( 99.87094702832897042, -29.26198151734326203, 261.6746728949581779 ) ) ;
#37636=CARTESIAN_POINT ( 'NONE',  ( 107.0664832912739399, -36.72944715994095333, 302.6356252759109680 ) ) ;
#37637=AXIS2_PLACEMENT_3D ( 'NONE', #36182, #85253, #8941 ) ;
#37638=CARTESIAN_POINT ( 'NONE',  ( 142.0664832912740394, -46.72944715994099596, -5.074374724088994704 ) ) ;
#37640=VERTEX_POINT ( 'NONE', #85803 ) ;
#37641=CARTESIAN_POINT ( 'NONE',  ( 99.09473700806925933, -30.55172784210162362, 56.80234965928513446 ) ) ;
#37643=EDGE_CURVE ( 'NONE', #52987, #17905, #77629, .T. ) ;
#37645=CARTESIAN_POINT ( 'NONE',  ( 98.93870468184483968, -41.20551083899233902, 24.54523322673496466 ) ) ;
#37646=CARTESIAN_POINT ( 'NONE',  ( 172.5664832912729878, -18.82844715994071194, 78.92562527591199739 ) ) ;
#37648=AXIS2_PLACEMENT_3D ( 'NONE', #32531, #10752, #11204 ) ;
#37649=DIRECTION ( 'NONE',  ( 1.000000000000000000, 4.163336342344333240E-14, 0.000000000000000000 ) ) ;
#37651=DIRECTION ( 'NONE',  ( 0.8543009526837940237, 0.03605348183280988883, -0.5185267868599396923 ) ) ;
#37652=FACE_OUTER_BOUND ( 'NONE', #22380, .T. ) ;
#37653=ORIENTED_EDGE ( 'NONE', *, *, #38599, .F. ) ;
#37654=CARTESIAN_POINT ( 'NONE',  ( 98.85774631673514534, -43.21346936515602266, 91.85848241876892928 ) ) ;
#37655=ORIENTED_EDGE ( 'NONE', *, *, #84824, .F. ) ;
#37657=CARTESIAN_POINT ( 'NONE',  ( 115.6047007430436366, -36.96391350797230757, 43.22670554236196239 ) ) ;
#37658=DIRECTION ( 'NONE',  ( 1.000000000000000078E-15, 0.000000000000000000, -1.000000000000000000 ) ) ;
#37659=CARTESIAN_POINT ( 'NONE',  ( 110.2353755222631833, -45.00509823041481638, 59.29872616303999422 ) ) ;
#37661=DIRECTION ( 'NONE',  ( 2.900000000000000265E-14, -2.000000000000000155E-15, 1.000000000000000000 ) ) ;
#37665=CARTESIAN_POINT ( 'NONE',  ( 107.6079817216441796, -48.59237387041279987, 38.61276813305397582 ) ) ;
#37666=CARTESIAN_POINT ( 'NONE',  ( 51.24204729617298426, -31.76306994223730840, -5.074374724088000832 ) ) ;
#37671=CARTESIAN_POINT ( 'NONE',  ( 107.6554453082189013, -47.17114389581161049, 148.6213395616249784 ) ) ;
#37672=DIRECTION ( 'NONE',  ( -4.237773401492740281E-14, 1.000000000000000000, 0.000000000000000000 ) ) ;
#37673=EDGE_LOOP ( 'NONE', ( #6687, #13428, #79553, #336 ) ) ;
#37674=ORIENTED_EDGE ( 'NONE', *, *, #260, .T. ) ;
#37676=AXIS2_PLACEMENT_3D ( 'NONE', #28347, #36531, #42416 ) ;
#37678=CARTESIAN_POINT ( 'NONE',  ( 104.3638673426610666, -27.29495504168057707, 225.2984824187689981 ) ) ;
#37682=CARTESIAN_POINT ( 'NONE',  ( 99.12745497205600032, -44.42007846243786418, 37.95086337114900488 ) ) ;
#37685=CARTESIAN_POINT ( 'NONE',  ( 97.07202416812739898, -35.37890067388282489, 172.2189264459942990 ) ) ;
#37686=AXIS2_PLACEMENT_3D ( 'NONE', #46516, #48296, #41492 ) ;
#37687=DIRECTION ( 'NONE',  ( 1.000000000000000078E-15, -1.000000000000000083E-30, -1.000000000000000000 ) ) ;
#37688=VERTEX_POINT ( 'NONE', #86234 ) ;
#37689=AXIS2_PLACEMENT_3D ( 'NONE', #42804, #77348, #8313 ) ;
#37690=AXIS2_PLACEMENT_3D ( 'NONE', #4256, #54156, #81917 ) ;
#37693=CARTESIAN_POINT ( 'NONE',  ( 98.85650974919595058, -29.36329775763224603, 235.7565776568629872 ) ) ;
#37695=EDGE_CURVE ( 'NONE', #37421, #30351, #50350, .T. ) ;
#37696=CARTESIAN_POINT ( 'NONE',  ( 107.0667039024479834, -67.87844715994100397, 160.9178068554150229 ) ) ;
#37698=ADVANCED_FACE ( 'NONE', ( #36294 ), #72608, .T. ) ;
#37699=CARTESIAN_POINT ( 'NONE',  ( 113.8843833678302389, -31.58431642611541434, 218.7638483995049796 ) ) ;
#37701=CARTESIAN_POINT ( 'NONE',  ( 99.31004196827758790, -43.71529311364903947, 52.90991099019698396 ) ) ;
#37703=CARTESIAN_POINT ( 'NONE',  ( 97.94803474170373647, -41.87343025248883777, 136.7356252759109623 ) ) ;
#37704=ORIENTED_EDGE ( 'NONE', *, *, #48226, .F. ) ;
#37705=DIRECTION ( 'NONE',  ( 0.7071067811865491270, -0.7071067811865459074, 7.071067811865492096E-16 ) ) ;
#37706=ORIENTED_EDGE ( 'NONE', *, *, #58306, .F. ) ;
#37707=AXIS2_PLACEMENT_3D ( 'NONE', #31956, #46007, #60544 ) ;
#37710=CARTESIAN_POINT ( 'NONE',  ( 102.0670549289058471, -27.97049807668956944, 66.48979194539977300 ) ) ;
#37712=DIRECTION ( 'NONE',  ( 1.000000000000000078E-15, 1.000000000000000083E-30, -1.000000000000000000 ) ) ;
#37713=VERTEX_POINT ( 'NONE', #78980 ) ;
#37717=CARTESIAN_POINT ( 'NONE',  ( 179.7974245136208538, -36.32844715993469009, 237.4678068554150059 ) ) ;
#37718=CIRCLE ( 'NONE', #82657, 2.029999999999997140 ) ;
#37719=CARTESIAN_POINT ( 'NONE',  ( 142.8698897858160706, -0.9167816978817300289, 394.9756252759100903 ) ) ;
#37720=CARTESIAN_POINT ( 'NONE',  ( 184.3595971212628228, -48.62134037874749737, 300.4678068554149490 ) ) ;
#37722=EDGE_CURVE ( 'NONE', #45890, #7448, #85091, .T. ) ;
#37723=CARTESIAN_POINT ( 'NONE',  ( 98.31770816264274515, -42.43955203770550355, 101.7870538473399620 ) ) ;
#37724=DIRECTION ( 'NONE',  ( 0.000000000000000000, 0.000000000000000000, 1.000000000000000000 ) ) ;
#37725=CYLINDRICAL_SURFACE ( 'NONE', #3155, 0.2500000000000039968 ) ;
#37726=DIRECTION ( 'NONE',  ( 0.000000000000000000, 0.000000000000000000, 1.000000000000000000 ) ) ;
#37729=VECTOR ( 'NONE', #6975, 1000.000000000000000 ) ;
#37731=CARTESIAN_POINT ( 'NONE',  ( 177.0371591254543659, -48.62818131005480637, 249.9678068554149775 ) ) ;
#37732=CARTESIAN_POINT ( 'NONE',  ( 141.8164832912740110, -45.62589376934770513, 14.92562527591100618 ) ) ;
#37735=CYLINDRICAL_SURFACE ( 'NONE', #42231, 2.030000000001310312 ) ;
#37738=DIRECTION ( 'NONE',  ( 1.000000000000000078E-15, -1.000000000000000000, 0.000000000000000000 ) ) ;
#37739=CARTESIAN_POINT ( 'NONE',  ( 116.7860849611260647, -31.33117650353040062, 175.2299109901959753 ) ) ;
#37740=DIRECTION ( 'NONE',  ( 0.000000000000000000, 0.000000000000000000, -1.000000000000000000 ) ) ;
#37742=CARTESIAN_POINT ( 'NONE',  ( 99.63325261332707328, -43.08637385293071276, 27.88991099019594344 ) ) ;
#37743=DIRECTION ( 'NONE',  ( -0.7071067811874389708, 0.7071067811856560636, 0.000000000000000000 ) ) ;
#37744=CARTESIAN_POINT ( 'NONE',  ( 75.31670390244798341, -57.40094715994099772, 37.63480685541480852 ) ) ;
#37747=ORIENTED_EDGE ( 'NONE', *, *, #3074, .F. ) ;
#37748=CARTESIAN_POINT ( 'NONE',  ( 41.56648329127399677, -18.82844715994099971, 136.8086252759119645 ) ) ;
#37749=ORIENTED_EDGE ( 'NONE', *, *, #72053, .F. ) ;
#37750=ORIENTED_EDGE ( 'NONE', *, *, #29084, .F. ) ;
#37752=CARTESIAN_POINT ( 'NONE',  ( 110.1519232268686181, -46.31854332990749867, 204.2558690201829847 ) ) ;
#37754=CYLINDRICAL_SURFACE ( 'NONE', #58869, 3.000000000000002665 ) ;
#37755=CARTESIAN_POINT ( 'NONE',  ( 110.0319707555399447, -45.11204900458633915, 34.27872616304095033 ) ) ;
#37757=DIRECTION ( 'NONE',  ( 1.000000000000000000, 4.299999999999999979E-14, 1.000000000000000078E-15 ) ) ;
#37758=VECTOR ( 'NONE', #47806, 1000.000000000000000 ) ;
#37759=DIRECTION ( 'NONE',  ( 0.8571673007021091140, -8.250245410175212261E-16, 0.5150380749100597066 ) ) ;
#37760=VERTEX_POINT ( 'NONE', #65766 ) ;
#37761=CARTESIAN_POINT ( 'NONE',  ( 21.03715912545738220, -47.82818131006197149, 193.9678068554150627 ) ) ;
#37762=DIRECTION ( 'NONE',  ( -0.7071067811855900054, -0.7071067811875051401, 0.000000000000000000 ) ) ;
#37764=CARTESIAN_POINT ( 'NONE',  ( 118.6297112294784029, -39.20734283244436114, 258.6584824187679033 ) ) ;
#37766=VERTEX_POINT ( 'NONE', #37189 ) ;
#37768=DIRECTION ( 'NONE',  ( 1.000000000000000078E-15, -1.000000000000000083E-30, -1.000000000000000000 ) ) ;
#37769=CIRCLE ( 'NONE', #39180, 7.499999999999996447 ) ;
#37770=CARTESIAN_POINT ( 'NONE',  ( 182.2420472961722737, -31.76306994223702418, 342.9256252759109884 ) ) ;
#37772=CARTESIAN_POINT ( 'NONE',  ( 109.3463552500793554, -26.51205201248422583, 220.9013395616249795 ) ) ;
#37774=ORIENTED_EDGE ( 'NONE', *, *, #72997, .F. ) ;
#37776=CARTESIAN_POINT ( 'NONE',  ( 104.7259408665080116, -47.57930243624250721, 28.41943479971997988 ) ) ;
#37778=CARTESIAN_POINT ( 'NONE',  ( 110.8926993666852496, -26.99363814275770679, 269.7784824187681920 ) ) ;
#37780=AXIS2_PLACEMENT_3D ( 'NONE', #89288, #76091, #70173 ) ;
#37781=CARTESIAN_POINT ( 'NONE',  ( 78.21292805806618276, -38.76093376056942930, 7.655955902689210113 ) ) ;
#37782=CARTESIAN_POINT ( 'NONE',  ( 115.7840071928116004, -41.80079596848010937, 19.40698120903841684 ) ) ;
#37784=CARTESIAN_POINT ( 'NONE',  ( 113.4089301560035068, -41.86784124614906233, 86.10237608387694763 ) ) ;
#37785=CARTESIAN_POINT ( 'NONE',  ( 117.7987307161850907, -31.64603138916173464, 210.1784824187679703 ) ) ;
#37789=CIRCLE ( 'NONE', #10234, 6.571100913904384555 ) ;
#37791=VERTEX_POINT ( 'NONE', #3114 ) ;
#37793=ORIENTED_EDGE ( 'NONE', *, *, #84660, .T. ) ;
#37795=CARTESIAN_POINT ( 'NONE',  ( 108.3349140068648637, -46.73468863093219738, 168.6781975528624002 ) ) ;
#37796=B_SPLINE_CURVE_WITH_KNOTS ( 'NONE', 3,
 ( #7778, #12923, #20183, #33800, #64537, #43173, #63185, #29122, #962, #63638, #54211, #89226, #84554, #15945, #19720, #22768, #82422, #49086 ),
 .UNSPECIFIED., .F., .F.,
 ( 4, 2, 2, 2, 2, 2, 2, 2, 4 ),
 ( 0.000000000000000000, 0.06249999972775545365, 0.1249999994555109073, 0.1874999991832663748, 0.2499999989110218146, 0.3124999986387772544, 0.3749999983665327496, 0.4374999980942881894, 0.4999999978220436292 ),
 .UNSPECIFIED. ) ;
#37797=CARTESIAN_POINT ( 'NONE',  ( 97.39129913838408470, -39.27854586558702721, 42.53143958753435783 ) ) ;
#37798=EDGE_CURVE ( 'NONE', #33917, #14322, #86649, .T. ) ;
#37799=CARTESIAN_POINT ( 'NONE',  ( 108.0930535991856800, -45.20896867503704897, 117.0952769709339663 ) ) ;
#37800=CARTESIAN_POINT ( 'NONE',  ( 96.67081033544403113, -37.96906397156782731, 41.42133956162496844 ) ) ;
#37803=EDGE_CURVE ( 'NONE', #58395, #55190, #26708, .T. ) ;
#37806=CARTESIAN_POINT ( 'NONE',  ( 97.53181971261398076, -39.74887774678698804, 137.5705102554088626 ) ) ;
#37810=LINE ( 'NONE', #59565, #29984 ) ;
#37813=CARTESIAN_POINT ( 'NONE',  ( 99.99420790045508056, -28.96206233275049158, 285.6641967044822650 ) ) ;
#37816=CARTESIAN_POINT ( 'NONE',  ( 112.6638099339533028, -45.52472799210174514, 263.0270538473394595 ) ) ;
#37817=CARTESIAN_POINT ( 'NONE',  ( 100.5235407922616133, -27.76354498484767674, 26.56610146638793779 ) ) ;
#37818=CARTESIAN_POINT ( 'NONE',  ( 105.7154773228390781, -46.72385839126379636, 118.4689586086422253 ) ) ;
#37819=CARTESIAN_POINT ( 'NONE',  ( 134.0664832912740110, -46.72944715994100306, -0.5743747240890021422 ) ) ;
#37821=DIRECTION ( 'NONE',  ( -0.7071067811864676367, -0.7071067811866273978, -7.071067811864669709E-16 ) ) ;
#37823=DIRECTION ( 'NONE',  ( 0.000000000000000000, 0.000000000000000000, -1.000000000000000000 ) ) ;
#37824=EDGE_CURVE ( 'NONE', #81352, #26573, #18415, .T. ) ;
#37827=LINE ( 'NONE', #45061, #85175 ) ;
#37831=CARTESIAN_POINT ( 'NONE',  ( 104.2289649446409783, -46.80690502001216657, 22.35848241876792031 ) ) ;
#37832=CARTESIAN_POINT ( 'NONE',  ( 96.65005459693196599, -37.15429219901626823, 157.3584824187679487 ) ) ;
#37833=CARTESIAN_POINT ( 'NONE',  ( 96.17045672112728028, -38.71987694442820782, 47.48229194257797303 ) ) ;
#37835=CARTESIAN_POINT ( 'NONE',  ( 151.0371591254573218, -24.95799193692592866, 300.4678068554149490 ) ) ;
#37836=CARTESIAN_POINT ( 'NONE',  ( 82.57637212003993454, -35.60518726036713133, 2.783021291302837152 ) ) ;
#37838=CARTESIAN_POINT ( 'NONE',  ( 98.34985896129799698, -31.65658472717509397, 186.9064586016984038 ) ) ;
#37839=ORIENTED_EDGE ( 'NONE', *, *, #38532, .T. ) ;
#37840=AXIS2_PLACEMENT_3D ( 'NONE', #76429, #69174, #84616 ) ;
#37841=CARTESIAN_POINT ( 'NONE',  ( 109.7352083718000131, -46.17358189742679286, 68.79562527591099297 ) ) ;
#37844=AXIS2_PLACEMENT_3D ( 'NONE', #41940, #56924, #36503 ) ;
#37845=CARTESIAN_POINT ( 'NONE',  ( 134.0664832912740110, -46.72944715994100306, -0.8743747240890020755 ) ) ;
#37846=CARTESIAN_POINT ( 'NONE',  ( 114.7977927517517855, -29.71579763117551565, 205.4127681330539872 ) ) ;
#37849=CARTESIAN_POINT ( 'NONE',  ( 50.56670390244699576, -18.82844715994031048, 335.8680179914122732 ) ) ;
#37850=CIRCLE ( 'NONE', #1808, 2.500000000000002220 ) ;
#37852=FACE_BOUND ( 'NONE', #28837, .T. ) ;
#37853=CARTESIAN_POINT ( 'NONE',  ( 99.50454240397225192, -43.30556165129220858, 96.89604753381240698 ) ) ;
#37854=CARTESIAN_POINT ( 'NONE',  ( 102.5967720069230324, -27.99243076246517603, 120.4527681330539792 ) ) ;
#37856=ORIENTED_EDGE ( 'NONE', *, *, #41781, .F. ) ;
#37857=EDGE_CURVE ( 'NONE', #17090, #39460, #83053, .T. ) ;
#37858=CARTESIAN_POINT ( 'NONE',  ( 116.2543158056996333, -38.69420140005939857, 105.1025356868499614 ) ) ;
#37859=AXIS2_PLACEMENT_3D ( 'NONE', #37332, #50045, #79578 ) ;
#37861=CARTESIAN_POINT ( 'NONE',  ( 101.7545977962314652, -44.98157700518526525, 218.1213395616249784 ) ) ;
#37863=LINE ( 'NONE', #71942, #53578 ) ;
#37864=CARTESIAN_POINT ( 'NONE',  ( 97.06107378353082993, -37.99643432997152814, 112.4278404525605737 ) ) ;
#37865=EDGE_CURVE ( 'NONE', #12019, #19567, #88955, .T. ) ;
#37867=DIRECTION ( 'NONE',  ( 0.000000000000000000, 0.000000000000000000, 1.000000000000000000 ) ) ;
#37869=LINE ( 'NONE', #71509, #24089 ) ;
#37870=CARTESIAN_POINT ( 'NONE',  ( 97.81366378802354689, -42.73395665195503312, 146.7965776568629508 ) ) ;
#37871=EDGE_LOOP ( 'NONE', ( #50782, #81355, #10902, #24839 ) ) ;
#37872=ORIENTED_EDGE ( 'NONE', *, *, #11566, .F. ) ;
#37873=CIRCLE ( 'NONE', #88650, 2.517500000000005844 ) ;
#37875=CARTESIAN_POINT ( 'NONE',  ( 113.2454987164303901, -28.75867296000128093, 150.5522919406864162 ) ) ;
#37877=CARTESIAN_POINT ( 'NONE',  ( 97.81820226091151937, -40.53330621887679541, 102.6369915585742092 ) ) ;
#37878=EDGE_CURVE ( 'NONE', #66869, #10930, #1582, .T. ) ;
#37879=CARTESIAN_POINT ( 'NONE',  ( 112.0659024056236603, -45.48840166505959104, 268.9897911008726510 ) ) ;
#37880=CARTESIAN_POINT ( 'NONE',  ( 117.0684261367714072, -39.67022423017687771, 183.5984824187679578 ) ) ;
#37881=CARTESIAN_POINT ( 'NONE',  ( 135.4471649165523672, -39.11090284777271364, 7.925007058950424010 ) ) ;
#37885=AXIS2_PLACEMENT_3D ( 'NONE', #85740, #72970, #58880 ) ;
#37886=CARTESIAN_POINT ( 'NONE',  ( 98.82648729870214765, -42.42054397291916956, 62.80801425164322893 ) ) ;
#37888=CARTESIAN_POINT ( 'NONE',  ( 131.9645448811436950, -34.94667115357206910, 7.474641677891152192 ) ) ;
#37890=CARTESIAN_POINT ( 'NONE',  ( 98.69997382787508400, -39.74003663468293013, 263.0330118773257482 ) ) ;
#37892=CARTESIAN_POINT ( 'NONE',  ( 80.06648329127402519, -46.72944715994105991, 4.925625275910944012 ) ) ;
#37893=ORIENTED_EDGE ( 'NONE', *, *, #80306, .T. ) ;
#37894=CARTESIAN_POINT ( 'NONE',  ( 111.4380389023045552, -44.06754350613674376, 9.635625275910941312 ) ) ;
#37895=CARTESIAN_POINT ( 'NONE',  ( 188.5667039024486087, -48.82844715993430640, 137.2178068554150059 ) ) ;
#37896=ORIENTED_EDGE ( 'NONE', *, *, #7663, .F. ) ;
#37898=CARTESIAN_POINT ( 'NONE',  ( 110.8587645964465338, -45.98247965540819848, 112.8859944073334844 ) ) ;
#37900=ORIENTED_EDGE ( 'NONE', *, *, #84779, .F. ) ;
#37901=CARTESIAN_POINT ( 'NONE',  ( 115.5202298134134367, -37.95022619834508504, 28.13527697093398672 ) ) ;
#37902=CARTESIAN_POINT ( 'NONE',  ( 104.5572623809163701, -48.33710955716689028, 182.4070538473399665 ) ) ;
#37904=CARTESIAN_POINT ( 'NONE',  ( 117.1049515565469221, -33.87427183379790563, 149.0470538473389581 ) ) ;
#37905=CARTESIAN_POINT ( 'NONE',  ( 48.79742451361996558, -36.32844715994077944, 117.4678068554150485 ) ) ;
#37906=CARTESIAN_POINT ( 'NONE',  ( 100.1387811872355371, -44.51978932219680019, 262.9984824187678782 ) ) ;
#37910=ORIENTED_EDGE ( 'NONE', *, *, #19643, .T. ) ;
#37911=EDGE_LOOP ( 'NONE', ( #57408, #20507, #75097, #69372, #40865, #48214, #44398, #87942 ) ) ;
#37912=AXIS2_PLACEMENT_3D ( 'NONE', #58150, #71790, #78176 ) ;
#37913=VECTOR ( 'NONE', #43127, 1000.000000000000000 ) ;
#37914=CARTESIAN_POINT ( 'NONE',  ( 97.38432216341050207, -42.15794967186695175, 181.7451490854349743 ) ) ;
#37915=ORIENTED_EDGE ( 'NONE', *, *, #82792, .F. ) ;
#37916=CARTESIAN_POINT ( 'NONE',  ( 96.64983689172015602, -37.15430107835312157, 161.3584824187679487 ) ) ;
#37917=DIRECTION ( 'NONE',  ( 0.000000000000000000, 0.000000000000000000, 1.000000000000000000 ) ) ;
#37918=DIRECTION ( 'NONE',  ( 0.9825752044328147639, 0.1858654557302462929, 0.000000000000000000 ) ) ;
#37920=DIRECTION ( 'NONE',  ( 3.999999999999999995E-14, -1.000000000000000000, 4.100000000000000342E-29 ) ) ;
#37922=CARTESIAN_POINT ( 'NONE',  ( 116.8666056714781973, -37.25052799200011577, 14.78419670448194445 ) ) ;
#37923=DIRECTION ( 'NONE',  ( 0.000000000000000000, 0.000000000000000000, 1.000000000000000000 ) ) ;
#37924=LINE ( 'NONE', #23429, #27946 ) ;
#37925=CARTESIAN_POINT ( 'NONE',  ( 116.3115597373110290, -32.94279827685361539, 270.1356252759109680 ) ) ;
#37926=EDGE_CURVE ( 'NONE', #86883, #85398, #23319, .T. ) ;
#37927=CYLINDRICAL_SURFACE ( 'NONE', #25415, 9.999999999999998224 ) ;
#37928=ADVANCED_FACE ( 'NONE', ( #57094 ), #36224, .F. ) ;
#37929=CARTESIAN_POINT ( 'NONE',  ( 76.06670390244805446, -58.72944715994109544, 239.5838068554169809 ) ) ;
#37931=CARTESIAN_POINT ( 'NONE',  ( 98.80107334477645509, -37.99123951698243928, 195.5838068554173219 ) ) ;
#37933=CARTESIAN_POINT ( 'NONE',  ( 136.3179110785966088, -20.31136518417599035, 7.339178645738122952 ) ) ;
#37934=CARTESIAN_POINT ( 'NONE',  ( 96.02321403599634664, -35.86825885766610611, 191.2765776568629690 ) ) ;
#37935=CARTESIAN_POINT ( 'NONE',  ( 103.9574082008755198, -47.33640867427461529, 58.33753003781600199 ) ) ;
#37936=CARTESIAN_POINT ( 'NONE',  ( 115.8919449742516861, -44.71207447090664999, 229.2413395616249545 ) ) ;
#37938=CARTESIAN_POINT ( 'NONE',  ( 133.6498166246070127, 12.92155284005802507, 349.2756252759110680 ) ) ;
#37939=LINE ( 'NONE', #60143, #69639 ) ;
#37940=DIRECTION ( 'NONE',  ( 0.000000000000000000, 0.000000000000000000, 1.000000000000000000 ) ) ;
#37941=DIRECTION ( 'NONE',  ( 0.000000000000000000, 0.000000000000000000, -1.000000000000000000 ) ) ;
#37942=CARTESIAN_POINT ( 'NONE',  ( 32.15435173583699680, -31.62489322948790971, 313.9678068554150059 ) ) ;
#37943=CIRCLE ( 'NONE', #49526, 5.599999999999994316 ) ;
#37945=ORIENTED_EDGE ( 'NONE', *, *, #75957, .F. ) ;
#37946=ORIENTED_EDGE ( 'NONE', *, *, #63878, .T. ) ;
#37947=CARTESIAN_POINT ( 'NONE',  ( 115.5093363421805606, -33.45364150533647063, 93.53146744712398686 ) ) ;
#37950=CARTESIAN_POINT ( 'NONE',  ( 101.7670726180548542, -27.05576796868586698, 96.46324432352997746 ) ) ;
#37951=DIRECTION ( 'NONE',  ( 5.512527431108029424E-15, -1.000000000000000000, 0.000000000000000000 ) ) ;
#37953=CARTESIAN_POINT ( 'NONE',  ( 78.22143491580753505, -16.68812225915645797, 7.662832107308280349 ) ) ;
#37955=CARTESIAN_POINT ( 'NONE',  ( 97.33063403691424753, -33.15845143124434458, 21.03467289495897319 ) ) ;
#37957=VERTEX_POINT ( 'NONE', #49832 ) ;
#37959=FACE_OUTER_BOUND ( 'NONE', #53938, .T. ) ;
#37960=FACE_OUTER_BOUND ( 'NONE', #19153, .T. ) ;
#37966=FACE_OUTER_BOUND ( 'NONE', #43041, .T. ) ;
#37967=VECTOR ( 'NONE', #14139, 1000.000000000000000 ) ;
#37969=CARTESIAN_POINT ( 'NONE',  ( 101.1533894386775074, -27.41820966596953468, 65.51467289495799662 ) ) ;
#37973=LINE ( 'NONE', #11621, #28891 ) ;
#37974=VECTOR ( 'NONE', #36263, 999.9999999999998863 ) ;
#37976=CARTESIAN_POINT ( 'NONE',  ( 98.22859028455410169, -39.55567757615634861, 129.3909475124479798 ) ) ;
#37980=DIRECTION ( 'NONE',  ( -0.7071067811892183252, 0.7071067811838767092, -7.071067811892191094E-16 ) ) ;
#37981=EDGE_LOOP ( 'NONE', ( #62663, #38789 ) ) ;
#37985=ORIENTED_EDGE ( 'NONE', *, *, #79026, .F. ) ;
#37986=ORIENTED_EDGE ( 'NONE', *, *, #35643, .F. ) ;
#37989=CARTESIAN_POINT ( 'NONE',  ( 97.29374130088892514, -39.17162219779756782, 162.9530118773259630 ) ) ;
#37991=CARTESIAN_POINT ( 'NONE',  ( 31.78666935232982738, -36.02818131005922453, 237.4678068554150059 ) ) ;
#37992=CARTESIAN_POINT ( 'NONE',  ( 107.3345073157536689, -26.28600797661530208, 116.0556252759109555 ) ) ;
#37993=CARTESIAN_POINT ( 'NONE',  ( 97.07207208091389816, -35.37844104438559611, 121.2189585969273509 ) ) ;
#37994=VECTOR ( 'NONE', #56236, 1000.000000000000000 ) ;
#37996=CARTESIAN_POINT ( 'NONE',  ( 97.83900511596046101, -40.58358500529822521, 16.64132214453083947 ) ) ;
#37997=ORIENTED_EDGE ( 'NONE', *, *, #42821, .F. ) ;
#38000=EDGE_LOOP ( 'NONE', ( #41407, #47348, #76885, #88836 ) ) ;
#38002=CIRCLE ( 'NONE', #88794, 1.000000000000000888 ) ;
#38003=CARTESIAN_POINT ( 'NONE',  ( 106.6101046285737510, -27.46188816740816918, 192.9338046553059485 ) ) ;
#38004=CARTESIAN_POINT ( 'NONE',  ( 109.9170780819575839, -46.81718586395340509, 72.79562527591099297 ) ) ;
#38005=ORIENTED_EDGE ( 'NONE', *, *, #37307, .F. ) ;
#38006=CARTESIAN_POINT ( 'NONE',  ( 105.4244226815142156, -47.00233879195506148, 37.44991099019695469 ) ) ;
#38007=CARTESIAN_POINT ( 'NONE',  ( 116.7939007044644200, -39.39219064343244980, 253.6148464904360367 ) ) ;
#38008=DIRECTION ( 'NONE',  ( 1.000000000000000078E-15, -1.000000000000000083E-30, -1.000000000000000000 ) ) ;
#38009=CARTESIAN_POINT ( 'NONE',  ( 113.6324552648963504, -29.12879861577680529, 195.5092680403551810 ) ) ;
#38010=CARTESIAN_POINT ( 'NONE',  ( 118.9175753851156401, -36.92810247848812821, 149.8127681330539644 ) ) ;
#38012=EDGE_CURVE ( 'NONE', #61339, #29424, #41618, .T. ) ;
#38013=CARTESIAN_POINT ( 'NONE',  ( 117.0608945242948238, -38.08045311361057372, 263.7189586098177756 ) ) ;
#38014=ORIENTED_EDGE ( 'NONE', *, *, #73041, .F. ) ;
#38018=FACE_OUTER_BOUND ( 'NONE', #75619, .T. ) ;
#38023=CARTESIAN_POINT ( 'NONE',  ( 98.30753417268519456, -41.72887546008843884, 176.7397919400707167 ) ) ;
#38024=CARTESIAN_POINT ( 'NONE',  ( 110.4566641872556403, -47.25017721759432732, 57.83657765686300678 ) ) ;
#38025=DIRECTION ( 'NONE',  ( 0.9963424814100680926, -0.08544974978095730422, 0.000000000000000000 ) ) ;
#38026=LINE ( 'NONE', #67067, #85527 ) ;
#38028=CARTESIAN_POINT ( 'NONE',  ( 113.9027609268606369, -43.72435554967460547, 73.19276813305496887 ) ) ;
#38029=LINE ( 'NONE', #39364, #33327 ) ;
#38030=CARTESIAN_POINT ( 'NONE',  ( 95.93334478249057895, -32.74178691125834462, 172.0527681330539735 ) ) ;
#38031=CYLINDRICAL_SURFACE ( 'NONE', #56742, 5.599999999999994316 ) ;
#38032=CARTESIAN_POINT ( 'NONE',  ( 46.03715912545432332, -48.62818131006086020, 249.9678068554150343 ) ) ;
#38034=LINE ( 'NONE', #23093, #12133 ) ;
#38035=EDGE_CURVE ( 'NONE', #84821, #44708, #28499, .T. ) ;
#38036=CARTESIAN_POINT ( 'NONE',  ( 83.06670390244796920, -67.87844715994100397, 231.5838068554150198 ) ) ;
#38037=EDGE_CURVE ( 'NONE', #21182, #38055, #1262, .T. ) ;
#38038=LINE ( 'NONE', #18473, #32814 ) ;
#38039=ADVANCED_FACE ( 'NONE', ( #84398 ), #22165, .T. ) ;
#38040=LINE ( 'NONE', #10336, #86858 ) ;
#38041=CARTESIAN_POINT ( 'NONE',  ( 99.72210660708088881, -29.26842865273154004, 225.6956252759109702 ) ) ;
#38042=ORIENTED_EDGE ( 'NONE', *, *, #9386, .T. ) ;
#38043=CARTESIAN_POINT ( 'NONE',  ( 97.79835618974222200, -40.48471054006801495, 146.6328135905738179 ) ) ;
#38044=CARTESIAN_POINT ( 'NONE',  ( 110.9006160922534150, -26.97349402997008383, 265.7784824187680783 ) ) ;
#38045=CARTESIAN_POINT ( 'NONE',  ( 117.6248412043677121, -33.30620651169719082, 130.0880062282919880 ) ) ;
#38046=EDGE_CURVE ( 'NONE', #19093, #26394, #35924, .T. ) ;
#38047=CARTESIAN_POINT ( 'NONE',  ( 104.4929451592478955, -26.97798605588400278, 251.2871328988943844 ) ) ;
#38049=CARTESIAN_POINT ( 'NONE',  ( 82.81647637678393892, -36.77596264856293828, 6.749779334551927690 ) ) ;
#38050=PLANE ( 'NONE',  #6575 ) ;
#38051=CARTESIAN_POINT ( 'NONE',  ( 151.0371591254584871, -46.82818131005592477, 180.4678068554149775 ) ) ;
#38052=ORIENTED_EDGE ( 'NONE', *, *, #64363, .T. ) ;
#38053=AXIS2_PLACEMENT_3D ( 'NONE', #5254, #74742, #61104 ) ;
#38055=VERTEX_POINT ( 'NONE', #3931 ) ;
#38057=CARTESIAN_POINT ( 'NONE',  ( 101.9936209245900756, -45.44607152936009697, 72.15645860776081122 ) ) ;
#38058=CARTESIAN_POINT ( 'NONE',  ( 116.5819428025096585, -42.35350697836285860, 279.4137205140061724 ) ) ;
#38059=CARTESIAN_POINT ( 'NONE',  ( 134.0664832912740110, -46.72944715994100306, 1.625625275910997480 ) ) ;
#38060=CARTESIAN_POINT ( 'NONE',  ( 177.0664832912740110, 12.92155284005802685, 336.5756252759111362 ) ) ;
#38063=CARTESIAN_POINT ( 'NONE',  ( 172.5667039024480687, -36.32844715993499563, 129.9678068554150059 ) ) ;
#38064=CARTESIAN_POINT ( 'NONE',  ( 99.44356389104279970, -40.64648710652873831, 196.1267055423629699 ) ) ;
#38065=ORIENTED_EDGE ( 'NONE', *, *, #43405, .T. ) ;
#38067=ORIENTED_EDGE ( 'NONE', *, *, #74199, .F. ) ;
#38068=VECTOR ( 'NONE', #41021, 1000.000000000000000 ) ;
#38072=CARTESIAN_POINT ( 'NONE',  ( 105.4490071354754406, -45.46730099742844544, 8.861583305896925111 ) ) ;
#38078=CARTESIAN_POINT ( 'NONE',  ( 103.2781190732607115, -27.47481063885592434, 56.38565936678559609 ) ) ;
#38079=EDGE_LOOP ( 'NONE', ( #56396, #15489, #43955 ) ) ;
#38081=CARTESIAN_POINT ( 'NONE',  ( 110.4716576677765119, -44.14797218061634254, 25.73666179816297372 ) ) ;
#38082=DIRECTION ( 'NONE',  ( 0.000000000000000000, 1.000000000000000000, 1.914177628664063178E-15 ) ) ;
#38083=ADVANCED_FACE ( 'NONE', ( #65270 ), #18446, .F. ) ;
#38085=DIRECTION ( 'NONE',  ( -0.7071067811865443531, -0.7071067811865506814, -7.071067811865450681E-16 ) ) ;
#38086=DIRECTION ( 'NONE',  ( 0.000000000000000000, 0.000000000000000000, -1.000000000000000000 ) ) ;
#38090=LINE ( 'NONE', #46673, #48427 ) ;
#38092=ORIENTED_EDGE ( 'NONE', *, *, #22027, .F. ) ;
#38093=CARTESIAN_POINT ( 'NONE',  ( 98.58988425959138624, -43.82355431373886034, 71.86895860924397539 ) ) ;
#38094=ORIENTED_EDGE ( 'NONE', *, *, #36349, .F. ) ;
#38095=CARTESIAN_POINT ( 'NONE',  ( 104.1257281832662613, -27.47619977921510781, 54.74384839950496939 ) ) ;
#38096=EDGE_CURVE ( 'NONE', #80398, #63665, #34426, .T. ) ;
#38097=CARTESIAN_POINT ( 'NONE',  ( 102.8437810223914255, -45.83527424000978812, 88.23010560950143599 ) ) ;
#38098=CARTESIAN_POINT ( 'NONE',  ( 98.44267559312871185, -33.00030968290830202, 57.44539282970595195 ) ) ;
#38099=CARTESIAN_POINT ( 'NONE',  ( 113.1772940493579966, -44.75261571957639717, 14.09386025446782753 ) ) ;
#38101=DIRECTION ( 'NONE',  ( 1.000000000000000000, 0.000000000000000000, 0.000000000000000000 ) ) ;
#38103=CARTESIAN_POINT ( 'NONE',  ( 112.1919128969917097, -27.58564230820396190, 30.66991099019694644 ) ) ;
#38104=CARTESIAN_POINT ( 'NONE',  ( 194.5667039024485803, -47.82844715993405060, 129.9678068554150343 ) ) ;
#38106=ORIENTED_EDGE ( 'NONE', *, *, #47577, .T. ) ;
#38107=DIRECTION ( 'NONE',  ( -1.000000000000000078E-15, 1.000000000000000083E-30, 1.000000000000000000 ) ) ;
#38108=ORIENTED_EDGE ( 'NONE', *, *, #86610, .T. ) ;
#38111=ORIENTED_EDGE ( 'NONE', *, *, #55670, .F. ) ;
#38113=CARTESIAN_POINT ( 'NONE',  ( 53.56670390244828184, -48.82844715994055917, 300.4678068554150059 ) ) ;
#38114=CARTESIAN_POINT ( 'NONE',  ( 112.6540662323892263, -44.79745133516141209, 203.0584824187689605 ) ) ;
#38115=CARTESIAN_POINT ( 'NONE',  ( 98.08598099046197660, -32.25672833729997535, 125.9577075789795373 ) ) ;
#38116=CARTESIAN_POINT ( 'NONE',  ( 163.2449138992999735, -32.11662333284611748, -5.074374724088000832 ) ) ;
#38117=CARTESIAN_POINT ( 'NONE',  ( 114.3531094850664260, -44.18515411228707279, 69.19276813305397411 ) ) ;
#38118=EDGE_CURVE ( 'NONE', #35473, #12869, #38888, .T. ) ;
#38119=CARTESIAN_POINT ( 'NONE',  ( 115.0371363339966280, -42.90862416454874051, 44.30227608399194139 ) ) ;
#38120=ORIENTED_EDGE ( 'NONE', *, *, #37388, .T. ) ;
#38121=CARTESIAN_POINT ( 'NONE',  ( 97.80863031437060329, -40.50995291785646657, 172.6349830369815663 ) ) ;
#38122=CARTESIAN_POINT ( 'NONE',  ( 184.5664832912729878, -71.37844715994266664, 342.9256252759109884 ) ) ;
#38124=ORIENTED_EDGE ( 'NONE', *, *, #6118, .T. ) ;
#38126=DIRECTION ( 'NONE',  ( 1.000000000000000000, -6.836348673800234255E-15, 0.000000000000000000 ) ) ;
#38127=DIRECTION ( 'NONE',  ( 0.000000000000000000, 0.000000000000000000, -1.000000000000000000 ) ) ;
#38128=CARTESIAN_POINT ( 'NONE',  ( 106.9407056411434951, -47.75886249174727283, 232.5794347997199907 ) ) ;
#38129=LINE ( 'NONE', #39011, #6604 ) ;
#38131=CARTESIAN_POINT ( 'NONE',  ( 19.56670390244796920, -48.82844715994099971, 300.9178068554150514 ) ) ;
#38132=CARTESIAN_POINT ( 'NONE',  ( 114.4310042120387862, -41.05610445278038156, 237.8267055423629586 ) ) ;
#38133=AXIS2_PLACEMENT_3D ( 'NONE', #4745, #75125, #20170 ) ;
#38135=CARTESIAN_POINT ( 'NONE',  ( 104.2200364793041700, -25.25138339198311144, 86.26991099019699050 ) ) ;
#38137=CARTESIAN_POINT ( 'NONE',  ( 114.0516219551475245, -28.93108169718528444, 114.4956252759109816 ) ) ;
#38138=ORIENTED_EDGE ( 'NONE', *, *, #11367, .T. ) ;
#38139=CARTESIAN_POINT ( 'NONE',  ( 132.8827458516715581, -21.21170328187201903, 8.006085407567432810 ) ) ;
#38143=DIRECTION ( 'NONE',  ( -3.999999999999999995E-14, 1.000000000000000000, -4.100000000000000342E-29 ) ) ;
#38144=EDGE_LOOP ( 'NONE', ( #7725, #57541 ) ) ;
#38145=EDGE_CURVE ( 'NONE', #31941, #62004, #22848, .T. ) ;
#38146=CARTESIAN_POINT ( 'NONE',  ( 97.07202004682035579, -35.37880823152836030, 51.21898755952398830 ) ) ;
#38147=CARTESIAN_POINT ( 'NONE',  ( 109.2642598482130154, -47.00181652296804913, 107.7441967044829880 ) ) ;
#38148=VERTEX_POINT ( 'NONE', #11650 ) ;
#38149=DIRECTION ( 'NONE',  ( -1.000000000000000000, -4.299999999999999979E-14, -1.000000000000000078E-15 ) ) ;
#38150=EDGE_CURVE ( 'NONE', #10055, #71324, #4388, .T. ) ;
#38151=CARTESIAN_POINT ( 'NONE',  ( 116.3175913315759402, -32.94491325663879877, 165.1356252759109680 ) ) ;
#38152=DIRECTION ( 'NONE',  ( -2.999999999999999839E-15, 1.000000000000000000, -2.999999999999999900E-30 ) ) ;
#38153=ORIENTED_EDGE ( 'NONE', *, *, #32446, .F. ) ;
#38154=CARTESIAN_POINT ( 'NONE',  ( 103.1971861921166038, -46.47197777470199753, 117.2756252759109543 ) ) ;
#38156=CARTESIAN_POINT ( 'NONE',  ( 141.8664832912729992, -71.52944715994142655, 342.9256252759109884 ) ) ;
#38157=CARTESIAN_POINT ( 'NONE',  ( 41.56648329127399677, 0.2215528400590013880, 196.8086252759119645 ) ) ;
#38158=FACE_OUTER_BOUND ( 'NONE', #60040, .T. ) ;
#38159=DIRECTION ( 'NONE',  ( 1.000000000000000000, 6.145690160522480771E-16, 0.000000000000000000 ) ) ;
#38161=TOROIDAL_SURFACE ( 'NONE', #22222, 11.75000000000000000, 2.550000000000000266 ) ;
#38162=ORIENTED_EDGE ( 'NONE', *, *, #75316, .T. ) ;
#38164=B_SPLINE_CURVE_WITH_KNOTS ( 'NONE', 3,
 ( #20717, #69317, #32535, #60240, #25733, #18921, #53408, #12111, #67511, #270, #8897, #29776, #62933, #83851, #69766, #78391, #49301, #2071, #56569, #22518, #50649, #57467, #712, #7091, #57013, #16153, #84312, #70211, #7981, #84755, #28419, #50198, #8440, #55645, #7538, #34785, #43828, #77931, #22083, #42479, #56103, #71122 ),
 .UNSPECIFIED., .F., .F.,
 ( 4, 2, 1, 1, 1, 1, 1, 1, 2, 2, 2, 2, 2, 2, 2, 2, 2, 2, 2, 2, 2, 2, 2, 4 ),
 ( 0.4999355867161964229, 0.5000576727545975597, 0.5001797587929986966, 0.5004239308697975286, 0.5009122750233935273, 0.5018889633305889664, 0.5038423399449779572, 0.5077490931737559388, 0.5155625996313152326, 0.5311896125464334872, 0.5624436383766713288, 0.6249516900371467898, 0.6562057158673846313, 0.6874597416976223618, 0.7187137675278600923, 0.7499677933580979339, 0.7812218191883356644, 0.8124758450185733949, 0.8437298708488112364, 0.8749838966790488559, 0.9062379225092866974, 0.9374919483395244280, 0.9687459741697621585, 1.000000000000000000 ),
 .UNSPECIFIED. ) ;
#38165=CARTESIAN_POINT ( 'NONE',  ( 97.81169951533574647, -40.51743117454552134, 102.6356342116286413 ) ) ;
#38166=LINE ( 'NONE', #74027, #83634 ) ;
#38167=CARTESIAN_POINT ( 'NONE',  ( 116.6018603435394141, -39.73108032723776972, 249.5838075904518121 ) ) ;
#38169=CYLINDRICAL_SURFACE ( 'NONE', #1609, 1.000000000002049694 ) ;
#38170=CIRCLE ( 'NONE', #77334, 18.00000000000000000 ) ;
#38171=EDGE_CURVE ( 'NONE', #43446, #83511, #85244, .T. ) ;
#38172=ORIENTED_EDGE ( 'NONE', *, *, #60114, .F. ) ;
#38173=CARTESIAN_POINT ( 'NONE',  ( 108.3334482501379767, -46.73485933287561522, 33.67729195491988747 ) ) ;
#38174=CARTESIAN_POINT ( 'NONE',  ( 102.9544237342424395, -27.85507949283302764, 176.4213395616249898 ) ) ;
#38175=CARTESIAN_POINT ( 'NONE',  ( 83.06670390244796920, -58.35344715994099829, 207.5838068554149913 ) ) ;
#38177=CARTESIAN_POINT ( 'NONE',  ( 111.6283393632454022, -28.07768985461837730, 55.68991099019593349 ) ) ;
#38178=LINE ( 'NONE', #16407, #15405 ) ;
#38179=DIRECTION ( 'NONE',  ( 9.351236661543306751E-17, -3.725950533538267725E-29, -1.000000000000000000 ) ) ;
#38180=ORIENTED_EDGE ( 'NONE', *, *, #65431, .F. ) ;
#38181=CARTESIAN_POINT ( 'NONE',  ( 41.56648329127399677, 0.2215528400590013880, 261.0426252759119734 ) ) ;
#38183=ORIENTED_EDGE ( 'NONE', *, *, #61358, .F. ) ;
#38184=EDGE_CURVE ( 'NONE', #75304, #26158, #41675, .T. ) ;
#38185=CARTESIAN_POINT ( 'NONE',  ( 109.2250051346758113, -28.10373483931914151, 196.3130118773259767 ) ) ;
#38186=VECTOR ( 'NONE', #88432, 1000.000000000000000 ) ;
#38187=CARTESIAN_POINT ( 'NONE',  ( 59.68306514483412428, -72.55903866283681225, 396.9756252759102040 ) ) ;
#38190=B_SPLINE_CURVE_WITH_KNOTS ( 'NONE', 3,
 ( #53854, #26627, #54303, #81623, #82070, #19820, #19373, #67966, #74782, #61583, #89320, #87970, #60239, #47501, #89772, #62038, #75238, #13013 ),
 .UNSPECIFIED., .F., .F.,
 ( 4, 2, 2, 2, 2, 2, 2, 2, 4 ),
 ( 0.000000000000000000, 0.06250000002888209116, 0.1250000000577641823, 0.1875000000866462735, 0.2500000001155283647, 0.3125000001444104836, 0.3750000001732925470, 0.4375000002021746104, 0.5000000002310567293 ),
 .UNSPECIFIED. ) ;
#38191=EDGE_CURVE ( 'NONE', #42224, #32980, #14612, .T. ) ;
#38192=EDGE_CURVE ( 'NONE', #39230, #63968, #67686, .T. ) ;
#38193=FACE_OUTER_BOUND ( 'NONE', #27834, .T. ) ;
#38194=CARTESIAN_POINT ( 'NONE',  ( 107.0664832912739968, -36.72944715994100306, 287.6356252759109680 ) ) ;
#38195=VERTEX_POINT ( 'NONE', #81156 ) ;
#38196=DIRECTION ( 'NONE',  ( -1.000000000000000078E-15, 1.000000000000000083E-30, 1.000000000000000000 ) ) ;
#38197=ADVANCED_FACE ( 'NONE', ( #49162 ), #74324, .T. ) ;
#38198=CARTESIAN_POINT ( 'NONE',  ( 97.81045233035079889, -40.51440448977106001, 37.63507460729699972 ) ) ;
#38199=EDGE_LOOP ( 'NONE', ( #83213, #78619, #32480, #18047 ) ) ;
#38200=CARTESIAN_POINT ( 'NONE',  ( 115.7579298488887076, -31.01215564512770229, 254.2899109901966028 ) ) ;
#38203=EDGE_CURVE ( 'NONE', #28839, #8744, #76894, .T. ) ;
#38204=CARTESIAN_POINT ( 'NONE',  ( 116.3170820643562564, -32.94538914428453324, 169.1356252759109680 ) ) ;
#38205=CARTESIAN_POINT ( 'NONE',  ( 48.45959712129000252, -28.98061976758940617, 313.9678068554150059 ) ) ;
#38208=CARTESIAN_POINT ( 'NONE',  ( 109.6164515631795524, -26.53946793531281756, 195.8813395616249977 ) ) ;
#38211=VERTEX_POINT ( 'NONE', #74764 ) ;
#38212=CARTESIAN_POINT ( 'NONE',  ( 112.8417677104678063, -27.25086138798909374, 45.62895860924398761 ) ) ;
#38213=CARTESIAN_POINT ( 'NONE',  ( 163.1639762274897976, -34.03355364505781466, 237.4678068554150059 ) ) ;
#38215=CARTESIAN_POINT ( 'NONE',  ( 115.6554515427140473, -30.75822225795367970, 279.3099109901966131 ) ) ;
#38216=ORIENTED_EDGE ( 'NONE', *, *, #34914, .T. ) ;
#38218=VECTOR ( 'NONE', #72808, 1000.000000000000000 ) ;
#38219=CARTESIAN_POINT ( 'NONE',  ( 80.94673009889297077, -16.12360705087681012, 1.744847597652003701 ) ) ;
#38220=CARTESIAN_POINT ( 'NONE',  ( 98.15087327529982986, -41.26140878761783881, 17.70046935524347376 ) ) ;
#38221=CARTESIAN_POINT ( 'NONE',  ( 105.7138906618339433, -46.72361789148295941, 152.4694709838751692 ) ) ;
#38222=CARTESIAN_POINT ( 'NONE',  ( 104.0433210460927000, -44.34148882339519560, 115.0938046553049503 ) ) ;
#38223=CARTESIAN_POINT ( 'NONE',  ( 107.2496171063691577, -24.85558036374148472, 226.0641967044829812 ) ) ;
#38225=EDGE_LOOP ( 'NONE', ( #23149, #88742, #50780, #29950 ) ) ;
#38226=CARTESIAN_POINT ( 'NONE',  ( 136.2737402105819911, -38.37320971852938101, 2.471387388682165565 ) ) ;
#38229=AXIS2_PLACEMENT_3D ( 'NONE', #81692, #30626, #71087 ) ;
#38230=DIRECTION ( 'NONE',  ( 0.7071067811865171526, 0.7071067811865779928, 7.071067811865164719E-16 ) ) ;
#38231=ORIENTED_EDGE ( 'NONE', *, *, #20579, .T. ) ;
#38232=ORIENTED_EDGE ( 'NONE', *, *, #20769, .T. ) ;
#38233=CARTESIAN_POINT ( 'NONE',  ( 194.5667039024479834, -67.87844715994100397, 20.91780685541479912 ) ) ;
#38236=CARTESIAN_POINT ( 'NONE',  ( 99.80400324059088746, -42.13953531443270606, 111.2705150661719671 ) ) ;
#38237=CARTESIAN_POINT ( 'NONE',  ( 97.03298259997053776, -33.74021148472603215, 31.09562527591097592 ) ) ;
#38239=DIRECTION ( 'NONE',  ( 4.299999999999999979E-14, -1.000000000000000000, 0.000000000000000000 ) ) ;
#38240=ORIENTED_EDGE ( 'NONE', *, *, #41219, .F. ) ;
#38243=DIRECTION ( 'NONE',  ( 0.000000000000000000, -1.000000000000000000, 0.000000000000000000 ) ) ;
#38244=CARTESIAN_POINT ( 'NONE',  ( 107.0664832912739968, -36.72944715994100306, 287.6356252759109680 ) ) ;
#38246=FACE_OUTER_BOUND ( 'NONE', #83781, .T. ) ;
#38247=AXIS2_PLACEMENT_3D ( 'NONE', #13020, #67516, #68430 ) ;
#38249=ORIENTED_EDGE ( 'NONE', *, *, #76975, .T. ) ;
#38250=CARTESIAN_POINT ( 'NONE',  ( 104.8412335932644766, -26.50818645216173408, 260.2470538473397710 ) ) ;
#38251=CARTESIAN_POINT ( 'NONE',  ( 96.64589536673427972, -32.90729728488415162, 17.03467289495896964 ) ) ;
#38258=CYLINDRICAL_SURFACE ( 'NONE', #51389, 5.599999999999994316 ) ;
#38259=DIRECTION ( 'NONE',  ( -0.7071067811865336949, -0.7071067811865614505, 0.000000000000000000 ) ) ;
#38260=CARTESIAN_POINT ( 'NONE',  ( 107.3678158256761179, -26.30747296201684549, 321.5865679059475610 ) ) ;
#38261=CARTESIAN_POINT ( 'NONE',  ( 163.0664832912739826, -18.82844715994099971, 333.4006252759120343 ) ) ;
#38262=CARTESIAN_POINT ( 'NONE',  ( 101.5858402103170590, -47.29319095008832363, 17.19562527591095247 ) ) ;
#38263=CARTESIAN_POINT ( 'NONE',  ( 97.40207042353749500, -40.63861732370358482, 202.6327681330539860 ) ) ;
#38264=CARTESIAN_POINT ( 'NONE',  ( 96.93562038266055936, -32.25163268508860881, 51.98324432352996638 ) ) ;
#38266=CARTESIAN_POINT ( 'NONE',  ( 46.83715912545429205, -47.82818131006082751, 249.9678068554150343 ) ) ;
#38267=CARTESIAN_POINT ( 'NONE',  ( 81.14852608520830302, -34.20116861175197442, 1.807989644435456400 ) ) ;
#38268=EDGE_CURVE ( 'NONE', #44745, #31084, #21944, .T. ) ;
#38269=VECTOR ( 'NONE', #21336, 1000.000000000000000 ) ;
#38270=VECTOR ( 'NONE', #83426, 1000.000000000000000 ) ;
#38272=CARTESIAN_POINT ( 'NONE',  ( 183.6524903400783444, -48.32844715993452667, 249.9678068554149775 ) ) ;
#38273=VERTEX_POINT ( 'NONE', #88856 ) ;
#38274=CARTESIAN_POINT ( 'NONE',  ( 98.20607846729137691, -32.50961293922097894, 71.97276813305397525 ) ) ;
#38275=CARTESIAN_POINT ( 'NONE',  ( 41.56670390244695312, -36.32844715994109208, 129.9678068554150911 ) ) ;
#38276=ORIENTED_EDGE ( 'NONE', *, *, #84094, .F. ) ;
#38277=CIRCLE ( 'NONE', #64362, 7.499999999999992895 ) ;
#38278=PLANE ( 'NONE',  #2619 ) ;
#38279=CARTESIAN_POINT ( 'NONE',  ( 103.7301789885933943, -26.21598454391068600, 201.3089586092439731 ) ) ;
#38280=CARTESIAN_POINT ( 'NONE',  ( 97.81021718220807770, -40.51802218317752846, 192.6354414398782353 ) ) ;
#38281=CARTESIAN_POINT ( 'NONE',  ( 110.8542886837690702, -45.98431238365922269, 147.8856095171690868 ) ) ;
#38286=CARTESIAN_POINT ( 'NONE',  ( 116.5394839232220505, -34.29517225379350975, 124.0270538473399426 ) ) ;
#38288=EDGE_LOOP ( 'NONE', ( #33045, #77514, #52566, #83049, #47703, #76566 ) ) ;
#38289=CARTESIAN_POINT ( 'NONE',  ( 111.6972492074939396, -29.17403283370891032, 91.07015473446894305 ) ) ;
#38290=LINE ( 'NONE', #64667, #16753 ) ;
#38291=CARTESIAN_POINT ( 'NONE',  ( 102.5357197525642192, -45.39752751535328201, 208.1927681330529651 ) ) ;
#38299=EDGE_CURVE ( 'NONE', #18892, #56405, #7845, .T. ) ;
#38301=CARTESIAN_POINT ( 'NONE',  ( 117.6812658759005217, -39.72780374360938538, 143.6194347997209775 ) ) ;
#38304=ORIENTED_EDGE ( 'NONE', *, *, #14781, .F. ) ;
#38305=EDGE_CURVE ( 'NONE', #2705, #72232, #50222, .T. ) ;
#38307=CARTESIAN_POINT ( 'NONE',  ( 116.3159136950847170, -32.94903743517052419, 150.1356252759109680 ) ) ;
#38310=VECTOR ( 'NONE', #34675, 1000.000000000000000 ) ;
#38312=VECTOR ( 'NONE', #24178, 1000.000000000000000 ) ;
#38313=CARTESIAN_POINT ( 'NONE',  ( 107.9182787209079919, -47.15539321873765743, 177.6413395616249886 ) ) ;
#38314=CARTESIAN_POINT ( 'NONE',  ( 151.5667039024485518, -48.82844715993590512, 180.4678068554149775 ) ) ;
#38315=ORIENTED_EDGE ( 'NONE', *, *, #42308, .F. ) ;
#38317=EDGE_LOOP ( 'NONE', ( #43572, #5337, #44310, #48514, #72136 ) ) ;
#38318=EDGE_CURVE ( 'NONE', #15093, #81490, #65435, .T. ) ;
#38319=CARTESIAN_POINT ( 'NONE',  ( 102.6169236507442974, -45.73916775254092215, 63.21228203591902428 ) ) ;
#38320=FACE_OUTER_BOUND ( 'NONE', #68652, .T. ) ;
#38321=CARTESIAN_POINT ( 'NONE',  ( 132.1570028295015220, -34.74831852142843047, 7.618261863067814943 ) ) ;
#38322=CARTESIAN_POINT ( 'NONE',  ( 101.2106992548341822, -44.07698544542078167, 268.4606309249448941 ) ) ;
#38323=CARTESIAN_POINT ( 'NONE',  ( 87.31648329127402519, -36.72944715994105991, -4.824374724089048883 ) ) ;
#38324=ORIENTED_EDGE ( 'NONE', *, *, #79233, .T. ) ;
#38326=CARTESIAN_POINT ( 'NONE',  ( 81.50686229671583760, -16.38644903112324869, 7.895285856720303919 ) ) ;
#38327=ORIENTED_EDGE ( 'NONE', *, *, #34187, .T. ) ;
#38328=ORIENTED_EDGE ( 'NONE', *, *, #36190, .F. ) ;
#38329=AXIS2_PLACEMENT_3D ( 'NONE', #85556, #38706, #45948 ) ;
#38331=VERTEX_POINT ( 'NONE', #16020 ) ;
#38335=CARTESIAN_POINT ( 'NONE',  ( 105.1568233002730182, -45.58189704936153674, 31.84194363760095570 ) ) ;
#38337=CARTESIAN_POINT ( 'NONE',  ( 117.2187229798756363, -34.26400738748503727, 209.0156252759109634 ) ) ;
#38338=CONICAL_SURFACE ( 'NONE', #58827, 11.57110091390439699, 0.7853981633974452814 ) ;
#38339=CARTESIAN_POINT ( 'NONE',  ( 102.7067583520260712, -46.86140753836549777, 137.2651490854349561 ) ) ;
#38340=CARTESIAN_POINT ( 'NONE',  ( 25.56670390244797275, -62.87844715994099687, 295.9678068554150059 ) ) ;
#38341=CARTESIAN_POINT ( 'NONE',  ( 111.6084932380418735, -46.11308361340533679, 243.9356252759109509 ) ) ;
#38342=DIRECTION ( 'NONE',  ( 0.7071067811865157093, 0.7071067811865794361, 7.071067811865461528E-16 ) ) ;
#38343=LINE ( 'NONE', #24722, #78746 ) ;
#38346=EDGE_CURVE ( 'NONE', #5969, #48953, #70759, .T. ) ;
#38347=CARTESIAN_POINT ( 'NONE',  ( 115.5532354207493171, -29.57487366316678745, 224.3718157521009573 ) ) ;
#38349=CARTESIAN_POINT ( 'NONE',  ( 97.67451187568107684, -41.25469890874477841, 171.6841967044819626 ) ) ;
#38353=DIRECTION ( 'NONE',  ( 1.000000000000000000, 0.000000000000000000, 9.462128050782575008E-16 ) ) ;
#38355=CARTESIAN_POINT ( 'NONE',  ( 41.56648329127398966, -27.82844715994070484, 18.92562527591200094 ) ) ;
#38356=CARTESIAN_POINT ( 'NONE',  ( 142.8698897858160706, -0.9167816978817300289, 540.9756252759101471 ) ) ;
#38357=CARTESIAN_POINT ( 'NONE',  ( 102.3890460933095454, -47.58756240099337731, 283.2527681330539053 ) ) ;
#38358=PLANE ( 'NONE',  #61214 ) ;
#38362=CARTESIAN_POINT ( 'NONE',  ( 167.6524903400755306, -48.32844715993520879, 180.4678068554150059 ) ) ;
#38363=CYLINDRICAL_SURFACE ( 'NONE', #33289, 2.517500000000005844 ) ;
#38364=CARTESIAN_POINT ( 'NONE',  ( 98.61271160274297642, -35.32052061661691056, 195.5838068554172082 ) ) ;
#38366=DIRECTION ( 'NONE',  ( -0.7071067812163274180, 0.7071067811567677275, -2.899137802742863655E-29 ) ) ;
#38367=CARTESIAN_POINT ( 'NONE',  ( 113.7648918053778715, -44.74678383396227588, 193.1299109901969757 ) ) ;
#38368=CARTESIAN_POINT ( 'NONE',  ( 115.1668113632844808, -43.29200554620488361, 84.28419670448195689 ) ) ;
#38369=CARTESIAN_POINT ( 'NONE',  ( 107.2499990610067329, -24.83081552997016317, 226.0641967044829812 ) ) ;
#38370=DIRECTION ( 'NONE',  ( 0.000000000000000000, 0.000000000000000000, -1.000000000000000000 ) ) ;
#38373=CARTESIAN_POINT ( 'NONE',  ( 115.9153499428093568, -41.43328348718500820, 39.43728031067852413 ) ) ;
#38374=CARTESIAN_POINT ( 'NONE',  ( 80.06648329127399677, -18.72944715994105991, -5.074374724089057764 ) ) ;
#38375=CARTESIAN_POINT ( 'NONE',  ( 62.03715912545744260, -47.82818131006020934, 117.4678068554150485 ) ) ;
#38376=AXIS2_PLACEMENT_3D ( 'NONE', #18153, #60374, #24975 ) ;
#38377=CARTESIAN_POINT ( 'NONE',  ( 97.70663229711287556, -40.25150714490782633, 66.61337454916048273 ) ) ;
#38378=EDGE_CURVE ( 'NONE', #13645, #45890, #63177, .T. ) ;
#38379=VECTOR ( 'NONE', #38578, 1000.000000000000000 ) ;
#38380=VERTEX_POINT ( 'NONE', #32300 ) ;
#38381=ORIENTED_EDGE ( 'NONE', *, *, #89567, .T. ) ;
#38382=CARTESIAN_POINT ( 'NONE',  ( 100.3410792892688761, -42.04179533522079026, 91.28099125664796532 ) ) ;
#38384=ORIENTED_EDGE ( 'NONE', *, *, #15684, .F. ) ;
#38385=CARTESIAN_POINT ( 'NONE',  ( 113.3016265961369697, -28.35762455946455773, 100.5670538473389684 ) ) ;
#38386=FACE_OUTER_BOUND ( 'NONE', #68713, .T. ) ;
#38387=DIRECTION ( 'NONE',  ( 0.7071067811874278686, -0.7071067811856670549, 6.612322855868390075E-17 ) ) ;
#38389=CARTESIAN_POINT ( 'NONE',  ( 115.3963617111076445, -41.85549503053864839, 18.38705384734096171 ) ) ;
#38392=ORIENTED_EDGE ( 'NONE', *, *, #68168, .F. ) ;
#38393=AXIS2_PLACEMENT_3D ( 'NONE', #72736, #17329, #44561 ) ;
#38394=DIRECTION ( 'NONE',  ( 0.000000000000000000, 1.000000000000000000, 0.000000000000000000 ) ) ;
#38396=LINE ( 'NONE', #52879, #81032 ) ;
#38397=CARTESIAN_POINT ( 'NONE',  ( 188.5667039024479834, -48.82844715994099971, 293.2178068554150627 ) ) ;
#38398=VECTOR ( 'NONE', #31985, 1000.000000000000000 ) ;
#38399=FACE_OUTER_BOUND ( 'NONE', #60775, .T. ) ;
#38400=CARTESIAN_POINT ( 'NONE',  ( 72.26949937496601706, -71.54137415153812185, 394.9756252759101471 ) ) ;
#38401=EDGE_CURVE ( 'NONE', #33618, #11918, #46813, .T. ) ;
#38402=AXIS2_PLACEMENT_3D ( 'NONE', #88765, #26523, #55092 ) ;
#38403=CARTESIAN_POINT ( 'NONE',  ( 71.06648329127399677, -8.729447159940999512, 17.92562527591199739 ) ) ;
#38406=DIRECTION ( 'NONE',  ( -1.000000000000000078E-15, 1.000000000000000083E-30, 1.000000000000000000 ) ) ;
#38407=CARTESIAN_POINT ( 'NONE',  ( 100.4250012405661039, -28.72198927997973783, 40.62705384733894221 ) ) ;
#38408=VERTEX_POINT ( 'NONE', #45471 ) ;
#38409=ADVANCED_FACE ( 'NONE', ( #25500, #80478 ), #12326, .T. ) ;
#38410=ORIENTED_EDGE ( 'NONE', *, *, #71354, .F. ) ;
#38414=CARTESIAN_POINT ( 'NONE',  ( 108.3053489883007927, -28.16931545225084221, 147.7918998934009664 ) ) ;
#38415=AXIS2_PLACEMENT_3D ( 'NONE', #27406, #12902, #19264 ) ;
#38416=DIRECTION ( 'NONE',  ( 1.000000000000000000, 0.000000000000000000, 0.000000000000000000 ) ) ;
#38419=EDGE_CURVE ( 'NONE', #70942, #74787, #31408, .T. ) ;
#38421=EDGE_LOOP ( 'NONE', ( #87159, #66098, #55395, #52270 ) ) ;
#38423=EDGE_CURVE ( 'NONE', #55083, #22706, #4166, .T. ) ;
#38424=CARTESIAN_POINT ( 'NONE',  ( 156.5667039024481255, -42.82844715993568485, 254.7178068554149490 ) ) ;
#38425=CARTESIAN_POINT ( 'NONE',  ( 113.7804517773139708, -30.94577135814159519, 180.8244404487539612 ) ) ;
#38426=DIRECTION ( 'NONE',  ( 0.7071067811865171526, 0.7071067811865779928, 7.071067811865475333E-16 ) ) ;
#38427=CARTESIAN_POINT ( 'NONE',  ( 25.56670390244797275, -62.87844715994099687, 293.2178068554150627 ) ) ;
#38428=VECTOR ( 'NONE', #78414, 1000.000000000000000 ) ;
#38430=ORIENTED_EDGE ( 'NONE', *, *, #70071, .F. ) ;
#38431=EDGE_LOOP ( 'NONE', ( #37223, #26036, #39783, #58328 ) ) ;
#38432=ORIENTED_EDGE ( 'NONE', *, *, #33170, .F. ) ;
#38433=CARTESIAN_POINT ( 'NONE',  ( 114.3567987304369495, -40.40109894280344349, 201.2738046553059803 ) ) ;
#38434=CARTESIAN_POINT ( 'NONE',  ( 109.2596401224901541, -46.98022400537049492, 107.7441967044829880 ) ) ;
#38435=CARTESIAN_POINT ( 'NONE',  ( 103.4847015977353379, -25.45917443855071838, 55.32133956162594046 ) ) ;
#38436=CARTESIAN_POINT ( 'NONE',  ( 108.3310854594628125, -46.73512723405534075, 252.6774446765812172 ) ) ;
#38437=CARTESIAN_POINT ( 'NONE',  ( 116.3232968930447839, -32.93863405887816498, 194.1356252759109680 ) ) ;
#38438=DIRECTION ( 'NONE',  ( 1.000000000000000000, 4.163336342344333240E-14, 0.000000000000000000 ) ) ;
#38439=CARTESIAN_POINT ( 'NONE',  ( 117.0170930581839457, -33.62013007832896960, 170.0670538473399631 ) ) ;
#38443=EDGE_LOOP ( 'NONE', ( #4037, #80466 ) ) ;
#38444=ORIENTED_EDGE ( 'NONE', *, *, #57475, .F. ) ;
#38445=DIRECTION ( 'NONE',  ( 1.000000000000000000, 2.999999999999999839E-15, 1.000000000000000078E-15 ) ) ;
#38446=EDGE_LOOP ( 'NONE', ( #15241, #5116, #26885, #5789 ) ) ;
#38448=LINE ( 'NONE', #24838, #83757 ) ;
#38451=AXIS2_PLACEMENT_3D ( 'NONE', #28008, #8484, #49344 ) ;
#38453=CARTESIAN_POINT ( 'NONE',  ( 105.9884003220067399, -26.36003215364494423, 50.15848241876796720 ) ) ;
#38457=DIRECTION ( 'NONE',  ( -1.000000000000000078E-15, 1.000000000000000083E-30, 1.000000000000000000 ) ) ;
#38458=DIRECTION ( 'NONE',  ( 0.000000000000000000, 0.000000000000000000, -1.000000000000000000 ) ) ;
#38459=CARTESIAN_POINT ( 'NONE',  ( 96.71749658230658042, -40.79275330125902599, 96.62419670448296927 ) ) ;
#38460=DIRECTION ( 'NONE',  ( 1.639958061481212836E-42, -4.100000000000000342E-29, -1.000000000000000000 ) ) ;
#38461=CARTESIAN_POINT ( 'NONE',  ( 116.9962961068553113, -33.62662860631130712, 170.0670538473399631 ) ) ;
#38462=CARTESIAN_POINT ( 'NONE',  ( 83.06670390244796920, -64.87844715994098976, 231.5838068554150198 ) ) ;
#38463=LINE ( 'NONE', #66167, #16297 ) ;
#38464=VERTEX_POINT ( 'NONE', #73192 ) ;
#38465=CARTESIAN_POINT ( 'NONE',  ( 164.9190312289449878, -35.91149509761181235, -5.074374724088000832 ) ) ;
#38466=VECTOR ( 'NONE', #33236, 1000.000000000000000 ) ;
#38467=CARTESIAN_POINT ( 'NONE',  ( 33.78309357196401663, -29.99615139349950965, 237.4678068554150059 ) ) ;
#38470=DIRECTION ( 'NONE',  ( -1.000000000000000078E-15, 1.000000000000000083E-30, 1.000000000000000000 ) ) ;
#38471=CARTESIAN_POINT ( 'NONE',  ( 101.1758151987629333, -45.38431258166273352, 197.1013395616249966 ) ) ;
#38472=ORIENTED_EDGE ( 'NONE', *, *, #57358, .T. ) ;
#38474=CARTESIAN_POINT ( 'NONE',  ( 103.9327720845255669, -26.76365000536165439, 246.3184824187679567 ) ) ;
#38475=CARTESIAN_POINT ( 'NONE',  ( 114.0511858335762270, -28.93156859308855644, 110.4956252759109816 ) ) ;
#38477=CARTESIAN_POINT ( 'NONE',  ( 81.77795131940523277, -38.88977919477280665, 7.751962620090976586 ) ) ;
#38478=CIRCLE ( 'NONE', #64562, 10.00000000000000711 ) ;
#38481=ORIENTED_EDGE ( 'NONE', *, *, #4149, .T. ) ;
#38486=ORIENTED_EDGE ( 'NONE', *, *, #75361, .T. ) ;
#38487=CARTESIAN_POINT ( 'NONE',  ( 117.0608945231560654, -38.08045312473117860, 73.71895860893197039 ) ) ;
#38488=CARTESIAN_POINT ( 'NONE',  ( 115.0547525607699697, -30.03093676393617173, 265.3813395616251682 ) ) ;
#38489=CARTESIAN_POINT ( 'NONE',  ( 119.0814029968458811, -31.76540601701525901, 293.6369201390379544 ) ) ;
#38490=CARTESIAN_POINT ( 'NONE',  ( 124.7998166246059810, 12.92155284005730387, 358.9756252759109998 ) ) ;
#38493=DIRECTION ( 'NONE',  ( 4.299999999999999979E-14, -1.000000000000000000, 4.400000000000000367E-29 ) ) ;
#38494=CARTESIAN_POINT ( 'NONE',  ( 112.1400416112072946, -28.01322161120737064, 149.6567520850730943 ) ) ;
#38495=CARTESIAN_POINT ( 'NONE',  ( 115.0883484252707376, -39.66301350383546520, 217.9695626852199837 ) ) ;
#38496=ORIENTED_EDGE ( 'NONE', *, *, #74313, .T. ) ;
#38497=EDGE_LOOP ( 'NONE', ( #43797, #74853, #13295 ) ) ;
#38499=ORIENTED_EDGE ( 'NONE', *, *, #17102, .T. ) ;
#38501=VECTOR ( 'NONE', #11569, 1000.000000000000000 ) ;
#38502=CARTESIAN_POINT ( 'NONE',  ( 99.50485777685048561, -43.30593340888767528, 181.8960846843701802 ) ) ;
#38503=EDGE_CURVE ( 'NONE', #24616, #30145, #86705, .T. ) ;
#38505=CARTESIAN_POINT ( 'NONE',  ( 106.3742716537777113, -27.86474340539431793, 21.57015473446893949 ) ) ;
#38507=CARTESIAN_POINT ( 'NONE',  ( 45.77381068363526850, -48.62134037875087245, 300.4678068554150059 ) ) ;
#38508=ADVANCED_FACE ( 'NONE', ( #25956 ), #74998, .F. ) ;
#38509=DIRECTION ( 'NONE',  ( 0.000000000000000000, -1.000000000000000000, 0.000000000000000000 ) ) ;
#38511=CARTESIAN_POINT ( 'NONE',  ( 103.2771927011866637, -27.47518992547664141, 56.38573900610595047 ) ) ;
#38512=ORIENTED_EDGE ( 'NONE', *, *, #55287, .T. ) ;
#38514=CARTESIAN_POINT ( 'NONE',  ( 105.0496896133374918, -44.66766052993097702, 45.19666179816294971 ) ) ;
#38519=VECTOR ( 'NONE', #31248, 1000.000000000000114 ) ;
#38523=ORIENTED_EDGE ( 'NONE', *, *, #44746, .T. ) ;
#38524=CARTESIAN_POINT ( 'NONE',  ( 107.0664832912750057, -36.72944715993903486, 9.125625275910969947 ) ) ;
#38528=CARTESIAN_POINT ( 'NONE',  ( 114.7262375871959392, -43.80158930977980702, 123.2327681330539519 ) ) ;
#38529=ORIENTED_EDGE ( 'NONE', *, *, #38419, .F. ) ;
#38531=CARTESIAN_POINT ( 'NONE',  ( 98.14502816950557929, -38.28518133910327492, 45.87432458998197404 ) ) ;
#38532=EDGE_CURVE ( 'NONE', #64255, #40462, #75897, .T. ) ;
#38533=AXIS2_PLACEMENT_3D ( 'NONE', #68792, #6129, #74267 ) ;
#38534=CARTESIAN_POINT ( 'NONE',  ( 115.7201795117171628, -41.77810559249323319, 89.40546331780193157 ) ) ;
#38535=CARTESIAN_POINT ( 'NONE',  ( 99.86128698970316009, -42.75951115570669714, 68.30063092494498278 ) ) ;
#38536=CARTESIAN_POINT ( 'NONE',  ( 135.9140641843780202, -20.77438500681861910, 2.186796636981966468 ) ) ;
#38537=CARTESIAN_POINT ( 'NONE',  ( 33.91903122894598965, -35.91149509761320502, 342.9256252759109884 ) ) ;
#38538=ADVANCED_FACE ( 'NONE', ( #49058 ), #84068, .T. ) ;
#38540=CARTESIAN_POINT ( 'NONE',  ( 111.4245298313290107, -46.22390286880558818, 23.91848241876792969 ) ) ;
#38542=VERTEX_POINT ( 'NONE', #61352 ) ;
#38545=CARTESIAN_POINT ( 'NONE',  ( 77.58678459499434155, -19.92005462651998826, 2.747931806390634168 ) ) ;
#38547=VECTOR ( 'NONE', #56358, 1000.000000000000000 ) ;
#38549=FACE_OUTER_BOUND ( 'NONE', #10189, .T. ) ;
#38550=ORIENTED_EDGE ( 'NONE', *, *, #25364, .F. ) ;
#38551=CARTESIAN_POINT ( 'NONE',  ( 103.5361331145922890, -27.60804031003065262, 215.3699109901969848 ) ) ;
#38554=CARTESIAN_POINT ( 'NONE',  ( 103.4771999316985500, -25.43557003456049870, 51.32133956162493149 ) ) ;
#38556=ORIENTED_EDGE ( 'NONE', *, *, #59814, .F. ) ;
#38557=CARTESIAN_POINT ( 'NONE',  ( 103.9658006590860992, -27.21632154753857691, 171.3272140054234853 ) ) ;
#38558=DIRECTION ( 'NONE',  ( 1.639958061481212836E-42, -4.100000000000000342E-29, -1.000000000000000000 ) ) ;
#38559=VERTEX_POINT ( 'NONE', #76790 ) ;
#38560=DIRECTION ( 'NONE',  ( 9.351236661543306751E-17, -3.725950533538267725E-29, -1.000000000000000000 ) ) ;
#38561=CARTESIAN_POINT ( 'NONE',  ( 179.7974245136209959, -36.32844715993469009, 193.9678068554150059 ) ) ;
#38562=CARTESIAN_POINT ( 'NONE',  ( 117.4688788178166732, -35.86077403649778006, 253.8927681330538348 ) ) ;
#38563=AXIS2_PLACEMENT_3D ( 'NONE', #12527, #24814, #46474 ) ;
#38564=CARTESIAN_POINT ( 'NONE',  ( 32.06670390244660496, -32.29483332968541731, 313.9678068554150059 ) ) ;
#38567=CARTESIAN_POINT ( 'NONE',  ( 77.33253953643580303, -37.07457063615774473, 3.076560393663061443 ) ) ;
#38568=CARTESIAN_POINT ( 'NONE',  ( 105.3911398957759076, -27.82967838469355115, 279.6590864947435762 ) ) ;
#38569=CARTESIAN_POINT ( 'NONE',  ( 119.5435152932140426, -31.57448135767196362, 290.1356252759106837 ) ) ;
#38570=CARTESIAN_POINT ( 'NONE',  ( 115.1902516771092451, -44.19056033372781656, 74.22324432352993995 ) ) ;
#38572=CARTESIAN_POINT ( 'NONE',  ( 98.42220671263785903, -30.82325138971081557, 120.8499109901969604 ) ) ;
#38573=EDGE_LOOP ( 'NONE', ( #66133, #60164, #83433, #68475, #78547, #25003, #53534, #49778, #573, #14199, #89047, #51718 ) ) ;
#38574=DIRECTION ( 'NONE',  ( 0.000000000000000000, 1.000000000000000000, 0.000000000000000000 ) ) ;
#38575=VERTEX_POINT ( 'NONE', #61798 ) ;
#38578=DIRECTION ( 'NONE',  ( -0.7071067811864676367, -0.7071067811866273978, -7.071067811864981309E-16 ) ) ;
#38580=CARTESIAN_POINT ( 'NONE',  ( 97.81169138727440782, -40.51741131469341184, 51.63568823874075520 ) ) ;
#38581=CARTESIAN_POINT ( 'NONE',  ( 118.9539009387050186, -36.16544432761327954, 118.8641967044819836 ) ) ;
#38582=VERTEX_POINT ( 'NONE', #89535 ) ;
#38583=CARTESIAN_POINT ( 'NONE',  ( 63.03715912545741418, -46.82818131006016671, 116.4678068554151054 ) ) ;
#38586=CARTESIAN_POINT ( 'NONE',  ( 134.0664832912740110, -8.350947159940998787, 296.1531252759119752 ) ) ;
#38587=AXIS2_PLACEMENT_3D ( 'NONE', #31929, #12852, #60519 ) ;
#38588=ORIENTED_EDGE ( 'NONE', *, *, #63517, .F. ) ;
#38589=CARTESIAN_POINT ( 'NONE',  ( 98.43795593625375773, -42.68233540891471023, 126.8070538473389490 ) ) ;
#38590=VECTOR ( 'NONE', #31803, 1000.000000000000000 ) ;
#38592=EDGE_CURVE ( 'NONE', #36440, #27470, #14119, .T. ) ;
#38593=( LENGTH_UNIT ( ) NAMED_UNIT ( * ) SI_UNIT ( .MILLI., .METRE. ) );
#38595=LINE ( 'NONE', #4080, #54432 ) ;
#38596=ADVANCED_FACE ( 'NONE', ( #41795 ), #47717, .T. ) ;
#38599=EDGE_CURVE ( 'NONE', #64255, #44076, #56321, .T. ) ;
#38600=ORIENTED_EDGE ( 'NONE', *, *, #81571, .T. ) ;
#38601=DIRECTION ( 'NONE',  ( 0.000000000000000000, 1.000000000000000000, 0.000000000000000000 ) ) ;
#38603=CARTESIAN_POINT ( 'NONE',  ( 180.3503142329310265, -29.99615139349890569, -5.074374724088000832 ) ) ;
#38604=EDGE_CURVE ( 'NONE', #87723, #40273, #60547, .T. ) ;
#38605=EDGE_CURVE ( 'NONE', #5006, #56141, #56593, .T. ) ;
#38607=DIRECTION ( 'NONE',  ( -1.000000000000000078E-15, 0.000000000000000000, 1.000000000000000000 ) ) ;
#38610=EDGE_CURVE ( 'NONE', #57647, #46563, #72182, .T. ) ;
#38612=AXIS2_PLACEMENT_3D ( 'NONE', #51119, #50680, #17941 ) ;
#38613=CYLINDRICAL_SURFACE ( 'NONE', #34627, 0.5000000000000004441 ) ;
#38614=EDGE_CURVE ( 'NONE', #8963, #12604, #56261, .T. ) ;
#38615=CARTESIAN_POINT ( 'NONE',  ( 113.3375292005773929, -44.23527279707077042, 189.1299109901959525 ) ) ;
#38616=LINE ( 'NONE', #81764, #9509 ) ;
#38617=ORIENTED_EDGE ( 'NONE', *, *, #74580, .T. ) ;
#38618=CARTESIAN_POINT ( 'NONE',  ( 116.8124865092210456, -37.88235468918157522, 49.73276813305294297 ) ) ;
#38619=CARTESIAN_POINT ( 'NONE',  ( 104.4079370647588547, -46.45804145048838052, 52.36485282198370328 ) ) ;
#38620=DIRECTION ( 'NONE',  ( 4.194175870806139918E-14, -1.000000000000000000, 0.000000000000000000 ) ) ;
#38621=EDGE_CURVE ( 'NONE', #62011, #13421, #82731, .T. ) ;
#38622=CARTESIAN_POINT ( 'NONE',  ( 179.8608231853568213, -35.55794170701179269, 237.4678068554150059 ) ) ;
#38626=ORIENTED_EDGE ( 'NONE', *, *, #28415, .T. ) ;
#38627=CARTESIAN_POINT ( 'NONE',  ( 107.2166699364993292, -45.61986748510933865, 209.0215833058969963 ) ) ;
#38628=DIRECTION ( 'NONE',  ( 0.7071067811865046071, 0.7071067811865904273, 7.071067811865039488E-16 ) ) ;
#38630=DIRECTION ( 'NONE',  ( 0.000000000000000000, 0.000000000000000000, -1.000000000000000000 ) ) ;
#38632=ORIENTED_EDGE ( 'NONE', *, *, #63522, .T. ) ;
#38634=CARTESIAN_POINT ( 'NONE',  ( 99.09325496367249286, -30.55370301960245527, 36.80227106180009145 ) ) ;
#38635=ORIENTED_EDGE ( 'NONE', *, *, #41981, .F. ) ;
#38636=CARTESIAN_POINT ( 'NONE',  ( 102.7552189479022928, -25.69072042043729098, 20.37276813305294354 ) ) ;
#38641=CARTESIAN_POINT ( 'NONE',  ( 31.71315051185499811, -33.70561438052090608, -5.074374724088000832 ) ) ;
#38642=DIRECTION ( 'NONE',  ( -0.7071067811866279529, 0.7071067811864671926, -7.071067811866286874E-16 ) ) ;
#38644=EDGE_CURVE ( 'NONE', #51938, #73307, #34994, .T. ) ;
#38645=AXIS2_PLACEMENT_3D ( 'NONE', #63820, #1598, #29303 ) ;
#38646=CARTESIAN_POINT ( 'NONE',  ( 110.7114656039092893, -48.05751922203765503, 203.8241967044819489 ) ) ;
#38651=CARTESIAN_POINT ( 'NONE',  ( 96.67154112854022685, -38.24047072676557946, 62.44133956162495025 ) ) ;
#38652=VECTOR ( 'NONE', #56961, 1000.000000000000000 ) ;
#38653=DIRECTION ( 'NONE',  ( 0.000000000000000000, 0.000000000000000000, -1.000000000000000000 ) ) ;
#38654=AXIS2_PLACEMENT_3D ( 'NONE', #12733, #4571, #67688 ) ;
#38655=VERTEX_POINT ( 'NONE', #28176 ) ;
#38657=ORIENTED_EDGE ( 'NONE', *, *, #53234, .F. ) ;
#38658=CARTESIAN_POINT ( 'NONE',  ( 80.06648329127399677, -15.97944715994105813, 1.625625275910943746 ) ) ;
#38659=CARTESIAN_POINT ( 'NONE',  ( 116.8182710663954254, -34.15736811344609691, 154.0318915783644513 ) ) ;
#38660=CARTESIAN_POINT ( 'NONE',  ( 111.9717725103620722, -43.25385221418022752, 140.9080903695919460 ) ) ;
#38661=CARTESIAN_POINT ( 'NONE',  ( 107.5109549264149251, -47.16686560604517098, 233.6099109901969655 ) ) ;
#38664=CIRCLE ( 'NONE', #5288, 2.517500000000005844 ) ;
#38665=CARTESIAN_POINT ( 'NONE',  ( 136.6368519841214777, -37.70758306363786971, 2.855952960430258258 ) ) ;
#38667=ORIENTED_EDGE ( 'NONE', *, *, #13261, .F. ) ;
#38668=FACE_OUTER_BOUND ( 'NONE', #18583, .T. ) ;
#38670=VERTEX_POINT ( 'NONE', #33662 ) ;
#38671=FACE_OUTER_BOUND ( 'NONE', #25458, .T. ) ;
#38673=CARTESIAN_POINT ( 'NONE',  ( 99.09504479792080645, -30.55131775994448873, 25.80237912473876349 ) ) ;
#38674=CARTESIAN_POINT ( 'NONE',  ( 113.1264120695652622, -29.99967374510735141, 158.9276579233149391 ) ) ;
#38675=CARTESIAN_POINT ( 'NONE',  ( 116.1968789481791191, -43.04691504047773520, 13.35657765686298859 ) ) ;
#38676=EDGE_LOOP ( 'NONE', ( #5589, #21526, #12030, #148 ) ) ;
#38681=CARTESIAN_POINT ( 'NONE',  ( 83.06670390244802604, -43.72944715994108122, 231.5838068554169524 ) ) ;
#38683=DIRECTION ( 'NONE',  ( 0.000000000000000000, 0.000000000000000000, 1.000000000000000000 ) ) ;
#38684=EDGE_CURVE ( 'NONE', #38195, #84879, #35439, .T. ) ;
#38685=AXIS2_PLACEMENT_3D ( 'NONE', #8782, #1517, #77360 ) ;
#38686=LINE ( 'NONE', #39583, #10360 ) ;
#38688=CARTESIAN_POINT ( 'NONE',  ( 99.04884357002234196, -44.37228004027687689, 36.92038718067297509 ) ) ;
#38689=CARTESIAN_POINT ( 'NONE',  ( 115.7091107927249283, -43.69381994074442588, 39.27467289495895386 ) ) ;
#38693=CARTESIAN_POINT ( 'NONE',  ( 105.9487191471789060, -25.32458681355470276, 323.3977233678749030 ) ) ;
#38695=DIRECTION ( 'NONE',  ( 0.000000000000000000, 0.000000000000000000, 1.000000000000000000 ) ) ;
#38696=CARTESIAN_POINT ( 'NONE',  ( 133.6896269580427656, -39.47945062088879808, 8.225625248534990774 ) ) ;
#38697=ADVANCED_FACE ( 'NONE', ( #84526 ), #37248, .T. ) ;
#38698=DIRECTION ( 'NONE',  ( 0.000000000000000000, 0.000000000000000000, 1.000000000000000000 ) ) ;
#38701=CARTESIAN_POINT ( 'NONE',  ( 115.6474790210939290, -28.48352029850561706, 39.43562527591099354 ) ) ;
#38702=CARTESIAN_POINT ( 'NONE',  ( 101.3491664457538945, -46.18916536780651683, 198.1318157521009482 ) ) ;
#38703=CARTESIAN_POINT ( 'NONE',  ( 104.0364404988798270, -47.38327494250712135, 63.36800622829197494 ) ) ;
#38706=DIRECTION ( 'NONE',  ( 0.000000000000000000, 0.000000000000000000, 1.000000000000000000 ) ) ;
#38707=LINE ( 'NONE', #61390, #78456 ) ;
#38708=EDGE_CURVE ( 'NONE', #52826, #30532, #80949, .T. ) ;
#38709=AXIS2_PLACEMENT_3D ( 'NONE', #70217, #7989, #28890 ) ;
#38710=VECTOR ( 'NONE', #60988, 1000.000000000000000 ) ;
#38711=AXIS2_PLACEMENT_3D ( 'NONE', #74850, #38971, #18526 ) ;
#38713=CARTESIAN_POINT ( 'NONE',  ( 97.31584368363401438, -39.30597587385430103, 187.5314585990350906 ) ) ;
#38714=ORIENTED_EDGE ( 'NONE', *, *, #53476, .T. ) ;
#38715=EDGE_CURVE ( 'NONE', #43667, #43353, #12795, .T. ) ;
#38716=CARTESIAN_POINT ( 'NONE',  ( 102.5967720069230893, -27.99243076246528261, 116.4527681330529703 ) ) ;
#38718=ORIENTED_EDGE ( 'NONE', *, *, #53885, .T. ) ;
#38719=CARTESIAN_POINT ( 'NONE',  ( 21.03689327557705369, -23.42844715994186089, 313.9678068554150059 ) ) ;
#38720=CARTESIAN_POINT ( 'NONE',  ( 111.1189502094634776, -27.14789314160936229, 240.7584824187679544 ) ) ;
#38721=DIRECTION ( 'NONE',  ( 0.000000000000000000, 0.000000000000000000, -1.000000000000000000 ) ) ;
#38725=DIRECTION ( 'NONE',  ( 0.000000000000000000, 0.000000000000000000, 1.000000000000000000 ) ) ;
#38726=ADVANCED_FACE ( 'NONE', ( #9989 ), #30875, .F. ) ;
#38729=VECTOR ( 'NONE', #72655, 1000.000000000000000 ) ;
#38730=CARTESIAN_POINT ( 'NONE',  ( 98.64540312569886282, -41.76920806142285159, 161.7556252759109725 ) ) ;
#38731=ORIENTED_EDGE ( 'NONE', *, *, #10532, .T. ) ;
#38732=ORIENTED_EDGE ( 'NONE', *, *, #39133, .T. ) ;
#38733=CARTESIAN_POINT ( 'NONE',  ( 112.4631721614844651, -29.03839555594388955, 81.00920235351600240 ) ) ;
#38734=AXIS2_PLACEMENT_3D ( 'NONE', #32828, #54587, #61866 ) ;
#38735=LINE ( 'NONE', #30149, #22597 ) ;
#38736=CARTESIAN_POINT ( 'NONE',  ( 97.17009264939177626, -31.66255117090388538, 241.9499109901959741 ) ) ;
#38737=FACE_OUTER_BOUND ( 'NONE', #41504, .T. ) ;
#38740=B_SPLINE_CURVE_WITH_KNOTS ( 'NONE', 3,
 ( #76986, #82914, #40657, #6156, #48796, #61540, #55153, #75189, #12970, #221, #20675, #48343, #14766, #56059, #19774, #89276, #82024, #55602 ),
 .UNSPECIFIED., .F., .F.,
 ( 4, 2, 2, 2, 2, 2, 2, 2, 4 ),
 ( 0.4999695546683612934, 0.5624733603348160971, 0.6249771660012709562, 0.6874809716677258153, 0.7499847773341805635, 0.8124885830006354226, 0.8749923886670902817, 0.9374961943335451409, 1.000000000000000000 ),
 .UNSPECIFIED. ) ;
#38743=LINE ( 'NONE', #53237, #1429 ) ;
#38744=FACE_OUTER_BOUND ( 'NONE', #17150, .T. ) ;
#38745=CARTESIAN_POINT ( 'NONE',  ( 109.3536845750984412, -25.93905639472648872, 184.9222919425779708 ) ) ;
#38746=VERTEX_POINT ( 'NONE', #65395 ) ;
#38747=ORIENTED_EDGE ( 'NONE', *, *, #70202, .F. ) ;
#38748=DIRECTION ( 'NONE',  ( 0.000000000000000000, 0.000000000000000000, -1.000000000000000000 ) ) ;
#38750=DIRECTION ( 'NONE',  ( 0.000000000000000000, 0.000000000000000000, 1.000000000000000000 ) ) ;
#38752=EDGE_CURVE ( 'NONE', #223, #55129, #15476, .T. ) ;
#38755=DIRECTION ( 'NONE',  ( 1.000000000000000000, 0.000000000000000000, 0.000000000000000000 ) ) ;
#38756=CARTESIAN_POINT ( 'NONE',  ( 106.9749943965245365, -47.15435292659226718, 187.5699109901969734 ) ) ;
#38757=DIRECTION ( 'NONE',  ( 0.000000000000000000, 0.000000000000000000, -1.000000000000000000 ) ) ;
#38759=ORIENTED_EDGE ( 'NONE', *, *, #40752, .F. ) ;
#38761=CARTESIAN_POINT ( 'NONE',  ( 98.40642892645681172, -41.73694030736349703, 62.74414883732655568 ) ) ;
#38762=LINE ( 'NONE', #73738, #57261 ) ;
#38763=DIRECTION ( 'NONE',  ( 1.000000000000000000, 4.163336342344333240E-14, 0.000000000000000000 ) ) ;
#38764=CARTESIAN_POINT ( 'NONE',  ( 106.2223766104409037, -28.61050573088338922, 47.97666179816295795 ) ) ;
#38765=CARTESIAN_POINT ( 'NONE',  ( 188.5667039024479834, -65.37844715994100397, 142.0928068554150059 ) ) ;
#38768=AXIS2_PLACEMENT_3D ( 'NONE', #63934, #8072, #57550 ) ;
#38769=DIRECTION ( 'NONE',  ( -0.9254794337955620787, -0.3787978585227822492, 0.000000000000000000 ) ) ;
#38771=ORIENTED_EDGE ( 'NONE', *, *, #24983, .T. ) ;
#38772=ORIENTED_EDGE ( 'NONE', *, *, #27601, .T. ) ;
#38774=VECTOR ( 'NONE', #81097, 1000.000000000000000 ) ;
#38776=ORIENTED_EDGE ( 'NONE', *, *, #10196, .T. ) ;
#38779=CARTESIAN_POINT ( 'NONE',  ( 97.39259002536323351, -35.90094442973985167, 35.68099125664797810 ) ) ;
#38780=CARTESIAN_POINT ( 'NONE',  ( 107.6557532049571932, -47.79055931493532938, 197.6308633711489620 ) ) ;
#38781=CARTESIAN_POINT ( 'NONE',  ( 101.9826776100855454, -46.51815199768669373, 167.1832443235299763 ) ) ;
#38783=FACE_OUTER_BOUND ( 'NONE', #22806, .T. ) ;
#38784=CARTESIAN_POINT ( 'NONE',  ( 117.4297252914212066, -35.59555830959087075, 274.9127681330538735 ) ) ;
#38785=CARTESIAN_POINT ( 'NONE',  ( 42.66648329127298922, 12.92155284005730387, 358.9756252759109998 ) ) ;
#38789=ORIENTED_EDGE ( 'NONE', *, *, #67409, .T. ) ;
#38790=VECTOR ( 'NONE', #25909, 1000.000000000000000 ) ;
#38792=CIRCLE ( 'NONE', #38734, 3.300000000000000711 ) ;
#38793=CARTESIAN_POINT ( 'NONE',  ( 97.81556692073944248, -40.52688746123195074, 111.6364388057383792 ) ) ;
#38794=CARTESIAN_POINT ( 'NONE',  ( 104.3127904766024443, -25.97630531626002437, 245.2880062282919482 ) ) ;
#38795=ORIENTED_EDGE ( 'NONE', *, *, #22416, .T. ) ;
#38796=CARTESIAN_POINT ( 'NONE',  ( 96.67388729539801773, -35.53787041403403180, 206.2356252759109623 ) ) ;
#38797=CARTESIAN_POINT ( 'NONE',  ( 134.0664832912740110, 0.2215528400590013880, 311.1531252759119752 ) ) ;
#38800=CARTESIAN_POINT ( 'NONE',  ( 176.7669697523282935, -48.62818131005432321, 300.4678068554149490 ) ) ;
#38801=ADVANCED_FACE ( 'NONE', ( #2288 ), #8657, .F. ) ;
#38802=CARTESIAN_POINT ( 'NONE',  ( 191.6377717143134873, -67.87844715994100397, 13.84673904354932006 ) ) ;
#38803=DIRECTION ( 'NONE',  ( 0.000000000000000000, 0.000000000000000000, 1.000000000000000000 ) ) ;
#38804=CARTESIAN_POINT ( 'NONE',  ( 100.2615012876618295, -45.41023301258249489, 273.0594347997205773 ) ) ;
#38805=CARTESIAN_POINT ( 'NONE',  ( 163.2449138992999735, -32.11662333284611748, -5.074374724088000832 ) ) ;
#38808=DIRECTION ( 'NONE',  ( 0.000000000000000000, 0.000000000000000000, 1.000000000000000000 ) ) ;
#38809=ADVANCED_FACE ( 'NONE', ( #57223 ), #72218, .T. ) ;
#38810=FACE_OUTER_BOUND ( 'NONE', #11978, .T. ) ;
#38815=ADVANCED_FACE ( 'NONE', ( #42689 ), #58560, .T. ) ;
#38816=DIRECTION ( 'NONE',  ( 0.000000000000000000, 1.000000000000000000, 0.000000000000000000 ) ) ;
#38817=CARTESIAN_POINT ( 'NONE',  ( 114.1397626436471171, -29.04081378529519597, 199.4841967044819739 ) ) ;
#38818=CARTESIAN_POINT ( 'NONE',  ( 96.02786343543940006, -37.29764797185995207, 117.3794347997199594 ) ) ;
#38819=CARTESIAN_POINT ( 'NONE',  ( 109.9722659835539389, -48.26927123350142779, 238.7727681330539724 ) ) ;
#38820=DIRECTION ( 'NONE',  ( 1.000000000000000078E-15, 0.000000000000000000, -1.000000000000000000 ) ) ;
#38821=DIRECTION ( 'NONE',  ( 4.299999999999999979E-14, -1.000000000000000000, 0.000000000000000000 ) ) ;
#38822=DIRECTION ( 'NONE',  ( -1.907762142705490052E-15, -7.167082501179359715E-16, 1.000000000000000000 ) ) ;
#38826=AXIS2_PLACEMENT_3D ( 'NONE', #48144, #6384, #27273 ) ;
#38827=CARTESIAN_POINT ( 'NONE',  ( 132.3573525511424691, -20.88611802718810395, 2.101554303219792086 ) ) ;
#38831=CARTESIAN_POINT ( 'NONE',  ( 106.2553484193443865, -46.40481216151710697, 111.9324198280769735 ) ) ;
#38833=EDGE_LOOP ( 'NONE', ( #12786, #71605, #35717, #1955 ) ) ;
#38834=CARTESIAN_POINT ( 'NONE',  ( 98.29923130492889527, -31.06375673945267124, 141.8699109901969564 ) ) ;
#38835=CARTESIAN_POINT ( 'NONE',  ( 182.3467384525650061, -29.62846900982231446, -5.074374724088000832 ) ) ;
#38836=CARTESIAN_POINT ( 'NONE',  ( 79.32178306376293619, -16.08035908359608612, 8.141856907855881786 ) ) ;
#38837=DIRECTION ( 'NONE',  ( -1.000000000000000078E-15, 1.000000000000000083E-30, 1.000000000000000000 ) ) ;
#38838=CARTESIAN_POINT ( 'NONE',  ( 151.5667039024485518, -48.82844715993590512, 180.4678068554149775 ) ) ;
#38839=CARTESIAN_POINT ( 'NONE',  ( 114.7041265136728612, -43.74408836545399737, 78.22324432353094892 ) ) ;
#38840=VERTEX_POINT ( 'NONE', #64508 ) ;
#38845=CARTESIAN_POINT ( 'NONE',  ( 107.8912859324307192, -26.39220933555703752, 111.0251490854339806 ) ) ;
#38846=CARTESIAN_POINT ( 'NONE',  ( 25.56670390244797275, -67.87844715994100397, 137.2178068554150059 ) ) ;
#38847=DIRECTION ( 'NONE',  ( 4.237773401492740281E-14, -1.000000000000000000, 0.000000000000000000 ) ) ;
#38849=CARTESIAN_POINT ( 'NONE',  ( 32.16397622746000451, -34.03355364505800651, -5.074374724088000832 ) ) ;
#38850=AXIS2_PLACEMENT_3D ( 'NONE', #39853, #47559, #82124 ) ;
#38852=FACE_OUTER_BOUND ( 'NONE', #88958, .T. ) ;
#38853=CARTESIAN_POINT ( 'NONE',  ( 107.8666756518570935, -26.35696637107986717, 70.01562527591099183 ) ) ;
#38854=ORIENTED_EDGE ( 'NONE', *, *, #70925, .F. ) ;
#38855=EDGE_LOOP ( 'NONE', ( #39864, #25332, #68907, #35789 ) ) ;
#38856=CIRCLE ( 'NONE', #44615, 2.999999999999999112 ) ;
#38857=LINE ( 'NONE', #66564, #41554 ) ;
#38858=DIRECTION ( 'NONE',  ( -1.000000000000000000, -1.000000000000000078E-15, -1.000000000000000078E-15 ) ) ;
#38863=CARTESIAN_POINT ( 'NONE',  ( 99.93348902297414327, -31.82829241803101894, 163.6776141791149826 ) ) ;
#38864=CIRCLE ( 'NONE', #50468, 12.99999999999999822 ) ;
#38866=CARTESIAN_POINT ( 'NONE',  ( 87.06648329127389729, -54.72944906728955772, -4.970821333495855754 ) ) ;
#38867=ORIENTED_EDGE ( 'NONE', *, *, #39421, .F. ) ;
#38868=VERTEX_POINT ( 'NONE', #2734 ) ;
#38869=DIRECTION ( 'NONE',  ( 1.000000000000000000, 4.272717921125146745E-14, 0.000000000000000000 ) ) ;
#38872=DIRECTION ( 'NONE',  ( -0.3787978585227821382, 0.9254794337955621897, 0.000000000000000000 ) ) ;
#38873=CARTESIAN_POINT ( 'NONE',  ( 107.2218274976867463, -26.65737820016106951, 226.4958690201829654 ) ) ;
#38875=VECTOR ( 'NONE', #12860, 1000.000000000000000 ) ;
#38881=ADVANCED_FACE ( 'NONE', ( #9103 ), #58129, .F. ) ;
#38882=ORIENTED_EDGE ( 'NONE', *, *, #22230, .T. ) ;
#38884=CARTESIAN_POINT ( 'NONE',  ( 114.3355458017429811, -42.49630604348746488, 196.1109475124489450 ) ) ;
#38885=CARTESIAN_POINT ( 'NONE',  ( 114.7877796877764922, -44.67155160988957618, 118.2022919425779719 ) ) ;
#38886=CARTESIAN_POINT ( 'NONE',  ( 117.4257108620838181, -37.68603989742254612, 78.75276813305399060 ) ) ;
#38888=LINE ( 'NONE', #10734, #8387 ) ;
#38889=CARTESIAN_POINT ( 'NONE',  ( 117.7034974245586483, -39.73408348695345182, 139.6194347997199827 ) ) ;
#38893=ORIENTED_EDGE ( 'NONE', *, *, #36787, .F. ) ;
#38895=CYLINDRICAL_SURFACE ( 'NONE', #50608, 2.117000000000007987 ) ;
#38896=LINE ( 'NONE', #5744, #66350 ) ;
#38898=ORIENTED_EDGE ( 'NONE', *, *, #2014, .F. ) ;
#38899=CARTESIAN_POINT ( 'NONE',  ( 107.0664832912739968, -36.72944715994100306, 311.6356252759112522 ) ) ;
#38900=ORIENTED_EDGE ( 'NONE', *, *, #1912, .T. ) ;
#38901=CARTESIAN_POINT ( 'NONE',  ( 116.3247715116346939, -32.94624160847306626, 99.13562527591096796 ) ) ;
#38902=CARTESIAN_POINT ( 'NONE',  ( 118.0022803299065686, -38.33799637688264994, 73.72229194257801055 ) ) ;
#38903=FACE_OUTER_BOUND ( 'NONE', #21392, .T. ) ;
#38904=DIRECTION ( 'NONE',  ( 0.000000000000000000, 0.000000000000000000, -1.000000000000000000 ) ) ;
#38905=CARTESIAN_POINT ( 'NONE',  ( 83.73314995794051185, 12.92155284005802685, 336.5756252759109657 ) ) ;
#38906=CARTESIAN_POINT ( 'NONE',  ( 97.42673588038233845, -38.38435052442954998, 91.46133956162594814 ) ) ;
#38907=CARTESIAN_POINT ( 'NONE',  ( 106.5510518188671227, -25.28190781890620542, 320.5359728645732389 ) ) ;
#38908=CARTESIAN_POINT ( 'NONE',  ( 113.0097079652340000, -45.31096836313445664, 199.0584824187679374 ) ) ;
#38909=CARTESIAN_POINT ( 'NONE',  ( 25.56670390244797275, -62.87844715994099687, 257.2178068554150059 ) ) ;
#38910=EDGE_CURVE ( 'NONE', #73307, #40784, #5406, .T. ) ;
#38911=DIRECTION ( 'NONE',  ( 0.000000000000000000, 0.000000000000000000, 1.000000000000000000 ) ) ;
#38912=VERTEX_POINT ( 'NONE', #38131 ) ;
#38914=CIRCLE ( 'NONE', #69401, 3.000000000000002665 ) ;
#38917=EDGE_CURVE ( 'NONE', #25576, #71344, #37282, .T. ) ;
#38919=CIRCLE ( 'NONE', #70847, 0.5000000000000004441 ) ;
#38920=DIRECTION ( 'NONE',  ( 1.000000000000000000, 0.000000000000000000, 0.000000000000000000 ) ) ;
#38921=CARTESIAN_POINT ( 'NONE',  ( 96.81521419041753518, -34.60385362728553815, 216.1641967044819808 ) ) ;
#38925=CARTESIAN_POINT ( 'NONE',  ( 111.7488185767529245, -27.39065688012293265, 275.7070538473396937 ) ) ;
#38926=CARTESIAN_POINT ( 'NONE',  ( 117.7233698349432132, -39.83239211553974712, 134.5889586092439743 ) ) ;
#38929=CARTESIAN_POINT ( 'NONE',  ( 82.76600038373194934, -37.25405382162458068, 6.823682607502961517 ) ) ;
#38930=LINE ( 'NONE', #72577, #23970 ) ;
#38935=EDGE_CURVE ( 'NONE', #54796, #28391, #88208, .T. ) ;
#38936=AXIS2_PLACEMENT_3D ( 'NONE', #30424, #71323, #58121 ) ;
#38937=ORIENTED_EDGE ( 'NONE', *, *, #72510, .T. ) ;
#38939=CARTESIAN_POINT ( 'NONE',  ( 117.5188882057536830, -36.54585972124053939, 284.8413395616252615 ) ) ;
#38941=EDGE_CURVE ( 'NONE', #86581, #87871, #4952, .T. ) ;
#38946=CARTESIAN_POINT ( 'NONE',  ( 98.70294500015674544, -34.99527330041078699, 215.5867055423629779 ) ) ;
#38949=VERTEX_POINT ( 'NONE', #45370 ) ;
#38950=EDGE_LOOP ( 'NONE', ( #76891, #44961, #9925, #68580 ) ) ;
#38954=CARTESIAN_POINT ( 'NONE',  ( 111.3597915011938539, -28.37217101237177985, 16.14253568684992501 ) ) ;
#38956=DIRECTION ( 'NONE',  ( -1.000000000000000078E-15, 1.000000000000000083E-30, 1.000000000000000000 ) ) ;
#38957=CARTESIAN_POINT ( 'NONE',  ( 117.3720538532507618, -35.57445771113444977, 233.9032443235299752 ) ) ;
#38958=CARTESIAN_POINT ( 'NONE',  ( 34.67381068361984120, -26.00627455219439099, 193.9678068554150911 ) ) ;
#38960=CIRCLE ( 'NONE', #34622, 3.000000000000002665 ) ;
#38962=VERTEX_POINT ( 'NONE', #79490 ) ;
#38963=CARTESIAN_POINT ( 'NONE',  ( 71.06648329127399677, -18.82844715994099971, 323.8756252759120002 ) ) ;
#38965=CARTESIAN_POINT ( 'NONE',  ( 113.7569007282865101, -30.30027569836345336, 37.25380465530597718 ) ) ;
#38966=AXIS2_PLACEMENT_3D ( 'NONE', #81868, #54112, #26880 ) ;
#38968=CARTESIAN_POINT ( 'NONE',  ( 135.6382054840660487, -16.47341874818684104, 7.827313014939066171 ) ) ;
#38969=EDGE_CURVE ( 'NONE', #78219, #52482, #59451, .T. ) ;
#38970=DIRECTION ( 'NONE',  ( 0.000000000000000000, 0.000000000000000000, -1.000000000000000000 ) ) ;
#38971=DIRECTION ( 'NONE',  ( -1.000000000000000078E-15, 1.000000000000000083E-30, 1.000000000000000000 ) ) ;
#38972=VERTEX_POINT ( 'NONE', #3609 ) ;
#38973=CARTESIAN_POINT ( 'NONE',  ( 182.0667039024469886, -33.35206098992630075, -5.074374724088000832 ) ) ;
#38974=CONICAL_SURFACE ( 'NONE', #12870, 1.258750000000002922, 1.029744258676650093 ) ;
#38976=ORIENTED_EDGE ( 'NONE', *, *, #79800, .F. ) ;
#38977=CARTESIAN_POINT ( 'NONE',  ( 97.57106248370669732, -31.07117258718254149, 130.9108633711489915 ) ) ;
#38979=CARTESIAN_POINT ( 'NONE',  ( 102.0495883242188171, -29.81664044981240025, 74.99813411379096806 ) ) ;
#38980=CIRCLE ( 'NONE', #63639, 0.5000000000000004441 ) ;
#38981=CARTESIAN_POINT ( 'NONE',  ( 97.89409425326189762, -40.71365990706227223, 87.65209274241340154 ) ) ;
#38982=CARTESIAN_POINT ( 'NONE',  ( 113.9519893150074239, -42.30780582616069552, 84.71586902018296428 ) ) ;
#38985=CARTESIAN_POINT ( 'NONE',  ( 102.7462986198438273, -25.66788047019655394, 16.37276813305293999 ) ) ;
#38986=LINE ( 'NONE', #79910, #35069 ) ;
#38987=EDGE_LOOP ( 'NONE', ( #57975, #50052, #85851, #77484 ) ) ;
#38988=CARTESIAN_POINT ( 'NONE',  ( 100.8874123674214189, -44.70017568039049394, 257.0521985988731899 ) ) ;
#38990=EDGE_CURVE ( 'NONE', #11421, #68641, #19901, .T. ) ;
#38993=ORIENTED_EDGE ( 'NONE', *, *, #18727, .F. ) ;
#38994=CIRCLE ( 'NONE', #17232, 3.299999999999997158 ) ;
#38997=CARTESIAN_POINT ( 'NONE',  ( 114.7458293810857128, -30.61868467657531312, 244.3613395616259822 ) ) ;
#38998=CARTESIAN_POINT ( 'NONE',  ( 97.66901493533356415, -40.15138444804937023, 126.6038837173656901 ) ) ;
#38999=CARTESIAN_POINT ( 'NONE',  ( 117.0608945212723739, -38.08045314311991802, 189.7189586074687497 ) ) ;
#39000=CARTESIAN_POINT ( 'NONE',  ( 99.98074987894446508, -44.37633341885192095, 42.98133956162492098 ) ) ;
#39001=CARTESIAN_POINT ( 'NONE',  ( 98.54755185453446131, -41.97681824699740361, 42.76578874115597273 ) ) ;
#39005=LINE ( 'NONE', #45803, #33111 ) ;
#39008=DIRECTION ( 'NONE',  ( -1.000000000000000078E-15, 1.000000000000000083E-30, 1.000000000000000000 ) ) ;
#39009=CARTESIAN_POINT ( 'NONE',  ( 113.1760029588135410, -44.75358003032814480, 114.0945772493509764 ) ) ;
#39010=CARTESIAN_POINT ( 'NONE',  ( 116.5068947302722222, -41.18400185692905069, 228.4756252759109714 ) ) ;
#39011=CARTESIAN_POINT ( 'NONE',  ( 82.81648329127402519, -36.72944715994107412, -5.074374724089055100 ) ) ;
#39012=ADVANCED_FACE ( 'NONE', ( #81723 ), #83497, .T. ) ;
#39015=CARTESIAN_POINT ( 'NONE',  ( 101.4222765643661006, -43.81150905960179642, 271.4514674471243438 ) ) ;
#39016=CARTESIAN_POINT ( 'NONE',  ( 172.5664832912729878, -27.82844715994070484, 254.1756252759120400 ) ) ;
#39017=CARTESIAN_POINT ( 'NONE',  ( 95.37363933861288956, -34.96150835630653120, 67.20705384733894050 ) ) ;
#39019=CARTESIAN_POINT ( 'NONE',  ( 95.62691733261443972, -33.44842233792613229, 141.1041967044829732 ) ) ;
#39021=CARTESIAN_POINT ( 'NONE',  ( 134.0664828118825938, -21.47944715903993540, 8.225259175038406312 ) ) ;
#39023=DIRECTION ( 'NONE',  ( 1.000000000000000000, 4.101809204280141026E-14, 0.000000000000000000 ) ) ;
#39024=CARTESIAN_POINT ( 'NONE',  ( 180.3521107875713199, -35.65087443489230878, 313.9678068554149490 ) ) ;
#39025=CARTESIAN_POINT ( 'NONE',  ( 76.06670390244799762, -26.72944715994109899, 199.5838068554169524 ) ) ;
#39027=ORIENTED_EDGE ( 'NONE', *, *, #15902, .T. ) ;
#39030=CARTESIAN_POINT ( 'NONE',  ( 95.98102948456921979, -37.30005869795228080, 121.3794347997209684 ) ) ;
#39032=FACE_OUTER_BOUND ( 'NONE', #43792, .T. ) ;
#39034=VECTOR ( 'NONE', #73027, 999.9999999999998863 ) ;
#39035=DIRECTION ( 'NONE',  ( -4.299999999999999979E-14, 1.000000000000000000, 0.000000000000000000 ) ) ;
#39037=CIRCLE ( 'NONE', #7153, 3.000000000000002665 ) ;
#39038=CARTESIAN_POINT ( 'NONE',  ( 114.0958560388892380, -44.50609692678638396, 133.1613395616249989 ) ) ;
#39040=DIRECTION ( 'NONE',  ( 3.999999999999999995E-14, -1.000000000000000000, 4.100000000000000342E-29 ) ) ;
#39042=ORIENTED_EDGE ( 'NONE', *, *, #54168, .T. ) ;
#39043=EDGE_CURVE ( 'NONE', #11705, #9815, #26726, .T. ) ;
#39046=DIRECTION ( 'NONE',  ( -1.000000000000000000, -3.360405532702990443E-14, 0.000000000000000000 ) ) ;
#39049=CARTESIAN_POINT ( 'NONE',  ( 138.0667039024479550, -26.72944715994091069, 239.5838068554170377 ) ) ;
#39050=DIRECTION ( 'NONE',  ( 0.000000000000000000, 0.000000000000000000, -1.000000000000000000 ) ) ;
#39051=B_SPLINE_CURVE_WITH_KNOTS ( 'NONE', 3,
 ( #75856, #77654, #1803, #84026, #82692, #49472, #42649, #48566, #70388, #6807, #34510, #8163, #76302, #63571, #27703, #55380, #1352, #29055 ),
 .UNSPECIFIED., .F., .F.,
 ( 4, 2, 2, 2, 2, 2, 2, 2, 4 ),
 ( 0.4999487719651097284, 0.5624551754694709915, 0.6249615789738323102, 0.6874679824781936288, 0.7499743859825549475, 0.8124807894869161551, 0.8749871929912774737, 0.9374935964956387924, 1.000000000000000000 ),
 .UNSPECIFIED. ) ;
#39055=FACE_BOUND ( 'NONE', #39445, .T. ) ;
#39056=ORIENTED_EDGE ( 'NONE', *, *, #89798, .F. ) ;
#39058=VECTOR ( 'NONE', #6079, 1000.000000000000000 ) ;
#39059=CARTESIAN_POINT ( 'NONE',  ( 107.6181574201208520, -47.08485352040289484, 193.6308633711479672 ) ) ;
#39062=VERTEX_POINT ( 'NONE', #76683 ) ;
#39063=CARTESIAN_POINT ( 'NONE',  ( 112.4622727538958316, -27.87370092883246286, 45.62895860924398761 ) ) ;
#39064=DIRECTION ( 'NONE',  ( 1.000000000000000000, 0.000000000000000000, 0.000000000000000000 ) ) ;
#39067=ORIENTED_EDGE ( 'NONE', *, *, #72502, .T. ) ;
#39068=LINE ( 'NONE', #52665, #2306 ) ;
#39072=CARTESIAN_POINT ( 'NONE',  ( 98.38943151359886485, -34.93026649658274607, 212.5958690201829597 ) ) ;
#39075=EDGE_CURVE ( 'NONE', #58180, #80800, #85299, .T. ) ;
#39079=DIRECTION ( 'NONE',  ( 0.000000000000000000, 0.000000000000000000, -1.000000000000000000 ) ) ;
#39081=VERTEX_POINT ( 'NONE', #40804 ) ;
#39082=CARTESIAN_POINT ( 'NONE',  ( 105.0259480979001410, -25.88970440745768542, 280.2365776568631759 ) ) ;
#39083=VERTEX_POINT ( 'NONE', #7196 ) ;
#39085=CARTESIAN_POINT ( 'NONE',  ( 106.6756582537710187, -44.91051946355214852, 245.3566617981629463 ) ) ;
#39086=LINE ( 'NONE', #60416, #51734 ) ;
#39089=DIRECTION ( 'NONE',  ( 1.000000000000000000, 6.193183223602000661E-14, -8.992470601956076883E-43 ) ) ;
#39090=CARTESIAN_POINT ( 'NONE',  ( 106.4811776831737262, -24.84380329649774666, 191.1156252759109861 ) ) ;
#39091=AXIS2_PLACEMENT_3D ( 'NONE', #44316, #85255, #85692 ) ;
#39094=VERTEX_POINT ( 'NONE', #33546 ) ;
#39095=CARTESIAN_POINT ( 'NONE',  ( 112.7836381133937067, -27.91740111342080866, 65.61848241876793963 ) ) ;
#39096=EDGE_CURVE ( 'NONE', #74209, #67921, #27629, .T. ) ;
#39098=EDGE_LOOP ( 'NONE', ( #58088, #67939, #71377, #18677 ) ) ;
#39099=ORIENTED_EDGE ( 'NONE', *, *, #88661, .T. ) ;
#39100=ADVANCED_FACE ( 'NONE', ( #89422 ), #21268, .T. ) ;
#39102=VECTOR ( 'NONE', #9972, 1000.000000000000000 ) ;
#39107=CARTESIAN_POINT ( 'NONE',  ( 100.1874667927473439, -32.28399744105692548, 143.6880903695909524 ) ) ;
#39108=CARTESIAN_POINT ( 'NONE',  ( 116.0738972362454149, -42.02130438377608357, 234.4041967044819899 ) ) ;
#39109=EDGE_CURVE ( 'NONE', #8960, #40724, #89121, .T. ) ;
#39110=CARTESIAN_POINT ( 'NONE',  ( 117.0604620818703410, -38.08351184708308779, 59.71871305607316316 ) ) ;
#39111=EDGE_LOOP ( 'NONE', ( #29024, #68086, #87692, #18178 ) ) ;
#39116=VERTEX_POINT ( 'NONE', #20384 ) ;
#39117=ORIENTED_EDGE ( 'NONE', *, *, #47633, .T. ) ;
#39118=EDGE_CURVE ( 'NONE', #62403, #23016, #41240, .T. ) ;
#39121=VECTOR ( 'NONE', #89195, 1000.000000000000000 ) ;
#39122=VERTEX_POINT ( 'NONE', #36697 ) ;
#39123=EDGE_LOOP ( 'NONE', ( #10346, #37893, #33448, #15312 ) ) ;
#39124=DIRECTION ( 'NONE',  ( -1.000000000000000000, 6.036837696399451257E-13, 0.000000000000000000 ) ) ;
#39125=FACE_OUTER_BOUND ( 'NONE', #39111, .T. ) ;
#39126=EDGE_CURVE ( 'NONE', #1430, #76359, #56669, .T. ) ;
#39128=VECTOR ( 'NONE', #55642, 1000.000000000000000 ) ;
#39129=CARTESIAN_POINT ( 'NONE',  ( 115.5798344143896372, -39.81741137289535004, 172.9600388756959717 ) ) ;
#39130=CARTESIAN_POINT ( 'NONE',  ( 104.6386611584700432, -47.56081657070318158, 27.38895860924395009 ) ) ;
#39132=ORIENTED_EDGE ( 'NONE', *, *, #61262, .F. ) ;
#39133=EDGE_CURVE ( 'NONE', #60854, #9592, #74582, .T. ) ;
#39136=VERTEX_POINT ( 'NONE', #50299 ) ;
#39138=EDGE_LOOP ( 'NONE', ( #14270, #79423, #33132, #52540 ) ) ;
#39139=CARTESIAN_POINT ( 'NONE',  ( 97.41723905860696675, -33.98881011871176838, 167.1061884298218843 ) ) ;
#39141=CARTESIAN_POINT ( 'NONE',  ( 110.8585676902739436, -45.98256027422110748, 132.8859773635041961 ) ) ;
#39143=ORIENTED_EDGE ( 'NONE', *, *, #65389, .F. ) ;
#39144=CARTESIAN_POINT ( 'NONE',  ( 111.4247116192842810, -46.22429891269226943, 27.91848241876792969 ) ) ;
#39145=CARTESIAN_POINT ( 'NONE',  ( 104.7259408665080116, -47.57930243624250721, 28.41943479971997988 ) ) ;
#39148=DIRECTION ( 'NONE',  ( -4.237773401492740281E-14, 1.000000000000000000, 0.000000000000000000 ) ) ;
#39149=CARTESIAN_POINT ( 'NONE',  ( 107.0664832912739399, -36.72944715994095333, 315.1356252759112522 ) ) ;
#39150=FACE_OUTER_BOUND ( 'NONE', #41485, .T. ) ;
#39151=VECTOR ( 'NONE', #40532, 1000.000000000000000 ) ;
#39153=CARTESIAN_POINT ( 'NONE',  ( 172.5664832912740110, -27.82844715994070484, 83.67562527591201160 ) ) ;
#39155=EDGE_CURVE ( 'NONE', #37435, #19551, #14913, .T. ) ;
#39156=AXIS2_PLACEMENT_3D ( 'NONE', #63872, #14382, #22992 ) ;
#39157=ORIENTED_EDGE ( 'NONE', *, *, #59534, .F. ) ;
#39158=CARTESIAN_POINT ( 'NONE',  ( 115.7096504343579539, -43.69425479293489900, 43.27467289495795200 ) ) ;
#39159=CARTESIAN_POINT ( 'NONE',  ( 117.4126858048608000, -35.18755665659306686, 214.9441967044829767 ) ) ;
#39160=CARTESIAN_POINT ( 'NONE',  ( 101.1286207290677908, -27.37920684556040740, 61.51467289495899138 ) ) ;
#39162=LINE ( 'NONE', #5095, #40650 ) ;
#39163=DIRECTION ( 'NONE',  ( 0.000000000000000000, 1.000000000000000000, 0.000000000000000000 ) ) ;
#39169=CARTESIAN_POINT ( 'NONE',  ( 110.8343066518039990, -26.26926122352955062, 95.80133956162396203 ) ) ;
#39170=CIRCLE ( 'NONE', #40600, 2.500000000000002220 ) ;
#39172=ORIENTED_EDGE ( 'NONE', *, *, #78107, .T. ) ;
#39173=CARTESIAN_POINT ( 'NONE',  ( 113.2071528006339918, -45.12711609280817271, 224.0784824187679476 ) ) ;
#39175=CARTESIAN_POINT ( 'NONE',  ( 111.4688792442139089, -45.71428781796094398, 147.9390134094296911 ) ) ;
#39176=CARTESIAN_POINT ( 'NONE',  ( 50.96943157743499597, -34.03355364505720360, -5.074374724088000832 ) ) ;
#39177=CARTESIAN_POINT ( 'NONE',  ( 108.4174892451278822, -26.73503592659411510, 45.96895860979116577 ) ) ;
#39180=AXIS2_PLACEMENT_3D ( 'NONE', #30445, #8666, #3619 ) ;
#39181=CARTESIAN_POINT ( 'NONE',  ( 111.1483613326457913, -47.07112276671761464, 172.8756252759109771 ) ) ;
#39183=ORIENTED_EDGE ( 'NONE', *, *, #51400, .F. ) ;
#39184=CARTESIAN_POINT ( 'NONE',  ( 113.6158397245882128, -43.46609735470438807, 114.6339642582779561 ) ) ;
#39185=DIRECTION ( 'NONE',  ( 0.000000000000000000, 1.000000000000000000, 0.000000000000000000 ) ) ;
#39186=CARTESIAN_POINT ( 'NONE',  ( 105.7207279102414077, -46.41719084699259668, 253.4670538473389740 ) ) ;
#39188=DIRECTION ( 'NONE',  ( -4.237773401492740281E-14, 1.000000000000000000, 0.000000000000000000 ) ) ;
#39189=CARTESIAN_POINT ( 'NONE',  ( 131.0667039024480118, -58.35344715994099829, 204.3338068554149913 ) ) ;
#39191=PLANE ( 'NONE',  #54721 ) ;
#39193=DIRECTION ( 'NONE',  ( 1.000000000000000078E-15, 0.000000000000000000, -1.000000000000000000 ) ) ;
#39195=CARTESIAN_POINT ( 'NONE',  ( 114.9613132280022683, -29.02649429439048134, 194.4537205140059370 ) ) ;
#39199=CARTESIAN_POINT ( 'NONE',  ( 78.35491772851318615, -16.56918551487918734, 2.099346190912949162 ) ) ;
#39200=LINE ( 'NONE', #34167, #46119 ) ;
#39201=DIRECTION ( 'NONE',  ( 0.000000000000000000, 0.000000000000000000, -1.000000000000000000 ) ) ;
#39202=VECTOR ( 'NONE', #14527, 1000.000000000000000 ) ;
#39203=CARTESIAN_POINT ( 'NONE',  ( 97.06389154151803211, -37.34296565923806099, 96.37529339840247644 ) ) ;
#39204=EDGE_LOOP ( 'NONE', ( #86049, #2936 ) ) ;
#39205=CARTESIAN_POINT ( 'NONE',  ( 116.7942972139657059, -39.39077959468326640, 63.61454998365505276 ) ) ;
#39207=CARTESIAN_POINT ( 'NONE',  ( 110.4989391570660473, -26.88539935475378684, 209.8099109901969541 ) ) ;
#39210=VERTEX_POINT ( 'NONE', #64842 ) ;
#39212=AXIS2_PLACEMENT_3D ( 'NONE', #26350, #81345, #11830 ) ;
#39215=CARTESIAN_POINT ( 'NONE',  ( 184.5664832912740110, 15.62155284005900491, 328.6381252759109088 ) ) ;
#39216=CARTESIAN_POINT ( 'NONE',  ( 115.7824585771272012, -41.80340552830423917, 164.4063582027085602 ) ) ;
#39217=CARTESIAN_POINT ( 'NONE',  ( 99.05427501747529107, -38.42862543901446060, 29.31094751244794949 ) ) ;
#39219=EDGE_CURVE ( 'NONE', #62140, #30523, #65886, .T. ) ;
#39220=DIRECTION ( 'NONE',  ( 0.000000000000000000, 0.000000000000000000, 1.000000000000000000 ) ) ;
#39221=ORIENTED_EDGE ( 'NONE', *, *, #147, .F. ) ;
#39222=DIRECTION ( 'NONE',  ( 1.000000000000000000, 4.299999999999999979E-14, 1.000000000000000078E-15 ) ) ;
#39223=CARTESIAN_POINT ( 'NONE',  ( 81.23646709784242148, -16.23881677343980812, 8.012604157996248588 ) ) ;
#39224=VERTEX_POINT ( 'NONE', #58020 ) ;
#39226=ORIENTED_EDGE ( 'NONE', *, *, #60623, .T. ) ;
#39228=CARTESIAN_POINT ( 'NONE',  ( 41.56648329127398966, -27.57844715994070484, 255.9256252759120116 ) ) ;
#39230=VERTEX_POINT ( 'NONE', #16254 ) ;
#39231=FACE_OUTER_BOUND ( 'NONE', #16334, .T. ) ;
#39232=EDGE_CURVE ( 'NONE', #55351, #89686, #43929, .T. ) ;
#39233=CARTESIAN_POINT ( 'NONE',  ( 100.1685590971342776, -42.59726720982692427, 76.32194363760098099 ) ) ;
#39234=AXIS2_PLACEMENT_3D ( 'NONE', #9090, #36789, #85411 ) ;
#39235=CARTESIAN_POINT ( 'NONE',  ( 116.3972416472496434, -41.42873566659991269, 203.4556252759109611 ) ) ;
#39236=CARTESIAN_POINT ( 'NONE',  ( 95.93334478249045105, -32.74178691125829488, 176.0527681330539735 ) ) ;
#39237=CARTESIAN_POINT ( 'NONE',  ( 108.8425424519434159, -46.66004013212315016, 22.71840272409394146 ) ) ;
#39238=CARTESIAN_POINT ( 'NONE',  ( 100.0240874364964299, -28.99487838171179632, 281.6641967044822650 ) ) ;
#39239=CARTESIAN_POINT ( 'NONE',  ( 138.8167039024479834, -50.82844715994100682, 88.43480685541499042 ) ) ;
#39240=CARTESIAN_POINT ( 'NONE',  ( 165.3359832912740046, -36.32844715994100682, -5.074374724088000832 ) ) ;
#39241=EDGE_LOOP ( 'NONE', ( #88525, #28865, #32737, #87191 ) ) ;
#39242=EDGE_CURVE ( 'NONE', #81785, #37024, #37116, .T. ) ;
#39243=ORIENTED_EDGE ( 'NONE', *, *, #55714, .F. ) ;
#39245=EDGE_CURVE ( 'NONE', #8740, #82586, #25234, .T. ) ;
#39247=CARTESIAN_POINT ( 'NONE',  ( 113.0507064547910829, -46.07834852625790489, 218.0175300378159591 ) ) ;
#39249=CARTESIAN_POINT ( 'NONE',  ( 104.4536708109005332, -26.63686367483539996, 200.2784824187679362 ) ) ;
#39250=DIRECTION ( 'NONE',  ( 4.194175870806139918E-14, -1.000000000000000000, 0.000000000000000000 ) ) ;
#39254=CARTESIAN_POINT ( 'NONE',  ( 104.3811196497008211, -29.05541074625367060, 277.6356252759112522 ) ) ;
#39256=CARTESIAN_POINT ( 'NONE',  ( 116.3212776292303090, -32.94146857471486811, 175.1356252759109680 ) ) ;
#39259=CARTESIAN_POINT ( 'NONE',  ( 51.42025729302567072, -31.94127993907664020, 193.9678068554150911 ) ) ;
#39260=AXIS2_PLACEMENT_3D ( 'NONE', #5665, #40157, #19289 ) ;
#39263=CARTESIAN_POINT ( 'NONE',  ( 80.06648329127402519, -46.72944715994105991, 4.925625275910944012 ) ) ;
#39266=ORIENTED_EDGE ( 'NONE', *, *, #48527, .F. ) ;
#39267=CARTESIAN_POINT ( 'NONE',  ( 136.8164763767836121, -18.77596264856166997, 6.749779334552346022 ) ) ;
#39268=CARTESIAN_POINT ( 'NONE',  ( 104.4049122349322545, -25.97716923158638735, 240.2575300378159682 ) ) ;
#39269=CARTESIAN_POINT ( 'NONE',  ( 98.33631928459364246, -42.42740502779041378, 97.78705384733993355 ) ) ;
#39270=CARTESIAN_POINT ( 'NONE',  ( 112.4768706805521248, -45.73309770202773450, 234.0070538473389377 ) ) ;
#39271=LINE ( 'NONE', #61051, #75891 ) ;
#39272=EDGE_CURVE ( 'NONE', #45837, #67341, #58620, .T. ) ;
#39273=CARTESIAN_POINT ( 'NONE',  ( 182.0374245136172249, -23.42844715993459559, 237.4678068554150059 ) ) ;
#39275=CARTESIAN_POINT ( 'NONE',  ( 98.36167194966670024, -41.66165578274063819, 37.73640923713256257 ) ) ;
#39276=DIRECTION ( 'NONE',  ( -0.9254794337955620787, -0.3787978585227822492, 0.000000000000000000 ) ) ;
#39278=EDGE_LOOP ( 'NONE', ( #61302, #32053, #68894, #40725, #38108 ) ) ;
#39280=B_SPLINE_CURVE_WITH_KNOTS ( 'NONE', 3,
 ( #77702, #50422, #79048, #9999, #16814, #29547, #57232, #44496, #37710, #78165, #65407, #30886, #68084, #25400, #67634, #67180, #26298, #53974 ),
 .UNSPECIFIED., .F., .F.,
 ( 4, 2, 2, 2, 2, 2, 2, 2, 4 ),
 ( 0.4999999989579788640, 0.5624999990882315615, 0.6249999992184841480, 0.6874999993487367345, 0.7499999994789894320, 0.8124999996092421295, 0.8749999997394947160, 0.9374999998697473025, 1.000000000000000000 ),
 .UNSPECIFIED. ) ;
#39281=CARTESIAN_POINT ( 'NONE',  ( 99.62716111080935377, -40.92618603589043147, 136.1581341137909646 ) ) ;
#39283=VERTEX_POINT ( 'NONE', #79830 ) ;
#39284=CARTESIAN_POINT ( 'NONE',  ( 97.31588645854830588, -39.30608289716393244, 91.53079023596599484 ) ) ;
#39285=CARTESIAN_POINT ( 'NONE',  ( 99.43809884604152671, -27.69271567064635065, 146.6356252759109395 ) ) ;
#39286=DIRECTION ( 'NONE',  ( -1.000000000000000078E-15, -1.000000000000000083E-30, 1.000000000000000000 ) ) ;
#39287=VECTOR ( 'NONE', #73371, 1000.000000000000000 ) ;
#39289=CIRCLE ( 'NONE', #32216, 2.116999999999993776 ) ;
#39290=ADVANCED_FACE ( 'NONE', ( #52509 ), #87969, .T. ) ;
#39292=CARTESIAN_POINT ( 'NONE',  ( 193.0374249753374443, -23.42844715993432558, 300.4678068554149490 ) ) ;
#39293=CARTESIAN_POINT ( 'NONE',  ( 115.0479362680066515, -42.38275094372912122, 53.33562527591095659 ) ) ;
#39294=EDGE_LOOP ( 'NONE', ( #13231, #71807, #4653, #50515 ) ) ;
#39295=ORIENTED_EDGE ( 'NONE', *, *, #9847, .F. ) ;
#39300=CARTESIAN_POINT ( 'NONE',  ( 117.0460787713798965, -39.54838250520747778, 139.6194347997199827 ) ) ;
#39303=CARTESIAN_POINT ( 'NONE',  ( 182.0667039024469886, -33.35206098992630075, -5.074374724088000832 ) ) ;
#39304=DIRECTION ( 'NONE',  ( 0.000000000000000000, 0.000000000000000000, 1.000000000000000000 ) ) ;
#39307=CARTESIAN_POINT ( 'NONE',  ( 113.3292761056179359, -27.64973082387871628, 89.60800622829195561 ) ) ;
#39308=ORIENTED_EDGE ( 'NONE', *, *, #66210, .F. ) ;
#39310=DIRECTION ( 'NONE',  ( 0.7071067811866258435, -0.7071067811864693020, 7.071067811866266166E-16 ) ) ;
#39311=DIRECTION ( 'NONE',  ( 0.000000000000000000, 0.000000000000000000, -1.000000000000000000 ) ) ;
#39313=CARTESIAN_POINT ( 'NONE',  ( 107.8028422452843387, -28.59910946728008341, 152.8223760838769749 ) ) ;
#39314=EDGE_CURVE ( 'NONE', #14684, #51499, #29594, .T. ) ;
#39315=EDGE_CURVE ( 'NONE', #37614, #9481, #42666, .T. ) ;
#39317=ORIENTED_EDGE ( 'NONE', *, *, #4246, .T. ) ;
#39321=EDGE_CURVE ( 'NONE', #14135, #29287, #25731, .T. ) ;
#39322=EDGE_LOOP ( 'NONE', ( #342, #50286, #24820, #74899 ) ) ;
#39323=ORIENTED_EDGE ( 'NONE', *, *, #24270, .F. ) ;
#39325=CARTESIAN_POINT ( 'NONE',  ( 117.0318879909729048, -38.19962202173364574, 220.1415833058969724 ) ) ;
#39326=EDGE_CURVE ( 'NONE', #22294, #4135, #54254, .T. ) ;
#39327=CARTESIAN_POINT ( 'NONE',  ( 97.81168895331838087, -40.51742574516882200, 287.6356252759109680 ) ) ;
#39329=CARTESIAN_POINT ( 'NONE',  ( 181.8884939055940038, -32.11662333284530746, -5.074374724088000832 ) ) ;
#39334=VECTOR ( 'NONE', #50951, 1000.000000000000000 ) ;
#39335=VERTEX_POINT ( 'NONE', #81173 ) ;
#39336=ORIENTED_EDGE ( 'NONE', *, *, #61358, .T. ) ;
#39337=EDGE_CURVE ( 'NONE', #51959, #34521, #31075, .T. ) ;
#39338=CARTESIAN_POINT ( 'NONE',  ( 110.6228153916969603, -44.07670705792993715, 245.7538046553059701 ) ) ;
#39339=CARTESIAN_POINT ( 'NONE',  ( 109.7758433794879664, -47.46978277150036263, 92.78514908543495210 ) ) ;
#39340=CARTESIAN_POINT ( 'NONE',  ( 103.6060256796756534, -46.54035428658124118, 57.30705384733997221 ) ) ;
#39344=CARTESIAN_POINT ( 'NONE',  ( 115.4866590905505603, -31.25382064240195845, 195.2850823816886532 ) ) ;
#39345=CARTESIAN_POINT ( 'NONE',  ( 98.85664311730629095, -30.30429143764317601, 151.7984824187679465 ) ) ;
#39348=DIRECTION ( 'NONE',  ( -0.7071067811865171526, -0.7071067811865779928, -6.612322855854603498E-17 ) ) ;
#39349=EDGE_LOOP ( 'NONE', ( #13534, #41645, #58597, #29532 ) ) ;
#39350=CIRCLE ( 'NONE', #46593, 2.116999999999980009 ) ;
#39351=ORIENTED_EDGE ( 'NONE', *, *, #9732, .T. ) ;
#39352=CARTESIAN_POINT ( 'NONE',  ( 116.3251085584666527, -32.94148239642360210, 265.1356252759109680 ) ) ;
#39354=VERTEX_POINT ( 'NONE', #58456 ) ;
#39355=VECTOR ( 'NONE', #78402, 1000.000000000000000 ) ;
#39357=ORIENTED_EDGE ( 'NONE', *, *, #7427, .F. ) ;
#39359=CARTESIAN_POINT ( 'NONE',  ( 95.48778530930356112, -34.20472165425801592, 106.1556252759109640 ) ) ;
#39361=LINE ( 'NONE', #3947, #14444 ) ;
#39362=CARTESIAN_POINT ( 'NONE',  ( 80.06648329127399677, 0.2215528400590013880, 4.925625275911999168 ) ) ;
#39363=CARTESIAN_POINT ( 'NONE',  ( 102.0841886111852261, -27.63463957783707770, 100.4632443235309580 ) ) ;
#39364=CARTESIAN_POINT ( 'NONE',  ( 41.56648329127499153, -32.07844715994070839, 203.6756252759119832 ) ) ;
#39365=CARTESIAN_POINT ( 'NONE',  ( 113.7366723824214318, -44.71300795807891149, 189.1299109901969757 ) ) ;
#39367=DIRECTION ( 'NONE',  ( 1.000000000000000000, 0.000000000000000000, 0.000000000000000000 ) ) ;
#39368=ORIENTED_EDGE ( 'NONE', *, *, #2004, .T. ) ;
#39369=VECTOR ( 'NONE', #2947, 1000.000000000000000 ) ;
#39370=CARTESIAN_POINT ( 'NONE',  ( 163.0664832912739826, -0.7548456658610993575, 335.0256252759120343 ) ) ;
#39372=CARTESIAN_POINT ( 'NONE',  ( 113.2475547418459598, -28.76023609674211201, 134.5522767884087898 ) ) ;
#39373=AXIS2_PLACEMENT_3D ( 'NONE', #13457, #27086, #39796 ) ;
#39374=CARTESIAN_POINT ( 'NONE',  ( 123.6837132603321692, -16.81243780205712568, 249.5838068554165261 ) ) ;
#39375=CARTESIAN_POINT ( 'NONE',  ( 115.4954577264304731, -29.50689403799194110, 229.4022919425779605 ) ) ;
#39377=CARTESIAN_POINT ( 'NONE',  ( 97.78494874870966669, -40.45152301011977158, 146.6299652419585584 ) ) ;
#39378=CARTESIAN_POINT ( 'NONE',  ( 118.5708186345730724, -33.89864261627929665, 10.01848241876795953 ) ) ;
#39379=CARTESIAN_POINT ( 'NONE',  ( 103.1584010082818850, -27.01760528431355368, 126.3813395616259783 ) ) ;
#39383=CARTESIAN_POINT ( 'NONE',  ( 62.03715912545824551, -47.82818131006021645, 300.4678068554150627 ) ) ;
#39384=DIRECTION ( 'NONE',  ( 4.299999999999999979E-14, -1.000000000000000000, 4.400000000000000367E-29 ) ) ;
#39385=ORIENTED_EDGE ( 'NONE', *, *, #36547, .T. ) ;
#39387=ORIENTED_EDGE ( 'NONE', *, *, #77021, .T. ) ;
#39389=ORIENTED_EDGE ( 'NONE', *, *, #34753, .T. ) ;
#39390=DIRECTION ( 'NONE',  ( 1.000000000000000078E-15, -1.000000000000000000, 0.000000000000000000 ) ) ;
#39391=CARTESIAN_POINT ( 'NONE',  ( 97.82856912889593559, -29.34641599088761765, 41.78991099019596334 ) ) ;
#39392=DIRECTION ( 'NONE',  ( 0.000000000000000000, 0.000000000000000000, -1.000000000000000000 ) ) ;
#39394=DIRECTION ( 'NONE',  ( 1.000000000000000000, 4.163336342344333240E-14, 0.000000000000000000 ) ) ;
#39396=CIRCLE ( 'NONE', #26308, 3.000000000000002665 ) ;
#39397=CARTESIAN_POINT ( 'NONE',  ( 104.8904560483511545, -27.93868065388478428, 239.6800388756959705 ) ) ;
#39399=EDGE_LOOP ( 'NONE', ( #14425, #49903, #45960, #56314 ) ) ;
#39401=AXIS2_PLACEMENT_3D ( 'NONE', #54841, #48468, #13540 ) ;
#39402=EDGE_CURVE ( 'NONE', #53017, #87676, #72985, .T. ) ;
#39404=CARTESIAN_POINT ( 'NONE',  ( 97.84203259209142800, -40.59156174939596440, 101.6424438322808896 ) ) ;
#39405=DIRECTION ( 'NONE',  ( 1.000000000000000078E-15, -1.000000000000000083E-30, -1.000000000000000000 ) ) ;
#39407=CARTESIAN_POINT ( 'NONE',  ( 110.4493835822141676, -45.49486465592072904, 14.28920235351599466 ) ) ;
#39410=CARTESIAN_POINT ( 'NONE',  ( 105.7207279102414077, -46.41719084699269615, 257.4670538473400825 ) ) ;
#39411=CYLINDRICAL_SURFACE ( 'NONE', #83472, 9.999999999999998224 ) ;
#39415=FACE_OUTER_BOUND ( 'NONE', #13148, .T. ) ;
#39417=CARTESIAN_POINT ( 'NONE',  ( 114.6445280793269603, -33.69580855137893138, 51.94809036959197357 ) ) ;
#39419=DIRECTION ( 'NONE',  ( -1.000000000000000000, -3.999999999999999995E-14, -1.000000000000000078E-15 ) ) ;
#39421=EDGE_CURVE ( 'NONE', #75636, #28680, #49874, .T. ) ;
#39428=ORIENTED_EDGE ( 'NONE', *, *, #14771, .F. ) ;
#39429=CARTESIAN_POINT ( 'NONE',  ( 108.3194705677269809, -47.07918403323724021, 117.6727681330539639 ) ) ;
#39430=ORIENTED_EDGE ( 'NONE', *, *, #45969, .F. ) ;
#39432=CARTESIAN_POINT ( 'NONE',  ( 99.88917683200891418, -30.19057113389683167, 80.16099125664798919 ) ) ;
#39433=AXIS2_PLACEMENT_3D ( 'NONE', #32425, #19708, #25627 ) ;
#39434=LINE ( 'NONE', #18996, #86656 ) ;
#39435=CARTESIAN_POINT ( 'NONE',  ( 103.7844689056781675, -44.99325446404193940, 113.7072975916109669 ) ) ;
#39436=EDGE_CURVE ( 'NONE', #59657, #85115, #45506, .T. ) ;
#39439=CARTESIAN_POINT ( 'NONE',  ( 104.7308122791112908, -47.55672043936114335, 28.41943479971997988 ) ) ;
#39440=CARTESIAN_POINT ( 'NONE',  ( 109.7253519077453632, -27.00093404018718246, 180.8651952712820332 ) ) ;
#39441=ORIENTED_EDGE ( 'NONE', *, *, #14660, .T. ) ;
#39442=CARTESIAN_POINT ( 'NONE',  ( 130.5667039024482960, -36.72944715994102438, 249.5838068554162987 ) ) ;
#39443=ORIENTED_EDGE ( 'NONE', *, *, #42244, .F. ) ;
#39444=CARTESIAN_POINT ( 'NONE',  ( 77.53592152231151147, -19.80596063775423588, 2.807537029278938334 ) ) ;
#39445=EDGE_LOOP ( 'NONE', ( #74542, #86490 ) ) ;
#39448=DIRECTION ( 'NONE',  ( 1.000000000000000078E-15, -1.000000000000000000, 0.000000000000000000 ) ) ;
#39449=ORIENTED_EDGE ( 'NONE', *, *, #13507, .T. ) ;
#39450=CARTESIAN_POINT ( 'NONE',  ( 97.17009264939167679, -31.66255117090383564, 245.9499109901979637 ) ) ;
#39452=CARTESIAN_POINT ( 'NONE',  ( 97.04389485639831037, -36.22610523983841091, 126.2859809355158518 ) ) ;
#39453=CARTESIAN_POINT ( 'NONE',  ( 108.3334480168114311, -46.73485936460039625, 188.6772919363633321 ) ) ;
#39454=CARTESIAN_POINT ( 'NONE',  ( 113.4595210239597520, -46.70760751678911049, 64.02991099019695298 ) ) ;
#39455=CARTESIAN_POINT ( 'NONE',  ( 113.2489316331219413, -28.76130024733460999, 95.55172767996501193 ) ) ;
#39457=DIRECTION ( 'NONE',  ( 1.000000000000000000, 4.163336342344333240E-14, 0.000000000000000000 ) ) ;
#39458=CARTESIAN_POINT ( 'NONE',  ( 182.2300522401179705, -33.89581943343660697, 117.4678068554150627 ) ) ;
#39459=AXIS2_PLACEMENT_3D ( 'NONE', #44505, #59472, #4529 ) ;
#39460=VERTEX_POINT ( 'NONE', #60686 ) ;
#39461=VECTOR ( 'NONE', #63833, 1000.000000000000000 ) ;
#39462=DIRECTION ( 'NONE',  ( -1.000000000000000078E-15, 1.000000000000000083E-30, 1.000000000000000000 ) ) ;
#39463=DIRECTION ( 'NONE',  ( 0.7071067811868666508, 0.7071067811862283836, 7.071067811868969987E-16 ) ) ;
#39464=CARTESIAN_POINT ( 'NONE',  ( 116.5620552962771654, -42.34175257684902505, 283.4137205140060587 ) ) ;
#39466=DIRECTION ( 'NONE',  ( -1.000000000000000078E-15, 1.000000000000000083E-30, 1.000000000000000000 ) ) ;
#39468=CARTESIAN_POINT ( 'NONE',  ( 115.6077113496922948, -36.78907078068826308, 263.2438483995052820 ) ) ;
#39470=CARTESIAN_POINT ( 'NONE',  ( 115.2499566122392736, -44.12502604085369029, 79.25372051400697160 ) ) ;
#39472=CARTESIAN_POINT ( 'NONE',  ( 114.7398264468854592, -44.75021323582976862, 113.1718157521009687 ) ) ;
#39473=ORIENTED_EDGE ( 'NONE', *, *, #74088, .T. ) ;
#39474=CARTESIAN_POINT ( 'NONE',  ( 163.0664832912739826, -8.350947159940998787, 333.4006252759120343 ) ) ;
#39476=DIRECTION ( 'NONE',  ( -0.7071067811865456854, -7.071067811865457584E-16, 0.7071067811865493491 ) ) ;
#39479=CARTESIAN_POINT ( 'NONE',  ( 63.03715912545733602, -46.82818131006016671, 193.9678068554150911 ) ) ;
#39480=ORIENTED_EDGE ( 'NONE', *, *, #17869, .T. ) ;
#39481=AXIS2_PLACEMENT_3D ( 'NONE', #18873, #74291, #59741 ) ;
#39483=CARTESIAN_POINT ( 'NONE',  ( 98.82181093208917844, -30.27703119756231942, 155.7984824187679465 ) ) ;
#39487=EDGE_CURVE ( 'NONE', #21457, #11589, #33442, .T. ) ;
#39488=DIRECTION ( 'NONE',  ( -0.7071067811874389708, 0.7071067811856560636, 0.000000000000000000 ) ) ;
#39489=VECTOR ( 'NONE', #48416, 1000.000000000000000 ) ;
#39490=LINE ( 'NONE', #18147, #29237 ) ;
#39492=VECTOR ( 'NONE', #46591, 1000.000000000000000 ) ;
#39493=CARTESIAN_POINT ( 'NONE',  ( 117.2437917682886592, -42.84961121563711828, 128.3956252759109873 ) ) ;
#39495=EDGE_CURVE ( 'NONE', #42455, #33402, #89771, .T. ) ;
#39496=DIRECTION ( 'NONE',  ( 0.000000000000000000, 0.000000000000000000, -1.000000000000000000 ) ) ;
#39498=ORIENTED_EDGE ( 'NONE', *, *, #61973, .T. ) ;
#39499=AXIS2_PLACEMENT_3D ( 'NONE', #12114, #61150, #81178 ) ;
#39500=EDGE_LOOP ( 'NONE', ( #27385, #72535 ) ) ;
#39501=CARTESIAN_POINT ( 'NONE',  ( 37.06648329127400388, 12.92155284005802685, 334.6228282640712450 ) ) ;
#39502=CARTESIAN_POINT ( 'NONE',  ( 108.9650027145310673, -26.85270947969657129, 249.9258047739795359 ) ) ;
#39504=DIRECTION ( 'NONE',  ( -0.7071067811866258435, 0.7071067811864693020, -7.071067811866266166E-16 ) ) ;
#39506=DIRECTION ( 'NONE',  ( 0.000000000000000000, 0.000000000000000000, 1.000000000000000000 ) ) ;
#39507=CARTESIAN_POINT ( 'NONE',  ( 194.0371591254584587, -46.82818131005407736, 180.4678068554150343 ) ) ;
#39508=ORIENTED_EDGE ( 'NONE', *, *, #53663, .F. ) ;
#39509=EDGE_CURVE ( 'NONE', #72918, #88176, #6635, .T. ) ;
#39511=CARTESIAN_POINT ( 'NONE',  ( 101.7740290765682829, -45.64733444449320388, 203.1622919425769567 ) ) ;
#39512=FACE_BOUND ( 'NONE', #42553, .T. ) ;
#39514=CIRCLE ( 'NONE', #62732, 10.00000000000000888 ) ;
#39515=CARTESIAN_POINT ( 'NONE',  ( 117.3261810260835603, -38.23854875528750341, 69.72229194257801055 ) ) ;
#39517=CARTESIAN_POINT ( 'NONE',  ( 117.0724228248738257, -35.46685996557965126, 13.92770122325937443 ) ) ;
#39519=ORIENTED_EDGE ( 'NONE', *, *, #74827, .F. ) ;
#39521=ORIENTED_EDGE ( 'NONE', *, *, #66895, .F. ) ;
#39522=ORIENTED_EDGE ( 'NONE', *, *, #53995, .F. ) ;
#39523=CARTESIAN_POINT ( 'NONE',  ( 112.2971567814265512, -43.88265157833087926, 224.5101547344679886 ) ) ;
#39524=CIRCLE ( 'NONE', #74363, 0.5000000000000004441 ) ;
#39525=CARTESIAN_POINT ( 'NONE',  ( 41.56648329127499153, -36.32844715994070839, 143.6756252759119832 ) ) ;
#39526=DIRECTION ( 'NONE',  ( -0.000000000000000000, -0.000000000000000000, 1.000000000000000000 ) ) ;
#39527=CARTESIAN_POINT ( 'NONE',  ( 163.2569089553707329, -33.54226604284440327, 237.4678068554150059 ) ) ;
#39528=LINE ( 'NONE', #61309, #9619 ) ;
#39529=ORIENTED_EDGE ( 'NONE', *, *, #68360, .T. ) ;
#39530=CARTESIAN_POINT ( 'NONE',  ( 172.5664832912729878, -27.57844715994070484, 141.9256252759119832 ) ) ;
#39532=ORIENTED_EDGE ( 'NONE', *, *, #6017, .T. ) ;
#39533=CARTESIAN_POINT ( 'NONE',  ( 116.2977993645976227, -41.52656014244018223, 288.4441967044823514 ) ) ;
#39534=ORIENTED_EDGE ( 'NONE', *, *, #28485, .F. ) ;
#39536=ORIENTED_EDGE ( 'NONE', *, *, #15223, .F. ) ;
#39537=CARTESIAN_POINT ( 'NONE',  ( 109.3322008939200458, -45.72736107978396092, 240.5909475124479684 ) ) ;
#39538=CIRCLE ( 'NONE', #56915, 0.5000000000000004441 ) ;
#39539=CARTESIAN_POINT ( 'NONE',  ( 96.37928053093608582, -33.66421044892479131, 141.1041967044829732 ) ) ;
#39543=CARTESIAN_POINT ( 'NONE',  ( 113.1252749404788034, -46.02936877844707197, 219.0480062282919960 ) ) ;
#39545=ORIENTED_EDGE ( 'NONE', *, *, #56240, .T. ) ;
#39546=AXIS2_PLACEMENT_3D ( 'NONE', #75566, #20599, #81945 ) ;
#39547=CARTESIAN_POINT ( 'NONE',  ( 108.9932425643425802, -47.01927604342903777, 78.72419670448194040 ) ) ;
#39548=FACE_OUTER_BOUND ( 'NONE', #13424, .T. ) ;
#39549=ORIENTED_EDGE ( 'NONE', *, *, #34364, .F. ) ;
#39551=ORIENTED_EDGE ( 'NONE', *, *, #28883, .T. ) ;
#39552=ADVANCED_FACE ( 'NONE', ( #55201 ), #26185, .F. ) ;
#39553=LINE ( 'NONE', #67257, #8593 ) ;
#39554=CARTESIAN_POINT ( 'NONE',  ( 188.5667039024479834, -62.87844715994099687, 259.9678068554150059 ) ) ;
#39555=ADVANCED_FACE ( 'NONE', ( #19819 ), #54751, .F. ) ;
#39557=CARTESIAN_POINT ( 'NONE',  ( 108.3053489883007927, -28.16931545225084221, 147.7918998934009664 ) ) ;
#39558=CARTESIAN_POINT ( 'NONE',  ( 101.3928372362931896, -45.54357991663450633, 218.1213395616249784 ) ) ;
#39560=ORIENTED_EDGE ( 'NONE', *, *, #84615, .T. ) ;
#39561=DIRECTION ( 'NONE',  ( 0.000000000000000000, 0.000000000000000000, -1.000000000000000000 ) ) ;
#39563=ORIENTED_EDGE ( 'NONE', *, *, #74293, .T. ) ;
#39564=CARTESIAN_POINT ( 'NONE',  ( 32.09598329127638294, -23.42844715994147364, 117.4678068554150485 ) ) ;
#39565=EDGE_LOOP ( 'NONE', ( #80896, #57656, #15402, #47978, #86761 ) ) ;
#39566=ORIENTED_EDGE ( 'NONE', *, *, #73258, .T. ) ;
#39567=CARTESIAN_POINT ( 'NONE',  ( 105.7167123138976024, -46.72404028231114381, 168.4698306292383734 ) ) ;
#39569=CARTESIAN_POINT ( 'NONE',  ( 163.0664832912739826, 19.62155284005901024, 333.4006252759110112 ) ) ;
#39570=CARTESIAN_POINT ( 'NONE',  ( 112.4313655287739948, -30.08308194412713021, 163.9581341137909476 ) ) ;
#39571=CARTESIAN_POINT ( 'NONE',  ( 100.4373464023292826, -44.86011580501824625, 12.03276813305398463 ) ) ;
#39572=CARTESIAN_POINT ( 'NONE',  ( 115.0873078068954243, -30.61556636850841073, 125.3441650706716928 ) ) ;
#39573=ORIENTED_EDGE ( 'NONE', *, *, #67301, .T. ) ;
#39574=AXIS2_PLACEMENT_3D ( 'NONE', #62411, #7456, #41953 ) ;
#39576=ORIENTED_EDGE ( 'NONE', *, *, #65477, .T. ) ;
#39577=CARTESIAN_POINT ( 'NONE',  ( 156.5667039024483529, -48.82844715993569196, 293.2178068554149490 ) ) ;
#39578=ORIENTED_EDGE ( 'NONE', *, *, #83520, .T. ) ;
#39579=DIRECTION ( 'NONE',  ( 0.7071067811989671936, 0.7071067811741279519, 6.612322855971028274E-17 ) ) ;
#39582=VECTOR ( 'NONE', #49029, 1000.000000000000000 ) ;
#39583=CARTESIAN_POINT ( 'NONE',  ( 51.56670390244799762, -33.35206098992650681, -5.074374724088000832 ) ) ;
#39585=CARTESIAN_POINT ( 'NONE',  ( 96.66386919200992622, -42.45828961175909200, 26.72705384733997747 ) ) ;
#39586=CARTESIAN_POINT ( 'NONE',  ( 117.1334281162953346, -32.05460809866745109, 55.16038718067301261 ) ) ;
#39587=DIRECTION ( 'NONE',  ( 1.000000000000000078E-15, 1.000000000000000083E-30, -1.000000000000000000 ) ) ;
#39589=EDGE_CURVE ( 'NONE', #75243, #3441, #82515, .T. ) ;
#39591=CARTESIAN_POINT ( 'NONE',  ( 106.0962982257710792, -25.30864543579675896, 322.6234344337125890 ) ) ;
#39592=FACE_BOUND ( 'NONE', #20408, .T. ) ;
#39593=CARTESIAN_POINT ( 'NONE',  ( 162.7131505118679797, -31.94127993907790852, -5.074374724088000832 ) ) ;
#39595=VERTEX_POINT ( 'NONE', #5751 ) ;
#39596=CARTESIAN_POINT ( 'NONE',  ( 96.14704956656235879, -38.72415284237285960, 51.48229194257797303 ) ) ;
#39597=CARTESIAN_POINT ( 'NONE',  ( 106.8516137164961464, -47.78059241960190207, 223.5489586092439538 ) ) ;
#39598=CARTESIAN_POINT ( 'NONE',  ( 117.3927859964040437, -32.72286779764937847, 90.10895860924395606 ) ) ;
#39599=DIRECTION ( 'NONE',  ( 0.000000000000000000, 0.000000000000000000, -1.000000000000000000 ) ) ;
#39600=DIRECTION ( 'NONE',  ( -0.7071067811865506814, 0.7071067811865443531, -7.071067811865500971E-16 ) ) ;
#39603=EDGE_CURVE ( 'NONE', #82293, #76316, #20278, .T. ) ;
#39604=VECTOR ( 'NONE', #10968, 1000.000000000000000 ) ;
#39606=EDGE_LOOP ( 'NONE', ( #59723, #64645 ) ) ;
#39607=CARTESIAN_POINT ( 'NONE',  ( 112.9545114599701492, -28.19305977888952697, 85.60800622829195561 ) ) ;
#39608=ADVANCED_FACE ( 'NONE', ( #7089 ), #6198, .T. ) ;
#39611=CARTESIAN_POINT ( 'NONE',  ( 110.0457755916377494, -26.10929462018219382, 215.8708633711489711 ) ) ;
#39613=FACE_OUTER_BOUND ( 'NONE', #15523, .T. ) ;
#39615=DIRECTION ( 'NONE',  ( -1.000000000000000078E-15, 1.000000000000000083E-30, 1.000000000000000000 ) ) ;
#39617=ADVANCED_FACE ( 'NONE', ( #13453 ), #55643, .F. ) ;
#39618=DIRECTION ( 'NONE',  ( 0.000000000000000000, 1.000000000000000000, 0.000000000000000000 ) ) ;
#39620=CARTESIAN_POINT ( 'NONE',  ( 97.26456095925928480, -36.24355304347522377, 171.2870538473399620 ) ) ;
#39622=EDGE_LOOP ( 'NONE', ( #71250, #12259, #79993, #34308, #67470, #39117, #30882, #19451 ) ) ;
#39624=CARTESIAN_POINT ( 'NONE',  ( 115.4287739208600527, -39.66208659201188880, 129.9901547344679500 ) ) ;
#39625=CARTESIAN_POINT ( 'NONE',  ( 134.0664832912740110, -41.22944715994101017, 4.925625275910997303 ) ) ;
#39626=CARTESIAN_POINT ( 'NONE',  ( 111.5675350091814266, -45.45035926415653194, 268.9556252759110180 ) ) ;
#39627=DIRECTION ( 'NONE',  ( 0.000000000000000000, 0.000000000000000000, -1.000000000000000000 ) ) ;
#39630=EDGE_CURVE ( 'NONE', #65123, #16063, #61145, .T. ) ;
#39631=PLANE ( 'NONE',  #46032 ) ;
#39634=DIRECTION ( 'NONE',  ( 1.000000000000000000, 1.261617073437676668E-15, 9.462128050782575008E-16 ) ) ;
#39636=CARTESIAN_POINT ( 'NONE',  ( 98.68348088377346983, -30.50934295487596515, 180.8184824187679567 ) ) ;
#39637=DIRECTION ( 'NONE',  ( 0.7071067811865165975, 0.7071067811865784369, 7.071067811865158803E-16 ) ) ;
#39638=ORIENTED_EDGE ( 'NONE', *, *, #60749, .F. ) ;
#39640=ORIENTED_EDGE ( 'NONE', *, *, #16299, .F. ) ;
#39642=CARTESIAN_POINT ( 'NONE',  ( 77.80861903143292579, -17.15582774925911735, 2.518078172590604957 ) ) ;
#39646=ORIENTED_EDGE ( 'NONE', *, *, #31428, .T. ) ;
#39647=CARTESIAN_POINT ( 'NONE',  ( 152.5667039024470171, -23.42844715993586036, 249.9678068554149490 ) ) ;
#39648=B_SPLINE_CURVE_WITH_KNOTS ( 'NONE', 3,
 ( #61278, #34014, #11804, #39502, #5889, #33578, #89001, #61715, #32683, #89453, #27211, #89912, #48975, #70801, #22209, #83988, #28547, #55780 ),
 .UNSPECIFIED., .F., .F.,
 ( 4, 2, 2, 2, 2, 2, 2, 2, 4 ),
 ( 0.08963260634764534662, 0.1409350762971974258, 0.1922375462467494911, 0.2435400161963015564, 0.2948424861458536217, 0.3461449560954056870, 0.3974474260449577523, 0.4487498959945098176, 0.5000523659440618829 ),
 .UNSPECIFIED. ) ;
#39649=CARTESIAN_POINT ( 'NONE',  ( 101.4045521927434805, -45.52538047655821885, 222.1213395616249784 ) ) ;
#39650=CARTESIAN_POINT ( 'NONE',  ( 134.4432975232679439, -39.47944369577152912, 8.225625303283962353 ) ) ;
#39652=ORIENTED_EDGE ( 'NONE', *, *, #85613, .T. ) ;
#39653=EDGE_CURVE ( 'NONE', #28842, #71659, #71565, .T. ) ;
#39655=DIRECTION ( 'NONE',  ( 4.299999999999999979E-14, -1.000000000000000000, 0.000000000000000000 ) ) ;
#39656=ADVANCED_FACE ( 'NONE', ( #2069 ), #29774, .T. ) ;
#39657=CARTESIAN_POINT ( 'NONE',  ( 97.81167943543778165, -40.51737693692245301, 166.6360185166829808 ) ) ;
#39659=CARTESIAN_POINT ( 'NONE',  ( 98.91757684337089529, -33.81461462136097396, 23.88332846482899186 ) ) ;
#39660=CARTESIAN_POINT ( 'NONE',  ( 117.6028659061361736, -33.31333136338176359, 130.0880062282919880 ) ) ;
#39661=DIRECTION ( 'NONE',  ( 0.000000000000000000, 1.000000000000000000, 0.000000000000000000 ) ) ;
#39662=ORIENTED_EDGE ( 'NONE', *, *, #49263, .F. ) ;
#39663=ADVANCED_FACE ( 'NONE', ( #35679 ), #64298, .F. ) ;
#39664=CARTESIAN_POINT ( 'NONE',  ( 107.0664832912739968, -36.72944715994100306, 287.6356252759109680 ) ) ;
#39665=LINE ( 'NONE', #67364, #32870 ) ;
#39666=ORIENTED_EDGE ( 'NONE', *, *, #53114, .F. ) ;
#39667=ORIENTED_EDGE ( 'NONE', *, *, #33326, .T. ) ;
#39668=VECTOR ( 'NONE', #82076, 1000.000000000000000 ) ;
#39671=ORIENTED_EDGE ( 'NONE', *, *, #35202, .F. ) ;
#39672=DIRECTION ( 'NONE',  ( -0.7071067811865849873, 0.7071067811865101582, 0.000000000000000000 ) ) ;
#39674=CARTESIAN_POINT ( 'NONE',  ( 98.78342310422263495, -33.06835657602663758, 55.40575316140994033 ) ) ;
#39675=CARTESIAN_POINT ( 'NONE',  ( 107.2435442917537500, -47.21071675017731906, 212.5899109901969837 ) ) ;
#39676=CARTESIAN_POINT ( 'NONE',  ( 102.6926969729869938, -27.29023857175969781, 180.4213395616249898 ) ) ;
#39678=CARTESIAN_POINT ( 'NONE',  ( 96.85498737197835339, -38.89503640450122646, 27.49276813305395706 ) ) ;
#39680=DIRECTION ( 'NONE',  ( 0.000000000000000000, 0.000000000000000000, -1.000000000000000000 ) ) ;
#39681=ORIENTED_EDGE ( 'NONE', *, *, #87736, .T. ) ;
#39683=CARTESIAN_POINT ( 'NONE',  ( 163.1639762274590169, -34.03355364505800651, -5.074374724088000832 ) ) ;
#39684=CARTESIAN_POINT ( 'NONE',  ( 96.09181007874647662, -35.06528625842698688, 221.1946728949589840 ) ) ;
#39685=AXIS2_PLACEMENT_3D ( 'NONE', #10822, #17212, #32602 ) ;
#39687=CARTESIAN_POINT ( 'NONE',  ( 97.05801352979682406, -41.42088835504144839, 211.6632443235299945 ) ) ;
#39688=CARTESIAN_POINT ( 'NONE',  ( 102.0670548988634891, -27.97049809344460769, 35.48979194811688842 ) ) ;
#39689=VECTOR ( 'NONE', #72590, 999.9999999999998863 ) ;
#39690=CARTESIAN_POINT ( 'NONE',  ( 98.38037815814482201, -41.69519609451472775, 22.73975804005023704 ) ) ;
#39692=CARTESIAN_POINT ( 'NONE',  ( 107.9134447035117432, -28.68416811027461222, 277.6356252759110248 ) ) ;
#39693=CARTESIAN_POINT ( 'NONE',  ( 125.0664851986225159, -56.72944715994101728, 14.67562527591098842 ) ) ;
#39694=LINE ( 'NONE', #18815, #40920 ) ;
#39696=CARTESIAN_POINT ( 'NONE',  ( 31.71315051185499811, -33.70561438052090608, 237.4678068554150059 ) ) ;
#39699=DIRECTION ( 'NONE',  ( -1.000000000000000000, -2.756263715554006823E-15, 0.000000000000000000 ) ) ;
#39701=ORIENTED_EDGE ( 'NONE', *, *, #50181, .F. ) ;
#39702=DIRECTION ( 'NONE',  ( 1.000000000000000078E-15, -1.000000000000000083E-30, -1.000000000000000000 ) ) ;
#39703=CARTESIAN_POINT ( 'NONE',  ( 112.2159804458396479, -45.81949903116512246, 212.9870538473389558 ) ) ;
#39704=CARTESIAN_POINT ( 'NONE',  ( 96.02365317015762969, -37.20890873343472549, 112.3489586092449599 ) ) ;
#39705=CARTESIAN_POINT ( 'NONE',  ( 114.6369858128092858, -29.49892357452570124, 230.4327681330539690 ) ) ;
#39706=LINE ( 'NONE', #17930, #10589 ) ;
#39708=CARTESIAN_POINT ( 'NONE',  ( 165.2725846195380086, -35.55794170701810941, -5.074374724088000832 ) ) ;
#39709=CARTESIAN_POINT ( 'NONE',  ( 97.81169418859235520, -40.51741816698509524, 47.63568902202231925 ) ) ;
#39710=CARTESIAN_POINT ( 'NONE',  ( 93.79911539042399227, -35.59159216677125670, 299.5571190294419921 ) ) ;
#39712=DIRECTION ( 'NONE',  ( 1.000000000000000000, 0.000000000000000000, 3.062684205862500216E-15 ) ) ;
#39713=ORIENTED_EDGE ( 'NONE', *, *, #15688, .F. ) ;
#39714=EDGE_CURVE ( 'NONE', #6819, #40280, #87685, .T. ) ;
#39716=CARTESIAN_POINT ( 'NONE',  ( 115.2241057928380599, -39.35723584706951783, 158.0009912566479500 ) ) ;
#39717=EDGE_CURVE ( 'NONE', #14045, #54558, #26788, .T. ) ;
#39719=ORIENTED_EDGE ( 'NONE', *, *, #24060, .T. ) ;
#39720=CARTESIAN_POINT ( 'NONE',  ( 180.3164832912730162, 12.92155284005730387, 355.9756252759109998 ) ) ;
#39721=CARTESIAN_POINT ( 'NONE',  ( 102.3226935662337524, -26.77152163616663927, 136.4422919425779526 ) ) ;
#39722=LINE ( 'NONE', #53783, #7684 ) ;
#39723=DIRECTION ( 'NONE',  ( 1.000000000000000000, 0.000000000000000000, 0.000000000000000000 ) ) ;
#39724=ADVANCED_FACE ( 'NONE', ( #51090, #49746 ), #15253, .F. ) ;
#39727=CARTESIAN_POINT ( 'NONE',  ( 98.30753419510237734, -41.72887549885788872, 107.7397919432831799 ) ) ;
#39728=CARTESIAN_POINT ( 'NONE',  ( 97.54819157151548836, -32.61351373332768588, 61.01372051400699803 ) ) ;
#39729=ORIENTED_EDGE ( 'NONE', *, *, #58306, .T. ) ;
#39730=EDGE_LOOP ( 'NONE', ( #236, #32918, #76068, #74713, #15351, #53603, #49718, #53015, #27321, #87507, #46895, #42884 ) ) ;
#39735=CARTESIAN_POINT ( 'NONE',  ( 101.2684584845352163, -45.32493232151062301, 148.0918157521009562 ) ) ;
#39736=FACE_BOUND ( 'NONE', #45000, .T. ) ;
#39737=CIRCLE ( 'NONE', #16544, 37.00000000000000711 ) ;
#39739=EDGE_CURVE ( 'NONE', #25266, #51283, #56101, .T. ) ;
#39741=LINE ( 'NONE', #54241, #60504 ) ;
#39742=LINE ( 'NONE', #74727, #68067 ) ;
#39743=CARTESIAN_POINT ( 'NONE',  ( 72.26648329127297643, -71.52944715994142655, 342.9256252759110453 ) ) ;
#39744=CARTESIAN_POINT ( 'NONE',  ( 112.5028774994482035, -27.85959465031275784, 94.63848241876793566 ) ) ;
#39748=FACE_BOUND ( 'NONE', #48502, .T. ) ;
#39751=CARTESIAN_POINT ( 'NONE',  ( 103.1635642379172850, -29.56027560196853088, 143.2909475124489518 ) ) ;
#39753=AXIS2_PLACEMENT_3D ( 'NONE', #61385, #75483, #19454 ) ;
#39755=DIRECTION ( 'NONE',  ( -0.7071067811734105257, 0.7071067811996846197, 0.000000000000000000 ) ) ;
#39756=ORIENTED_EDGE ( 'NONE', *, *, #37152, .F. ) ;
#39757=VERTEX_POINT ( 'NONE', #23424 ) ;
#39758=CARTESIAN_POINT ( 'NONE',  ( 31.78666935232860169, -29.62846900982351528, 193.9678068554150911 ) ) ;
#39759=ORIENTED_EDGE ( 'NONE', *, *, #78100, .T. ) ;
#39762=EDGE_CURVE ( 'NONE', #63148, #11683, #33983, .T. ) ;
#39763=CARTESIAN_POINT ( 'NONE',  ( 98.23266987703472353, -35.71659467859123538, 202.6672975916109465 ) ) ;
#39764=CARTESIAN_POINT ( 'NONE',  ( 107.0664832912739541, -36.72944715994095333, 308.7195067599733420 ) ) ;
#39765=ADVANCED_FACE ( 'NONE', ( #28878 ), #56567, .F. ) ;
#39766=CYLINDRICAL_SURFACE ( 'NONE', #31300, 0.5000000000000079936 ) ;
#39767=CARTESIAN_POINT ( 'NONE',  ( 107.0664832912739399, -36.72944715994096754, 300.2406250056037038 ) ) ;
#39770=ORIENTED_EDGE ( 'NONE', *, *, #74811, .T. ) ;
#39772=CARTESIAN_POINT ( 'NONE',  ( 104.6179474607139213, -28.94263790944830106, 248.1366617981629474 ) ) ;
#39773=CARTESIAN_POINT ( 'NONE',  ( 112.8139912305532704, -47.12176010715679553, 102.9784824187679817 ) ) ;
#39774=CARTESIAN_POINT ( 'NONE',  ( 110.7866772467784955, -46.44483816919306918, 62.86705384733992474 ) ) ;
#39775=CARTESIAN_POINT ( 'NONE',  ( 99.75758940074024395, -33.13488748790386751, 249.5838068554174072 ) ) ;
#39776=CARTESIAN_POINT ( 'NONE',  ( 134.0664832912739826, -15.97944715994100306, 8.225625275910998013 ) ) ;
#39778=CARTESIAN_POINT ( 'NONE',  ( 98.53766203808953605, -30.73430783891158669, 201.8384824187679385 ) ) ;
#39780=VERTEX_POINT ( 'NONE', #36135 ) ;
#39781=CARTESIAN_POINT ( 'NONE',  ( 61.67079006425790766, -0.9306969701470987344, 542.9756252759101471 ) ) ;
#39782=ORIENTED_EDGE ( 'NONE', *, *, #75235, .F. ) ;
#39783=ORIENTED_EDGE ( 'NONE', *, *, #2132, .F. ) ;
#39784=DIRECTION ( 'NONE',  ( 0.7071067811874278686, -0.7071067811856670549, 6.612322855868390075E-17 ) ) ;
#39785=VERTEX_POINT ( 'NONE', #77032 ) ;
#39787=CARTESIAN_POINT ( 'NONE',  ( 113.1782937589909181, -44.75186860218948937, 178.0939586081543666 ) ) ;
#39788=CARTESIAN_POINT ( 'NONE',  ( 109.6839073351967642, -47.46854297047285343, 87.75467289495897205 ) ) ;
#39789=CARTESIAN_POINT ( 'NONE',  ( 113.2492940411024449, -28.76157773499452119, 254.5522619721145645 ) ) ;
#39793=DIRECTION ( 'NONE',  ( 0.000000000000000000, -1.000000000000000000, 0.000000000000000000 ) ) ;
#39794=CARTESIAN_POINT ( 'NONE',  ( 126.0667039024479266, -14.72944715994094977, 239.5838068554170377 ) ) ;
#39795=CARTESIAN_POINT ( 'NONE',  ( 98.27975524859429868, -42.29919363830185119, 182.7756252759109543 ) ) ;
#39796=DIRECTION ( 'NONE',  ( 8.673617379884035472E-16, 1.000000000000000000, 0.000000000000000000 ) ) ;
#39797=CARTESIAN_POINT ( 'NONE',  ( 123.6837132603319560, -53.34645651782485487, 219.5838068554170093 ) ) ;
#39799=CARTESIAN_POINT ( 'NONE',  ( 34.96670390244699433, -26.71338133339301635, -5.074374724088000832 ) ) ;
#39801=CARTESIAN_POINT ( 'NONE',  ( 97.12563366290001454, -37.99751694395044410, 136.4276054474069326 ) ) ;
#39802=DIRECTION ( 'NONE',  ( 0.000000000000000000, 0.000000000000000000, 1.000000000000000000 ) ) ;
#39803=CARTESIAN_POINT ( 'NONE',  ( 113.8278214188052999, -26.93592357317604424, 239.5956252759109759 ) ) ;
#39806=CARTESIAN_POINT ( 'NONE',  ( 105.8911342260945645, -47.14568079332288875, 278.4870538473395527 ) ) ;
#39807=CARTESIAN_POINT ( 'NONE',  ( 112.1411864721344642, -47.49320580990715968, 133.9270538473399768 ) ) ;
#39812=CARTESIAN_POINT ( 'NONE',  ( 188.5667039024479834, -48.82844715994099971, 257.2178068554150059 ) ) ;
#39813=CARTESIAN_POINT ( 'NONE',  ( 107.0664832912739968, -36.72944715994100306, 249.5838068554170093 ) ) ;
#39814=DIRECTION ( 'NONE',  ( 4.299999999999999979E-14, -1.000000000000000000, 4.400000000000000367E-29 ) ) ;
#39817=AXIS2_PLACEMENT_3D ( 'NONE', #19512, #33590, #61725 ) ;
#39818=AXIS2_PLACEMENT_3D ( 'NONE', #74671, #33336, #19705 ) ;
#39822=VERTEX_POINT ( 'NONE', #45590 ) ;
#39823=CIRCLE ( 'NONE', #26791, 2.749999999999974687 ) ;
#39824=VECTOR ( 'NONE', #57274, 1000.000000000000000 ) ;
#39825=EDGE_CURVE ( 'NONE', #84501, #55506, #32421, .T. ) ;
#39827=DIRECTION ( 'NONE',  ( 0.000000000000000000, -1.000000000000000000, 0.000000000000000000 ) ) ;
#39828=CARTESIAN_POINT ( 'NONE',  ( 107.1951288810177090, -26.32694189238808491, 31.06705384733893283 ) ) ;
#39833=CARTESIAN_POINT ( 'NONE',  ( 59.67078992371374113, -0.9290567490904538817, 396.9756252759102040 ) ) ;
#39835=CARTESIAN_POINT ( 'NONE',  ( 112.5827476457113079, -28.73936235024410024, 239.0181341137909783 ) ) ;
#39837=ORIENTED_EDGE ( 'NONE', *, *, #25076, .T. ) ;
#39838=ORIENTED_EDGE ( 'NONE', *, *, #81919, .F. ) ;
#39842=DIRECTION ( 'NONE',  ( 0.000000000000000000, 0.000000000000000000, 1.000000000000000000 ) ) ;
#39844=CARTESIAN_POINT ( 'NONE',  ( 98.34910283431410960, -31.65794092288606976, 275.9061490951863789 ) ) ;
#39845=CARTESIAN_POINT ( 'NONE',  ( 110.5196960824274868, -45.46740155661881033, 19.31967854399191253 ) ) ;
#39846=EDGE_CURVE ( 'NONE', #51283, #23552, #76077, .T. ) ;
#39848=DIRECTION ( 'NONE',  ( 0.02150753337724187197, 0.0009076677972194977960, 0.9997682742251811083 ) ) ;
#39849=CARTESIAN_POINT ( 'NONE',  ( 111.5675350091857325, -45.45035926415926752, 272.9556252759110180 ) ) ;
#39850=CYLINDRICAL_SURFACE ( 'NONE', #84990, 3.249999999999975131 ) ;
#39851=EDGE_CURVE ( 'NONE', #36809, #35978, #17911, .T. ) ;
#39853=CARTESIAN_POINT ( 'NONE',  ( 182.3467384525654893, -29.62846900981658393, 313.9678068554149490 ) ) ;
#39855=CARTESIAN_POINT ( 'NONE',  ( 113.8053744393198485, -42.15975756917345763, 41.09285227435299959 ) ) ;
#39856=CIRCLE ( 'NONE', #16662, 11.45913725231036118 ) ;
#39857=CARTESIAN_POINT ( 'NONE',  ( 136.7302760451841266, -18.02416100036293400, 6.874390491351639376 ) ) ;
#39860=CARTESIAN_POINT ( 'NONE',  ( 71.24025061656124080, 8.642044024269639024, 542.9756252759101471 ) ) ;
#39861=VERTEX_POINT ( 'NONE', #24298 ) ;
#39862=DIRECTION ( 'NONE',  ( 0.7071067811861728725, -0.7071067811869222730, 0.000000000000000000 ) ) ;
#39864=ORIENTED_EDGE ( 'NONE', *, *, #2652, .F. ) ;
#39865=CARTESIAN_POINT ( 'NONE',  ( 113.0770494671172628, -28.21122406429266150, 129.5870538473399449 ) ) ;
#39867=CARTESIAN_POINT ( 'NONE',  ( 113.7032067727884197, -42.10625226631949403, 87.70670554236198768 ) ) ;
#39868=CARTESIAN_POINT ( 'NONE',  ( 167.7413838386819123, -48.33240602328260849, 180.4678068554150059 ) ) ;
#39869=CARTESIAN_POINT ( 'NONE',  ( 102.3355707743008765, -29.23633396390525618, 106.9558690201829734 ) ) ;
#39870=CARTESIAN_POINT ( 'NONE',  ( 34.33598329127390514, -36.32844715994140472, 117.4678068554150485 ) ) ;
#39873=CARTESIAN_POINT ( 'NONE',  ( 113.5195425369480233, -28.51389573442233427, 75.54705384733995288 ) ) ;
#39874=FACE_OUTER_BOUND ( 'NONE', #25934, .T. ) ;
#39876=VECTOR ( 'NONE', #20543, 1000.000000000000000 ) ;
#39878=CARTESIAN_POINT ( 'NONE',  ( 188.5667039024479834, -62.87844715994099687, 139.9678068554150059 ) ) ;
#39879=VECTOR ( 'NONE', #23017, 999.9999999999998863 ) ;
#39880=CIRCLE ( 'NONE', #12347, 2.500000000000002220 ) ;
#39882=ORIENTED_EDGE ( 'NONE', *, *, #43674, .F. ) ;
#39886=ORIENTED_EDGE ( 'NONE', *, *, #60978, .T. ) ;
#39887=CARTESIAN_POINT ( 'NONE',  ( 113.3831382903590992, -27.58002901871518020, 239.5956252759109759 ) ) ;
#39888=CARTESIAN_POINT ( 'NONE',  ( 117.7011894673193382, -39.82593390098057284, 134.5889586092439743 ) ) ;
#39889=B_SPLINE_CURVE_WITH_KNOTS ( 'NONE', 3,
 ( #50748, #22171, #83950, #35771, #23077, #78483, #16245, #43920, #21720, #50287, #85747, #63482, #49392, #48932, #1270, #28974, #56660, #77565, #15352, #43021, #8534, #36231, #63942, #57100, #15799, #71214, #60223, #11658, #3938 ),
 .UNSPECIFIED., .F., .F.,
 ( 4, 2, 2, 2, 2, 2, 2, 2, 2, 2, 1, 1, 1, 1, 1, 2, 4 ),
 ( 0.000000000000000000, 0.06249314710935460759, 0.1249862942187092152, 0.1874794413280638228, 0.2499725884374184304, 0.3124657355467730380, 0.3749588826561276456, 0.4374520297654822532, 0.4686986033201598345, 0.4843218900974986529, 0.4921335334861677846, 0.4960393551805025170, 0.4979922660276701052, 0.4989687214512539271, 0.4994569491630460045, 0.4997010630189421820, 0.4999451768748383040 ),
 .UNSPECIFIED. ) ;
#39890=CARTESIAN_POINT ( 'NONE',  ( 103.5243996547270626, -27.35269840695457688, 125.3628851967883975 ) ) ;
#39892=CARTESIAN_POINT ( 'NONE',  ( 108.5379568639253449, -26.40872756427751611, 100.9641967044829727 ) ) ;
#39895=DIRECTION ( 'NONE',  ( 1.000000000000000078E-15, -1.000000000000000083E-30, -1.000000000000000000 ) ) ;
#39897=CARTESIAN_POINT ( 'NONE',  ( 131.3164832912739826, -18.72944715994100662, 14.92562527591099553 ) ) ;
#39898=AXIS2_PLACEMENT_3D ( 'NONE', #17834, #58276, #72366 ) ;
#39900=EDGE_CURVE ( 'NONE', #7066, #58062, #89186, .T. ) ;
#39902=DIRECTION ( 'NONE',  ( -1.000000000000000000, 0.000000000000000000, 0.000000000000000000 ) ) ;
#39903=CARTESIAN_POINT ( 'NONE',  ( 100.4652087429556815, -44.82591848225601439, 12.03276813305398463 ) ) ;
#39904=DIRECTION ( 'NONE',  ( 4.299999999999999979E-14, -1.000000000000000000, 4.400000000000000367E-29 ) ) ;
#39905=CARTESIAN_POINT ( 'NONE',  ( 152.0371591254582881, -47.82818131005588214, 300.4678068554149490 ) ) ;
#39906=CARTESIAN_POINT ( 'NONE',  ( 77.58678459498953828, -37.92005462650905656, 2.747931806396151977 ) ) ;
#39907=CARTESIAN_POINT ( 'NONE',  ( 106.3786087989843736, -45.75936958534449417, 266.9505150661723860 ) ) ;
#39908=CARTESIAN_POINT ( 'NONE',  ( 80.06648329127398256, -9.029447159941060619, 4.925625275910944012 ) ) ;
#39909=CARTESIAN_POINT ( 'NONE',  ( 118.8180844208008722, -35.40729807334668777, 79.91562527591095488 ) ) ;
#39910=CARTESIAN_POINT ( 'NONE',  ( 163.2569089553709603, -33.54226604284439617, 117.4678068554150485 ) ) ;
#39911=CARTESIAN_POINT ( 'NONE',  ( 109.8678013061348508, -26.64186650728397865, 174.8613395616249591 ) ) ;
#39912=ORIENTED_EDGE ( 'NONE', *, *, #22510, .F. ) ;
#39914=EDGE_LOOP ( 'NONE', ( #10858, #48543, #3555, #11375 ) ) ;
#39915=DIRECTION ( 'NONE',  ( -1.000000000000000078E-15, 0.000000000000000000, 1.000000000000000000 ) ) ;
#39916=CARTESIAN_POINT ( 'NONE',  ( 32.15435173583698969, -31.62489322948785997, 342.9256252759109884 ) ) ;
#39918=VERTEX_POINT ( 'NONE', #3402 ) ;
#39919=CARTESIAN_POINT ( 'NONE',  ( 140.9629299006807059, -46.47944715994099596, 14.92562527591100618 ) ) ;
#39920=CARTESIAN_POINT ( 'NONE',  ( 117.6526747975261458, -33.39096950974673916, 129.0575300378159795 ) ) ;
#39927=CYLINDRICAL_SURFACE ( 'NONE', #53954, 0.5000000000000031086 ) ;
#39931=DIRECTION ( 'NONE',  ( 0.000000000000000000, 1.000000000000000000, 0.000000000000000000 ) ) ;
#39932=DIRECTION ( 'NONE',  ( -0.7071067811864666375, -0.7071067811866283970, -7.071067811864659848E-16 ) ) ;
#39935=ADVANCED_FACE ( 'NONE', ( #86972 ), #46042, .F. ) ;
#39936=ORIENTED_EDGE ( 'NONE', *, *, #15960, .T. ) ;
#39940=CARTESIAN_POINT ( 'NONE',  ( 20.03715912545735378, -24.42818131006189830, 249.9678068554150059 ) ) ;
#39941=EDGE_CURVE ( 'NONE', #42715, #22615, #61609, .T. ) ;
#39945=AXIS2_PLACEMENT_3D ( 'NONE', #40415, #89472, #54910 ) ;
#39949=VECTOR ( 'NONE', #19421, 1000.000000000000000 ) ;
#39951=CARTESIAN_POINT ( 'NONE',  ( 103.9298229712114363, -26.84510867568836545, 201.3089586092439731 ) ) ;
#39952=EDGE_CURVE ( 'NONE', #19365, #67921, #6092, .T. ) ;
#39955=AXIS2_PLACEMENT_3D ( 'NONE', #38266, #2871, #31443 ) ;
#39956=CARTESIAN_POINT ( 'NONE',  ( 112.5987260342904648, -28.66361022110277545, 40.59848241876795782 ) ) ;
#39957=CARTESIAN_POINT ( 'NONE',  ( 165.2748236753148205, -30.08671355699731009, 117.4678068554150485 ) ) ;
#39959=AXIS2_PLACEMENT_3D ( 'NONE', #8882, #1615, #8424 ) ;
#39961=VERTEX_POINT ( 'NONE', #46494 ) ;
#39962=DIRECTION ( 'NONE',  ( 1.000000000000000000, 0.000000000000000000, 0.000000000000000000 ) ) ;
#39963=ORIENTED_EDGE ( 'NONE', *, *, #59032, .F. ) ;
#39964=EDGE_LOOP ( 'NONE', ( #63915, #7357, #28359, #62462 ) ) ;
#39965=CIRCLE ( 'NONE', #47217, 0.5000000000000016653 ) ;
#39966=CARTESIAN_POINT ( 'NONE',  ( 116.4035850909244090, -35.68299815489336879, 230.3349166392299594 ) ) ;
#39968=CARTESIAN_POINT ( 'NONE',  ( 32.16397622746000451, -34.03355364505800651, -5.074374724088000832 ) ) ;
#39969=FACE_OUTER_BOUND ( 'NONE', #33825, .T. ) ;
#39971=CARTESIAN_POINT ( 'NONE',  ( 179.4595971212906704, -28.98061976758350511, 237.4678068554150059 ) ) ;
#39972=CARTESIAN_POINT ( 'NONE',  ( 82.61444500289060500, -37.76411817599981902, 2.828498113172249084 ) ) ;
#39976=ORIENTED_EDGE ( 'NONE', *, *, #20860, .T. ) ;
#39977=CARTESIAN_POINT ( 'NONE',  ( 97.23737678141878860, -33.32131919061083636, 286.0613395616252888 ) ) ;
#39978=VERTEX_POINT ( 'NONE', #81065 ) ;
#39979=AXIS2_PLACEMENT_3D ( 'NONE', #87047, #80235, #11168 ) ;
#39981=CARTESIAN_POINT ( 'NONE',  ( 115.7114656938015429, -36.32299383444259888, 266.6699951314962505 ) ) ;
#39983=CARTESIAN_POINT ( 'NONE',  ( 102.6065612795739952, -27.36740250608067626, 140.4422919425779526 ) ) ;
#39985=CARTESIAN_POINT ( 'NONE',  ( 122.7090602494120049, -38.07100823150197755, 293.6356252759109680 ) ) ;
#39987=EDGE_CURVE ( 'NONE', #69327, #59306, #5012, .T. ) ;
#39989=CARTESIAN_POINT ( 'NONE',  ( 100.7971853062899896, -45.88878125878837011, 238.1108633711489517 ) ) ;
#39990=DIRECTION ( 'NONE',  ( -1.000000000000000078E-15, 1.000000000000000083E-30, 1.000000000000000000 ) ) ;
#39991=ORIENTED_EDGE ( 'NONE', *, *, #35099, .T. ) ;
#39992=CARTESIAN_POINT ( 'NONE',  ( 116.1615364674122333, -29.05539214145830229, 70.38419670448192278 ) ) ;
#39993=CARTESIAN_POINT ( 'NONE',  ( 25.56670390244828894, -48.82844715994168183, 293.2178068554150059 ) ) ;
#39994=VECTOR ( 'NONE', #51603, 1000.000000000000114 ) ;
#39995=EDGE_CURVE ( 'NONE', #12231, #56697, #88762, .T. ) ;
#39996=ORIENTED_EDGE ( 'NONE', *, *, #29084, .T. ) ;
#39998=EDGE_LOOP ( 'NONE', ( #28694, #89177, #39560, #34320, #52138 ) ) ;
#39999=CARTESIAN_POINT ( 'NONE',  ( 80.06648329127402519, -46.72944715994105991, 4.925625275910944012 ) ) ;
#40000=DIRECTION ( 'NONE',  ( -1.000000000000000078E-15, 0.000000000000000000, 1.000000000000000000 ) ) ;
#40001=CARTESIAN_POINT ( 'NONE',  ( 113.1760499632551529, -44.75354527206816613, 153.0944392216708536 ) ) ;
#40002=CARTESIAN_POINT ( 'NONE',  ( 116.3457274436100164, -36.88499157630047165, 151.6309475124489552 ) ) ;
#40003=CARTESIAN_POINT ( 'NONE',  ( 118.1046235831494755, -32.34975429571041161, 245.1270538473389706 ) ) ;
#40004=DIRECTION ( 'NONE',  ( 4.299999999999999979E-14, -1.000000000000000000, 4.400000000000000367E-29 ) ) ;
#40005=ORIENTED_EDGE ( 'NONE', *, *, #16860, .F. ) ;
#40007=CARTESIAN_POINT ( 'NONE',  ( 136.7495928495827968, -37.33856210726968072, 3.004220725469414432 ) ) ;
#40009=VERTEX_POINT ( 'NONE', #67856 ) ;
#40010=EDGE_CURVE ( 'NONE', #16561, #76973, #47840, .T. ) ;
#40013=AXIS2_PLACEMENT_3D ( 'NONE', #70037, #76846, #55927 ) ;
#40014=ORIENTED_EDGE ( 'NONE', *, *, #53641, .T. ) ;
#40016=CARTESIAN_POINT ( 'NONE',  ( 172.5667039024480118, -36.32844715993499563, 180.4678068554150059 ) ) ;
#40017=DIRECTION ( 'NONE',  ( -0.7071067811866258435, 0.7071067811864693020, -7.071067811866266166E-16 ) ) ;
#40020=CARTESIAN_POINT ( 'NONE',  ( 115.6043783821399558, -39.74888713174190968, 177.9905150661719802 ) ) ;
#40021=CARTESIAN_POINT ( 'NONE',  ( 99.95068698205643898, -44.40877713917536340, 46.98133956162592284 ) ) ;
#40024=DIRECTION ( 'NONE',  ( 0.7071067811862279395, -0.7071067811868672059, 7.071067811862286363E-16 ) ) ;
#40025=ORIENTED_EDGE ( 'NONE', *, *, #27745, .T. ) ;
#40026=DIRECTION ( 'NONE',  ( -0.000000000000000000, -0.000000000000000000, -1.000000000000000000 ) ) ;
#40028=CARTESIAN_POINT ( 'NONE',  ( 108.2977246876245374, -26.73284728312218661, 165.9788891058625779 ) ) ;
#40030=CARTESIAN_POINT ( 'NONE',  ( 109.6417562379821931, -46.48040302697471304, 132.7813811145545344 ) ) ;
#40032=DIRECTION ( 'NONE',  ( 0.000000000000000000, 1.000000000000000000, 0.000000000000000000 ) ) ;
#40034=CARTESIAN_POINT ( 'NONE',  ( 104.2349294074198411, -46.78572220631293277, 22.35848241876792031 ) ) ;
#40035=CARTESIAN_POINT ( 'NONE',  ( 107.8717034087400322, -26.29179415218835913, 66.01562527591097762 ) ) ;
#40038=CARTESIAN_POINT ( 'NONE',  ( 143.0664832912740110, -18.82844715994099971, 284.9256252759119548 ) ) ;
#40039=CARTESIAN_POINT ( 'NONE',  ( 76.24325998657066350, -5.906223855237660914, 14.67562527591093868 ) ) ;
#40040=CARTESIAN_POINT ( 'NONE',  ( 179.4595971212733900, -26.00627455218473472, 237.4678068554150059 ) ) ;
#40041=ADVANCED_FACE ( 'NONE', ( #61927 ), #5644, .F. ) ;
#40045=EDGE_LOOP ( 'NONE', ( #36362, #51070, #64696, #43225 ) ) ;
#40046=CARTESIAN_POINT ( 'NONE',  ( 101.1165878437261227, -28.07204926635110098, 50.55562527591095545 ) ) ;
#40047=CARTESIAN_POINT ( 'NONE',  ( 109.6893229801689813, -47.49076295823797267, 83.75467289495897205 ) ) ;
#40050=DIRECTION ( 'NONE',  ( 0.000000000000000000, 1.000000000000000000, 0.000000000000000000 ) ) ;
#40052=CARTESIAN_POINT ( 'NONE',  ( 130.3998166246059895, 12.92155284005730387, 355.9756252759109998 ) ) ;
#40053=ORIENTED_EDGE ( 'NONE', *, *, #29490, .F. ) ;
#40054=CARTESIAN_POINT ( 'NONE',  ( 107.3174176841070846, -26.95189801805073060, 116.0556252759109555 ) ) ;
#40055=ADVANCED_FACE ( 'NONE', ( #81956, #48279 ), #61032, .T. ) ;
#40056=LINE ( 'NONE', #80982, #87769 ) ;
#40057=ORIENTED_EDGE ( 'NONE', *, *, #67405, .T. ) ;
#40058=CARTESIAN_POINT ( 'NONE',  ( 96.14807755961388125, -35.16348456217431107, 222.2251490854349640 ) ) ;
#40059=CARTESIAN_POINT ( 'NONE',  ( 116.8172402583773390, -34.15334170113332135, 255.0318177960892854 ) ) ;
#40060=CARTESIAN_POINT ( 'NONE',  ( 117.0885934270242217, -37.65783532839622438, 148.7525704246621103 ) ) ;
#40062=CARTESIAN_POINT ( 'NONE',  ( 25.56670390244797275, -65.37844715994100397, 137.2178068554150059 ) ) ;
#40064=CARTESIAN_POINT ( 'NONE',  ( 131.3164832912740110, -36.72944715994100306, 3.101481641215535046 ) ) ;
#40066=AXIS2_PLACEMENT_3D ( 'NONE', #26696, #4926, #47128 ) ;
#40067=CARTESIAN_POINT ( 'NONE',  ( 102.2868918306627961, -45.93239726994513461, 167.1832443235309995 ) ) ;
#40070=VECTOR ( 'NONE', #54585, 999.9999999999998863 ) ;
#40071=CARTESIAN_POINT ( 'NONE',  ( 102.8293847037436421, -28.94642981657014147, 141.9044404487549684 ) ) ;
#40072=AXIS2_PLACEMENT_3D ( 'NONE', #18029, #60696, #4856 ) ;
#40073=LINE ( 'NONE', #67791, #79143 ) ;
#40075=CARTESIAN_POINT ( 'NONE',  ( 99.85651329999866732, -30.12038005271842422, 271.7356252759109907 ) ) ;
#40076=LINE ( 'NONE', #59615, #84005 ) ;
#40078=CARTESIAN_POINT ( 'NONE',  ( 151.0371591254575776, -24.42818131005592264, 129.9678068554149775 ) ) ;
#40080=LINE ( 'NONE', #67797, #35677 ) ;
#40081=DIRECTION ( 'NONE',  ( -0.7071067811865779928, 0.7071067811865171526, -6.612322855860441069E-17 ) ) ;
#40084=CARTESIAN_POINT ( 'NONE',  ( 95.43233898611173061, -38.84956357215551748, 201.4699109901969791 ) ) ;
#40089=CARTESIAN_POINT ( 'NONE',  ( 182.3467384525650061, -29.62846900982231446, -5.074374724088000832 ) ) ;
#40090=CARTESIAN_POINT ( 'NONE',  ( 168.5667039024481255, -48.82844715993497431, 300.4678068554149490 ) ) ;
#40093=DIRECTION ( 'NONE',  ( 0.000000000000000000, 0.000000000000000000, 1.000000000000000000 ) ) ;
#40097=CARTESIAN_POINT ( 'NONE',  ( 101.3490469528152715, -46.18936307759902604, 202.1318157521019430 ) ) ;
#40098=CARTESIAN_POINT ( 'NONE',  ( 136.7703230406660566, -37.23127003359719822, 6.817519769821919873 ) ) ;
#40099=ORIENTED_EDGE ( 'NONE', *, *, #73141, .F. ) ;
#40101=CYLINDRICAL_SURFACE ( 'NONE', #62311, 10.00000000000002487 ) ;
#40102=CARTESIAN_POINT ( 'NONE',  ( 116.3175913315759402, -32.94491325663879877, 165.1356252759109680 ) ) ;
#40103=CARTESIAN_POINT ( 'NONE',  ( 101.3472728536945198, -42.59232338312836674, 19.77951894102097796 ) ) ;
#40104=CARTESIAN_POINT ( 'NONE',  ( 95.75547692839532488, -40.34654347423973775, 127.5727681330539554 ) ) ;
#40105=CARTESIAN_POINT ( 'NONE',  ( 75.31670390244798341, -67.87844715994100397, 33.40080685541480676 ) ) ;
#40107=VECTOR ( 'NONE', #25809, 1000.000000000000000 ) ;
#40109=CARTESIAN_POINT ( 'NONE',  ( 82.45780623542046328, -17.36823420008072105, 7.200493380652300601 ) ) ;
#40114=ORIENTED_EDGE ( 'NONE', *, *, #71993, .T. ) ;
#40116=CARTESIAN_POINT ( 'NONE',  ( 193.0374249753374443, -23.42844715993432558, 313.9678068554149490 ) ) ;
#40117=CARTESIAN_POINT ( 'NONE',  ( 97.46629167631436985, -35.27791395320982559, 70.62956268521996606 ) ) ;
#40118=CARTESIAN_POINT ( 'NONE',  ( 113.8136090879065563, -26.95650955708257257, 239.5956252759109759 ) ) ;
#40119=CARTESIAN_POINT ( 'NONE',  ( 100.0229104548316172, -27.23016881827663127, 185.5841967044829630 ) ) ;
#40120=CARTESIAN_POINT ( 'NONE',  ( 116.8768348252332174, -39.04445432745385602, 23.64277192200612276 ) ) ;
#40121=CARTESIAN_POINT ( 'NONE',  ( 96.53701874497966173, -40.09164955422465937, 277.5603871806729899 ) ) ;
#40122=LINE ( 'NONE', #47374, #39121 ) ;
#40125=EDGE_CURVE ( 'NONE', #57293, #29733, #47864, .T. ) ;
#40127=CIRCLE ( 'NONE', #47377, 0.5000000000000172085 ) ;
#40129=CARTESIAN_POINT ( 'NONE',  ( 97.99847537351134008, -44.43658864837386346, 226.8870538473399563 ) ) ;
#40132=CARTESIAN_POINT ( 'NONE',  ( 106.4836019150615840, -24.89303152268002606, 195.1156252759109861 ) ) ;
#40133=PLANE ( 'NONE',  #31156 ) ;
#40135=CARTESIAN_POINT ( 'NONE',  ( 97.86658156426001653, -40.64923495551180821, 22.64698795026609446 ) ) ;
#40136=DIRECTION ( 'NONE',  ( -0.7071067811865270336, 0.7071067811865680008, -7.071067811865277132E-16 ) ) ;
#40137=CARTESIAN_POINT ( 'NONE',  ( 113.5672778988914757, -32.00674077076433832, 277.6356252759110248 ) ) ;
#40138=CARTESIAN_POINT ( 'NONE',  ( 163.0667039024470171, -32.29483332968611364, -5.074374724088000832 ) ) ;
#40139=CARTESIAN_POINT ( 'NONE',  ( 99.50469279378565091, -43.30574573221327483, 172.8960156217824249 ) ) ;
#40143=CARTESIAN_POINT ( 'NONE',  ( 51.23005224011598102, -33.89581943344511217, 237.4678068554150059 ) ) ;
#40147=ORIENTED_EDGE ( 'NONE', *, *, #55926, .F. ) ;
#40148=CARTESIAN_POINT ( 'NONE',  ( 136.7895896102216113, -19.11755991740597693, 6.789748280179294326 ) ) ;
#40149=CARTESIAN_POINT ( 'NONE',  ( 96.75080816152406271, -34.86525579675927844, 241.1841967044819626 ) ) ;
#40150=CARTESIAN_POINT ( 'NONE',  ( 102.9710815734590454, -46.31642646611675218, 88.25562527591095829 ) ) ;
#40151=CARTESIAN_POINT ( 'NONE',  ( 96.84642183402544902, -30.63342722027062592, 276.8984824187680829 ) ) ;
#40152=CARTESIAN_POINT ( 'NONE',  ( 188.5667039024485518, -48.82844715993430640, 173.2178068554150059 ) ) ;
#40153=CARTESIAN_POINT ( 'NONE',  ( 107.0664832912739968, 22.62155284005901024, 339.0006252759110339 ) ) ;
#40157=DIRECTION ( 'NONE',  ( -0.7071067811607679721, 0.7071067812123270624, 0.000000000000000000 ) ) ;
#40158=DIRECTION ( 'NONE',  ( -1.000000000000000078E-15, 1.000000000000000083E-30, 1.000000000000000000 ) ) ;
#40161=VERTEX_POINT ( 'NONE', #71009 ) ;
#40162=CARTESIAN_POINT ( 'NONE',  ( 103.2107857629706018, -44.35110894017614669, 126.6267055423619610 ) ) ;
#40163=ADVANCED_FACE ( 'NONE', ( #22406 ), #21968, .T. ) ;
#40165=EDGE_LOOP ( 'NONE', ( #6188, #25050, #73763, #227 ) ) ;
#40166=DIRECTION ( 'NONE',  ( -1.000000000000000078E-15, 0.000000000000000000, -1.000000000000000000 ) ) ;
#40167=CARTESIAN_POINT ( 'NONE',  ( 103.4759237351581049, -46.49349013887657378, 138.2956252759109645 ) ) ;
#40168=DIRECTION ( 'NONE',  ( -0.9834602067153815907, -0.1811243269341220596, 0.000000000000000000 ) ) ;
#40170=EDGE_CURVE ( 'NONE', #16891, #14442, #49634, .T. ) ;
#40174=EDGE_CURVE ( 'NONE', #42012, #42564, #1961, .T. ) ;
#40175=CARTESIAN_POINT ( 'NONE',  ( 115.1932381579440943, -43.17108053757048935, 48.30514908543492680 ) ) ;
#40176=ORIENTED_EDGE ( 'NONE', *, *, #52741, .T. ) ;
#40177=VERTEX_POINT ( 'NONE', #29657 ) ;
#40178=CIRCLE ( 'NONE', #88050, 1.000000000000000888 ) ;
#40180=CARTESIAN_POINT ( 'NONE',  ( 41.56648329127399677, -9.303447159940999356, 76.80862527591200717 ) ) ;
#40181=CARTESIAN_POINT ( 'NONE',  ( 103.2204921605864314, -27.09891563476517717, 171.3908633711489813 ) ) ;
#40182=DIRECTION ( 'NONE',  ( 0.000000000000000000, -1.000000000000000000, 0.000000000000000000 ) ) ;
#40185=DIRECTION ( 'NONE',  ( 0.000000000000000000, 1.000000000000000000, 0.000000000000000000 ) ) ;
#40187=CARTESIAN_POINT ( 'NONE',  ( 138.8167039024479834, -67.87844715994100397, 58.80080685541479824 ) ) ;
#40188=CARTESIAN_POINT ( 'NONE',  ( 117.5733473178508319, -42.15660255127708211, 93.44705384733897802 ) ) ;
#40189=ORIENTED_EDGE ( 'NONE', *, *, #52011, .T. ) ;
#40190=VERTEX_POINT ( 'NONE', #85090 ) ;
#40196=CARTESIAN_POINT ( 'NONE',  ( 103.0775956431641305, -44.40992243120454930, 165.0014237029239439 ) ) ;
#40197=CIRCLE ( 'NONE', #30100, 0.5000000000000004441 ) ;
#40198=VECTOR ( 'NONE', #32164, 1000.000000000000000 ) ;
#40199=VECTOR ( 'NONE', #28836, 1000.000000000000000 ) ;
#40200=EDGE_CURVE ( 'NONE', #22706, #75722, #40178, .T. ) ;
#40202=ORIENTED_EDGE ( 'NONE', *, *, #50070, .T. ) ;
#40203=ORIENTED_EDGE ( 'NONE', *, *, #18529, .T. ) ;
#40204=DIRECTION ( 'NONE',  ( -1.000000000000000000, -3.999999999999999995E-14, -1.000000000000000078E-15 ) ) ;
#40205=CARTESIAN_POINT ( 'NONE',  ( 136.1637134159087168, -20.51083119282026246, 2.376725019081067369 ) ) ;
#40206=ORIENTED_EDGE ( 'NONE', *, *, #60667, .T. ) ;
#40207=ORIENTED_EDGE ( 'NONE', *, *, #17484, .T. ) ;
#40208=CARTESIAN_POINT ( 'NONE',  ( 77.41433294703951162, -19.45719076514804868, 6.889371645759243101 ) ) ;
#40209=CARTESIAN_POINT ( 'NONE',  ( 102.2066036383193222, -44.77047292137198298, 198.5634880678019272 ) ) ;
#40210=AXIS2_PLACEMENT_3D ( 'NONE', #51635, #86630, #23958 ) ;
#40211=CIRCLE ( 'NONE', #34387, 18.00000000000000355 ) ;
#40212=AXIS2_PLACEMENT_3D ( 'NONE', #11198, #32087, #23954 ) ;
#40214=DIRECTION ( 'NONE',  ( -1.000000000000000000, 0.000000000000000000, 0.000000000000000000 ) ) ;
#40215=ORIENTED_EDGE ( 'NONE', *, *, #50310, .F. ) ;
#40218=ADVANCED_FACE ( 'NONE', ( #28298 ), #64621, .F. ) ;
#40222=EDGE_CURVE ( 'NONE', #59530, #36232, #50536, .T. ) ;
#40223=CARTESIAN_POINT ( 'NONE',  ( 109.3322008939200458, -45.72736107978396092, 240.5909475124479684 ) ) ;
#40225=CARTESIAN_POINT ( 'NONE',  ( 98.18350318933659082, -43.34670532666833509, 111.8480062282919647 ) ) ;
#40226=CARTESIAN_POINT ( 'NONE',  ( 114.3378803067696765, -44.16957155219879638, 73.19276813305397411 ) ) ;
#40227=CARTESIAN_POINT ( 'NONE',  ( 100.1629373784320762, -32.34215477114681647, 249.5838068554172082 ) ) ;
#40228=CARTESIAN_POINT ( 'NONE',  ( 133.6902059199458677, -15.99866847873243358, 8.209451181316913093 ) ) ;
#40229=CARTESIAN_POINT ( 'NONE',  ( 108.0801309524341463, -25.31521737950549067, 322.2013064277864487 ) ) ;
#40230=CARTESIAN_POINT ( 'NONE',  ( 98.26135236841564335, -42.31085888804770434, 182.7756252759109543 ) ) ;
#40231=CARTESIAN_POINT ( 'NONE',  ( 164.9212702847356127, -29.73316016638977644, 237.4678068554150059 ) ) ;
#40232=EDGE_LOOP ( 'NONE', ( #65583, #2610, #41659, #84208 ) ) ;
#40235=VERTEX_POINT ( 'NONE', #35564 ) ;
#40237=ORIENTED_EDGE ( 'NONE', *, *, #54046, .F. ) ;
#40239=ORIENTED_EDGE ( 'NONE', *, *, #23370, .F. ) ;
#40240=VECTOR ( 'NONE', #46958, 1000.000000000000000 ) ;
#40241=EDGE_CURVE ( 'NONE', #14889, #76782, #88551, .T. ) ;
#40243=CARTESIAN_POINT ( 'NONE',  ( 101.9936209152398163, -45.44607152400298844, 177.1564586071733913 ) ) ;
#40244=CARTESIAN_POINT ( 'NONE',  ( 116.9750915152277884, -33.48807190773455034, 89.07848241876791917 ) ) ;
#40245=CARTESIAN_POINT ( 'NONE',  ( 112.1432782410116005, -28.01507713225257135, 254.6564226208779473 ) ) ;
#40246=ADVANCED_FACE ( 'NONE', ( #81303 ), #18595, .F. ) ;
#40247=CARTESIAN_POINT ( 'NONE',  ( 136.8164812439621016, -36.63640413217029135, 6.749771997051099426 ) ) ;
#40248=DIRECTION ( 'NONE',  ( -0.7071067811864634178, 0.7071067811866316166, -7.071067811864642099E-16 ) ) ;
#40251=CARTESIAN_POINT ( 'NONE',  ( 110.1310368924891208, -26.13358316477614451, 210.8403871806729626 ) ) ;
#40253=CARTESIAN_POINT ( 'NONE',  ( 71.24076473329807868, 5.642044068322332961, 361.9756252759101471 ) ) ;
#40254=ORIENTED_EDGE ( 'NONE', *, *, #44744, .T. ) ;
#40256=ADVANCED_FACE ( 'NONE', ( #81744 ), #2472, .T. ) ;
#40257=CARTESIAN_POINT ( 'NONE',  ( 33.81648329127400388, 12.92155284005802685, 336.5756252759108520 ) ) ;
#40258=DIRECTION ( 'NONE',  ( -1.000000000000000000, 0.000000000000000000, 0.000000000000000000 ) ) ;
#40261=CARTESIAN_POINT ( 'NONE',  ( 118.7030916724021665, -39.22306760090339139, 258.6584824187677896 ) ) ;
#40263=DIRECTION ( 'NONE',  ( -1.000000000000000078E-15, -1.000000000000000083E-30, 1.000000000000000000 ) ) ;
#40264=CARTESIAN_POINT ( 'NONE',  ( 100.5976686157419806, -28.50914727160554207, 11.60705384733995515 ) ) ;
#40265=CARTESIAN_POINT ( 'NONE',  ( 117.8455077981468122, -34.08178244914028454, 160.0061014663869798 ) ) ;
#40267=FACE_BOUND ( 'NONE', #72290, .T. ) ;
#40270=CARTESIAN_POINT ( 'NONE',  ( 49.21437657594998427, -35.91149509761070391, -5.074374724088000832 ) ) ;
#40271=DIRECTION ( 'NONE',  ( 0.000000000000000000, 0.000000000000000000, 1.000000000000000000 ) ) ;
#40273=VERTEX_POINT ( 'NONE', #47176 ) ;
#40275=CIRCLE ( 'NONE', #78034, 6.999999999999997335 ) ;
#40276=EDGE_LOOP ( 'NONE', ( #77104, #82098, #6117, #39498 ) ) ;
#40278=EDGE_CURVE ( 'NONE', #55604, #70047, #11792, .T. ) ;
#40279=VECTOR ( 'NONE', #20772, 1000.000000000000000 ) ;
#40280=VERTEX_POINT ( 'NONE', #32669 ) ;
#40282=CARTESIAN_POINT ( 'NONE',  ( 96.71096103112840581, -32.93116260832598385, 17.03467289495896964 ) ) ;
#40283=DIRECTION ( 'NONE',  ( 0.000000000000000000, 1.000000000000000000, 0.000000000000000000 ) ) ;
#40284=EDGE_CURVE ( 'NONE', #28809, #25358, #49957, .T. ) ;
#40287=CARTESIAN_POINT ( 'NONE',  ( 117.1097670608697143, -36.65276801037281018, 118.8336923977722250 ) ) ;
#40288=DIRECTION ( 'NONE',  ( 1.000000000000000078E-15, 0.000000000000000000, 1.000000000000000000 ) ) ;
#40290=EDGE_CURVE ( 'NONE', #68161, #17652, #30992, .T. ) ;
#40292=CARTESIAN_POINT ( 'NONE',  ( 114.3529501776022244, -31.35170872818512322, 258.7428960185527558 ) ) ;
#40293=ORIENTED_EDGE ( 'NONE', *, *, #43889, .F. ) ;
#40294=ORIENTED_EDGE ( 'NONE', *, *, #41530, .F. ) ;
#40296=FACE_OUTER_BOUND ( 'NONE', #4237, .T. ) ;
#40297=CARTESIAN_POINT ( 'NONE',  ( 138.8167039024479834, -57.40094715994099772, 37.63480685541480852 ) ) ;
#40298=DIRECTION ( 'NONE',  ( -0.000000000000000000, -0.000000000000000000, 1.000000000000000000 ) ) ;
#40299=CARTESIAN_POINT ( 'NONE',  ( 116.3251852747984003, -32.94148267319277323, 269.1356252759109680 ) ) ;
#40300=CARTESIAN_POINT ( 'NONE',  ( 115.8966032383871436, -37.77400989437322210, 50.16444044875395747 ) ) ;
#40301=DIRECTION ( 'NONE',  ( -4.237773401492740281E-14, 1.000000000000000000, 0.000000000000000000 ) ) ;
#40303=CARTESIAN_POINT ( 'NONE',  ( 115.3604274781777264, -30.50455558986040572, 264.3508633711496714 ) ) ;
#40304=ORIENTED_EDGE ( 'NONE', *, *, #71386, .F. ) ;
#40305=DIRECTION ( 'NONE',  ( -0.7071067811856560636, -0.7071067811874389708, 0.000000000000000000 ) ) ;
#40306=VECTOR ( 'NONE', #42320, 1000.000000000000000 ) ;
#40307=CARTESIAN_POINT ( 'NONE',  ( 165.2748236753140247, -30.08671355700301575, -5.074374724088000832 ) ) ;
#40308=CARTESIAN_POINT ( 'NONE',  ( 111.5696292435227122, -29.33873666780462486, 47.44713798863897836 ) ) ;
#40310=CARTESIAN_POINT ( 'NONE',  ( 136.1934021726284243, -16.98608769072011881, 7.448832051635106311 ) ) ;
#40312=CARTESIAN_POINT ( 'NONE',  ( 141.8545562996767444, -1.932463243632623229, 361.9756252759100335 ) ) ;
#40313=ORIENTED_EDGE ( 'NONE', *, *, #77635, .F. ) ;
#40314=CARTESIAN_POINT ( 'NONE',  ( 77.54412859703519700, -35.63380991825863475, 7.053480412781513387 ) ) ;
#40316=CARTESIAN_POINT ( 'NONE',  ( 114.4629700169191580, -28.51537706926042404, 159.5051490854349652 ) ) ;
#40317=VERTEX_POINT ( 'NONE', #16482 ) ;
#40318=CARTESIAN_POINT ( 'NONE',  ( 116.7149163912777396, -35.64392129247566032, 83.33813411379098568 ) ) ;
#40320=CARTESIAN_POINT ( 'NONE',  ( 113.6158397245882128, -43.46609735470438807, 114.6339642582779561 ) ) ;
#40321=CARTESIAN_POINT ( 'NONE',  ( 64.68306507141296890, -72.55818180160879649, 361.9756252759101471 ) ) ;
#40323=DIRECTION ( 'NONE',  ( 1.000000000000000078E-15, -1.000000000000000083E-30, -1.000000000000000000 ) ) ;
#40324=CARTESIAN_POINT ( 'NONE',  ( 98.28804800891427362, -28.73186473263583807, 76.73848241876795839 ) ) ;
#40325=PLANE ( 'NONE',  #58482 ) ;
#40326=DIRECTION ( 'NONE',  ( 1.000000000000000078E-15, -1.000000000000000083E-30, -1.000000000000000000 ) ) ;
#40329=AXIS2_PLACEMENT_3D ( 'NONE', #67987, #88891, #54318 ) ;
#40330=DIRECTION ( 'NONE',  ( -0.7071067811865671127, -0.7071067811865279218, -7.071067811865664660E-16 ) ) ;
#40331=ORIENTED_EDGE ( 'NONE', *, *, #54252, .F. ) ;
#40333=ADVANCED_FACE ( 'NONE', ( #30554 ), #58252, .F. ) ;
#40335=CIRCLE ( 'NONE', #27315, 0.5000000000000031086 ) ;
#40336=ADVANCED_FACE ( 'NONE', ( #16929 ), #25409, .T. ) ;
#40337=CARTESIAN_POINT ( 'NONE',  ( 76.06670390244809710, -58.72944715994109544, 199.5838068554169524 ) ) ;
#40338=ORIENTED_EDGE ( 'NONE', *, *, #3657, .T. ) ;
#40339=CARTESIAN_POINT ( 'NONE',  ( 110.5849939505706772, -26.97450646431652643, 249.7889586092449576 ) ) ;
#40340=CARTESIAN_POINT ( 'NONE',  ( 108.0088980509730305, -26.32399177548269620, 151.0041967044829505 ) ) ;
#40341=DIRECTION ( 'NONE',  ( 0.9068632946707805287, -0.4214249218767882610, 9.493511560072084562E-16 ) ) ;
#40343=CARTESIAN_POINT ( 'NONE',  ( 115.1668113632844808, -43.29200554620488361, 84.28419670448195689 ) ) ;
#40344=CARTESIAN_POINT ( 'NONE',  ( 97.07216058387446367, -35.37757943919933012, 97.21864571800702493 ) ) ;
#40347=CARTESIAN_POINT ( 'NONE',  ( 21.03689327557615130, -23.42844715994197813, 180.4678068554150911 ) ) ;
#40351=CARTESIAN_POINT ( 'NONE',  ( 48.79742451362098166, -36.32844715994040996, -5.074374724088000832 ) ) ;
#40354=DIRECTION ( 'NONE',  ( 1.000000000000000078E-15, 0.000000000000000000, 1.000000000000000000 ) ) ;
#40355=LINE ( 'NONE', #33980, #52674 ) ;
#40356=CARTESIAN_POINT ( 'NONE',  ( 111.8540205700169139, -46.00543295620339990, 272.9556252759110180 ) ) ;
#40357=LINE ( 'NONE', #21266, #77985 ) ;
#40359=CARTESIAN_POINT ( 'NONE',  ( 117.0614924034066036, -38.07622789054436652, 93.71956107247139300 ) ) ;
#40360=ADVANCED_FACE ( 'NONE', ( #13572 ), #41262, .F. ) ;
#40361=CARTESIAN_POINT ( 'NONE',  ( 97.36980136507975203, -37.22440909395530184, 270.7895626852197779 ) ) ;
#40362=CARTESIAN_POINT ( 'NONE',  ( 113.2072602631850060, -28.80268442222084602, 99.55275712281951428 ) ) ;
#40363=CARTESIAN_POINT ( 'NONE',  ( 95.51222647996985415, -34.21005103128004521, 102.1556252759109640 ) ) ;
#40364=CARTESIAN_POINT ( 'NONE',  ( 182.5667039024469886, -33.35206098992650681, -5.074374724088000832 ) ) ;
#40365=CARTESIAN_POINT ( 'NONE',  ( 105.3088311808849937, -48.49934056980919905, 147.4584824187679715 ) ) ;
#40367=CARTESIAN_POINT ( 'NONE',  ( 182.4202572930268502, -31.94127993907054730, 117.4678068554150627 ) ) ;
#40370=LINE ( 'NONE', #32206, #10564 ) ;
#40371=CARTESIAN_POINT ( 'NONE',  ( 107.0664832912739541, -23.22944715994095688, 312.1356252759112522 ) ) ;
#40372=DIRECTION ( 'NONE',  ( -1.000000000000000000, -4.299999999999999979E-14, -1.000000000000000078E-15 ) ) ;
#40373=EDGE_LOOP ( 'NONE', ( #8012, #65968, #86478, #3380, #63350, #77943, #77112, #60136, #15509, #3318, #78633, #41180, #34666, #83837, #60376, #71970, #37580, #17874, #21000, #181, #64778, #80955, #23500, #7324, #37674, #8336, #20, #52388, #55666, #23780, #75466, #34263, #42895, #29519, #41789, #63238, #33078, #70635, #89604, #47215, #75055, #82950, #42647, #20504, #61005, #61464, #81984, #15005 ) ) ;
#40374=EDGE_CURVE ( 'NONE', #59914, #59817, #89899, .T. ) ;
#40376=CARTESIAN_POINT ( 'NONE',  ( 114.2052324763531743, -45.22952987728847063, 148.1203871806719405 ) ) ;
#40381=CARTESIAN_POINT ( 'NONE',  ( 112.0659116179119650, -45.48839626324947005, 118.9897919421637198 ) ) ;
#40382=EDGE_CURVE ( 'NONE', #52251, #46008, #27651, .T. ) ;
#40383=DIRECTION ( 'NONE',  ( 4.299999999999999979E-14, -1.000000000000000000, 0.000000000000000000 ) ) ;
#40387=ORIENTED_EDGE ( 'NONE', *, *, #22556, .F. ) ;
#40388=ORIENTED_EDGE ( 'NONE', *, *, #71880, .T. ) ;
#40389=VERTEX_POINT ( 'NONE', #83977 ) ;
#40392=CARTESIAN_POINT ( 'NONE',  ( 90.44969454456408187, -20.11243780205710507, 239.5838068554175209 ) ) ;
#40395=DIRECTION ( 'NONE',  ( 0.000000000000000000, 0.000000000000000000, 1.000000000000000000 ) ) ;
#40396=DIRECTION ( 'NONE',  ( 0.000000000000000000, 0.000000000000000000, -1.000000000000000000 ) ) ;
#40399=VECTOR ( 'NONE', #26768, 1000.000000000000000 ) ;
#40401=VERTEX_POINT ( 'NONE', #69888 ) ;
#40402=( BOUNDED_CURVE ( )  B_SPLINE_CURVE ( 3, ( #3888, #58836, #79767, #80211 ),
 .UNSPECIFIED., .F., .F. ) 
 B_SPLINE_CURVE_WITH_KNOTS ( ( 4, 4 ),
 ( 5.086905507537815818E-12, 1.570796326801274345 ),
 .UNSPECIFIED. ) 
 CURVE ( )  GEOMETRIC_REPRESENTATION_ITEM ( )  RATIONAL_B_SPLINE_CURVE ( ( 1.000000000000000000, 0.8047378541240607364, 0.8047378541240607364, 1.000000000000000000 ) ) 
 REPRESENTATION_ITEM ( '' )  );
#40403=DIRECTION ( 'NONE',  ( 4.299999999999999979E-14, -1.000000000000000000, 4.400000000000000367E-29 ) ) ;
#40404=CARTESIAN_POINT ( 'NONE',  ( 172.5664832912740110, -36.32844715994070839, 323.6756252759119548 ) ) ;
#40405=CARTESIAN_POINT ( 'NONE',  ( 114.3351522754912963, -30.13549343754564092, 205.4127681330539872 ) ) ;
#40407=EDGE_LOOP ( 'NONE', ( #25227, #46330 ) ) ;
#40409=CARTESIAN_POINT ( 'NONE',  ( 106.6854394624702849, -26.95610377642496758, 81.10705384733896040 ) ) ;
#40410=DIRECTION ( 'NONE',  ( -8.673617379884035472E-16, -1.000000000000000000, 0.000000000000000000 ) ) ;
#40413=ORIENTED_EDGE ( 'NONE', *, *, #71946, .F. ) ;
#40414=EDGE_CURVE ( 'NONE', #27495, #56128, #62165, .T. ) ;
#40415=CARTESIAN_POINT ( 'NONE',  ( 107.0667039024479834, -36.72944715994100306, 239.5838068554170093 ) ) ;
#40418=CARTESIAN_POINT ( 'NONE',  ( 109.5261983718769585, -46.49778922373468504, 239.2044404487539566 ) ) ;
#40419=ADVANCED_FACE ( 'NONE', ( #33567 ), #61706, .F. ) ;
#40422=CARTESIAN_POINT ( 'NONE',  ( 116.3215253324775773, -32.93968801256757217, 155.1356252759109680 ) ) ;
#40423=AXIS2_PLACEMENT_3D ( 'NONE', #44922, #46703, #60335 ) ;
#40425=ORIENTED_EDGE ( 'NONE', *, *, #40382, .T. ) ;
#40426=FACE_OUTER_BOUND ( 'NONE', #56034, .T. ) ;
#40427=CARTESIAN_POINT ( 'NONE',  ( 179.7974245136200011, -36.32844715994040996, -5.074374724088000832 ) ) ;
#40428=ORIENTED_EDGE ( 'NONE', *, *, #59083, .T. ) ;
#40429=CARTESIAN_POINT ( 'NONE',  ( 111.3232390708907786, -27.21277439355663219, 24.74133956162494030 ) ) ;
#40431=CARTESIAN_POINT ( 'NONE',  ( 111.2517653011026226, -44.30469234039772886, 250.7842808457816375 ) ) ;
#40432=DIRECTION ( 'NONE',  ( -0.7071067811865692221, -0.7071067811865259234, -7.071067811865685367E-16 ) ) ;
#40433=CARTESIAN_POINT ( 'NONE',  ( 112.9441315310009628, -44.54716313336201949, 143.0899109901969553 ) ) ;
#40434=CARTESIAN_POINT ( 'NONE',  ( 130.0664832912740110, -18.82844715994099971, 199.5838068554170093 ) ) ;
#40435=LINE ( 'NONE', #74515, #33123 ) ;
#40438=AXIS2_PLACEMENT_3D ( 'NONE', #12835, #39618, #11021 ) ;
#40439=CARTESIAN_POINT ( 'NONE',  ( 95.24589774366052097, -38.10235284316662074, 232.4184824187679794 ) ) ;
#40442=CARTESIAN_POINT ( 'NONE',  ( 103.2630468498471856, -47.15688066943211254, 93.28610146638693834 ) ) ;
#40445=ORIENTED_EDGE ( 'NONE', *, *, #36008, .T. ) ;
#40448=ORIENTED_EDGE ( 'NONE', *, *, #73394, .T. ) ;
#40451=CARTESIAN_POINT ( 'NONE',  ( 172.5664832912740110, -18.82844715994099971, 136.8086252759119645 ) ) ;
#40453=CARTESIAN_POINT ( 'NONE',  ( 48.16670390244701139, -28.27351298637280408, -5.074374724088000832 ) ) ;
#40454=CARTESIAN_POINT ( 'NONE',  ( 98.41263308787671349, -36.61538842024999241, 154.1461856076869594 ) ) ;
#40455=CARTESIAN_POINT ( 'NONE',  ( 96.86769303131731590, -30.64611497598638579, 276.8984824187680829 ) ) ;
#40456=CARTESIAN_POINT ( 'NONE',  ( 98.38040403964905067, -41.69523976407170096, 57.73976173181551275 ) ) ;
#40457=ORIENTED_EDGE ( 'NONE', *, *, #8162, .T. ) ;
#40459=CIRCLE ( 'NONE', #33203, 4.750000000000000888 ) ;
#40460=EDGE_CURVE ( 'NONE', #41221, #41944, #75360, .T. ) ;
#40461=DIRECTION ( 'NONE',  ( -2.999999999999999839E-15, 1.000000000000000000, -2.999999999999999900E-30 ) ) ;
#40462=VERTEX_POINT ( 'NONE', #21289 ) ;
#40463=ORIENTED_EDGE ( 'NONE', *, *, #36332, .F. ) ;
#40464=AXIS2_PLACEMENT_3D ( 'NONE', #29823, #65228, #17525 ) ;
#40466=EDGE_CURVE ( 'NONE', #30894, #89471, #7216, .T. ) ;
#40467=CARTESIAN_POINT ( 'NONE',  ( 165.6738106836030227, -28.98061976758901892, -5.074374724088000832 ) ) ;
#40470=CARTESIAN_POINT ( 'NONE',  ( 178.6914832912739826, 12.92155284005802685, 335.5992267699913327 ) ) ;
#40474=EDGE_CURVE ( 'NONE', #73333, #7861, #62617, .T. ) ;
#40475=CARTESIAN_POINT ( 'NONE',  ( 114.9272539996656377, -40.07076659875138347, 167.9295626852199632 ) ) ;
#40476=CARTESIAN_POINT ( 'NONE',  ( 117.0961560025638306, -31.97355093185684538, 64.19086337114899266 ) ) ;
#40477=LINE ( 'NONE', #33666, #79982 ) ;
#40478=ORIENTED_EDGE ( 'NONE', *, *, #41118, .T. ) ;
#40479=CARTESIAN_POINT ( 'NONE',  ( 164.9212702847350158, -29.73316016639540749, 117.4678068554150485 ) ) ;
#40481=AXIS2_PLACEMENT_3D ( 'NONE', #48001, #12168, #75739 ) ;
#40485=AXIS2_PLACEMENT_3D ( 'NONE', #1526, #29228, #56914 ) ;
#40486=FACE_OUTER_BOUND ( 'NONE', #21428, .T. ) ;
#40487=CARTESIAN_POINT ( 'NONE',  ( 98.15097650629928694, -41.26161077846109038, 131.7007372803578562 ) ) ;
#40488=B_SPLINE_CURVE_WITH_KNOTS ( 'NONE', 3,
 ( #40422, #26351, #33611, #60862, #5013, #4570, #46769, #13178, #19990, #5923, #68137, #25453, #89029, #18641, #61747, #20441, #88592, #47671 ),
 .UNSPECIFIED., .F., .F.,
 ( 4, 2, 2, 2, 2, 2, 2, 2, 4 ),
 ( 0.000000000000000000, 0.06250000028368622729, 0.1250000005673724546, 0.1875000008510586680, 0.2500000011347449091, 0.3125000014184311503, 0.3750000017021173360, 0.4375000019858035771, 0.5000000022694898183 ),
 .UNSPECIFIED. ) ;
#40490=EDGE_LOOP ( 'NONE', ( #34370, #64864, #10451, #49592 ) ) ;
#40491=CARTESIAN_POINT ( 'NONE',  ( 115.9104104090373539, -31.16785412357883800, 34.27276813305396530 ) ) ;
#40492=CARTESIAN_POINT ( 'NONE',  ( 106.9267702420067678, -26.22618599733332090, 56.08705384733997334 ) ) ;
#40496=CARTESIAN_POINT ( 'NONE',  ( 142.8682495647594806, 8.654319075478440482, 542.9756252759101471 ) ) ;
#40498=AXIS2_PLACEMENT_3D ( 'NONE', #83616, #48603, #47716 ) ;
#40499=DIRECTION ( 'NONE',  ( 0.000000000000000000, 1.000000000000000000, 0.000000000000000000 ) ) ;
#40501=CARTESIAN_POINT ( 'NONE',  ( 37.06648329127400388, 12.92155284005802685, 335.5992267699910485 ) ) ;
#40503=CARTESIAN_POINT ( 'NONE',  ( 96.61744970692362244, -37.56424831167382195, 97.38991099019594344 ) ) ;
#40508=CONICAL_SURFACE ( 'NONE', #23164, 1.219499999999975159, 1.047197551196598297 ) ;
#40509=DIRECTION ( 'NONE',  ( 0.000000000000000000, 0.000000000000000000, 1.000000000000000000 ) ) ;
#40510=ORIENTED_EDGE ( 'NONE', *, *, #60123, .T. ) ;
#40511=CARTESIAN_POINT ( 'NONE',  ( 106.1376555893193370, -47.80867374849567852, 108.5099109901959622 ) ) ;
#40513=ORIENTED_EDGE ( 'NONE', *, *, #53976, .T. ) ;
#40514=CARTESIAN_POINT ( 'NONE',  ( 100.7633749303631561, -45.78122309449478422, 233.0803871806729717 ) ) ;
#40515=FACE_OUTER_BOUND ( 'NONE', #5685, .T. ) ;
#40516=CARTESIAN_POINT ( 'NONE',  ( 110.8966428001789524, -45.96688915401393416, 147.8892538962421952 ) ) ;
#40517=FACE_OUTER_BOUND ( 'NONE', #792, .T. ) ;
#40518=FACE_OUTER_BOUND ( 'NONE', #69229, .T. ) ;
#40519=VECTOR ( 'NONE', #86318, 1000.000000000000000 ) ;
#40521=CARTESIAN_POINT ( 'NONE',  ( 161.4809174648185603, -49.32844715993547169, 180.4678068554150059 ) ) ;
#40522=CARTESIAN_POINT ( 'NONE',  ( 113.8091913586854531, -43.81457933525494042, 158.1813395616259754 ) ) ;
#40526=CARTESIAN_POINT ( 'NONE',  ( 108.8812380984771835, -28.05563920549329993, 136.3444404487549662 ) ) ;
#40529=PLANE ( 'NONE',  #19662 ) ;
#40530=CARTESIAN_POINT ( 'NONE',  ( 110.5849939505706487, -26.97450646431661880, 245.7889586092439629 ) ) ;
#40531=DIRECTION ( 'NONE',  ( 1.639958061481212836E-42, -4.100000000000000342E-29, -1.000000000000000000 ) ) ;
#40532=DIRECTION ( 'NONE',  ( 1.000000000000000078E-15, -1.000000000000000083E-30, -1.000000000000000000 ) ) ;
#40533=LINE ( 'NONE', #88706, #28691 ) ;
#40534=AXIS2_PLACEMENT_3D ( 'NONE', #43421, #758, #14405 ) ;
#40536=FACE_OUTER_BOUND ( 'NONE', #47118, .T. ) ;
#40539=CARTESIAN_POINT ( 'NONE',  ( 98.45302666770167832, -29.83944080489365902, 195.7775300378159784 ) ) ;
#40540=CARTESIAN_POINT ( 'NONE',  ( 31.71315051185510114, -33.70561438052087055, 313.9678068554150059 ) ) ;
#40541=ORIENTED_EDGE ( 'NONE', *, *, #77893, .F. ) ;
#40542=VERTEX_POINT ( 'NONE', #63513 ) ;
#40543=DIRECTION ( 'NONE',  ( -0.9254794337955620787, -0.3787978585227822492, 0.000000000000000000 ) ) ;
#40545=CIRCLE ( 'NONE', #18832, 1.571100913904416307 ) ;
#40546=CARTESIAN_POINT ( 'NONE',  ( 48.16670390244752298, -28.27351298637377397, 237.4678068554150059 ) ) ;
#40547=LINE ( 'NONE', #5134, #53464 ) ;
#40549=ORIENTED_EDGE ( 'NONE', *, *, #71550, .T. ) ;
#40550=DIRECTION ( 'NONE',  ( 0.000000000000000000, 0.000000000000000000, -1.000000000000000000 ) ) ;
#40551=CARTESIAN_POINT ( 'NONE',  ( 116.8576245982602870, -40.31003124190988274, 218.5470538473399529 ) ) ;
#40553=VERTEX_POINT ( 'NONE', #49868 ) ;
#40555=EDGE_CURVE ( 'NONE', #9081, #62285, #35838, .T. ) ;
#40558=EDGE_CURVE ( 'NONE', #55655, #13929, #50319, .T. ) ;
#40559=CARTESIAN_POINT ( 'NONE',  ( 99.04397795006340743, -42.84113160514387886, 162.8439467858095213 ) ) ;
#40560=CARTESIAN_POINT ( 'NONE',  ( 98.94126815719160106, -33.74921318831734851, 18.85285227435401367 ) ) ;
#40561=CARTESIAN_POINT ( 'NONE',  ( 96.03095270115332482, -35.77956804193283347, 182.2461014663869889 ) ) ;
#40563=ORIENTED_EDGE ( 'NONE', *, *, #24535, .F. ) ;
#40567=CARTESIAN_POINT ( 'NONE',  ( 114.8447031547741943, -43.15207964168884303, 68.27931773607517130 ) ) ;
#40568=ORIENTED_EDGE ( 'NONE', *, *, #14776, .T. ) ;
#40569=VERTEX_POINT ( 'NONE', #16716 ) ;
#40570=DIRECTION ( 'NONE',  ( 1.000000000000000078E-15, 0.000000000000000000, 1.000000000000000000 ) ) ;
#40572=EDGE_LOOP ( 'NONE', ( #27109, #22216, #14823, #41677 ) ) ;
#40575=CARTESIAN_POINT ( 'NONE',  ( 104.2253390597007581, -44.78450961640034222, 56.72956268521994616 ) ) ;
#40576=CARTESIAN_POINT ( 'NONE',  ( 117.5128880048294491, -35.85709896013243281, 253.8927681330537780 ) ) ;
#40577=CIRCLE ( 'NONE', #36249, 3.000000000000002665 ) ;
#40578=CARTESIAN_POINT ( 'NONE',  ( 100.6510976905701824, -26.79511100149714764, 220.5327681330539633 ) ) ;
#40579=CARTESIAN_POINT ( 'NONE',  ( 116.7834531110833325, -34.06957675735675650, 24.03834616677710656 ) ) ;
#40580=CARTESIAN_POINT ( 'NONE',  ( 100.4791399132689236, -44.80881982087480964, 8.032768133053981074 ) ) ;
#40581=DIRECTION ( 'NONE',  ( -1.000000000000000078E-15, 1.000000000000000083E-30, 1.000000000000000000 ) ) ;
#40582=LINE ( 'NONE', #13334, #38068 ) ;
#40583=CONICAL_SURFACE ( 'NONE', #11618, 1.625000000000001332, 1.029744258676650093 ) ;
#40584=EDGE_LOOP ( 'NONE', ( #70119, #4064, #89634, #87071 ) ) ;
#40587=LINE ( 'NONE', #11554, #48700 ) ;
#40588=CARTESIAN_POINT ( 'NONE',  ( 100.1093887754828984, -44.55284168805902567, 266.9984824187678782 ) ) ;
#40589=ORIENTED_EDGE ( 'NONE', *, *, #4550, .F. ) ;
#40590=CARTESIAN_POINT ( 'NONE',  ( 110.4989391570660473, -26.88539935475378684, 209.8099109901969541 ) ) ;
#40591=LINE ( 'NONE', #47385, #67395 ) ;
#40592=FACE_OUTER_BOUND ( 'NONE', #5281, .T. ) ;
#40594=CARTESIAN_POINT ( 'NONE',  ( 110.1624778137653067, -46.32779280511170583, 28.82556394023509938 ) ) ;
#40595=CARTESIAN_POINT ( 'NONE',  ( 99.76018885984304063, -32.42404554134276395, 277.6356252759108543 ) ) ;
#40596=LINE ( 'NONE', #82853, #63049 ) ;
#40599=CARTESIAN_POINT ( 'NONE',  ( 164.9190312289455278, -35.91149509760636960, 193.9678068554149775 ) ) ;
#40600=AXIS2_PLACEMENT_3D ( 'NONE', #22371, #43690, #8751 ) ;
#40602=LINE ( 'NONE', #8152, #70852 ) ;
#40604=CARTESIAN_POINT ( 'NONE',  ( 86.06670390244796920, -48.82844715994099971, 198.9178068554149945 ) ) ;
#40605=CARTESIAN_POINT ( 'NONE',  ( 101.0707582237941438, -29.13849289886354299, 195.5838068554168672 ) ) ;
#40606=ORIENTED_EDGE ( 'NONE', *, *, #51612, .T. ) ;
#40607=CARTESIAN_POINT ( 'NONE',  ( 25.56670390244797275, -65.37844715994100397, 288.3428068554150059 ) ) ;
#40608=CARTESIAN_POINT ( 'NONE',  ( 106.8511556536399780, -47.80415145147887301, 227.5489586092439538 ) ) ;
#40609=CARTESIAN_POINT ( 'NONE',  ( 114.0221110621602492, -28.96402831996850225, 110.4956252759109816 ) ) ;
#40610=CARTESIAN_POINT ( 'NONE',  ( 110.8324567285566076, -26.28842506301429083, 245.7889586092439629 ) ) ;
#40611=LINE ( 'NONE', #61494, #74467 ) ;
#40612=AXIS2_PLACEMENT_3D ( 'NONE', #81291, #5872, #5417 ) ;
#40617=DIRECTION ( 'NONE',  ( 0.000000000000000000, 0.000000000000000000, -1.000000000000000000 ) ) ;
#40619=ADVANCED_FACE ( 'NONE', ( #58044 ), #15825, .T. ) ;
#40623=CARTESIAN_POINT ( 'NONE',  ( 115.1266331755855958, -39.55612640683342107, 132.9809912566479397 ) ) ;
#40624=LINE ( 'NONE', #32909, #32840 ) ;
#40625=ORIENTED_EDGE ( 'NONE', *, *, #87090, .F. ) ;
#40627=CARTESIAN_POINT ( 'NONE',  ( 114.7100688122352494, -43.78666090992606996, 119.2327681330539804 ) ) ;
#40629=DIRECTION ( 'NONE',  ( 1.000000000000000078E-15, -1.000000000000000083E-30, -1.000000000000000000 ) ) ;
#40630=DIRECTION ( 'NONE',  ( 0.000000000000000000, 0.000000000000000000, 1.000000000000000000 ) ) ;
#40631=CARTESIAN_POINT ( 'NONE',  ( 107.0664832912739541, -23.72944715994095688, 315.6356252759111953 ) ) ;
#40632=CARTESIAN_POINT ( 'NONE',  ( 104.9021620152489191, -46.26774620671726268, 72.39848241876894974 ) ) ;
#40637=EDGE_CURVE ( 'NONE', #11683, #63148, #44519, .T. ) ;
#40638=CARTESIAN_POINT ( 'NONE',  ( 107.0664832912750057, -36.72944715993903486, 9.425625275910970657 ) ) ;
#40639=CARTESIAN_POINT ( 'NONE',  ( 102.2868918306628387, -45.93239726994502803, 163.1832443235289816 ) ) ;
#40640=CARTESIAN_POINT ( 'NONE',  ( 49.21213752015764697, -29.73316016639473958, 117.4678068554150485 ) ) ;
#40642=DIRECTION ( 'NONE',  ( -1.000000000000000000, -4.299999999999999979E-14, -1.000000000000000078E-15 ) ) ;
#40643=VECTOR ( 'NONE', #9942, 1000.000000000000000 ) ;
#40644=LINE ( 'NONE', #46095, #1358 ) ;
#40645=DIRECTION ( 'NONE',  ( -0.000000000000000000, -0.000000000000000000, 1.000000000000000000 ) ) ;
#40646=CARTESIAN_POINT ( 'NONE',  ( 116.6546583390153131, -32.60254457568996855, 79.14991099019697174 ) ) ;
#40647=VERTEX_POINT ( 'NONE', #29004 ) ;
#40648=ORIENTED_EDGE ( 'NONE', *, *, #16064, .T. ) ;
#40650=VECTOR ( 'NONE', #82315, 1000.000000000000114 ) ;
#40651=EDGE_CURVE ( 'NONE', #54776, #7655, #4446, .T. ) ;
#40655=CARTESIAN_POINT ( 'NONE',  ( 108.8610815749077574, -28.26302276435299987, 182.7404713219719667 ) ) ;
#40656=VECTOR ( 'NONE', #56336, 1000.000000000000000 ) ;
#40657=CARTESIAN_POINT ( 'NONE',  ( 97.06104777439192333, -37.99628893422420362, 27.42740443400874994 ) ) ;
#40660=ORIENTED_EDGE ( 'NONE', *, *, #31694, .T. ) ;
#40662=DIRECTION ( 'NONE',  ( 0.000000000000000000, 0.000000000000000000, -1.000000000000000000 ) ) ;
#40663=CARTESIAN_POINT ( 'NONE',  ( 136.5411229421876271, -19.94037323191022892, 2.740176903249453844 ) ) ;
#40665=VERTEX_POINT ( 'NONE', #35798 ) ;
#40666=CARTESIAN_POINT ( 'NONE',  ( 194.0371591254582313, -46.82818131005407736, 300.4678068554149490 ) ) ;
#40668=CARTESIAN_POINT ( 'NONE',  ( 112.1317502087781293, -44.64270164792750961, 214.4492023535159717 ) ) ;
#40670=FACE_BOUND ( 'NONE', #25581, .T. ) ;
#40674=CARTESIAN_POINT ( 'NONE',  ( 63.03715912545820999, -46.82818131006018092, 300.4678068554150627 ) ) ;
#40676=ORIENTED_EDGE ( 'NONE', *, *, #38192, .T. ) ;
#40678=CARTESIAN_POINT ( 'NONE',  ( 101.1728908740289512, -31.04189437634028437, 248.5338046553059428 ) ) ;
#40679=CARTESIAN_POINT ( 'NONE',  ( 108.6520877210037952, -25.77347123183324484, 149.9737205140059473 ) ) ;
#40680=AXIS2_PLACEMENT_3D ( 'NONE', #57935, #10237, #37941 ) ;
#40681=CARTESIAN_POINT ( 'NONE',  ( 117.3319688044107920, -38.62265419183311366, 88.68133956162493803 ) ) ;
#40682=CARTESIAN_POINT ( 'NONE',  ( 105.9148582384516999, -44.85806553849772627, 249.5838068554170945 ) ) ;
#40684=DIRECTION ( 'NONE',  ( 0.000000000000000000, 0.000000000000000000, -1.000000000000000000 ) ) ;
#40685=DIRECTION ( 'NONE',  ( 0.000000000000000000, 0.000000000000000000, -1.000000000000000000 ) ) ;
#40686=CARTESIAN_POINT ( 'NONE',  ( 96.64436219916188975, -36.48069147925158262, 192.3070538473399438 ) ) ;
#40687=CARTESIAN_POINT ( 'NONE',  ( 41.56670390244718050, -42.82844715994109208, 180.4678068554150911 ) ) ;
#40688=ORIENTED_EDGE ( 'NONE', *, *, #30314, .T. ) ;
#40689=CARTESIAN_POINT ( 'NONE',  ( 138.8167039024479834, -67.87844715994100397, 86.31780685541500020 ) ) ;
#40692=LINE ( 'NONE', #12100, #66218 ) ;
#40693=VECTOR ( 'NONE', #77881, 1000.000000000000000 ) ;
#40695=CARTESIAN_POINT ( 'NONE',  ( 36.65249034007450746, -49.32844715994130524, 129.9678068554150911 ) ) ;
#40696=CARTESIAN_POINT ( 'NONE',  ( 117.3640430381357334, -38.35649778030718693, 113.7013395616249767 ) ) ;
#40698=CARTESIAN_POINT ( 'NONE',  ( 136.5970563715325170, -35.65296049054685312, 7.043700149390024201 ) ) ;
#40699=CARTESIAN_POINT ( 'NONE',  ( 41.56648329127399677, 0.2215528400590013880, 318.9256252759120116 ) ) ;
#40700=CARTESIAN_POINT ( 'NONE',  ( 188.5667039024484097, -48.82844715993431350, 257.2178068554150059 ) ) ;
#40702=CARTESIAN_POINT ( 'NONE',  ( 98.55548742614595881, -30.74683778668247669, 201.8384824187679385 ) ) ;
#40703=DIRECTION ( 'NONE',  ( -0.000000000000000000, 1.000000000000000000, 0.000000000000000000 ) ) ;
#40704=CARTESIAN_POINT ( 'NONE',  ( 116.3215253324775773, -32.93968801256757217, 155.1356252759109680 ) ) ;
#40705=EDGE_LOOP ( 'NONE', ( #45251, #68832, #796, #52900 ) ) ;
#40708=DIRECTION ( 'NONE',  ( 2.900000000000000265E-14, -2.000000000000000155E-15, 1.000000000000000000 ) ) ;
#40709=AXIS2_PLACEMENT_3D ( 'NONE', #51772, #79523, #15947 ) ;
#40711=CARTESIAN_POINT ( 'NONE',  ( 106.9399074540173871, -47.82885535071048366, 232.5794347997199907 ) ) ;
#40713=CARTESIAN_POINT ( 'NONE',  ( 115.6649034994425307, -31.56786279214498947, 194.2562958305554162 ) ) ;
#40714=CARTESIAN_POINT ( 'NONE',  ( 111.1289525437170056, -47.00905435842401658, 18.88800622829195319 ) ) ;
#40715=CARTESIAN_POINT ( 'NONE',  ( 116.7009037750506053, -40.82467873942847802, 164.5070538473399608 ) ) ;
#40716=CARTESIAN_POINT ( 'NONE',  ( 112.1393455939420249, -28.01282275174989422, 30.65645861365223723 ) ) ;
#40717=LINE ( 'NONE', #76137, #48913 ) ;
#40718=LINE ( 'NONE', #19391, #82636 ) ;
#40720=CARTESIAN_POINT ( 'NONE',  ( 109.7248659574642318, -27.00080519035325111, 189.8647919396041459 ) ) ;
#40724=VERTEX_POINT ( 'NONE', #78065 ) ;
#40725=ORIENTED_EDGE ( 'NONE', *, *, #58740, .T. ) ;
#40726=CIRCLE ( 'NONE', #52298, 15.69999999999999041 ) ;
#40727=EDGE_LOOP ( 'NONE', ( #57203, #12628, #70593, #2832 ) ) ;
#40728=DIRECTION ( 'NONE',  ( 0.000000000000000000, 1.000000000000000000, 0.000000000000000000 ) ) ;
#40729=CARTESIAN_POINT ( 'NONE',  ( 112.1705331031350283, -27.62378402076942763, 30.66991099019694644 ) ) ;
#40730=DIRECTION ( 'NONE',  ( 0.000000000000000000, 0.000000000000000000, -1.000000000000000000 ) ) ;
#40731=DIRECTION ( 'NONE',  ( 3.999999999999999995E-14, -1.000000000000000000, 4.100000000000000342E-29 ) ) ;
#40733=CARTESIAN_POINT ( 'NONE',  ( 98.55846751192062527, -35.97459669770627499, 230.6781341137909465 ) ) ;
#40735=ORIENTED_EDGE ( 'NONE', *, *, #71436, .F. ) ;
#40736=ORIENTED_EDGE ( 'NONE', *, *, #85310, .T. ) ;
#40737=EDGE_CURVE ( 'NONE', #72283, #86684, #35805, .T. ) ;
#40738=FACE_OUTER_BOUND ( 'NONE', #56783, .T. ) ;
#40739=CARTESIAN_POINT ( 'NONE',  ( 114.5914593468340712, -43.34783535320182324, 183.2524815427824763 ) ) ;
#40741=DIRECTION ( 'NONE',  ( 0.000000000000000000, 0.000000000000000000, -1.000000000000000000 ) ) ;
#40742=AXIS2_PLACEMENT_3D ( 'NONE', #22829, #77788, #77331 ) ;
#40743=DIRECTION ( 'NONE',  ( -4.237773401492740281E-14, 1.000000000000000000, 0.000000000000000000 ) ) ;
#40747=CARTESIAN_POINT ( 'NONE',  ( 115.4101910119110386, -30.57141770992054219, 259.3203871806734355 ) ) ;
#40751=ORIENTED_EDGE ( 'NONE', *, *, #55906, .F. ) ;
#40752=EDGE_CURVE ( 'NONE', #48213, #28502, #55224, .T. ) ;
#40753=CARTESIAN_POINT ( 'NONE',  ( 34.33598329127499227, -36.32844715994100682, -5.074374724088000832 ) ) ;
#40754=VECTOR ( 'NONE', #44218, 1000.000000000000000 ) ;
#40756=CARTESIAN_POINT ( 'NONE',  ( 112.7718126367562093, -42.56716444297848767, 71.01094751244896486 ) ) ;
#40759=PLANE ( 'NONE',  #30538 ) ;
#40761=FACE_OUTER_BOUND ( 'NONE', #11826, .T. ) ;
#40762=CARTESIAN_POINT ( 'NONE',  ( 100.9546728091797974, -28.70702572886692039, 45.59395860945408430 ) ) ;
#40763=ORIENTED_EDGE ( 'NONE', *, *, #28672, .F. ) ;
#40764=CARTESIAN_POINT ( 'NONE',  ( 79.87807227644366037, -33.97944715994105991, 8.225625275910942946 ) ) ;
#40766=CARTESIAN_POINT ( 'NONE',  ( 108.9452245070828411, -26.43885738637160543, 164.9327681330529742 ) ) ;
#40768=EDGE_CURVE ( 'NONE', #53177, #64680, #82493, .T. ) ;
#40770=CARTESIAN_POINT ( 'NONE',  ( 97.98128717666138243, -40.91104618832473250, 87.66925762342037842 ) ) ;
#40771=CARTESIAN_POINT ( 'NONE',  ( 99.53176374547611260, -42.34233651421938305, 108.2796785439919773 ) ) ;
#40774=CARTESIAN_POINT ( 'NONE',  ( 107.8700274897790479, -26.31351822515222949, 66.01562527591097762 ) ) ;
#40775=VECTOR ( 'NONE', #34003, 1000.000000000000000 ) ;
#40776=CARTESIAN_POINT ( 'NONE',  ( 109.6428311413115750, -46.48013238632621125, 257.7813333649102105 ) ) ;
#40777=VERTEX_POINT ( 'NONE', #13034 ) ;
#40782=EDGE_CURVE ( 'NONE', #10976, #79006, #40717, .T. ) ;
#40783=DIRECTION ( 'NONE',  ( 0.000000000000000000, 0.000000000000000000, -1.000000000000000000 ) ) ;
#40784=VERTEX_POINT ( 'NONE', #289 ) ;
#40785=CARTESIAN_POINT ( 'NONE',  ( 116.8470136369842720, -36.79772195930841150, 263.8213395616257912 ) ) ;
#40786=CARTESIAN_POINT ( 'NONE',  ( 112.1306244020896941, -47.47080300746646486, 133.9270538473399768 ) ) ;
#40787=ADVANCED_FACE ( 'NONE', ( #33906 ), #61600, .F. ) ;
#40789=CARTESIAN_POINT ( 'NONE',  ( 98.34985891780978307, -31.65658480061700430, 141.9064586084259645 ) ) ;
#40790=CARTESIAN_POINT ( 'NONE',  ( 98.33631928459364246, -42.42740502779041378, 97.78705384733993355 ) ) ;
#40791=VECTOR ( 'NONE', #31653, 1000.000000000000000 ) ;
#40792=CARTESIAN_POINT ( 'NONE',  ( 41.56648329127399677, -18.82844715994099971, 316.8086252759120498 ) ) ;
#40795=DIRECTION ( 'NONE',  ( -0.7071067811865758834, 0.7071067811865192621, -2.899137802864845566E-29 ) ) ;
#40797=CARTESIAN_POINT ( 'NONE',  ( 107.0664832912739399, -36.72944715994095333, 357.5272416190308604 ) ) ;
#40798=EDGE_LOOP ( 'NONE', ( #57995, #77158, #11125, #63469 ) ) ;
#40799=LINE ( 'NONE', #88075, #44559 ) ;
#40801=CARTESIAN_POINT ( 'NONE',  ( 113.7419942178973287, -29.10023054337252546, 289.5032443235301116 ) ) ;
#40803=CARTESIAN_POINT ( 'NONE',  ( 80.06648329127399677, 0.2215528400590013880, 308.6356252759119911 ) ) ;
#40804=CARTESIAN_POINT ( 'NONE',  ( 45.76696975232907505, -48.62818131005967359, 249.9678068554150343 ) ) ;
#40805=CARTESIAN_POINT ( 'NONE',  ( 105.2812310726300922, -46.37359664056156561, 12.42991099019696932 ) ) ;
#40806=CARTESIAN_POINT ( 'NONE',  ( 115.6667067228004129, -31.57200485274490376, 99.25677482824653453 ) ) ;
#40807=CARTESIAN_POINT ( 'NONE',  ( 116.5783909117431136, -29.70293872869714846, 105.3327681330539463 ) ) ;
#40809=CARTESIAN_POINT ( 'NONE',  ( 98.24359417337518607, -31.02780217081950909, 145.8699109901969848 ) ) ;
#40811=ORIENTED_EDGE ( 'NONE', *, *, #28361, .F. ) ;
#40814=CARTESIAN_POINT ( 'NONE',  ( 82.81648329127402519, -36.72944715994107412, -5.074374724089055100 ) ) ;
#40816=ORIENTED_EDGE ( 'NONE', *, *, #30250, .F. ) ;
#40817=DIRECTION ( 'NONE',  ( 1.639958061481212836E-42, -4.100000000000000342E-29, -1.000000000000000000 ) ) ;
#40818=CARTESIAN_POINT ( 'NONE',  ( 102.2925893952339749, -26.70832846991215703, 140.4422919425769578 ) ) ;
#40819=ORIENTED_EDGE ( 'NONE', *, *, #32422, .F. ) ;
#40820=LINE ( 'NONE', #82188, #4481 ) ;
#40822=CIRCLE ( 'NONE', #39459, 2.116999999999993776 ) ;
#40824=CARTESIAN_POINT ( 'NONE',  ( 32.06670390244800473, -32.29483332968611364, -5.074374724088000832 ) ) ;
#40826=VERTEX_POINT ( 'NONE', #6655 ) ;
#40829=CARTESIAN_POINT ( 'NONE',  ( 19.56648329127400032, 0.2215528400590013880, -5.074374724088000832 ) ) ;
#40831=CARTESIAN_POINT ( 'NONE',  ( 117.0718954874996172, -35.46248236767254980, 158.9272919416701200 ) ) ;
#40832=CARTESIAN_POINT ( 'NONE',  ( 72.25757238336808541, -1.944390235229867425, 361.9756252759101471 ) ) ;
#40837=ORIENTED_EDGE ( 'NONE', *, *, #84078, .T. ) ;
#40838=ORIENTED_EDGE ( 'NONE', *, *, #10212, .F. ) ;
#40839=DIRECTION ( 'NONE',  ( 0.000000000000000000, 0.000000000000000000, -1.000000000000000000 ) ) ;
#40840=CARTESIAN_POINT ( 'NONE',  ( 107.0664832912739399, -36.72944715994095333, 315.6356252759111953 ) ) ;
#40841=EDGE_CURVE ( 'NONE', #58498, #64389, #31562, .T. ) ;
#40842=CARTESIAN_POINT ( 'NONE',  ( 97.17009264939177626, -31.66255117090388538, 241.9499109901959741 ) ) ;
#40845=EDGE_CURVE ( 'NONE', #78707, #14442, #86689, .T. ) ;
#40846=CARTESIAN_POINT ( 'NONE',  ( 99.96923091713372855, -43.45941328387849723, 77.92991099019597812 ) ) ;
#40847=CARTESIAN_POINT ( 'NONE',  ( 113.2129946629323882, -44.63276428892469028, 53.10250874954972033 ) ) ;
#40848=AXIS2_PLACEMENT_3D ( 'NONE', #81177, #53857, #76123 ) ;
#40849=CARTESIAN_POINT ( 'NONE',  ( 103.9512555245577659, -27.22114335906981708, 21.32843223802335331 ) ) ;
#40850=ADVANCED_FACE ( 'NONE', ( #57029 ), #64317, .F. ) ;
#40851=ORIENTED_EDGE ( 'NONE', *, *, #43316, .T. ) ;
#40853=EDGE_CURVE ( 'NONE', #52054, #16163, #29791, .T. ) ;
#40854=VERTEX_POINT ( 'NONE', #8917 ) ;
#40855=ORIENTED_EDGE ( 'NONE', *, *, #29915, .F. ) ;
#40856=DIRECTION ( 'NONE',  ( 0.000000000000000000, 1.000000000000000000, 0.000000000000000000 ) ) ;
#40857=CARTESIAN_POINT ( 'NONE',  ( 100.5340721669357009, -30.74146890971161739, 272.1672975916113160 ) ) ;
#40858=EDGE_CURVE ( 'NONE', #78957, #46739, #85230, .T. ) ;
#40860=FACE_OUTER_BOUND ( 'NONE', #15648, .T. ) ;
#40861=ADVANCED_FACE ( 'NONE', ( #50214 ), #49318, .F. ) ;
#40863=CARTESIAN_POINT ( 'NONE',  ( 81.24991378862220870, -39.21189172704054471, 1.845048092478625001 ) ) ;
#40864=AXIS2_PLACEMENT_3D ( 'NONE', #48863, #1195, #64756 ) ;
#40865=ORIENTED_EDGE ( 'NONE', *, *, #56626, .T. ) ;
#40867=CARTESIAN_POINT ( 'NONE',  ( 34.96670390244745619, -26.71338133339230581, 237.4678068554150059 ) ) ;
#40868=ORIENTED_EDGE ( 'NONE', *, *, #74317, .F. ) ;
#40869=CARTESIAN_POINT ( 'NONE',  ( 110.7945467183388502, -46.46538951521414873, 62.86705384733992474 ) ) ;
#40871=CARTESIAN_POINT ( 'NONE',  ( 115.2284764178246661, -36.04786338006340429, 251.7109475124485414 ) ) ;
#40872=EDGE_CURVE ( 'NONE', #18180, #25402, #15720, .T. ) ;
#40873=FACE_BOUND ( 'NONE', #10765, .T. ) ;
#40874=CARTESIAN_POINT ( 'NONE',  ( 101.2684584845351736, -45.32493232151070828, 152.0918157521019509 ) ) ;
#40876=LINE ( 'NONE', #12295, #51956 ) ;
#40877=CARTESIAN_POINT ( 'NONE',  ( 80.06648329127399677, -8.350947159940998787, 311.1531252759119752 ) ) ;
#40878=VECTOR ( 'NONE', #4867, 1000.000000000000000 ) ;
#40879=DIRECTION ( 'NONE',  ( 1.000000000000000078E-15, 1.000000000000000083E-30, -1.000000000000000000 ) ) ;
#40881=CARTESIAN_POINT ( 'NONE',  ( 101.6280127420326522, -45.67461444920139257, 243.1413395616249886 ) ) ;
#40884=CIRCLE ( 'NONE', #48133, 4.874999999999990230 ) ;
#40885=CARTESIAN_POINT ( 'NONE',  ( 113.3408031569382644, -28.30502284670691182, 100.5670538473389684 ) ) ;
#40886=LINE ( 'NONE', #49485, #23670 ) ;
#40887=EDGE_LOOP ( 'NONE', ( #80566, #10107 ) ) ;
#40888=VERTEX_POINT ( 'NONE', #36616 ) ;
#40891=CARTESIAN_POINT ( 'NONE',  ( 33.78129701732998313, -35.65087443492610930, -5.074374724088000832 ) ) ;
#40892=CARTESIAN_POINT ( 'NONE',  ( 80.06648329127399677, 0.2215528400590013880, 291.1181252759119502 ) ) ;
#40893=CARTESIAN_POINT ( 'NONE',  ( 63.03715912545729338, -24.42818131006027826, 313.9678068554150059 ) ) ;
#40894=CARTESIAN_POINT ( 'NONE',  ( 103.1394548971403680, -44.44173430692483606, 170.0318998934009755 ) ) ;
#40895=CARTESIAN_POINT ( 'NONE',  ( 106.8359569501641744, -47.17378133968975362, 268.5584824187679374 ) ) ;
#40897=CARTESIAN_POINT ( 'NONE',  ( 99.08953455931535359, -42.79546436554615241, 57.84391660217934827 ) ) ;
#40898=ADVANCED_FACE ( 'NONE', ( #1192 ), #44286, .T. ) ;
#40901=EDGE_CURVE ( 'NONE', #25043, #43140, #12710, .T. ) ;
#40902=CYLINDRICAL_SURFACE ( 'NONE', #85340, 10.00000000000002665 ) ;
#40903=ORIENTED_EDGE ( 'NONE', *, *, #87419, .T. ) ;
#40904=CIRCLE ( 'NONE', #22075, 3.299999999999997158 ) ;
#40906=VECTOR ( 'NONE', #33538, 1000.000000000000000 ) ;
#40909=ORIENTED_EDGE ( 'NONE', *, *, #46420, .F. ) ;
#40912=DIRECTION ( 'NONE',  ( 1.000000000000000078E-15, 0.000000000000000000, 1.000000000000000000 ) ) ;
#40913=DIRECTION ( 'NONE',  ( 0.000000000000000000, 0.000000000000000000, 1.000000000000000000 ) ) ;
#40914=CARTESIAN_POINT ( 'NONE',  ( 115.9692459539148643, -35.07008363779494431, 203.4076579233149573 ) ) ;
#40916=CARTESIAN_POINT ( 'NONE',  ( 118.0351107906133876, -38.43300062509310067, 68.69181575210198787 ) ) ;
#40917=LINE ( 'NONE', #5976, #72764 ) ;
#40918=ORIENTED_EDGE ( 'NONE', *, *, #33860, .T. ) ;
#40919=DIRECTION ( 'NONE',  ( 1.000000000000000000, -6.745093096447288888E-17, -4.496403249731880833E-15 ) ) ;
#40920=VECTOR ( 'NONE', #53303, 1000.000000000000000 ) ;
#40922=LINE ( 'NONE', #47729, #78064 ) ;
#40923=ORIENTED_EDGE ( 'NONE', *, *, #40555, .T. ) ;
#40926=CARTESIAN_POINT ( 'NONE',  ( 182.2300522401149863, -33.89581943344511217, -5.074374724088000832 ) ) ;
#40927=ADVANCED_FACE ( 'NONE', ( #42498 ), #71138, .F. ) ;
#40928=DIRECTION ( 'NONE',  ( 0.000000000000000000, 1.000000000000000000, 0.000000000000000000 ) ) ;
#40929=ORIENTED_EDGE ( 'NONE', *, *, #32043, .T. ) ;
#40930=CARTESIAN_POINT ( 'NONE',  ( 106.9270552135175620, -26.24760940922973163, 60.08705384733897858 ) ) ;
#40932=CARTESIAN_POINT ( 'NONE',  ( 160.7738106836348209, -48.62134037874901082, 300.4678068554149490 ) ) ;
#40935=CARTESIAN_POINT ( 'NONE',  ( 41.56648329127399677, -18.82844715994099971, 18.92562527591200094 ) ) ;
#40936=ORIENTED_EDGE ( 'NONE', *, *, #27978, .F. ) ;
#40937=CIRCLE ( 'NONE', #54007, 2.117000000000007987 ) ;
#40941=EDGE_LOOP ( 'NONE', ( #62575, #78316, #44196, #34592, #5090 ) ) ;
#40942=CARTESIAN_POINT ( 'NONE',  ( 103.8345913547307333, -46.70111052772084292, 78.32705384733995402 ) ) ;
#40943=CIRCLE ( 'NONE', #88824, 0.5000000000000004441 ) ;
#40944=PLANE ( 'NONE',  #1502 ) ;
#40945=DIRECTION ( 'NONE',  ( 0.000000000000000000, 0.000000000000000000, -1.000000000000000000 ) ) ;
#40948=CIRCLE ( 'NONE', #33700, 2.029999999999997140 ) ;
#40949=EDGE_CURVE ( 'NONE', #11998, #36895, #56119, .T. ) ;
#40951=ORIENTED_EDGE ( 'NONE', *, *, #56137, .T. ) ;
#40952=EDGE_CURVE ( 'NONE', #60508, #54515, #84329, .T. ) ;
#40953=CARTESIAN_POINT ( 'NONE',  ( 108.4956486572523602, -46.43878675094416764, 138.6927681330529936 ) ) ;
#40954=CARTESIAN_POINT ( 'NONE',  ( 34.96670390244699433, -26.71338133339301635, -5.074374724088000832 ) ) ;
#40956=EDGE_CURVE ( 'NONE', #52594, #51252, #49764, .T. ) ;
#40957=CARTESIAN_POINT ( 'NONE',  ( 118.6297112294782892, -39.20734283244433982, 254.6584824187681022 ) ) ;
#40961=CARTESIAN_POINT ( 'NONE',  ( 115.0889047229540836, -30.61763667849448822, 45.34395860938102629 ) ) ;
#40964=EDGE_CURVE ( 'NONE', #72082, #47060, #57932, .T. ) ;
#40966=CARTESIAN_POINT ( 'NONE',  ( 98.33750497493203113, -41.21483588869663350, 196.7041967044829676 ) ) ;
#40967=ORIENTED_EDGE ( 'NONE', *, *, #89737, .T. ) ;
#40968=ORIENTED_EDGE ( 'NONE', *, *, #2900, .T. ) ;
#40969=CARTESIAN_POINT ( 'NONE',  ( 109.1422557193553047, -45.34451810791325954, 129.1958690201829825 ) ) ;
#40970=EDGE_CURVE ( 'NONE', #41295, #79108, #19969, .T. ) ;
#40973=CARTESIAN_POINT ( 'NONE',  ( 101.5279499456468528, -29.13990343739101974, 26.99777378208800727 ) ) ;
#40974=DIRECTION ( 'NONE',  ( 0.000000000000000000, 1.000000000000000000, 0.000000000000000000 ) ) ;
#40975=DIRECTION ( 'NONE',  ( 1.000000000000000000, -1.025452301070031786E-14, 0.000000000000000000 ) ) ;
#40976=EDGE_CURVE ( 'NONE', #46082, #61174, #78407, .T. ) ;
#40978=DIRECTION ( 'NONE',  ( 1.000000000000000000, 0.000000000000000000, 0.000000000000000000 ) ) ;
#40980=DIRECTION ( 'NONE',  ( 1.000000000000000000, 2.999999999999999839E-15, 1.000000000000000078E-15 ) ) ;
#40981=CARTESIAN_POINT ( 'NONE',  ( 107.0664832912739968, -36.72944715994100306, 287.6356252759109680 ) ) ;
#40982=CARTESIAN_POINT ( 'NONE',  ( 117.4525030917818782, -36.13006561810994555, 228.8727681330539667 ) ) ;
#40983=DIRECTION ( 'NONE',  ( 0.000000000000000000, -1.000000000000000000, 0.000000000000000000 ) ) ;
#40985=EDGE_LOOP ( 'NONE', ( #28935, #11874, #66712, #43571 ) ) ;
#40986=EDGE_CURVE ( 'NONE', #60225, #85887, #23875, .T. ) ;
#40988=CARTESIAN_POINT ( 'NONE',  ( 80.06648281188262217, -21.47944715903999224, 8.225259175037979986 ) ) ;
#40989=CARTESIAN_POINT ( 'NONE',  ( 105.8001629020714489, -26.72394735792939713, 185.1776961641718913 ) ) ;
#40990=FACE_OUTER_BOUND ( 'NONE', #55327, .T. ) ;
#40991=CYLINDRICAL_SURFACE ( 'NONE', #81863, 7.499999999999996447 ) ;
#40994=CARTESIAN_POINT ( 'NONE',  ( 117.7765707488592710, -31.65652763686493998, 214.1784824187679419 ) ) ;
#40996=CIRCLE ( 'NONE', #1865, 5.599999999999994316 ) ;
#40997=DIRECTION ( 'NONE',  ( -1.000000000000000078E-15, 0.000000000000000000, 1.000000000000000000 ) ) ;
#40998=CARTESIAN_POINT ( 'NONE',  ( 34.67381068362099228, -26.00627455219321860, -5.074374724088000832 ) ) ;
#40999=CARTESIAN_POINT ( 'NONE',  ( 111.0302909011776507, -45.91071616320562043, 167.9007897230142987 ) ) ;
#41000=CARTESIAN_POINT ( 'NONE',  ( 112.0721450080970669, -44.54221119967598241, 65.84809036959194373 ) ) ;
#41001=CARTESIAN_POINT ( 'NONE',  ( 118.9423443782970082, -36.92851767163586629, 149.8127681330539644 ) ) ;
#41003=VERTEX_POINT ( 'NONE', #53316 ) ;
#41004=EDGE_CURVE ( 'NONE', #26689, #63598, #18374, .T. ) ;
#41006=CARTESIAN_POINT ( 'NONE',  ( 98.13538023319908632, -41.23056087969936101, 66.69855942027353990 ) ) ;
#41007=ORIENTED_EDGE ( 'NONE', *, *, #40010, .T. ) ;
#41008=EDGE_LOOP ( 'NONE', ( #47788, #17536, #11487, #39449 ) ) ;
#41010=DIRECTION ( 'NONE',  ( 1.000000000000000000, 0.000000000000000000, 0.000000000000000000 ) ) ;
#41013=CARTESIAN_POINT ( 'NONE',  ( 162.5667039024460223, -22.48495420874110806, 342.9256252759109884 ) ) ;
#41014=CARTESIAN_POINT ( 'NONE',  ( 109.7746843348460857, -45.37110888865593239, 52.22861030426695095 ) ) ;
#41015=CARTESIAN_POINT ( 'NONE',  ( 104.4049122349322545, -25.97716923158638735, 240.2575300378159682 ) ) ;
#41016=CARTESIAN_POINT ( 'NONE',  ( 109.3321198358312074, -26.57584895156206173, 224.9013395616249511 ) ) ;
#41017=CARTESIAN_POINT ( 'NONE',  ( 90.44969454456405344, -20.11243780205715481, 229.5838068554169809 ) ) ;
#41018=CARTESIAN_POINT ( 'NONE',  ( 116.1393041698827346, -43.00708073170991952, 9.356577656862985037 ) ) ;
#41019=DIRECTION ( 'NONE',  ( -0.9254794337955623007, -0.3787978585227819162, 0.000000000000000000 ) ) ;
#41021=DIRECTION ( 'NONE',  ( 1.000000000000000000, 0.000000000000000000, 0.000000000000000000 ) ) ;
#41022=EDGE_CURVE ( 'NONE', #15321, #10458, #87432, .T. ) ;
#41024=ORIENTED_EDGE ( 'NONE', *, *, #65658, .T. ) ;
#41025=CARTESIAN_POINT ( 'NONE',  ( 101.4370486012140020, -28.02035706366309853, 70.54514908543596619 ) ) ;
#41027=EDGE_CURVE ( 'NONE', #59691, #23038, #63465, .T. ) ;
#41028=CARTESIAN_POINT ( 'NONE',  ( 113.5334051825838202, -28.49624685289517245, 79.54705384733995288 ) ) ;
#41029=CARTESIAN_POINT ( 'NONE',  ( 115.6917119993852054, -30.73301325301421016, 279.3099109901964994 ) ) ;
#41030=VERTEX_POINT ( 'NONE', #86991 ) ;
#41031=CARTESIAN_POINT ( 'NONE',  ( 100.8231516252168234, -45.85084492350206631, 242.1108633711489517 ) ) ;
#41032=DIRECTION ( 'NONE',  ( -1.000000000000000000, 0.000000000000000000, 0.000000000000000000 ) ) ;
#41035=CARTESIAN_POINT ( 'NONE',  ( 21.03715912545824551, -47.82818131006186491, 300.4678068554150059 ) ) ;
#41037=CARTESIAN_POINT ( 'NONE',  ( 98.24075285659111501, -36.10665116910172401, 277.6356252759110816 ) ) ;
#41038=CARTESIAN_POINT ( 'NONE',  ( 120.0664832912739399, -36.72944715994095333, 294.6356252759106837 ) ) ;
#41039=CARTESIAN_POINT ( 'NONE',  ( 97.82711386317197366, -40.55490885176772764, 172.6388511831666506 ) ) ;
#41041=VECTOR ( 'NONE', #32169, 1000.000000000000000 ) ;
#41043=CARTESIAN_POINT ( 'NONE',  ( 97.81168895331838087, -40.51742574516882200, 287.6356252759109680 ) ) ;
#41044=CARTESIAN_POINT ( 'NONE',  ( 172.5664832912728457, -27.82844715994070484, 21.92562527591199739 ) ) ;
#41045=FACE_OUTER_BOUND ( 'NONE', #30173, .T. ) ;
#41049=CARTESIAN_POINT ( 'NONE',  ( 110.0583800183467957, -26.06436417334086642, 219.8708633711489711 ) ) ;
#41050=CARTESIAN_POINT ( 'NONE',  ( 117.1259760753171548, -33.86829196857838298, 145.0470538473399529 ) ) ;
#41051=CARTESIAN_POINT ( 'NONE',  ( 105.1008636489907673, -25.80544433381534475, 271.2061014663873380 ) ) ;
#41052=FACE_OUTER_BOUND ( 'NONE', #18506, .T. ) ;
#41053=DIRECTION ( 'NONE',  ( -1.000000000000000078E-15, 1.000000000000000083E-30, 1.000000000000000000 ) ) ;
#41054=CARTESIAN_POINT ( 'NONE',  ( 162.5667039024470171, -33.35206098992711077, -5.074374724088000832 ) ) ;
#41055=CYLINDRICAL_SURFACE ( 'NONE', #87126, 15.99999999999999822 ) ;
#41059=EDGE_LOOP ( 'NONE', ( #35650, #43789, #81980, #31784 ) ) ;
#41060=ADVANCED_FACE ( 'NONE', ( #51982 ), #57627, .F. ) ;
#41061=CARTESIAN_POINT ( 'NONE',  ( 103.1716831446340166, -28.55367798840643090, 139.8648007804579549 ) ) ;
#41063=EDGE_LOOP ( 'NONE', ( #38381, #79527 ) ) ;
#41064=AXIS2_PLACEMENT_3D ( 'NONE', #50007, #15962, #71380 ) ;
#41065=LINE ( 'NONE', #87891, #17012 ) ;
#41067=CARTESIAN_POINT ( 'NONE',  ( 96.03721982003250446, -36.58408020053186505, 152.3280062282919971 ) ) ;
#41068=CARTESIAN_POINT ( 'NONE',  ( 116.7940342761296932, -39.39171570160217328, 149.6152268520635857 ) ) ;
#41069=EDGE_CURVE ( 'NONE', #55351, #24376, #53249, .T. ) ;
#41070=PLANE ( 'NONE',  #38533 ) ;
#41072=EDGE_CURVE ( 'NONE', #1305, #36080, #58375, .T. ) ;
#41074=CARTESIAN_POINT ( 'NONE',  ( 107.8912859324307334, -26.39220933555693094, 115.0251490854349612 ) ) ;
#41077=ORIENTED_EDGE ( 'NONE', *, *, #87574, .T. ) ;
#41079=CARTESIAN_POINT ( 'NONE',  ( 150.5667039024485234, -47.82844715993594065, 180.4678068554149775 ) ) ;
#41080=CARTESIAN_POINT ( 'NONE',  ( 108.8290724220007206, -27.07506712556666173, 160.9327681330529742 ) ) ;
#41082=CARTESIAN_POINT ( 'NONE',  ( 113.2462102393686081, -28.75921903332401541, 54.55156195206926384 ) ) ;
#41085=CYLINDRICAL_SURFACE ( 'NONE', #79417, 9.999999999999998224 ) ;
#41088=CARTESIAN_POINT ( 'NONE',  ( 109.6783822832554449, -47.44587409406599932, 87.75467289495897205 ) ) ;
#41089=ORIENTED_EDGE ( 'NONE', *, *, #24666, .T. ) ;
#41091=VERTEX_POINT ( 'NONE', #52419 ) ;
#41092=LINE ( 'NONE', #19320, #2368 ) ;
#41095=CARTESIAN_POINT ( 'NONE',  ( 105.0207293620135118, -28.82725652202227096, 198.0966617981629554 ) ) ;
#41100=ORIENTED_EDGE ( 'NONE', *, *, #4259, .F. ) ;
#41101=EDGE_LOOP ( 'NONE', ( #8172, #21756, #41162, #67743 ) ) ;
#41102=CARTESIAN_POINT ( 'NONE',  ( 46.48091746482126041, -48.32844715994084339, 300.4678068554150059 ) ) ;
#41103=DIRECTION ( 'NONE',  ( -0.000000000000000000, 1.000000000000000000, 0.000000000000000000 ) ) ;
#41105=ORIENTED_EDGE ( 'NONE', *, *, #58108, .T. ) ;
#41106=DIRECTION ( 'NONE',  ( 0.000000000000000000, 0.000000000000000000, -1.000000000000000000 ) ) ;
#41107=CARTESIAN_POINT ( 'NONE',  ( 115.1751221500829701, -40.30411560180680652, 249.9272975916113637 ) ) ;
#41110=DIRECTION ( 'NONE',  ( -0.000000000000000000, 1.000000000000000000, 0.000000000000000000 ) ) ;
#41112=ORIENTED_EDGE ( 'NONE', *, *, #21911, .T. ) ;
#41114=DIRECTION ( 'NONE',  ( 1.000000000000000078E-15, 1.000000000000000083E-30, -1.000000000000000000 ) ) ;
#41115=VECTOR ( 'NONE', #21661, 1000.000000000000000 ) ;
#41116=ORIENTED_EDGE ( 'NONE', *, *, #567, .F. ) ;
#41118=EDGE_CURVE ( 'NONE', #76706, #9747, #18833, .T. ) ;
#41119=CARTESIAN_POINT ( 'NONE',  ( 112.3381529121750191, -29.09364788469061480, 237.4138046553059951 ) ) ;
#41121=CARTESIAN_POINT ( 'NONE',  ( 96.00433110544545912, -37.29885927265511469, 121.3794347997209684 ) ) ;
#41122=CARTESIAN_POINT ( 'NONE',  ( 116.5783909117432842, -29.70293872869703833, 109.3327681330539605 ) ) ;
#41123=CARTESIAN_POINT ( 'NONE',  ( 108.1460423962843578, -44.98105793649955331, 249.5838068554170093 ) ) ;
#41124=DIRECTION ( 'NONE',  ( 1.000000000000000078E-15, -1.000000000000000083E-30, -1.000000000000000000 ) ) ;
#41125=CARTESIAN_POINT ( 'NONE',  ( 116.7952044851831488, -40.57305441194377948, 189.5270538473389479 ) ) ;
#41126=CARTESIAN_POINT ( 'NONE',  ( 161.4809174648186172, -49.32844715993547169, 129.9678068554149775 ) ) ;
#41127=ORIENTED_EDGE ( 'NONE', *, *, #2460, .T. ) ;
#41130=ORIENTED_EDGE ( 'NONE', *, *, #18534, .F. ) ;
#41131=CARTESIAN_POINT ( 'NONE',  ( 107.0664832912739968, -36.72944715994100306, 287.6356252759109680 ) ) ;
#41132=EDGE_LOOP ( 'NONE', ( #45148, #80967 ) ) ;
#41133=AXIS2_PLACEMENT_3D ( 'NONE', #54827, #82593, #20350 ) ;
#41136=CARTESIAN_POINT ( 'NONE',  ( 98.09668637883959263, -31.41627731406707724, 85.90133956162493689 ) ) ;
#41139=DIRECTION ( 'NONE',  ( 1.000000000000000078E-15, 0.000000000000000000, -1.000000000000000000 ) ) ;
#41142=CARTESIAN_POINT ( 'NONE',  ( 114.5897159479185490, -29.54407062678539830, 230.4327681330539690 ) ) ;
#41143=DIRECTION ( 'NONE',  ( -0.7071067811865758834, 0.7071067811865192621, -7.071067811865765240E-16 ) ) ;
#41145=ORIENTED_EDGE ( 'NONE', *, *, #43798, .F. ) ;
#41149=LINE ( 'NONE', #33453, #81107 ) ;
#41150=CARTESIAN_POINT ( 'NONE',  ( 111.1446672340677111, -27.08708843538706645, 244.7584824187679544 ) ) ;
#41151=ORIENTED_EDGE ( 'NONE', *, *, #20153, .T. ) ;
#41153=CARTESIAN_POINT ( 'NONE',  ( 116.8162545570497741, -32.97600546270004429, 139.1184824187679396 ) ) ;
#41154=CARTESIAN_POINT ( 'NONE',  ( 96.19318211390864803, -38.71572558720041712, 47.48229194257797303 ) ) ;
#41155=CARTESIAN_POINT ( 'NONE',  ( 97.91841856125127208, -30.44371649139010927, 161.8594347997199918 ) ) ;
#41156=CARTESIAN_POINT ( 'NONE',  ( 115.8254323877286822, -31.73001881851844530, 30.23979194345921684 ) ) ;
#41157=CARTESIAN_POINT ( 'NONE',  ( 97.06382073701963975, -37.34192062437319493, 102.3751593848355270 ) ) ;
#41159=DIRECTION ( 'NONE',  ( -0.9254794337955620787, -0.3787978585227822492, 0.000000000000000000 ) ) ;
#41160=CARTESIAN_POINT ( 'NONE',  ( 63.03715912545740707, -46.82818131006016671, 129.9678068554150911 ) ) ;
#41161=DIRECTION ( 'NONE',  ( 0.7071067811865192621, 0.7071067811865758834, 7.071067811865186413E-16 ) ) ;
#41162=ORIENTED_EDGE ( 'NONE', *, *, #63270, .T. ) ;
#41164=VECTOR ( 'NONE', #68521, 1000.000000000000000 ) ;
#41167=EDGE_CURVE ( 'NONE', #16580, #68878, #10233, .T. ) ;
#41168=ORIENTED_EDGE ( 'NONE', *, *, #73481, .T. ) ;
#41170=CARTESIAN_POINT ( 'NONE',  ( 110.5478855402367913, -46.57039549162846015, 33.84705384733993583 ) ) ;
#41171=LINE ( 'NONE', #63886, #38270 ) ;
#41172=ADVANCED_FACE ( 'NONE', ( #3421 ), #52854, .F. ) ;
#41173=CARTESIAN_POINT ( 'NONE',  ( 115.7706392458028262, -41.72622577560414925, 118.4133232042899664 ) ) ;
#41174=CARTESIAN_POINT ( 'NONE',  ( 107.9218213793745633, -47.19875523359718983, 173.6413395616249886 ) ) ;
#41175=EDGE_CURVE ( 'NONE', #43691, #66199, #73339, .T. ) ;
#41176=LINE ( 'NONE', #6232, #88879 ) ;
#41177=CARTESIAN_POINT ( 'NONE',  ( 114.2024335102360908, -32.03537151136463734, 253.7124198280768042 ) ) ;
#41178=ORIENTED_EDGE ( 'NONE', *, *, #64590, .T. ) ;
#41180=ORIENTED_EDGE ( 'NONE', *, *, #43515, .T. ) ;
#41181=VECTOR ( 'NONE', #29494, 1000.000000000000000 ) ;
#41182=DIRECTION ( 'NONE',  ( 0.000000000000000000, 0.000000000000000000, 1.000000000000000000 ) ) ;
#41184=CARTESIAN_POINT ( 'NONE',  ( 117.0609387842264795, -38.08014165370412485, 103.7187873333342623 ) ) ;
#41186=DIRECTION ( 'NONE',  ( 4.299999999999999979E-14, -1.000000000000000000, 4.400000000000000367E-29 ) ) ;
#41187=CARTESIAN_POINT ( 'NONE',  ( 104.4871749466078086, -26.97957198089340025, 275.2812583354421463 ) ) ;
#41190=EDGE_CURVE ( 'NONE', #79915, #34970, #35911, .T. ) ;
#41192=CARTESIAN_POINT ( 'NONE',  ( 97.33767738115261636, -34.07173134274512449, 176.1148459244018909 ) ) ;
#41193=EDGE_CURVE ( 'NONE', #68797, #73231, #27876, .T. ) ;
#41194=CARTESIAN_POINT ( 'NONE',  ( 98.19951187208806687, -40.85743130997450834, 256.6727681330542623 ) ) ;
#41195=DIRECTION ( 'NONE',  ( 0.000000000000000000, 0.000000000000000000, -1.000000000000000000 ) ) ;
#41197=DIRECTION ( 'NONE',  ( 0.000000000000000000, 0.000000000000000000, -1.000000000000000000 ) ) ;
#41198=DIRECTION ( 'NONE',  ( 1.000000000000000078E-15, 0.000000000000000000, 1.000000000000000000 ) ) ;
#41199=CARTESIAN_POINT ( 'NONE',  ( 101.1433531317129280, -42.34605246296819558, 79.74809036959096886 ) ) ;
#41201=FACE_OUTER_BOUND ( 'NONE', #76395, .T. ) ;
#41203=CARTESIAN_POINT ( 'NONE',  ( 78.98444042533645870, -34.20116865955463936, 8.043260881865755607 ) ) ;
#41204=ORIENTED_EDGE ( 'NONE', *, *, #45961, .T. ) ;
#41205=CARTESIAN_POINT ( 'NONE',  ( 116.7957173713512873, -32.98391181527420457, 139.1184824187679396 ) ) ;
#41207=LINE ( 'NONE', #21238, #18487 ) ;
#41208=CARTESIAN_POINT ( 'NONE',  ( 115.1688055144990415, -30.74420868983300537, 105.7644404487539589 ) ) ;
#41211=CARTESIAN_POINT ( 'NONE',  ( 103.5915305487281302, -46.58145011825330783, 53.30705384733997221 ) ) ;
#41212=AXIS2_PLACEMENT_3D ( 'NONE', #84336, #42954, #76604 ) ;
#41213=CARTESIAN_POINT ( 'NONE',  ( 113.1782937600539896, -44.75186860135764988, 84.09395860812267642 ) ) ;
#41215=CYLINDRICAL_SURFACE ( 'NONE', #58449, 3.299999999999997158 ) ;
#41216=CIRCLE ( 'NONE', #25220, 3.250000000000002665 ) ;
#41218=ORIENTED_EDGE ( 'NONE', *, *, #36787, .T. ) ;
#41219=EDGE_CURVE ( 'NONE', #21567, #6566, #54213, .T. ) ;
#41221=VERTEX_POINT ( 'NONE', #61495 ) ;
#41222=CARTESIAN_POINT ( 'NONE',  ( 113.9608400058234849, -28.00707201207230668, 274.5441967044828857 ) ) ;
#41223=CARTESIAN_POINT ( 'NONE',  ( 103.8005819418147411, -26.80618422321597194, 161.3299109901969643 ) ) ;
#41225=CARTESIAN_POINT ( 'NONE',  ( 102.0670549670224858, -27.97049805543147372, 141.4897919419518644 ) ) ;
#41226=CARTESIAN_POINT ( 'NONE',  ( 115.2670960386832775, -44.14051530504124088, 79.25372051400697160 ) ) ;
#41227=CARTESIAN_POINT ( 'NONE',  ( 109.7284190798694539, -27.00174801899234822, 95.86393833725837510 ) ) ;
#41228=ORIENTED_EDGE ( 'NONE', *, *, #45632, .T. ) ;
#41230=CARTESIAN_POINT ( 'NONE',  ( 115.7833820338481559, -41.80184616455515823, 159.4063391417902267 ) ) ;
#41231=ORIENTED_EDGE ( 'NONE', *, *, #60236, .T. ) ;
#41232=DIRECTION ( 'NONE',  ( -1.000000000000000000, -3.999999999999999995E-14, -1.000000000000000078E-15 ) ) ;
#41233=ADVANCED_FACE ( 'NONE', ( #6109 ), #74688, .T. ) ;
#41234=CIRCLE ( 'NONE', #16631, 2.999999999999919176 ) ;
#41235=VECTOR ( 'NONE', #83999, 1000.000000000000000 ) ;
#41236=DIRECTION ( 'NONE',  ( 0.9999999853157766072, 0.0001713722456134502174, -0.000000000000000000 ) ) ;
#41237=CARTESIAN_POINT ( 'NONE',  ( 110.8846227072672121, -27.01418920731891404, 269.7784824187681920 ) ) ;
#41239=DIRECTION ( 'NONE',  ( 4.299999999999999979E-14, -1.000000000000000000, 4.400000000000000367E-29 ) ) ;
#41240=LINE ( 'NONE', #68526, #12216 ) ;
#41241=CARTESIAN_POINT ( 'NONE',  ( 115.8929839771518573, -32.51563103440816604, 19.18133956162593279 ) ) ;
#41242=CARTESIAN_POINT ( 'NONE',  ( 97.15605172367796172, -34.93424641287688104, 101.1850621333696694 ) ) ;
#41243=CARTESIAN_POINT ( 'NONE',  ( 117.5589153096731110, -33.32758106675091625, 130.0880062282919880 ) ) ;
#41244=LINE ( 'NONE', #5865, #75567 ) ;
#41245=CARTESIAN_POINT ( 'NONE',  ( 117.0593108693811786, -33.60693806652478344, 174.0670538473389399 ) ) ;
#41246=DIRECTION ( 'NONE',  ( -1.000000000000000000, -4.299999999999999979E-14, -1.000000000000000078E-15 ) ) ;
#41247=ORIENTED_EDGE ( 'NONE', *, *, #55853, .T. ) ;
#41248=DIRECTION ( 'NONE',  ( -1.000000000000000078E-15, 0.000000000000000000, 1.000000000000000000 ) ) ;
#41250=AXIS2_PLACEMENT_3D ( 'NONE', #55125, #68345, #41508 ) ;
#41251=DIRECTION ( 'NONE',  ( 0.000000000000000000, 0.000000000000000000, -1.000000000000000000 ) ) ;
#41252=DIRECTION ( 'NONE',  ( 0.000000000000000000, 0.000000000000000000, 1.000000000000000000 ) ) ;
#41254=ADVANCED_FACE ( 'NONE', ( #81973 ), #54658, .F. ) ;
#41255=EDGE_CURVE ( 'NONE', #71209, #70634, #68777, .T. ) ;
#41256=CARTESIAN_POINT ( 'NONE',  ( 100.9560082937595666, -28.70598565321984452, 61.59410917070462688 ) ) ;
#41257=CARTESIAN_POINT ( 'NONE',  ( 97.94803474170373647, -41.87343025248883777, 136.7356252759109623 ) ) ;
#41258=VERTEX_POINT ( 'NONE', #69222 ) ;
#41259=CARTESIAN_POINT ( 'NONE',  ( 181.9790560690580037, -31.62489322948711035, -5.074374724088000832 ) ) ;
#41260=CARTESIAN_POINT ( 'NONE',  ( 97.90015701271006776, -41.74100594024375965, 217.7241967044829494 ) ) ;
#41262=CYLINDRICAL_SURFACE ( 'NONE', #8297, 2.517499999999998739 ) ;
#41265=ORIENTED_EDGE ( 'NONE', *, *, #21524, .F. ) ;
#41266=ADVANCED_FACE ( 'NONE', ( #33354 ), #48295, .T. ) ;
#41267=ORIENTED_EDGE ( 'NONE', *, *, #80513, .T. ) ;
#41268=ORIENTED_EDGE ( 'NONE', *, *, #4663, .F. ) ;
#41271=CARTESIAN_POINT ( 'NONE',  ( 96.67410449796260252, -35.53789531767939991, 202.2356252759109623 ) ) ;
#41273=DIRECTION ( 'NONE',  ( 9.351236661543306751E-17, -3.725950533538267725E-29, -1.000000000000000000 ) ) ;
#41275=CARTESIAN_POINT ( 'NONE',  ( 29.56670390244797630, -48.82844715994099971, 20.91780685541479912 ) ) ;
#41277=VERTEX_POINT ( 'NONE', #6543 ) ;
#41279=ORIENTED_EDGE ( 'NONE', *, *, #43782, .F. ) ;
#41280=FACE_OUTER_BOUND ( 'NONE', #55590, .T. ) ;
#41281=CIRCLE ( 'NONE', #25338, 3.000000000000002665 ) ;
#41282=LINE ( 'NONE', #55354, #67958 ) ;
#41283=CARTESIAN_POINT ( 'NONE',  ( 110.8764511561472119, -27.72125199330416478, 240.7584824187679544 ) ) ;
#41286=CARTESIAN_POINT ( 'NONE',  ( 112.1775644307543587, -28.39036538331633963, 90.63848241876793566 ) ) ;
#41288=EDGE_CURVE ( 'NONE', #4876, #89309, #13807, .T. ) ;
#41289=EDGE_CURVE ( 'NONE', #22204, #58575, #56246, .T. ) ;
#41291=ORIENTED_EDGE ( 'NONE', *, *, #5463, .T. ) ;
#41292=DIRECTION ( 'NONE',  ( 0.000000000000000000, 0.000000000000000000, -1.000000000000000000 ) ) ;
#41294=ORIENTED_EDGE ( 'NONE', *, *, #56546, .F. ) ;
#41295=VERTEX_POINT ( 'NONE', #89228 ) ;
#41297=CARTESIAN_POINT ( 'NONE',  ( 115.9273305379513062, -35.98950415022901694, 250.3244404487543022 ) ) ;
#41298=CARTESIAN_POINT ( 'NONE',  ( 101.9936208522100003, -45.44607148789093287, 192.1564586011733411 ) ) ;
#41301=AXIS2_PLACEMENT_3D ( 'NONE', #80461, #5952, #4598 ) ;
#41302=FACE_OUTER_BOUND ( 'NONE', #39123, .T. ) ;
#41304=VECTOR ( 'NONE', #32883, 1000.000000000000000 ) ;
#41305=VERTEX_POINT ( 'NONE', #12924 ) ;
#41307=AXIS2_PLACEMENT_3D ( 'NONE', #80874, #88133, #68124 ) ;
#41308=CARTESIAN_POINT ( 'NONE',  ( 80.06648329127402519, -46.72944715994105991, 4.925625275910944012 ) ) ;
#41309=ORIENTED_EDGE ( 'NONE', *, *, #38268, .T. ) ;
#41310=CARTESIAN_POINT ( 'NONE',  ( 112.1813298990327183, -27.60452245592377807, 34.66991099019695355 ) ) ;
#41311=VERTEX_POINT ( 'NONE', #88783 ) ;
#41312=CARTESIAN_POINT ( 'NONE',  ( 103.3964814340166498, -45.24903370896166876, 285.0709475124485266 ) ) ;
#41313=CARTESIAN_POINT ( 'NONE',  ( 107.0664832912739399, -36.72944715994095333, 289.6356252759107406 ) ) ;
#41314=CARTESIAN_POINT ( 'NONE',  ( 102.8912152862169762, -46.22186109533351583, 132.2346728949589760 ) ) ;
#41315=DIRECTION ( 'NONE',  ( -0.000000000000000000, 1.000000000000000000, 0.000000000000000000 ) ) ;
#41316=DIRECTION ( 'NONE',  ( 1.000000000000000000, 0.000000000000000000, 0.000000000000000000 ) ) ;
#41317=DIRECTION ( 'NONE',  ( -4.237773401492740281E-14, 1.000000000000000000, 0.000000000000000000 ) ) ;
#41320=CARTESIAN_POINT ( 'NONE',  ( 97.57588284487002284, -41.14775938459609250, 252.6727681330536655 ) ) ;
#41323=VERTEX_POINT ( 'NONE', #81533 ) ;
#41324=CARTESIAN_POINT ( 'NONE',  ( 118.9531587402301511, -36.16547954148851574, 114.8641967044819694 ) ) ;
#41325=CARTESIAN_POINT ( 'NONE',  ( 75.31670390244798341, -50.82844715994100682, 35.51780685541480409 ) ) ;
#41327=CIRCLE ( 'NONE', #9454, 2.125000000000001776 ) ;
#41328=ORIENTED_EDGE ( 'NONE', *, *, #55195, .T. ) ;
#41330=CARTESIAN_POINT ( 'NONE',  ( 115.0889058099493951, -30.61763831142564740, 265.3439584562066784 ) ) ;
#41331=DIRECTION ( 'NONE',  ( -0.7071067811567310901, 0.7071067812163639443, 0.000000000000000000 ) ) ;
#41332=CARTESIAN_POINT ( 'NONE',  ( 107.0664832912739399, -36.72944715994095333, 293.6356252759106837 ) ) ;
#41334=CARTESIAN_POINT ( 'NONE',  ( 99.48373692063242402, -40.90112338471579534, 174.5328522743529618 ) ) ;
#41335=CARTESIAN_POINT ( 'NONE',  ( 118.3644662943939636, -33.07169432158188727, 280.0756252759109657 ) ) ;
#41336=FACE_OUTER_BOUND ( 'NONE', #70875, .T. ) ;
#41337=ORIENTED_EDGE ( 'NONE', *, *, #10802, .F. ) ;
#41339=CARTESIAN_POINT ( 'NONE',  ( 98.30752531352220558, -41.72886023108350884, 41.73921390539881315 ) ) ;
#41341=ORIENTED_EDGE ( 'NONE', *, *, #35530, .T. ) ;
#41343=CARTESIAN_POINT ( 'NONE',  ( 172.5664832912740110, -18.82844715994099971, 198.9256252759119832 ) ) ;
#41345=EDGE_LOOP ( 'NONE', ( #73013, #46214, #17942, #17949 ) ) ;
#41348=CARTESIAN_POINT ( 'NONE',  ( 99.09565760681786628, -30.55049705524844583, 15.80229833326679945 ) ) ;
#41352=CARTESIAN_POINT ( 'NONE',  ( 115.9822952273240304, -35.14169155943780964, 198.3771817328379825 ) ) ;
#41353=CARTESIAN_POINT ( 'NONE',  ( 101.0407447616467351, -27.40725005837418138, 70.54514908543497143 ) ) ;
#41355=ORIENTED_EDGE ( 'NONE', *, *, #7156, .F. ) ;
#41356=EDGE_CURVE ( 'NONE', #66655, #12481, #89675, .T. ) ;
#41357=DIRECTION ( 'NONE',  ( 0.7071067811865473507, 0.7071067811865476838, 0.000000000000000000 ) ) ;
#41359=EDGE_CURVE ( 'NONE', #61092, #74286, #47859, .T. ) ;
#41360=ADVANCED_FACE ( 'NONE', ( #41052, #69669 ), #49201, .F. ) ;
#41361=EDGE_LOOP ( 'NONE', ( #20606, #24322, #26470, #61500 ) ) ;
#41365=ADVANCED_FACE ( 'NONE', ( #77378, #8342 ), #35580, .F. ) ;
#41366=DIRECTION ( 'NONE',  ( 1.000000000000000078E-15, -1.000000000000000083E-30, -1.000000000000000000 ) ) ;
#41369=CARTESIAN_POINT ( 'NONE',  ( 112.8299879122683791, -27.27019477826133453, 49.62895860924498947 ) ) ;
#41370=AXIS2_PLACEMENT_3D ( 'NONE', #15181, #55581, #1560 ) ;
#41373=DIRECTION ( 'NONE',  ( 1.000000000000000000, 0.000000000000000000, 0.000000000000000000 ) ) ;
#41376=CARTESIAN_POINT ( 'NONE',  ( 132.7641780748903670, -16.30680158338876140, 1.893168945964847083 ) ) ;
#41379=CARTESIAN_POINT ( 'NONE',  ( 97.46090605037130672, -39.66038733884047929, 122.5612088153949770 ) ) ;
#41380=ADVANCED_FACE ( 'NONE', ( #21984, #15156 ), #42832, .F. ) ;
#41381=VECTOR ( 'NONE', #34923, 1000.000000000000000 ) ;
#41385=CARTESIAN_POINT ( 'NONE',  ( 100.9304087016431453, -28.27451679452656919, 71.57562527591099411 ) ) ;
#41393=CARTESIAN_POINT ( 'NONE',  ( 96.03815445040697796, -38.18343476501374312, 147.4299109901959923 ) ) ;
#41395=ORIENTED_EDGE ( 'NONE', *, *, #75910, .T. ) ;
#41396=CARTESIAN_POINT ( 'NONE',  ( 110.8846227072671979, -27.01418920731900641, 265.7784824187680783 ) ) ;
#41397=CARTESIAN_POINT ( 'NONE',  ( 97.81217157231137094, -40.51860488209471356, 252.6356829567330067 ) ) ;
#41399=FACE_OUTER_BOUND ( 'NONE', #22372, .T. ) ;
#41403=DIRECTION ( 'NONE',  ( -1.000000000000000000, 6.036837696399451257E-13, 0.000000000000000000 ) ) ;
#41404=EDGE_CURVE ( 'NONE', #37614, #11261, #616, .T. ) ;
#41405=CARTESIAN_POINT ( 'NONE',  ( 97.28849942844331622, -36.49606577720025768, 196.3070538473399438 ) ) ;
#41407=ORIENTED_EDGE ( 'NONE', *, *, #23422, .F. ) ;
#41409=CARTESIAN_POINT ( 'NONE',  ( 103.5819202103828474, -28.00394742224748157, 171.8225356868499603 ) ) ;
#41411=CARTESIAN_POINT ( 'NONE',  ( 97.18779024860596394, -39.88384922728100435, 277.5603871806723646 ) ) ;
#41412=CARTESIAN_POINT ( 'NONE',  ( 78.88305248756961419, -34.24700279812927306, 1.845048209624124524 ) ) ;
#41414=CARTESIAN_POINT ( 'NONE',  ( 107.0664832912739968, -36.72944715994100306, 287.6356252759109680 ) ) ;
#41416=DIRECTION ( 'NONE',  ( -1.000000000000000000, -4.299999999999999979E-14, -1.000000000000000078E-15 ) ) ;
#41418=CARTESIAN_POINT ( 'NONE',  ( 97.19046783542276557, -39.99946004141662570, 241.5813395616249863 ) ) ;
#41419=CARTESIAN_POINT ( 'NONE',  ( 104.4905646008501492, -26.97862835665753067, 170.2804552535220353 ) ) ;
#41420=ORIENTED_EDGE ( 'NONE', *, *, #41453, .F. ) ;
#41421=EDGE_LOOP ( 'NONE', ( #29817, #28423, #17446, #81212 ) ) ;
#41422=CARTESIAN_POINT ( 'NONE',  ( 113.1782937619596936, -44.75186859986670385, 88.09395860831342873 ) ) ;
#41423=CARTESIAN_POINT ( 'NONE',  ( 82.72821098188319411, -19.44060378571146330, 6.877169033952460708 ) ) ;
#41427=DIRECTION ( 'NONE',  ( 0.000000000000000000, 0.000000000000000000, 1.000000000000000000 ) ) ;
#41429=VECTOR ( 'NONE', #82669, 1000.000000000000000 ) ;
#41430=CARTESIAN_POINT ( 'NONE',  ( 115.4796304032075653, -43.01888039838633659, 24.31562527591096767 ) ) ;
#41431=AXIS2_PLACEMENT_3D ( 'NONE', #27691, #69029, #76290 ) ;
#41432=VECTOR ( 'NONE', #48893, 1000.000000000000000 ) ;
#41433=CARTESIAN_POINT ( 'NONE',  ( 97.01631923850186467, -33.95794342121210718, 251.1127681330538337 ) ) ;
#41434=ORIENTED_EDGE ( 'NONE', *, *, #85507, .T. ) ;
#41436=LINE ( 'NONE', #21929, #54384 ) ;
#41437=CARTESIAN_POINT ( 'NONE',  ( 113.6980717437190833, -44.24279107308028358, 168.1518506361709626 ) ) ;
#41438=CARTESIAN_POINT ( 'NONE',  ( 104.6989491262461769, -45.05385146434951338, 65.18618560768597092 ) ) ;
#41439=CARTESIAN_POINT ( 'NONE',  ( 117.3314307007336481, -34.78826007317788083, 154.9756252759109714 ) ) ;
#41440=CARTESIAN_POINT ( 'NONE',  ( 51.06648329127400388, -0.2185775633790978945, 333.4006252759120343 ) ) ;
#41441=ORIENTED_EDGE ( 'NONE', *, *, #36236, .F. ) ;
#41442=VECTOR ( 'NONE', #66311, 1000.000000000000000 ) ;
#41443=PLANE ( 'NONE',  #37840 ) ;
#41444=EDGE_CURVE ( 'NONE', #63459, #83484, #42386, .T. ) ;
#41445=ORIENTED_EDGE ( 'NONE', *, *, #44793, .T. ) ;
#41446=VERTEX_POINT ( 'NONE', #14562 ) ;
#41447=CARTESIAN_POINT ( 'NONE',  ( 69.25757238336807120, -1.944390235229864539, 361.9756252759101471 ) ) ;
#41450=CARTESIAN_POINT ( 'NONE',  ( 161.4809174648184182, -49.32844715993547879, 249.9678068554149490 ) ) ;
#41453=EDGE_CURVE ( 'NONE', #19998, #10951, #47699, .T. ) ;
#41454=CARTESIAN_POINT ( 'NONE',  ( 98.52328466580365784, -37.41198607556916755, 100.8124198280769832 ) ) ;
#41455=CARTESIAN_POINT ( 'NONE',  ( 104.1796880194223576, -26.65200820554803585, 225.2984824187679749 ) ) ;
#41456=EDGE_CURVE ( 'NONE', #29419, #87456, #50430, .T. ) ;
#41457=CARTESIAN_POINT ( 'NONE',  ( 106.4848323041101850, -24.91801670280273129, 195.1156252759109861 ) ) ;
#41458=CARTESIAN_POINT ( 'NONE',  ( 112.9508454419805332, -28.15023113465295879, 40.59848241876795782 ) ) ;
#41464=EDGE_CURVE ( 'NONE', #72856, #86673, #12764, .T. ) ;
#41465=CARTESIAN_POINT ( 'NONE',  ( 116.9564367646783722, -33.61053620760070260, 129.0575300378169743 ) ) ;
#41466=CARTESIAN_POINT ( 'NONE',  ( 117.1340566916381789, -32.05431620389533265, 59.16038718067295576 ) ) ;
#41467=CARTESIAN_POINT ( 'NONE',  ( 116.9671346634708442, -41.74840980516093936, 248.4651490854349731 ) ) ;
#41469=CARTESIAN_POINT ( 'NONE',  ( 103.8197072928965810, -48.12676840017521585, 217.3556252759109668 ) ) ;
#41470=CARTESIAN_POINT ( 'NONE',  ( 98.34985886569381819, -31.65658488862931819, 35.90645861648791737 ) ) ;
#41472=CARTESIAN_POINT ( 'NONE',  ( 101.9930969677325407, -45.44575997282210267, 23.15640987073907553 ) ) ;
#41473=CARTESIAN_POINT ( 'NONE',  ( 29.56670390244743629, -48.82844715994161078, 180.4678068554150911 ) ) ;
#41474=CARTESIAN_POINT ( 'NONE',  ( 107.0664832912739257, -18.82844715994099971, 239.5838068554170093 ) ) ;
#41475=DIRECTION ( 'NONE',  ( 1.000000000000000000, 4.163336342344333240E-14, 0.000000000000000000 ) ) ;
#41477=CARTESIAN_POINT ( 'NONE',  ( 107.0664832912740252, -46.47944715994103149, -4.824374724089029343 ) ) ;
#41478=EDGE_CURVE ( 'NONE', #31607, #22927, #6925, .T. ) ;
#41480=CARTESIAN_POINT ( 'NONE',  ( 134.0664832912740110, -8.729447159940999512, 311.1531252759119752 ) ) ;
#41481=LINE ( 'NONE', #69211, #25616 ) ;
#41482=LINE ( 'NONE', #70106, #65199 ) ;
#41483=EDGE_CURVE ( 'NONE', #9653, #16775, #20917, .T. ) ;
#41484=CARTESIAN_POINT ( 'NONE',  ( 71.25416588882602298, -72.55705569728901594, 542.9756252759101471 ) ) ;
#41485=EDGE_LOOP ( 'NONE', ( #30508, #51677, #39545, #15160 ) ) ;
#41487=CARTESIAN_POINT ( 'NONE',  ( 116.9057501799638601, -41.81710558299434410, 243.4346728949589647 ) ) ;
#41488=CARTESIAN_POINT ( 'NONE',  ( 114.2399097434533246, -45.14383888093294672, 149.1508633711489722 ) ) ;
#41489=CARTESIAN_POINT ( 'NONE',  ( 96.97452011921430426, -33.94641660286638540, 247.1127681330539758 ) ) ;
#41490=VECTOR ( 'NONE', #51713, 1000.000000000000000 ) ;
#41491=DIRECTION ( 'NONE',  ( 0.7071067811865475727, -0.7071067811865475727, 0.000000000000000000 ) ) ;
#41492=DIRECTION ( 'NONE',  ( 0.000000000000000000, 0.000000000000000000, -1.000000000000000000 ) ) ;
#41494=CARTESIAN_POINT ( 'NONE',  ( 116.3289480479917017, -32.94026123176625731, 29.13562527591096085 ) ) ;
#41495=DIRECTION ( 'NONE',  ( 0.0001713722456129695634, -0.9999999853157764962, 0.000000000000000000 ) ) ;
#41496=VECTOR ( 'NONE', #19208, 1000.000000000000000 ) ;
#41498=AXIS2_PLACEMENT_3D ( 'NONE', #44437, #9490, #37649 ) ;
#41499=ORIENTED_EDGE ( 'NONE', *, *, #84347, .T. ) ;
#41502=CARTESIAN_POINT ( 'NONE',  ( 115.0466524894680731, -42.26004630958951935, 162.7667055423629847 ) ) ;
#41503=CARTESIAN_POINT ( 'NONE',  ( 97.81151477712479902, -40.51751189930152464, 186.6359914586728337 ) ) ;
#41504=EDGE_LOOP ( 'NONE', ( #31749, #64385, #14071, #70528 ) ) ;
#41505=LINE ( 'NONE', #27890, #5466 ) ;
#41506=CARTESIAN_POINT ( 'NONE',  ( 98.02603654163385727, -30.41010087969375775, 156.8289586092439549 ) ) ;
#41507=CARTESIAN_POINT ( 'NONE',  ( 61.67079006425790766, -0.9306969701460061639, 542.9756252759101471 ) ) ;
#41508=DIRECTION ( 'NONE',  ( -1.110223024625155531E-13, -1.000000000000000000, 0.000000000000000000 ) ) ;
#41510=DIRECTION ( 'NONE',  ( 0.000000000000000000, 0.000000000000000000, 1.000000000000000000 ) ) ;
#41511=ADVANCED_FACE ( 'NONE', ( #5954, #33644 ), #54053, .F. ) ;
#41512=AXIS2_PLACEMENT_3D ( 'NONE', #47378, #81058, #75113 ) ;
#41513=CARTESIAN_POINT ( 'NONE',  ( 97.42673588038233845, -38.38435052442954998, 91.46133956162594814 ) ) ;
#41514=ORIENTED_EDGE ( 'NONE', *, *, #88693, .T. ) ;
#41517=DIRECTION ( 'NONE',  ( -1.000000000000000000, 0.000000000000000000, 0.000000000000000000 ) ) ;
#41518=CARTESIAN_POINT ( 'NONE',  ( 112.7790632652331482, -27.19118669266625687, 200.6470538473389809 ) ) ;
#41520=AXIS2_PLACEMENT_3D ( 'NONE', #22109, #29808, #47641 ) ;
#41523=DIRECTION ( 'NONE',  ( 1.000000000000000000, 0.000000000000000000, 0.000000000000000000 ) ) ;
#41526=CARTESIAN_POINT ( 'NONE',  ( 96.62907006607237292, -36.88702529232764249, 136.3384824187679385 ) ) ;
#41528=ORIENTED_EDGE ( 'NONE', *, *, #69189, .T. ) ;
#41529=ORIENTED_EDGE ( 'NONE', *, *, #27908, .F. ) ;
#41530=EDGE_CURVE ( 'NONE', #28914, #34067, #69965, .T. ) ;
#41531=CARTESIAN_POINT ( 'NONE',  ( 177.8371591254543205, -47.82818131005477369, 300.4678068554149490 ) ) ;
#41534=CARTESIAN_POINT ( 'NONE',  ( 98.43814749271325582, -36.05658283995993685, 189.0947570362579597 ) ) ;
#41535=EDGE_CURVE ( 'NONE', #27470, #85514, #88625, .T. ) ;
#41536=CARTESIAN_POINT ( 'NONE',  ( 123.6837132603318565, -20.11243780205705534, 229.5838068554170093 ) ) ;
#41542=ORIENTED_EDGE ( 'NONE', *, *, #85853, .T. ) ;
#41545=CARTESIAN_POINT ( 'NONE',  ( 110.1832024441707460, -27.86589328696400969, 251.2511071154212061 ) ) ;
#41547=AXIS2_PLACEMENT_3D ( 'NONE', #49823, #14887, #56180 ) ;
#41548=LINE ( 'NONE', #61552, #11714 ) ;
#41550=AXIS2_PLACEMENT_3D ( 'NONE', #79555, #78222, #70953 ) ;
#41551=ORIENTED_EDGE ( 'NONE', *, *, #75159, .T. ) ;
#41552=ORIENTED_EDGE ( 'NONE', *, *, #49249, .T. ) ;
#41553=VECTOR ( 'NONE', #71905, 1000.000000000000000 ) ;
#41554=VECTOR ( 'NONE', #58847, 1000.000000000000000 ) ;
#41555=CARTESIAN_POINT ( 'NONE',  ( 119.2637946045969954, -42.39761235918182791, 25.56312527591098416 ) ) ;
#41557=ORIENTED_EDGE ( 'NONE', *, *, #13817, .F. ) ;
#41558=EDGE_CURVE ( 'NONE', #34951, #60793, #19563, .T. ) ;
#41559=ADVANCED_FACE ( 'NONE', ( #74980 ), #54948, .T. ) ;
#41560=CARTESIAN_POINT ( 'NONE',  ( 110.7520593201813597, -44.56232478875543990, 285.7328522743533767 ) ) ;
#41561=CARTESIAN_POINT ( 'NONE',  ( 97.55101884832849635, -31.05922868340991627, 130.9108633711489915 ) ) ;
#41563=CARTESIAN_POINT ( 'NONE',  ( 101.6894933626719819, -27.09867346898205298, 105.4937205140069665 ) ) ;
#41564=CARTESIAN_POINT ( 'NONE',  ( 101.3006676746225310, -42.31480118910680233, 249.5838068554172651 ) ) ;
#41566=CARTESIAN_POINT ( 'NONE',  ( 118.8773263846236148, -37.69826137473897631, 184.7613395616249647 ) ) ;
#41567=CARTESIAN_POINT ( 'NONE',  ( 32.06670390244571678, -32.29483332968550258, 193.9678068554150911 ) ) ;
#41571=VERTEX_POINT ( 'NONE', #62691 ) ;
#41573=VERTEX_POINT ( 'NONE', #34978 ) ;
#41577=AXIS2_PLACEMENT_3D ( 'NONE', #18454, #33878, #47036 ) ;
#41578=CARTESIAN_POINT ( 'NONE',  ( 98.45854724665603896, -30.84808103350501085, 120.8499109901969604 ) ) ;
#41580=LINE ( 'NONE', #75683, #27529 ) ;
#41584=CARTESIAN_POINT ( 'NONE',  ( 115.4423046205436094, -29.55243945206544609, 225.4022919425769658 ) ) ;
#41586=DIRECTION ( 'NONE',  ( 1.000000000000000000, 4.163336342344333240E-14, 0.000000000000000000 ) ) ;
#41591=FACE_OUTER_BOUND ( 'NONE', #48231, .T. ) ;
#41593=CARTESIAN_POINT ( 'NONE',  ( 105.0129988258793645, -25.82091521352475283, 280.2365776568630622 ) ) ;
#41594=ORIENTED_EDGE ( 'NONE', *, *, #84094, .T. ) ;
#41596=CARTESIAN_POINT ( 'NONE',  ( 117.0443417989465758, -39.94358261462815562, 158.5784824187679476 ) ) ;
#41597=CARTESIAN_POINT ( 'NONE',  ( 99.29379691555868703, -43.72992423520055638, 52.90991099019698396 ) ) ;
#41598=CARTESIAN_POINT ( 'NONE',  ( 113.6418603426413938, -28.58344220020606130, 160.5356252759109736 ) ) ;
#41599=CARTESIAN_POINT ( 'NONE',  ( 97.81168736999980240, -40.51740164104307240, 32.63591986563997693 ) ) ;
#41600=CARTESIAN_POINT ( 'NONE',  ( 112.1392343750146381, -28.01276493709994853, 100.6565439726868760 ) ) ;
#41603=DIRECTION ( 'NONE',  ( 0.000000000000000000, 0.000000000000000000, 1.000000000000000000 ) ) ;
#41604=FACE_OUTER_BOUND ( 'NONE', #15009, .T. ) ;
#41605=LINE ( 'NONE', #13476, #65409 ) ;
#41606=ORIENTED_EDGE ( 'NONE', *, *, #50817, .F. ) ;
#41609=ORIENTED_EDGE ( 'NONE', *, *, #53554, .T. ) ;
#41611=CARTESIAN_POINT ( 'NONE',  ( 136.8164832912739826, -36.72944715994100306, 14.92562527591100263 ) ) ;
#41612=CARTESIAN_POINT ( 'NONE',  ( 98.73996931189277859, -42.96625968561437503, 62.83848241876793850 ) ) ;
#41613=DIRECTION ( 'NONE',  ( 0.000000000000000000, 1.000000000000000000, 0.000000000000000000 ) ) ;
#41615=CARTESIAN_POINT ( 'NONE',  ( 103.7937703862009613, -26.78548768338485075, 161.3299109901969643 ) ) ;
#41618=CIRCLE ( 'NONE', #2488, 2.750000000000002665 ) ;
#41619=EDGE_CURVE ( 'NONE', #59006, #79006, #34535, .T. ) ;
#41620=CARTESIAN_POINT ( 'NONE',  ( 98.46141696562543189, -39.55439615822902510, 286.0133722090292849 ) ) ;
#41623=EDGE_LOOP ( 'NONE', ( #11384, #65838, #31734, #45434 ) ) ;
#41624=AXIS2_PLACEMENT_3D ( 'NONE', #18822, #66062, #3855 ) ;
#41626=CARTESIAN_POINT ( 'NONE',  ( 131.0667039024480118, -61.87844715994100397, 231.5838068554150198 ) ) ;
#41628=CARTESIAN_POINT ( 'NONE',  ( 115.0884725098965049, -30.61707623100678077, 160.3440144957833127 ) ) ;
#41629=DIRECTION ( 'NONE',  ( 1.000000000000000078E-15, -1.000000000000000000, 0.000000000000000000 ) ) ;
#41630=CARTESIAN_POINT ( 'NONE',  ( 76.06670390244809710, -58.72944715994109544, 199.5838068554169524 ) ) ;
#41632=DIRECTION ( 'NONE',  ( 0.000000000000000000, 0.000000000000000000, -1.000000000000000000 ) ) ;
#41633=PLANE ( 'NONE',  #2790 ) ;
#41634=CARTESIAN_POINT ( 'NONE',  ( 105.1675567143510079, -46.98732170830152910, 12.42991099019596923 ) ) ;
#41636=ORIENTED_EDGE ( 'NONE', *, *, #79124, .F. ) ;
#41637=DIRECTION ( 'NONE',  ( 0.000000000000000000, 0.000000000000000000, -1.000000000000000000 ) ) ;
#41639=DIRECTION ( 'NONE',  ( 0.000000000000000000, 0.000000000000000000, -1.000000000000000000 ) ) ;
#41640=CARTESIAN_POINT ( 'NONE',  ( 112.1086029179114547, -30.31019831854434443, 77.36523322673394887 ) ) ;
#41642=EDGE_CURVE ( 'NONE', #62557, #80300, #82428, .T. ) ;
#41643=CYLINDRICAL_SURFACE ( 'NONE', #16562, 2.500000000000002220 ) ;
#41644=CARTESIAN_POINT ( 'NONE',  ( 63.03715912545737865, -24.89890238295017966, 249.9678068554150343 ) ) ;
#41645=ORIENTED_EDGE ( 'NONE', *, *, #52464, .F. ) ;
#41647=CARTESIAN_POINT ( 'NONE',  ( 77.61460381940253228, -35.48272374588488276, 7.134497377257247308 ) ) ;
#41648=VERTEX_POINT ( 'NONE', #15899 ) ;
#41649=CARTESIAN_POINT ( 'NONE',  ( 101.7694246217487972, -45.70876760617753831, 162.1527681330539679 ) ) ;
#41652=CARTESIAN_POINT ( 'NONE',  ( 113.3955173535308063, -30.52198670013464010, 145.8758690201829609 ) ) ;
#41654=CARTESIAN_POINT ( 'NONE',  ( 101.1286207290677908, -27.37920684556040740, 61.51467289495899138 ) ) ;
#41655=VECTOR ( 'NONE', #61164, 1000.000000000000114 ) ;
#41657=ORIENTED_EDGE ( 'NONE', *, *, #30022, .F. ) ;
#41659=ORIENTED_EDGE ( 'NONE', *, *, #50746, .T. ) ;
#41660=ORIENTED_EDGE ( 'NONE', *, *, #66414, .T. ) ;
#41661=ADVANCED_FACE ( 'NONE', ( #919 ), #63595, .F. ) ;
#41663=EDGE_LOOP ( 'NONE', ( #38626, #52190, #68367, #39357 ) ) ;
#41665=CARTESIAN_POINT ( 'NONE',  ( 97.82554479137630210, -33.52525840161893456, 286.0613395616258572 ) ) ;
#41666=CARTESIAN_POINT ( 'NONE',  ( 102.0714078572591319, -27.55412165564507632, 141.4727681330539895 ) ) ;
#41667=DIRECTION ( 'NONE',  ( 0.3818493186865920541, -0.9242245927363030855, 0.000000000000000000 ) ) ;
#41669=EDGE_CURVE ( 'NONE', #85162, #41221, #1166, .T. ) ;
#41670=CARTESIAN_POINT ( 'NONE',  ( 116.9748844278823015, -33.48813965163778050, 85.07848241876791917 ) ) ;
#41671=CARTESIAN_POINT ( 'NONE',  ( 105.7154773592118460, -46.72385839588265100, 262.4689586115381985 ) ) ;
#41673=CARTESIAN_POINT ( 'NONE',  ( 97.78516791111108830, -40.45206948340641162, 116.6303087853498255 ) ) ;
#41675=CIRCLE ( 'NONE', #31573, 3.250000000000002665 ) ;
#41677=ORIENTED_EDGE ( 'NONE', *, *, #41072, .T. ) ;
#41680=CIRCLE ( 'NONE', #2565, 0.5000000000000104361 ) ;
#41681=DIRECTION ( 'NONE',  ( 0.000000000000000000, 0.000000000000000000, 1.000000000000000000 ) ) ;
#41682=CARTESIAN_POINT ( 'NONE',  ( 99.12728904495253346, -44.42023919799950704, 41.95086337114900488 ) ) ;
#41683=DIRECTION ( 'NONE',  ( 4.299999999999999979E-14, -1.000000000000000000, 0.000000000000000000 ) ) ;
#41684=VECTOR ( 'NONE', #78789, 1000.000000000000000 ) ;
#41685=DIRECTION ( 'NONE',  ( 0.7071067811865496822, -0.7071067811865453523, 7.071067811865490124E-16 ) ) ;
#41686=DIRECTION ( 'NONE',  ( -0.9254794337955620787, -0.3787978585227822492, 0.000000000000000000 ) ) ;
#41687=CARTESIAN_POINT ( 'NONE',  ( 98.36549455146187881, -40.29075363668734155, 11.63562527591094309 ) ) ;
#41688=LINE ( 'NONE', #53513, #30426 ) ;
#41689=CARTESIAN_POINT ( 'NONE',  ( 117.8338636819850365, -39.12263375953639155, 99.64038718067195077 ) ) ;
#41691=CARTESIAN_POINT ( 'NONE',  ( 117.2351557800294870, -41.18040025386632408, 208.4861014663869696 ) ) ;
#41692=CARTESIAN_POINT ( 'NONE',  ( 32.16397622748888097, -34.03355364506390401, 117.4678068554150485 ) ) ;
#41693=ADVANCED_FACE ( 'NONE', ( #85847 ), #51277, .T. ) ;
#41694=ORIENTED_EDGE ( 'NONE', *, *, #45278, .T. ) ;
#41697=EDGE_CURVE ( 'NONE', #17090, #5230, #22719, .T. ) ;
#41698=CARTESIAN_POINT ( 'NONE',  ( 136.8164482479831463, -36.55833207210741165, 3.101428811466717228 ) ) ;
#41699=ORIENTED_EDGE ( 'NONE', *, *, #15960, .F. ) ;
#41700=AXIS2_PLACEMENT_3D ( 'NONE', #49744, #64295, #63389 ) ;
#41701=PLANE ( 'NONE',  #85387 ) ;
#41702=CARTESIAN_POINT ( 'NONE',  ( 99.97821182074206092, -27.16988623491039334, 185.5841967044829630 ) ) ;
#41704=PLANE ( 'NONE',  #46540 ) ;
#41705=CARTESIAN_POINT ( 'NONE',  ( 110.7038792373522824, -48.03394190404919328, 203.8241967044819489 ) ) ;
#41709=DIRECTION ( 'NONE',  ( 0.000000000000000000, 0.000000000000000000, -1.000000000000000000 ) ) ;
#41710=CARTESIAN_POINT ( 'NONE',  ( 57.56670390244829605, -48.82844715994039575, 293.2178068554150627 ) ) ;
#41711=VERTEX_POINT ( 'NONE', #79024 ) ;
#41715=ORIENTED_EDGE ( 'NONE', *, *, #55064, .T. ) ;
#41717=DIRECTION ( 'NONE',  ( 1.000000000000000078E-15, -1.000000000000000083E-30, -1.000000000000000000 ) ) ;
#41718=CARTESIAN_POINT ( 'NONE',  ( 116.0551108448461264, -42.01026737563550029, 234.4041967044819899 ) ) ;
#41719=CARTESIAN_POINT ( 'NONE',  ( 151.5667039024483813, -48.82844715993591223, 249.9678068554149490 ) ) ;
#41720=CARTESIAN_POINT ( 'NONE',  ( 136.5461822395285765, -17.53884010538699201, 2.747932095387902063 ) ) ;
#41721=CARTESIAN_POINT ( 'NONE',  ( 37.56670390244801183, -48.82844715994099971, 300.4678068554150059 ) ) ;
#41723=DIRECTION ( 'NONE',  ( -1.000000000000000078E-15, -1.000000000000000083E-30, 1.000000000000000000 ) ) ;
#41724=EDGE_CURVE ( 'NONE', #33505, #38464, #51894, .T. ) ;
#41725=CARTESIAN_POINT ( 'NONE',  ( 115.9640307963821186, -42.20482783266999149, 18.38705384733896153 ) ) ;
#41726=ORIENTED_EDGE ( 'NONE', *, *, #7549, .T. ) ;
#41728=VERTEX_POINT ( 'NONE', #56305 ) ;
#41732=CARTESIAN_POINT ( 'NONE',  ( 117.4008144674644285, -32.62901037329578458, 245.1270538473389706 ) ) ;
#41734=CARTESIAN_POINT ( 'NONE',  ( 116.4859054502388744, -39.36344060769043551, 94.60991099019594230 ) ) ;
#41736=CARTESIAN_POINT ( 'NONE',  ( 97.12555970502634750, -37.99686556195802467, 22.42726576103899916 ) ) ;
#41737=ORIENTED_EDGE ( 'NONE', *, *, #37022, .T. ) ;
#41738=CARTESIAN_POINT ( 'NONE',  ( 172.5664832912740110, -9.303447159940999356, 78.92562527591199739 ) ) ;
#41740=VERTEX_POINT ( 'NONE', #64048 ) ;
#41742=CARTESIAN_POINT ( 'NONE',  ( 114.8460652499425123, -41.03528437643323201, 259.8558690201828654 ) ) ;
#41743=VECTOR ( 'NONE', #85344, 1000.000000000000000 ) ;
#41744=CARTESIAN_POINT ( 'NONE',  ( 51.42025729304100423, -33.70561438051981185, -5.074374724088000832 ) ) ;
#41746=ADVANCED_FACE ( 'NONE', ( #84050 ), #29078, .T. ) ;
#41747=CARTESIAN_POINT ( 'NONE',  ( 116.3195061320206207, -32.94150711290046729, 139.1356252759109680 ) ) ;
#41748=CARTESIAN_POINT ( 'NONE',  ( 97.31584370922533367, -39.30597597294169532, 86.53145860710328918 ) ) ;
#41751=CARTESIAN_POINT ( 'NONE',  ( 53.35959712126282994, -48.62134037875357251, 249.9678068554150343 ) ) ;
#41752=DIRECTION ( 'NONE',  ( 1.000000000000000078E-15, -1.000000000000000000, 0.000000000000000000 ) ) ;
#41754=CARTESIAN_POINT ( 'NONE',  ( 117.4547340842499210, -37.95832963484174627, 53.73276813305394484 ) ) ;
#41756=CARTESIAN_POINT ( 'NONE',  ( 101.7271154311333135, -43.54062005560803073, 274.8776141791153691 ) ) ;
#41757=AXIS2_PLACEMENT_3D ( 'NONE', #67172, #52175, #18577 ) ;
#41758=ADVANCED_FACE ( 'NONE', ( #21825 ), #71759, .F. ) ;
#41759=CARTESIAN_POINT ( 'NONE',  ( 136.8164832912739826, -18.72944715994099951, -5.074374724088999145 ) ) ;
#41760=CARTESIAN_POINT ( 'NONE',  ( 103.1049807579881161, -45.67203811392948865, 177.2441967044829596 ) ) ;
#41761=LINE ( 'NONE', #83579, #47656 ) ;
#41762=LINE ( 'NONE', #14983, #89741 ) ;
#41763=PLANE ( 'NONE',  #28873 ) ;
#41764=AXIS2_PLACEMENT_3D ( 'NONE', #81167, #27077, #53848 ) ;
#41766=CARTESIAN_POINT ( 'NONE',  ( 100.6295653500825154, -44.98529764103543727, 228.0499109901969348 ) ) ;
#41769=CARTESIAN_POINT ( 'NONE',  ( 172.5664832912729878, -27.82844715994070484, 138.9256252759119832 ) ) ;
#41771=CARTESIAN_POINT ( 'NONE',  ( 97.57754503199339524, -30.97118795507763167, 121.8803871806729546 ) ) ;
#41772=DIRECTION ( 'NONE',  ( -4.237773401492740281E-14, 1.000000000000000000, 0.000000000000000000 ) ) ;
#41773=ORIENTED_EDGE ( 'NONE', *, *, #23367, .F. ) ;
#41774=ORIENTED_EDGE ( 'NONE', *, *, #44649, .F. ) ;
#41777=CARTESIAN_POINT ( 'NONE',  ( 99.09571867114192401, -30.55041957953722687, 266.8022907182795507 ) ) ;
#41780=DIRECTION ( 'NONE',  ( -0.7071067811865253683, 0.7071067811865696662, -7.071067811865261355E-16 ) ) ;
#41781=EDGE_CURVE ( 'NONE', #43903, #32539, #43579, .T. ) ;
#41782=CARTESIAN_POINT ( 'NONE',  ( 115.2023469127646820, -39.68048904007974897, 171.3557094172109885 ) ) ;
#41783=CARTESIAN_POINT ( 'NONE',  ( 105.8911342260945645, -47.14568079332288875, 278.4870538473395527 ) ) ;
#41784=CARTESIAN_POINT ( 'NONE',  ( 163.0667039024470171, -33.35206098992711077, -5.074374724088000832 ) ) ;
#41789=ORIENTED_EDGE ( 'NONE', *, *, #39118, .T. ) ;
#41791=DIRECTION ( 'NONE',  ( 2.900000000000000265E-14, -2.000000000000000155E-15, 1.000000000000000000 ) ) ;
#41792=CARTESIAN_POINT ( 'NONE',  ( 19.56670390244796920, -67.87844715994100397, 300.9178068554150514 ) ) ;
#41793=CARTESIAN_POINT ( 'NONE',  ( 113.2454827304145226, -28.75865971940361376, 14.55229357420379976 ) ) ;
#41794=CARTESIAN_POINT ( 'NONE',  ( 138.8167039024479834, -57.40094715994099772, 35.51780685541480409 ) ) ;
#41795=FACE_OUTER_BOUND ( 'NONE', #48868, .T. ) ;
#41796=CARTESIAN_POINT ( 'NONE',  ( 98.86656133049426387, -40.57313681482517609, 211.0857531614099685 ) ) ;
#41797=CARTESIAN_POINT ( 'NONE',  ( 115.6098187009959304, -42.78073513203698042, 53.33562527591095659 ) ) ;
#41799=CARTESIAN_POINT ( 'NONE',  ( 37.36643805256647966, -48.62818131006027755, 180.4678068554150911 ) ) ;
#41801=ORIENTED_EDGE ( 'NONE', *, *, #59814, .T. ) ;
#41807=CARTESIAN_POINT ( 'NONE',  ( 116.3181387014812458, -32.94505625723229514, 15.13562527591094664 ) ) ;
#41810=AXIS2_PLACEMENT_3D ( 'NONE', #11917, #16949, #80977 ) ;
#41811=DIRECTION ( 'NONE',  ( -1.000000000000000000, 0.000000000000000000, 7.043400939473319300E-33 ) ) ;
#41814=CARTESIAN_POINT ( 'NONE',  ( 97.75265732597522117, -31.99668793782200993, 50.95276813305294183 ) ) ;
#41818=CARTESIAN_POINT ( 'NONE',  ( 131.3164832912739826, -18.72944715994100662, 3.101481641215524832 ) ) ;
#41822=CONICAL_SURFACE ( 'NONE', #72329, 16.00000000000090239, 0.7853981633974503884 ) ;
#41825=EDGE_LOOP ( 'NONE', ( #78302, #4029, #47736, #38430 ) ) ;
#41826=CARTESIAN_POINT ( 'NONE',  ( 113.9312237880395600, -28.03689036367077492, 120.5565776568639507 ) ) ;
#41829=DIRECTION ( 'NONE',  ( 0.000000000000000000, 0.000000000000000000, 1.000000000000000000 ) ) ;
#41831=LINE ( 'NONE', #7342, #37558 ) ;
#41832=ADVANCED_FACE ( 'NONE', ( #71318 ), #37229, .F. ) ;
#41833=CARTESIAN_POINT ( 'NONE',  ( 117.0460787713798965, -39.54838250520747778, 139.6194347997199827 ) ) ;
#41834=AXIS2_PLACEMENT_3D ( 'NONE', #73873, #24395, #37578 ) ;
#41835=FACE_OUTER_BOUND ( 'NONE', #47259, .T. ) ;
#41836=ORIENTED_EDGE ( 'NONE', *, *, #72850, .T. ) ;
#41837=CARTESIAN_POINT ( 'NONE',  ( 105.6350724880777534, -47.03380199863519806, 253.4670538473393719 ) ) ;
#41838=DIRECTION ( 'NONE',  ( 0.4214249218767882055, 0.9068632946707806397, 4.214249218767890910E-16 ) ) ;
#41841=DIRECTION ( 'NONE',  ( 0.000000000000000000, 1.000000000000000000, 0.000000000000000000 ) ) ;
#41843=DIRECTION ( 'NONE',  ( 0.000000000000000000, 0.000000000000000000, -1.000000000000000000 ) ) ;
#41844=CARTESIAN_POINT ( 'NONE',  ( 116.5710038106515611, -34.42130396933979597, 209.0156252759109634 ) ) ;
#41845=ORIENTED_EDGE ( 'NONE', *, *, #50957, .T. ) ;
#41846=ORIENTED_EDGE ( 'NONE', *, *, #18812, .T. ) ;
#41848=CARTESIAN_POINT ( 'NONE',  ( 97.67166470235704878, -36.60562237181873257, 152.7596785439919813 ) ) ;
#41849=CARTESIAN_POINT ( 'NONE',  ( 116.3183510266638336, -32.94967450325654568, 119.1356252759109537 ) ) ;
#41851=CARTESIAN_POINT ( 'NONE',  ( 105.4490071354754406, -45.46730099742844544, 8.861583305896925111 ) ) ;
#41854=DIRECTION ( 'NONE',  ( 1.000000000000000000, 1.816601132648505598E-15, 0.000000000000000000 ) ) ;
#41857=CARTESIAN_POINT ( 'NONE',  ( 177.8371591254543489, -47.82818131005477369, 249.9678068554149775 ) ) ;
#41859=CARTESIAN_POINT ( 'NONE',  ( 98.85650974919595058, -29.36329775763224603, 235.7565776568629872 ) ) ;
#41860=CARTESIAN_POINT ( 'NONE',  ( 98.34975502646139489, -31.65672867875580465, 170.9057125034062778 ) ) ;
#41861=VERTEX_POINT ( 'NONE', #79922 ) ;
#41863=ADVANCED_FACE ( 'NONE', ( #4040 ), #58547, .F. ) ;
#41864=EDGE_CURVE ( 'NONE', #19262, #13968, #69377, .T. ) ;
#41865=DIRECTION ( 'NONE',  ( -4.237773401492740281E-14, 1.000000000000000000, 0.000000000000000000 ) ) ;
#41866=CARTESIAN_POINT ( 'NONE',  ( 82.77032304066598556, -19.23127003359734744, 6.817519769821898556 ) ) ;
#41867=FACE_OUTER_BOUND ( 'NONE', #46793, .T. ) ;
#41868=DIRECTION ( 'NONE',  ( 1.000000000000000078E-15, 1.000000000000000083E-30, -1.000000000000000000 ) ) ;
#41872=EDGE_CURVE ( 'NONE', #7655, #37616, #14092, .T. ) ;
#41874=CARTESIAN_POINT ( 'NONE',  ( 96.64589536673427972, -32.90729728488415162, 17.03467289495896964 ) ) ;
#41876=CARTESIAN_POINT ( 'NONE',  ( 96.77592423366979801, -40.76472679528808385, 246.6118157521009664 ) ) ;
#41877=VERTEX_POINT ( 'NONE', #81264 ) ;
#41878=VECTOR ( 'NONE', #5027, 1000.000000000000000 ) ;
#41879=CARTESIAN_POINT ( 'NONE',  ( 77.59226090854122049, -37.93375462384054941, 7.110117206087036124 ) ) ;
#41880=ADVANCED_FACE ( 'NONE', ( #4936 ), #80360, .T. ) ;
#41881=DIRECTION ( 'NONE',  ( -2.900000000000000265E-14, 2.000000000000000155E-15, -1.000000000000000000 ) ) ;
#41882=CARTESIAN_POINT ( 'NONE',  ( 110.8548770769551908, -45.98407163414527332, 167.8856600767107352 ) ) ;
#41884=CARTESIAN_POINT ( 'NONE',  ( 113.4406056323916090, -42.58363279299825876, 76.04142370292498754 ) ) ;
#41885=CARTESIAN_POINT ( 'NONE',  ( 101.7584646134851596, -45.72734648786122591, 158.1527681330539963 ) ) ;
#41889=CARTESIAN_POINT ( 'NONE',  ( 41.56648329127499153, -36.32844715994070839, 323.6756252759119548 ) ) ;
#41890=EDGE_LOOP ( 'NONE', ( #66698, #46299 ) ) ;
#41892=CARTESIAN_POINT ( 'NONE',  ( 33.91903122894391487, -35.91149509761189762, 117.4678068554150485 ) ) ;
#41893=VERTEX_POINT ( 'NONE', #51723 ) ;
#41894=ORIENTED_EDGE ( 'NONE', *, *, #58672, .F. ) ;
#41896=B_SPLINE_CURVE_WITH_KNOTS ( 'NONE', 3,
 ( #63860, #85214, #16159, #1640, #43837, #29340, #37038, #64743, #42487, #77040, #23432, #44276, #78839, #51099, #9780, #65189, #2968, #30667 ),
 .UNSPECIFIED., .F., .F.,
 ( 4, 2, 2, 2, 2, 2, 2, 2, 4 ),
 ( 0.000000000000000000, 0.06249999992548026240, 0.1249999998509605248, 0.1874999997764407733, 0.2499999997019210496, 0.3124999996274013259, 0.3749999995528815466, 0.4374999994783618229, 0.4999999994038420992 ),
 .UNSPECIFIED. ) ;
#41898=CARTESIAN_POINT ( 'NONE',  ( 113.7363519267670995, -42.85525508308114695, 77.64575316141092287 ) ) ;
#41899=CARTESIAN_POINT ( 'NONE',  ( 97.89977465614410335, -41.74121498826879417, 221.7241967044819546 ) ) ;
#41901=CARTESIAN_POINT ( 'NONE',  ( 97.07914014679025172, -41.41098531455293141, 211.6632443235299945 ) ) ;
#41902=CARTESIAN_POINT ( 'NONE',  ( 106.9276426037745011, -26.29176787048590214, 56.08705384733997334 ) ) ;
#41904=DIRECTION ( 'NONE',  ( 0.7071067811578790607, 0.7071067812152160847, 0.000000000000000000 ) ) ;
#41905=DIRECTION ( 'NONE',  ( -4.299999999999999979E-14, 1.000000000000000000, -4.400000000000000367E-29 ) ) ;
#41907=VERTEX_POINT ( 'NONE', #10683 ) ;
#41908=CARTESIAN_POINT ( 'NONE',  ( 117.0718954859017629, -35.46248235935014748, 178.9272919423596591 ) ) ;
#41909=EDGE_CURVE ( 'NONE', #38962, #60267, #51957, .T. ) ;
#41910=CARTESIAN_POINT ( 'NONE',  ( 152.0371591254585155, -47.82818131005588214, 193.9678068554149775 ) ) ;
#41912=VECTOR ( 'NONE', #50246, 999.9999999999998863 ) ;
#41913=CARTESIAN_POINT ( 'NONE',  ( 113.5922197990811213, -29.44396856740769408, 114.4956252759109816 ) ) ;
#41914=CARTESIAN_POINT ( 'NONE',  ( 115.3018890743646665, -44.17195851134204077, 83.25372051400698581 ) ) ;
#41915=CARTESIAN_POINT ( 'NONE',  ( 101.2695147780440266, -26.33598991146258328, 255.4813395616251626 ) ) ;
#41917=CARTESIAN_POINT ( 'NONE',  ( 109.9602307476630330, -48.22147533147688847, 242.7727681330539724 ) ) ;
#41922=LINE ( 'NONE', #63283, #68019 ) ;
#41924=CARTESIAN_POINT ( 'NONE',  ( 63.56670390244796920, -40.82844715994016127, 300.4678068554150627 ) ) ;
#41928=CARTESIAN_POINT ( 'NONE',  ( 113.2375375036158403, -28.75258929711289468, 39.55219311040522001 ) ) ;
#41930=CYLINDRICAL_SURFACE ( 'NONE', #80587, 4.749999999999976907 ) ;
#41933=DIRECTION ( 'NONE',  ( 1.000000000000000078E-15, -1.000000000000000083E-30, -1.000000000000000000 ) ) ;
#41934=CARTESIAN_POINT ( 'NONE',  ( 106.1363778353814666, -47.76712558329867875, 262.4975300378158067 ) ) ;
#41935=CARTESIAN_POINT ( 'NONE',  ( 107.6529936739636639, -47.12767891731729009, 148.6213395616249784 ) ) ;
#41936=CARTESIAN_POINT ( 'NONE',  ( 115.7313686325390876, -42.60420177353093862, 269.3527681330536439 ) ) ;
#41939=CARTESIAN_POINT ( 'NONE',  ( 81.78920663580979067, -34.57943358556376978, 7.744922197170968303 ) ) ;
#41940=CARTESIAN_POINT ( 'NONE',  ( 107.0664832912739399, -36.72944715994095333, 357.5272416190308604 ) ) ;
#41941=DIRECTION ( 'NONE',  ( 1.000000000000000078E-15, 0.000000000000000000, 1.000000000000000000 ) ) ;
#41942=AXIS2_PLACEMENT_3D ( 'NONE', #55791, #14049, #83546 ) ;
#41944=VERTEX_POINT ( 'NONE', #85242 ) ;
#41945=DIRECTION ( 'NONE',  ( -2.900000000000000265E-14, 2.000000000000000155E-15, -1.000000000000000000 ) ) ;
#41947=CARTESIAN_POINT ( 'NONE',  ( 106.9915265980828849, -45.27055441931952373, 186.9924198280769758 ) ) ;
#41949=CARTESIAN_POINT ( 'NONE',  ( 116.7934678734580132, -39.39373051261830483, 188.6148988220920444 ) ) ;
#41950=EDGE_LOOP ( 'NONE', ( #89311, #71444, #84698, #21389 ) ) ;
#41951=CARTESIAN_POINT ( 'NONE',  ( 135.3838309168194485, -60.54606547621062163, 394.9756252759104314 ) ) ;
#41952=CARTESIAN_POINT ( 'NONE',  ( 111.4081670832168953, -47.72935575799004226, 168.8756252759109486 ) ) ;
#41953=DIRECTION ( 'NONE',  ( 0.000000000000000000, 0.000000000000000000, -1.000000000000000000 ) ) ;
#41954=PLANE ( 'NONE',  #10963 ) ;
#41956=LINE ( 'NONE', #48769, #63603 ) ;
#41959=CARTESIAN_POINT ( 'NONE',  ( 116.9446180447427821, -41.83184233209006209, 93.44705384733997278 ) ) ;
#41960=VERTEX_POINT ( 'NONE', #44307 ) ;
#41962=EDGE_LOOP ( 'NONE', ( #85431, #9860, #81447 ) ) ;
#41963=CARTESIAN_POINT ( 'NONE',  ( 112.5007446479794453, -45.21116328700192355, 64.46158330589696561 ) ) ;
#41964=DIRECTION ( 'NONE',  ( 0.9068632946707805287, -0.4214249218767882610, 1.035655806553318316E-15 ) ) ;
#41965=CARTESIAN_POINT ( 'NONE',  ( 99.06478422775796844, -31.10483629442216014, 201.8384824187669437 ) ) ;
#41969=DIRECTION ( 'NONE',  ( 0.000000000000000000, -1.000000000000000000, 0.000000000000000000 ) ) ;
#41971=CIRCLE ( 'NONE', #34790, 4.750000000000004441 ) ;
#41973=ADVANCED_FACE ( 'NONE', ( #17517 ), #23010, .F. ) ;
#41974=DIRECTION ( 'NONE',  ( 0.000000000000000000, 0.000000000000000000, -1.000000000000000000 ) ) ;
#41975=DIRECTION ( 'NONE',  ( 1.639958061481212836E-42, -4.100000000000000342E-29, -1.000000000000000000 ) ) ;
#41976=CARTESIAN_POINT ( 'NONE',  ( 117.6568287320716877, -39.81301747186228113, 138.5889586092439743 ) ) ;
#41977=ORIENTED_EDGE ( 'NONE', *, *, #10942, .T. ) ;
#41979=ORIENTED_EDGE ( 'NONE', *, *, #43004, .T. ) ;
#41980=EDGE_CURVE ( 'NONE', #19751, #48239, #51999, .T. ) ;
#41981=EDGE_CURVE ( 'NONE', #10481, #77722, #75202, .T. ) ;
#41984=DIRECTION ( 'NONE',  ( 1.000000000000000078E-15, -1.000000000000000083E-30, -1.000000000000000000 ) ) ;
#41985=CARTESIAN_POINT ( 'NONE',  ( 100.3991921706488171, -43.18259834960616672, 189.7566617981629804 ) ) ;
#41986=AXIS2_PLACEMENT_3D ( 'NONE', #6913, #63674, #42310 ) ;
#41987=EDGE_CURVE ( 'NONE', #13081, #686, #12969, .T. ) ;
#41988=FACE_OUTER_BOUND ( 'NONE', #61837, .T. ) ;
#41990=CARTESIAN_POINT ( 'NONE',  ( 76.06670390244792657, -14.72944715994109899, 239.5838068554169809 ) ) ;
#41993=EDGE_LOOP ( 'NONE', ( #48880, #56507, #68933, #61060 ) ) ;
#41994=AXIS2_PLACEMENT_3D ( 'NONE', #63329, #22013, #49685 ) ;
#41997=ORIENTED_EDGE ( 'NONE', *, *, #4777, .T. ) ;
#41998=CARTESIAN_POINT ( 'NONE',  ( 78.21292805808276682, -20.76093376058618389, 7.655955902700432247 ) ) ;
#41999=EDGE_CURVE ( 'NONE', #55592, #15222, #86565, .T. ) ;
#42000=CARTESIAN_POINT ( 'NONE',  ( 107.4435086560219474, -45.58304137281263024, 234.0415833058969781 ) ) ;
#42003=ORIENTED_EDGE ( 'NONE', *, *, #36048, .T. ) ;
#42004=CARTESIAN_POINT ( 'NONE',  ( 194.0371591254582313, -46.82818131005407736, 313.9678068554149490 ) ) ;
#42005=ADVANCED_FACE ( 'NONE', ( #8935 ), #64774, .T. ) ;
#42008=VERTEX_POINT ( 'NONE', #57948 ) ;
#42011=DIRECTION ( 'NONE',  ( -0.7071067811864691910, -0.7071067811866257324, -7.071067811864685486E-16 ) ) ;
#42012=VERTEX_POINT ( 'NONE', #85683 ) ;
#42013=EDGE_LOOP ( 'NONE', ( #87849, #18350, #65683, #41294 ) ) ;
#42014=B_SPLINE_CURVE_WITH_KNOTS ( 'NONE', 3,
 ( #67420, #32904, #60603, #88343, #26103, #53772, #81538, #46962, #74693, #73799, #12474, #5666, #67880, #38827, #61057, #33805, #61499, #88788, #26544, #54217, #81978, #19727, #47416, #75144, #54663, #25196, #12928, #4321, #32009, #46064, #82430 ),
 .UNSPECIFIED., .F., .F.,
 ( 4, 2, 2, 1, 2, 2, 2, 2, 2, 2, 2, 1, 1, 2, 2, 2, 4 ),
 ( 0.000000000000000000, 0.1250000000000155431, 0.1875000000000143219, 0.2187500000000218991, 0.2343750000000257017, 0.2500000000000294764, 0.3750000000000295874, 0.4375000000000235367, 0.5000000000000174305, 0.6249999999999963363, 0.6874999999999857891, 0.7187499999999805711, 0.7343749999999779066, 0.7421874999999765743, 0.7499999999999752420, 0.8749999999999876765, 1.000000000000000000 ),
 .UNSPECIFIED. ) ;
#42015=CARTESIAN_POINT ( 'NONE',  ( 115.1807610290764075, -35.84162759104140150, 276.7309475124485516 ) ) ;
#42016=AXIS2_PLACEMENT_3D ( 'NONE', #63817, #1595, #84724 ) ;
#42017=CARTESIAN_POINT ( 'NONE',  ( 104.9583746955643448, -25.04227923723010463, 125.2184824187689856 ) ) ;
#42018=CARTESIAN_POINT ( 'NONE',  ( 118.8789388927533111, -36.16900092901214947, 118.8641967044819836 ) ) ;
#42019=DIRECTION ( 'NONE',  ( -1.000000000000000078E-15, 1.000000000000000083E-30, 1.000000000000000000 ) ) ;
#42020=CARTESIAN_POINT ( 'NONE',  ( 62.03742497533751532, -23.42844715994041849, 249.9678068554150343 ) ) ;
#42021=CARTESIAN_POINT ( 'NONE',  ( 106.9404422130490815, -47.78196244520037084, 228.5794347997199907 ) ) ;
#42023=CARTESIAN_POINT ( 'NONE',  ( 107.0664832912739257, -50.04551884050745514, 305.7141315223800007 ) ) ;
#42024=ORIENTED_EDGE ( 'NONE', *, *, #35421, .T. ) ;
#42026=ORIENTED_EDGE ( 'NONE', *, *, #20290, .F. ) ;
#42028=ORIENTED_EDGE ( 'NONE', *, *, #34364, .T. ) ;
#42029=CIRCLE ( 'NONE', #2889, 0.5000000000000004441 ) ;
#42030=DIRECTION ( 'NONE',  ( -1.000000000000000000, 0.000000000000000000, 0.000000000000000000 ) ) ;
#42034=CARTESIAN_POINT ( 'NONE',  ( 104.9628152733504720, -25.06689740840304381, 125.2184824187689856 ) ) ;
#42037=DIRECTION ( 'NONE',  ( 4.299999999999999979E-14, -1.000000000000000000, 4.400000000000000367E-29 ) ) ;
#42039=DIRECTION ( 'NONE',  ( 0.9242245927363031965, 0.3818493186865917766, 0.000000000000000000 ) ) ;
#42040=CARTESIAN_POINT ( 'NONE',  ( 106.2286657330468245, -47.72771449247510844, 263.5280062282920994 ) ) ;
#42041=LINE ( 'NONE', #7983, #17656 ) ;
#42043=ORIENTED_EDGE ( 'NONE', *, *, #62090, .T. ) ;
#42045=DIRECTION ( 'NONE',  ( 0.000000000000000000, 0.000000000000000000, 1.000000000000000000 ) ) ;
#42046=CARTESIAN_POINT ( 'NONE',  ( 87.31648329127402519, -56.72944715994104570, 14.67562527591095112 ) ) ;
#42049=CARTESIAN_POINT ( 'NONE',  ( 117.5632142390390555, -36.54506796471968499, 288.8413395616251478 ) ) ;
#42050=ORIENTED_EDGE ( 'NONE', *, *, #79660, .F. ) ;
#42052=CARTESIAN_POINT ( 'NONE',  ( 102.0711994968067984, -27.55373892369285826, 145.4727681330539610 ) ) ;
#42053=CARTESIAN_POINT ( 'NONE',  ( 116.7270850375765576, -31.35852969783502786, 25.24229194257798881 ) ) ;
#42054=CARTESIAN_POINT ( 'NONE',  ( 107.6554453082189013, -47.17114389581161049, 148.6213395616249784 ) ) ;
#42055=CARTESIAN_POINT ( 'NONE',  ( 107.0667039024467613, -36.72944715994091780, 196.8538068554170195 ) ) ;
#42056=CARTESIAN_POINT ( 'NONE',  ( 97.31301912648670793, -38.96037348457183214, 102.5053915444232047 ) ) ;
#42059=DIRECTION ( 'NONE',  ( -0.7071067811855830110, -0.7071067811875120235, 0.000000000000000000 ) ) ;
#42060=FACE_OUTER_BOUND ( 'NONE', #15467, .T. ) ;
#42062=ORIENTED_EDGE ( 'NONE', *, *, #32059, .F. ) ;
#42063=EDGE_CURVE ( 'NONE', #33219, #29809, #6130, .T. ) ;
#42065=ORIENTED_EDGE ( 'NONE', *, *, #76668, .F. ) ;
#42068=CARTESIAN_POINT ( 'NONE',  ( 96.94826409162261882, -39.14818769109201213, 52.51276813305394597 ) ) ;
#42069=DIRECTION ( 'NONE',  ( -0.7071067811865779928, 0.7071067811865171526, -7.071067811865785947E-16 ) ) ;
#42070=CIRCLE ( 'NONE', #4417, 2.116999999999993776 ) ;
#42071=CARTESIAN_POINT ( 'NONE',  ( 41.56670390244783420, -36.32844715994104234, 249.9678068554150343 ) ) ;
#42072=CARTESIAN_POINT ( 'NONE',  ( 112.5087493249093455, -26.14677957921270846, 165.6984824187679521 ) ) ;
#42073=CARTESIAN_POINT ( 'NONE',  ( 111.3857387752846790, -29.74709210828544670, 289.0581341137911409 ) ) ;
#42074=VERTEX_POINT ( 'NONE', #88358 ) ;
#42076=VERTEX_POINT ( 'NONE', #25658 ) ;
#42077=ORIENTED_EDGE ( 'NONE', *, *, #27021, .T. ) ;
#42078=EDGE_LOOP ( 'NONE', ( #82482, #62908 ) ) ;
#42082=CARTESIAN_POINT ( 'NONE',  ( 97.06102870941442973, -37.99614388472145521, 21.42670149929413626 ) ) ;
#42086=EDGE_CURVE ( 'NONE', #26963, #37193, #45625, .T. ) ;
#42087=DIRECTION ( 'NONE',  ( 1.000000000000000078E-15, -1.000000000000000083E-30, -1.000000000000000000 ) ) ;
#42091=LINE ( 'NONE', #22133, #18723 ) ;
#42092=CARTESIAN_POINT ( 'NONE',  ( 111.4827405772851847, -46.11507286351704238, 287.9146728949591534 ) ) ;
#42094=ORIENTED_EDGE ( 'NONE', *, *, #66274, .F. ) ;
#42095=ADVANCED_FACE ( 'NONE', ( #66994 ), #46972, .T. ) ;
#42097=VECTOR ( 'NONE', #84977, 1000.000000000000000 ) ;
#42098=CARTESIAN_POINT ( 'NONE',  ( 172.5664832912740110, -18.82844715994099971, 196.8086252759119645 ) ) ;
#42099=CARTESIAN_POINT ( 'NONE',  ( 106.7484768184134083, -28.57294068349449034, 82.92523322673494590 ) ) ;
#42101=CARTESIAN_POINT ( 'NONE',  ( 107.0664832912739968, -36.72944715994100306, 287.6356252759109680 ) ) ;
#42103=CIRCLE ( 'NONE', #81312, 9.571100913904395213 ) ;
#42104=CARTESIAN_POINT ( 'NONE',  ( 105.7995184857070541, -26.72403496612070484, 45.17729194272746440 ) ) ;
#42105=ORIENTED_EDGE ( 'NONE', *, *, #84715, .T. ) ;
#42106=ORIENTED_EDGE ( 'NONE', *, *, #57899, .T. ) ;
#42107=CARTESIAN_POINT ( 'NONE',  ( 79.11888855179115865, -34.14703303315388183, 8.087249882927796563 ) ) ;
#42108=ORIENTED_EDGE ( 'NONE', *, *, #87021, .T. ) ;
#42110=CARTESIAN_POINT ( 'NONE',  ( 108.3334481331651347, -46.73485934878011250, 68.67729194561684380 ) ) ;
#42111=CARTESIAN_POINT ( 'NONE',  ( 100.0878889097611335, -31.26788461136058217, 152.2301547344689538 ) ) ;
#42112=CARTESIAN_POINT ( 'NONE',  ( 99.33030919034192152, -39.89585591585919389, 11.13025956287383700 ) ) ;
#42114=CARTESIAN_POINT ( 'NONE',  ( 96.62018903270816850, -36.61901565639288236, 107.3184824187679567 ) ) ;
#42115=CARTESIAN_POINT ( 'NONE',  ( 115.0372574996102344, -42.90846257582342815, 84.30229194168035178 ) ) ;
#42116=ORIENTED_EDGE ( 'NONE', *, *, #14288, .T. ) ;
#42118=ORIENTED_EDGE ( 'NONE', *, *, #87928, .F. ) ;
#42121=CARTESIAN_POINT ( 'NONE',  ( 182.0667039024480118, -32.29483332968430886, 342.9256252759119548 ) ) ;
#42123=CARTESIAN_POINT ( 'NONE',  ( 110.2773916389478188, -46.62487827714380018, 12.82705384733995402 ) ) ;
#42124=CARTESIAN_POINT ( 'NONE',  ( 112.7920458925406422, -45.46759294451666022, 174.0384824187679556 ) ) ;
#42126=DIRECTION ( 'NONE',  ( 1.000000000000000000, 0.000000000000000000, 1.261617073437676668E-15 ) ) ;
#42127=CARTESIAN_POINT ( 'NONE',  ( 112.1200623320449097, -47.44840020502576294, 133.9270538473399768 ) ) ;
#42128=CARTESIAN_POINT ( 'NONE',  ( 82.81648329127399677, -36.72944715994107412, 14.92562527591094579 ) ) ;
#42132=EDGE_CURVE ( 'NONE', #64265, #69742, #5681, .T. ) ;
#42133=ORIENTED_EDGE ( 'NONE', *, *, #48198, .T. ) ;
#42134=VECTOR ( 'NONE', #42704, 1000.000000000000000 ) ;
#42136=LINE ( 'NONE', #15358, #43503 ) ;
#42137=CARTESIAN_POINT ( 'NONE',  ( 109.6119907475197550, -25.15530020966791369, 29.90419670448196854 ) ) ;
#42140=CARTESIAN_POINT ( 'NONE',  ( 116.7962177220229307, -39.38393268333770436, 93.61551088916660035 ) ) ;
#42141=CARTESIAN_POINT ( 'NONE',  ( 114.8626455990942361, -41.33732585285711991, 282.8362293518863453 ) ) ;
#42142=CARTESIAN_POINT ( 'NONE',  ( 97.80809361765332710, -40.50863056222199532, 111.6348687641118715 ) ) ;
#42143=CARTESIAN_POINT ( 'NONE',  ( 96.72090476913471946, -37.82382852467499390, 122.4099109901969626 ) ) ;
#42145=DIRECTION ( 'NONE',  ( -1.000000000000000078E-15, 1.000000000000000083E-30, 1.000000000000000000 ) ) ;
#42148=DIRECTION ( 'NONE',  ( -1.000000000000000000, 0.000000000000000000, 0.000000000000000000 ) ) ;
#42151=VERTEX_POINT ( 'NONE', #11598 ) ;
#42153=CARTESIAN_POINT ( 'NONE',  ( 102.9497400982657069, -26.42094052169726837, 175.3908633711489813 ) ) ;
#42154=ORIENTED_EDGE ( 'NONE', *, *, #31459, .F. ) ;
#42156=CARTESIAN_POINT ( 'NONE',  ( 99.73785018541691727, -29.28442226721861275, 221.6956252759109702 ) ) ;
#42157=CARTESIAN_POINT ( 'NONE',  ( 114.3835678416600672, -44.21631923246377482, 69.19276813305397411 ) ) ;
#42160=CYLINDRICAL_SURFACE ( 'NONE', #1750, 2.116999999999993776 ) ;
#42161=ORIENTED_EDGE ( 'NONE', *, *, #11843, .T. ) ;
#42164=VERTEX_POINT ( 'NONE', #73360 ) ;
#42169=CARTESIAN_POINT ( 'NONE',  ( 141.8164832912740394, -36.72944715994099596, -4.824374724088994704 ) ) ;
#42170=CARTESIAN_POINT ( 'NONE',  ( 117.4906655440605334, -35.85895469176247019, 249.8927681330537780 ) ) ;
#42172=CARTESIAN_POINT ( 'NONE',  ( 136.8004280042375456, -18.38432671278184927, 3.076561810304713873 ) ) ;
#42173=LINE ( 'NONE', #854, #30831 ) ;
#42176=VECTOR ( 'NONE', #15589, 1000.000000000000000 ) ;
#42177=CARTESIAN_POINT ( 'NONE',  ( 116.7476796835742192, -31.34707987858772427, 29.24229194257799236 ) ) ;
#42179=ORIENTED_EDGE ( 'NONE', *, *, #28883, .F. ) ;
#42180=AXIS2_PLACEMENT_3D ( 'NONE', #25937, #80462, #67716 ) ;
#42182=CARTESIAN_POINT ( 'NONE',  ( 105.2318265017784000, -27.12228994480481248, 231.2270538473389649 ) ) ;
#42183=EDGE_CURVE ( 'NONE', #74787, #50559, #56313, .T. ) ;
#42184=B_SPLINE_CURVE_WITH_KNOTS ( 'NONE', 3,
 ( #83501, #63045, #15368, #63955, #22185, #84861, #43033, #43484, #63497, #21272, #56210, #28987, #56673, #78043, #84417, #29435, #48945, #8547 ),
 .UNSPECIFIED., .F., .F.,
 ( 4, 2, 2, 2, 2, 2, 2, 2, 4 ),
 ( 0.4999999997859982392, 0.5624999998127484524, 0.6249999998394986100, 0.6874999998662488787, 0.7499999998929991474, 0.8124999999197493050, 0.8749999999464994627, 0.9374999999732497313, 1.000000000000000000 ),
 .UNSPECIFIED. ) ;
#42186=CARTESIAN_POINT ( 'NONE',  ( 97.30000116515917341, -37.25789978020652171, 72.36991099019596163 ) ) ;
#42187=EDGE_CURVE ( 'NONE', #11825, #76939, #46122, .T. ) ;
#42188=CARTESIAN_POINT ( 'NONE',  ( 107.0664832912739968, -36.72944715994100306, 287.6356252759109680 ) ) ;
#42190=CARTESIAN_POINT ( 'NONE',  ( 97.07203280649774513, -35.37881615147394854, 22.21891955711141264 ) ) ;
#42191=AXIS2_PLACEMENT_3D ( 'NONE', #66645, #72587, #86661 ) ;
#42192=ORIENTED_EDGE ( 'NONE', *, *, #77186, .F. ) ;
#42194=ADVANCED_FACE ( 'NONE', ( #84232 ), #15173, .F. ) ;
#42195=EDGE_LOOP ( 'NONE', ( #17746, #79364, #88310, #80870 ) ) ;
#42198=CARTESIAN_POINT ( 'NONE',  ( 102.1597156073931671, -27.93204209654597037, 251.9130118773254026 ) ) ;
#42200=LINE ( 'NONE', #84013, #83543 ) ;
#42201=CARTESIAN_POINT ( 'NONE',  ( 112.1389085449243765, -28.01257236761306402, 139.6564983914183813 ) ) ;
#42202=CARTESIAN_POINT ( 'NONE',  ( 48.45959712129000252, -28.98061976758940617, 342.9256252759119548 ) ) ;
#42206=EDGE_LOOP ( 'NONE', ( #13592, #23315 ) ) ;
#42209=ORIENTED_EDGE ( 'NONE', *, *, #48971, .T. ) ;
#42210=CARTESIAN_POINT ( 'NONE',  ( 105.4209491665783105, -47.02406944081578644, 37.44991099019695469 ) ) ;
#42211=ORIENTED_EDGE ( 'NONE', *, *, #10720, .T. ) ;
#42212=CARTESIAN_POINT ( 'NONE',  ( 111.2046685188893775, -28.67413054290084062, 19.13337220902994318 ) ) ;
#42215=CARTESIAN_POINT ( 'NONE',  ( 113.6884830475839152, -29.53135334845044468, 199.4841967044829687 ) ) ;
#42216=CARTESIAN_POINT ( 'NONE',  ( 20.03715912545735378, -24.42818131006189830, 249.9678068554150059 ) ) ;
#42217=DIRECTION ( 'NONE',  ( 0.000000000000000000, 1.000000000000000000, 0.000000000000000000 ) ) ;
#42218=DIRECTION ( 'NONE',  ( 0.000000000000000000, 0.000000000000000000, -1.000000000000000000 ) ) ;
#42220=CARTESIAN_POINT ( 'NONE',  ( 97.46669833601751520, -32.60829619471579122, 12.00419670448293985 ) ) ;
#42223=DIRECTION ( 'NONE',  ( -1.000000000000000078E-15, 1.000000000000000083E-30, 1.000000000000000000 ) ) ;
#42224=VERTEX_POINT ( 'NONE', #55126 ) ;
#42225=CARTESIAN_POINT ( 'NONE',  ( 114.0153296496652615, -28.07433117884028206, 115.5261014663869474 ) ) ;
#42227=ORIENTED_EDGE ( 'NONE', *, *, #89737, .F. ) ;
#42231=AXIS2_PLACEMENT_3D ( 'NONE', #58166, #2773, #44074 ) ;
#42232=CARTESIAN_POINT ( 'NONE',  ( 104.4081005327850846, -46.45808910606737641, 122.3647919321082327 ) ) ;
#42235=DIRECTION ( 'NONE',  ( -4.299999999999999979E-14, 1.000000000000000000, -4.400000000000000367E-29 ) ) ;
#42236=DIRECTION ( 'NONE',  ( 1.000000000000000000, 0.000000000000000000, 0.000000000000000000 ) ) ;
#42237=CARTESIAN_POINT ( 'NONE',  ( 99.51751092519847930, -40.96193357599213414, 179.5633284648289703 ) ) ;
#42238=CARTESIAN_POINT ( 'NONE',  ( 99.36548562555644537, -29.67027625815665104, 271.7356252759109907 ) ) ;
#42241=CARTESIAN_POINT ( 'NONE',  ( 126.8164832912740394, -54.62589567669621005, -5.074374724089010691 ) ) ;
#42243=CIRCLE ( 'NONE', #42300, 2.500000000000002220 ) ;
#42244=EDGE_CURVE ( 'NONE', #41711, #47853, #49220, .T. ) ;
#42245=ORIENTED_EDGE ( 'NONE', *, *, #2580, .T. ) ;
#42246=ORIENTED_EDGE ( 'NONE', *, *, #13085, .T. ) ;
#42247=CARTESIAN_POINT ( 'NONE',  ( 81.91406418436724834, -20.77438500682750799, 2.186796636973903141 ) ) ;
#42248=DIRECTION ( 'NONE',  ( -0.04216478779797398074, 0.9991106698809455455, 0.000000000000000000 ) ) ;
#42249=CARTESIAN_POINT ( 'NONE',  ( 97.07205744801414937, -35.37854429503371989, 16.21896654171250773 ) ) ;
#42250=EDGE_CURVE ( 'NONE', #82044, #18839, #21548, .T. ) ;
#42253=CARTESIAN_POINT ( 'NONE',  ( 99.94932728663779642, -31.12955780999732980, 200.2305150661719892 ) ) ;
#42254=CARTESIAN_POINT ( 'NONE',  ( 115.2011789175540741, -43.31984874952732412, 88.28419670448195689 ) ) ;
#42255=ORIENTED_EDGE ( 'NONE', *, *, #21768, .F. ) ;
#42259=EDGE_LOOP ( 'NONE', ( #24012, #84536, #23284, #4084, #12044 ) ) ;
#42262=EDGE_LOOP ( 'NONE', ( #51717, #30087, #37100, #48905 ) ) ;
#42264=FACE_OUTER_BOUND ( 'NONE', #72974, .T. ) ;
#42266=VECTOR ( 'NONE', #58370, 1000.000000000000000 ) ;
#42268=ORIENTED_EDGE ( 'NONE', *, *, #52800, .F. ) ;
#42269=EDGE_CURVE ( 'NONE', #16654, #44045, #195, .T. ) ;
#42270=CARTESIAN_POINT ( 'NONE',  ( 101.0534108623914591, -27.42684531413746285, 70.54514908543497143 ) ) ;
#42274=CARTESIAN_POINT ( 'NONE',  ( 131.5238707403503327, -17.68172011937277333, 2.822018711113663425 ) ) ;
#42275=EDGE_LOOP ( 'NONE', ( #39385, #87116, #33925, #3132 ) ) ;
#42276=LINE ( 'NONE', #50439, #2493 ) ;
#42277=DIRECTION ( 'NONE',  ( 0.000000000000000000, 0.000000000000000000, 1.000000000000000000 ) ) ;
#42280=CARTESIAN_POINT ( 'NONE',  ( 114.7420861883949215, -43.81622209775510157, 119.2327681330539804 ) ) ;
#42281=DIRECTION ( 'NONE',  ( -0.7071067811865476838, -0.7071067811865473507, 0.000000000000000000 ) ) ;
#42282=FACE_OUTER_BOUND ( 'NONE', #87900, .T. ) ;
#42286=CARTESIAN_POINT ( 'NONE',  ( 98.54774150848832903, -41.53511815344519675, 132.7356252759109623 ) ) ;
#42287=CARTESIAN_POINT ( 'NONE',  ( 131.0667039024480403, -51.22944715994093201, 231.5838068554170093 ) ) ;
#42290=CARTESIAN_POINT ( 'NONE',  ( 111.8540205700168713, -46.00543295620330753, 268.9556252759110180 ) ) ;
#42291=DIRECTION ( 'NONE',  ( -4.237773401492740281E-14, 1.000000000000000000, 0.000000000000000000 ) ) ;
#42292=CARTESIAN_POINT ( 'NONE',  ( 150.5667039024473297, -25.42844715993594562, 300.4678068554149490 ) ) ;
#42293=CARTESIAN_POINT ( 'NONE',  ( 107.0664832912739968, 22.62155284005901024, 333.4006252759110112 ) ) ;
#42294=EDGE_CURVE ( 'NONE', #79790, #65097, #20649, .T. ) ;
#42296=CARTESIAN_POINT ( 'NONE',  ( 34.27482367531460028, -30.08671355700332839, 237.4678068554150059 ) ) ;
#42298=CARTESIAN_POINT ( 'NONE',  ( 106.9806506443342755, -46.50983917909375265, 187.5699109901969734 ) ) ;
#42300=AXIS2_PLACEMENT_3D ( 'NONE', #17271, #39035, #32671 ) ;
#42302=CARTESIAN_POINT ( 'NONE',  ( 103.5362709388849254, -28.56900242483978047, 151.8330118773259585 ) ) ;
#42303=AXIS2_PLACEMENT_3D ( 'NONE', #3827, #52383, #51075 ) ;
#42304=DIRECTION ( 'NONE',  ( 1.000000000000000000, 4.163336342344347755E-14, 0.000000000000000000 ) ) ;
#42305=CARTESIAN_POINT ( 'NONE',  ( 102.4274648318396146, -45.67098835673295554, 13.62729759161196341 ) ) ;
#42306=DIRECTION ( 'NONE',  ( -1.000000000000000078E-15, 0.000000000000000000, -1.000000000000000000 ) ) ;
#42307=CYLINDRICAL_SURFACE ( 'NONE', #89584, 0.9999999999992039701 ) ;
#42308=EDGE_CURVE ( 'NONE', #1932, #61346, #41956, .T. ) ;
#42310=DIRECTION ( 'NONE',  ( 0.000000000000000000, 1.000000000000000000, 1.914177628664063178E-15 ) ) ;
#42311=DIRECTION ( 'NONE',  ( 0.000000000000000000, 1.000000000000000000, 0.000000000000000000 ) ) ;
#42313=CARTESIAN_POINT ( 'NONE',  ( 116.8369567342160451, -40.30247308064095790, 218.5470538473399529 ) ) ;
#42314=DIRECTION ( 'NONE',  ( 0.000000000000000000, 0.000000000000000000, -1.000000000000000000 ) ) ;
#42317=VECTOR ( 'NONE', #40856, 1000.000000000000000 ) ;
#42320=DIRECTION ( 'NONE',  ( -1.000000000000000078E-15, 1.000000000000000083E-30, 1.000000000000000000 ) ) ;
#42323=DIRECTION ( 'NONE',  ( 0.7071067811865171526, 0.7071067811865779928, 7.071067811865164719E-16 ) ) ;
#42324=EDGE_LOOP ( 'NONE', ( #58946, #77905 ) ) ;
#42325=CARTESIAN_POINT ( 'NONE',  ( 115.9822161205003397, -42.21601869724081268, 14.38705384733995984 ) ) ;
#42326=CARTESIAN_POINT ( 'NONE',  ( 118.0409265538620787, -35.41009787725452185, 238.9337205140059552 ) ) ;
#42327=ORIENTED_EDGE ( 'NONE', *, *, #50979, .T. ) ;
#42328=VECTOR ( 'NONE', #33109, 999.9999999999998863 ) ;
#42330=PLANE ( 'NONE',  #23959 ) ;
#42331=CARTESIAN_POINT ( 'NONE',  ( 117.0504484085820707, -35.92752602142036267, 168.8902974104038890 ) ) ;
#42332=AXIS2_PLACEMENT_3D ( 'NONE', #23755, #37369, #2857 ) ;
#42333=CARTESIAN_POINT ( 'NONE',  ( 102.3683448235669715, -29.46113098739592928, 68.36332846482901004 ) ) ;
#42334=CARTESIAN_POINT ( 'NONE',  ( 109.4502800619034417, -25.91266766229690433, 175.8918157521009391 ) ) ;
#42335=CARTESIAN_POINT ( 'NONE',  ( 41.56648329127399677, -9.303447159940999356, 138.9256252759119832 ) ) ;
#42336=ORIENTED_EDGE ( 'NONE', *, *, #21954, .F. ) ;
#42339=VERTEX_POINT ( 'NONE', #22441 ) ;
#42340=VERTEX_POINT ( 'NONE', #71928 ) ;
#42342=VERTEX_POINT ( 'NONE', #64222 ) ;
#42344=CARTESIAN_POINT ( 'NONE',  ( 115.7842719947117160, -41.80033795913374206, 169.4071411100227920 ) ) ;
#42345=ADVANCED_FACE ( 'NONE', ( #29693, #86457 ), #30586, .F. ) ;
#42346=CARTESIAN_POINT ( 'NONE',  ( 107.7585303169594511, -25.29108704099150629, 321.0964939388218227 ) ) ;
#42347=CARTESIAN_POINT ( 'NONE',  ( 108.6385355886969108, -45.12496878139073431, 82.14670554236298017 ) ) ;
#42348=CARTESIAN_POINT ( 'NONE',  ( 105.1048729065459355, -25.82772592887830854, 275.2061014663870537 ) ) ;
#42349=CARTESIAN_POINT ( 'NONE',  ( 97.78191787992076911, -41.50032452247409509, 196.7041967044819728 ) ) ;
#42350=LINE ( 'NONE', #34659, #64396 ) ;
#42351=CARTESIAN_POINT ( 'NONE',  ( 101.9927051845395169, -45.44550660328174985, 93.15637402092625052 ) ) ;
#42352=ORIENTED_EDGE ( 'NONE', *, *, #11373, .T. ) ;
#42353=CARTESIAN_POINT ( 'NONE',  ( 97.80889870804310249, -40.51851473143300097, 41.63518016758125384 ) ) ;
#42354=AXIS2_PLACEMENT_3D ( 'NONE', #29006, #29903, #57589 ) ;
#42355=DIRECTION ( 'NONE',  ( 1.907762142705490052E-15, 7.167082501179359715E-16, -1.000000000000000000 ) ) ;
#42358=CARTESIAN_POINT ( 'NONE',  ( 107.3174176841070846, -26.95189801805063823, 120.0556252759109555 ) ) ;
#42359=CARTESIAN_POINT ( 'NONE',  ( 96.87811797401508329, -32.32375813437732859, 61.01372051400599616 ) ) ;
#42360=CARTESIAN_POINT ( 'NONE',  ( 96.22219577434788107, -34.35999324012363587, 256.1432443235299843 ) ) ;
#42361=ORIENTED_EDGE ( 'NONE', *, *, #14103, .F. ) ;
#42362=EDGE_CURVE ( 'NONE', #4781, #43151, #10144, .T. ) ;
#42363=CARTESIAN_POINT ( 'NONE',  ( 106.8516092256838306, -47.78082339050276772, 227.5489586092439538 ) ) ;
#42364=CARTESIAN_POINT ( 'NONE',  ( 116.3212776292294279, -32.94146857471271517, 75.13562527591093954 ) ) ;
#42367=DIRECTION ( 'NONE',  ( -4.299999999999999979E-14, 1.000000000000000000, -4.400000000000000367E-29 ) ) ;
#42369=DIRECTION ( 'NONE',  ( 1.000000000000000000, 4.299999999999999979E-14, 1.000000000000000078E-15 ) ) ;
#42370=CARTESIAN_POINT ( 'NONE',  ( 180.3503142329310265, -29.99615139349890569, 117.4678068554150627 ) ) ;
#42372=LINE ( 'NONE', #84201, #48410 ) ;
#42375=CARTESIAN_POINT ( 'NONE',  ( 105.7995184592378024, -26.72403496912623666, 11.17729194477459842 ) ) ;
#42378=CIRCLE ( 'NONE', #52475, 2.999999999999947153 ) ;
#42379=CARTESIAN_POINT ( 'NONE',  ( 112.1393456339030337, -28.01282277639932161, 259.6564586099611915 ) ) ;
#42381=EDGE_CURVE ( 'NONE', #41907, #23638, #14328, .T. ) ;
#42382=FACE_OUTER_BOUND ( 'NONE', #16009, .T. ) ;
#42383=CARTESIAN_POINT ( 'NONE',  ( 111.6181759772156994, -46.13308781976898842, 247.9356252759109509 ) ) ;
#42384=CARTESIAN_POINT ( 'NONE',  ( 108.6487146914112287, -25.79677769486274386, 145.9737205140069420 ) ) ;
#42385=CARTESIAN_POINT ( 'NONE',  ( 96.66430309996448500, -42.45805065352005414, 22.72705384733997391 ) ) ;
#42386=LINE ( 'NONE', #84215, #64968 ) ;
#42387=CARTESIAN_POINT ( 'NONE',  ( 49.21213752016101495, -29.73316016639650172, -5.074374724088000832 ) ) ;
#42388=CARTESIAN_POINT ( 'NONE',  ( 46.32460016641721978, -48.34074026909785005, 300.4678068554150059 ) ) ;
#42391=VECTOR ( 'NONE', #74880, 1000.000000000000000 ) ;
#42392=ADVANCED_FACE ( 'NONE', ( #43758, #22895 ), #57838, .F. ) ;
#42393=ORIENTED_EDGE ( 'NONE', *, *, #84378, .F. ) ;
#42394=CARTESIAN_POINT ( 'NONE',  ( 116.3212776292296127, -32.94146857471318413, 10.13562527591094309 ) ) ;
#42395=ORIENTED_EDGE ( 'NONE', *, *, #72322, .T. ) ;
#42397=CARTESIAN_POINT ( 'NONE',  ( 105.9636396274569137, -27.08297541922676643, 159.5895626852199598 ) ) ;
#42398=CARTESIAN_POINT ( 'NONE',  ( 33.91903122894480305, -35.91149509761181235, 237.4678068554150059 ) ) ;
#42401=CARTESIAN_POINT ( 'NONE',  ( 117.0023065291008066, -39.93004192841230804, 154.5784824187679476 ) ) ;
#42402=CARTESIAN_POINT ( 'NONE',  ( 120.0056275895821898, -31.38355669832866468, 290.1356252759106837 ) ) ;
#42404=ADVANCED_FACE ( 'NONE', ( #37852, #58716 ), #78313, .T. ) ;
#42405=CARTESIAN_POINT ( 'NONE',  ( 115.6778355879448981, -31.59694472422848577, 85.25382685634609459 ) ) ;
#42408=CARTESIAN_POINT ( 'NONE',  ( 96.71749658230658042, -40.79275330125902599, 96.62419670448296927 ) ) ;
#42409=EDGE_LOOP ( 'NONE', ( #89359, #87854, #86808, #65631 ) ) ;
#42412=CARTESIAN_POINT ( 'NONE',  ( 104.4236822747140678, -45.74566190472552307, 58.76920235351595778 ) ) ;
#42413=CARTESIAN_POINT ( 'NONE',  ( 188.5667039024479834, -67.87844715994100397, 178.0928068554149775 ) ) ;
#42414=CARTESIAN_POINT ( 'NONE',  ( 110.4719531740380063, -47.31314961125941210, 203.8241967044819489 ) ) ;
#42415=CARTESIAN_POINT ( 'NONE',  ( 135.3756687995053483, -12.91806617559082504, 394.9756252759104314 ) ) ;
#42416=DIRECTION ( 'NONE',  ( 1.000000000000000000, 0.000000000000000000, 9.462128050782575008E-16 ) ) ;
#42418=LINE ( 'NONE', #56503, #47470 ) ;
#42419=ADVANCED_FACE ( 'NONE', ( #29254 ), #23352, .T. ) ;
#42420=AXIS2_PLACEMENT_3D ( 'NONE', #34472, #48521, #7674 ) ;
#42423=ADVANCED_FACE ( 'NONE', ( #75050 ), #19631, .T. ) ;
#42424=CARTESIAN_POINT ( 'NONE',  ( 107.9437834512411598, -25.73425880284244016, 115.0251490854349612 ) ) ;
#42425=ORIENTED_EDGE ( 'NONE', *, *, #25475, .F. ) ;
#42427=ORIENTED_EDGE ( 'NONE', *, *, #19389, .T. ) ;
#42431=EDGE_CURVE ( 'NONE', #26572, #49295, #15826, .T. ) ;
#42432=DIRECTION ( 'NONE',  ( 1.000000000000000000, 4.299999999999999979E-14, 1.000000000000000078E-15 ) ) ;
#42434=CARTESIAN_POINT ( 'NONE',  ( 102.6333607924234883, -43.61639954521550067, 219.9395189410199691 ) ) ;
#42436=DIRECTION ( 'NONE',  ( 1.000000000000000078E-15, -1.000000000000000083E-30, -1.000000000000000000 ) ) ;
#42440=CARTESIAN_POINT ( 'NONE',  ( 116.4818944900138149, -33.33401923526724175, 65.10204591046331757 ) ) ;
#42442=ORIENTED_EDGE ( 'NONE', *, *, #73346, .T. ) ;
#42443=CARTESIAN_POINT ( 'NONE',  ( 78.76282073105750214, -21.15113447711886963, 7.957506268074834743 ) ) ;
#42444=CIRCLE ( 'NONE', #48209, 0.5000000000000004441 ) ;
#42445=CARTESIAN_POINT ( 'NONE',  ( 116.9161372654479578, -38.84013935494854763, 255.0901547344684559 ) ) ;
#42447=ORIENTED_EDGE ( 'NONE', *, *, #44609, .F. ) ;
#42450=VERTEX_POINT ( 'NONE', #67781 ) ;
#42454=ORIENTED_EDGE ( 'NONE', *, *, #74212, .F. ) ;
#42455=VERTEX_POINT ( 'NONE', #67323 ) ;
#42456=CIRCLE ( 'NONE', #14939, 3.000000000000002665 ) ;
#42457=CARTESIAN_POINT ( 'NONE',  ( 97.79975852078015919, -37.20246216128834504, 269.1852332267342831 ) ) ;
#42458=CARTESIAN_POINT ( 'NONE',  ( 97.77451808712464754, -42.75935979880518545, 146.7965776568629508 ) ) ;
#42459=CARTESIAN_POINT ( 'NONE',  ( 101.5125196766230289, -27.93273449574867229, 110.5241967044819944 ) ) ;
#42460=LINE ( 'NONE', #692, #82037 ) ;
#42461=CARTESIAN_POINT ( 'NONE',  ( 164.9667039024459996, -26.71338133339301635, -5.074374724088000832 ) ) ;
#42462=CARTESIAN_POINT ( 'NONE',  ( 115.2517161551258766, -30.21613035964762517, 240.3613395616249875 ) ) ;
#42463=CARTESIAN_POINT ( 'NONE',  ( 48.85858412958059205, -30.08671355700274574, 237.4678068554150059 ) ) ;
#42464=CARTESIAN_POINT ( 'NONE',  ( 80.06648329127401098, -41.22944715994105280, 10.42562527591094401 ) ) ;
#42465=ORIENTED_EDGE ( 'NONE', *, *, #18820, .F. ) ;
#42467=ORIENTED_EDGE ( 'NONE', *, *, #63237, .F. ) ;
#42469=LINE ( 'NONE', #68855, #64887 ) ;
#42470=CARTESIAN_POINT ( 'NONE',  ( 37.06648329127400388, 12.92155284005802685, 336.5756252759108520 ) ) ;
#42471=EDGE_LOOP ( 'NONE', ( #16399, #9364, #83586, #31361 ) ) ;
#42473=CARTESIAN_POINT ( 'NONE',  ( 105.3162203493976676, -48.44985994433862686, 147.4584824187679715 ) ) ;
#42474=FACE_OUTER_BOUND ( 'NONE', #72517, .T. ) ;
#42475=CARTESIAN_POINT ( 'NONE',  ( 136.1531896714324148, -34.93816060012501623, 7.482180659744297024 ) ) ;
#42476=DIRECTION ( 'NONE',  ( 2.900000000000000265E-14, -2.000000000000000155E-15, 1.000000000000000000 ) ) ;
#42479=CARTESIAN_POINT ( 'NONE',  ( 117.0188616982925396, -35.22807495305379888, 58.94555671601543168 ) ) ;
#42480=CARTESIAN_POINT ( 'NONE',  ( 115.3062145713271747, -45.21207857638179917, 264.1899109901965517 ) ) ;
#42481=DIRECTION ( 'NONE',  ( -0.7071067811865774377, 0.7071067811865175967, -7.071067811865470403E-16 ) ) ;
#42484=EDGE_CURVE ( 'NONE', #72034, #30378, #14022, .T. ) ;
#42486=DIRECTION ( 'NONE',  ( 0.000000000000000000, 0.000000000000000000, 1.000000000000000000 ) ) ;
#42487=CARTESIAN_POINT ( 'NONE',  ( 112.0659116373989121, -45.48839625182279889, 258.9897919439433167 ) ) ;
#42488=EDGE_CURVE ( 'NONE', #12869, #68689, #5570, .T. ) ;
#42489=FACE_OUTER_BOUND ( 'NONE', #44438, .T. ) ;
#42490=CARTESIAN_POINT ( 'NONE',  ( 111.8844023637430638, -46.06429852124467317, 272.9556252759110180 ) ) ;
#42491=VERTEX_POINT ( 'NONE', #80529 ) ;
#42492=EDGE_CURVE ( 'NONE', #24816, #43944, #54122, .T. ) ;
#42493=FACE_OUTER_BOUND ( 'NONE', #51249, .T. ) ;
#42494=CARTESIAN_POINT ( 'NONE',  ( 108.3688725116650602, -47.72941199507204146, 162.6822919425769669 ) ) ;
#42495=CARTESIAN_POINT ( 'NONE',  ( 110.3719271596222882, -47.27686491584164941, 48.80610146638797175 ) ) ;
#42496=CARTESIAN_POINT ( 'NONE',  ( 97.01638781908712872, -41.44040028630095662, 207.6632443235299661 ) ) ;
#42497=FACE_OUTER_BOUND ( 'NONE', #41101, .T. ) ;
#42498=FACE_OUTER_BOUND ( 'NONE', #62307, .T. ) ;
#42501=CARTESIAN_POINT ( 'NONE',  ( 97.81169150544869240, -40.51741169384158781, 71.63577594787710723 ) ) ;
#42503=ORIENTED_EDGE ( 'NONE', *, *, #12666, .T. ) ;
#42505=VECTOR ( 'NONE', #61961, 1000.000000000000000 ) ;
#42506=DIRECTION ( 'NONE',  ( -1.000000000000000078E-15, 1.000000000000000083E-30, 1.000000000000000000 ) ) ;
#42507=EDGE_CURVE ( 'NONE', #84121, #63446, #72360, .T. ) ;
#42508=ORIENTED_EDGE ( 'NONE', *, *, #10297, .T. ) ;
#42509=ORIENTED_EDGE ( 'NONE', *, *, #70299, .F. ) ;
#42512=CARTESIAN_POINT ( 'NONE',  ( 101.1533894386775501, -27.41820966596962705, 61.51467289495899138 ) ) ;
#42513=CARTESIAN_POINT ( 'NONE',  ( 180.3503142329310265, -29.99615139349890569, -5.074374724088000832 ) ) ;
#42514=EDGE_CURVE ( 'NONE', #23923, #52978, #59301, .T. ) ;
#42516=CARTESIAN_POINT ( 'NONE',  ( 117.3342495501102007, -34.51337161069084658, 179.9956252759109532 ) ) ;
#42517=CARTESIAN_POINT ( 'NONE',  ( 100.7304913082922440, -30.25890808522221320, 270.1276579233149278 ) ) ;
#42520=ORIENTED_EDGE ( 'NONE', *, *, #76042, .T. ) ;
#42522=ORIENTED_EDGE ( 'NONE', *, *, #33467, .F. ) ;
#42523=CARTESIAN_POINT ( 'NONE',  ( 71.24189083761805819, -0.9290567490904538817, 361.9756252759101471 ) ) ;
#42524=CARTESIAN_POINT ( 'NONE',  ( 123.6837132603320413, -23.41243780205712710, 249.5838068554165261 ) ) ;
#42527=DIRECTION ( 'NONE',  ( 0.000000000000000000, 1.000000000000000000, 0.000000000000000000 ) ) ;
#42528=LINE ( 'NONE', #85257, #6968 ) ;
#42529=LINE ( 'NONE', #83441, #58162 ) ;
#42531=LINE ( 'NONE', #7590, #84032 ) ;
#42532=CARTESIAN_POINT ( 'NONE',  ( 102.6689224787387502, -46.93780143634764812, 287.2527681330543601 ) ) ;
#42536=CARTESIAN_POINT ( 'NONE',  ( 115.8254324148542622, -31.73001888479201682, 269.2397919377605717 ) ) ;
#42538=DIRECTION ( 'NONE',  ( 4.194175870806139918E-14, -1.000000000000000000, 0.000000000000000000 ) ) ;
#42539=CARTESIAN_POINT ( 'NONE',  ( 112.0375358597863027, -29.64498801284190321, 82.39570941720997155 ) ) ;
#42542=DIRECTION ( 'NONE',  ( 0.7071067811865969777, -0.7071067811864980568, 0.000000000000000000 ) ) ;
#42543=ORIENTED_EDGE ( 'NONE', *, *, #26453, .T. ) ;
#42544=VERTEX_POINT ( 'NONE', #527 ) ;
#42545=CARTESIAN_POINT ( 'NONE',  ( 117.0609687849609770, -38.07993266210836225, 138.7175048411430396 ) ) ;
#42546=AXIS2_PLACEMENT_3D ( 'NONE', #52320, #45516, #38721 ) ;
#42548=ORIENTED_EDGE ( 'NONE', *, *, #2040, .T. ) ;
#42549=CARTESIAN_POINT ( 'NONE',  ( 116.1082436049511415, -39.28347229878176705, 140.0511071154209617 ) ) ;
#42551=CARTESIAN_POINT ( 'NONE',  ( 106.6594888599963298, -26.29050016388675104, 81.10705384733896040 ) ) ;
#42553=EDGE_LOOP ( 'NONE', ( #47938, #41355 ) ) ;
#42554=VERTEX_POINT ( 'NONE', #13718 ) ;
#42556=CARTESIAN_POINT ( 'NONE',  ( 41.56648329127499153, -27.82844715994070484, 143.6756252759119832 ) ) ;
#42558=CARTESIAN_POINT ( 'NONE',  ( 111.4827405772851847, -46.11507286351704238, 287.9146728949591534 ) ) ;
#42559=CARTESIAN_POINT ( 'NONE',  ( 112.4974222397575545, -26.16880547358812947, 165.6984824187679521 ) ) ;
#42561=CARTESIAN_POINT ( 'NONE',  ( 134.0664832912739826, -36.72944715994100306, 14.92562527591099908 ) ) ;
#42562=CARTESIAN_POINT ( 'NONE',  ( 102.6161641507259219, -46.84718603934155823, 128.2346728949589760 ) ) ;
#42563=DIRECTION ( 'NONE',  ( 0.000000000000000000, 0.000000000000000000, -1.000000000000000000 ) ) ;
#42564=VERTEX_POINT ( 'NONE', #14168 ) ;
#42566=ORIENTED_EDGE ( 'NONE', *, *, #67788, .T. ) ;
#42567=DIRECTION ( 'NONE',  ( 0.000000000000000000, 0.000000000000000000, 1.000000000000000000 ) ) ;
#42568=EDGE_CURVE ( 'NONE', #14045, #311, #70943, .T. ) ;
#42572=CARTESIAN_POINT ( 'NONE',  ( 194.5664832912739826, 25.62155284005901379, 323.8756252759109202 ) ) ;
#42573=CARTESIAN_POINT ( 'NONE',  ( 106.2521265061568130, -26.30051002661620885, 25.13848241876792855 ) ) ;
#42578=CARTESIAN_POINT ( 'NONE',  ( 117.0718954850937052, -35.46248235514278235, 74.92729194266681247 ) ) ;
#42580=CARTESIAN_POINT ( 'NONE',  ( 102.1671273105904447, -43.72604531649727733, 281.5124198280768155 ) ) ;
#42581=CARTESIAN_POINT ( 'NONE',  ( 108.4172477039653586, -26.73499932200780549, 109.9689778000439730 ) ) ;
#42582=CARTESIAN_POINT ( 'NONE',  ( 112.1095002620001253, -47.42599740258504681, 133.9270538473399768 ) ) ;
#42584=LINE ( 'NONE', #28989, #13309 ) ;
#42585=ORIENTED_EDGE ( 'NONE', *, *, #73671, .F. ) ;
#42586=CARTESIAN_POINT ( 'NONE',  ( 62.03742497533659872, -23.42844715994041493, 129.9678068554150911 ) ) ;
#42587=EDGE_CURVE ( 'NONE', #15894, #25446, #82332, .T. ) ;
#42589=DIRECTION ( 'NONE',  ( 0.000000000000000000, 0.000000000000000000, -1.000000000000000000 ) ) ;
#42590=VERTEX_POINT ( 'NONE', #47766 ) ;
#42592=CARTESIAN_POINT ( 'NONE',  ( 138.8545562996768012, -1.932463243632620342, 394.9756252759100903 ) ) ;
#42593=CARTESIAN_POINT ( 'NONE',  ( 116.8478532179160680, -43.50835558345241338, 163.3441967044829823 ) ) ;
#42595=DIRECTION ( 'NONE',  ( 0.0001484127182338930157, -0.8660253910675250744, 0.5000000000000052180 ) ) ;
#42596=CARTESIAN_POINT ( 'NONE',  ( 108.1840971438632550, -47.11637154254925974, 198.6613395616249989 ) ) ;
#42597=CARTESIAN_POINT ( 'NONE',  ( 117.4143231396408851, -32.71451144048268844, 90.10895860924395606 ) ) ;
#42599=CARTESIAN_POINT ( 'NONE',  ( 109.7223420879504943, -27.00013639330362381, 190.8647559210611178 ) ) ;
#42600=CARTESIAN_POINT ( 'NONE',  ( 116.8171228662985470, -34.15291832007721951, 79.03145860929339506 ) ) ;
#42601=ORIENTED_EDGE ( 'NONE', *, *, #18189, .F. ) ;
#42603=AXIS2_PLACEMENT_3D ( 'NONE', #30388, #63563, #9494 ) ;
#42605=CIRCLE ( 'NONE', #3462, 2.550000000000006040 ) ;
#42607=EDGE_CURVE ( 'NONE', #31400, #45771, #83978, .T. ) ;
#42608=ORIENTED_EDGE ( 'NONE', *, *, #71469, .T. ) ;
#42609=VECTOR ( 'NONE', #57957, 1000.000000000000000 ) ;
#42610=ORIENTED_EDGE ( 'NONE', *, *, #89297, .T. ) ;
#42612=CARTESIAN_POINT ( 'NONE',  ( 111.6084932380418735, -46.11308361340533679, 243.9356252759109509 ) ) ;
#42614=CARTESIAN_POINT ( 'NONE',  ( 136.7325000480764743, -18.03188439720356939, 2.979900720422836269 ) ) ;
#42617=LINE ( 'NONE', #76716, #736 ) ;
#42618=DIRECTION ( 'NONE',  ( 1.000000000000000000, 1.000000000000000078E-15, 1.000000000000000078E-15 ) ) ;
#42619=CARTESIAN_POINT ( 'NONE',  ( 118.2322726120735155, -40.77409347166903331, 23.54991099019593292 ) ) ;
#42622=DIRECTION ( 'NONE',  ( 0.000000000000000000, 0.000000000000000000, -1.000000000000000000 ) ) ;
#42623=CARTESIAN_POINT ( 'NONE',  ( 97.39126582715591951, -39.27842219038148386, 17.53169798143252223 ) ) ;
#42624=CARTESIAN_POINT ( 'NONE',  ( 114.7458293810856418, -30.61868467657538062, 240.3613395616249875 ) ) ;
#42625=CARTESIAN_POINT ( 'NONE',  ( 107.0664832912739399, -36.72944715994095333, 293.6369201390379544 ) ) ;
#42626=CARTESIAN_POINT ( 'NONE',  ( 107.3174176841070846, -26.95189801805073060, 116.0556252759109555 ) ) ;
#42629=EDGE_LOOP ( 'NONE', ( #75164, #77279, #26613, #63309 ) ) ;
#42630=CARTESIAN_POINT ( 'NONE',  ( 32.16397622746000451, -34.03355364505800651, 313.9678068554150059 ) ) ;
#42632=ORIENTED_EDGE ( 'NONE', *, *, #75738, .T. ) ;
#42633=EDGE_CURVE ( 'NONE', #18458, #18701, #87570, .T. ) ;
#42635=CARTESIAN_POINT ( 'NONE',  ( 98.34725308318749626, -40.22966859802066608, 248.0739642582779538 ) ) ;
#42636=VECTOR ( 'NONE', #12910, 1000.000000000000000 ) ;
#42637=LINE ( 'NONE', #70373, #50254 ) ;
#42640=DIRECTION ( 'NONE',  ( 0.5180656453708486486, 0.02186357193551463976, 0.8550613845266940016 ) ) ;
#42641=CARTESIAN_POINT ( 'NONE',  ( 51.24204729617298426, -31.76306994223730840, 313.9678068554150059 ) ) ;
#42643=CARTESIAN_POINT ( 'NONE',  ( 142.8830277309893404, -77.57998310118428265, 542.9756252759101471 ) ) ;
#42644=CYLINDRICAL_SURFACE ( 'NONE', #52750, 4.874999999999990230 ) ;
#42646=CARTESIAN_POINT ( 'NONE',  ( 104.7356349775885320, -47.53436426244870461, 32.41943479972098174 ) ) ;
#42647=ORIENTED_EDGE ( 'NONE', *, *, #68497, .T. ) ;
#42648=CARTESIAN_POINT ( 'NONE',  ( 116.1953253310505119, -40.03623866633203932, 22.97241982807796035 ) ) ;
#42649=CARTESIAN_POINT ( 'NONE',  ( 105.7166318498146325, -46.72402321261439795, 127.4690705953080965 ) ) ;
#42650=CARTESIAN_POINT ( 'NONE',  ( 103.2980200187117390, -27.06831524915186904, 170.3603871806729444 ) ) ;
#42651=ADVANCED_FACE ( 'NONE', ( #35948 ), #51237, .T. ) ;
#42652=CARTESIAN_POINT ( 'NONE',  ( 143.0664832912740110, -18.82844715994099971, 323.8756252759120002 ) ) ;
#42654=CARTESIAN_POINT ( 'NONE',  ( 107.0664832912739968, -36.72944715994100306, 287.6356252759109680 ) ) ;
#42655=DIRECTION ( 'NONE',  ( 1.000000000000000000, 4.299999999999999979E-14, 1.000000000000000078E-15 ) ) ;
#42656=CARTESIAN_POINT ( 'NONE',  ( 100.1487569102796300, -45.40945638099971404, 268.0289586092443415 ) ) ;
#42660=CARTESIAN_POINT ( 'NONE',  ( 136.7765779009440621, -37.19711456032074892, 6.808568500765878717 ) ) ;
#42661=VECTOR ( 'NONE', #40093, 1000.000000000000000 ) ;
#42662=VERTEX_POINT ( 'NONE', #31246 ) ;
#42663=CARTESIAN_POINT ( 'NONE',  ( 117.9205228141932054, -39.05050820906062370, 104.6708633711489824 ) ) ;
#42664=LINE ( 'NONE', #82706, #10544 ) ;
#42666=CIRCLE ( 'NONE', #3526, 1.000000000000000888 ) ;
#42669=EDGE_LOOP ( 'NONE', ( #40918, #81132, #63826, #2463 ) ) ;
#42672=AXIS2_PLACEMENT_3D ( 'NONE', #87781, #12373, #33711 ) ;
#42673=CARTESIAN_POINT ( 'NONE',  ( 115.8254327561651280, -31.73001971868101023, 265.2397918660585105 ) ) ;
#42674=CARTESIAN_POINT ( 'NONE',  ( 179.1667039024460166, -26.71338133339251542, -5.074374724088000832 ) ) ;
#42677=CARTESIAN_POINT ( 'NONE',  ( 104.7356836917145699, -47.53413844247978659, 28.41943479971997988 ) ) ;
#42679=ORIENTED_EDGE ( 'NONE', *, *, #33588, .T. ) ;
#42682=EDGE_LOOP ( 'NONE', ( #80483, #32248, #16291 ) ) ;
#42684=DIRECTION ( 'NONE',  ( 0.000000000000000000, 0.000000000000000000, -1.000000000000000000 ) ) ;
#42685=DIRECTION ( 'NONE',  ( 0.7071067811865764385, -0.7071067811865187069, 7.071067811865771156E-16 ) ) ;
#42687=EDGE_CURVE ( 'NONE', #19992, #39136, #44880, .T. ) ;
#42688=CARTESIAN_POINT ( 'NONE',  ( 71.25529199314597406, -79.12815651470189948, 361.9756252759101471 ) ) ;
#42689=FACE_OUTER_BOUND ( 'NONE', #34289, .T. ) ;
#42690=EDGE_CURVE ( 'NONE', #22696, #17346, #42740, .T. ) ;
#42691=CARTESIAN_POINT ( 'NONE',  ( 115.5441482490607257, -35.68765611295631857, 193.3467055423629688 ) ) ;
#42692=CARTESIAN_POINT ( 'NONE',  ( 107.0667039024467329, -19.99944715994091027, 195.5838068554170093 ) ) ;
#42694=CARTESIAN_POINT ( 'NONE',  ( 118.8926602832294037, -35.39890769255473657, 83.91562527591095488 ) ) ;
#42695=ORIENTED_EDGE ( 'NONE', *, *, #30943, .F. ) ;
#42696=CARTESIAN_POINT ( 'NONE',  ( 32.24491389930098251, -32.11662333284611748, -5.074374724088000832 ) ) ;
#42698=EDGE_CURVE ( 'NONE', #40009, #48304, #32141, .T. ) ;
#42699=CARTESIAN_POINT ( 'NONE',  ( 98.34844285637596784, -31.65902197265687334, 276.9066052923088250 ) ) ;
#42700=ORIENTED_EDGE ( 'NONE', *, *, #3038, .F. ) ;
#42701=CARTESIAN_POINT ( 'NONE',  ( 104.4897565938694584, -26.97885740413062550, 50.28147460018952586 ) ) ;
#42702=EDGE_CURVE ( 'NONE', #9938, #36669, #25925, .T. ) ;
#42704=DIRECTION ( 'NONE',  ( 0.000000000000000000, -1.000000000000007375E-15, -1.000000000000000000 ) ) ;
#42707=FACE_OUTER_BOUND ( 'NONE', #47460, .T. ) ;
#42708=ORIENTED_EDGE ( 'NONE', *, *, #49885, .F. ) ;
#42709=CARTESIAN_POINT ( 'NONE',  ( 109.6484814735558189, -46.85267042889636002, 47.77562527591094721 ) ) ;
#42713=LINE ( 'NONE', #8227, #84421 ) ;
#42714=CARTESIAN_POINT ( 'NONE',  ( 101.9936209166423993, -45.44607152480659096, 142.1564586070478526 ) ) ;
#42715=VERTEX_POINT ( 'NONE', #73032 ) ;
#42716=EDGE_CURVE ( 'NONE', #19408, #36906, #87128, .T. ) ;
#42717=CARTESIAN_POINT ( 'NONE',  ( 115.5843262439540808, -31.42642995851512566, 120.2690150466928571 ) ) ;
#42718=CYLINDRICAL_SURFACE ( 'NONE', #86082, 2.749999999999974687 ) ;
#42720=CARTESIAN_POINT ( 'NONE',  ( 98.13097783494514204, -43.27482323654912477, 102.8175300378159847 ) ) ;
#42721=DIRECTION ( 'NONE',  ( 0.000000000000000000, 0.000000000000000000, -1.000000000000000000 ) ) ;
#42722=DIRECTION ( 'NONE',  ( -8.843517682682131024E-16, 1.000000000000000000, 1.156482317317870556E-31 ) ) ;
#42725=ORIENTED_EDGE ( 'NONE', *, *, #23596, .T. ) ;
#42726=AXIS2_PLACEMENT_3D ( 'NONE', #15505, #83650, #35926 ) ;
#42727=VECTOR ( 'NONE', #50345, 1000.000000000000000 ) ;
#42728=AXIS2_PLACEMENT_3D ( 'NONE', #43826, #63848, #1173 ) ;
#42730=CARTESIAN_POINT ( 'NONE',  ( 113.6473777113567820, -44.00994186338851932, 129.1613395616249704 ) ) ;
#42731=CARTESIAN_POINT ( 'NONE',  ( 156.5667039024482108, -42.82844715993568485, 295.7178068554149490 ) ) ;
#42733=AXIS2_PLACEMENT_3D ( 'NONE', #40138, #6528, #81516 ) ;
#42735=CARTESIAN_POINT ( 'NONE',  ( 112.4780167374715631, -46.34085331822165443, 253.9965776568634510 ) ) ;
#42736=FACE_BOUND ( 'NONE', #38443, .T. ) ;
#42737=CARTESIAN_POINT ( 'NONE',  ( 184.5667039024483245, -48.82844715993448403, 300.4678068554149490 ) ) ;
#42739=PLANE ( 'NONE',  #9439 ) ;
#42740=LINE ( 'NONE', #66666, #68006 ) ;
#42741=CARTESIAN_POINT ( 'NONE',  ( 97.81193015299326987, -40.51731617131004271, 31.63594527021773573 ) ) ;
#42742=CARTESIAN_POINT ( 'NONE',  ( 96.86352172870815025, -32.31225822881502552, 211.0013395616259686 ) ) ;
#42744=ORIENTED_EDGE ( 'NONE', *, *, #2457, .F. ) ;
#42745=EDGE_CURVE ( 'NONE', #25185, #36098, #52119, .T. ) ;
#42746=CARTESIAN_POINT ( 'NONE',  ( 115.3457950989190408, -42.46736495413998824, 159.7758690201829666 ) ) ;
#42747=CARTESIAN_POINT ( 'NONE',  ( 83.06670390244801183, -42.97311385574013798, 231.5838068554169524 ) ) ;
#42748=CARTESIAN_POINT ( 'NONE',  ( 98.59875070808803343, -39.34206841476268579, 17.99586902018296541 ) ) ;
#42750=ADVANCED_FACE ( 'NONE', ( #70480 ), #3998, .F. ) ;
#42751=VECTOR ( 'NONE', #37026, 1000.000000000000000 ) ;
#42754=CARTESIAN_POINT ( 'NONE',  ( 112.1393456400033699, -28.01282278016224225, 105.6564586093976601 ) ) ;
#42755=DIRECTION ( 'NONE',  ( 0.000000000000000000, 1.000000000000000000, 0.000000000000000000 ) ) ;
#42756=CARTESIAN_POINT ( 'NONE',  ( 113.2071528006340628, -45.12711609280825087, 228.0784824187679760 ) ) ;
#42757=CARTESIAN_POINT ( 'NONE',  ( 97.70686550411159033, -40.25212671267365749, 171.6131552557610860 ) ) ;
#42760=CARTESIAN_POINT ( 'NONE',  ( 116.7951252700267304, -39.38782979579554677, 88.61479194211217703 ) ) ;
#42764=CARTESIAN_POINT ( 'NONE',  ( 115.3461623907573710, -31.52268719801068642, 30.27276813305296344 ) ) ;
#42765=CARTESIAN_POINT ( 'NONE',  ( 194.5667039024479834, -67.87844715994100397, 300.9178068554150514 ) ) ;
#42767=EDGE_CURVE ( 'NONE', #58352, #36440, #16743, .T. ) ;
#42768=DIRECTION ( 'NONE',  ( -4.237773401492740281E-14, 1.000000000000000000, 0.000000000000000000 ) ) ;
#42772=CARTESIAN_POINT ( 'NONE',  ( 100.8483124575627414, -45.14135884264823773, 257.0699109901967745 ) ) ;
#42773=ORIENTED_EDGE ( 'NONE', *, *, #39272, .T. ) ;
#42774=CARTESIAN_POINT ( 'NONE',  ( 25.56670390244797275, -67.87844715994100397, 298.0928068554150627 ) ) ;
#42776=CARTESIAN_POINT ( 'NONE',  ( 110.8537518669637194, -45.98453207236645568, 167.8855633520927597 ) ) ;
#42777=CARTESIAN_POINT ( 'NONE',  ( 106.9575452361726491, -28.53976946500068124, 57.90523322673496409 ) ) ;
#42778=CARTESIAN_POINT ( 'NONE',  ( 113.7646124051505154, -44.74644941934948861, 189.1299109901969757 ) ) ;
#42779=LINE ( 'NONE', #70522, #27577 ) ;
#42780=ORIENTED_EDGE ( 'NONE', *, *, #17087, .F. ) ;
#42781=CARTESIAN_POINT ( 'NONE',  ( 152.0371591254585724, -47.82818131005588214, 129.9678068554149775 ) ) ;
#42782=ORIENTED_EDGE ( 'NONE', *, *, #11536, .T. ) ;
#42785=CIRCLE ( 'NONE', #10903, 2.030000000001807248 ) ;
#42786=FACE_OUTER_BOUND ( 'NONE', #28338, .T. ) ;
#42788=ORIENTED_EDGE ( 'NONE', *, *, #58904, .F. ) ;
#42789=ORIENTED_EDGE ( 'NONE', *, *, #84455, .T. ) ;
#42790=PLANE ( 'NONE',  #30931 ) ;
#42791=AXIS2_PLACEMENT_3D ( 'NONE', #81476, #46903, #63248 ) ;
#42792=CARTESIAN_POINT ( 'NONE',  ( 106.7492034591024890, -25.27298593721235065, 320.5317020237883980 ) ) ;
#42793=ADVANCED_FACE ( 'NONE', ( #44422, #72158 ), #79883, .F. ) ;
#42794=CARTESIAN_POINT ( 'NONE',  ( 112.3425469992411649, -30.01235824646559891, 78.96956268521998368 ) ) ;
#42795=VECTOR ( 'NONE', #48183, 1000.000000000000000 ) ;
#42796=CARTESIAN_POINT ( 'NONE',  ( 102.3692588328596571, -47.63350050119395007, 287.2527681330535643 ) ) ;
#42797=DIRECTION ( 'NONE',  ( 1.000000000000000000, 6.508581945447490214E-14, 1.000000000000000078E-15 ) ) ;
#42798=ADVANCED_FACE ( 'NONE', ( #58506 ), #86232, .F. ) ;
#42801=EDGE_CURVE ( 'NONE', #73498, #32398, #57453, .T. ) ;
#42803=CARTESIAN_POINT ( 'NONE',  ( 131.0667039024480118, -64.87844715994098976, 225.9838068554150254 ) ) ;
#42804=CARTESIAN_POINT ( 'NONE',  ( 107.0664832912739968, -18.82844715994099971, 333.4006252759120343 ) ) ;
#42807=CARTESIAN_POINT ( 'NONE',  ( 105.0928733274061670, -25.78792777683064585, 125.2184824187689856 ) ) ;
#42808=CARTESIAN_POINT ( 'NONE',  ( 114.7585751371172051, -43.83144610948713193, 123.2327681330539519 ) ) ;
#42809=LINE ( 'NONE', #57799, #65416 ) ;
#42811=CARTESIAN_POINT ( 'NONE',  ( 99.53925745938779812, -29.46537268684611632, 250.7156252759109520 ) ) ;
#42812=DIRECTION ( 'NONE',  ( 8.673617379884035472E-16, 1.000000000000000000, 0.000000000000000000 ) ) ;
#42814=CARTESIAN_POINT ( 'NONE',  ( 98.42298862519912461, -41.77040527891428923, 27.74721501551390546 ) ) ;
#42818=DIRECTION ( 'NONE',  ( -0.000000000000000000, -0.000000000000000000, 1.000000000000000000 ) ) ;
#42821=EDGE_CURVE ( 'NONE', #77789, #16763, #50619, .T. ) ;
#42826=CARTESIAN_POINT ( 'NONE',  ( 97.06107110202495392, -37.99641200327471324, 261.4272919457318380 ) ) ;
#42827=ORIENTED_EDGE ( 'NONE', *, *, #27206, .F. ) ;
#42829=CARTESIAN_POINT ( 'NONE',  ( 97.53973001301494605, -43.81993288943278486, 261.8356252759109566 ) ) ;
#42830=CARTESIAN_POINT ( 'NONE',  ( 105.7204281913532355, -24.95562743476950018, 156.1670538473399574 ) ) ;
#42831=CARTESIAN_POINT ( 'NONE',  ( 100.5841487926172277, -28.49196697857695781, 11.60705384733995515 ) ) ;
#42832=PLANE ( 'NONE',  #72235 ) ;
#42834=CARTESIAN_POINT ( 'NONE',  ( 82.45780623542886190, -35.36823420009603325, 7.200493380643411712 ) ) ;
#42835=DIRECTION ( 'NONE',  ( -0.7071067811865170416, -0.7071067811865778818, -7.071067811865162747E-16 ) ) ;
#42839=CARTESIAN_POINT ( 'NONE',  ( 139.7494832912729805, -71.52944715994142655, 342.9256252759109884 ) ) ;
#42841=CARTESIAN_POINT ( 'NONE',  ( 102.9572487778789878, -44.79956872283601399, 171.6362293518859587 ) ) ;
#42844=CARTESIAN_POINT ( 'NONE',  ( 152.0371591254585155, -47.82818131005588214, 180.4678068554149775 ) ) ;
#42845=CARTESIAN_POINT ( 'NONE',  ( 109.4403364888816981, -25.95778788316477304, 175.8918157521009391 ) ) ;
#42848=DIRECTION ( 'NONE',  ( 0.000000000000000000, 0.000000000000000000, -1.000000000000000000 ) ) ;
#42850=CARTESIAN_POINT ( 'NONE',  ( 172.5664832912740110, -9.303447159940999356, 258.9256252759120116 ) ) ;
#42851=CARTESIAN_POINT ( 'NONE',  ( 99.36524671511898532, -42.81259845621070781, 91.85848241876892928 ) ) ;
#42853=ORIENTED_EDGE ( 'NONE', *, *, #50054, .F. ) ;
#42855=ORIENTED_EDGE ( 'NONE', *, *, #82005, .T. ) ;
#42856=AXIS2_PLACEMENT_3D ( 'NONE', #76283, #41292, #7250 ) ;
#42857=CARTESIAN_POINT ( 'NONE',  ( 113.2603198993755882, -43.06700715444978300, 69.62444044875392990 ) ) ;
#42858=AXIS2_PLACEMENT_3D ( 'NONE', #46418, #54120, #13271 ) ;
#42859=FACE_OUTER_BOUND ( 'NONE', #58136, .T. ) ;
#42860=CARTESIAN_POINT ( 'NONE',  ( 114.4768422515204094, -30.34587328852060395, 180.3927681330529538 ) ) ;
#42862=AXIS2_PLACEMENT_3D ( 'NONE', #59841, #74838, #88479 ) ;
#42863=CARTESIAN_POINT ( 'NONE',  ( 41.56648329127399677, -9.303447159940999356, 258.9256252759120116 ) ) ;
#42866=VECTOR ( 'NONE', #47413, 1000.000000000000000 ) ;
#42870=CARTESIAN_POINT ( 'NONE',  ( 98.47430666977638225, -42.65725675464092603, 126.8070538473389490 ) ) ;
#42871=ORIENTED_EDGE ( 'NONE', *, *, #45371, .T. ) ;
#42873=ORIENTED_EDGE ( 'NONE', *, *, #35302, .F. ) ;
#42874=AXIS2_PLACEMENT_3D ( 'NONE', #72811, #9254, #59602 ) ;
#42877=CARTESIAN_POINT ( 'NONE',  ( 115.0372575023011450, -42.90846257223464022, 79.30229194203350573 ) ) ;
#42879=VECTOR ( 'NONE', #55794, 1000.000000000000000 ) ;
#42880=CARTESIAN_POINT ( 'NONE',  ( 115.1674193411231784, -35.52216783720512439, 216.7623760838769726 ) ) ;
#42884=ORIENTED_EDGE ( 'NONE', *, *, #23161, .F. ) ;
#42886=ORIENTED_EDGE ( 'NONE', *, *, #69446, .T. ) ;
#42887=DIRECTION ( 'NONE',  ( 1.000000000000000000, 0.000000000000000000, 0.000000000000000000 ) ) ;
#42888=VERTEX_POINT ( 'NONE', #33935 ) ;
#42889=ORIENTED_EDGE ( 'NONE', *, *, #1410, .T. ) ;
#42890=DIRECTION ( 'NONE',  ( 0.000000000000000000, -1.000000000000000000, 0.000000000000000000 ) ) ;
#42891=DIRECTION ( 'NONE',  ( -1.000000000000000000, -4.299999999999999979E-14, -1.000000000000000078E-15 ) ) ;
#42892=CARTESIAN_POINT ( 'NONE',  ( 116.4035850909244090, -35.68299815489336879, 230.3349166392299594 ) ) ;
#42894=CARTESIAN_POINT ( 'NONE',  ( 116.8171228894634481, -34.15291837667594166, 274.0314586044273710 ) ) ;
#42895=ORIENTED_EDGE ( 'NONE', *, *, #19126, .T. ) ;
#42896=DIRECTION ( 'NONE',  ( 1.000000000000000000, 0.000000000000000000, 0.000000000000000000 ) ) ;
#42897=DIRECTION ( 'NONE',  ( 0.000000000000000000, 0.000000000000000000, -1.000000000000000000 ) ) ;
#42898=ORIENTED_EDGE ( 'NONE', *, *, #57479, .T. ) ;
#42899=VERTEX_POINT ( 'NONE', #27131 ) ;
#42901=CARTESIAN_POINT ( 'NONE',  ( 41.56648329127398966, -18.82844715994071194, 18.92562527591200094 ) ) ;
#42905=ADVANCED_FACE ( 'NONE', ( #12163 ), #68015, .F. ) ;
#42906=CARTESIAN_POINT ( 'NONE',  ( 105.1260075982565212, -28.80065313513137326, 283.0852332267343172 ) ) ;
#42907=CARTESIAN_POINT ( 'NONE',  ( 117.4484615961127218, -30.96329225543088270, 179.2299109901959753 ) ) ;
#42908=CARTESIAN_POINT ( 'NONE',  ( 101.7670726180548115, -27.05576796868577460, 100.4632443235299633 ) ) ;
#42910=CARTESIAN_POINT ( 'NONE',  ( 117.2274905824790778, -41.08006910540670731, 209.5165776568640013 ) ) ;
#42911=DIRECTION ( 'NONE',  ( 1.000000000000000078E-15, -1.000000000000000083E-30, -1.000000000000000000 ) ) ;
#42912=ADVANCED_FACE ( 'NONE', ( #54807 ), #40508, .T. ) ;
#42915=DIRECTION ( 'NONE',  ( -1.000000000000000078E-15, -1.000000000000000083E-30, 1.000000000000000000 ) ) ;
#42916=ORIENTED_EDGE ( 'NONE', *, *, #41404, .T. ) ;
#42918=CARTESIAN_POINT ( 'NONE',  ( 34.67381068360336371, -28.98061976759059988, 193.9678068554150911 ) ) ;
#42921=VERTEX_POINT ( 'NONE', #19871 ) ;
#42922=CARTESIAN_POINT ( 'NONE',  ( 108.3194705677269809, -47.07918403323724021, 117.6727681330539639 ) ) ;
#42923=CARTESIAN_POINT ( 'NONE',  ( 97.31575241016307132, -39.30575056309270110, 256.5314103656009479 ) ) ;
#42926=CARTESIAN_POINT ( 'NONE',  ( 52.65249034007830176, -49.32844715994059470, 300.4678068554150059 ) ) ;
#42927=CARTESIAN_POINT ( 'NONE',  ( 34.96670390244654669, -26.71338133339322951, 117.4678068554150485 ) ) ;
#42928=PLANE ( 'NONE',  #51359 ) ;
#42929=CARTESIAN_POINT ( 'NONE',  ( 117.4688788178165737, -35.86077403649778716, 249.8927681330537780 ) ) ;
#42932=LINE ( 'NONE', #84316, #55598 ) ;
#42934=DIRECTION ( 'NONE',  ( 0.000000000000000000, 0.000000000000000000, 1.000000000000000000 ) ) ;
#42935=EDGE_CURVE ( 'NONE', #88995, #67882, #73905, .T. ) ;
#42939=CARTESIAN_POINT ( 'NONE',  ( 115.6917119993852054, -30.73301325301421016, 279.3099109901964994 ) ) ;
#42940=ORIENTED_EDGE ( 'NONE', *, *, #55826, .F. ) ;
#42941=CARTESIAN_POINT ( 'NONE',  ( 85.58420390244806697, -58.72944715994107412, 231.5838068554169524 ) ) ;
#42942=CARTESIAN_POINT ( 'NONE',  ( 111.4265353497823128, -47.77589283047310431, 172.8756252759109771 ) ) ;
#42943=CARTESIAN_POINT ( 'NONE',  ( 107.6068523407233926, -48.56763185392661342, 38.61276813305397582 ) ) ;
#42944=CARTESIAN_POINT ( 'NONE',  ( 103.2878376434171628, -26.96651641063459337, 211.3699109901969848 ) ) ;
#42946=CARTESIAN_POINT ( 'NONE',  ( 32.06670390244683233, -33.35206098992750157, 117.4678068554150485 ) ) ;
#42947=DIRECTION ( 'NONE',  ( 0.000000000000000000, 1.000000000000000000, 0.000000000000000000 ) ) ;
#42948=AXIS2_PLACEMENT_3D ( 'NONE', #31532, #80156, #25163 ) ;
#42951=CARTESIAN_POINT ( 'NONE',  ( 97.06107109463341942, -37.99641194202747130, 71.42729194085987388 ) ) ;
#42952=LINE ( 'NONE', #84774, #45085 ) ;
#42954=DIRECTION ( 'NONE',  ( -4.299999999999999979E-14, 1.000000000000000000, -4.400000000000000367E-29 ) ) ;
#42955=ORIENTED_EDGE ( 'NONE', *, *, #70758, .F. ) ;
#42956=ORIENTED_EDGE ( 'NONE', *, *, #17708, .F. ) ;
#42957=CYLINDRICAL_SURFACE ( 'NONE', #51636, 9.999999999999998224 ) ;
#42958=EDGE_LOOP ( 'NONE', ( #11446, #20638 ) ) ;
#42959=CARTESIAN_POINT ( 'NONE',  ( 105.9906760191434358, -26.38192068051327510, 46.15848241876796720 ) ) ;
#42960=CARTESIAN_POINT ( 'NONE',  ( 75.31670390244798341, -57.40094715994099772, 88.43480685541499042 ) ) ;
#42962=CARTESIAN_POINT ( 'NONE',  ( 117.8455077981468122, -34.08178244914028454, 160.0061014663869798 ) ) ;
#42963=CARTESIAN_POINT ( 'NONE',  ( 98.99648076951073961, -33.93126856627920773, 285.4838483995053480 ) ) ;
#42964=EDGE_LOOP ( 'NONE', ( #38776, #36566 ) ) ;
#42967=ORIENTED_EDGE ( 'NONE', *, *, #49494, .F. ) ;
#42968=CARTESIAN_POINT ( 'NONE',  ( 83.56670559755329464, -40.03837296219064967, 239.5838068554176914 ) ) ;
#42969=PLANE ( 'NONE',  #55030 ) ;
#42970=DIRECTION ( 'NONE',  ( 0.000000000000000000, -1.000000000000000000, 0.000000000000000000 ) ) ;
#42971=CARTESIAN_POINT ( 'NONE',  ( 97.07207205724220955, -35.37844121140676634, 76.21895861022630925 ) ) ;
#42973=DIRECTION ( 'NONE',  ( 0.7071067811739204512, -0.7071067811991745833, 0.000000000000000000 ) ) ;
#42976=CARTESIAN_POINT ( 'NONE',  ( 115.7453557663426409, -41.23947501269460503, 288.4441967044829767 ) ) ;
#42979=DIRECTION ( 'NONE',  ( 0.1858654558203329255, -0.9825752044157738396, 0.000000000000000000 ) ) ;
#42981=CARTESIAN_POINT ( 'NONE',  ( 98.94907028073869526, -37.58812756235333552, 124.2280903695919818 ) ) ;
#42982=CIRCLE ( 'NONE', #51676, 5.599999999999994316 ) ;
#42984=EDGE_CURVE ( 'NONE', #27190, #37008, #85475, .T. ) ;
#42986=ADVANCED_FACE ( 'NONE', ( #13062 ), #21677, .F. ) ;
#42987=DIRECTION ( 'NONE',  ( 4.299999999999999979E-14, -1.000000000000000000, 4.400000000000000367E-29 ) ) ;
#42988=FACE_OUTER_BOUND ( 'NONE', #24520, .T. ) ;
#42990=ORIENTED_EDGE ( 'NONE', *, *, #55580, .F. ) ;
#42991=EDGE_CURVE ( 'NONE', #44647, #59006, #42531, .T. ) ;
#42992=CARTESIAN_POINT ( 'NONE',  ( 113.1785701771607080, -44.75166289368706174, 138.0916005355700236 ) ) ;
#42994=ORIENTED_EDGE ( 'NONE', *, *, #57242, .T. ) ;
#42995=EDGE_CURVE ( 'NONE', #24712, #54590, #11526, .T. ) ;
#42996=CARTESIAN_POINT ( 'NONE',  ( 108.1711956065674229, -46.05983505851052229, 159.1139642582779459 ) ) ;
#42997=EDGE_CURVE ( 'NONE', #83770, #63582, #4263, .T. ) ;
#42999=AXIS2_PLACEMENT_3D ( 'NONE', #73641, #87282, #31402 ) ;
#43000=CARTESIAN_POINT ( 'NONE',  ( 97.20510023974232183, -31.68580462152881339, 91.96229194257693962 ) ) ;
#43002=CARTESIAN_POINT ( 'NONE',  ( 57.56670390244832447, -48.82844715994039575, 254.7178068554150627 ) ) ;
#43003=ORIENTED_EDGE ( 'NONE', *, *, #56232, .T. ) ;
#43004=EDGE_CURVE ( 'NONE', #667, #35758, #21219, .T. ) ;
#43005=ORIENTED_EDGE ( 'NONE', *, *, #48526, .T. ) ;
#43006=ORIENTED_EDGE ( 'NONE', *, *, #17191, .T. ) ;
#43007=EDGE_CURVE ( 'NONE', #22595, #57623, #14412, .T. ) ;
#43008=CARTESIAN_POINT ( 'NONE',  ( 106.8407094991504209, -48.60307516909384873, 77.56133956162491927 ) ) ;
#43009=ORIENTED_EDGE ( 'NONE', *, *, #25897, .F. ) ;
#43010=CARTESIAN_POINT ( 'NONE',  ( 115.9511604156667772, -42.07746527209881293, 278.3832443235305618 ) ) ;
#43011=CARTESIAN_POINT ( 'NONE',  ( 114.9943830143096335, -28.99422824087939432, 190.4537205140059655 ) ) ;
#43012=EDGE_CURVE ( 'NONE', #30145, #24616, #47754, .T. ) ;
#43013=DIRECTION ( 'NONE',  ( 0.000000000000000000, 1.000000000000000000, 0.000000000000000000 ) ) ;
#43015=CARTESIAN_POINT ( 'NONE',  ( 103.2054172826541816, -46.45125265344608323, 113.2756252759109827 ) ) ;
#43017=DIRECTION ( 'NONE',  ( 0.000000000000000000, -1.000000000000000000, 0.000000000000000000 ) ) ;
#43021=CARTESIAN_POINT ( 'NONE',  ( 98.15086158280806217, -41.26138559404058981, 132.7011821357229451 ) ) ;
#43023=ORIENTED_EDGE ( 'NONE', *, *, #13070, .T. ) ;
#43026=CARTESIAN_POINT ( 'NONE',  ( 100.5975332644244844, -28.50897509465477597, 15.60705384733995871 ) ) ;
#43027=CARTESIAN_POINT ( 'NONE',  ( 163.2569089553700223, -33.54226604285010893, 342.9256252759119548 ) ) ;
#43028=CARTESIAN_POINT ( 'NONE',  ( 71.24025061656124080, 8.642044024269713631, 394.9756252759102040 ) ) ;
#43030=CARTESIAN_POINT ( 'NONE',  ( 98.38136461969642710, -29.78821554292430207, 45.78991099019597044 ) ) ;
#43031=DIRECTION ( 'NONE',  ( -1.000000000000000078E-15, 0.000000000000000000, -1.000000000000000000 ) ) ;
#43032=CARTESIAN_POINT ( 'NONE',  ( 100.8994224252809033, -45.87202276647009569, 148.0918157521009562 ) ) ;
#43033=CARTESIAN_POINT ( 'NONE',  ( 99.09570907051013933, -30.55043176026986984, 71.80229194329096742 ) ) ;
#43035=ORIENTED_EDGE ( 'NONE', *, *, #67009, .T. ) ;
#43036=CARTESIAN_POINT ( 'NONE',  ( 116.3212776292296127, -32.94146857471318413, 287.6356252759109680 ) ) ;
#43037=EDGE_CURVE ( 'NONE', #5230, #1134, #84362, .T. ) ;
#43040=EDGE_CURVE ( 'NONE', #24376, #68890, #42091, .T. ) ;
#43041=EDGE_LOOP ( 'NONE', ( #68964, #2355, #49483, #33900, #86000, #44747, #12900, #11138, #29484 ) ) ;
#43042=ADVANCED_FACE ( 'NONE', ( #14865 ), #41633, .F. ) ;
#43043=CARTESIAN_POINT ( 'NONE',  ( 34.33598329127499227, -36.32844715994100682, 313.9678068554150059 ) ) ;
#43044=CARTESIAN_POINT ( 'NONE',  ( 117.5314631938956182, -40.43040369381473198, 178.5680062282919778 ) ) ;
#43045=EDGE_LOOP ( 'NONE', ( #18333, #67971, #27489, #88493 ) ) ;
#43046=FACE_OUTER_BOUND ( 'NONE', #86237, .T. ) ;
#43047=CARTESIAN_POINT ( 'NONE',  ( 101.3928372362931896, -45.54357991663450633, 218.1213395616249784 ) ) ;
#43048=CARTESIAN_POINT ( 'NONE',  ( 97.50257212865312795, -32.47214954040395440, 96.99276813305395706 ) ) ;
#43051=CARTESIAN_POINT ( 'NONE',  ( 80.06648281188265059, -39.47944715903999224, 8.225259175037734849 ) ) ;
#43053=EDGE_LOOP ( 'NONE', ( #77072, #22632, #48015, #16653 ) ) ;
#43056=AXIS2_PLACEMENT_3D ( 'NONE', #7157, #13075, #27590 ) ;
#43057=EDGE_LOOP ( 'NONE', ( #23356, #63779, #79698, #49971 ) ) ;
#43058=ORIENTED_EDGE ( 'NONE', *, *, #50231, .F. ) ;
#43059=ORIENTED_EDGE ( 'NONE', *, *, #44049, .T. ) ;
#43060=CARTESIAN_POINT ( 'NONE',  ( 75.31670390244798341, -67.87844715994100397, 63.03480685541479289 ) ) ;
#43061=CARTESIAN_POINT ( 'NONE',  ( 100.2482148738244661, -28.84314871041893014, 256.6441967044821695 ) ) ;
#43062=CARTESIAN_POINT ( 'NONE',  ( 116.3212776292292716, -32.94146857471233147, 105.1356252759109680 ) ) ;
#43063=CARTESIAN_POINT ( 'NONE',  ( 134.7196861477300445, -16.05633243510672159, 1.689562801604479692 ) ) ;
#43064=VECTOR ( 'NONE', #32928, 1000.000000000000000 ) ;
#43065=LINE ( 'NONE', #62632, #23590 ) ;
#43068=AXIS2_PLACEMENT_3D ( 'NONE', #4610, #59993, #30969 ) ;
#43069=CARTESIAN_POINT ( 'NONE',  ( 100.3969032678572262, -28.68811230323557027, 40.62705384733894221 ) ) ;
#43070=ORIENTED_EDGE ( 'NONE', *, *, #30832, .T. ) ;
#43071=VERTEX_POINT ( 'NONE', #15754 ) ;
#43072=ORIENTED_EDGE ( 'NONE', *, *, #76042, .F. ) ;
#43074=LINE ( 'NONE', #9472, #29653 ) ;
#43076=CARTESIAN_POINT ( 'NONE',  ( 100.6033219294153724, -44.83909144599376617, 268.0289586092438867 ) ) ;
#43077=LINE ( 'NONE', #9476, #70525 ) ;
#43078=CARTESIAN_POINT ( 'NONE',  ( 98.49710108934571906, -31.94619897774425610, 106.9213395616249755 ) ) ;
#43079=DIRECTION ( 'NONE',  ( -1.000000000000000000, -1.000000000000000078E-15, -1.000000000000000078E-15 ) ) ;
#43081=ORIENTED_EDGE ( 'NONE', *, *, #69897, .F. ) ;
#43083=CARTESIAN_POINT ( 'NONE',  ( 97.31307424872157696, -38.96060643753106945, 57.50540973980124448 ) ) ;
#43084=EDGE_LOOP ( 'NONE', ( #28323, #79803 ) ) ;
#43085=EDGE_LOOP ( 'NONE', ( #59049, #56183, #84419, #2829 ) ) ;
#43087=CARTESIAN_POINT ( 'NONE',  ( 115.2453386458995652, -37.16432389609550313, 16.60237608387699026 ) ) ;
#43088=AXIS2_PLACEMENT_3D ( 'NONE', #80847, #74012, #65515 ) ;
#43089=FACE_OUTER_BOUND ( 'NONE', #13002, .T. ) ;
#43092=CARTESIAN_POINT ( 'NONE',  ( 116.3212776292269268, -32.94146857470660450, 84.13562527591095375 ) ) ;
#43095=CARTESIAN_POINT ( 'NONE',  ( 90.44969454456408187, -53.34645651782490461, 239.5838068554174356 ) ) ;
#43097=DIRECTION ( 'NONE',  ( 0.7071067811865671127, 0.7071067811865279218, 7.071067811865664660E-16 ) ) ;
#43099=CARTESIAN_POINT ( 'NONE',  ( 117.3536837868190332, -38.62665896660388398, 88.68133956162493803 ) ) ;
#43100=ORIENTED_EDGE ( 'NONE', *, *, #45759, .F. ) ;
#43101=CARTESIAN_POINT ( 'NONE',  ( 111.1942201901869680, -30.05669425270436790, 287.4538046553057029 ) ) ;
#43102=EDGE_CURVE ( 'NONE', #81215, #30264, #40644, .T. ) ;
#43103=DIRECTION ( 'NONE',  ( 0.9242245927363033076, 0.3818493186865918321, 0.000000000000000000 ) ) ;
#43104=CARTESIAN_POINT ( 'NONE',  ( 113.2764755850018048, -45.03455287549805774, 188.0994347997209672 ) ) ;
#43108=VECTOR ( 'NONE', #47143, 1000.000000000000000 ) ;
#43109=FACE_OUTER_BOUND ( 'NONE', #20677, .T. ) ;
#43110=CARTESIAN_POINT ( 'NONE',  ( 112.6870894866849966, -45.56130799126797370, 259.0270538473393458 ) ) ;
#43112=EDGE_CURVE ( 'NONE', #16580, #49393, #25989, .T. ) ;
#43113=ORIENTED_EDGE ( 'NONE', *, *, #20314, .T. ) ;
#43114=FACE_OUTER_BOUND ( 'NONE', #70483, .T. ) ;
#43116=VERTEX_POINT ( 'NONE', #19315 ) ;
#43117=CARTESIAN_POINT ( 'NONE',  ( 117.2805452986850412, -39.02698501918706597, 144.6499109901969859 ) ) ;
#43118=VECTOR ( 'NONE', #48453, 1000.000000000000000 ) ;
#43120=AXIS2_PLACEMENT_3D ( 'NONE', #32491, #18421, #38416 ) ;
#43121=VERTEX_POINT ( 'NONE', #60178 ) ;
#43124=DIRECTION ( 'NONE',  ( -4.237773401492740281E-14, 1.000000000000000000, 0.000000000000000000 ) ) ;
#43125=CARTESIAN_POINT ( 'NONE',  ( 102.0670659567350214, -27.97049192634999315, 266.4897909478353881 ) ) ;
#43126=CARTESIAN_POINT ( 'NONE',  ( 20.03715912545818867, -46.82818131006190043, 313.9678068554150059 ) ) ;
#43127=DIRECTION ( 'NONE',  ( 0.7071067811989784069, -0.7071067811741166276, 7.071067811989791923E-16 ) ) ;
#43129=CARTESIAN_POINT ( 'NONE',  ( 111.4154404335798745, -46.20410067450679037, 23.91848241876792969 ) ) ;
#43130=EDGE_CURVE ( 'NONE', #89527, #11288, #27026, .T. ) ;
#43132=VERTEX_POINT ( 'NONE', #4793 ) ;
#43133=VECTOR ( 'NONE', #88967, 1000.000000000000000 ) ;
#43135=AXIS2_PLACEMENT_3D ( 'NONE', #50925, #78670, #37757 ) ;
#43136=VECTOR ( 'NONE', #15357, 1000.000000000000000 ) ;
#43137=CARTESIAN_POINT ( 'NONE',  ( 180.2121375201600131, -29.73316016639650172, -5.074374724088000832 ) ) ;
#43139=EDGE_CURVE ( 'NONE', #81096, #85439, #17308, .T. ) ;
#43140=VERTEX_POINT ( 'NONE', #74283 ) ;
#43141=VECTOR ( 'NONE', #77464, 1000.000000000000000 ) ;
#43142=CARTESIAN_POINT ( 'NONE',  ( 81.30995888129837113, -21.18301917769388254, 1.868341932364300684 ) ) ;
#43143=DIRECTION ( 'NONE',  ( 0.000000000000000000, 0.000000000000000000, 1.000000000000000000 ) ) ;
#43145=PLANE ( 'NONE',  #52077 ) ;
#43147=CARTESIAN_POINT ( 'NONE',  ( 101.8145705177301892, -43.46543587290290134, 231.4724198280769940 ) ) ;
#43148=DIRECTION ( 'NONE',  ( 0.000000000000000000, 0.000000000000000000, -1.000000000000000000 ) ) ;
#43150=CARTESIAN_POINT ( 'NONE',  ( 106.8402339230401452, -48.62808610490878891, 77.56133956162491927 ) ) ;
#43151=VERTEX_POINT ( 'NONE', #47889 ) ;
#43152=CARTESIAN_POINT ( 'NONE',  ( 41.56648329127499153, -36.32844715994070839, 203.6756252759119832 ) ) ;
#43153=EDGE_LOOP ( 'NONE', ( #6790, #31029 ) ) ;
#43154=LINE ( 'NONE', #72228, #36277 ) ;
#43155=CYLINDRICAL_SURFACE ( 'NONE', #48412, 2.750000000000002665 ) ;
#43156=ORIENTED_EDGE ( 'NONE', *, *, #10795, .F. ) ;
#43159=CARTESIAN_POINT ( 'NONE',  ( 25.56670390244832447, -48.82844715994168183, 257.2178068554150059 ) ) ;
#43160=EDGE_CURVE ( 'NONE', #36969, #63446, #39742, .T. ) ;
#43161=LINE ( 'NONE', #64081, #82449 ) ;
#43163=CARTESIAN_POINT ( 'NONE',  ( 107.0664832912739399, -36.72944715994095333, 311.3356252759109566 ) ) ;
#43164=ORIENTED_EDGE ( 'NONE', *, *, #2035, .F. ) ;
#43165=CARTESIAN_POINT ( 'NONE',  ( 108.9893125699443175, -46.99828796752551341, 82.72419670448194040 ) ) ;
#43167=CARTESIAN_POINT ( 'NONE',  ( 142.0664832912740110, -45.72944715994096754, -4.970821333495747396 ) ) ;
#43169=CARTESIAN_POINT ( 'NONE',  ( 25.56670390244797275, -58.35344715994099829, 170.4678068554149775 ) ) ;
#43172=CARTESIAN_POINT ( 'NONE',  ( 194.0371591254575208, -24.89890238294407254, 180.4678068554150343 ) ) ;
#43173=CARTESIAN_POINT ( 'NONE',  ( 109.7248659599222407, -27.00080519107385157, 154.8647919394014423 ) ) ;
#43175=EDGE_CURVE ( 'NONE', #62608, #25721, #26569, .T. ) ;
#43176=CARTESIAN_POINT ( 'NONE',  ( 108.2792189108890568, -26.31750842948725122, 125.9841967044819597 ) ) ;
#43177=AXIS2_PLACEMENT_3D ( 'NONE', #54073, #52275, #67276 ) ;
#43178=CARTESIAN_POINT ( 'NONE',  ( 116.3149231129805941, -32.94053081170188335, 174.1356252759109680 ) ) ;
#43179=DIRECTION ( 'NONE',  ( 1.000000000000000000, 4.163336342344333240E-14, 0.000000000000000000 ) ) ;
#43181=EDGE_CURVE ( 'NONE', #17890, #27372, #14399, .T. ) ;
#43183=CIRCLE ( 'NONE', #24339, 3.250000000000002665 ) ;
#43185=CARTESIAN_POINT ( 'NONE',  ( 102.0969121991173125, -45.15362633196975395, 158.1527681330539963 ) ) ;
#43189=CARTESIAN_POINT ( 'NONE',  ( 110.3395589168170545, -45.98151452051992294, 33.84705384733993583 ) ) ;
#43190=PLANE ( 'NONE',  #74472 ) ;
#43191=DIRECTION ( 'NONE',  ( -1.000000000000000000, 0.000000000000000000, 0.000000000000000000 ) ) ;
#43192=CYLINDRICAL_SURFACE ( 'NONE', #32751, 5.599999999999994316 ) ;
#43193=DIRECTION ( 'NONE',  ( 1.000000000000000000, 4.163336342344333240E-14, 0.000000000000000000 ) ) ;
#43194=FACE_BOUND ( 'NONE', #16382, .T. ) ;
#43195=VECTOR ( 'NONE', #88486, 1000.000000000000000 ) ;
#43196=VECTOR ( 'NONE', #59118, 1000.000000000000000 ) ;
#43197=CARTESIAN_POINT ( 'NONE',  ( 101.1405520526759574, -45.23956608920065037, 237.0803871806729717 ) ) ;
#43198=ORIENTED_EDGE ( 'NONE', *, *, #60133, .F. ) ;
#43199=EDGE_LOOP ( 'NONE', ( #31204, #69347, #26040, #40254 ) ) ;
#43200=CARTESIAN_POINT ( 'NONE',  ( 115.5299003720540014, -39.45574047089768754, 155.0101547344689550 ) ) ;
#43201=AXIS2_PLACEMENT_3D ( 'NONE', #67111, #64111, #31242 ) ;
#43202=DIRECTION ( 'NONE',  ( -1.000000000000000000, -4.163336342344333240E-14, 0.000000000000000000 ) ) ;
#43203=CARTESIAN_POINT ( 'NONE',  ( 114.3823783366371316, -42.62471689273790076, 39.70634521065896649 ) ) ;
#43205=EDGE_CURVE ( 'NONE', #59488, #45550, #32929, .T. ) ;
#43207=FACE_OUTER_BOUND ( 'NONE', #79763, .T. ) ;
#43209=CARTESIAN_POINT ( 'NONE',  ( 165.3359832912747436, -36.32844715993532958, 313.9678068554149490 ) ) ;
#43210=EDGE_CURVE ( 'NONE', #4783, #74866, #63790, .T. ) ;
#43211=DIRECTION ( 'NONE',  ( 0.000000000000000000, 0.000000000000000000, -1.000000000000000000 ) ) ;
#43212=CARTESIAN_POINT ( 'NONE',  ( 99.39760893136102027, -29.69972230079146769, 275.7356252759109907 ) ) ;
#43213=FACE_OUTER_BOUND ( 'NONE', #12289, .T. ) ;
#43214=ORIENTED_EDGE ( 'NONE', *, *, #57465, .T. ) ;
#43215=ORIENTED_EDGE ( 'NONE', *, *, #78860, .F. ) ;
#43216=ADVANCED_FACE ( 'NONE', ( #76063 ), #62431, .F. ) ;
#43219=CARTESIAN_POINT ( 'NONE',  ( 62.03715912545739286, -47.82818131006020934, 180.4678068554151196 ) ) ;
#43220=DIRECTION ( 'NONE',  ( -1.000000000000000078E-15, 1.000000000000000000, 0.000000000000000000 ) ) ;
#43221=AXIS2_PLACEMENT_3D ( 'NONE', #15002, #72201, #23619 ) ;
#43222=CARTESIAN_POINT ( 'NONE',  ( 99.63325261332707328, -43.08637385293071276, 27.88991099019594344 ) ) ;
#43223=CARTESIAN_POINT ( 'NONE',  ( 128.0667039024480118, -50.82844715994100682, 265.9178068554150514 ) ) ;
#43225=ORIENTED_EDGE ( 'NONE', *, *, #77867, .T. ) ;
#43227=DIRECTION ( 'NONE',  ( 1.000000000000000078E-15, -1.000000000000000083E-30, -1.000000000000000000 ) ) ;
#43228=CARTESIAN_POINT ( 'NONE',  ( 104.8412335932644766, -26.50818645216173408, 260.2470538473397710 ) ) ;
#43234=CARTESIAN_POINT ( 'NONE',  ( 112.3828903148906306, -42.92343960232698663, 105.9595189410199652 ) ) ;
#43235=CARTESIAN_POINT ( 'NONE',  ( 117.2133579748808927, -41.17085908628773439, 204.4861014663869696 ) ) ;
#43236=DIRECTION ( 'NONE',  ( -0.08544974978095701279, -0.9963424814100680926, 0.000000000000000000 ) ) ;
#43237=ORIENTED_EDGE ( 'NONE', *, *, #21768, .T. ) ;
#43239=ORIENTED_EDGE ( 'NONE', *, *, #64096, .F. ) ;
#43241=CIRCLE ( 'NONE', #12799, 2.117000000000007987 ) ;
#43243=CARTESIAN_POINT ( 'NONE',  ( 97.81168569434709070, -40.51740311210409828, 127.6359003399277441 ) ) ;
#43246=FACE_BOUND ( 'NONE', #47615, .T. ) ;
#43247=CARTESIAN_POINT ( 'NONE',  ( 97.60785294300944770, -39.98231928252738498, 42.59004589039252409 ) ) ;
#43248=CARTESIAN_POINT ( 'NONE',  ( 115.7032693465968975, -34.00573701374007385, 128.4800388756959819 ) ) ;
#43249=CARTESIAN_POINT ( 'NONE',  ( 101.0739185617116078, -45.28721829360737416, 282.0899109901967563 ) ) ;
#43250=CIRCLE ( 'NONE', #64995, 0.9999999999999800160 ) ;
#43251=CARTESIAN_POINT ( 'NONE',  ( 51.42025729303989579, -33.70561438052008896, 117.4678068554150485 ) ) ;
#43253=VECTOR ( 'NONE', #24341, 1000.000000000000000 ) ;
#43256=AXIS2_PLACEMENT_3D ( 'NONE', #51695, #65778, #3125 ) ;
#43258=LINE ( 'NONE', #70998, #89900 ) ;
#43259=ADVANCED_FACE ( 'NONE', ( #77412 ), #15643, .F. ) ;
#43260=CARTESIAN_POINT ( 'NONE',  ( 32.24491389930098251, -32.11662333284611748, 342.9256252759119548 ) ) ;
#43261=CARTESIAN_POINT ( 'NONE',  ( 98.11178232766683038, -43.28888419983005775, 106.8175300378159704 ) ) ;
#43262=CARTESIAN_POINT ( 'NONE',  ( 104.5776654613874683, -26.56013282928604724, 285.2670538473396391 ) ) ;
#43263=ORIENTED_EDGE ( 'NONE', *, *, #82694, .T. ) ;
#43265=CARTESIAN_POINT ( 'NONE',  ( 99.38138666193238180, -29.68485204926252763, 275.7356252759109907 ) ) ;
#43267=DIRECTION ( 'NONE',  ( 0.000000000000000000, -1.000000000000000000, 0.000000000000000000 ) ) ;
#43268=CARTESIAN_POINT ( 'NONE',  ( 97.93120746083486949, -40.79885511280051702, 27.66041246454429015 ) ) ;
#43269=CYLINDRICAL_SURFACE ( 'NONE', #52038, 0.5000000000000079936 ) ;
#43270=CARTESIAN_POINT ( 'NONE',  ( 20.03715912545639100, -24.42818131006202265, 180.4678068554150911 ) ) ;
#43272=DIRECTION ( 'NONE',  ( 0.000000000000000000, 0.000000000000000000, 1.000000000000000000 ) ) ;
#43275=DIRECTION ( 'NONE',  ( 5.512527431108029424E-15, -1.000000000000000000, 0.000000000000000000 ) ) ;
#43277=PLANE ( 'NONE',  #5743 ) ;
#43281=CARTESIAN_POINT ( 'NONE',  ( 108.0161133123553725, -24.89170165127225332, 265.0127681330534415 ) ) ;
#43282=CARTESIAN_POINT ( 'NONE',  ( 109.4453082753925770, -25.93522777273083335, 175.8918157521009391 ) ) ;
#43283=CARTESIAN_POINT ( 'NONE',  ( 98.40574028604457624, -42.07939390257583767, 7.768006228291934434 ) ) ;
#43285=CARTESIAN_POINT ( 'NONE',  ( 116.3212776292296127, -32.94146857471318413, 287.6356252759109680 ) ) ;
#43286=CARTESIAN_POINT ( 'NONE',  ( 82.11134023506164681, -34.88977106732058076, 7.516154048600878212 ) ) ;
#43288=VECTOR ( 'NONE', #38837, 1000.000000000000000 ) ;
#43289=EDGE_CURVE ( 'NONE', #56032, #2462, #27464, .T. ) ;
#43291=CARTESIAN_POINT ( 'NONE',  ( 182.5667039024459939, -19.82844715994031048, -5.074374724088000832 ) ) ;
#43293=CARTESIAN_POINT ( 'NONE',  ( 114.9272539996656377, -40.07076659875138347, 167.9295626852199632 ) ) ;
#43294=CARTESIAN_POINT ( 'NONE',  ( 134.0664832912740110, -46.42944715994100591, 10.42562527591099553 ) ) ;
#43295=ORIENTED_EDGE ( 'NONE', *, *, #36808, .T. ) ;
#43296=LINE ( 'NONE', #27443, #75094 ) ;
#43297=CARTESIAN_POINT ( 'NONE',  ( 117.3921119255896599, -35.46056622170122807, 189.9241967044829664 ) ) ;
#43298=DIRECTION ( 'NONE',  ( 0.000000000000000000, 0.000000000000000000, 1.000000000000000000 ) ) ;
#43299=DIRECTION ( 'NONE',  ( 1.000000000000000000, 4.299999999999999979E-14, 1.000000000000000078E-15 ) ) ;
#43300=CARTESIAN_POINT ( 'NONE',  ( 162.5667039024470171, -32.29483332968611364, -5.074374724088000832 ) ) ;
#43301=CARTESIAN_POINT ( 'NONE',  ( 110.8691032742908078, -27.48061958891991807, 85.76620976841263655 ) ) ;
#43302=CIRCLE ( 'NONE', #9936, 2.500000000000002220 ) ;
#43303=CARTESIAN_POINT ( 'NONE',  ( 41.56648329127398966, -27.82844715994070484, 198.9256252759119832 ) ) ;
#43304=CARTESIAN_POINT ( 'NONE',  ( 111.5934792397330568, -45.65282444717340127, 97.95005873871468793 ) ) ;
#43305=CARTESIAN_POINT ( 'NONE',  ( 98.20106483660278229, -31.34956418181668880, 125.8803871806729546 ) ) ;
#43306=ORIENTED_EDGE ( 'NONE', *, *, #45559, .F. ) ;
#43307=ORIENTED_EDGE ( 'NONE', *, *, #4153, .F. ) ;
#43308=CONICAL_SURFACE ( 'NONE', #24461, 3.299999999999999822, 0.7853981633974602694 ) ;
#43309=CARTESIAN_POINT ( 'NONE',  ( 106.8749774919903359, -46.80089345537784595, 73.99301187732598351 ) ) ;
#43311=CYLINDRICAL_SURFACE ( 'NONE', #26927, 0.2500000000000002220 ) ;
#43312=CARTESIAN_POINT ( 'NONE',  ( 115.8019334949657804, -41.12891815432276843, 199.4556252759109611 ) ) ;
#43314=CARTESIAN_POINT ( 'NONE',  ( 109.7256335582158897, -27.00101042015257136, 54.86366401989379682 ) ) ;
#43315=CARTESIAN_POINT ( 'NONE',  ( 102.0670441177828849, -27.97050408116591314, 111.4901724250200630 ) ) ;
#43316=EDGE_CURVE ( 'NONE', #29300, #16763, #22456, .T. ) ;
#43318=VECTOR ( 'NONE', #56283, 1000.000000000000114 ) ;
#43320=ADVANCED_FACE ( 'NONE', ( #69255 ), #75333, .T. ) ;
#43322=CARTESIAN_POINT ( 'NONE',  ( 96.72090476913461998, -37.82382852467500811, 126.4099109901969626 ) ) ;
#43323=ORIENTED_EDGE ( 'NONE', *, *, #3038, .T. ) ;
#43327=AXIS2_PLACEMENT_3D ( 'NONE', #36959, #64670, #72822 ) ;
#43329=DIRECTION ( 'NONE',  ( 1.000000000000000000, 4.299999999999999979E-14, 1.000000000000000078E-15 ) ) ;
#43331=CARTESIAN_POINT ( 'NONE',  ( 97.06386241311420804, -37.34254974993516640, 131.3752592778957080 ) ) ;
#43332=CARTESIAN_POINT ( 'NONE',  ( 109.6426267301161346, -46.48019266381861314, 103.7814271469466263 ) ) ;
#43333=CARTESIAN_POINT ( 'NONE',  ( 100.6713832604498577, -30.89818480590637861, 228.5442808457819979 ) ) ;
#43334=DIRECTION ( 'NONE',  ( -1.000000000000000078E-15, 0.000000000000000000, 1.000000000000000000 ) ) ;
#43335=CARTESIAN_POINT ( 'NONE',  ( 97.79409093757406879, -42.74665822538010929, 146.7965776568629508 ) ) ;
#43337=ORIENTED_EDGE ( 'NONE', *, *, #28144, .F. ) ;
#43340=EDGE_CURVE ( 'NONE', #50424, #89909, #34727, .T. ) ;
#43341=LINE ( 'NONE', #36992, #69468 ) ;
#43343=ORIENTED_EDGE ( 'NONE', *, *, #89403, .F. ) ;
#43344=DIRECTION ( 'NONE',  ( -0.9999999853157766072, -0.0001713722456143218888, 0.000000000000000000 ) ) ;
#43345=CARTESIAN_POINT ( 'NONE',  ( 133.0080215814378732, -34.19118199975286387, 8.051357469095956176 ) ) ;
#43346=CARTESIAN_POINT ( 'NONE',  ( 106.0694874169909809, -45.56507127853855366, 278.9187261630399917 ) ) ;
#43347=CARTESIAN_POINT ( 'NONE',  ( 194.0667039024482392, -40.32844715993407192, 129.9678068554150343 ) ) ;
#43348=ORIENTED_EDGE ( 'NONE', *, *, #21601, .F. ) ;
#43349=CARTESIAN_POINT ( 'NONE',  ( 110.9723524473886158, -44.29053194721960551, 9.635625275910937759 ) ) ;
#43350=AXIS2_PLACEMENT_3D ( 'NONE', #9255, #36950, #64658 ) ;
#43351=DIRECTION ( 'NONE',  ( 4.299999999999999979E-14, -1.000000000000000000, 0.000000000000000000 ) ) ;
#43352=ORIENTED_EDGE ( 'NONE', *, *, #54779, .T. ) ;
#43353=VERTEX_POINT ( 'NONE', #83336 ) ;
#43354=CARTESIAN_POINT ( 'NONE',  ( 115.0521663075109444, -42.80382784462421597, 113.3088412358543309 ) ) ;
#43357=CARTESIAN_POINT ( 'NONE',  ( 113.5315931691687439, -43.38514287343249265, 266.0080903695914003 ) ) ;
#43358=CARTESIAN_POINT ( 'NONE',  ( 107.9200767535970584, -47.17740107552570805, 177.6413395616249886 ) ) ;
#43359=CARTESIAN_POINT ( 'NONE',  ( 102.9221092647373865, -27.14930527916904168, 155.4013395616249795 ) ) ;
#43360=FACE_OUTER_BOUND ( 'NONE', #80385, .T. ) ;
#43361=DIRECTION ( 'NONE',  ( 0.7071067811864676367, 0.7071067811866273978, 7.071067811864981309E-16 ) ) ;
#43362=CARTESIAN_POINT ( 'NONE',  ( 115.3879430501622636, -30.44965457351534255, 215.3413395616249773 ) ) ;
#43364=CARTESIAN_POINT ( 'NONE',  ( 25.56670390244719471, -42.82844715994178131, 170.7178068554150627 ) ) ;
#43365=VERTEX_POINT ( 'NONE', #63333 ) ;
#43369=ORIENTED_EDGE ( 'NONE', *, *, #82529, .T. ) ;
#43370=EDGE_CURVE ( 'NONE', #42491, #67284, #28822, .T. ) ;
#43371=AXIS2_PLACEMENT_3D ( 'NONE', #89497, #34960, #42218 ) ;
#43372=CARTESIAN_POINT ( 'NONE',  ( 113.1812204092734220, -26.51970732500450012, 204.6470538473399756 ) ) ;
#43373=EDGE_LOOP ( 'NONE', ( #13622, #40968, #13674, #44197 ) ) ;
#43374=CARTESIAN_POINT ( 'NONE',  ( 117.8008629928215782, -34.09274860618955216, 164.0061014663869798 ) ) ;
#43375=PLANE ( 'NONE',  #68913 ) ;
#43376=ADVANCED_FACE ( 'NONE', ( #82902 ), #56504, .T. ) ;
#43381=CARTESIAN_POINT ( 'NONE',  ( 112.6519946835718144, -45.50616226388157770, 259.0270538473393458 ) ) ;
#43382=LINE ( 'NONE', #21173, #36540 ) ;
#43388=CARTESIAN_POINT ( 'NONE',  ( 98.34985889887454391, -31.65658483259429445, 256.9064586113552764 ) ) ;
#43389=CYLINDRICAL_SURFACE ( 'NONE', #69475, 9.999999999999998224 ) ;
#43390=CARTESIAN_POINT ( 'NONE',  ( 100.2183167550744685, -45.46532142855728864, 277.0594347997204068 ) ) ;
#43391=ORIENTED_EDGE ( 'NONE', *, *, #18321, .F. ) ;
#43393=CARTESIAN_POINT ( 'NONE',  ( 116.8272927809998123, -43.49410631979629471, 163.3441967044829823 ) ) ;
#43394=CARTESIAN_POINT ( 'NONE',  ( 116.1236770753320542, -29.08733643602844054, 70.38419670448192278 ) ) ;
#43395=CARTESIAN_POINT ( 'NONE',  ( 101.9632951345543148, -45.91070444983295573, 183.1727681330539781 ) ) ;
#43398=DIRECTION ( 'NONE',  ( 0.000000000000000000, 0.000000000000000000, -1.000000000000000000 ) ) ;
#43400=DIRECTION ( 'NONE',  ( -4.237773401492740281E-14, 1.000000000000000000, 0.000000000000000000 ) ) ;
#43401=CARTESIAN_POINT ( 'NONE',  ( 104.4899544625536976, -26.97880758202075668, 70.28145860838544934 ) ) ;
#43403=EDGE_LOOP ( 'NONE', ( #45358, #49453, #46866, #34997 ) ) ;
#43405=EDGE_CURVE ( 'NONE', #40009, #20465, #20662, .T. ) ;
#43406=ORIENTED_EDGE ( 'NONE', *, *, #32428, .T. ) ;
#43407=ORIENTED_EDGE ( 'NONE', *, *, #5307, .F. ) ;
#43409=ORIENTED_EDGE ( 'NONE', *, *, #85672, .F. ) ;
#43410=CARTESIAN_POINT ( 'NONE',  ( 98.66494773507974969, -43.87633619481167102, 72.89943479972099283 ) ) ;
#43412=PLANE ( 'NONE',  #32558 ) ;
#43414=DIRECTION ( 'NONE',  ( -0.9999999853157766072, -0.0001713722456133601202, 9.999999853157765648E-16 ) ) ;
#43415=CARTESIAN_POINT ( 'NONE',  ( 98.43953089107090193, -39.48415132980177589, 280.9828960185531059 ) ) ;
#43416=EDGE_LOOP ( 'NONE', ( #36103, #86823, #52136, #13562 ) ) ;
#43417=AXIS2_PLACEMENT_3D ( 'NONE', #67454, #73827, #88816 ) ;
#43420=CARTESIAN_POINT ( 'NONE',  ( 100.8874678886941894, -44.70022137831526265, 107.0522919429965754 ) ) ;
#43421=CARTESIAN_POINT ( 'NONE',  ( 41.56648329127398966, -27.82844715994070484, 198.9256252759119832 ) ) ;
#43423=CARTESIAN_POINT ( 'NONE',  ( 116.3212776292269837, -32.94146857470673240, 74.13562527591093954 ) ) ;
#43425=CARTESIAN_POINT ( 'NONE',  ( 107.0664832912739399, -36.72944715994095333, 247.7440089327910755 ) ) ;
#43426=CARTESIAN_POINT ( 'NONE',  ( 139.7494832912729805, -1.929447159941395817, 342.9256252759109316 ) ) ;
#43428=CARTESIAN_POINT ( 'NONE',  ( 100.4929927897290014, -27.87207479535954135, 35.59657765686397113 ) ) ;
#43430=ORIENTED_EDGE ( 'NONE', *, *, #19752, .F. ) ;
#43433=CARTESIAN_POINT ( 'NONE',  ( 73.06670390244801183, -48.82844715994099971, 198.9178068554149945 ) ) ;
#43434=CARTESIAN_POINT ( 'NONE',  ( 107.7548360709104855, -28.10233318731983232, 112.8433284648289430 ) ) ;
#43435=CONICAL_SURFACE ( 'NONE', #81213, 3.299999999999999822, 0.7853981633974602694 ) ;
#43436=VECTOR ( 'NONE', #43344, 1000.000000000000114 ) ;
#43437=DIRECTION ( 'NONE',  ( 0.7071067811989676377, 0.7071067811741275078, 7.071067811989982236E-16 ) ) ;
#43439=CARTESIAN_POINT ( 'NONE',  ( 177.3246001664173264, -48.34074026909179622, 249.9678068554149775 ) ) ;
#43440=ORIENTED_EDGE ( 'NONE', *, *, #60749, .T. ) ;
#43445=EDGE_LOOP ( 'NONE', ( #1219, #70017 ) ) ;
#43446=VERTEX_POINT ( 'NONE', #24677 ) ;
#43449=CARTESIAN_POINT ( 'NONE',  ( 101.8133294234851860, -44.51716929413077395, 148.5234880678019351 ) ) ;
#43450=DIRECTION ( 'NONE',  ( -2.999999999999999839E-15, 1.000000000000000000, -2.999999999999999900E-30 ) ) ;
#43451=AXIS2_PLACEMENT_3D ( 'NONE', #2266, #49036, #5725 ) ;
#43452=CARTESIAN_POINT ( 'NONE',  ( 109.7757303681923418, -47.46933477669593771, 88.78514908543493789 ) ) ;
#43453=CARTESIAN_POINT ( 'NONE',  ( 97.81944854975840542, -40.53634262228253959, 16.63725235658089119 ) ) ;
#43454=ORIENTED_EDGE ( 'NONE', *, *, #30524, .T. ) ;
#43455=AXIS2_PLACEMENT_3D ( 'NONE', #4660, #89131, #5108 ) ;
#43456=ORIENTED_EDGE ( 'NONE', *, *, #36386, .F. ) ;
#43458=CONICAL_SURFACE ( 'NONE', #46302, 1.571100913904471819, 1.047197551196592302 ) ;
#43459=CARTESIAN_POINT ( 'NONE',  ( 112.7537747436706184, -27.22417719680832704, 54.65943479971996055 ) ) ;
#43460=EDGE_LOOP ( 'NONE', ( #78702, #48415, #48439, #52953 ) ) ;
#43461=CARTESIAN_POINT ( 'NONE',  ( 112.1705331031350994, -27.62378402076933526, 34.66991099019695355 ) ) ;
#43462=CARTESIAN_POINT ( 'NONE',  ( 111.4263534857568771, -47.77543206737910708, 168.8756252759109486 ) ) ;
#43465=CARTESIAN_POINT ( 'NONE',  ( 97.61704402414061121, -30.99515748980318719, 121.8803871806729546 ) ) ;
#43466=CARTESIAN_POINT ( 'NONE',  ( 97.81171236172070849, -40.51746256574213589, 261.6350867226296941 ) ) ;
#43467=ORIENTED_EDGE ( 'NONE', *, *, #77980, .F. ) ;
#43469=ORIENTED_EDGE ( 'NONE', *, *, #68047, .F. ) ;
#43471=EDGE_LOOP ( 'NONE', ( #74365, #41247, #58917, #59374 ) ) ;
#43472=ORIENTED_EDGE ( 'NONE', *, *, #16921, .F. ) ;
#43473=CARTESIAN_POINT ( 'NONE',  ( 41.56648329127399677, -9.303447159940999356, 256.8086252759120498 ) ) ;
#43474=CARTESIAN_POINT ( 'NONE',  ( 45.76696975232739817, -48.62818131006041256, 180.4678068554150911 ) ) ;
#43475=CARTESIAN_POINT ( 'NONE',  ( 96.83338659586634378, -38.89961736000394410, 31.49276813305495892 ) ) ;
#43479=DIRECTION ( 'NONE',  ( 0.000000000000000000, 0.000000000000000000, -1.000000000000000000 ) ) ;
#43480=CARTESIAN_POINT ( 'NONE',  ( 118.0115280580378396, -34.77548253539073642, 48.96705384733996169 ) ) ;
#43481=B_SPLINE_CURVE_WITH_KNOTS ( 'NONE', 3,
 ( #45801, #73526, #32635, #66713, #87613, #4500, #25377, #53046, #80813, #60333, #55300, #54847, #63479, #76673, #28972, #55738, #21259, #14454, #48929, #77563, #62585, #56656, #84403, #41673, #83058, #63029, #48473, #83486, #82611 ),
 .UNSPECIFIED., .F., .F.,
 ( 4, 2, 2, 2, 2, 2, 2, 2, 2, 2, 1, 1, 1, 1, 1, 2, 4 ),
 ( 0.000000000000000000, 0.06250785763960332864, 0.1250157152792066573, 0.1875235729188099720, 0.2500314305584133145, 0.3125392881980166848, 0.3750471458376199441, 0.4375550034772233143, 0.4688089322970249717, 0.4844358967069258837, 0.4922493789118762009, 0.4961561200143512762, 0.4981094905655886751, 0.4990861758412074023, 0.4995745184790165716, 0.4998186897979214338, 0.5000628611168262960 ),
 .UNSPECIFIED. ) ;
#43482=DIRECTION ( 'NONE',  ( -0.0001713722456127291687, 0.9999999853157766072, 1.713722456127291814E-19 ) ) ;
#43483=CARTESIAN_POINT ( 'NONE',  ( 97.97553865104319470, -30.48296430071277641, 161.8594347997199918 ) ) ;
#43484=CARTESIAN_POINT ( 'NONE',  ( 100.9546728049728443, -28.70702573201124252, 71.59395860986847993 ) ) ;
#43488=CIRCLE ( 'NONE', #21737, 2.030000000000003801 ) ;
#43493=CARTESIAN_POINT ( 'NONE',  ( 182.5667039024477276, -33.35206098992057377, 237.4678068554150059 ) ) ;
#43494=CARTESIAN_POINT ( 'NONE',  ( 97.63486134215516188, -41.27380337981261960, 171.6841967044819626 ) ) ;
#43495=ORIENTED_EDGE ( 'NONE', *, *, #87704, .F. ) ;
#43497=CARTESIAN_POINT ( 'NONE',  ( 112.4229354917722787, -46.42447813297522430, 248.9661014663869878 ) ) ;
#43498=CARTESIAN_POINT ( 'NONE',  ( 98.26973918885833825, -28.71518450514261289, 76.73848241876795839 ) ) ;
#43499=CARTESIAN_POINT ( 'NONE',  ( 116.3186249068867539, -32.94868901193379429, 250.1356252759109395 ) ) ;
#43500=DIRECTION ( 'NONE',  ( 5.512527431108029424E-15, -1.000000000000000000, 0.000000000000000000 ) ) ;
#43501=DIRECTION ( 'NONE',  ( 0.000000000000000000, 0.000000000000000000, 1.000000000000000000 ) ) ;
#43503=VECTOR ( 'NONE', #49396, 1000.000000000000000 ) ;
#43506=VERTEX_POINT ( 'NONE', #31476 ) ;
#43507=VECTOR ( 'NONE', #78699, 1000.000000000000000 ) ;
#43510=DIRECTION ( 'NONE',  ( 1.000000000000000078E-15, 0.000000000000000000, -1.000000000000000000 ) ) ;
#43511=CARTESIAN_POINT ( 'NONE',  ( 96.77613930368880801, -40.76464245898888095, 242.6118157521009664 ) ) ;
#43513=CARTESIAN_POINT ( 'NONE',  ( 131.4961476553979765, -35.75123073100127158, 2.855912073278335406 ) ) ;
#43515=EDGE_CURVE ( 'NONE', #71741, #231, #29710, .T. ) ;
#43516=CIRCLE ( 'NONE', #84213, 4.749999999999976907 ) ;
#43517=DIRECTION ( 'NONE',  ( 0.000000000000000000, 1.000000000000000000, 0.000000000000000000 ) ) ;
#43518=CARTESIAN_POINT ( 'NONE',  ( 51.56670390244899238, -32.29483332968450782, -5.074374724088000832 ) ) ;
#43520=B_SPLINE_CURVE_WITH_KNOTS ( 'NONE', 3,
 ( #70426, #14572, #22730, #22279, #78600, #77241, #15011, #16352, #49954, #50408, #7742, #8198, #44030, #77686, #49053, #35435, #15471, #71767, #42247, #64946, #69976, #37240, #63151, #43142, #70883, #30429, #8653, #36348, #64060, #1836 ),
 .UNSPECIFIED., .F., .F.,
 ( 4, 2, 2, 2, 1, 2, 2, 2, 2, 2, 2, 2, 1, 2, 2, 4 ),
 ( 0.5000000000000000000, 0.5624999999999789058, 0.5937499999999682476, 0.6093749999999633626, 0.6171874999999610312, 0.6210937499999602540, 0.6249999999999593658, 0.6874999999999669154, 0.7187499999999722444, 0.7499999999999774625, 0.8124999999999885647, 0.8437499999999955591, 0.8593750000000006661, 0.8671875000000031086, 0.8750000000000056621, 1.000000000000000000 ),
 .UNSPECIFIED. ) ;
#43521=CARTESIAN_POINT ( 'NONE',  ( 97.33091451745008271, -32.84266655496112008, 41.02419670448193045 ) ) ;
#43523=EDGE_CURVE ( 'NONE', #52647, #67095, #58302, .T. ) ;
#43524=ORIENTED_EDGE ( 'NONE', *, *, #39714, .T. ) ;
#43525=ORIENTED_EDGE ( 'NONE', *, *, #28775, .T. ) ;
#43528=EDGE_CURVE ( 'NONE', #66670, #53468, #64235, .T. ) ;
#43529=CARTESIAN_POINT ( 'NONE',  ( 100.5669465097398358, -44.03830869352244548, 262.9984824187674235 ) ) ;
#43531=CARTESIAN_POINT ( 'NONE',  ( 164.9190312289439930, -35.91149509761220315, -5.074374724088000832 ) ) ;
#43532=CARTESIAN_POINT ( 'NONE',  ( 116.7274023843878581, -38.25590632018514725, 109.7013395616249767 ) ) ;
#43535=ORIENTED_EDGE ( 'NONE', *, *, #78784, .T. ) ;
#43538=VERTEX_POINT ( 'NONE', #24238 ) ;
#43539=CIRCLE ( 'NONE', #4397, 0.4999999999999994449 ) ;
#43541=CARTESIAN_POINT ( 'NONE',  ( 114.6306032519149198, -32.52409173292234357, 27.06047132197198124 ) ) ;
#43542=FACE_OUTER_BOUND ( 'NONE', #26946, .T. ) ;
#43543=DIRECTION ( 'NONE',  ( -6.938893903907222067E-15, -1.000000000000000000, 0.000000000000000000 ) ) ;
#43546=AXIS2_PLACEMENT_3D ( 'NONE', #57628, #50818, #30382 ) ;
#43547=CARTESIAN_POINT ( 'NONE',  ( 19.56670390244796920, -48.82844715994099971, 20.91780685541479912 ) ) ;
#43548=ADVANCED_FACE ( 'NONE', ( #16977 ), #64676, .F. ) ;
#43551=CARTESIAN_POINT ( 'NONE',  ( 117.5955728976552166, -42.16808282502534411, 93.44705384733897802 ) ) ;
#43552=ORIENTED_EDGE ( 'NONE', *, *, #72373, .T. ) ;
#43553=EDGE_CURVE ( 'NONE', #28735, #49139, #50587, .T. ) ;
#43554=CARTESIAN_POINT ( 'NONE',  ( 97.39259002536323351, -35.90094442973985167, 35.68099125664797810 ) ) ;
#43556=VECTOR ( 'NONE', #78742, 1000.000000000000000 ) ;
#43557=CARTESIAN_POINT ( 'NONE',  ( 75.26949937496598864, -71.54137415153812185, 361.9756252759101471 ) ) ;
#43558=CARTESIAN_POINT ( 'NONE',  ( 107.8656169629272483, -46.51081515578112402, 177.6413395616259834 ) ) ;
#43560=DIRECTION ( 'NONE',  ( 1.000000000000000000, -2.914335439641033394E-13, 0.000000000000000000 ) ) ;
#43564=CARTESIAN_POINT ( 'NONE',  ( 113.7840377202001036, -29.05235663984046823, 285.5032443235299979 ) ) ;
#43565=VECTOR ( 'NONE', #74009, 999.9999999999998863 ) ;
#43566=VERTEX_POINT ( 'NONE', #17421 ) ;
#43567=DIRECTION ( 'NONE',  ( 0.7071067811865171526, 0.7071067811865779928, 7.071067811865164719E-16 ) ) ;
#43569=CARTESIAN_POINT ( 'NONE',  ( 109.5186955991938191, -46.90685520642291806, 128.7641967044819751 ) ) ;
#43570=CARTESIAN_POINT ( 'NONE',  ( 172.5667039024478413, -36.32844715993500273, 249.9678068554149775 ) ) ;
#43571=ORIENTED_EDGE ( 'NONE', *, *, #56847, .F. ) ;
#43572=ORIENTED_EDGE ( 'NONE', *, *, #82410, .F. ) ;
#43573=ORIENTED_EDGE ( 'NONE', *, *, #39075, .F. ) ;
#43575=CARTESIAN_POINT ( 'NONE',  ( 63.06670390244736524, -24.92844715994017690, 249.9678068554150343 ) ) ;
#43576=DIRECTION ( 'NONE',  ( 3.999999999999999995E-14, -1.000000000000000000, 4.100000000000000342E-29 ) ) ;
#43579=LINE ( 'NONE', #44470, #17115 ) ;
#43580=CARTESIAN_POINT ( 'NONE',  ( 118.5708186345730724, -33.89864261627929665, 10.01848241876795953 ) ) ;
#43581=DIRECTION ( 'NONE',  ( 0.000000000000000000, 0.000000000000000000, -1.000000000000000000 ) ) ;
#43583=CARTESIAN_POINT ( 'NONE',  ( 163.0667039024476423, -33.35206098992141222, 313.9678068554149490 ) ) ;
#43585=CARTESIAN_POINT ( 'NONE',  ( 46.32460016641727663, -48.34074026909785005, 249.9678068554150343 ) ) ;
#43586=ORIENTED_EDGE ( 'NONE', *, *, #49533, .T. ) ;
#43587=ORIENTED_EDGE ( 'NONE', *, *, #60447, .F. ) ;
#43588=DIRECTION ( 'NONE',  ( 2.900000000000000265E-14, -2.000000000000000155E-15, 1.000000000000000000 ) ) ;
#43589=DIRECTION ( 'NONE',  ( 1.000000000000000000, 0.000000000000000000, 0.000000000000000000 ) ) ;
#43590=CARTESIAN_POINT ( 'NONE',  ( 83.06670390244804025, -42.21678055153920184, 207.5838068554169809 ) ) ;
#43591=CARTESIAN_POINT ( 'NONE',  ( 139.7494832912729805, -71.52944715994142655, 361.9756252759109998 ) ) ;
#43592=CARTESIAN_POINT ( 'NONE',  ( 172.5664832912740110, -18.82844715994099971, 258.9256252759120116 ) ) ;
#43593=AXIS2_PLACEMENT_3D ( 'NONE', #71302, #42655, #36770 ) ;
#43594=CARTESIAN_POINT ( 'NONE',  ( 111.9487353400944158, -44.35678517904902662, 217.4400388756959615 ) ) ;
#43595=DIRECTION ( 'NONE',  ( -1.000000000000000000, -3.999999999999999995E-14, -1.000000000000000078E-15 ) ) ;
#43596=CARTESIAN_POINT ( 'NONE',  ( 96.21590750669005843, -38.71157422997261932, 47.48229194257797303 ) ) ;
#43598=CARTESIAN_POINT ( 'NONE',  ( 113.3690198962888758, -27.59211078819982887, 89.60800622829195561 ) ) ;
#43599=ORIENTED_EDGE ( 'NONE', *, *, #7325, .T. ) ;
#43600=FACE_OUTER_BOUND ( 'NONE', #24044, .T. ) ;
#43602=AXIS2_PLACEMENT_3D ( 'NONE', #46062, #86994, #37500 ) ;
#43603=CARTESIAN_POINT ( 'NONE',  ( 107.0664832912739968, -36.72944715994100306, 287.6356252759109680 ) ) ;
#43604=CARTESIAN_POINT ( 'NONE',  ( 97.06141937736202863, -37.99914660572866154, 277.4274653756244220 ) ) ;
#43606=LINE ( 'NONE', #56790, #67916 ) ;
#43608=DIRECTION ( 'NONE',  ( -9.351236661543306751E-17, 3.725950533538267165E-29, 1.000000000000000000 ) ) ;
#43610=VECTOR ( 'NONE', #37651, 1000.000000000000000 ) ;
#43613=CARTESIAN_POINT ( 'NONE',  ( 96.01222827763220380, -41.06966167057572648, 96.62419670448197451 ) ) ;
#43614=CARTESIAN_POINT ( 'NONE',  ( 181.5667039024459939, -22.48495420874030515, 342.9256252759119548 ) ) ;
#43615=LINE ( 'NONE', #8681, #33613 ) ;
#43616=ADVANCED_FACE ( 'NONE', ( #65566 ), #72828, .T. ) ;
#43618=ORIENTED_EDGE ( 'NONE', *, *, #89197, .T. ) ;
#43619=B_SPLINE_CURVE_WITH_KNOTS ( 'NONE', 3,
 ( #28615, #35874, #1370, #83595, #15895, #42232, #70867, #77226, #34974, #85403, #84508, #22715, #21821, #29521, #69512, #50847, #14998, #22266 ),
 .UNSPECIFIED., .F., .F.,
 ( 4, 2, 2, 2, 2, 2, 2, 2, 4 ),
 ( 0.4999999970439366614, 0.5624999974134445857, 0.6249999977829525655, 0.6874999981524604342, 0.7499999985219683030, 0.8124999988914762827, 0.8749999992609842625, 0.9374999996304921313, 1.000000000000000000 ),
 .UNSPECIFIED. ) ;
#43621=LINE ( 'NONE', #83643, #61989 ) ;
#43622=DIRECTION ( 'NONE',  ( 0.000000000000000000, 1.000000000000000000, 0.000000000000000000 ) ) ;
#43623=VECTOR ( 'NONE', #48781, 1000.000000000000000 ) ;
#43624=CARTESIAN_POINT ( 'NONE',  ( 143.0664832912740110, -18.82844715994099971, -5.074374724088000832 ) ) ;
#43625=VECTOR ( 'NONE', #55451, 1000.000000000000000 ) ;
#43628=EDGE_CURVE ( 'NONE', #25323, #28403, #38743, .T. ) ;
#43629=DIRECTION ( 'NONE',  ( 0.0001211784769727619030, -0.7071067708032375831, -0.7071067811865434649 ) ) ;
#43630=DIRECTION ( 'NONE',  ( -0.000000000000000000, 1.000000000000000000, 0.000000000000000000 ) ) ;
#43631=DIRECTION ( 'NONE',  ( -0.7071067811734105257, 0.7071067811996846197, 0.000000000000000000 ) ) ;
#43632=VECTOR ( 'NONE', #25862, 1000.000000000000000 ) ;
#43633=EDGE_CURVE ( 'NONE', #13081, #32398, #81007, .T. ) ;
#43637=CARTESIAN_POINT ( 'NONE',  ( 102.2986265273211615, -45.30740241592380357, 183.1727681330529833 ) ) ;
#43638=CIRCLE ( 'NONE', #21946, 0.9999999999999800160 ) ;
#43640=ORIENTED_EDGE ( 'NONE', *, *, #79294, .F. ) ;
#43641=CARTESIAN_POINT ( 'NONE',  ( 102.3890460933095454, -47.58756240099337731, 283.2527681330539053 ) ) ;
#43642=CYLINDRICAL_SURFACE ( 'NONE', #41064, 0.5000000000000104361 ) ;
#43644=DIRECTION ( 'NONE',  ( 0.7071067811866279529, -0.7071067811864671926, 7.071067811866286874E-16 ) ) ;
#43645=CARTESIAN_POINT ( 'NONE',  ( 101.9927642735531919, -45.44554305791272242, 12.15655162758104701 ) ) ;
#43646=AXIS2_PLACEMENT_3D ( 'NONE', #38909, #10757, #66166 ) ;
#43647=EDGE_CURVE ( 'NONE', #5214, #65668, #50750, .T. ) ;
#43648=CARTESIAN_POINT ( 'NONE',  ( 97.06104264810085169, -37.99626338996256436, 31.42750358927145271 ) ) ;
#43649=CARTESIAN_POINT ( 'NONE',  ( 110.8764511561472546, -27.72125199330407241, 244.7584824187689492 ) ) ;
#43651=ORIENTED_EDGE ( 'NONE', *, *, #8569, .F. ) ;
#43652=ADVANCED_FACE ( 'NONE', ( #46437 ), #88708, .F. ) ;
#43653=CARTESIAN_POINT ( 'NONE',  ( 109.6768956016245227, -27.70380185851407973, 211.2720594963729752 ) ) ;
#43654=CARTESIAN_POINT ( 'NONE',  ( 115.7848594079097211, -41.79936060917356144, 54.40633938901413558 ) ) ;
#43655=CARTESIAN_POINT ( 'NONE',  ( 100.4594818976507753, -42.68004899263244312, 53.34158330589694685 ) ) ;
#43657=B_SPLINE_CURVE_WITH_KNOTS ( 'NONE', 3,
 ( #79321, #50694, #71609, #2114, #3889, #31139, #17080, #16635, #30268, #44768, #52008, #10692, #23467, #37079, #65661, #51136, #58837, #16197 ),
 .UNSPECIFIED., .F., .F.,
 ( 4, 2, 2, 2, 2, 2, 2, 2, 4 ),
 ( 0.5000000001806115257, 0.5625000001580351405, 0.6250000001354586443, 0.6875000001128821481, 0.7500000000903057629, 0.8125000000677293777, 0.8750000000451528814, 0.9375000000225763852, 1.000000000000000000 ),
 .UNSPECIFIED. ) ;
#43658=VECTOR ( 'NONE', #83260, 1000.000000000000000 ) ;
#43659=DIRECTION ( 'NONE',  ( 0.0001713722456134502174, -0.9999999853157766072, 0.000000000000000000 ) ) ;
#43660=CYLINDRICAL_SURFACE ( 'NONE', #76338, 3.250000000000002665 ) ;
#43663=CARTESIAN_POINT ( 'NONE',  ( 37.03715912545347777, -48.62818131006128652, 129.9678068554150911 ) ) ;
#43664=CARTESIAN_POINT ( 'NONE',  ( 97.80786240601167947, -40.50806667358143898, 37.63452979473162685 ) ) ;
#43665=CARTESIAN_POINT ( 'NONE',  ( 110.8089421659425824, -26.35361831834155311, 249.7889586092445882 ) ) ;
#43667=VERTEX_POINT ( 'NONE', #74169 ) ;
#43668=ORIENTED_EDGE ( 'NONE', *, *, #69173, .F. ) ;
#43670=CARTESIAN_POINT ( 'NONE',  ( 112.0659116168554164, -45.48839626386907042, 82.98979194206674492 ) ) ;
#43671=CYLINDRICAL_SURFACE ( 'NONE', #15732, 10.00000000000000711 ) ;
#43672=FACE_OUTER_BOUND ( 'NONE', #67074, .T. ) ;
#43674=EDGE_CURVE ( 'NONE', #66320, #87303, #52780, .T. ) ;
#43676=CARTESIAN_POINT ( 'NONE',  ( 115.0479362680065663, -42.38275094372907859, 49.33562527591095659 ) ) ;
#43680=CARTESIAN_POINT ( 'NONE',  ( 114.1199461662357919, -46.31379764262941023, 29.08133956162595268 ) ) ;
#43681=LINE ( 'NONE', #36443, #72920 ) ;
#43682=CARTESIAN_POINT ( 'NONE',  ( 105.3166869522846838, -26.42980843014500181, 15.20991099019697401 ) ) ;
#43683=ORIENTED_EDGE ( 'NONE', *, *, #18573, .T. ) ;
#43685=CARTESIAN_POINT ( 'NONE',  ( 99.50485981225885723, -43.30594324741348089, 17.89604700636049017 ) ) ;
#43687=CARTESIAN_POINT ( 'NONE',  ( 104.1662843248667230, -44.88357317080683373, 100.1347570362589892 ) ) ;
#43688=CARTESIAN_POINT ( 'NONE',  ( 117.9552932246042332, -34.69990928640298478, 199.9851490854349549 ) ) ;
#43689=CIRCLE ( 'NONE', #23434, 4.750000000000004441 ) ;
#43690=DIRECTION ( 'NONE',  ( -3.999999999999999995E-14, 1.000000000000000000, -4.100000000000000342E-29 ) ) ;
#43691=VERTEX_POINT ( 'NONE', #88263 ) ;
#43692=DIRECTION ( 'NONE',  ( 0.000000000000000000, 0.000000000000000000, 1.000000000000000000 ) ) ;
#43693=VERTEX_POINT ( 'NONE', #54584 ) ;
#43694=CIRCLE ( 'NONE', #59632, 2.750000000000002665 ) ;
#43696=EDGE_CURVE ( 'NONE', #68029, #22204, #53689, .T. ) ;
#43697=DIRECTION ( 'NONE',  ( 0.9068632946707807507, -0.4214249218767881500, 9.068605531941956314E-16 ) ) ;
#43698=ORIENTED_EDGE ( 'NONE', *, *, #23157, .T. ) ;
#43699=VERTEX_POINT ( 'NONE', #60066 ) ;
#43700=LINE ( 'NONE', #49613, #29516 ) ;
#43701=CARTESIAN_POINT ( 'NONE',  ( 97.70650073344890529, -40.25115704673319073, 42.61283759994312703 ) ) ;
#43702=CARTESIAN_POINT ( 'NONE',  ( 103.8778598771455677, -28.80550795996352420, 129.8038483995049432 ) ) ;
#43703=AXIS2_PLACEMENT_3D ( 'NONE', #54524, #26404, #75461 ) ;
#43704=CARTESIAN_POINT ( 'NONE',  ( 115.9256476412969192, -30.08033833575881033, 264.3508633711492735 ) ) ;
#43708=VERTEX_POINT ( 'NONE', #46879 ) ;
#43710=CARTESIAN_POINT ( 'NONE',  ( 53.35959712126277310, -48.62134037875357251, 300.4678068554150059 ) ) ;
#43712=EDGE_CURVE ( 'NONE', #65595, #85915, #67798, .T. ) ;
#43713=CARTESIAN_POINT ( 'NONE',  ( 112.8260979389708183, -47.14365076028245483, 102.9784824187679817 ) ) ;
#43714=CARTESIAN_POINT ( 'NONE',  ( 116.6223143332234997, -42.37736834728454483, 283.4137205140060018 ) ) ;
#43716=CARTESIAN_POINT ( 'NONE',  ( 115.7763152052227156, -31.00006163510664337, 254.2899109901966028 ) ) ;
#43717=CARTESIAN_POINT ( 'NONE',  ( 97.81168731305311326, -40.51740136754563082, 36.63591984386916067 ) ) ;
#43719=CARTESIAN_POINT ( 'NONE',  ( 101.1247409750737631, -44.88967807114817532, 28.07730664055660696 ) ) ;
#43720=ADVANCED_FACE ( 'NONE', ( #80546 ), #33279, .F. ) ;
#43721=DIRECTION ( 'NONE',  ( 2.900000000000000265E-14, -2.000000000000000155E-15, 1.000000000000000000 ) ) ;
#43723=DIRECTION ( 'NONE',  ( -1.000000000000000000, 0.000000000000000000, 0.000000000000000000 ) ) ;
#43725=DIRECTION ( 'NONE',  ( 1.000000000000000078E-15, -1.000000000000000083E-30, -1.000000000000000000 ) ) ;
#43726=AXIS2_PLACEMENT_3D ( 'NONE', #70229, #64320, #8003 ) ;
#43727=EDGE_CURVE ( 'NONE', #30159, #82436, #81193, .T. ) ;
#43730=CARTESIAN_POINT ( 'NONE',  ( 101.9937722986115176, -45.44616494378649918, 162.1562847702247154 ) ) ;
#43732=ADVANCED_FACE ( 'NONE', ( #40536 ), #61419, .F. ) ;
#43733=CARTESIAN_POINT ( 'NONE',  ( 51.06648329127400388, -18.82844715994099971, 333.4006252759120343 ) ) ;
#43734=CARTESIAN_POINT ( 'NONE',  ( 109.6227372377152847, -25.10643708164309018, 29.90419670448196854 ) ) ;
#43735=CARTESIAN_POINT ( 'NONE',  ( 117.4572939498068820, -40.49840382496243052, 169.5375300378159693 ) ) ;
#43736=CARTESIAN_POINT ( 'NONE',  ( 111.4988423704183020, -26.55354146975621177, 280.7375300378156453 ) ) ;
#43739=DIRECTION ( 'NONE',  ( 4.299999999999999979E-14, -1.000000000000000000, 0.000000000000000000 ) ) ;
#43740=CARTESIAN_POINT ( 'NONE',  ( 82.27770840670791586, -35.08426318373102504, 2.472582314369259571 ) ) ;
#43741=ADVANCED_FACE ( 'NONE', ( #59621, #45987 ), #73719, .F. ) ;
#43742=CIRCLE ( 'NONE', #55336, 0.2999999999999943823 ) ;
#43744=DIRECTION ( 'NONE',  ( -0.9254794337955620787, -0.3787978585227822492, 0.000000000000000000 ) ) ;
#43745=ORIENTED_EDGE ( 'NONE', *, *, #60857, .T. ) ;
#43746=EDGE_CURVE ( 'NONE', #49287, #79347, #29155, .T. ) ;
#43747=CARTESIAN_POINT ( 'NONE',  ( 96.75683229781660089, -37.84742820979678868, 77.40038718067299328 ) ) ;
#43749=ORIENTED_EDGE ( 'NONE', *, *, #85239, .F. ) ;
#43750=CARTESIAN_POINT ( 'NONE',  ( 116.3181333158508295, -32.94392590426259204, 50.13562527591097506 ) ) ;
#43751=CARTESIAN_POINT ( 'NONE',  ( 117.9257662994439499, -34.79559216868042171, 194.9546728949589749 ) ) ;
#43752=CARTESIAN_POINT ( 'NONE',  ( 150.5667039024482960, -47.82844715993594775, 300.4678068554149490 ) ) ;
#43753=CARTESIAN_POINT ( 'NONE',  ( 98.04154693352651861, -41.04191595932115888, 146.6812072298401404 ) ) ;
#43754=LINE ( 'NONE', #57383, #34172 ) ;
#43755=DIRECTION ( 'NONE',  ( 0.000000000000000000, 0.000000000000000000, 1.000000000000000000 ) ) ;
#43758=FACE_BOUND ( 'NONE', #41063, .T. ) ;
#43759=DIRECTION ( 'NONE',  ( -4.237773401492740281E-14, 1.000000000000000000, 0.000000000000000000 ) ) ;
#43760=CARTESIAN_POINT ( 'NONE',  ( 116.5042510202519708, -34.04512512578503447, 149.0470538473399529 ) ) ;
#43761=ORIENTED_EDGE ( 'NONE', *, *, #349, .F. ) ;
#43762=VERTEX_POINT ( 'NONE', #34615 ) ;
#43764=CARTESIAN_POINT ( 'NONE',  ( 98.20303647727408247, -37.43757155718014928, 97.82158330589696504 ) ) ;
#43766=DIRECTION ( 'NONE',  ( 0.000000000000000000, 1.000000000000000000, 0.000000000000000000 ) ) ;
#43767=CARTESIAN_POINT ( 'NONE',  ( 104.5747221139661605, -26.66317121150818892, 236.2575300378149734 ) ) ;
#43768=CYLINDRICAL_SURFACE ( 'NONE', #43327, 0.2500000000000002220 ) ;
#43770=CARTESIAN_POINT ( 'NONE',  ( 100.9546619336613844, -28.70703383231385430, 111.5943577614134199 ) ) ;
#43775=CARTESIAN_POINT ( 'NONE',  ( 100.8994224252808323, -45.87202276647018095, 152.0918157521009562 ) ) ;
#43776=ORIENTED_EDGE ( 'NONE', *, *, #75845, .T. ) ;
#43777=ORIENTED_EDGE ( 'NONE', *, *, #6513, .F. ) ;
#43778=ORIENTED_EDGE ( 'NONE', *, *, #3644, .T. ) ;
#43779=DIRECTION ( 'NONE',  ( -0.1858654557293184517, 0.9825752044329902901, 0.000000000000000000 ) ) ;
#43780=CARTESIAN_POINT ( 'NONE',  ( 115.0876195537187670, -30.61596616040899832, 129.3441257015518602 ) ) ;
#43781=CARTESIAN_POINT ( 'NONE',  ( 97.81334898132925559, -40.52147985742783476, 102.6359742825680144 ) ) ;
#43782=EDGE_CURVE ( 'NONE', #68461, #61667, #9671, .T. ) ;
#43783=CARTESIAN_POINT ( 'NONE',  ( 113.5820732635001491, -31.81245485458596889, 217.1595189410199396 ) ) ;
#43784=CARTESIAN_POINT ( 'NONE',  ( 116.8171232307727934, -34.15291921056556390, 270.0314585327250825 ) ) ;
#43785=CARTESIAN_POINT ( 'NONE',  ( 96.61862839515298162, -36.21153332102672806, 171.2870538473399620 ) ) ;
#43786=CARTESIAN_POINT ( 'NONE',  ( 107.0664832912739968, -36.72944715994100306, 287.6356252759109680 ) ) ;
#43787=ORIENTED_EDGE ( 'NONE', *, *, #32615, .F. ) ;
#43789=ORIENTED_EDGE ( 'NONE', *, *, #7078, .T. ) ;
#43790=DIRECTION ( 'NONE',  ( 0.000000000000000000, -1.000000000000000000, 0.000000000000000000 ) ) ;
#43792=EDGE_LOOP ( 'NONE', ( #77734, #51942, #5948, #87773 ) ) ;
#43794=CARTESIAN_POINT ( 'NONE',  ( 131.3325395364358883, -36.38432368374370185, 6.774690158159009101 ) ) ;
#43795=CARTESIAN_POINT ( 'NONE',  ( 116.6500553765360451, -33.62673909641207359, 280.5072975916113478 ) ) ;
#43796=CARTESIAN_POINT ( 'NONE',  ( 99.04406103905903080, -42.84125657712180413, 271.8439585032700734 ) ) ;
#43797=ORIENTED_EDGE ( 'NONE', *, *, #45886, .F. ) ;
#43798=EDGE_CURVE ( 'NONE', #10458, #42899, #49572, .T. ) ;
#43800=CARTESIAN_POINT ( 'NONE',  ( 108.2227403955006082, -44.96027198985901663, 9.635625275910943088 ) ) ;
#43801=DIRECTION ( 'NONE',  ( 0.000000000000000000, 0.000000000000000000, -1.000000000000000000 ) ) ;
#43803=ORIENTED_EDGE ( 'NONE', *, *, #71345, .T. ) ;
#43804=STYLED_ITEM ( 'NONE', ( #70190 ), #18841 ) ;
#43805=ADVANCED_FACE ( 'NONE', ( #20996 ), #69596, .T. ) ;
#43806=CARTESIAN_POINT ( 'NONE',  ( 110.8545864177290099, -45.98419052231162141, 112.8856351242157530 ) ) ;
#43807=VERTEX_POINT ( 'NONE', #27355 ) ;
#43808=ORIENTED_EDGE ( 'NONE', *, *, #36129, .F. ) ;
#43809=CARTESIAN_POINT ( 'NONE',  ( 101.7280645633873775, -29.41412380334073973, 29.98861030426797214 ) ) ;
#43810=CARTESIAN_POINT ( 'NONE',  ( 109.8619129364321481, -26.66307059906275612, 174.8613395616249591 ) ) ;
#43811=CARTESIAN_POINT ( 'NONE',  ( 102.3226935662337098, -26.77152163616654335, 140.4422919425769578 ) ) ;
#43812=CARTESIAN_POINT ( 'NONE',  ( 116.8574199659429098, -40.30995640862995799, 214.5470538473389581 ) ) ;
#43813=CARTESIAN_POINT ( 'NONE',  ( 116.8170375758959665, -34.15258794555239774, 100.0316818571836137 ) ) ;
#43814=CARTESIAN_POINT ( 'NONE',  ( 102.0659246755500362, -27.97116092501175189, 126.4898951673323637 ) ) ;
#43816=ORIENTED_EDGE ( 'NONE', *, *, #38203, .F. ) ;
#43818=ORIENTED_EDGE ( 'NONE', *, *, #57003, .T. ) ;
#43819=AXIS2_PLACEMENT_3D ( 'NONE', #11697, #39390, #67096 ) ;
#43821=CARTESIAN_POINT ( 'NONE',  ( 117.1106518157658343, -39.68263944894788864, 183.5984824187679578 ) ) ;
#43823=CARTESIAN_POINT ( 'NONE',  ( 109.4453579932576872, -25.93500217162640453, 179.8918157521019339 ) ) ;
#43824=LINE ( 'NONE', #30217, #12683 ) ;
#43825=LINE ( 'NONE', #22514, #24674 ) ;
#43826=CARTESIAN_POINT ( 'NONE',  ( 51.06648329127400388, 19.62155284005901024, 333.4006252759110112 ) ) ;
#43827=CARTESIAN_POINT ( 'NONE',  ( 97.95414082892358465, -40.28560263849463041, 277.6356252759110248 ) ) ;
#43828=CARTESIAN_POINT ( 'NONE',  ( 116.3184051949732805, -40.67301874499263192, 58.50512385792708869 ) ) ;
#43829=CARTESIAN_POINT ( 'NONE',  ( 117.4695305279093986, -36.80206755349690440, 259.8213395616249386 ) ) ;
#43830=DIRECTION ( 'NONE',  ( 0.000000000000000000, 0.000000000000000000, 1.000000000000000000 ) ) ;
#43832=DIRECTION ( 'NONE',  ( 0.000000000000000000, 0.000000000000000000, -1.000000000000000000 ) ) ;
#43834=CARTESIAN_POINT ( 'NONE',  ( 113.2419700359254904, -28.75597482911128822, 270.5522191222117385 ) ) ;
#43835=EDGE_CURVE ( 'NONE', #31385, #35045, #36233, .T. ) ;
#43836=LINE ( 'NONE', #83859, #76117 ) ;
#43837=CARTESIAN_POINT ( 'NONE',  ( 116.7951252733230945, -39.38782978238762666, 259.6147919431981563 ) ) ;
#43840=CARTESIAN_POINT ( 'NONE',  ( 115.0355867660158538, -32.94440492534615572, 195.5838068554167251 ) ) ;
#43841=ORIENTED_EDGE ( 'NONE', *, *, #51318, .F. ) ;
#43842=ADVANCED_FACE ( 'NONE', ( #62320 ), #76855, .T. ) ;
#43843=DIRECTION ( 'NONE',  ( 1.000000000000000000, 0.000000000000000000, 9.462128050782575008E-16 ) ) ;
#43844=CARTESIAN_POINT ( 'NONE',  ( 101.3369781660191222, -46.20933176663394448, 202.1318157521019430 ) ) ;
#43845=CARTESIAN_POINT ( 'NONE',  ( 110.3540904097210387, -25.34409450869410563, 60.85276813305395649 ) ) ;
#43846=CARTESIAN_POINT ( 'NONE',  ( 110.5132149073354242, -26.84445748292755951, 205.8099109901969541 ) ) ;
#43847=CARTESIAN_POINT ( 'NONE',  ( 194.5667039024482676, -40.82844715993405060, 129.9678068554150343 ) ) ;
#43848=CARTESIAN_POINT ( 'NONE',  ( 32.06670390244772051, -33.35206098992742341, 237.4678068554150059 ) ) ;
#43850=DIRECTION ( 'NONE',  ( 0.000000000000000000, 0.000000000000000000, -1.000000000000000000 ) ) ;
#43851=DIRECTION ( 'NONE',  ( -4.012088370409549976E-14, 1.000000000000000000, 0.000000000000000000 ) ) ;
#43853=ORIENTED_EDGE ( 'NONE', *, *, #10292, .T. ) ;
#43854=CARTESIAN_POINT ( 'NONE',  ( 113.2480160518910992, -28.76059550239980567, 64.55305391943088011 ) ) ;
#43855=EDGE_CURVE ( 'NONE', #8294, #51052, #71075, .T. ) ;
#43860=CARTESIAN_POINT ( 'NONE',  ( 115.2923595980251434, -39.02968425817515197, 98.03241982807698207 ) ) ;
#43861=LINE ( 'NONE', #30689, #73429 ) ;
#43863=AXIS2_PLACEMENT_3D ( 'NONE', #64879, #15837, #16728 ) ;
#43864=CARTESIAN_POINT ( 'NONE',  ( 117.3319688044106925, -38.62265419183309945, 84.68133956162593279 ) ) ;
#43865=DIRECTION ( 'NONE',  ( 4.299999999999999979E-14, -1.000000000000000000, 4.400000000000000367E-29 ) ) ;
#43866=DIRECTION ( 'NONE',  ( -0.7071067812159671506, -0.7071067811571278838, 2.899137802744108569E-29 ) ) ;
#43867=CARTESIAN_POINT ( 'NONE',  ( 97.33784131910049098, -34.07106450134590858, 177.1147919402304467 ) ) ;
#43868=CARTESIAN_POINT ( 'NONE',  ( 115.8115096128642136, -32.27542772465447030, 44.20133956162592170 ) ) ;
#43869=ORIENTED_EDGE ( 'NONE', *, *, #55100, .T. ) ;
#43871=ORIENTED_EDGE ( 'NONE', *, *, #89073, .T. ) ;
#43874=CARTESIAN_POINT ( 'NONE',  ( 21.03689327557613709, -23.42844715994198879, 117.4678068554150343 ) ) ;
#43875=CARTESIAN_POINT ( 'NONE',  ( 71.25580610988301089, -82.12815647064930147, 542.9756252759101471 ) ) ;
#43876=DIRECTION ( 'NONE',  ( -0.7071067811865171526, -0.7071067811865779928, -7.071067811865164719E-16 ) ) ;
#43878=CARTESIAN_POINT ( 'NONE',  ( 25.56670390244797275, -65.37844715994100397, 252.3428068554150059 ) ) ;
#43881=CARTESIAN_POINT ( 'NONE',  ( 117.9659426345832713, -38.42225801833666310, 68.69181575210198787 ) ) ;
#43882=TOROIDAL_SURFACE ( 'NONE', #27933, 13.50000000000000000, 0.5000000000000000000 ) ;
#43885=CARTESIAN_POINT ( 'NONE',  ( 41.56648329127398966, -27.82844715994070484, 74.17562527591199739 ) ) ;
#43887=CARTESIAN_POINT ( 'NONE',  ( 103.3817498881349906, -44.01315952142851984, 125.0223760838769778 ) ) ;
#43888=AXIS2_PLACEMENT_3D ( 'NONE', #71991, #42915, #15694 ) ;
#43889=EDGE_CURVE ( 'NONE', #66320, #5230, #28704, .T. ) ;
#43891=AXIS2_PLACEMENT_3D ( 'NONE', #86977, #47394, #26084 ) ;
#43893=ORIENTED_EDGE ( 'NONE', *, *, #58454, .T. ) ;
#43894=ORIENTED_EDGE ( 'NONE', *, *, #18321, .T. ) ;
#43896=ORIENTED_EDGE ( 'NONE', *, *, #13213, .T. ) ;
#43897=VERTEX_POINT ( 'NONE', #72724 ) ;
#43898=CARTESIAN_POINT ( 'NONE',  ( 99.15781305739687923, -40.79332027783682690, 193.1358690201829518 ) ) ;
#43900=CARTESIAN_POINT ( 'NONE',  ( 106.0743987232105212, -48.56321320874933889, 108.5099109901969712 ) ) ;
#43901=CARTESIAN_POINT ( 'NONE',  ( 98.34985898019030515, -31.65658469527032182, 120.9064585987749183 ) ) ;
#43902=CARTESIAN_POINT ( 'NONE',  ( 98.54780627451228270, -41.97722989217538725, 16.76585467579917221 ) ) ;
#43903=VERTEX_POINT ( 'NONE', #71837 ) ;
#43906=ORIENTED_EDGE ( 'NONE', *, *, #45880, .T. ) ;
#43907=CARTESIAN_POINT ( 'NONE',  ( 98.50976710839005079, -35.43193677023271704, 219.0128522743539747 ) ) ;
#43908=VECTOR ( 'NONE', #11596, 1000.000000000000000 ) ;
#43909=CARTESIAN_POINT ( 'NONE',  ( 110.8024161898992190, -46.48594086123524960, 62.86705384733992474 ) ) ;
#43911=CARTESIAN_POINT ( 'NONE',  ( 116.7496603916997202, -31.44741115753626204, 24.21181575210196257 ) ) ;
#43912=CARTESIAN_POINT ( 'NONE',  ( 107.9200411489893412, -47.17696527638128856, 173.6413395616249886 ) ) ;
#43913=DIRECTION ( 'NONE',  ( 1.000000000000000000, 0.000000000000000000, 0.000000000000000000 ) ) ;
#43915=CARTESIAN_POINT ( 'NONE',  ( 109.5084879329568679, -46.86449036543412205, 128.7641967044819751 ) ) ;
#43917=ORIENTED_EDGE ( 'NONE', *, *, #78107, .F. ) ;
#43918=DIRECTION ( 'NONE',  ( 0.000000000000000000, 0.000000000000000000, 1.000000000000000000 ) ) ;
#43920=CARTESIAN_POINT ( 'NONE',  ( 113.1789227100342430, -44.75140297935337230, 134.0951559795896628 ) ) ;
#43921=EDGE_LOOP ( 'NONE', ( #76285, #73951, #74554, #46029 ) ) ;
#43922=ORIENTED_EDGE ( 'NONE', *, *, #2118, .F. ) ;
#43925=CARTESIAN_POINT ( 'NONE',  ( 101.3624556188076440, -28.48975351766920738, 131.5580310753099695 ) ) ;
#43926=CARTESIAN_POINT ( 'NONE',  ( 98.30617374076959436, -28.74837815785401673, 80.73848241876795839 ) ) ;
#43928=FACE_OUTER_BOUND ( 'NONE', #65367, .T. ) ;
#43929=LINE ( 'NONE', #78931, #2049 ) ;
#43930=CARTESIAN_POINT ( 'NONE',  ( 104.6499073705539331, -46.24122592705978718, 47.37848241876896083 ) ) ;
#43932=CARTESIAN_POINT ( 'NONE',  ( 103.4759237351581049, -46.49349013887657378, 138.2956252759109645 ) ) ;
#43933=LINE ( 'NONE', #70775, #34955 ) ;
#43935=DIRECTION ( 'NONE',  ( 0.000000000000000000, 0.000000000000000000, 1.000000000000000000 ) ) ;
#43936=VERTEX_POINT ( 'NONE', #85484 ) ;
#43938=CARTESIAN_POINT ( 'NONE',  ( 51.56670390244699576, -22.48495420874030515, -5.074374724088000832 ) ) ;
#43939=EDGE_CURVE ( 'NONE', #50424, #63964, #58625, .T. ) ;
#43943=CARTESIAN_POINT ( 'NONE',  ( 110.5134301196510620, -26.84384026877932072, 209.8099109901969541 ) ) ;
#43944=VERTEX_POINT ( 'NONE', #30052 ) ;
#43945=ADVANCED_FACE ( 'NONE', ( #23263 ), #70952, .F. ) ;
#43947=CARTESIAN_POINT ( 'NONE',  ( 107.5109549264149251, -47.16686560604517098, 233.6099109901969655 ) ) ;
#43948=CARTESIAN_POINT ( 'NONE',  ( 104.0954500313802527, -46.76767116204542418, 103.3470538473389411 ) ) ;
#43949=LINE ( 'NONE', #72575, #46146 ) ;
#43950=DIRECTION ( 'NONE',  ( 0.000000000000000000, 0.000000000000000000, -1.000000000000000000 ) ) ;
#43951=LINE ( 'NONE', #70337, #37974 ) ;
#43953=AXIS2_PLACEMENT_3D ( 'NONE', #59357, #24413, #17594 ) ;
#43955=ORIENTED_EDGE ( 'NONE', *, *, #3649, .F. ) ;
#43956=VERTEX_POINT ( 'NONE', #1899 ) ;
#43959=ORIENTED_EDGE ( 'NONE', *, *, #82786, .F. ) ;
#43961=CARTESIAN_POINT ( 'NONE',  ( 115.6952998724001560, -42.57974731087075071, 269.3527681330536439 ) ) ;
#43963=DIRECTION ( 'NONE',  ( 1.000000000000000000, -3.885780586187990841E-13, 0.000000000000000000 ) ) ;
#43965=DIRECTION ( 'NONE',  ( 0.000000000000000000, -1.000000000000000000, 0.000000000000000000 ) ) ;
#43967=CYLINDRICAL_SURFACE ( 'NONE', #47210, 2.517500000000005844 ) ;
#43968=CARTESIAN_POINT ( 'NONE',  ( 104.7063189284543370, -28.49041042582816630, 224.7209912566489720 ) ) ;
#43969=VERTEX_POINT ( 'NONE', #37761 ) ;
#43970=ORIENTED_EDGE ( 'NONE', *, *, #64493, .F. ) ;
#43972=CARTESIAN_POINT ( 'NONE',  ( 107.0664832912748068, -36.72944715993923381, 13.92562527591097066 ) ) ;
#43973=AXIS2_PLACEMENT_3D ( 'NONE', #61279, #32230, #89003 ) ;
#43974=CARTESIAN_POINT ( 'NONE',  ( 110.8553449835648621, -45.98388008209910538, 182.8857003179606409 ) ) ;
#43975=CARTESIAN_POINT ( 'NONE',  ( 115.6529839569024602, -41.48189714014871043, 259.4241967044819717 ) ) ;
#43976=CARTESIAN_POINT ( 'NONE',  ( 37.03715912545347777, -48.62818131006128652, 129.9678068554150911 ) ) ;
#43978=CARTESIAN_POINT ( 'NONE',  ( 100.1408543393099393, -45.42701269980175738, 118.0413395616249659 ) ) ;
#43979=CARTESIAN_POINT ( 'NONE',  ( 80.06648329127399677, -8.350947159940998787, 291.1181252759119502 ) ) ;
#43981=CARTESIAN_POINT ( 'NONE',  ( 19.56670390244643443, -25.42844715994203852, 180.4678068554150911 ) ) ;
#43982=CARTESIAN_POINT ( 'NONE',  ( 78.21890182791160839, -34.68450975841992090, 2.186797062532628289 ) ) ;
#43985=CARTESIAN_POINT ( 'NONE',  ( 99.80492824067951574, -39.70159478663597241, 9.453804655305930282 ) ) ;
#43986=CIRCLE ( 'NONE', #64323, 2.500000000000002220 ) ;
#43987=CYLINDRICAL_SURFACE ( 'NONE', #79838, 2.750000000000002665 ) ;
#43988=ADVANCED_FACE ( 'NONE', ( #10053 ), #23697, .T. ) ;
#43989=CARTESIAN_POINT ( 'NONE',  ( 34.27258461953899626, -35.55794170701810941, -5.074374724088000832 ) ) ;
#43990=CARTESIAN_POINT ( 'NONE',  ( 115.0371709891030747, -42.90857240100309156, 194.3022695669546067 ) ) ;
#43991=EDGE_LOOP ( 'NONE', ( #25106, #62973, #52864, #3373, #57842, #22494 ) ) ;
#43992=LINE ( 'NONE', #2243, #75528 ) ;
#43993=DIRECTION ( 'NONE',  ( -1.000000000000000078E-15, 1.000000000000000083E-30, 1.000000000000000000 ) ) ;
#43995=CARTESIAN_POINT ( 'NONE',  ( 98.30617374076959436, -28.74837815785401673, 80.73848241876795839 ) ) ;
#43996=ORIENTED_EDGE ( 'NONE', *, *, #13593, .T. ) ;
#43997=CARTESIAN_POINT ( 'NONE',  ( 114.0673224709094598, -30.00197523691782209, 38.85813411379096749 ) ) ;
#43998=CARTESIAN_POINT ( 'NONE',  ( 113.7194588667589557, -44.22387875709570437, 89.15331731304537755 ) ) ;
#43999=CARTESIAN_POINT ( 'NONE',  ( 100.0889724914296863, -42.24093267880301994, 88.29015473446894191 ) ) ;
#44000=CARTESIAN_POINT ( 'NONE',  ( 98.30750078144184556, -41.72879384224769694, 12.73978492213259450 ) ) ;
#44003=CARTESIAN_POINT ( 'NONE',  ( 105.8886828556765494, -47.16740550586902003, 278.4870538473396664 ) ) ;
#44004=DIRECTION ( 'NONE',  ( 0.7071067809773464719, -0.7071067813957485626, 7.071067809773472419E-16 ) ) ;
#44005=VERTEX_POINT ( 'NONE', #51361 ) ;
#44006=AXIS2_PLACEMENT_3D ( 'NONE', #39799, #45708, #59796 ) ;
#44007=LINE ( 'NONE', #10401, #58929 ) ;
#44008=ORIENTED_EDGE ( 'NONE', *, *, #12726, .F. ) ;
#44009=CARTESIAN_POINT ( 'NONE',  ( 95.96792091384095613, -36.58316683298836125, 152.3280062282919971 ) ) ;
#44010=EDGE_CURVE ( 'NONE', #20111, #53395, #78673, .T. ) ;
#44013=ORIENTED_EDGE ( 'NONE', *, *, #80356, .T. ) ;
#44014=VERTEX_POINT ( 'NONE', #44101 ) ;
#44016=PLANE ( 'NONE',  #71050 ) ;
#44017=CARTESIAN_POINT ( 'NONE',  ( 152.5667039024472444, -23.42844715993586036, 237.4678068554150059 ) ) ;
#44018=CARTESIAN_POINT ( 'NONE',  ( 98.59486473514172644, -43.92970144294059054, 226.8870538473399563 ) ) ;
#44020=FACE_OUTER_BOUND ( 'NONE', #78646, .T. ) ;
#44022=CARTESIAN_POINT ( 'NONE',  ( 109.6119375470732109, -25.15554210634138954, 25.90419670448196143 ) ) ;
#44025=ORIENTED_EDGE ( 'NONE', *, *, #45278, .F. ) ;
#44026=CARTESIAN_POINT ( 'NONE',  ( 113.6007965834298545, -29.07570238281020636, 170.5145071421607668 ) ) ;
#44028=CARTESIAN_POINT ( 'NONE',  ( 104.4080901167367443, -46.45808640916315824, 42.36430364053295250 ) ) ;
#44029=ORIENTED_EDGE ( 'NONE', *, *, #16860, .T. ) ;
#44030=CARTESIAN_POINT ( 'NONE',  ( 82.54112294218050749, -19.94037323192172551, 2.740176903240867379 ) ) ;
#44032=CARTESIAN_POINT ( 'NONE',  ( 107.0664832912739968, -8.729447159940999512, 6.425625275911999168 ) ) ;
#44033=CARTESIAN_POINT ( 'NONE',  ( 100.8614382317054776, -45.12360235833661903, 257.0699109901967745 ) ) ;
#44036=FACE_OUTER_BOUND ( 'NONE', #44884, .T. ) ;
#44038=CARTESIAN_POINT ( 'NONE',  ( 112.1081655520365388, -43.62419673505787898, 227.5009912566479784 ) ) ;
#44039=CARTESIAN_POINT ( 'NONE',  ( 37.03715912545433042, -48.62818131006122258, 249.9678068554150343 ) ) ;
#44040=CARTESIAN_POINT ( 'NONE',  ( 115.8731522275743089, -31.19128430790907913, 30.27276813305396175 ) ) ;
#44042=CARTESIAN_POINT ( 'NONE',  ( 109.6949574390794169, -47.51388072328656165, 87.75467289495897205 ) ) ;
#44044=CARTESIAN_POINT ( 'NONE',  ( 131.7293641403231277, -20.17925173417497575, 7.255518600571654986 ) ) ;
#44045=VERTEX_POINT ( 'NONE', #44995 ) ;
#44046=AXIS2_PLACEMENT_3D ( 'NONE', #20280, #33887, #81175 ) ;
#44047=PLANE ( 'NONE',  #52192 ) ;
#44049=EDGE_CURVE ( 'NONE', #42899, #35086, #36427, .T. ) ;
#44051=CARTESIAN_POINT ( 'NONE',  ( 83.06670390244796920, -67.87844715994100397, 207.5838068554149913 ) ) ;
#44052=VERTEX_POINT ( 'NONE', #65892 ) ;
#44053=CARTESIAN_POINT ( 'NONE',  ( 82.81648329127398256, -18.72944715994105636, 14.92562527591094579 ) ) ;
#44056=LINE ( 'NONE', #50431, #7505 ) ;
#44058=CARTESIAN_POINT ( 'NONE',  ( 107.6042850712483698, -26.26048674992130572, 95.03562527591097364 ) ) ;
#44060=CARTESIAN_POINT ( 'NONE',  ( 97.07201595580151832, -35.37887681970044440, 166.2189934953664761 ) ) ;
#44061=FACE_OUTER_BOUND ( 'NONE', #70865, .T. ) ;
#44064=ADVANCED_FACE ( 'NONE', ( #8725 ), #22802, .T. ) ;
#44066=EDGE_CURVE ( 'NONE', #37352, #8193, #71139, .T. ) ;
#44071=B_SPLINE_CURVE_WITH_KNOTS ( 'NONE', 3,
 ( #59634, #60079, #5139, #6054, #33742, #75531, #88722, #46451, #80559, #74624, #26037, #52791, #61432, #39205, #73732, #18315, #54149, #89159 ),
 .UNSPECIFIED., .F., .F.,
 ( 4, 2, 2, 2, 2, 2, 2, 2, 4 ),
 ( 0.4999874552890923862, 0.5624890233779558102, 0.6249905914668192342, 0.6874921595556827691, 0.7499937276445461931, 0.8124952957334096171, 0.8749968638222731521, 0.9374984319111365760, 1.000000000000000000 ),
 .UNSPECIFIED. ) ;
#44072=DIRECTION ( 'NONE',  ( 0.000000000000000000, 1.000000000000000000, 0.000000000000000000 ) ) ;
#44073=DIRECTION ( 'NONE',  ( 0.000000000000000000, 0.000000000000000000, -1.000000000000000000 ) ) ;
#44074=DIRECTION ( 'NONE',  ( 0.1811243268507065352, -0.9834602067307444129, 0.000000000000000000 ) ) ;
#44075=AXIS2_PLACEMENT_3D ( 'NONE', #65520, #78732, #64628 ) ;
#44076=VERTEX_POINT ( 'NONE', #60866 ) ;
#44079=CARTESIAN_POINT ( 'NONE',  ( 108.8290724220007206, -27.07506712556666173, 160.9327681330529742 ) ) ;
#44080=LINE ( 'NONE', #71813, #57338 ) ;
#44081=ORIENTED_EDGE ( 'NONE', *, *, #9388, .T. ) ;
#44082=CARTESIAN_POINT ( 'NONE',  ( 97.46604185887804306, -38.76544784714101155, 27.49276813305395706 ) ) ;
#44083=FACE_BOUND ( 'NONE', #49150, .T. ) ;
#44084=LINE ( 'NONE', #16850, #6693 ) ;
#44085=CARTESIAN_POINT ( 'NONE',  ( 164.9667039024476765, -26.71338133338732135, 117.4678068554150485 ) ) ;
#44086=CARTESIAN_POINT ( 'NONE',  ( 109.7260889235150785, -27.00112954045210856, 29.86492210598321506 ) ) ;
#44087=CARTESIAN_POINT ( 'NONE',  ( 97.63766479707255996, -34.12929003103648284, 251.1127681330543737 ) ) ;
#44088=EDGE_LOOP ( 'NONE', ( #22242, #14780, #86855, #43803, #36201, #45190, #27993, #83840 ) ) ;
#44090=CARTESIAN_POINT ( 'NONE',  ( 98.20738808897236538, -36.51799785534514342, 192.7387261630399564 ) ) ;
#44091=CARTESIAN_POINT ( 'NONE',  ( 193.0371591254584303, -47.82818131005411999, 249.9678068554149775 ) ) ;
#44092=CARTESIAN_POINT ( 'NONE',  ( 106.6757791475081376, -27.34201535943007499, 36.52920235351597711 ) ) ;
#44095=AXIS2_PLACEMENT_3D ( 'NONE', #7639, #54858, #48486 ) ;
#44097=CARTESIAN_POINT ( 'NONE',  ( 113.2454986998394162, -28.75867294625993154, 79.55229194239187507 ) ) ;
#44098=LINE ( 'NONE', #22800, #89447 ) ;
#44099=CONICAL_SURFACE ( 'NONE', #19533, 16.00000000000090239, 0.7853981633974503884 ) ;
#44101=CARTESIAN_POINT ( 'NONE',  ( 182.5667039024459939, -19.82844715994031048, -5.074374724088000832 ) ) ;
#44103=CARTESIAN_POINT ( 'NONE',  ( 97.03753386688401861, -33.96379371595038776, 251.1127681330538337 ) ) ;
#44105=ORIENTED_EDGE ( 'NONE', *, *, #33806, .T. ) ;
#44107=DIRECTION ( 'NONE',  ( 1.000000000000000000, 4.163336342344333240E-14, 0.000000000000000000 ) ) ;
#44108=DIRECTION ( 'NONE',  ( 0.000000000000000000, -1.000000000000000000, 0.000000000000000000 ) ) ;
#44109=FACE_BOUND ( 'NONE', #56926, .T. ) ;
#44110=CARTESIAN_POINT ( 'NONE',  ( 100.8863495415024829, -28.40209871822986543, 31.59657765686296926 ) ) ;
#44112=ORIENTED_EDGE ( 'NONE', *, *, #20251, .T. ) ;
#44113=CARTESIAN_POINT ( 'NONE',  ( 117.5312049024071257, -37.01681686833584450, 39.80419670448193159 ) ) ;
#44114=EDGE_CURVE ( 'NONE', #27939, #3527, #7322, .T. ) ;
#44115=CARTESIAN_POINT ( 'NONE',  ( 107.0664832912739257, -52.57944715994094764, 302.6356252759109680 ) ) ;
#44116=CARTESIAN_POINT ( 'NONE',  ( 116.1397716810727303, -31.55208187140975795, 289.2384824187681716 ) ) ;
#44117=EDGE_CURVE ( 'NONE', #48818, #45118, #25913, .T. ) ;
#44118=ORIENTED_EDGE ( 'NONE', *, *, #24154, .F. ) ;
#44119=EDGE_CURVE ( 'NONE', #33965, #19079, #56586, .T. ) ;
#44120=PLANE ( 'NONE',  #11496 ) ;
#44121=CARTESIAN_POINT ( 'NONE',  ( 108.3343131715331822, -46.73476620053450148, 18.67790446994724007 ) ) ;
#44123=CARTESIAN_POINT ( 'NONE',  ( 99.39318122740648676, -32.72677799018995870, 88.74999513149600716 ) ) ;
#44124=CARTESIAN_POINT ( 'NONE',  ( 115.4053350490088548, -30.43652969535880359, 215.3413395616249773 ) ) ;
#44128=EDGE_CURVE ( 'NONE', #14756, #63362, #46325, .T. ) ;
#44129=LINE ( 'NONE', #16902, #70866 ) ;
#44134=DIRECTION ( 'NONE',  ( 1.000000000000000000, 4.163336342344333240E-14, 0.000000000000000000 ) ) ;
#44135=ORIENTED_EDGE ( 'NONE', *, *, #39987, .T. ) ;
#44139=CARTESIAN_POINT ( 'NONE',  ( 97.07206694318691120, -35.37847583654921380, 42.21889330128750117 ) ) ;
#44140=CARTESIAN_POINT ( 'NONE',  ( 115.3391490808644875, -34.60362203641794565, 123.4495626852199734 ) ) ;
#44141=CARTESIAN_POINT ( 'NONE',  ( 106.8359473341788686, -47.17421700602214685, 272.5584824187680510 ) ) ;
#44142=CARTESIAN_POINT ( 'NONE',  ( 34.96670390244699433, -28.27351298637401200, 342.9256252759119548 ) ) ;
#44144=ORIENTED_EDGE ( 'NONE', *, *, #80019, .F. ) ;
#44145=DIRECTION ( 'NONE',  ( 4.299999999999999979E-14, -1.000000000000000000, 4.400000000000000367E-29 ) ) ;
#44146=ORIENTED_EDGE ( 'NONE', *, *, #52392, .T. ) ;
#44148=FACE_OUTER_BOUND ( 'NONE', #37566, .T. ) ;
#44149=CARTESIAN_POINT ( 'NONE',  ( 97.92338214298322896, -40.78104107816966462, 131.6584137149031619 ) ) ;
#44150=CARTESIAN_POINT ( 'NONE',  ( 96.84578370412310733, -30.63304659132085206, 280.8984824187681397 ) ) ;
#44152=VERTEX_POINT ( 'NONE', #10931 ) ;
#44154=CARTESIAN_POINT ( 'NONE',  ( 112.4118754778678380, -46.40445981238691076, 252.9661014663871583 ) ) ;
#44155=VECTOR ( 'NONE', #49095, 1000.000000000000000 ) ;
#44156=CARTESIAN_POINT ( 'NONE',  ( 97.06313332029375829, -39.81586545721199144, 17.56419670448195092 ) ) ;
#44159=AXIS2_PLACEMENT_3D ( 'NONE', #73774, #58357, #82404 ) ;
#44160=CARTESIAN_POINT ( 'NONE',  ( 66.21896343372186777, -72.55791859125245935, 542.9756252759101471 ) ) ;
#44162=CARTESIAN_POINT ( 'NONE',  ( 116.3228127852087113, -32.93589129790882453, 90.13562527591095375 ) ) ;
#44163=CARTESIAN_POINT ( 'NONE',  ( 107.0664832912739968, 19.62155284005901024, 327.8006252759110453 ) ) ;
#44165=CARTESIAN_POINT ( 'NONE',  ( 152.5667039024469602, -23.42844715993586036, 300.4678068554149490 ) ) ;
#44166=AXIS2_PLACEMENT_3D ( 'NONE', #22408, #71011, #14247 ) ;
#44167=VECTOR ( 'NONE', #26339, 999.9999999999998863 ) ;
#44168=CARTESIAN_POINT ( 'NONE',  ( 97.81168895331838087, -40.51742574516882200, 287.6356252759109680 ) ) ;
#44169=CARTESIAN_POINT ( 'NONE',  ( 116.7953080883038552, -39.38717811076809028, 163.6146878284437491 ) ) ;
#44171=DIRECTION ( 'NONE',  ( 0.000000000000000000, 0.000000000000000000, -1.000000000000000000 ) ) ;
#44173=CARTESIAN_POINT ( 'NONE',  ( 112.3495078575228376, -28.18909723048616911, 289.6356252759109680 ) ) ;
#44174=CARTESIAN_POINT ( 'NONE',  ( 117.0682170987564774, -39.67016276869777869, 179.5984824187679294 ) ) ;
#44175=CARTESIAN_POINT ( 'NONE',  ( 111.9390199320367145, -27.48847072138506320, 55.68991099019693536 ) ) ;
#44176=EDGE_CURVE ( 'NONE', #2919, #74183, #46772, .T. ) ;
#44177=CARTESIAN_POINT ( 'NONE',  ( 84.06648329127399677, -18.82844715994099971, 93.42562527591199739 ) ) ;
#44178=CARTESIAN_POINT ( 'NONE',  ( 119.2637946045970097, -42.39761235918182791, 0.4256252759109831474 ) ) ;
#44179=FACE_OUTER_BOUND ( 'NONE', #7943, .T. ) ;
#44180=CIRCLE ( 'NONE', #47094, 1.000000000000000888 ) ;
#44181=ORIENTED_EDGE ( 'NONE', *, *, #50186, .F. ) ;
#44182=DIRECTION ( 'NONE',  ( -1.000000000000000000, -2.999999999999999839E-15, -1.000000000000000078E-15 ) ) ;
#44183=VERTEX_POINT ( 'NONE', #52238 ) ;
#44184=CARTESIAN_POINT ( 'NONE',  ( 110.1509004715571507, -26.04776408289600909, 60.85276813305296173 ) ) ;
#44186=ORIENTED_EDGE ( 'NONE', *, *, #66138, .F. ) ;
#44188=CARTESIAN_POINT ( 'NONE',  ( 96.66614461754338095, -36.48121138304695421, 192.3070538473399438 ) ) ;
#44190=CARTESIAN_POINT ( 'NONE',  ( 34.96670390244699433, -26.71338133339301635, -5.074374724088000832 ) ) ;
#44191=LINE ( 'NONE', #24656, #44294 ) ;
#44193=DIRECTION ( 'NONE',  ( 0.7071067811865192621, 0.7071067811865758834, 7.071067811865186413E-16 ) ) ;
#44194=CARTESIAN_POINT ( 'NONE',  ( 117.0282276649355993, -35.31238565241870475, 98.93927789852577348 ) ) ;
#44195=CARTESIAN_POINT ( 'NONE',  ( 98.15811136316399654, -31.42099212808717468, 130.9108633711499863 ) ) ;
#44196=ORIENTED_EDGE ( 'NONE', *, *, #9847, .T. ) ;
#44197=ORIENTED_EDGE ( 'NONE', *, *, #15559, .F. ) ;
#44198=CARTESIAN_POINT ( 'NONE',  ( 115.8107094469502272, -38.34209669562990541, 85.11301187732594542 ) ) ;
#44199=CARTESIAN_POINT ( 'NONE',  ( 45.76696975232739817, -48.62818131006041256, 180.4678068554150911 ) ) ;
#44200=CARTESIAN_POINT ( 'NONE',  ( 115.9419818307743668, -40.91744192719421847, 224.4756252759109714 ) ) ;
#44201=DIRECTION ( 'NONE',  ( 1.000000000000000078E-15, -1.000000000000000083E-30, -1.000000000000000000 ) ) ;
#44203=DIRECTION ( 'NONE',  ( 0.000000000000000000, 0.000000000000000000, -1.000000000000000000 ) ) ;
#44207=CARTESIAN_POINT ( 'NONE',  ( 192.5667039024472444, -23.42844715993434335, 300.4678068554149490 ) ) ;
#44208=CARTESIAN_POINT ( 'NONE',  ( 118.8928063919343998, -36.92768728534039724, 153.8127681330539644 ) ) ;
#44211=LINE ( 'NONE', #71954, #38710 ) ;
#44213=CYLINDRICAL_SURFACE ( 'NONE', #21462, 2.117000000000000881 ) ;
#44215=CARTESIAN_POINT ( 'NONE',  ( 99.07378970379950545, -35.07216769230775810, 213.9823760838769715 ) ) ;
#44216=VECTOR ( 'NONE', #80643, 1000.000000000000000 ) ;
#44217=CIRCLE ( 'NONE', #71808, 1.000000000000000888 ) ;
#44218=DIRECTION ( 'NONE',  ( -1.000000000000000078E-15, -1.000000000000000083E-30, 1.000000000000000000 ) ) ;
#44219=AXIS2_PLACEMENT_3D ( 'NONE', #41626, #62084, #83003 ) ;
#44220=AXIS2_PLACEMENT_3D ( 'NONE', #52701, #80920, #18668 ) ;
#44221=EDGE_CURVE ( 'NONE', #49665, #66874, #80437, .T. ) ;
#44222=CARTESIAN_POINT ( 'NONE',  ( 116.3504430951951605, -44.09481043651530996, 198.2927681330539542 ) ) ;
#44223=ADVANCED_FACE ( 'NONE', ( #5017 ), #45432, .F. ) ;
#44224=FACE_OUTER_BOUND ( 'NONE', #585, .T. ) ;
#44226=ORIENTED_EDGE ( 'NONE', *, *, #21486, .F. ) ;
#44228=CIRCLE ( 'NONE', #16705, 0.4999999999999982236 ) ;
#44231=DIRECTION ( 'NONE',  ( 4.299999999999999979E-14, -1.000000000000000000, 4.128053709984630540E-29 ) ) ;
#44233=CARTESIAN_POINT ( 'NONE',  ( 118.5256205435843526, -36.72944715994100306, 292.6356252759106837 ) ) ;
#44234=CARTESIAN_POINT ( 'NONE',  ( 134.0664832912739826, -33.97944715994100306, 8.225625275910998013 ) ) ;
#44235=CARTESIAN_POINT ( 'NONE',  ( 114.7786440655094680, -32.32849264894101537, 285.6701547344685537 ) ) ;
#44236=ADVANCED_FACE ( 'NONE', ( #40426 ), #68141, .F. ) ;
#44237=DIRECTION ( 'NONE',  ( -4.237773401492740281E-14, 1.000000000000000000, 0.000000000000000000 ) ) ;
#44238=ORIENTED_EDGE ( 'NONE', *, *, #18517, .T. ) ;
#44240=CARTESIAN_POINT ( 'NONE',  ( 111.4682881893262305, -44.05286453299024885, 9.635625275910939536 ) ) ;
#44241=FACE_OUTER_BOUND ( 'NONE', #75264, .T. ) ;
#44242=ORIENTED_EDGE ( 'NONE', *, *, #49885, .T. ) ;
#44245=CARTESIAN_POINT ( 'NONE',  ( 114.5728715930965933, -43.36891021780796507, 113.2502506786379968 ) ) ;
#44248=VECTOR ( 'NONE', #4292, 1000.000000000000000 ) ;
#44249=EDGE_CURVE ( 'NONE', #58867, #26619, #43539, .T. ) ;
#44250=CARTESIAN_POINT ( 'NONE',  ( 116.1953253310505119, -40.03623866633203932, 22.97241982807796035 ) ) ;
#44251=CARTESIAN_POINT ( 'NONE',  ( 98.07151883162052286, -42.11266039418816121, 161.7556252759109725 ) ) ;
#44252=CARTESIAN_POINT ( 'NONE',  ( 100.8994224252808323, -45.87202276647018095, 152.0918157521009562 ) ) ;
#44254=CARTESIAN_POINT ( 'NONE',  ( 112.4117637605556297, -46.40425760712833636, 248.9661014663869878 ) ) ;
#44255=DIRECTION ( 'NONE',  ( -0.000000000000000000, -0.000000000000000000, -1.000000000000000000 ) ) ;
#44258=ORIENTED_EDGE ( 'NONE', *, *, #39043, .T. ) ;
#44259=EDGE_CURVE ( 'NONE', #54314, #11434, #34501, .T. ) ;
#44260=ORIENTED_EDGE ( 'NONE', *, *, #74531, .F. ) ;
#44261=CIRCLE ( 'NONE', #26896, 1.000000000000000888 ) ;
#44262=CARTESIAN_POINT ( 'NONE',  ( 103.7090067442367314, -26.14926592973559138, 205.3089586092439731 ) ) ;
#44263=ORIENTED_EDGE ( 'NONE', *, *, #45775, .F. ) ;
#44264=CARTESIAN_POINT ( 'NONE',  ( 117.0173010276973287, -33.62006509304910651, 174.0670538473389399 ) ) ;
#44266=CIRCLE ( 'NONE', #18214, 2.030000000001869864 ) ;
#44270=CYLINDRICAL_SURFACE ( 'NONE', #32495, 9.999999999999998224 ) ;
#44271=CARTESIAN_POINT ( 'NONE',  ( 117.4970320020026406, -36.54623693216563396, 284.8413395616252615 ) ) ;
#44272=DIRECTION ( 'NONE',  ( 0.000000000000000000, 0.000000000000000000, -1.000000000000000000 ) ) ;
#44273=CARTESIAN_POINT ( 'NONE',  ( 150.5667039024475571, -25.42844715993593852, 180.4678068554149775 ) ) ;
#44275=FACE_OUTER_BOUND ( 'NONE', #62295, .T. ) ;
#44276=CARTESIAN_POINT ( 'NONE',  ( 105.7154773553531015, -46.72385839539258257, 258.4689586112310167 ) ) ;
#44278=CARTESIAN_POINT ( 'NONE',  ( 109.3644549449422954, -44.39418949346432441, 195.5838068554168956 ) ) ;
#44280=CARTESIAN_POINT ( 'NONE',  ( 134.0664828118825938, -21.47944715903993540, 8.225259175038406312 ) ) ;
#44281=CARTESIAN_POINT ( 'NONE',  ( 102.8350101556302434, -46.28146260531957523, 177.2441967044819648 ) ) ;
#44282=CARTESIAN_POINT ( 'NONE',  ( 101.9605410436089699, -27.64034152677590583, 56.48419670448296159 ) ) ;
#44283=CARTESIAN_POINT ( 'NONE',  ( 104.4428039971878803, -26.59488813107328653, 196.2784824187679362 ) ) ;
#44285=EDGE_CURVE ( 'NONE', #13477, #39062, #21795, .T. ) ;
#44286=PLANE ( 'NONE',  #82357 ) ;
#44287=CARTESIAN_POINT ( 'NONE',  ( 182.3467384525657735, -36.02818131005238200, 313.9678068554149490 ) ) ;
#44289=DIRECTION ( 'NONE',  ( 1.000000000000000078E-15, 1.000000000000000083E-30, -1.000000000000000000 ) ) ;
#44290=DIRECTION ( 'NONE',  ( -1.000000000000000078E-15, 0.000000000000000000, 1.000000000000000000 ) ) ;
#44291=EDGE_LOOP ( 'NONE', ( #78716, #53619, #55392, #22828 ) ) ;
#44292=CARTESIAN_POINT ( 'NONE',  ( 107.0664832912739968, -36.72944715994100306, 312.6356252759112522 ) ) ;
#44294=VECTOR ( 'NONE', #52322, 1000.000000000000000 ) ;
#44295=VECTOR ( 'NONE', #18290, 1000.000000000000000 ) ;
#44297=ORIENTED_EDGE ( 'NONE', *, *, #36753, .T. ) ;
#44298=VECTOR ( 'NONE', #69671, 1000.000000000000000 ) ;
#44299=CARTESIAN_POINT ( 'NONE',  ( 99.58293739761768393, -32.55228987500129278, 110.3438483995049495 ) ) ;
#44302=CARTESIAN_POINT ( 'NONE',  ( 102.9796410358630254, -46.29638950891617100, 88.25562527591095829 ) ) ;
#44303=LINE ( 'NONE', #51563, #73085 ) ;
#44304=AXIS2_PLACEMENT_3D ( 'NONE', #7073, #35663, #76562 ) ;
#44305=DIRECTION ( 'NONE',  ( 0.000000000000000000, 0.000000000000000000, 1.000000000000000000 ) ) ;
#44307=CARTESIAN_POINT ( 'NONE',  ( 118.4837085360594671, -37.70862757085654238, 296.0306255462182321 ) ) ;
#44309=CARTESIAN_POINT ( 'NONE',  ( 98.07879527422882404, -32.87106628761745952, 16.00419670448294340 ) ) ;
#44310=ORIENTED_EDGE ( 'NONE', *, *, #20064, .T. ) ;
#44311=EDGE_LOOP ( 'NONE', ( #29289, #44997, #4352, #63070 ) ) ;
#44314=CARTESIAN_POINT ( 'NONE',  ( 141.0667039024479834, -50.82844715994100682, 310.9178068554150514 ) ) ;
#44315=CARTESIAN_POINT ( 'NONE',  ( 134.0664832912740110, -41.22944715994101017, 1.625625275910997480 ) ) ;
#44316=CARTESIAN_POINT ( 'NONE',  ( 188.5667039024483529, -48.82844715993431350, 293.2178068554150059 ) ) ;
#44318=AXIS2_PLACEMENT_3D ( 'NONE', #62388, #35123, #62834 ) ;
#44323=CARTESIAN_POINT ( 'NONE',  ( 110.7866772467784955, -46.44483816919306918, 62.86705384733992474 ) ) ;
#44324=VECTOR ( 'NONE', #38426, 1000.000000000000114 ) ;
#44325=ORIENTED_EDGE ( 'NONE', *, *, #74809, .T. ) ;
#44329=CARTESIAN_POINT ( 'NONE',  ( 98.00070950526129820, -34.75266269402447250, 103.9738046553059547 ) ) ;
#44330=AXIS2_PLACEMENT_3D ( 'NONE', #25843, #19023, #59889 ) ;
#44331=AXIS2_PLACEMENT_3D ( 'NONE', #31167, #72527, #14551 ) ;
#44333=CARTESIAN_POINT ( 'NONE',  ( 163.0664832912739826, 25.62155284005901379, 339.0006252759110339 ) ) ;
#44335=DIRECTION ( 'NONE',  ( 2.999999999999999839E-15, -1.000000000000000000, 2.999999999999999900E-30 ) ) ;
#44340=ORIENTED_EDGE ( 'NONE', *, *, #36349, .T. ) ;
#44341=VERTEX_POINT ( 'NONE', #5927 ) ;
#44342=CARTESIAN_POINT ( 'NONE',  ( 99.32274084468600961, -31.40864097607868999, 162.2911071154209708 ) ) ;
#44344=LINE ( 'NONE', #63921, #14824 ) ;
#44345=CARTESIAN_POINT ( 'NONE',  ( 117.1470005940874728, -33.86231210335883901, 145.0470538473399529 ) ) ;
#44346=DIRECTION ( 'NONE',  ( 0.000000000000000000, 1.000000000000000000, 0.000000000000000000 ) ) ;
#44349=EDGE_LOOP ( 'NONE', ( #27776, #47166 ) ) ;
#44350=EDGE_CURVE ( 'NONE', #55131, #57944, #55819, .T. ) ;
#44351=VECTOR ( 'NONE', #20880, 1000.000000000000000 ) ;
#44356=CARTESIAN_POINT ( 'NONE',  ( 99.23015118009998048, -40.40270512654389279, 209.4814237029249568 ) ) ;
#44357=CARTESIAN_POINT ( 'NONE',  ( 115.2845782536562353, -44.15631435451261666, 83.25372051400698581 ) ) ;
#44359=CARTESIAN_POINT ( 'NONE',  ( 106.6078071710152244, -25.70885557892963647, 40.09753003781596448 ) ) ;
#44360=CARTESIAN_POINT ( 'NONE',  ( 111.9917837115123547, -28.59708332594661684, 249.5838068554156166 ) ) ;
#44361=DIRECTION ( 'NONE',  ( -0.000000000000000000, 1.000000000000000000, 0.000000000000000000 ) ) ;
#44362=CARTESIAN_POINT ( 'NONE',  ( 115.9655611776390458, -32.07238166515693933, 195.2103538287998106 ) ) ;
#44363=CARTESIAN_POINT ( 'NONE',  ( 105.3162569294398168, -48.44961499074708655, 143.4584824187689662 ) ) ;
#44367=ORIENTED_EDGE ( 'NONE', *, *, #34373, .T. ) ;
#44368=DIRECTION ( 'NONE',  ( 0.000000000000000000, 0.000000000000000000, -1.000000000000000000 ) ) ;
#44370=AXIS2_PLACEMENT_3D ( 'NONE', #13948, #5800, #62542 ) ;
#44371=VERTEX_POINT ( 'NONE', #41751 ) ;
#44372=CARTESIAN_POINT ( 'NONE',  ( 82.81648064515525220, -36.72944715939136273, 6.749772901088423538 ) ) ;
#44373=CARTESIAN_POINT ( 'NONE',  ( 48.16670390244701139, -28.27351298637280408, 237.4678068554150059 ) ) ;
#44374=CARTESIAN_POINT ( 'NONE',  ( 110.3719962439868425, -47.27708535874812412, 52.80610146638697699 ) ) ;
#44377=FACE_OUTER_BOUND ( 'NONE', #80930, .T. ) ;
#44378=CARTESIAN_POINT ( 'NONE',  ( 116.3212776292294279, -32.94146857471271517, 75.13562527591093954 ) ) ;
#44379=CARTESIAN_POINT ( 'NONE',  ( 97.54819157151548836, -32.61351373332768588, 61.01372051400699803 ) ) ;
#44380=DIRECTION ( 'NONE',  ( -0.9254794337955620787, -0.3787978585227822492, 0.000000000000000000 ) ) ;
#44381=CARTESIAN_POINT ( 'NONE',  ( 102.7067583520261138, -46.86140753836539119, 133.2651490854349561 ) ) ;
#44383=CARTESIAN_POINT ( 'NONE',  ( 41.56648329127398966, -18.82844715994071194, 78.92562527591199739 ) ) ;
#44387=DIRECTION ( 'NONE',  ( -4.237773401492740281E-14, 1.000000000000000000, 0.000000000000000000 ) ) ;
#44388=LINE ( 'NONE', #72998, #59279 ) ;
#44389=CARTESIAN_POINT ( 'NONE',  ( 113.1812204092734220, -26.51970732500450012, 204.6470538473399756 ) ) ;
#44390=ORIENTED_EDGE ( 'NONE', *, *, #73679, .F. ) ;
#44391=CARTESIAN_POINT ( 'NONE',  ( 97.39140141746301538, -39.27893455387799548, 146.5314937606656258 ) ) ;
#44392=CARTESIAN_POINT ( 'NONE',  ( 117.5124522703044931, -35.85713534702714611, 249.8927681330537780 ) ) ;
#44393=CARTESIAN_POINT ( 'NONE',  ( 103.3469782872468130, -47.18711328981185460, 98.31657765686297523 ) ) ;
#44397=FACE_OUTER_BOUND ( 'NONE', #57612, .T. ) ;
#44398=ORIENTED_EDGE ( 'NONE', *, *, #84045, .F. ) ;
#44399=ORIENTED_EDGE ( 'NONE', *, *, #36633, .F. ) ;
#44400=ORIENTED_EDGE ( 'NONE', *, *, #61262, .T. ) ;
#44403=CARTESIAN_POINT ( 'NONE',  ( 115.6552720357279753, -30.75834705514724732, 275.3099109901965562 ) ) ;
#44404=CARTESIAN_POINT ( 'NONE',  ( 163.1639762274738814, -34.03355364506054315, 342.9256252759109884 ) ) ;
#44406=LINE ( 'NONE', #79418, #11970 ) ;
#44409=CYLINDRICAL_SURFACE ( 'NONE', #86346, 2.500000000000002220 ) ;
#44410=CARTESIAN_POINT ( 'NONE',  ( 98.86656133049426387, -40.57313681482517609, 211.0857531614099685 ) ) ;
#44412=ORIENTED_EDGE ( 'NONE', *, *, #11329, .T. ) ;
#44413=VECTOR ( 'NONE', #59622, 1000.000000000000000 ) ;
#44416=CIRCLE ( 'NONE', #70574, 11.45913725231036118 ) ;
#44417=CIRCLE ( 'NONE', #63305, 1.000000000000000888 ) ;
#44418=CARTESIAN_POINT ( 'NONE',  ( 36.23715912545424089, -47.82818131006125384, 300.4678068554150059 ) ) ;
#44420=CARTESIAN_POINT ( 'NONE',  ( 111.4502655538902758, -27.98611278301861560, 275.7070538473389547 ) ) ;
#44422=FACE_BOUND ( 'NONE', #69360, .T. ) ;
#44425=EDGE_LOOP ( 'NONE', ( #38600, #80301 ) ) ;
#44426=CYLINDRICAL_SURFACE ( 'NONE', #31720, 11.45913725231036118 ) ;
#44427=ORIENTED_EDGE ( 'NONE', *, *, #41909, .T. ) ;
#44430=CARTESIAN_POINT ( 'NONE',  ( 110.8184301750971485, -28.11564833443670608, 281.1692023535160843 ) ) ;
#44432=CARTESIAN_POINT ( 'NONE',  ( 163.2449138993006841, -32.11662333284040471, 237.4678068554150059 ) ) ;
#44433=AXIS2_PLACEMENT_3D ( 'NONE', #56597, #85235, #47188 ) ;
#44435=EDGE_CURVE ( 'NONE', #7721, #83824, #75470, .T. ) ;
#44437=CARTESIAN_POINT ( 'NONE',  ( 183.6524903400785718, -49.32844715993451956, 180.4678068554150343 ) ) ;
#44438=EDGE_LOOP ( 'NONE', ( #28708, #85658, #13360, #29459 ) ) ;
#44439=CARTESIAN_POINT ( 'NONE',  ( 97.81169962758427516, -40.51743340529665005, 76.63548575323150658 ) ) ;
#44440=PLANE ( 'NONE',  #32413 ) ;
#44441=EDGE_CURVE ( 'NONE', #66807, #76993, #78647, .T. ) ;
#44442=ORIENTED_EDGE ( 'NONE', *, *, #19913, .T. ) ;
#44443=CARTESIAN_POINT ( 'NONE',  ( 106.6603292229642790, -26.31205452386275212, 85.10705384733896040 ) ) ;
#44444=ORIENTED_EDGE ( 'NONE', *, *, #60221, .F. ) ;
#44445=EDGE_CURVE ( 'NONE', #38408, #62285, #49464, .T. ) ;
#44446=CARTESIAN_POINT ( 'NONE',  ( 98.27686124684872482, -40.85414981714398408, 61.09813411379100501 ) ) ;
#44447=CARTESIAN_POINT ( 'NONE',  ( 116.6873719206527511, -39.68605214187660124, 89.58883501578704056 ) ) ;
#44448=CARTESIAN_POINT ( 'NONE',  ( 106.7212481586559392, -27.87455634666363835, 81.53872616303998200 ) ) ;
#44449=CARTESIAN_POINT ( 'NONE',  ( 100.8871946602138649, -44.69999506278231394, 13.05226384497917458 ) ) ;
#44453=CIRCLE ( 'NONE', #5319, 1.000000000000000888 ) ;
#44454=CARTESIAN_POINT ( 'NONE',  ( 115.9636596525004677, -42.20459941147550609, 14.38705384733995984 ) ) ;
#44457=CARTESIAN_POINT ( 'NONE',  ( 37.03715912545342093, -48.62818131006128652, 193.9678068554150911 ) ) ;
#44459=CARTESIAN_POINT ( 'NONE',  ( 105.3089409210114269, -48.49860570903479129, 143.4584824187689662 ) ) ;
#44460=LINE ( 'NONE', #78130, #36691 ) ;
#44462=ORIENTED_EDGE ( 'NONE', *, *, #29604, .F. ) ;
#44464=CARTESIAN_POINT ( 'NONE',  ( 32.06670390244800473, -33.35206098992711077, -5.074374724088000832 ) ) ;
#44465=DIRECTION ( 'NONE',  ( -0.0001211784769810537456, 0.7071067708032344745, 0.7071067811865466846 ) ) ;
#44466=CARTESIAN_POINT ( 'NONE',  ( 97.71246005893821973, -41.20616857227592789, 216.6937205140069409 ) ) ;
#44467=CYLINDRICAL_SURFACE ( 'NONE', #24021, 2.117000000000007987 ) ;
#44468=EDGE_CURVE ( 'NONE', #63506, #41573, #43992, .T. ) ;
#44469=DIRECTION ( 'NONE',  ( -4.299999999999999979E-14, 1.000000000000000000, 0.000000000000000000 ) ) ;
#44470=CARTESIAN_POINT ( 'NONE',  ( 172.5664832912729878, -27.57844715994070484, 315.9256252759120116 ) ) ;
#44471=CARTESIAN_POINT ( 'NONE',  ( 96.34427168469159142, -39.41376207380771746, 12.53372051400597442 ) ) ;
#44474=CARTESIAN_POINT ( 'NONE',  ( 103.2778153200627713, -27.47493501435859642, 171.3856854448868887 ) ) ;
#44475=VECTOR ( 'NONE', #61008, 1000.000000000000000 ) ;
#44478=VECTOR ( 'NONE', #86541, 1000.000000000000000 ) ;
#44480=VECTOR ( 'NONE', #41865, 1000.000000000000000 ) ;
#44482=CARTESIAN_POINT ( 'NONE',  ( 97.19046783542276557, -39.99946004141662570, 241.5813395616249863 ) ) ;
#44486=CARTESIAN_POINT ( 'NONE',  ( 29.56648329127298069, -71.37844715994266664, 361.9756252759109998 ) ) ;
#44487=CARTESIAN_POINT ( 'NONE',  ( 116.6718245901296171, -38.14650263757180682, 223.1324198280769622 ) ) ;
#44489=CARTESIAN_POINT ( 'NONE',  ( 117.4658636684176543, -37.01502254527064650, 39.80419670448193159 ) ) ;
#44491=CARTESIAN_POINT ( 'NONE',  ( 117.0754465142714054, -30.29129860725820222, 144.2813395616249750 ) ) ;
#44492=VERTEX_POINT ( 'NONE', #9493 ) ;
#44493=CARTESIAN_POINT ( 'NONE',  ( 180.2143765759491885, -35.91149509761089575, 342.9256252759109884 ) ) ;
#44496=CARTESIAN_POINT ( 'NONE',  ( 100.9546727804262076, -28.70702575035819848, 66.59395861228354363 ) ) ;
#44497=CARTESIAN_POINT ( 'NONE',  ( 107.9134757390494030, -26.74391507959751735, 276.0090606567454188 ) ) ;
#44500=VERTEX_POINT ( 'NONE', #30829 ) ;
#44502=CARTESIAN_POINT ( 'NONE',  ( 41.56648329127499153, -36.32844715994070839, 258.9256252759120116 ) ) ;
#44503=AXIS2_PLACEMENT_3D ( 'NONE', #40467, #29533, #2728 ) ;
#44504=EDGE_CURVE ( 'NONE', #74932, #11728, #15872, .T. ) ;
#44505=CARTESIAN_POINT ( 'NONE',  ( 41.56648329127399677, 0.2215528400590013880, 78.92562527591199739 ) ) ;
#44506=VERTEX_POINT ( 'NONE', #44439 ) ;
#44507=CARTESIAN_POINT ( 'NONE',  ( 113.5198117145332475, -28.51355303769357619, 79.54705384733995288 ) ) ;
#44508=CARTESIAN_POINT ( 'NONE',  ( 142.0664832912740394, -45.72944715994099596, -4.824374724088994704 ) ) ;
#44509=ADVANCED_FACE ( 'NONE', ( #86246 ), #72172, .F. ) ;
#44511=CARTESIAN_POINT ( 'NONE',  ( 33.91903122894598965, -35.91149509761181235, 313.9678068554150059 ) ) ;
#44512=ORIENTED_EDGE ( 'NONE', *, *, #9737, .F. ) ;
#44514=PLANE ( 'NONE',  #81748 ) ;
#44517=DIRECTION ( 'NONE',  ( 0.000000000000000000, 1.000000000000000000, 0.000000000000000000 ) ) ;
#44518=DIRECTION ( 'NONE',  ( 0.000000000000000000, 0.000000000000000000, -1.000000000000000000 ) ) ;
#44519=CIRCLE ( 'NONE', #63415, 2.500000000000002220 ) ;
#44520=VERTEX_POINT ( 'NONE', #43547 ) ;
#44523=CARTESIAN_POINT ( 'NONE',  ( 96.73459541816653484, -35.84013382243349355, 182.2461014663859658 ) ) ;
#44524=DIRECTION ( 'NONE',  ( -4.093947403305260305E-16, 1.000000000000000000, -6.162975822039159109E-32 ) ) ;
#44526=CARTESIAN_POINT ( 'NONE',  ( 115.0831197249979851, -29.02584261466837390, 35.43562527591098643 ) ) ;
#44527=LINE ( 'NONE', #81664, #84670 ) ;
#44528=CYLINDRICAL_SURFACE ( 'NONE', #34246, 2.116999999999993776 ) ;
#44529=DIRECTION ( 'NONE',  ( 0.000000000000000000, 1.000000000000000000, 0.000000000000000000 ) ) ;
#44532=CARTESIAN_POINT ( 'NONE',  ( 107.0664832912739968, -36.72944715994100306, 287.6356252759109680 ) ) ;
#44535=CARTESIAN_POINT ( 'NONE',  ( 101.0525363619397012, -44.44280425155412217, 232.0499109901969632 ) ) ;
#44536=ORIENTED_EDGE ( 'NONE', *, *, #52438, .T. ) ;
#44537=EDGE_LOOP ( 'NONE', ( #41514, #6053, #69540, #13932 ) ) ;
#44538=CARTESIAN_POINT ( 'NONE',  ( 115.5682375124590635, -39.22913789569613385, 180.0301547344689936 ) ) ;
#44539=FACE_OUTER_BOUND ( 'NONE', #22666, .T. ) ;
#44540=AXIS2_PLACEMENT_3D ( 'NONE', #7708, #49015, #443 ) ;
#44541=CARTESIAN_POINT ( 'NONE',  ( 116.9829645355111154, -34.95910688594825189, 45.39872616303996722 ) ) ;
#44544=CARTESIAN_POINT ( 'NONE',  ( 33.91903122894489542, -35.91149509761202552, 117.4678068554150485 ) ) ;
#44545=ORIENTED_EDGE ( 'NONE', *, *, #41558, .F. ) ;
#44546=DIRECTION ( 'NONE',  ( -1.000000000000000000, -2.756263715554006823E-15, 0.000000000000000000 ) ) ;
#44549=CARTESIAN_POINT ( 'NONE',  ( 96.79764630557882299, -40.75620882907056597, 246.6118157521009664 ) ) ;
#44551=EDGE_CURVE ( 'NONE', #78013, #56843, #9946, .T. ) ;
#44558=CARTESIAN_POINT ( 'NONE',  ( 107.0664832912739968, -0.7548456658612000547, 331.7756252759120343 ) ) ;
#44559=VECTOR ( 'NONE', #40354, 1000.000000000000000 ) ;
#44560=CARTESIAN_POINT ( 'NONE',  ( 112.5987260342904648, -28.66361022110277545, 40.59848241876795782 ) ) ;
#44561=DIRECTION ( 'NONE',  ( 0.000000000000000000, -1.000000000000000000, 0.000000000000000000 ) ) ;
#44562=AXIS2_PLACEMENT_3D ( 'NONE', #32369, #47339, #26911 ) ;
#44564=CARTESIAN_POINT ( 'NONE',  ( 105.4141053104174830, -47.06688527371949249, 33.44991099019695469 ) ) ;
#44566=CARTESIAN_POINT ( 'NONE',  ( 113.7561043996362287, -29.08408549058404091, 289.5032443235301116 ) ) ;
#44567=EDGE_LOOP ( 'NONE', ( #13065, #6565, #4721, #46774 ) ) ;
#44572=CARTESIAN_POINT ( 'NONE',  ( 59.67079009362632291, -0.9310397146383333489, 540.9756252759101471 ) ) ;
#44575=CARTESIAN_POINT ( 'NONE',  ( 115.1095529034481331, -33.53414494269306800, 96.95761417911496949 ) ) ;
#44576=CARTESIAN_POINT ( 'NONE',  ( 113.0346028865331363, -45.34691455509256031, 199.0584824187679374 ) ) ;
#44580=DIRECTION ( 'NONE',  ( 0.000000000000000000, 0.000000000000000000, -1.000000000000000000 ) ) ;
#44581=EDGE_LOOP ( 'NONE', ( #9519, #25752, #43535, #14903, #13658, #39837, #38216, #14026 ) ) ;
#44584=DIRECTION ( 'NONE',  ( 1.000000000000000000, 6.145690160522439356E-16, 0.000000000000000000 ) ) ;
#44585=ORIENTED_EDGE ( 'NONE', *, *, #77186, .T. ) ;
#44586=ORIENTED_EDGE ( 'NONE', *, *, #63680, .F. ) ;
#44587=CARTESIAN_POINT ( 'NONE',  ( 116.0733447696779592, -32.33582790950384833, 40.18770276530661079 ) ) ;
#44588=CARTESIAN_POINT ( 'NONE',  ( 115.6810990589499397, -33.93640840262257541, 133.5105150661719620 ) ) ;
#44589=CARTESIAN_POINT ( 'NONE',  ( 100.3828542815028015, -28.67117381486349004, 40.62705384733894221 ) ) ;
#44591=ORIENTED_EDGE ( 'NONE', *, *, #14435, .F. ) ;
#44593=ORIENTED_EDGE ( 'NONE', *, *, #22455, .F. ) ;
#44594=DIRECTION ( 'NONE',  ( 1.000000000000000078E-15, -1.000000000000000000, 0.000000000000000000 ) ) ;
#44595=AXIS2_PLACEMENT_3D ( 'NONE', #7748, #13665, #55422 ) ;
#44598=VECTOR ( 'NONE', #49883, 1000.000000000000000 ) ;
#44599=CARTESIAN_POINT ( 'NONE',  ( 182.0667039024478981, -33.35206098992058799, 193.9678068554150059 ) ) ;
#44602=CIRCLE ( 'NONE', #46086, 2.517500000000005844 ) ;
#44603=CARTESIAN_POINT ( 'NONE',  ( 100.1386363970297992, -44.51995214173314963, 266.9984824187679919 ) ) ;
#44604=CARTESIAN_POINT ( 'NONE',  ( 105.3131098409624542, -26.40875552125079295, 11.20991099019697046 ) ) ;
#44606=CARTESIAN_POINT ( 'NONE',  ( 188.5667039024479834, -58.35344715994099829, 137.2178068554150059 ) ) ;
#44607=DIRECTION ( 'NONE',  ( -1.000000000000000000, -6.814610998690690172E-14, -1.000000000000000078E-15 ) ) ;
#44609=EDGE_CURVE ( 'NONE', #54188, #5456, #16759, .T. ) ;
#44610=CARTESIAN_POINT ( 'NONE',  ( 106.5177191205505665, -25.28303833615382601, 323.5373862996826233 ) ) ;
#44611=CARTESIAN_POINT ( 'NONE',  ( 156.5667039024485518, -48.82844715993568485, 173.2178068554149775 ) ) ;
#44612=FACE_OUTER_BOUND ( 'NONE', #43057, .T. ) ;
#44613=CARTESIAN_POINT ( 'NONE',  ( 107.3428450438784694, -25.27364292152175551, 322.4523926293242653 ) ) ;
#44615=AXIS2_PLACEMENT_3D ( 'NONE', #8659, #1843, #36357 ) ;
#44616=DIRECTION ( 'NONE',  ( 1.000000000000000000, 2.999999999999999839E-15, 1.000000000000000078E-15 ) ) ;
#44617=CARTESIAN_POINT ( 'NONE',  ( 162.5667039024470171, -32.29483332968611364, -5.074374724088000832 ) ) ;
#44618=CARTESIAN_POINT ( 'NONE',  ( 96.51457183773001702, -40.09881715592517537, 281.5603871806727625 ) ) ;
#44619=CARTESIAN_POINT ( 'NONE',  ( 117.2915085808104436, -34.52259632565112213, 179.9956252759109532 ) ) ;
#44620=CARTESIAN_POINT ( 'NONE',  ( 97.26802889450139844, -33.10625101732204456, 62.04419670448196911 ) ) ;
#44622=CARTESIAN_POINT ( 'NONE',  ( 41.56648329127499153, -36.32844715994070839, 198.9256252759119832 ) ) ;
#44624=DIRECTION ( 'NONE',  ( -1.000000000000000000, -4.299999999999999979E-14, -1.000000000000000078E-15 ) ) ;
#44625=AXIS2_PLACEMENT_3D ( 'NONE', #59834, #87566, #25326 ) ;
#44626=ADVANCED_FACE ( 'NONE', ( #15429 ), #63561, .F. ) ;
#44627=VERTEX_POINT ( 'NONE', #57632 ) ;
#44631=CARTESIAN_POINT ( 'NONE',  ( 101.3216544293210291, -28.81361639883588310, 71.57562527591099411 ) ) ;
#44632=ADVANCED_FACE ( 'NONE', ( #3129 ), #64019, .T. ) ;
#44636=CARTESIAN_POINT ( 'NONE',  ( 116.3579325164319016, -41.40893824611048757, 199.4556252759109611 ) ) ;
#44638=CARTESIAN_POINT ( 'NONE',  ( 29.56670390244797630, -67.87844715994100397, 300.9178068554150514 ) ) ;
#44639=CARTESIAN_POINT ( 'NONE',  ( 134.0664832912740110, 0.2215528400590013880, 4.925625275911999168 ) ) ;
#44643=CARTESIAN_POINT ( 'NONE',  ( 188.5667039024479834, -62.87844715994099687, 293.2178068554150627 ) ) ;
#44644=CARTESIAN_POINT ( 'NONE',  ( 97.83898487876174954, -40.58353653247343829, 96.64131800056416921 ) ) ;
#44645=CARTESIAN_POINT ( 'NONE',  ( 98.32242264099468798, -42.30440888850458947, 141.7661014663879655 ) ) ;
#44646=ORIENTED_EDGE ( 'NONE', *, *, #74819, .T. ) ;
#44647=VERTEX_POINT ( 'NONE', #72620 ) ;
#44648=AXIS2_PLACEMENT_3D ( 'NONE', #8185, #35878, #57664 ) ;
#44649=EDGE_CURVE ( 'NONE', #44152, #61107, #58073, .T. ) ;
#44650=CARTESIAN_POINT ( 'NONE',  ( 113.9519893150074239, -42.30780582616069552, 84.71586902018296428 ) ) ;
#44653=CARTESIAN_POINT ( 'NONE',  ( 97.78144721833434971, -39.80378292816723018, 237.5813395616249579 ) ) ;
#44654=CYLINDRICAL_SURFACE ( 'NONE', #15794, 5.599999999999994316 ) ;
#44656=ADVANCED_FACE ( 'NONE', ( #24911 ), #46215, .T. ) ;
#44662=CARTESIAN_POINT ( 'NONE',  ( 113.6008039948045933, -28.63430547549723570, 164.5356252759109736 ) ) ;
#44663=ORIENTED_EDGE ( 'NONE', *, *, #11337, .T. ) ;
#44669=FACE_OUTER_BOUND ( 'NONE', #27484, .T. ) ;
#44671=AXIS2_PLACEMENT_3D ( 'NONE', #4879, #73459, #34696 ) ;
#44672=AXIS2_PLACEMENT_3D ( 'NONE', #37263, #87203, #65843 ) ;
#44673=FACE_OUTER_BOUND ( 'NONE', #59198, .T. ) ;
#44674=CARTESIAN_POINT ( 'NONE',  ( 112.7802237386950992, -45.44955040250216172, 178.0384824187679556 ) ) ;
#44675=DIRECTION ( 'NONE',  ( 1.000000000000000000, 0.000000000000000000, 0.000000000000000000 ) ) ;
#44677=ORIENTED_EDGE ( 'NONE', *, *, #35543, .F. ) ;
#44679=EDGE_CURVE ( 'NONE', #59746, #63259, #73952, .T. ) ;
#44681=CARTESIAN_POINT ( 'NONE',  ( 116.2822504412707474, -40.65736861940501257, 64.50652713745955680 ) ) ;
#44683=EDGE_CURVE ( 'NONE', #39224, #57751, #4012, .T. ) ;
#44685=EDGE_CURVE ( 'NONE', #34522, #65168, #60755, .T. ) ;
#44686=CARTESIAN_POINT ( 'NONE',  ( 111.0839405624553251, -29.06298261359865975, 12.49856656006798161 ) ) ;
#44687=VECTOR ( 'NONE', #89193, 1000.000000000000000 ) ;
#44691=AXIS2_PLACEMENT_3D ( 'NONE', #44051, #77705, #71786 ) ;
#44692=CARTESIAN_POINT ( 'NONE',  ( 114.0862517022053026, -42.18719852450433194, 9.635625275910939536 ) ) ;
#44694=EDGE_LOOP ( 'NONE', ( #4251, #30443, #62974, #38771 ) ) ;
#44695=ORIENTED_EDGE ( 'NONE', *, *, #62088, .T. ) ;
#44696=CARTESIAN_POINT ( 'NONE',  ( 98.54785696274898044, -41.97731333288708555, 111.7658622444392194 ) ) ;
#44697=ORIENTED_EDGE ( 'NONE', *, *, #20741, .T. ) ;
#44699=AXIS2_PLACEMENT_3D ( 'NONE', #6390, #55412, #76781 ) ;
#44700=CARTESIAN_POINT ( 'NONE',  ( 111.2570682682515439, -29.25341213619239156, 34.09241982807698434 ) ) ;
#44701=CARTESIAN_POINT ( 'NONE',  ( 99.99311136543857970, -27.18998042936580362, 185.5841967044829630 ) ) ;
#44702=CARTESIAN_POINT ( 'NONE',  ( 108.0049669398584911, -26.36739623290726442, 155.0041967044819557 ) ) ;
#44703=CARTESIAN_POINT ( 'NONE',  ( 41.56648329127499153, -36.32844715994070839, 23.67562527591200094 ) ) ;
#44704=CARTESIAN_POINT ( 'NONE',  ( 115.7761331719916171, -31.00018137778016936, 250.2899109901966028 ) ) ;
#44708=VERTEX_POINT ( 'NONE', #25799 ) ;
#44712=CARTESIAN_POINT ( 'NONE',  ( 98.22399452165288380, -42.33453934503185678, 186.7756252759109543 ) ) ;
#44714=CARTESIAN_POINT ( 'NONE',  ( 116.8067323440835565, -43.47985705614018315, 163.3441967044829823 ) ) ;
#44715=CARTESIAN_POINT ( 'NONE',  ( 182.3467384525655746, -29.62846900981658393, 237.4678068554150059 ) ) ;
#44716=LINE ( 'NONE', #17910, #81236 ) ;
#44718=DIRECTION ( 'NONE',  ( -1.000000000000000078E-15, 0.000000000000000000, 1.000000000000000000 ) ) ;
#44720=CARTESIAN_POINT ( 'NONE',  ( 115.5963437193832277, -42.63132022635295471, 9.356577656862985037 ) ) ;
#44721=FACE_OUTER_BOUND ( 'NONE', #39278, .T. ) ;
#44725=CARTESIAN_POINT ( 'NONE',  ( 128.7748166246070127, 12.92155284005802685, 335.5992267699912190 ) ) ;
#44726=DIRECTION ( 'NONE',  ( 0.000000000000000000, 0.000000000000000000, -1.000000000000000000 ) ) ;
#44727=CARTESIAN_POINT ( 'NONE',  ( 115.3744406058151384, -34.23201694794762062, 195.5838068554167535 ) ) ;
#44729=CIRCLE ( 'NONE', #73788, 10.00000000000000711 ) ;
#44730=CARTESIAN_POINT ( 'NONE',  ( 136.1600792930010471, -20.51483178662487816, 7.477467810847014285 ) ) ;
#44731=CARTESIAN_POINT ( 'NONE',  ( 95.38311866650811055, -38.85853310224461410, 201.4699109901969791 ) ) ;
#44732=CARTESIAN_POINT ( 'NONE',  ( 101.1410050838726846, -27.39870825576502966, 61.51467289495899138 ) ) ;
#44733=CARTESIAN_POINT ( 'NONE',  ( 113.0503328260151079, -46.07776482166018184, 214.0175300378159591 ) ) ;
#44734=DIRECTION ( 'NONE',  ( -0.7071067811892205457, 0.7071067811838745998, -7.071067811891901187E-16 ) ) ;
#44736=DIRECTION ( 'NONE',  ( 0.000000000000000000, 0.000000000000000000, 1.000000000000000000 ) ) ;
#44737=CARTESIAN_POINT ( 'NONE',  ( 97.81298107105155282, -40.52058258403540236, 37.63560581694255802 ) ) ;
#44741=CARTESIAN_POINT ( 'NONE',  ( 102.0683761184610603, -27.96971721533909161, 65.49117886461755234 ) ) ;
#44743=AXIS2_PLACEMENT_3D ( 'NONE', #67245, #53592, #66346 ) ;
#44744=EDGE_CURVE ( 'NONE', #50014, #71626, #81239, .T. ) ;
#44745=VERTEX_POINT ( 'NONE', #65781 ) ;
#44746=EDGE_CURVE ( 'NONE', #16504, #67149, #37789, .T. ) ;
#44747=ORIENTED_EDGE ( 'NONE', *, *, #42507, .T. ) ;
#44748=CARTESIAN_POINT ( 'NONE',  ( 111.7654875973913278, -45.22591620450738503, 102.4009912566479557 ) ) ;
#44750=EDGE_CURVE ( 'NONE', #54515, #42076, #88035, .T. ) ;
#44751=DIRECTION ( 'NONE',  ( 0.7071067811868657627, 0.7071067811862293828, 7.071067811868962098E-16 ) ) ;
#44752=ORIENTED_EDGE ( 'NONE', *, *, #533, .F. ) ;
#44753=CARTESIAN_POINT ( 'NONE',  ( 101.5125196766230857, -27.93273449574876111, 106.5241967044819944 ) ) ;
#44754=DIRECTION ( 'NONE',  ( 3.999999999999999995E-14, -1.000000000000000000, 4.100000000000000342E-29 ) ) ;
#44757=EDGE_CURVE ( 'NONE', #45388, #88176, #53469, .T. ) ;
#44758=EDGE_CURVE ( 'NONE', #20709, #3896, #86695, .T. ) ;
#44760=CIRCLE ( 'NONE', #1269, 11.45913725231036118 ) ;
#44761=CARTESIAN_POINT ( 'NONE',  ( 117.3951115944451402, -37.65585020919953507, 33.74324432352998571 ) ) ;
#44763=ORIENTED_EDGE ( 'NONE', *, *, #57679, .T. ) ;
#44764=VERTEX_POINT ( 'NONE', #81681 ) ;
#44766=FACE_OUTER_BOUND ( 'NONE', #86984, .T. ) ;
#44767=DIRECTION ( 'NONE',  ( 1.000000000000000000, 4.163336342344333240E-14, 0.000000000000000000 ) ) ;
#44768=CARTESIAN_POINT ( 'NONE',  ( 104.4899544570823622, -26.97880758339827878, 116.2814586088303912 ) ) ;
#44771=ADVANCED_FACE ( 'NONE', ( #80333 ), #2977, .F. ) ;
#44772=CARTESIAN_POINT ( 'NONE',  ( 97.06381352669615126, -37.34181605626559275, 52.37546128077145369 ) ) ;
#44773=AXIS2_PLACEMENT_3D ( 'NONE', #65711, #31185, #58885 ) ;
#44776=CARTESIAN_POINT ( 'NONE',  ( 117.2454586689012359, -38.87819698039184146, 63.66133956162494911 ) ) ;
#44777=ORIENTED_EDGE ( 'NONE', *, *, #85729, .F. ) ;
#44780=DIRECTION ( 'NONE',  ( -1.000000000000000078E-15, 1.000000000000000083E-30, 1.000000000000000000 ) ) ;
#44783=CARTESIAN_POINT ( 'NONE',  ( 107.8241526860280430, -28.10814435038363968, 107.8128522743529771 ) ) ;
#44785=EDGE_CURVE ( 'NONE', #28914, #41711, #70615, .T. ) ;
#44786=CARTESIAN_POINT ( 'NONE',  ( 179.4595971212725090, -26.00627455218570105, 193.9678068554150059 ) ) ;
#44787=LINE ( 'NONE', #84816, #54639 ) ;
#44789=VERTEX_POINT ( 'NONE', #7043 ) ;
#44790=CARTESIAN_POINT ( 'NONE',  ( 29.56670390244797630, -67.87844715994100397, 310.9178068554150514 ) ) ;
#44791=ORIENTED_EDGE ( 'NONE', *, *, #16790, .T. ) ;
#44793=EDGE_CURVE ( 'NONE', #1145, #48357, #7492, .T. ) ;
#44794=CARTESIAN_POINT ( 'NONE',  ( 99.72946911866242203, -30.86048229651775543, 192.2092023535159626 ) ) ;
#44797=EDGE_CURVE ( 'NONE', #34742, #89397, #34739, .T. ) ;
#44798=CARTESIAN_POINT ( 'NONE',  ( 113.0894857754661587, -28.19359922731340262, 125.5870538473399591 ) ) ;
#44799=CARTESIAN_POINT ( 'NONE',  ( 104.4899545353706856, -26.97880756368666155, 120.2814586024699679 ) ) ;
#44800=CARTESIAN_POINT ( 'NONE',  ( 105.7154773078611640, -46.72385838936182978, 83.46895860744972140 ) ) ;
#44801=EDGE_LOOP ( 'NONE', ( #8536, #43552 ) ) ;
#44803=VERTEX_POINT ( 'NONE', #14765 ) ;
#44805=CARTESIAN_POINT ( 'NONE',  ( 99.49937927431119533, -39.79027430526630127, 204.4509475124479536 ) ) ;
#44806=CIRCLE ( 'NONE', #10018, 10.00000000000002665 ) ;
#44807=CARTESIAN_POINT ( 'NONE',  ( 118.0253644177900156, -38.34139182134431678, 73.72229194257801055 ) ) ;
#44809=CARTESIAN_POINT ( 'NONE',  ( 118.0525141433398773, -37.71481444994964960, 33.74324432352998571 ) ) ;
#44810=FACE_OUTER_BOUND ( 'NONE', #27683, .T. ) ;
#44811=CARTESIAN_POINT ( 'NONE',  ( 116.3263622980238097, -32.93962144782776846, 195.1356252759109680 ) ) ;
#44812=CARTESIAN_POINT ( 'NONE',  ( 114.5121600660089030, -29.42679343410769377, 145.4441967044819819 ) ) ;
#44814=ORIENTED_EDGE ( 'NONE', *, *, #80664, .T. ) ;
#44815=AXIS2_PLACEMENT_3D ( 'NONE', #75060, #6034, #33724 ) ;
#44817=ORIENTED_EDGE ( 'NONE', *, *, #14443, .F. ) ;
#44821=ORIENTED_EDGE ( 'NONE', *, *, #83241, .T. ) ;
#44822=EDGE_CURVE ( 'NONE', #21130, #22928, #49248, .T. ) ;
#44823=DIRECTION ( 'NONE',  ( 0.1041461484700691442, -0.008931931031208442673, 0.9945218953682739560 ) ) ;
#44825=CARTESIAN_POINT ( 'NONE',  ( 115.7287795988047634, -43.59557489936061359, 48.30514908543492680 ) ) ;
#44826=CARTESIAN_POINT ( 'NONE',  ( 71.25416588882602298, -72.55705569728901594, 396.9756252759102040 ) ) ;
#44827=LINE ( 'NONE', #87519, #57941 ) ;
#44828=DIRECTION ( 'NONE',  ( -4.237773401492740281E-14, 1.000000000000000000, 0.000000000000000000 ) ) ;
#44829=CARTESIAN_POINT ( 'NONE',  ( 100.7170190823676279, -45.85612711270997011, 87.09276813305393716 ) ) ;
#44830=CARTESIAN_POINT ( 'NONE',  ( 168.0371591254545365, -48.62818131005519007, 193.9678068554149775 ) ) ;
#44831=CARTESIAN_POINT ( 'NONE',  ( 104.5678333644584228, -48.28820816006142991, 178.4070538473399665 ) ) ;
#44832=DIRECTION ( 'NONE',  ( 0.000000000000000000, 1.000000000000000000, 0.000000000000000000 ) ) ;
#44834=EDGE_LOOP ( 'NONE', ( #11285, #35356, #22215, #56293 ) ) ;
#44835=AXIS2_PLACEMENT_3D ( 'NONE', #37696, #16358, #63608 ) ;
#44836=CARTESIAN_POINT ( 'NONE',  ( 83.73314995793998605, 12.92155284005730387, 361.9756252759109998 ) ) ;
#44837=LINE ( 'NONE', #18027, #26767 ) ;
#44838=CARTESIAN_POINT ( 'NONE',  ( 97.70690373477779644, -40.25222842886677199, 136.6132999708127613 ) ) ;
#44839=LINE ( 'NONE', #58906, #34646 ) ;
#44840=CARTESIAN_POINT ( 'NONE',  ( 106.2986956077118208, -47.17057584017531724, 222.5184824187679453 ) ) ;
#44842=DIRECTION ( 'NONE',  ( 2.041950104878631501E-14, -0.7071067811865493491, 0.7071067811865455743 ) ) ;
#44843=CARTESIAN_POINT ( 'NONE',  ( 115.9784307414374780, -30.15203137637957909, 255.3203871806729524 ) ) ;
#44844=CARTESIAN_POINT ( 'NONE',  ( 113.9455412938869330, -28.01876065682782624, 120.5565776568639507 ) ) ;
#44845=DIRECTION ( 'NONE',  ( 0.7071067811865171526, 0.7071067811865779928, 7.071067811865164719E-16 ) ) ;
#44848=ADVANCED_FACE ( 'NONE', ( #76984 ), #76529, .F. ) ;
#44849=LINE ( 'NONE', #3519, #55817 ) ;
#44850=CARTESIAN_POINT ( 'NONE',  ( 100.8872838973176584, -44.70006880583113684, 263.0523720315491687 ) ) ;
#44853=ORIENTED_EDGE ( 'NONE', *, *, #8866, .T. ) ;
#44855=ORIENTED_EDGE ( 'NONE', *, *, #81603, .F. ) ;
#44858=CARTESIAN_POINT ( 'NONE',  ( 100.8874678687824229, -44.70022136308342908, 72.05229194101603696 ) ) ;
#44859=CARTESIAN_POINT ( 'NONE',  ( 105.7763715259175257, -26.38449191207581634, 266.1756252759109884 ) ) ;
#44861=CARTESIAN_POINT ( 'NONE',  ( 131.4836309258849383, -35.78502016655559714, 2.871594975603882993 ) ) ;
#44863=ADVANCED_FACE ( 'NONE', ( #28368 ), #1581, .F. ) ;
#44866=CARTESIAN_POINT ( 'NONE',  ( 48.16670390244701139, -26.71338133339251542, -5.074374724088000832 ) ) ;
#44867=CARTESIAN_POINT ( 'NONE',  ( 112.5429177363308924, -43.28420096851815657, 192.5524198280769781 ) ) ;
#44869=ORIENTED_EDGE ( 'NONE', *, *, #48532, .F. ) ;
#44870=AXIS2_PLACEMENT_3D ( 'NONE', #22628, #43482, #43031 ) ;
#44873=ADVANCED_FACE ( 'NONE', ( #14311 ), #83805, .F. ) ;
#44876=CARTESIAN_POINT ( 'NONE',  ( 97.51798391995397708, -31.03399779358258215, 276.8984824187675713 ) ) ;
#44880=LINE ( 'NONE', #11255, #23033 ) ;
#44882=VERTEX_POINT ( 'NONE', #1126 ) ;
#44883=CARTESIAN_POINT ( 'NONE',  ( 20.03715912545741418, -46.82818131006202123, 117.4678068554150485 ) ) ;
#44884=EDGE_LOOP ( 'NONE', ( #1620, #75749, #75884, #17673 ) ) ;
#44885=CARTESIAN_POINT ( 'NONE',  ( 105.1735626975883662, -45.17443245699572429, 25.20713798863899413 ) ) ;
#44886=CARTESIAN_POINT ( 'NONE',  ( 165.6738106836199904, -26.00627455219321860, -5.074374724088000832 ) ) ;
#44889=CARTESIAN_POINT ( 'NONE',  ( 176.7669697523281229, -48.62818131005231947, 129.9678068554150059 ) ) ;
#44890=ORIENTED_EDGE ( 'NONE', *, *, #12787, .F. ) ;
#44893=ORIENTED_EDGE ( 'NONE', *, *, #50413, .F. ) ;
#44894=CARTESIAN_POINT ( 'NONE',  ( 95.34890500915419409, -34.95776856631113105, 71.20705384733993526 ) ) ;
#44896=CARTESIAN_POINT ( 'NONE',  ( 116.0863591824327443, -37.53846460971577415, 33.16575316141096152 ) ) ;
#44897=CARTESIAN_POINT ( 'NONE',  ( 179.8585841295800094, -30.08671355700241179, -5.074374724088000832 ) ) ;
#44898=CARTESIAN_POINT ( 'NONE',  ( 101.3137116872897820, -44.99844491211269570, 83.52444044875394979 ) ) ;
#44900=CARTESIAN_POINT ( 'NONE',  ( 107.0664832912739968, -18.82844715994099971, 168.9256252759119832 ) ) ;
#44901=ADVANCED_FACE ( 'NONE', ( #36548 ), #22471, .T. ) ;
#44904=CARTESIAN_POINT ( 'NONE',  ( 100.5371587349295055, -27.78220587661078156, 26.56610146638793779 ) ) ;
#44905=CARTESIAN_POINT ( 'NONE',  ( 179.8608231853560255, -35.55794170701751256, -5.074374724088000832 ) ) ;
#44908=ORIENTED_EDGE ( 'NONE', *, *, #78221, .T. ) ;
#44909=PLANE ( 'NONE',  #17807 ) ;
#44910=VERTEX_POINT ( 'NONE', #49704 ) ;
#44912=DIRECTION ( 'NONE',  ( 2.900000000000000265E-14, -2.000000000000000155E-15, 1.000000000000000000 ) ) ;
#44914=CARTESIAN_POINT ( 'NONE',  ( 106.9482321581270270, -47.09886382165569785, 232.5794347997209854 ) ) ;
#44917=CARTESIAN_POINT ( 'NONE',  ( 107.3210293350295501, -25.67914459413323058, 71.04610146638795243 ) ) ;
#44918=LINE ( 'NONE', #87172, #65374 ) ;
#44920=CARTESIAN_POINT ( 'NONE',  ( 97.06384307882487406, -37.34221630416103466, 172.3751823342733758 ) ) ;
#44921=CIRCLE ( 'NONE', #5784, 5.500000000000000888 ) ;
#44922=CARTESIAN_POINT ( 'NONE',  ( 172.5664832912740110, -36.32844715994070839, 318.9256252759120116 ) ) ;
#44924=CIRCLE ( 'NONE', #70898, 2.749999999999974687 ) ;
#44926=ADVANCED_FACE ( 'NONE', ( #41988 ), #63803, .F. ) ;
#44928=CYLINDRICAL_SURFACE ( 'NONE', #23750, 2.750000000000002665 ) ;
#44929=CARTESIAN_POINT ( 'NONE',  ( 100.7633749303630850, -45.78122309449486949, 237.0803871806729717 ) ) ;
#44932=DIRECTION ( 'NONE',  ( 1.000000000000000000, 0.000000000000000000, -7.043400939473319300E-33 ) ) ;
#44933=CARTESIAN_POINT ( 'NONE',  ( 106.4400806841681231, -45.24788313703638210, 221.9409912566479477 ) ) ;
#44935=CARTESIAN_POINT ( 'NONE',  ( 114.5517459224756038, -44.00510994954048982, 94.21276813305395592 ) ) ;
#44937=CARTESIAN_POINT ( 'NONE',  ( 114.7585751371172051, -43.83144610948713193, 123.2327681330539519 ) ) ;
#44938=ORIENTED_EDGE ( 'NONE', *, *, #46092, .T. ) ;
#44940=ORIENTED_EDGE ( 'NONE', *, *, #34513, .T. ) ;
#44941=VECTOR ( 'NONE', #66818, 1000.000000000000000 ) ;
#44943=DIRECTION ( 'NONE',  ( -0.7071067812160279908, 0.7071067811570671546, -6.612322856135836109E-17 ) ) ;
#44944=LINE ( 'NONE', #60810, #38379 ) ;
#44946=DIRECTION ( 'NONE',  ( -1.000000000000000000, -4.299999999999999979E-14, -1.000000000000000078E-15 ) ) ;
#44947=ORIENTED_EDGE ( 'NONE', *, *, #47214, .F. ) ;
#44949=AXIS2_PLACEMENT_3D ( 'NONE', #29074, #63591, #915 ) ;
#44953=CARTESIAN_POINT ( 'NONE',  ( 98.18350318933659082, -43.34670532666833509, 111.8480062282919647 ) ) ;
#44955=CARTESIAN_POINT ( 'NONE',  ( 97.60795516317995180, -39.98261623142427368, 166.5900807200408735 ) ) ;
#44957=DIRECTION ( 'NONE',  ( -6.524622321627019585E-16, -3.741823817616790462E-31, -1.000000000000000000 ) ) ;
#44959=EDGE_CURVE ( 'NONE', #32600, #87802, #48795, .T. ) ;
#44960=EDGE_CURVE ( 'NONE', #66809, #29859, #32062, .T. ) ;
#44961=ORIENTED_EDGE ( 'NONE', *, *, #27025, .T. ) ;
#44962=FACE_OUTER_BOUND ( 'NONE', #60788, .T. ) ;
#44963=CARTESIAN_POINT ( 'NONE',  ( 177.8371591254544910, -47.82818131005477369, 193.9678068554150059 ) ) ;
#44964=ADVANCED_FACE ( 'NONE', ( #78787 ), #59192, .T. ) ;
#44965=DIRECTION ( 'NONE',  ( -0.1811243269278930978, 0.9834602067165288952, 0.000000000000000000 ) ) ;
#44966=EDGE_CURVE ( 'NONE', #10962, #20321, #16991, .T. ) ;
#44967=CARTESIAN_POINT ( 'NONE',  ( 37.56670390244743629, -48.82844715994126261, 180.4678068554150911 ) ) ;
#44969=DIRECTION ( 'NONE',  ( 0.7071067811865774377, -0.7071067811865175967, 7.071067811865782003E-16 ) ) ;
#44970=AXIS2_PLACEMENT_3D ( 'NONE', #64570, #86803, #45873 ) ;
#44971=ORIENTED_EDGE ( 'NONE', *, *, #63136, .F. ) ;
#44972=DIRECTION ( 'NONE',  ( 1.000000000000000000, 6.831565154159360295E-14, 0.000000000000000000 ) ) ;
#44973=CARTESIAN_POINT ( 'NONE',  ( 99.18511857479145988, -30.88155312011797804, 176.8184824187669619 ) ) ;
#44974=ADVANCED_FACE ( 'NONE', ( #44673 ), #78343, .F. ) ;
#44978=CARTESIAN_POINT ( 'NONE',  ( 103.0217603822331398, -26.37318333953113836, 16.37276813305293999 ) ) ;
#44979=CARTESIAN_POINT ( 'NONE',  ( 141.8664832912729992, -1.929447159941394263, 342.9256252759109316 ) ) ;
#44980=CARTESIAN_POINT ( 'NONE',  ( 138.8545562996767444, -1.932463243632620342, 361.9756252759100335 ) ) ;
#44982=VECTOR ( 'NONE', #23768, 1000.000000000000000 ) ;
#44987=CARTESIAN_POINT ( 'NONE',  ( 113.8438844162330810, -30.22226962059244215, 185.8549166392299696 ) ) ;
#44991=LINE ( 'NONE', #24567, #8409 ) ;
#44992=AXIS2_PLACEMENT_3D ( 'NONE', #5389, #20368, #60786 ) ;
#44993=FACE_OUTER_BOUND ( 'NONE', #71823, .T. ) ;
#44994=ORIENTED_EDGE ( 'NONE', *, *, #77395, .F. ) ;
#44995=CARTESIAN_POINT ( 'NONE',  ( 34.96670390244619853, -28.27351298637401200, 342.9256252759109884 ) ) ;
#44997=ORIENTED_EDGE ( 'NONE', *, *, #69352, .T. ) ;
#44998=CARTESIAN_POINT ( 'NONE',  ( 115.6772654923307613, -42.56752007954070649, 273.3527681330537575 ) ) ;
#45000=EDGE_LOOP ( 'NONE', ( #78706, #32118 ) ) ;
#45003=AXIS2_PLACEMENT_3D ( 'NONE', #28993, #36250, #52395 ) ;
#45006=EDGE_CURVE ( 'NONE', #45258, #66312, #16105, .T. ) ;
#45007=CARTESIAN_POINT ( 'NONE',  ( 96.14593026560288536, -32.00158989507077223, 207.0013395616249738 ) ) ;
#45009=ORIENTED_EDGE ( 'NONE', *, *, #25487, .F. ) ;
#45010=CARTESIAN_POINT ( 'NONE',  ( 96.88468944541251915, -39.16338508605922186, 52.51276813305394597 ) ) ;
#45011=DIRECTION ( 'NONE',  ( -2.999999999999999839E-15, 1.000000000000000000, -2.999999999999999900E-30 ) ) ;
#45012=ADVANCED_FACE ( 'NONE', ( #52356 ), #58316, .T. ) ;
#45013=CARTESIAN_POINT ( 'NONE',  ( 102.3791524630845799, -47.61053145109372764, 287.2527681330536780 ) ) ;
#45015=AXIS2_PLACEMENT_3D ( 'NONE', #63734, #43267, #36481 ) ;
#45016=AXIS2_PLACEMENT_3D ( 'NONE', #64638, #4203, #87324 ) ;
#45017=CARTESIAN_POINT ( 'NONE',  ( 80.71968614772718809, -16.05633243510678554, 1.689562801603858633 ) ) ;
#45018=CARTESIAN_POINT ( 'NONE',  ( 116.3162594664470788, -32.94075446336835000, 20.13562527591095019 ) ) ;
#45020=CARTESIAN_POINT ( 'NONE',  ( 111.3320211711901067, -29.76992759232029329, 92.45666179816296903 ) ) ;
#45021=CARTESIAN_POINT ( 'NONE',  ( 109.9662181263222891, -48.24525319228295217, 238.7727681330539724 ) ) ;
#45022=PLANE ( 'NONE',  #56544 ) ;
#45023=ORIENTED_EDGE ( 'NONE', *, *, #29807, .F. ) ;
#45026=ORIENTED_EDGE ( 'NONE', *, *, #33163, .F. ) ;
#45027=ORIENTED_EDGE ( 'NONE', *, *, #24762, .T. ) ;
#45028=EDGE_CURVE ( 'NONE', #8645, #39224, #53640, .T. ) ;
#45029=CARTESIAN_POINT ( 'NONE',  ( 41.56648329127398966, -27.57844715994070484, 195.9256252759119832 ) ) ;
#45030=ORIENTED_EDGE ( 'NONE', *, *, #78640, .T. ) ;
#45032=CARTESIAN_POINT ( 'NONE',  ( 97.81493411881378108, -40.51644251795452334, 167.6359250042934264 ) ) ;
#45034=CARTESIAN_POINT ( 'NONE',  ( 103.3756532791179126, -27.43539013423222173, 41.37728782345830325 ) ) ;
#45035=CARTESIAN_POINT ( 'NONE',  ( 110.9399543235443559, -27.82625392046294266, 134.1724198280769826 ) ) ;
#45036=CARTESIAN_POINT ( 'NONE',  ( 116.8111099997371554, -31.41389126640522989, 24.21181575210196257 ) ) ;
#45037=ORIENTED_EDGE ( 'NONE', *, *, #76850, .T. ) ;
#45040=ORIENTED_EDGE ( 'NONE', *, *, #48793, .T. ) ;
#45042=CYLINDRICAL_SURFACE ( 'NONE', #47543, 9.999999999999998224 ) ;
#45043=ORIENTED_EDGE ( 'NONE', *, *, #60188, .F. ) ;
#45044=CARTESIAN_POINT ( 'NONE',  ( 97.96455956878604354, -32.51352612137473841, 166.9808845455257824 ) ) ;
#45045=CARTESIAN_POINT ( 'NONE',  ( 107.3678158256761179, -26.30747296201684549, 321.5865679059475610 ) ) ;
#45046=FACE_OUTER_BOUND ( 'NONE', #1149, .T. ) ;
#45048=CARTESIAN_POINT ( 'NONE',  ( 63.03715912545733602, -46.82818131006016671, 193.9678068554150911 ) ) ;
#45050=CARTESIAN_POINT ( 'NONE',  ( 96.76314818047262634, -35.13937921927007579, 266.2041967044821149 ) ) ;
#45051=CARTESIAN_POINT ( 'NONE',  ( 114.1199461662357919, -46.31379764262941023, 29.08133956162595268 ) ) ;
#45055=CARTESIAN_POINT ( 'NONE',  ( 106.2252769208846530, -25.30081914710235580, 323.4954383871191794 ) ) ;
#45058=PLANE ( 'NONE',  #75988 ) ;
#45059=ADVANCED_FACE ( 'NONE', ( #16542 ), #69757, .F. ) ;
#45060=AXIS2_PLACEMENT_3D ( 'NONE', #27169, #43017, #77561 ) ;
#45061=CARTESIAN_POINT ( 'NONE',  ( 125.9611475301391721, -14.72944715994100484, 239.5838068554164977 ) ) ;
#45063=CARTESIAN_POINT ( 'NONE',  ( 116.3268456006857718, -32.93825467094161752, 164.1356252759109680 ) ) ;
#45064=LINE ( 'NONE', #85991, #761 ) ;
#45065=CARTESIAN_POINT ( 'NONE',  ( 117.4283214861109457, -38.22576773620406954, 28.71276813305395592 ) ) ;
#45066=CARTESIAN_POINT ( 'NONE',  ( 117.1971262914088499, -34.26925207598063849, 205.0156252759109634 ) ) ;
#45067=CARTESIAN_POINT ( 'NONE',  ( 106.5169537372109545, -25.66675205370546919, 41.12800622829193742 ) ) ;
#45068=CARTESIAN_POINT ( 'NONE',  ( 50.56670390244699576, -18.82844715994031048, -5.074374724088000832 ) ) ;
#45069=DIRECTION ( 'NONE',  ( 0.7071067811864666375, 0.7071067811866283970, 7.071067811864659848E-16 ) ) ;
#45072=CYLINDRICAL_SURFACE ( 'NONE', #41810, 0.9999999999999974465 ) ;
#45073=ORIENTED_EDGE ( 'NONE', *, *, #3845, .F. ) ;
#45074=VECTOR ( 'NONE', #39222, 1000.000000000000000 ) ;
#45075=CARTESIAN_POINT ( 'NONE',  ( 104.0406618471960627, -46.06530165129700549, 78.32705384733895926 ) ) ;
#45076=EDGE_CURVE ( 'NONE', #36080, #38972, #78868, .T. ) ;
#45077=CARTESIAN_POINT ( 'NONE',  ( 162.8913605087219878, -31.76306994223740432, -5.074374724088000832 ) ) ;
#45079=CARTESIAN_POINT ( 'NONE',  ( 134.0664832912740110, -8.729447159940999512, 293.6356252759119911 ) ) ;
#45080=CARTESIAN_POINT ( 'NONE',  ( 99.10268845779070546, -29.98093639561600909, 211.7670538473399517 ) ) ;
#45081=CARTESIAN_POINT ( 'NONE',  ( 180.3503142329310265, -29.99615139349890569, 193.9678068554150059 ) ) ;
#45082=CARTESIAN_POINT ( 'NONE',  ( 110.8554123912721394, -45.98385248439223716, 147.8857061149965375 ) ) ;
#45084=LINE ( 'NONE', #45966, #63175 ) ;
#45085=VECTOR ( 'NONE', #70230, 1000.000000000000000 ) ;
#45086=LINE ( 'NONE', #73240, #57410 ) ;
#45087=DIRECTION ( 'NONE',  ( 0.000000000000000000, 0.000000000000000000, 1.000000000000000000 ) ) ;
#45088=CARTESIAN_POINT ( 'NONE',  ( 104.4066424557107382, -46.45766250888145521, 97.36474845812441004 ) ) ;
#45089=CARTESIAN_POINT ( 'NONE',  ( 96.70615320395830850, -37.17927570127479697, 116.3489586092449599 ) ) ;
#45090=VERTEX_POINT ( 'NONE', #9726 ) ;
#45092=EDGE_LOOP ( 'NONE', ( #10744, #25341, #48173, #74458 ) ) ;
#45093=CARTESIAN_POINT ( 'NONE',  ( 115.4889021248300196, -33.97424487988631370, 85.51015473446898341 ) ) ;
#45095=LINE ( 'NONE', #44199, #86392 ) ;
#45096=CARTESIAN_POINT ( 'NONE',  ( 116.7732407090125690, -35.28285290846963562, 214.9441967044819819 ) ) ;
#45097=DIRECTION ( 'NONE',  ( -0.7071067812163254196, 0.7071067811567697259, -2.899137802742872063E-29 ) ) ;
#45098=CARTESIAN_POINT ( 'NONE',  ( 188.5667039024479834, -62.87844715994099687, 252.3428068554150059 ) ) ;
#45102=CARTESIAN_POINT ( 'NONE',  ( 21.03689327557706790, -23.42844715994186089, 300.4678068554150059 ) ) ;
#45104=CARTESIAN_POINT ( 'NONE',  ( 97.97553865104310944, -30.48296430071270535, 165.8594347997199634 ) ) ;
#45105=EDGE_LOOP ( 'NONE', ( #76802, #63481, #20653, #39534, #69627 ) ) ;
#45106=ORIENTED_EDGE ( 'NONE', *, *, #61227, .F. ) ;
#45107=CIRCLE ( 'NONE', #21934, 3.000000000000002665 ) ;
#45109=CARTESIAN_POINT ( 'NONE',  ( 109.7248659615483319, -27.00080519155043035, 150.8647919392679455 ) ) ;
#45110=CARTESIAN_POINT ( 'NONE',  ( 193.0374249753377001, -23.42844715993435400, 117.4678068554150627 ) ) ;
#45111=CARTESIAN_POINT ( 'NONE',  ( 100.8869784611931379, -44.69984695892584625, 103.0522436344614192 ) ) ;
#45112=AXIS2_PLACEMENT_3D ( 'NONE', #61704, #27198, #54874 ) ;
#45115=CARTESIAN_POINT ( 'NONE',  ( 111.4173512164996254, -47.75262429423162303, 172.8756252759109771 ) ) ;
#45116=CARTESIAN_POINT ( 'NONE',  ( 165.3359832912747720, -36.32844715993532958, 237.4678068554150059 ) ) ;
#45117=ORIENTED_EDGE ( 'NONE', *, *, #61886, .F. ) ;
#45118=VERTEX_POINT ( 'NONE', #45998 ) ;
#45119=ORIENTED_EDGE ( 'NONE', *, *, #84179, .T. ) ;
#45120=AXIS2_PLACEMENT_3D ( 'NONE', #15237, #69751, #56999 ) ;
#45121=CARTESIAN_POINT ( 'NONE',  ( 97.81255050737648560, -40.51953087483806826, 62.63627117197549410 ) ) ;
#45123=CARTESIAN_POINT ( 'NONE',  ( 132.6459363690105135, -34.36767598605985796, 7.908804215159092266 ) ) ;
#45124=VECTOR ( 'NONE', #78609, 1000.000000000000000 ) ;
#45125=CARTESIAN_POINT ( 'NONE',  ( 114.9297498758896126, -40.81563990160193356, 284.8758690201828472 ) ) ;
#45126=DIRECTION ( 'NONE',  ( -0.000000000000000000, -0.000000000000000000, 1.000000000000000000 ) ) ;
#45127=VERTEX_POINT ( 'NONE', #39647 ) ;
#45128=CARTESIAN_POINT ( 'NONE',  ( 116.3768930211383150, -39.34642689581756514, 9.635625275910943088 ) ) ;
#45129=CARTESIAN_POINT ( 'NONE',  ( 82.11134023506700430, -16.88977106732933819, 7.516154048596654036 ) ) ;
#45131=ORIENTED_EDGE ( 'NONE', *, *, #20771, .F. ) ;
#45134=VERTEX_POINT ( 'NONE', #60532 ) ;
#45135=ORIENTED_EDGE ( 'NONE', *, *, #5457, .F. ) ;
#45137=CARTESIAN_POINT ( 'NONE',  ( 112.8214380862813755, -44.54936551000075440, 32.50384839950498872 ) ) ;
#45138=CARTESIAN_POINT ( 'NONE',  ( 96.83676235526975518, -34.60832162431106696, 216.1641967044819808 ) ) ;
#45140=CARTESIAN_POINT ( 'NONE',  ( 117.1424269838423839, -34.14023410701941685, 124.0270538473399426 ) ) ;
#45142=CARTESIAN_POINT ( 'NONE',  ( 108.0140931804088211, -24.91688388787635589, 261.0127681330534415 ) ) ;
#45143=DIRECTION ( 'NONE',  ( -6.524622321627019585E-16, -4.013151879589939944E-16, -1.000000000000000000 ) ) ;
#45145=EDGE_CURVE ( 'NONE', #394, #31817, #84303, .T. ) ;
#45146=ORIENTED_EDGE ( 'NONE', *, *, #9911, .F. ) ;
#45148=ORIENTED_EDGE ( 'NONE', *, *, #26899, .F. ) ;
#45149=VECTOR ( 'NONE', #41811, 1000.000000000000000 ) ;
#45151=CARTESIAN_POINT ( 'NONE',  ( 117.3784280654263341, -34.92100556036569259, 243.9641967044819637 ) ) ;
#45152=ORIENTED_EDGE ( 'NONE', *, *, #59743, .T. ) ;
#45153=CARTESIAN_POINT ( 'NONE',  ( 114.5276809309653459, -28.57754439525472989, 154.4746728949589851 ) ) ;
#45156=ADVANCED_FACE ( 'NONE', ( #12867 ), #33294, .T. ) ;
#45157=DIRECTION ( 'NONE',  ( 0.000000000000000000, 0.000000000000000000, -1.000000000000000000 ) ) ;
#45159=CARTESIAN_POINT ( 'NONE',  ( 21.03689327557619748, -23.42844715994197813, 129.9678068554150627 ) ) ;
#45160=CARTESIAN_POINT ( 'NONE',  ( 49.21437657594998427, -35.91149509761070391, 237.4678068554150059 ) ) ;
#45161=CARTESIAN_POINT ( 'NONE',  ( 97.00695478131298444, -39.24785563725447446, 12.53372051400597442 ) ) ;
#45162=CARTESIAN_POINT ( 'NONE',  ( 188.5667039024479834, -65.37844715994100397, 257.2178068554150059 ) ) ;
#45163=FACE_OUTER_BOUND ( 'NONE', #79858, .T. ) ;
#45166=PLANE ( 'NONE',  #5340 ) ;
#45168=CARTESIAN_POINT ( 'NONE',  ( 97.06107109496848295, -37.99641194480408757, 77.42729194108127899 ) ) ;
#45170=CARTESIAN_POINT ( 'NONE',  ( 100.5161095773857198, -41.59610960965854787, 195.5838068554171514 ) ) ;
#45172=CARTESIAN_POINT ( 'NONE',  ( 136.7282109818895037, -19.44060378568062220, 6.877169033943577148 ) ) ;
#45173=CARTESIAN_POINT ( 'NONE',  ( 101.9737040637596124, -45.89197751792076474, 187.1727681330539781 ) ) ;
#45174=CARTESIAN_POINT ( 'NONE',  ( 100.9432064590905469, -28.29215089373294489, 71.57562527591099411 ) ) ;
#45175=CARTESIAN_POINT ( 'NONE',  ( 118.8391071721064662, -38.46623720595516005, 219.7099109901969882 ) ) ;
#45176=DIRECTION ( 'NONE',  ( 4.299999999999999979E-14, -1.000000000000000000, 0.000000000000000000 ) ) ;
#45178=DIRECTION ( 'NONE',  ( -4.299999999999999979E-14, 1.000000000000000000, -4.400000000000000367E-29 ) ) ;
#45179=CARTESIAN_POINT ( 'NONE',  ( 116.6494290552723356, -33.84902491101575350, 40.05854322555403968 ) ) ;
#45180=CARTESIAN_POINT ( 'NONE',  ( 41.56648329127399677, 0.2215528400590013880, 318.9256252759120116 ) ) ;
#45181=FACE_OUTER_BOUND ( 'NONE', #20232, .T. ) ;
#45183=CARTESIAN_POINT ( 'NONE',  ( 97.60796143750529552, -39.98263668746941590, 66.59062261628206159 ) ) ;
#45187=CARTESIAN_POINT ( 'NONE',  ( 98.02882863141191194, -40.27788709084830998, 96.04670554236294322 ) ) ;
#45188=EDGE_CURVE ( 'NONE', #31084, #44882, #44071, .T. ) ;
#45189=CARTESIAN_POINT ( 'NONE',  ( 107.0664832912739968, -36.72944715994100306, 293.2242906452868851 ) ) ;
#45190=ORIENTED_EDGE ( 'NONE', *, *, #45961, .F. ) ;
#45191=CARTESIAN_POINT ( 'NONE',  ( 108.5348814579965904, -26.43029805172858460, 100.9641967044829727 ) ) ;
#45196=CARTESIAN_POINT ( 'NONE',  ( 77.31651901074916111, -18.55810522839905019, 6.749822759741312517 ) ) ;
#45197=CARTESIAN_POINT ( 'NONE',  ( 32.24491389930067697, -32.11662333284641591, 237.4678068554150059 ) ) ;
#45199=CARTESIAN_POINT ( 'NONE',  ( 111.1466539572802787, -45.61852150023370456, 27.91848241876893155 ) ) ;
#45200=ORIENTED_EDGE ( 'NONE', *, *, #80174, .T. ) ;
#45201=ORIENTED_EDGE ( 'NONE', *, *, #54042, .F. ) ;
#45203=DIRECTION ( 'NONE',  ( 0.7071067811865449082, 0.7071067811865501263, 7.071067811865448709E-16 ) ) ;
#45204=FACE_OUTER_BOUND ( 'NONE', #6732, .T. ) ;
#45206=CARTESIAN_POINT ( 'NONE',  ( 46.83715912545339677, -47.82818131006086304, 180.4678068554150911 ) ) ;
#45207=DIRECTION ( 'NONE',  ( 0.000000000000000000, 0.000000000000000000, 1.000000000000000000 ) ) ;
#45210=AXIS2_PLACEMENT_3D ( 'NONE', #68888, #7114, #82093 ) ;
#45212=CARTESIAN_POINT ( 'NONE',  ( 113.4461594614341777, -46.68675298423774223, 68.02991099019695298 ) ) ;
#45213=VERTEX_POINT ( 'NONE', #70969 ) ;
#45214=ORIENTED_EDGE ( 'NONE', *, *, #16864, .T. ) ;
#45218=CARTESIAN_POINT ( 'NONE',  ( 41.56648329127398966, -27.82844715994070484, 318.9256252759120116 ) ) ;
#45219=CARTESIAN_POINT ( 'NONE',  ( 100.0993174663912697, -32.47640984694866262, 168.7080903695919858 ) ) ;
#45220=CIRCLE ( 'NONE', #6083, 2.029999999999997140 ) ;
#45222=ORIENTED_EDGE ( 'NONE', *, *, #88611, .F. ) ;
#45224=FACE_OUTER_BOUND ( 'NONE', #61423, .T. ) ;
#45225=ORIENTED_EDGE ( 'NONE', *, *, #27471, .T. ) ;
#45227=EDGE_LOOP ( 'NONE', ( #7706, #25611, #85824, #38667 ) ) ;
#45229=CARTESIAN_POINT ( 'NONE',  ( 103.3408556358882890, -28.68905057859731755, 176.8530118773259687 ) ) ;
#45230=DIRECTION ( 'NONE',  ( 0.000000000000000000, 0.000000000000000000, 1.000000000000000000 ) ) ;
#45231=DIRECTION ( 'NONE',  ( 0.000000000000000000, 0.000000000000000000, 1.000000000000000000 ) ) ;
#45232=VECTOR ( 'NONE', #47185, 1000.000000000000000 ) ;
#45233=CARTESIAN_POINT ( 'NONE',  ( 111.0245712168574528, -45.91317361515658035, 17.90029448042019666 ) ) ;
#45235=VECTOR ( 'NONE', #31633, 1000.000000000000000 ) ;
#45236=ADVANCED_FACE ( 'NONE', ( #554 ), #77319, .T. ) ;
#45237=EDGE_LOOP ( 'NONE', ( #14529, #26654, #33019, #67105 ) ) ;
#45238=ORIENTED_EDGE ( 'NONE', *, *, #52535, .F. ) ;
#45240=AXIS2_PLACEMENT_3D ( 'NONE', #29436, #36702, #69873 ) ;
#45241=CARTESIAN_POINT ( 'NONE',  ( 112.3000890867684234, -42.99355894011079471, 190.9480903695919665 ) ) ;
#45243=CARTESIAN_POINT ( 'NONE',  ( 98.84041870859987000, -43.22715631800404879, 91.85848241876892928 ) ) ;
#45244=CARTESIAN_POINT ( 'NONE',  ( 112.7298150101557894, -27.26422151970076158, 54.65943479971996055 ) ) ;
#45248=CARTESIAN_POINT ( 'NONE',  ( 102.0818258798731506, -27.57325825325154867, 141.4727681330539895 ) ) ;
#45249=VECTOR ( 'NONE', #37821, 1000.000000000000000 ) ;
#45250=FACE_OUTER_BOUND ( 'NONE', #40572, .T. ) ;
#45251=ORIENTED_EDGE ( 'NONE', *, *, #10248, .T. ) ;
#45252=DIRECTION ( 'NONE',  ( -6.831565154159360295E-14, 1.000000000000000000, 0.000000000000000000 ) ) ;
#45253=EDGE_CURVE ( 'NONE', #43903, #47547, #175, .T. ) ;
#45255=ADVANCED_FACE ( 'NONE', ( #70509 ), #5276, .F. ) ;
#45257=CARTESIAN_POINT ( 'NONE',  ( 164.9190312289453004, -35.91149509760637670, 313.9678068554149490 ) ) ;
#45258=VERTEX_POINT ( 'NONE', #30101 ) ;
#45259=EDGE_LOOP ( 'NONE', ( #46274, #67176, #28951, #52903, #44444 ) ) ;
#45262=DIRECTION ( 'NONE',  ( 0.000000000000000000, 0.000000000000000000, 1.000000000000000000 ) ) ;
#45263=VERTEX_POINT ( 'NONE', #71453 ) ;
#45264=CARTESIAN_POINT ( 'NONE',  ( 80.06648329127402519, -46.72944715994105991, 10.42562527591094401 ) ) ;
#45265=CARTESIAN_POINT ( 'NONE',  ( 115.5739025235967716, -42.75529552070533867, 53.33562527591095659 ) ) ;
#45268=DIRECTION ( 'NONE',  ( 0.000000000000000000, 0.000000000000000000, -1.000000000000000000 ) ) ;
#45270=CARTESIAN_POINT ( 'NONE',  ( 97.83387747045368599, -32.00739517038274329, 95.96229194257799122 ) ) ;
#45271=CARTESIAN_POINT ( 'NONE',  ( 108.1794352217186201, -47.07304438381563472, 198.6613395616249989 ) ) ;
#45276=CARTESIAN_POINT ( 'NONE',  ( 131.0667039024480118, -58.72944715994098175, 231.5838068554150198 ) ) ;
#45277=CARTESIAN_POINT ( 'NONE',  ( 163.1543517358360020, -31.62489322948790971, -5.074374724088000832 ) ) ;
#45278=EDGE_CURVE ( 'NONE', #65138, #85910, #30590, .T. ) ;
#45279=CYLINDRICAL_SURFACE ( 'NONE', #88360, 4.875000000000017764 ) ;
#45280=CARTESIAN_POINT ( 'NONE',  ( 95.35850850670631473, -38.86301786728916596, 201.4699109901969791 ) ) ;
#45282=CARTESIAN_POINT ( 'NONE',  ( 97.31311150169676694, -38.96077725005761749, 146.5054517158104375 ) ) ;
#45283=CARTESIAN_POINT ( 'NONE',  ( 109.9662181263222891, -48.24525319228295217, 238.7727681330539724 ) ) ;
#45284=CARTESIAN_POINT ( 'NONE',  ( 97.57754503199339524, -30.97118795507763167, 121.8803871806729546 ) ) ;
#45285=CARTESIAN_POINT ( 'NONE',  ( 112.1432778728667614, -28.01507690458955935, 250.6602456620354360 ) ) ;
#45286=VECTOR ( 'NONE', #35701, 1000.000000000000000 ) ;
#45287=CARTESIAN_POINT ( 'NONE',  ( 82.78958961022135554, -37.11755991740238159, 6.789748280179635387 ) ) ;
#45288=DIRECTION ( 'NONE',  ( 1.000000000000000000, 4.299999999999999979E-14, 1.000000000000000078E-15 ) ) ;
#45289=CARTESIAN_POINT ( 'NONE',  ( 109.6423641557757378, -46.48024981121521648, 263.7815675321390358 ) ) ;
#45290=ORIENTED_EDGE ( 'NONE', *, *, #52638, .F. ) ;
#45291=CIRCLE ( 'NONE', #55455, 2.517500000000005844 ) ;
#45294=ORIENTED_EDGE ( 'NONE', *, *, #39219, .T. ) ;
#45295=CARTESIAN_POINT ( 'NONE',  ( 109.6430121181781630, -46.48008673860459083, 72.78145860822925783 ) ) ;
#45296=CARTESIAN_POINT ( 'NONE',  ( 100.1775528843425178, -45.37332466565996469, 268.0289586092443415 ) ) ;
#45298=CARTESIAN_POINT ( 'NONE',  ( 132.9233478419689334, -34.22821065591859480, 1.829869330583430154 ) ) ;
#45300=EDGE_CURVE ( 'NONE', #26394, #19093, #36437, .T. ) ;
#45303=EDGE_CURVE ( 'NONE', #79111, #51120, #16924, .T. ) ;
#45304=CARTESIAN_POINT ( 'NONE',  ( 109.8786884439187759, -28.66423582349726118, 209.2324198280769849 ) ) ;
#45306=ORIENTED_EDGE ( 'NONE', *, *, #54784, .F. ) ;
#45307=ORIENTED_EDGE ( 'NONE', *, *, #37294, .T. ) ;
#45308=CIRCLE ( 'NONE', #68547, 0.5000000000000016653 ) ;
#45309=FACE_BOUND ( 'NONE', #78453, .T. ) ;
#45310=CARTESIAN_POINT ( 'NONE',  ( 97.81847205893258490, -40.53396210923573051, 181.6370475531321915 ) ) ;
#45312=CARTESIAN_POINT ( 'NONE',  ( 105.0114852080080254, -45.89751720821543302, 23.82063092494396273 ) ) ;
#45315=DIRECTION ( 'NONE',  ( -1.000000000000000078E-15, 1.000000000000000083E-30, 1.000000000000000000 ) ) ;
#45316=CARTESIAN_POINT ( 'NONE',  ( 107.0664832912739541, -36.72944715994095333, 307.1356252759109680 ) ) ;
#45317=VERTEX_POINT ( 'NONE', #71003 ) ;
#45318=LINE ( 'NONE', #60293, #85454 ) ;
#45319=ORIENTED_EDGE ( 'NONE', *, *, #51306, .F. ) ;
#45321=CARTESIAN_POINT ( 'NONE',  ( 103.0685998583681311, -29.61280089403793525, 58.30237608387695047 ) ) ;
#45322=CARTESIAN_POINT ( 'NONE',  ( 136.4140944162825804, -17.29397280667294012, 7.245803660783974642 ) ) ;
#45323=FACE_OUTER_BOUND ( 'NONE', #81044, .T. ) ;
#45326=CARTESIAN_POINT ( 'NONE',  ( 51.56670390244683944, -33.35206098992766499, 117.4678068554150485 ) ) ;
#45328=CIRCLE ( 'NONE', #85966, 1.000000000000000888 ) ;
#45329=ORIENTED_EDGE ( 'NONE', *, *, #5463, .F. ) ;
#45330=CARTESIAN_POINT ( 'NONE',  ( 103.3623838164489541, -47.14379949381606849, 102.3165776568629752 ) ) ;
#45331=VERTEX_POINT ( 'NONE', #36477 ) ;
#45332=CARTESIAN_POINT ( 'NONE',  ( 99.45175552060571533, -32.86007347668476086, 50.37527697093396739 ) ) ;
#45333=DIRECTION ( 'NONE',  ( 0.7071067811868672059, 0.7071067811862279395, 6.612322855857878503E-17 ) ) ;
#45334=CARTESIAN_POINT ( 'NONE',  ( 113.9863769398668296, -43.08488557356476889, 74.65491663922996679 ) ) ;
#45339=CARTESIAN_POINT ( 'NONE',  ( 118.2318068709390815, -40.77392476355825579, 19.54991099019698453 ) ) ;
#45340=DIRECTION ( 'NONE',  ( -1.000000000000000000, -1.000000000000000078E-15, -1.000000000000000078E-15 ) ) ;
#45341=ORIENTED_EDGE ( 'NONE', *, *, #18820, .T. ) ;
#45342=AXIS2_PLACEMENT_3D ( 'NONE', #11402, #54043, #74522 ) ;
#45343=CARTESIAN_POINT ( 'NONE',  ( 31.78666935232998725, -36.02818131005891189, -5.074374724088000832 ) ) ;
#45344=ORIENTED_EDGE ( 'NONE', *, *, #85850, .F. ) ;
#45349=EDGE_CURVE ( 'NONE', #10055, #69050, #8888, .T. ) ;
#45353=CARTESIAN_POINT ( 'NONE',  ( 96.86352172870815025, -32.31225822881502552, 211.0013395616259686 ) ) ;
#45354=CARTESIAN_POINT ( 'NONE',  ( 138.8167039024479834, -50.82844715994100682, 86.31780685541500020 ) ) ;
#45356=CARTESIAN_POINT ( 'NONE',  ( 96.92116189526866776, -32.34237133930066221, 57.01372051400599616 ) ) ;
#45357=CARTESIAN_POINT ( 'NONE',  ( 97.82506921874286832, -40.54997709253600391, 42.63842632371162722 ) ) ;
#45358=ORIENTED_EDGE ( 'NONE', *, *, #26500, .F. ) ;
#45359=CARTESIAN_POINT ( 'NONE',  ( 103.2775475522615665, -27.47504464129099233, 171.3857084645095767 ) ) ;
#45360=EDGE_CURVE ( 'NONE', #63964, #61092, #42809, .T. ) ;
#45366=CARTESIAN_POINT ( 'NONE',  ( 104.4067455066945200, -46.45769128758091426, 113.3653941873491391 ) ) ;
#45367=CARTESIAN_POINT ( 'NONE',  ( 116.5858064714421829, -40.92601143571970823, 253.4956252759109532 ) ) ;
#45370=CARTESIAN_POINT ( 'NONE',  ( 188.5667039024479834, -62.87844715994099687, 170.4678068554149775 ) ) ;
#45371=EDGE_CURVE ( 'NONE', #11705, #65895, #26238, .T. ) ;
#45372=CARTESIAN_POINT ( 'NONE',  ( 100.7827017321902758, -30.20819270671951173, 265.0971817328389761 ) ) ;
#45375=CARTESIAN_POINT ( 'NONE',  ( 117.4257108620837329, -37.68603989742253191, 74.75276813305397638 ) ) ;
#45377=CARTESIAN_POINT ( 'NONE',  ( 117.2652295300992193, -42.86250289712283745, 128.3956252759109873 ) ) ;
#45385=ADVANCED_FACE ( 'NONE', ( #5072 ), #65943, .F. ) ;
#45387=CARTESIAN_POINT ( 'NONE',  ( 103.2628093650484828, -47.15753175352042348, 97.28610146638693834 ) ) ;
#45388=VERTEX_POINT ( 'NONE', #25971 ) ;
#45389=FACE_OUTER_BOUND ( 'NONE', #49291, .T. ) ;
#45390=CYLINDRICAL_SURFACE ( 'NONE', #5539, 0.9999999999991942001 ) ;
#45391=CARTESIAN_POINT ( 'NONE',  ( 81.80795390244800558, -42.97311385574014508, 231.5838068554169524 ) ) ;
#45393=CARTESIAN_POINT ( 'NONE',  ( 113.0897370140187235, -28.19324317000061697, 129.5870538473399449 ) ) ;
#45396=CARTESIAN_POINT ( 'NONE',  ( 149.4532656544377289, -72.54365454176046057, 543.8623766218582887 ) ) ;
#45397=DIRECTION ( 'NONE',  ( -1.000000000000000000, 0.000000000000000000, 0.000000000000000000 ) ) ;
#45398=ORIENTED_EDGE ( 'NONE', *, *, #25806, .F. ) ;
#45399=AXIS2_PLACEMENT_3D ( 'NONE', #86563, #66089, #29364 ) ;
#45401=DIRECTION ( 'NONE',  ( 1.000000000000000078E-15, -1.000000000000000083E-30, -1.000000000000000000 ) ) ;
#45404=FACE_OUTER_BOUND ( 'NONE', #33508, .T. ) ;
#45405=LINE ( 'NONE', #37278, #3586 ) ;
#45408=AXIS2_PLACEMENT_3D ( 'NONE', #21549, #89245, #49221 ) ;
#45410=DIRECTION ( 'NONE',  ( -0.7071067811578587436, 0.7071067812152364018, 0.000000000000000000 ) ) ;
#45411=CARTESIAN_POINT ( 'NONE',  ( 104.6152064257953640, -27.26083179018629465, 196.2784824187679362 ) ) ;
#45412=DIRECTION ( 'NONE',  ( 0.9068632946707805287, -0.4214249218767882610, 9.061988307341536250E-16 ) ) ;
#45414=CARTESIAN_POINT ( 'NONE',  ( 97.55373691267115532, -39.00345059616618215, 52.51276813305294411 ) ) ;
#45415=FACE_OUTER_BOUND ( 'NONE', #25455, .T. ) ;
#45416=DIRECTION ( 'NONE',  ( 0.000000000000000000, 1.000000000000000000, 0.000000000000000000 ) ) ;
#45417=CARTESIAN_POINT ( 'NONE',  ( 182.5667039024480118, -32.29483332968450782, -5.074374724088000832 ) ) ;
#45419=ADVANCED_FACE ( 'NONE', ( #25067, #60468 ), #66849, .F. ) ;
#45423=CARTESIAN_POINT ( 'NONE',  ( 112.6928898907800090, -44.25407833457246909, 184.5311071154209799 ) ) ;
#45425=EDGE_CURVE ( 'NONE', #43762, #223, #17365, .T. ) ;
#45426=CARTESIAN_POINT ( 'NONE',  ( 116.3176178399231873, -32.93748434060082531, 55.13562527591098217 ) ) ;
#45429=CYLINDRICAL_SURFACE ( 'NONE', #88165, 2.517500000000000071 ) ;
#45430=CARTESIAN_POINT ( 'NONE',  ( 188.5667039024479834, -67.87844715994100397, 288.3428068554150059 ) ) ;
#45432=CYLINDRICAL_SURFACE ( 'NONE', #5830, 3.300000000000000711 ) ;
#45433=CARTESIAN_POINT ( 'NONE',  ( 104.4836364144456979, -26.98054529041288419, 36.28151591486695793 ) ) ;
#45434=ORIENTED_EDGE ( 'NONE', *, *, #77160, .F. ) ;
#45435=CARTESIAN_POINT ( 'NONE',  ( 100.0388059118472341, -29.01104360887432776, 285.6641967044823787 ) ) ;
#45439=DIRECTION ( 'NONE',  ( -1.000000000000000078E-15, 1.000000000000000083E-30, 1.000000000000000000 ) ) ;
#45442=CARTESIAN_POINT ( 'NONE',  ( 117.9939971868874125, -34.78344139941312108, 194.9546728949589749 ) ) ;
#45444=ORIENTED_EDGE ( 'NONE', *, *, #78228, .T. ) ;
#45445=CARTESIAN_POINT ( 'NONE',  ( 96.87875409107806490, -32.32403320637130406, 57.01372051400599616 ) ) ;
#45448=ORIENTED_EDGE ( 'NONE', *, *, #20090, .T. ) ;
#45449=EDGE_CURVE ( 'NONE', #36567, #23413, #4182, .T. ) ;
#45450=EDGE_CURVE ( 'NONE', #74767, #44052, #5964, .T. ) ;
#45452=AXIS2_PLACEMENT_3D ( 'NONE', #75498, #75940, #20088 ) ;
#45454=CARTESIAN_POINT ( 'NONE',  ( 82.45999417310882507, -17.37149686611859423, 2.653088969735680536 ) ) ;
#45457=CARTESIAN_POINT ( 'NONE',  ( 115.3203086601475320, -34.12650808536288594, 126.8757094172099613 ) ) ;
#45458=CARTESIAN_POINT ( 'NONE',  ( 117.4960079497888472, -36.12755493457860467, 224.8727681330539667 ) ) ;
#45459=LINE ( 'NONE', #25042, #2939 ) ;
#45463=VERTEX_POINT ( 'NONE', #52289 ) ;
#45464=ORIENTED_EDGE ( 'NONE', *, *, #64868, .F. ) ;
#45465=VECTOR ( 'NONE', #42891, 1000.000000000000000 ) ;
#45469=CARTESIAN_POINT ( 'NONE',  ( 116.7802871385218282, -39.10473973501323286, 9.635625275910941312 ) ) ;
#45471=CARTESIAN_POINT ( 'NONE',  ( 90.44969454456405344, -22.62993780205715311, 239.5838068554169809 ) ) ;
#45472=ADVANCED_FACE ( 'NONE', ( #73661 ), #80052, .F. ) ;
#45473=CARTESIAN_POINT ( 'NONE',  ( 113.1668408875787435, -30.74627054922163438, 148.8667055423629790 ) ) ;
#45474=CARTESIAN_POINT ( 'NONE',  ( 116.7680724212777079, -31.33574231247038355, 29.24229194257799236 ) ) ;
#45476=FACE_OUTER_BOUND ( 'NONE', #8840, .T. ) ;
#45477=ORIENTED_EDGE ( 'NONE', *, *, #49334, .T. ) ;
#45479=ORIENTED_EDGE ( 'NONE', *, *, #52968, .F. ) ;
#45480=CARTESIAN_POINT ( 'NONE',  ( 141.8664832912729992, -71.52944715994142655, 342.9256252759109884 ) ) ;
#45482=CARTESIAN_POINT ( 'NONE',  ( 97.81219346325542574, -40.51865836701575319, 131.6357308845718421 ) ) ;
#45483=VECTOR ( 'NONE', #73781, 1000.000000000000114 ) ;
#45484=CARTESIAN_POINT ( 'NONE',  ( 164.9667039024473922, -26.71338133338732845, 313.9678068554149490 ) ) ;
#45486=CARTESIAN_POINT ( 'NONE',  ( 115.4624701790509391, -43.00605189524043936, 28.31562527591097123 ) ) ;
#45487=CARTESIAN_POINT ( 'NONE',  ( 106.6049252239556608, -25.63961115983148176, 36.09753003781596448 ) ) ;
#45488=VECTOR ( 'NONE', #15013, 1000.000000000000000 ) ;
#45494=LINE ( 'NONE', #10997, #77971 ) ;
#45496=CARTESIAN_POINT ( 'NONE',  ( 102.3692588328596571, -47.63350050119395007, 287.2527681330535643 ) ) ;
#45497=CARTESIAN_POINT ( 'NONE',  ( 107.6544996609965352, -47.76702919738148267, 193.6308633711489620 ) ) ;
#45498=CARTESIAN_POINT ( 'NONE',  ( 97.33132060198839497, -32.84282867815538509, 37.02419670448292521 ) ) ;
#45500=CARTESIAN_POINT ( 'NONE',  ( 20.03715912545820288, -46.82818131006190043, 300.4678068554150059 ) ) ;
#45502=PLANE ( 'NONE',  #56632 ) ;
#45503=AXIS2_PLACEMENT_3D ( 'NONE', #57179, #84481, #72173 ) ;
#45504=VECTOR ( 'NONE', #28963, 1000.000000000000000 ) ;
#45505=EDGE_CURVE ( 'NONE', #51700, #45388, #38686, .T. ) ;
#45506=CIRCLE ( 'NONE', #6376, 2.116999999999980009 ) ;
#45507=ORIENTED_EDGE ( 'NONE', *, *, #25161, .T. ) ;
#45509=VERTEX_POINT ( 'NONE', #30987 ) ;
#45510=CARTESIAN_POINT ( 'NONE',  ( 107.2219638487720488, -26.36052190073626988, 76.07657765686298035 ) ) ;
#45511=DIRECTION ( 'NONE',  ( 1.000000000000000000, 4.299999999999999979E-14, 1.000000000000000078E-15 ) ) ;
#45512=ORIENTED_EDGE ( 'NONE', *, *, #3195, .F. ) ;
#45513=VECTOR ( 'NONE', #70544, 1000.000000000000000 ) ;
#45515=CARTESIAN_POINT ( 'NONE',  ( 117.3134009501234658, -34.93240959161192905, 239.9641967044819637 ) ) ;
#45516=DIRECTION ( 'NONE',  ( -4.237773401492740281E-14, 1.000000000000000000, 0.000000000000000000 ) ) ;
#45517=FACE_OUTER_BOUND ( 'NONE', #45714, .T. ) ;
#45518=CARTESIAN_POINT ( 'NONE',  ( 165.2748236753147353, -30.08671355699731009, 193.9678068554149775 ) ) ;
#45519=DIRECTION ( 'NONE',  ( 0.9068632946707807507, -0.4214249218767880945, 9.080193194566099635E-16 ) ) ;
#45520=CARTESIAN_POINT ( 'NONE',  ( 133.1862368104815175, -39.33528726900525641, 1.744847506583675045 ) ) ;
#45522=CARTESIAN_POINT ( 'NONE',  ( 96.28008679191512442, -39.42493101749853679, 166.5213395616259788 ) ) ;
#45523=ORIENTED_EDGE ( 'NONE', *, *, #43139, .F. ) ;
#45525=CARTESIAN_POINT ( 'NONE',  ( 112.8380968919016425, -43.45378765227984275, 104.5730118773259534 ) ) ;
#45527=CARTESIAN_POINT ( 'NONE',  ( 63.03715912545732181, -24.89890238295017966, 300.4678068554150627 ) ) ;
#45528=CARTESIAN_POINT ( 'NONE',  ( 106.8648936900573148, -47.09757847023101363, 223.5489586092439538 ) ) ;
#45529=FACE_OUTER_BOUND ( 'NONE', #83178, .T. ) ;
#45530=FACE_BOUND ( 'NONE', #3217, .T. ) ;
#45534=CARTESIAN_POINT ( 'NONE',  ( 80.06648329127399677, -18.72944715994105991, -5.074374724089057764 ) ) ;
#45535=CARTESIAN_POINT ( 'NONE',  ( 87.06648329127402519, -56.72944715994104570, 14.67562527591094934 ) ) ;
#45536=CARTESIAN_POINT ( 'NONE',  ( 116.9962961068553966, -33.62662860631126449, 174.0670538473389399 ) ) ;
#45537=ORIENTED_EDGE ( 'NONE', *, *, #48325, .T. ) ;
#45540=CARTESIAN_POINT ( 'NONE',  ( 116.3212776292296127, -32.94146857471318413, 287.6356252759109680 ) ) ;
#45541=CARTESIAN_POINT ( 'NONE',  ( 25.56670390244797275, -62.87844715994099687, 168.3428068554150059 ) ) ;
#45542=CARTESIAN_POINT ( 'NONE',  ( 71.06648329127399677, -18.82844715994099971, 284.9256252759119548 ) ) ;
#45543=AXIS2_PLACEMENT_3D ( 'NONE', #35251, #77500, #21654 ) ;
#45544=CARTESIAN_POINT ( 'NONE',  ( 125.8897075496517317, -55.55267141831851774, 14.67562527591099020 ) ) ;
#45545=CARTESIAN_POINT ( 'NONE',  ( 103.0496837167155491, -26.43166057102584077, 170.3603871806729444 ) ) ;
#45546=CARTESIAN_POINT ( 'NONE',  ( 136.1031364520942475, -38.57950990141236502, 7.523361336355876006 ) ) ;
#45549=ORIENTED_EDGE ( 'NONE', *, *, #19963, .F. ) ;
#45550=VERTEX_POINT ( 'NONE', #60930 ) ;
#45551=EDGE_CURVE ( 'NONE', #59341, #25045, #39396, .T. ) ;
#45553=DIRECTION ( 'NONE',  ( -0.000000000000000000, -0.000000000000000000, 1.000000000000000000 ) ) ;
#45555=CARTESIAN_POINT ( 'NONE',  ( 101.9933011300245340, -45.44587426433803046, 163.1564290691892722 ) ) ;
#45556=CARTESIAN_POINT ( 'NONE',  ( 113.8488019003066825, -42.10541956792432217, 46.12332846482897253 ) ) ;
#45557=CARTESIAN_POINT ( 'NONE',  ( 97.81168895331838087, -40.51742574516882200, 287.6356252759109680 ) ) ;
#45558=VERTEX_POINT ( 'NONE', #76358 ) ;
#45559=EDGE_CURVE ( 'NONE', #35754, #22170, #54979, .T. ) ;
#45561=FACE_OUTER_BOUND ( 'NONE', #85712, .T. ) ;
#45564=VECTOR ( 'NONE', #89564, 1000.000000000000000 ) ;
#45565=CARTESIAN_POINT ( 'NONE',  ( 37.03715912545343514, -48.62818131006119415, 180.4678068554150911 ) ) ;
#45567=EDGE_LOOP ( 'NONE', ( #4594, #66575, #53825, #25419 ) ) ;
#45572=CARTESIAN_POINT ( 'NONE',  ( 104.7514827670518684, -44.95118086569023319, 21.78099125664900626 ) ) ;
#45573=CIRCLE ( 'NONE', #6446, 4.874999999999990230 ) ;
#45574=CARTESIAN_POINT ( 'NONE',  ( 110.7040309646834970, -48.03441345040916843, 207.8241967044819489 ) ) ;
#45575=CARTESIAN_POINT ( 'NONE',  ( 99.30484619187383544, -29.80227926343058797, 190.7470538473399415 ) ) ;
#45577=DIRECTION ( 'NONE',  ( 0.04216478779797398074, -0.9991106698809455455, 0.000000000000000000 ) ) ;
#45578=CARTESIAN_POINT ( 'NONE',  ( 97.22385571422852024, -40.27120027895552568, 262.6013395616254797 ) ) ;
#45579=DIRECTION ( 'NONE',  ( 1.000000000000000000, 4.299999999999999979E-14, 1.000000000000000078E-15 ) ) ;
#45580=LINE ( 'NONE', #74661, #25029 ) ;
#45584=CARTESIAN_POINT ( 'NONE',  ( 104.3993058286337146, -25.95452033834810024, 240.2575300378159682 ) ) ;
#45585=ORIENTED_EDGE ( 'NONE', *, *, #39739, .T. ) ;
#45586=CARTESIAN_POINT ( 'NONE',  ( 116.3504430951951605, -44.09481043651530996, 198.2927681330539542 ) ) ;
#45587=DIRECTION ( 'NONE',  ( 0.000000000000000000, 0.000000000000000000, -1.000000000000000000 ) ) ;
#45589=DIRECTION ( 'NONE',  ( 1.000000000000000078E-15, 1.000000000000000083E-30, -1.000000000000000000 ) ) ;
#45590=CARTESIAN_POINT ( 'NONE',  ( 184.3595971212628797, -48.62134037874749737, 249.9678068554149775 ) ) ;
#45592=FACE_OUTER_BOUND ( 'NONE', #11593, .T. ) ;
#45593=CARTESIAN_POINT ( 'NONE',  ( 117.8598252335457488, -34.07367295057271406, 10.01848241876795953 ) ) ;
#45595=CARTESIAN_POINT ( 'NONE',  ( 172.5664832912740110, 0.2215528400590013880, 198.9256252759119832 ) ) ;
#45596=LINE ( 'NONE', #33341, #42636 ) ;
#45600=CARTESIAN_POINT ( 'NONE',  ( 101.1610018191305187, -28.81527687121307224, 195.5838068554172366 ) ) ;
#45602=CARTESIAN_POINT ( 'NONE',  ( 135.4471649165409985, -21.11090284777780113, 7.925007058955543471 ) ) ;
#45603=CARTESIAN_POINT ( 'NONE',  ( 117.2137812332333766, -41.17104435167765075, 208.4861014663869696 ) ) ;
#45604=CARTESIAN_POINT ( 'NONE',  ( 116.5333143132291269, -32.36348817604392991, 100.1699109901969535 ) ) ;
#45605=CARTESIAN_POINT ( 'NONE',  ( 106.9399153568602259, -47.82816235210678002, 228.5794347997199907 ) ) ;
#45606=CARTESIAN_POINT ( 'NONE',  ( 50.88849390559370534, -32.11662333284569115, 193.9678068554150911 ) ) ;
#45607=DIRECTION ( 'NONE',  ( 1.000000000000000000, 4.299999999999999979E-14, 1.000000000000000078E-15 ) ) ;
#45609=CARTESIAN_POINT ( 'NONE',  ( 110.6285399601922848, -46.11599178581295888, 38.86459524923592568 ) ) ;
#45610=EDGE_CURVE ( 'NONE', #36943, #82153, #35009, .T. ) ;
#45611=FACE_OUTER_BOUND ( 'NONE', #15265, .T. ) ;
#45614=CARTESIAN_POINT ( 'NONE',  ( 97.80456843721749749, -40.50002885529080743, 66.63459087925632218 ) ) ;
#45616=EDGE_CURVE ( 'NONE', #67284, #29066, #54089, .T. ) ;
#45619=CARTESIAN_POINT ( 'NONE',  ( 115.4827349520354858, -33.38588942772360468, 98.56194363760096167 ) ) ;
#45622=CARTESIAN_POINT ( 'NONE',  ( 104.9672558511366276, -25.09151557957609668, 121.2184824187679766 ) ) ;
#45623=DIRECTION ( 'NONE',  ( -0.04216478779797398074, 0.9991106698809455455, 0.000000000000000000 ) ) ;
#45624=CARTESIAN_POINT ( 'NONE',  ( 77.45242755740714813, -17.85322059724255084, 6.943211687812394395 ) ) ;
#45625=LINE ( 'NONE', #46077, #79566 ) ;
#45627=CARTESIAN_POINT ( 'NONE',  ( 107.5734549334945456, -47.83597508069291138, 42.61276813305398292 ) ) ;
#45629=ORIENTED_EDGE ( 'NONE', *, *, #86607, .T. ) ;
#45631=VECTOR ( 'NONE', #35862, 1000.000000000000000 ) ;
#45632=EDGE_CURVE ( 'NONE', #29419, #83459, #8951, .T. ) ;
#45633=AXIS2_PLACEMENT_3D ( 'NONE', #56242, #15397, #84448 ) ;
#45635=VECTOR ( 'NONE', #75280, 1000.000000000000000 ) ;
#45636=CARTESIAN_POINT ( 'NONE',  ( 116.1942131220465768, -33.21547736372282600, 135.1184824187679396 ) ) ;
#45637=CARTESIAN_POINT ( 'NONE',  ( 57.56670390244744340, -48.82844715994040286, 173.2178068554150911 ) ) ;
#45639=LINE ( 'NONE', #37530, #78284 ) ;
#45641=VECTOR ( 'NONE', #34672, 1000.000000000000000 ) ;
#45646=CARTESIAN_POINT ( 'NONE',  ( 117.4328057974123567, -37.95573561897359838, 53.73276813305394484 ) ) ;
#45647=VERTEX_POINT ( 'NONE', #48178 ) ;
#45653=CARTESIAN_POINT ( 'NONE',  ( 104.5146602464430714, -28.97587216416100375, 163.1480903695919551 ) ) ;
#45654=ADVANCED_FACE ( 'NONE', ( #75011 ), #5988, .F. ) ;
#45657=EDGE_LOOP ( 'NONE', ( #24187, #3037, #14503, #4077 ) ) ;
#45658=EDGE_LOOP ( 'NONE', ( #53693, #60605, #17366, #74259, #20502 ) ) ;
#45660=EDGE_LOOP ( 'NONE', ( #28734, #52369, #54292, #16620, #30191 ) ) ;
#45663=EDGE_CURVE ( 'NONE', #16775, #88540, #19593, .T. ) ;
#45664=CARTESIAN_POINT ( 'NONE',  ( 110.7647657470428157, -46.09926102310604534, 169.3072975916109613 ) ) ;
#45665=DIRECTION ( 'NONE',  ( 0.000000000000000000, 0.000000000000000000, -1.000000000000000000 ) ) ;
#45667=AXIS2_PLACEMENT_3D ( 'NONE', #32073, #31177, #24824 ) ;
#45668=CARTESIAN_POINT ( 'NONE',  ( 116.3212776292269552, -32.94146857470667555, 79.13562527591095375 ) ) ;
#45671=VECTOR ( 'NONE', #50203, 1000.000000000000000 ) ;
#45673=VERTEX_POINT ( 'NONE', #89096 ) ;
#45674=EDGE_CURVE ( 'NONE', #74757, #9163, #35046, .T. ) ;
#45675=CARTESIAN_POINT ( 'NONE',  ( 115.5744916924636954, -35.14366089088881751, 201.8033284648299457 ) ) ;
#45676=CARTESIAN_POINT ( 'NONE',  ( 114.0369391955824483, -28.94747385925965943, 114.4956252759109816 ) ) ;
#45677=CARTESIAN_POINT ( 'NONE',  ( 95.37363933861277587, -34.96150835630652409, 71.20705384733993526 ) ) ;
#45678=ADVANCED_FACE ( 'NONE', ( #6418, #21402 ), #20946, .F. ) ;
#45680=DIRECTION ( 'NONE',  ( 0.000000000000000000, 0.000000000000000000, -1.000000000000000000 ) ) ;
#45681=CARTESIAN_POINT ( 'NONE',  ( 97.38209261381841486, -42.05735084626116560, 172.7146728949589942 ) ) ;
#45682=FACE_OUTER_BOUND ( 'NONE', #71731, .T. ) ;
#45684=ORIENTED_EDGE ( 'NONE', *, *, #63743, .T. ) ;
#45686=ORIENTED_EDGE ( 'NONE', *, *, #51920, .T. ) ;
#45688=CARTESIAN_POINT ( 'NONE',  ( 49.35211078756498893, -35.65087443492551245, -5.074374724088000832 ) ) ;
#45692=CARTESIAN_POINT ( 'NONE',  ( 74.38348329127296665, -71.52944715994141234, 352.4506252759078961 ) ) ;
#45693=ORIENTED_EDGE ( 'NONE', *, *, #16394, .F. ) ;
#45694=AXIS2_PLACEMENT_3D ( 'NONE', #53218, #68682, #47314 ) ;
#45695=AXIS2_PLACEMENT_3D ( 'NONE', #20324, #89819, #20757 ) ;
#45696=PLANE ( 'NONE',  #75424 ) ;
#45697=CARTESIAN_POINT ( 'NONE',  ( 116.1238663722925253, -29.08717671455551468, 74.38419670448293175 ) ) ;
#45699=AXIS2_PLACEMENT_3D ( 'NONE', #64492, #57662, #50850 ) ;
#45700=LINE ( 'NONE', #80274, #88431 ) ;
#45702=CARTESIAN_POINT ( 'NONE',  ( 103.5129713284349720, -46.47169217660404428, 97.28610146638794731 ) ) ;
#45704=CARTESIAN_POINT ( 'NONE',  ( 111.4081670832168953, -47.72935575799004226, 168.8756252759109486 ) ) ;
#45705=CARTESIAN_POINT ( 'NONE',  ( 100.9528829496750717, -28.70842646451748692, 60.59413823283402678 ) ) ;
#45707=ORIENTED_EDGE ( 'NONE', *, *, #56356, .T. ) ;
#45708=DIRECTION ( 'NONE',  ( -1.000000000000000000, -4.554376769437570034E-14, 0.000000000000000000 ) ) ;
#45709=AXIS2_PLACEMENT_3D ( 'NONE', #60708, #67990, #81642 ) ;
#45711=DIRECTION ( 'NONE',  ( 3.062684205862500216E-15, 0.000000000000000000, -1.000000000000000000 ) ) ;
#45712=CYLINDRICAL_SURFACE ( 'NONE', #49152, 2.500000000000002220 ) ;
#45713=CARTESIAN_POINT ( 'NONE',  ( 104.4426401758756100, -26.59425533393106633, 200.2784824187679362 ) ) ;
#45714=EDGE_LOOP ( 'NONE', ( #36511, #7373, #83, #5517 ) ) ;
#45715=CARTESIAN_POINT ( 'NONE',  ( 107.0667039024467329, -54.09444715994091979, 196.2188068554169433 ) ) ;
#45716=CARTESIAN_POINT ( 'NONE',  ( 96.95773401446056994, -39.36581715674629578, 272.5299109901966972 ) ) ;
#45717=CARTESIAN_POINT ( 'NONE',  ( 95.73188602939242742, -40.35408750269280631, 127.5727681330539554 ) ) ;
#45718=DIRECTION ( 'NONE',  ( 1.000000000000000078E-15, -1.000000000000000083E-30, -1.000000000000000000 ) ) ;
#45722=CARTESIAN_POINT ( 'NONE',  ( 108.3328468486845821, -46.73492755383839636, 263.6773967463404915 ) ) ;
#45725=EDGE_CURVE ( 'NONE', #83730, #53830, #27790, .T. ) ;
#45726=ORIENTED_EDGE ( 'NONE', *, *, #7986, .F. ) ;
#45727=ORIENTED_EDGE ( 'NONE', *, *, #83129, .T. ) ;
#45728=ORIENTED_EDGE ( 'NONE', *, *, #45360, .T. ) ;
#45729=DIRECTION ( 'NONE',  ( 0.000000000000000000, 0.000000000000000000, -1.000000000000000000 ) ) ;
#45730=CARTESIAN_POINT ( 'NONE',  ( 108.0140931804088211, -24.91688388787635589, 261.0127681330534415 ) ) ;
#45735=CARTESIAN_POINT ( 'NONE',  ( 104.3272728202184538, -28.09756461201434874, 204.7314674471249702 ) ) ;
#45736=ORIENTED_EDGE ( 'NONE', *, *, #54252, .T. ) ;
#45737=ORIENTED_EDGE ( 'NONE', *, *, #49272, .T. ) ;
#45739=ORIENTED_EDGE ( 'NONE', *, *, #34931, .F. ) ;
#45741=CARTESIAN_POINT ( 'NONE',  ( 142.8682495647594806, 8.654319075478467127, 394.9756252759102040 ) ) ;
#45743=DIRECTION ( 'NONE',  ( 1.639958061481212836E-42, -4.100000000000000342E-29, -1.000000000000000000 ) ) ;
#45744=FACE_OUTER_BOUND ( 'NONE', #59658, .T. ) ;
#45745=EDGE_CURVE ( 'NONE', #55155, #41030, #17623, .T. ) ;
#45746=CARTESIAN_POINT ( 'NONE',  ( 113.6566823882007355, -42.65376606380868196, 34.67586902018199169 ) ) ;
#45748=EDGE_CURVE ( 'NONE', #17890, #47593, #84086, .T. ) ;
#45749=CARTESIAN_POINT ( 'NONE',  ( 164.9667039024459996, -28.27351298637401200, -5.074374724088000832 ) ) ;
#45750=LINE ( 'NONE', #32588, #52945 ) ;
#45752=ORIENTED_EDGE ( 'NONE', *, *, #20696, .F. ) ;
#45753=EDGE_CURVE ( 'NONE', #44014, #18892, #70904, .T. ) ;
#45754=DIRECTION ( 'NONE',  ( 1.000000000000000078E-15, -1.000000000000000083E-30, -1.000000000000000000 ) ) ;
#45757=CARTESIAN_POINT ( 'NONE',  ( 105.7780793485435851, -44.78982812472496988, 35.26809036959094357 ) ) ;
#45758=EDGE_CURVE ( 'NONE', #73852, #37451, #15935, .T. ) ;
#45759=EDGE_CURVE ( 'NONE', #77606, #70760, #2755, .T. ) ;
#45762=CARTESIAN_POINT ( 'NONE',  ( 136.1531896714421634, -16.93816060013640268, 7.482180659736330064 ) ) ;
#45764=ADVANCED_FACE ( 'NONE', ( #42707 ), #16380, .T. ) ;
#45765=CARTESIAN_POINT ( 'NONE',  ( 41.56648329127399677, 0.2215528400590013880, 258.9256252759120116 ) ) ;
#45767=ORIENTED_EDGE ( 'NONE', *, *, #38145, .T. ) ;
#45771=VERTEX_POINT ( 'NONE', #8221 ) ;
#45772=CARTESIAN_POINT ( 'NONE',  ( 109.0723201335305816, -47.59939223872296310, 127.7337205140059382 ) ) ;
#45773=ORIENTED_EDGE ( 'NONE', *, *, #23364, .F. ) ;
#45774=CARTESIAN_POINT ( 'NONE',  ( 104.5191702102720939, -45.41989400652479958, 61.76003887569697781 ) ) ;
#45775=EDGE_CURVE ( 'NONE', #5926, #16504, #44056, .T. ) ;
#45776=CIRCLE ( 'NONE', #89330, 16.00000000000000000 ) ;
#45777=CARTESIAN_POINT ( 'NONE',  ( 116.3212776292294421, -32.94146857471278622, 70.13562527591093954 ) ) ;
#45778=CARTESIAN_POINT ( 'NONE',  ( 99.44206372185087162, -32.21319818083724584, 82.33301187732594428 ) ) ;
#45782=CARTESIAN_POINT ( 'NONE',  ( 100.4654578171049337, -27.83497312075872188, 31.59657765686396758 ) ) ;
#45783=CARTESIAN_POINT ( 'NONE',  ( 89.06648138392552028, -56.72944715994104570, 14.67562527591095289 ) ) ;
#45784=EDGE_LOOP ( 'NONE', ( #39713, #24646, #73065, #68082 ) ) ;
#45785=CARTESIAN_POINT ( 'NONE',  ( 115.7829627233165724, -41.80255438717769323, 258.4063611559658398 ) ) ;
#45788=VERTEX_POINT ( 'NONE', #30454 ) ;
#45790=ORIENTED_EDGE ( 'NONE', *, *, #3572, .T. ) ;
#45793=CARTESIAN_POINT ( 'NONE',  ( 112.7790632652332050, -27.19118669266615740, 204.6470538473399756 ) ) ;
#45794=EDGE_CURVE ( 'NONE', #36736, #33407, #81446, .T. ) ;
#45796=CARTESIAN_POINT ( 'NONE',  ( 141.8664832912729992, -71.52944715994142655, 361.9756252759109998 ) ) ;
#45797=CARTESIAN_POINT ( 'NONE',  ( 115.7285985590555129, -43.59543139906921283, 44.30514908543492680 ) ) ;
#45798=CARTESIAN_POINT ( 'NONE',  ( 109.6426967425594370, -46.48017342192625989, 43.78143288360754326 ) ) ;
#45799=EDGE_CURVE ( 'NONE', #56594, #47280, #77261, .T. ) ;
#45801=CARTESIAN_POINT ( 'NONE',  ( 116.3225472244029817, -32.94146556017791738, 114.1356252759109822 ) ) ;
#45802=EDGE_CURVE ( 'NONE', #10278, #66199, #68390, .T. ) ;
#45803=CARTESIAN_POINT ( 'NONE',  ( 179.4595971212889935, -28.98061976758940617, -5.074374724088000832 ) ) ;
#45806=CARTESIAN_POINT ( 'NONE',  ( 34.96670390244699433, -28.27351298637416122, 193.9678068554150911 ) ) ;
#45807=CARTESIAN_POINT ( 'NONE',  ( 110.8089421659425824, -26.35361831834155311, 249.7889586092445882 ) ) ;
#45808=FACE_OUTER_BOUND ( 'NONE', #68632, .T. ) ;
#45811=CARTESIAN_POINT ( 'NONE',  ( 114.3529501776022244, -31.35170872818512322, 258.7428960185527558 ) ) ;
#45812=DIRECTION ( 'NONE',  ( 1.000000000000000078E-15, -1.000000000000000083E-30, -1.000000000000000000 ) ) ;
#45813=CARTESIAN_POINT ( 'NONE',  ( 98.32466564902617279, -28.76522518762223157, 76.73848241876795839 ) ) ;
#45815=CARTESIAN_POINT ( 'NONE',  ( 117.4075167370973958, -38.36336677748749224, 113.7013395616249767 ) ) ;
#45816=ORIENTED_EDGE ( 'NONE', *, *, #59644, .F. ) ;
#45818=ORIENTED_EDGE ( 'NONE', *, *, #52968, .T. ) ;
#45820=CYLINDRICAL_SURFACE ( 'NONE', #40612, 2.500000000000002220 ) ;
#45821=CARTESIAN_POINT ( 'NONE',  ( 135.4870310422260502, -34.36767655968418467, 1.942446731272566174 ) ) ;
#45822=EDGE_LOOP ( 'NONE', ( #64806, #27720, #16081, #16455 ) ) ;
#45823=LINE ( 'NONE', #24963, #65065 ) ;
#45824=CARTESIAN_POINT ( 'NONE',  ( 108.0382549187111607, -25.67193643048636886, 109.9946728949589811 ) ) ;
#45825=EDGE_LOOP ( 'NONE', ( #78579, #41341 ) ) ;
#45826=CARTESIAN_POINT ( 'NONE',  ( 107.0664832912739968, -36.72944715994100306, 287.6356252759109680 ) ) ;
#45828=CARTESIAN_POINT ( 'NONE',  ( 182.0667039024476708, -33.35206098992059509, 313.9678068554149490 ) ) ;
#45829=CARTESIAN_POINT ( 'NONE',  ( 46.48091746482041486, -48.32844715994088602, 180.4678068554150911 ) ) ;
#45832=CARTESIAN_POINT ( 'NONE',  ( 102.6066768796756037, -46.86875521856975269, 132.2346728949579528 ) ) ;
#45834=VECTOR ( 'NONE', #37867, 1000.000000000000000 ) ;
#45835=PLANE ( 'NONE',  #19641 ) ;
#45837=VERTEX_POINT ( 'NONE', #1411 ) ;
#45838=ORIENTED_EDGE ( 'NONE', *, *, #69221, .F. ) ;
#45842=LINE ( 'NONE', #60381, #21195 ) ;
#45843=DIRECTION ( 'NONE',  ( -1.000000000000000078E-15, 1.000000000000000083E-30, 1.000000000000000000 ) ) ;
#45844=CARTESIAN_POINT ( 'NONE',  ( 49.21437657594998427, -35.91149509761070391, -5.074374724088000832 ) ) ;
#45845=CARTESIAN_POINT ( 'NONE',  ( 97.81168844167092402, -40.51740470302234343, 181.6357138554620576 ) ) ;
#45847=EDGE_LOOP ( 'NONE', ( #37839, #23112, #75912, #37653 ) ) ;
#45850=CARTESIAN_POINT ( 'NONE',  ( 172.5664832912740110, -32.07844715994070839, 143.6756252759119832 ) ) ;
#45851=ADVANCED_FACE ( 'NONE', ( #71353 ), #37265, .F. ) ;
#45852=CARTESIAN_POINT ( 'NONE',  ( 117.2610056464982904, -34.82931580038573571, 199.9851490854349549 ) ) ;
#45853=DIRECTION ( 'NONE',  ( 1.000000000000000078E-15, 1.000000000000000083E-30, -1.000000000000000000 ) ) ;
#45854=ORIENTED_EDGE ( 'NONE', *, *, #85976, .T. ) ;
#45855=EDGE_CURVE ( 'NONE', #5575, #60824, #79057, .T. ) ;
#45856=CARTESIAN_POINT ( 'NONE',  ( 104.2296407737279935, -46.70397019442127373, 63.36800622829197494 ) ) ;
#45857=CARTESIAN_POINT ( 'NONE',  ( 110.8542424614423823, -45.98433130124127644, 52.88560554285743365 ) ) ;
#45859=CARTESIAN_POINT ( 'NONE',  ( 188.5667039024479834, -67.87844715994100397, 298.0928068554150627 ) ) ;
#45860=EDGE_CURVE ( 'NONE', #15299, #80043, #66290, .T. ) ;
#45861=ORIENTED_EDGE ( 'NONE', *, *, #76446, .F. ) ;
#45863=EDGE_LOOP ( 'NONE', ( #44695, #56091, #53527, #67737 ) ) ;
#45865=CARTESIAN_POINT ( 'NONE',  ( 98.10010861879410982, -32.13871408278030373, 242.3815833058969815 ) ) ;
#45866=EDGE_CURVE ( 'NONE', #25323, #65644, #50999, .T. ) ;
#45867=CARTESIAN_POINT ( 'NONE',  ( 97.84270335286004183, -40.59238673107780215, 52.64166371051710769 ) ) ;
#45869=EDGE_CURVE ( 'NONE', #62271, #39918, #79510, .T. ) ;
#45872=EDGE_LOOP ( 'NONE', ( #79372, #36773, #46795, #10400, #36252, #89612, #43295, #21600, #44412, #68292, #32717, #67827 ) ) ;
#45873=DIRECTION ( 'NONE',  ( 1.000000000000000000, 0.000000000000000000, 0.000000000000000000 ) ) ;
#45874=CARTESIAN_POINT ( 'NONE',  ( 109.7165975557216342, -26.99861574449257162, 35.86486515683853327 ) ) ;
#45875=EDGE_LOOP ( 'NONE', ( #86388, #71294 ) ) ;
#45876=CARTESIAN_POINT ( 'NONE',  ( 96.55902551080266960, -40.08462249002853639, 281.5603871806728762 ) ) ;
#45877=ORIENTED_EDGE ( 'NONE', *, *, #30746, .F. ) ;
#45879=CARTESIAN_POINT ( 'NONE',  ( 98.80728567624888115, -32.50078473314371763, 243.7680903695909649 ) ) ;
#45880=EDGE_CURVE ( 'NONE', #2296, #86147, #11338, .T. ) ;
#45881=DIRECTION ( 'NONE',  ( 0.000000000000000000, -1.000000000000000000, 0.000000000000000000 ) ) ;
#45883=DIRECTION ( 'NONE',  ( 1.000000000000000078E-15, -1.000000000000000083E-30, -1.000000000000000000 ) ) ;
#45885=CIRCLE ( 'NONE', #38645, 2.500000000000002220 ) ;
#45886=EDGE_CURVE ( 'NONE', #47492, #72226, #39490, .T. ) ;
#45887=CARTESIAN_POINT ( 'NONE',  ( 104.1737878132142043, -26.63141132829087354, 221.2984824187679465 ) ) ;
#45888=AXIS2_PLACEMENT_3D ( 'NONE', #18754, #17860, #73259 ) ;
#45889=LINE ( 'NONE', #71851, #60167 ) ;
#45890=VERTEX_POINT ( 'NONE', #87648 ) ;
#45891=VECTOR ( 'NONE', #19381, 1000.000000000000000 ) ;
#45892=CARTESIAN_POINT ( 'NONE',  ( 98.68765228159747949, -43.00544673443933874, 62.83848241876793850 ) ) ;
#45893=CARTESIAN_POINT ( 'NONE',  ( 80.06648329127402519, -46.42944715994105565, 4.925625275910944012 ) ) ;
#45894=VECTOR ( 'NONE', #6798, 1000.000000000000000 ) ;
#45895=B_SPLINE_CURVE_WITH_KNOTS ( 'NONE', 3,
 ( #865, #34929, #8589, #14955, #28107, #57154, #28562, #56249, #42623, #63539, #84000, #35822, #1320, #21773, #77178, #70358, #70813, #63998, #7239, #69465, #29027, #8133, #56712, #84457, #22218, #49893, #15847 ),
 .UNSPECIFIED., .F., .F.,
 ( 4, 2, 1, 1, 1, 2, 2, 2, 2, 2, 2, 2, 2, 2, 4 ),
 ( 0.5000609409785667925, 0.5010373844532182153, 0.5020138279278696380, 0.5039667148771719285, 0.5078724887757768425, 0.5156840365729865594, 0.5313071321674062153, 0.5625533233562457491, 0.6250457057339249278, 0.6875380881116041065, 0.7500304704892832852, 0.8125228528669624639, 0.8750152352446416426, 0.9375076176223208213, 1.000000000000000000 ),
 .UNSPECIFIED. ) ;
#45898=ORIENTED_EDGE ( 'NONE', *, *, #37491, .T. ) ;
#45899=CARTESIAN_POINT ( 'NONE',  ( 82.54618223952044787, -17.53884010536265237, 2.747932095378487816 ) ) ;
#45900=CARTESIAN_POINT ( 'NONE',  ( 141.0664832912739826, -8.729447159940953327, -4.970821333495649696 ) ) ;
#45901=CARTESIAN_POINT ( 'NONE',  ( 108.3314640124533668, -46.73508453131670137, 152.6777937298070640 ) ) ;
#45902=CARTESIAN_POINT ( 'NONE',  ( 108.3793409795780036, -28.17508408765456096, 142.7614237029239632 ) ) ;
#45903=CARTESIAN_POINT ( 'NONE',  ( 117.3563231384421357, -34.92488217824808316, 239.9641967044819637 ) ) ;
#45904=CARTESIAN_POINT ( 'NONE',  ( 117.0722999933526012, -35.46582721381028591, 59.92702479522854730 ) ) ;
#45905=EDGE_CURVE ( 'NONE', #3093, #3392, #42243, .T. ) ;
#45907=EDGE_CURVE ( 'NONE', #53161, #45331, #62616, .T. ) ;
#45908=CARTESIAN_POINT ( 'NONE',  ( 134.8178559631103894, -39.40256188477528099, 1.690787648075052552 ) ) ;
#45909=EDGE_LOOP ( 'NONE', ( #20121, #69755, #20072, #10742, #39782, #60958, #54818, #51849 ) ) ;
#45912=ORIENTED_EDGE ( 'NONE', *, *, #3035, .T. ) ;
#45915=CARTESIAN_POINT ( 'NONE',  ( 48.45959712127140051, -26.00627455219179751, 193.9678068554150911 ) ) ;
#45916=DIRECTION ( 'NONE',  ( 0.000000000000000000, 0.000000000000000000, 1.000000000000000000 ) ) ;
#45917=CARTESIAN_POINT ( 'NONE',  ( 100.8033404080456705, -29.31000718268690619, 150.0581341137909703 ) ) ;
#45918=CARTESIAN_POINT ( 'NONE',  ( 111.3412100197261765, -27.17259740239810739, 24.74133956162494030 ) ) ;
#45920=CARTESIAN_POINT ( 'NONE',  ( 156.5667039024485518, -48.82844715993568485, 173.2178068554149775 ) ) ;
#45922=EDGE_CURVE ( 'NONE', #69972, #22750, #40822, .T. ) ;
#45923=CARTESIAN_POINT ( 'NONE',  ( 107.0664832912739968, -36.72944715994100306, 287.6356252759109680 ) ) ;
#45925=CARTESIAN_POINT ( 'NONE',  ( 25.56670390244797275, -62.87844715994099687, 132.3428068554150343 ) ) ;
#45926=CARTESIAN_POINT ( 'NONE',  ( 116.3212776292272537, -32.94146857470742162, 144.1356252759109680 ) ) ;
#45927=CARTESIAN_POINT ( 'NONE',  ( 97.82529165045187369, -40.55051507927917243, 131.6384725568923102 ) ) ;
#45931=CARTESIAN_POINT ( 'NONE',  ( 97.08353706812128792, -39.80957011747380392, 21.56419670448195092 ) ) ;
#45932=CARTESIAN_POINT ( 'NONE',  ( 97.31101637507774171, -32.83472251844465717, 37.02419670448292521 ) ) ;
#45936=DIRECTION ( 'NONE',  ( 0.000000000000000000, -1.000000000000000000, 0.000000000000000000 ) ) ;
#45937=CARTESIAN_POINT ( 'NONE',  ( 89.33314995793998037, 12.92155284005730387, 361.9756252759109998 ) ) ;
#45939=FACE_BOUND ( 'NONE', #11165, .T. ) ;
#45940=CARTESIAN_POINT ( 'NONE',  ( 53.56670390244828184, -48.82844715994055917, 300.4678068554150059 ) ) ;
#45942=CARTESIAN_POINT ( 'NONE',  ( 100.5231322539815153, -27.76298515809465073, 30.56610146638794134 ) ) ;
#45943=CARTESIAN_POINT ( 'NONE',  ( 110.4988674196275014, -26.88560509280327082, 205.8099109901969541 ) ) ;
#45944=CARTESIAN_POINT ( 'NONE',  ( 116.2507439086588761, -31.75083131158774918, 65.22133956162595325 ) ) ;
#45945=CIRCLE ( 'NONE', #14076, 18.00000000000000000 ) ;
#45946=AXIS2_PLACEMENT_3D ( 'NONE', #5907, #89018, #61298 ) ;
#45947=CARTESIAN_POINT ( 'NONE',  ( 116.7958306881861148, -39.38531486699053374, 173.6120842293531723 ) ) ;
#45948=DIRECTION ( 'NONE',  ( 1.000000000000000000, 0.000000000000000000, 0.000000000000000000 ) ) ;
#45951=AXIS2_PLACEMENT_3D ( 'NONE', #85491, #50936, #2357 ) ;
#45954=EDGE_CURVE ( 'NONE', #41305, #34264, #18597, .T. ) ;
#45955=FACE_OUTER_BOUND ( 'NONE', #53369, .T. ) ;
#45958=CARTESIAN_POINT ( 'NONE',  ( 98.49710108934571906, -31.94619897774425610, 106.9213395616249755 ) ) ;
#45960=ORIENTED_EDGE ( 'NONE', *, *, #44468, .F. ) ;
#45961=EDGE_CURVE ( 'NONE', #27646, #32492, #24529, .T. ) ;
#45962=CARTESIAN_POINT ( 'NONE',  ( 96.79764630557892247, -40.75620882907055176, 242.6118157521009664 ) ) ;
#45965=CARTESIAN_POINT ( 'NONE',  ( 110.8740616933906864, -45.97620365431721012, 147.8873101108567312 ) ) ;
#45966=CARTESIAN_POINT ( 'NONE',  ( 179.7974245136207685, -36.32844715993469720, 313.9678068554149490 ) ) ;
#45967=CARTESIAN_POINT ( 'NONE',  ( 97.81169418859235520, -40.51741816698509524, 47.63568902202231925 ) ) ;
#45969=EDGE_CURVE ( 'NONE', #48081, #8213, #52194, .T. ) ;
#45971=VECTOR ( 'NONE', #73374, 1000.000000000000114 ) ;
#45972=VECTOR ( 'NONE', #39008, 1000.000000000000000 ) ;
#45973=CARTESIAN_POINT ( 'NONE',  ( 107.8656169629272483, -46.51081515578112402, 177.6413395616259834 ) ) ;
#45974=EDGE_LOOP ( 'NONE', ( #8060, #30402, #85236, #495 ) ) ;
#45976=CARTESIAN_POINT ( 'NONE',  ( 103.2835872187480533, -45.32980894545860906, 128.6663452106589887 ) ) ;
#45977=AXIS2_PLACEMENT_3D ( 'NONE', #85034, #29602, #69600 ) ;
#45979=DIRECTION ( 'NONE',  ( 0.000000000000000000, 0.000000000000000000, 1.000000000000000000 ) ) ;
#45980=CARTESIAN_POINT ( 'NONE',  ( 98.14754276252335785, -43.36755551587071977, 257.8356252759109566 ) ) ;
#45983=DIRECTION ( 'NONE',  ( -0.7071067811578587436, 0.7071067812152364018, 0.000000000000000000 ) ) ;
#45984=ADVANCED_FACE ( 'NONE', ( #25411 ), #53533, .T. ) ;
#45985=LINE ( 'NONE', #17856, #21439 ) ;
#45986=CARTESIAN_POINT ( 'NONE',  ( 151.0371591254582881, -46.82818131005593187, 249.9678068554149490 ) ) ;
#45987=FACE_BOUND ( 'NONE', #81822, .T. ) ;
#45988=CARTESIAN_POINT ( 'NONE',  ( 188.5667039024479834, -65.37844715994100397, 137.2178068554150059 ) ) ;
#45989=CARTESIAN_POINT ( 'NONE',  ( 108.6716496925947126, -26.45072611336619772, 189.9527681330539792 ) ) ;
#45991=ORIENTED_EDGE ( 'NONE', *, *, #68364, .F. ) ;
#45995=DIRECTION ( 'NONE',  ( -1.000000000000000078E-15, -1.000000000000000083E-30, 1.000000000000000000 ) ) ;
#45997=VERTEX_POINT ( 'NONE', #10008 ) ;
#45998=CARTESIAN_POINT ( 'NONE',  ( 73.17003668186730181, -46.47944715994106701, 14.92562527591093691 ) ) ;
#45999=CARTESIAN_POINT ( 'NONE',  ( 97.47293644110631305, -40.89955093664978136, 231.6527681330539679 ) ) ;
#46002=ORIENTED_EDGE ( 'NONE', *, *, #48760, .F. ) ;
#46003=CARTESIAN_POINT ( 'NONE',  ( 97.81305373959743577, -40.51655628150228949, 62.63606721061723448 ) ) ;
#46005=CARTESIAN_POINT ( 'NONE',  ( 116.8175535499631792, -34.15458648068190683, 165.0313227694681757 ) ) ;
#46006=CARTESIAN_POINT ( 'NONE',  ( 110.4716576677765119, -44.14797218061634254, 25.73666179816297372 ) ) ;
#46007=DIRECTION ( 'NONE',  ( 9.351236661543306751E-17, -3.725950533538267725E-29, -1.000000000000000000 ) ) ;
#46008=VERTEX_POINT ( 'NONE', #37720 ) ;
#46009=VECTOR ( 'NONE', #40685, 1000.000000000000000 ) ;
#46011=CARTESIAN_POINT ( 'NONE',  ( 192.5667039024473013, -23.42844715993434335, 249.9678068554149775 ) ) ;
#46013=ORIENTED_EDGE ( 'NONE', *, *, #13347, .T. ) ;
#46014=EDGE_LOOP ( 'NONE', ( #30083, #33284, #9011, #31801, #29976, #58586, #46426, #44258, #50482, #13336, #67151, #42245 ) ) ;
#46015=AXIS2_PLACEMENT_3D ( 'NONE', #66756, #32229, #30462 ) ;
#46016=VECTOR ( 'NONE', #53020, 1000.000000000000000 ) ;
#46017=CARTESIAN_POINT ( 'NONE',  ( 97.81151477712479902, -40.51751189930152464, 186.6359914586728337 ) ) ;
#46018=AXIS2_PLACEMENT_3D ( 'NONE', #57530, #85270, #50713 ) ;
#46019=ORIENTED_EDGE ( 'NONE', *, *, #84663, .T. ) ;
#46022=CARTESIAN_POINT ( 'NONE',  ( 114.5755952152626946, -32.65889807719148052, 68.64384839950594142 ) ) ;
#46023=CARTESIAN_POINT ( 'NONE',  ( 103.5348926201861985, -26.85948109348520418, 190.3499109901969746 ) ) ;
#46024=CARTESIAN_POINT ( 'NONE',  ( 96.67182511810079859, -37.15340426533111895, 161.3584824187679487 ) ) ;
#46025=CARTESIAN_POINT ( 'NONE',  ( 41.56648329127399677, -9.303447159940999356, 141.0426252759120018 ) ) ;
#46026=CARTESIAN_POINT ( 'NONE',  ( 115.6552720357279753, -30.75834705514724732, 275.3099109901965562 ) ) ;
#46028=DIRECTION ( 'NONE',  ( 0.000000000000000000, 0.000000000000000000, 1.000000000000000000 ) ) ;
#46029=ORIENTED_EDGE ( 'NONE', *, *, #36741, .F. ) ;
#46030=TOROIDAL_SURFACE ( 'NONE', #72205, 11.75000000000000000, 2.125000000000000000 ) ;
#46032=AXIS2_PLACEMENT_3D ( 'NONE', #67333, #34613, #74608 ) ;
#46033=VECTOR ( 'NONE', #67563, 1000.000000000000000 ) ;
#46035=CARTESIAN_POINT ( 'NONE',  ( 72.31648329127399677, -9.833000550534366724, -5.074374724089063982 ) ) ;
#46036=CARTESIAN_POINT ( 'NONE',  ( 110.0646822317013118, -26.04189894992025955, 219.8708633711489711 ) ) ;
#46038=CARTESIAN_POINT ( 'NONE',  ( 101.2005795642084820, -45.34792753215401007, 197.1013395616249966 ) ) ;
#46039=CARTESIAN_POINT ( 'NONE',  ( 97.33774478695349330, -34.07145668252834980, 266.1148423016875881 ) ) ;
#46041=LINE ( 'NONE', #17474, #75458 ) ;
#46042=CYLINDRICAL_SURFACE ( 'NONE', #44159, 2.750000000000002665 ) ;
#46043=CARTESIAN_POINT ( 'NONE',  ( 113.8270003667112746, -32.37296061313053741, 277.6356252759109680 ) ) ;
#46045=CARTESIAN_POINT ( 'NONE',  ( 105.1131368864170526, -25.87365329830177529, 271.2061014663872243 ) ) ;
#46046=CARTESIAN_POINT ( 'NONE',  ( 100.8872181613150900, -44.70003033885427612, 173.0522674363715510 ) ) ;
#46048=CARTESIAN_POINT ( 'NONE',  ( 180.2143765759489895, -35.91149509761070391, -5.074374724088000832 ) ) ;
#46049=LINE ( 'NONE', #73783, #38501 ) ;
#46051=CYLINDRICAL_SURFACE ( 'NONE', #85516, 4.750000000000004441 ) ;
#46052=LINE ( 'NONE', #67407, #66034 ) ;
#46054=CARTESIAN_POINT ( 'NONE',  ( 136.7635286919467887, -19.26660482608927083, 6.827192804310395324 ) ) ;
#46055=CARTESIAN_POINT ( 'NONE',  ( 114.6215443236117153, -29.51367161159714314, 234.4327681330539690 ) ) ;
#46056=CARTESIAN_POINT ( 'NONE',  ( 101.5008874824296896, -27.91431070382771651, 106.5241967044819944 ) ) ;
#46057=CARTESIAN_POINT ( 'NONE',  ( 115.5527055449870772, -29.57532036350955806, 220.3718157521019521 ) ) ;
#46058=DIRECTION ( 'NONE',  ( 1.000000000000000000, 4.163336342344333240E-14, 0.000000000000000000 ) ) ;
#46059=DIRECTION ( 'NONE',  ( 1.000000000000000000, 2.106816776397999944E-14, 7.761631831580328254E-43 ) ) ;
#46061=CARTESIAN_POINT ( 'NONE',  ( 114.7049794032198520, -43.22496099079516796, 39.26526583603205722 ) ) ;
#46062=CARTESIAN_POINT ( 'NONE',  ( 32.06670390244800473, -32.29483332968611364, -5.074374724088000832 ) ) ;
#46063=AXIS2_PLACEMENT_3D ( 'NONE', #174, #14263, #55551 ) ;
#46064=CARTESIAN_POINT ( 'NONE',  ( 131.3165190107490332, -18.90078909148325792, 3.101427792080756252 ) ) ;
#46065=ORIENTED_EDGE ( 'NONE', *, *, #53919, .T. ) ;
#46066=ORIENTED_EDGE ( 'NONE', *, *, #41483, .T. ) ;
#46068=CARTESIAN_POINT ( 'NONE',  ( 109.0672552851176249, -45.03324407163384535, 132.1867055423619775 ) ) ;
#46070=EDGE_LOOP ( 'NONE', ( #30790, #19510, #32203, #71079 ) ) ;
#46072=EDGE_CURVE ( 'NONE', #75711, #15908, #83089, .T. ) ;
#46073=CARTESIAN_POINT ( 'NONE',  ( 108.6454077996538246, -25.81962716842098970, 145.9737205140069420 ) ) ;
#46074=LINE ( 'NONE', #61068, #19296 ) ;
#46076=LINE ( 'NONE', #16623, #29798 ) ;
#46077=CARTESIAN_POINT ( 'NONE',  ( 152.4409905591762708, -0.9151414768250908383, 542.9756252759101471 ) ) ;
#46080=VECTOR ( 'NONE', #83174, 1000.000000000000000 ) ;
#46081=CARTESIAN_POINT ( 'NONE',  ( 117.3261810260836597, -38.23854875528750341, 73.72229194257801055 ) ) ;
#46082=VERTEX_POINT ( 'NONE', #68992 ) ;
#46083=VERTEX_POINT ( 'NONE', #68545 ) ;
#46084=ORIENTED_EDGE ( 'NONE', *, *, #55209, .F. ) ;
#46086=AXIS2_PLACEMENT_3D ( 'NONE', #45079, #31876, #10104 ) ;
#46087=DIRECTION ( 'NONE',  ( 1.147230458779309805E-16, 3.204747427460360459E-31, 1.000000000000000000 ) ) ;
#46088=CARTESIAN_POINT ( 'NONE',  ( 117.1170091337236414, -34.17489915221372598, 165.0365776568629315 ) ) ;
#46089=CARTESIAN_POINT ( 'NONE',  ( 97.81168895331838087, -40.51742574516882200, 287.6356252759109680 ) ) ;
#46090=CARTESIAN_POINT ( 'NONE',  ( 31.90335556477799628, -33.89581943344391135, -5.074374724088000832 ) ) ;
#46092=EDGE_CURVE ( 'NONE', #39136, #18492, #307, .T. ) ;
#46093=CARTESIAN_POINT ( 'NONE',  ( 151.0371591254582881, -46.82818131005593187, 237.4678068554150059 ) ) ;
#46094=VECTOR ( 'NONE', #82575, 999.9999999999998863 ) ;
#46095=CARTESIAN_POINT ( 'NONE',  ( 46.83715912545343940, -47.82818131006086304, 129.9678068554150911 ) ) ;
#46096=CARTESIAN_POINT ( 'NONE',  ( 41.56648329127398966, -27.82844715994070484, 18.92562527591200094 ) ) ;
#46097=CARTESIAN_POINT ( 'NONE',  ( 118.8180844208009717, -35.40729807334668067, 83.91562527591095488 ) ) ;
#46098=ORIENTED_EDGE ( 'NONE', *, *, #82300, .T. ) ;
#46099=VERTEX_POINT ( 'NONE', #82645 ) ;
#46100=VECTOR ( 'NONE', #47822, 1000.000000000000000 ) ;
#46103=VECTOR ( 'NONE', #78990, 1000.000000000000000 ) ;
#46104=CIRCLE ( 'NONE', #60639, 2.030000000000003801 ) ;
#46105=CARTESIAN_POINT ( 'NONE',  ( 41.56648329127499153, -36.32844715994070839, 74.17562527591199739 ) ) ;
#46106=CARTESIAN_POINT ( 'NONE',  ( 114.9429295168758784, -34.48920150425379916, 146.8652332267339773 ) ) ;
#46108=B_SPLINE_CURVE_WITH_KNOTS ( 'NONE', 3,
 ( #24267, #5157, #53719, #59653, #51937, #31959, #32853, #81485, #60549, #74642, #52371, #60094, #12420, #80134, #87384, #32392, #40109, #67826, #5618, #33309, #25143, #80580, #17448, #45129, #52804, #66933, #18784, #59213, #18329, #46467, #10622, #38326, #73747, #39223, #11528, #25595, #68286 ),
 .UNSPECIFIED., .F., .F.,
 ( 4, 2, 2, 1, 2, 2, 2, 1, 1, 2, 2, 2, 2, 1, 2, 2, 2, 1, 1, 1, 2, 4 ),
 ( 0.6666501603260506226, 0.6874845253056601768, 0.6926931165505625376, 0.6979017077954648984, 0.7083188902852692870, 0.7499876202444850648, 0.7525919158669366338, 0.7551962114893882028, 0.7604048027342921179, 0.7708219852241017245, 0.7916563502037200495, 0.8124907151833384855, 0.8176993064282435109, 0.8229078976731485362, 0.8333250801629586979, 0.8749938101222022313, 0.8775981057446557987, 0.8802024013671094771, 0.8854109926120167229, 0.8958281751018317696, 0.9166625400814643054, 1.000000000000000000 ),
 .UNSPECIFIED. ) ;
#46110=EDGE_LOOP ( 'NONE', ( #23776, #79125, #3567, #25664 ) ) ;
#46112=VECTOR ( 'NONE', #56311, 1000.000000000000000 ) ;
#46115=ORIENTED_EDGE ( 'NONE', *, *, #62706, .F. ) ;
#46117=CARTESIAN_POINT ( 'NONE',  ( 115.3890540380527767, -39.77298043176836018, 214.9787261630399655 ) ) ;
#46118=DIRECTION ( 'NONE',  ( 0.000000000000000000, 0.000000000000000000, 1.000000000000000000 ) ) ;
#46119=VECTOR ( 'NONE', #81904, 1000.000000000000000 ) ;
#46120=ADVANCED_FACE ( 'NONE', ( #55771 ), #39927, .T. ) ;
#46121=CARTESIAN_POINT ( 'NONE',  ( 41.56670390244776314, -36.32844715994104234, 313.9678068554150059 ) ) ;
#46122=CIRCLE ( 'NONE', #12842, 0.5000000000000004441 ) ;
#46125=ORIENTED_EDGE ( 'NONE', *, *, #21802, .F. ) ;
#46126=ORIENTED_EDGE ( 'NONE', *, *, #51222, .T. ) ;
#46128=ADVANCED_FACE ( 'NONE', ( #46734 ), #19495, .T. ) ;
#46129=CARTESIAN_POINT ( 'NONE',  ( 99.00928370863422856, -39.88895027456798914, 244.4299951314959571 ) ) ;
#46130=CARTESIAN_POINT ( 'NONE',  ( 113.3557719660652339, -27.61131746675945209, 89.60800622829195561 ) ) ;
#46131=CARTESIAN_POINT ( 'NONE',  ( 98.11562048848810491, -31.42749274529980852, 85.90133956162493689 ) ) ;
#46132=FACE_OUTER_BOUND ( 'NONE', #67894, .T. ) ;
#46134=DIRECTION ( 'NONE',  ( -4.237773401492740281E-14, 1.000000000000000000, 0.000000000000000000 ) ) ;
#46135=CARTESIAN_POINT ( 'NONE',  ( 117.0331605330187728, -30.31849857022486816, 140.2813395616249750 ) ) ;
#46140=ORIENTED_EDGE ( 'NONE', *, *, #36470, .T. ) ;
#46141=LINE ( 'NONE', #87067, #11382 ) ;
#46142=CARTESIAN_POINT ( 'NONE',  ( 32.09598329127620531, -23.42844715994129956, 117.4678068554150485 ) ) ;
#46143=ORIENTED_EDGE ( 'NONE', *, *, #76553, .T. ) ;
#46145=DIRECTION ( 'NONE',  ( 0.000000000000000000, 0.000000000000000000, -1.000000000000000000 ) ) ;
#46146=VECTOR ( 'NONE', #51655, 1000.000000000000000 ) ;
#46150=CARTESIAN_POINT ( 'NONE',  ( 114.5675797908445475, -44.02050044317889643, 98.21276813305395592 ) ) ;
#46154=CARTESIAN_POINT ( 'NONE',  ( 96.76615086495793605, -37.93025403122317130, 86.43086337114897333 ) ) ;
#46156=CARTESIAN_POINT ( 'NONE',  ( 117.4047238282098249, -30.98758422922437106, 175.2299109901969700 ) ) ;
#46159=ORIENTED_EDGE ( 'NONE', *, *, #76774, .T. ) ;
#46160=CARTESIAN_POINT ( 'NONE',  ( 188.5667039024479834, -58.35344715994099829, 170.4678068554149775 ) ) ;
#46162=CARTESIAN_POINT ( 'NONE',  ( 194.5667039024482676, -40.82844715993405060, 129.9678068554150343 ) ) ;
#46163=CARTESIAN_POINT ( 'NONE',  ( 116.3197976069899795, -32.94561274469138112, 134.1356252759109680 ) ) ;
#46167=CARTESIAN_POINT ( 'NONE',  ( 114.6374585114582771, -29.49847210400304576, 234.4327681330539690 ) ) ;
#46168=ORIENTED_EDGE ( 'NONE', *, *, #57404, .T. ) ;
#46169=CARTESIAN_POINT ( 'NONE',  ( 97.06384626284506112, -37.34233656640287791, 146.3752414903799774 ) ) ;
#46170=CARTESIAN_POINT ( 'NONE',  ( 97.79230575738172604, -40.52535926896634777, 7.635625275910939536 ) ) ;
#46171=CARTESIAN_POINT ( 'NONE',  ( 117.7479605218750862, -39.74664297364158472, 139.6194347997199827 ) ) ;
#46174=CARTESIAN_POINT ( 'NONE',  ( 156.5667039024481255, -42.82844715993568485, 257.2178068554149490 ) ) ;
#46175=CARTESIAN_POINT ( 'NONE',  ( 123.6837132603319560, -52.08770651782484862, 218.8274735512161158 ) ) ;
#46177=EDGE_LOOP ( 'NONE', ( #60726, #84629 ) ) ;
#46180=ORIENTED_EDGE ( 'NONE', *, *, #72161, .T. ) ;
#46181=DIRECTION ( 'NONE',  ( 0.000000000000000000, 0.000000000000000000, -1.000000000000000000 ) ) ;
#46182=CARTESIAN_POINT ( 'NONE',  ( 101.6204011159890541, -47.22657592904984369, 13.19562527591094891 ) ) ;
#46184=CARTESIAN_POINT ( 'NONE',  ( 188.5667039024479834, -62.87844715994099687, 257.2178068554150059 ) ) ;
#46185=EDGE_CURVE ( 'NONE', #87456, #78504, #88552, .T. ) ;
#46186=CARTESIAN_POINT ( 'NONE',  ( 180.2121375201600131, -29.73316016639650172, -5.074374724088000832 ) ) ;
#46188=AXIS2_PLACEMENT_3D ( 'NONE', #22252, #34514, #7712 ) ;
#46189=CARTESIAN_POINT ( 'NONE',  ( 102.6292086192877946, -44.02785282196147421, 246.5638483995049626 ) ) ;
#46190=EDGE_LOOP ( 'NONE', ( #60201, #43906, #70700, #83113 ) ) ;
#46191=AXIS2_PLACEMENT_3D ( 'NONE', #76389, #14624, #85802 ) ;
#46192=ORIENTED_EDGE ( 'NONE', *, *, #64014, .T. ) ;
#46193=VERTEX_POINT ( 'NONE', #6760 ) ;
#46194=DIRECTION ( 'NONE',  ( 1.000000000000000078E-15, 1.000000000000000083E-30, -1.000000000000000000 ) ) ;
#46196=DIRECTION ( 'NONE',  ( 0.000000000000000000, 0.000000000000000000, 1.000000000000000000 ) ) ;
#46197=CARTESIAN_POINT ( 'NONE',  ( 110.6847694559308621, -28.64017749364363397, 21.17301187732595480 ) ) ;
#46199=ADVANCED_FACE ( 'NONE', ( #53984 ), #26311, .T. ) ;
#46200=DIRECTION ( 'NONE',  ( -1.000000000000000000, 0.000000000000000000, 2.820351377559424413E-14 ) ) ;
#46202=CARTESIAN_POINT ( 'NONE',  ( 116.2779988688840547, -41.49250982992363390, 243.4346728949589647 ) ) ;
#46203=CARTESIAN_POINT ( 'NONE',  ( 19.56670390244648416, -25.42844715994203852, 129.9678068554150627 ) ) ;
#46205=AXIS2_PLACEMENT_3D ( 'NONE', #65620, #58788, #10649 ) ;
#46207=DIRECTION ( 'NONE',  ( 0.000000000000000000, 0.000000000000000000, -1.000000000000000000 ) ) ;
#46208=CARTESIAN_POINT ( 'NONE',  ( 100.8021347340043690, -42.70095134221056554, 34.73856656006796584 ) ) ;
#46210=CONICAL_SURFACE ( 'NONE', #17203, 17.00000000000090239, 0.7853981633974447263 ) ;
#46211=CARTESIAN_POINT ( 'NONE',  ( 136.1113402350857484, -16.88977106734701294, 7.516154048581690006 ) ) ;
#46212=DIRECTION ( 'NONE',  ( 0.000000000000000000, 1.000000000000000000, 0.000000000000000000 ) ) ;
#46213=LINE ( 'NONE', #19429, #18420 ) ;
#46214=ORIENTED_EDGE ( 'NONE', *, *, #15559, .T. ) ;
#46215=CYLINDRICAL_SURFACE ( 'NONE', #16082, 0.5000000000000079936 ) ;
#46216=CIRCLE ( 'NONE', #56352, 2.517499999999998739 ) ;
#46219=CARTESIAN_POINT ( 'NONE',  ( 111.0826007845189736, -25.57995003598136208, 99.80133956162498521 ) ) ;
#46220=EDGE_LOOP ( 'NONE', ( #82687, #43352, #70894, #62181 ) ) ;
#46221=CARTESIAN_POINT ( 'NONE',  ( 98.53752338633383090, -37.19093893883378144, 75.79241982807700140 ) ) ;
#46222=VECTOR ( 'NONE', #81888, 1000.000000000000000 ) ;
#46223=CARTESIAN_POINT ( 'NONE',  ( 97.81554923370184440, -40.52685731699395433, 87.63597259388511418 ) ) ;
#46224=CARTESIAN_POINT ( 'NONE',  ( 97.69004538871082843, -40.41090301495324155, 93.05586902018298190 ) ) ;
#46225=CARTESIAN_POINT ( 'NONE',  ( 156.5667039024483529, -48.82844715993569196, 293.2178068554149490 ) ) ;
#46227=CARTESIAN_POINT ( 'NONE',  ( 168.3664380525668491, -48.62818131005487743, 129.9678068554150059 ) ) ;
#46228=CARTESIAN_POINT ( 'NONE',  ( 104.2350475155005114, -46.78530274442771031, 18.35848241876792031 ) ) ;
#46229=CARTESIAN_POINT ( 'NONE',  ( 97.81151460250711693, -40.51751193867107759, 182.6359910548048333 ) ) ;
#46230=ORIENTED_EDGE ( 'NONE', *, *, #59029, .T. ) ;
#46231=DIRECTION ( 'NONE',  ( 1.000000000000000078E-15, -1.000000000000000083E-30, -1.000000000000000000 ) ) ;
#46237=CARTESIAN_POINT ( 'NONE',  ( 80.06648329127402519, -46.72944715994105991, 1.625625275910943746 ) ) ;
#46239=CARTESIAN_POINT ( 'NONE',  ( 97.40895461294492463, -34.98419235835273611, 241.1841967044829573 ) ) ;
#46240=CARTESIAN_POINT ( 'NONE',  ( 97.03505442595846375, -37.08857983863578767, 126.3541045800583049 ) ) ;
#46242=CARTESIAN_POINT ( 'NONE',  ( 98.72253030179433608, -42.97932203522270100, 62.83848241876793850 ) ) ;
#46243=CARTESIAN_POINT ( 'NONE',  ( 99.08951106268413866, -42.79544243366853351, 42.84391520899005457 ) ) ;
#46244=ORIENTED_EDGE ( 'NONE', *, *, #15338, .T. ) ;
#46245=DIRECTION ( 'NONE',  ( -4.299999999999999979E-14, 1.000000000000000000, -4.400000000000000367E-29 ) ) ;
#46246=CARTESIAN_POINT ( 'NONE',  ( 194.5664832912729878, -71.37844715994266664, 361.9756252759109998 ) ) ;
#46249=DIRECTION ( 'NONE',  ( 1.000000000000000078E-15, -1.000000000000000083E-30, -1.000000000000000000 ) ) ;
#46252=CARTESIAN_POINT ( 'NONE',  ( 109.2074818670226222, -48.35976665079991221, 277.7213395616254843 ) ) ;
#46253=DIRECTION ( 'NONE',  ( 0.000000000000000000, 0.000000000000000000, -1.000000000000000000 ) ) ;
#46255=CARTESIAN_POINT ( 'NONE',  ( 77.31651901074906164, -36.90078909148913056, 3.101427792080711843 ) ) ;
#46256=CARTESIAN_POINT ( 'NONE',  ( 110.2012955024488718, -28.75291567525416170, 269.2009912566482512 ) ) ;
#46258=CARTESIAN_POINT ( 'NONE',  ( 117.9791962420229794, -38.33460093242096178, 69.72229194257801055 ) ) ;
#46260=CARTESIAN_POINT ( 'NONE',  ( 108.9929891821633134, -47.66111943275755181, 122.7032443235299723 ) ) ;
#46261=ORIENTED_EDGE ( 'NONE', *, *, #51430, .T. ) ;
#46262=CYLINDRICAL_SURFACE ( 'NONE', #71363, 2.517500000000005844 ) ;
#46264=EDGE_CURVE ( 'NONE', #44506, #37176, #13511, .T. ) ;
#46265=CARTESIAN_POINT ( 'NONE',  ( 19.56648329127303043, 15.62155284005731204, 361.9756252759109998 ) ) ;
#46266=DIRECTION ( 'NONE',  ( -1.000000000000000000, -1.000000000000000078E-15, -1.000000000000000078E-15 ) ) ;
#46267=CARTESIAN_POINT ( 'NONE',  ( 131.0667039024480118, -67.87844715994100397, 231.5838068554150198 ) ) ;
#46268=ORIENTED_EDGE ( 'NONE', *, *, #64992, .F. ) ;
#46269=EDGE_CURVE ( 'NONE', #64364, #7616, #58329, .T. ) ;
#46270=AXIS2_PLACEMENT_3D ( 'NONE', #52294, #85541, #16484 ) ;
#46272=CARTESIAN_POINT ( 'NONE',  ( 97.06384492438512268, -37.34231416522206359, 51.37523970808266682 ) ) ;
#46273=CARTESIAN_POINT ( 'NONE',  ( 114.5591802247839865, -28.54312911867770808, 154.4746728949589851 ) ) ;
#46274=ORIENTED_EDGE ( 'NONE', *, *, #9135, .F. ) ;
#46276=DIRECTION ( 'NONE',  ( 1.000000000000000000, 0.000000000000000000, 2.279500465453769633E-16 ) ) ;
#46277=DIRECTION ( 'NONE',  ( -0.0001713722455994026977, 0.9999999853157766072, 0.000000000000000000 ) ) ;
#46278=EDGE_CURVE ( 'NONE', #5529, #36268, #15827, .T. ) ;
#46280=DIRECTION ( 'NONE',  ( 1.000000000000000078E-15, -1.000000000000000083E-30, -1.000000000000000000 ) ) ;
#46282=VECTOR ( 'NONE', #31830, 1000.000000000000000 ) ;
#46283=CARTESIAN_POINT ( 'NONE',  ( 97.59689953814545049, -30.98293302709309671, 125.8803871806719599 ) ) ;
#46285=EDGE_CURVE ( 'NONE', #32339, #89909, #43951, .T. ) ;
#46286=DIRECTION ( 'NONE',  ( 0.000000000000000000, 1.000000000000000000, 0.000000000000000000 ) ) ;
#46289=ORIENTED_EDGE ( 'NONE', *, *, #32663, .T. ) ;
#46290=CYLINDRICAL_SURFACE ( 'NONE', #62637, 0.4999999999999976685 ) ;
#46292=DIRECTION ( 'NONE',  ( -0.9254794337955620787, -0.3787978585227822492, 0.000000000000000000 ) ) ;
#46293=ADVANCED_FACE ( 'NONE', ( #1752 ), #81574, .F. ) ;
#46295=CIRCLE ( 'NONE', #52059, 2.517500000000005844 ) ;
#46296=CARTESIAN_POINT ( 'NONE',  ( 98.34980471865662821, -31.65668200773688667, 105.9064674098472665 ) ) ;
#46297=CARTESIAN_POINT ( 'NONE',  ( 167.7413838386817133, -48.33240602328261559, 300.4678068554149490 ) ) ;
#46299=ORIENTED_EDGE ( 'NONE', *, *, #87943, .T. ) ;
#46300=CARTESIAN_POINT ( 'NONE',  ( 57.56670390244722313, -42.82844715994040996, 134.7178068554150911 ) ) ;
#46301=CARTESIAN_POINT ( 'NONE',  ( 110.2867295656602380, -27.49400189596552835, 205.8099109901959594 ) ) ;
#46302=AXIS2_PLACEMENT_3D ( 'NONE', #35778, #72106, #63492 ) ;
#46303=CARTESIAN_POINT ( 'NONE',  ( 107.0664832912740252, -36.72944715994103149, -5.074374724089029343 ) ) ;
#46305=EDGE_CURVE ( 'NONE', #87926, #86967, #70794, .T. ) ;
#46306=CARTESIAN_POINT ( 'NONE',  ( 103.8130989789263765, -45.95327097697893493, 53.30705384733897034 ) ) ;
#46307=CARTESIAN_POINT ( 'NONE',  ( 107.0664832912739968, -36.72944715994100306, 287.6356252759109680 ) ) ;
#46308=EDGE_CURVE ( 'NONE', #32467, #944, #71389, .T. ) ;
#46311=CARTESIAN_POINT ( 'NONE',  ( 97.81171347387959258, -40.51745984142272761, 22.63530404563221410 ) ) ;
#46315=ORIENTED_EDGE ( 'NONE', *, *, #20878, .T. ) ;
#46318=CARTESIAN_POINT ( 'NONE',  ( 111.6463204169710082, -44.35094448583814852, 234.4387261630399450 ) ) ;
#46319=DIRECTION ( 'NONE',  ( -1.000000000000000000, -4.299999999999999979E-14, -1.000000000000000078E-15 ) ) ;
#46322=DIRECTION ( 'NONE',  ( -1.907762142705490052E-15, -7.167082501179359715E-16, 1.000000000000000000 ) ) ;
#46323=ORIENTED_EDGE ( 'NONE', *, *, #78635, .F. ) ;
#46325=LINE ( 'NONE', #31818, #14518 ) ;
#46326=LINE ( 'NONE', #86804, #3461 ) ;
#46327=ORIENTED_EDGE ( 'NONE', *, *, #37291, .F. ) ;
#46328=CARTESIAN_POINT ( 'NONE',  ( 112.3272512417296980, -28.22507648531173530, 289.6356252759109680 ) ) ;
#46329=ORIENTED_EDGE ( 'NONE', *, *, #80192, .T. ) ;
#46330=ORIENTED_EDGE ( 'NONE', *, *, #44114, .T. ) ;
#46331=CARTESIAN_POINT ( 'NONE',  ( 102.5467118750096631, -28.62589253813684209, 253.2995189410198691 ) ) ;
#46335=CARTESIAN_POINT ( 'NONE',  ( 120.1849926298398401, -37.85453553205690724, 296.5517437918485939 ) ) ;
#46336=DIRECTION ( 'NONE',  ( 1.000000000000000078E-15, -1.000000000000000083E-30, -1.000000000000000000 ) ) ;
#46337=CARTESIAN_POINT ( 'NONE',  ( 110.1502920506493552, -26.06700738780482141, 210.8403871806729626 ) ) ;
#46338=CARTESIAN_POINT ( 'NONE',  ( 131.0667039024480118, -64.87844715994098976, 231.5838068554150198 ) ) ;
#46341=CARTESIAN_POINT ( 'NONE',  ( 114.3835678416600672, -44.21631923246377482, 69.19276813305397411 ) ) ;
#46343=ORIENTED_EDGE ( 'NONE', *, *, #44435, .T. ) ;
#46344=VERTEX_POINT ( 'NONE', #8112 ) ;
#46345=ORIENTED_EDGE ( 'NONE', *, *, #35655, .T. ) ;
#46346=VECTOR ( 'NONE', #25140, 1000.000000000000000 ) ;
#46347=DIRECTION ( 'NONE',  ( -0.7071067811865774377, 0.7071067811865175967, -7.071067811865782003E-16 ) ) ;
#46351=CARTESIAN_POINT ( 'NONE',  ( 114.9429295168758784, -34.48920150425379916, 146.8652332267339773 ) ) ;
#46352=CARTESIAN_POINT ( 'NONE',  ( 111.6179861195847849, -46.13269558042843244, 243.9356252759109509 ) ) ;
#46354=VERTEX_POINT ( 'NONE', #29451 ) ;
#46355=AXIS2_PLACEMENT_3D ( 'NONE', #28389, #1148, #68841 ) ;
#46357=ORIENTED_EDGE ( 'NONE', *, *, #42984, .T. ) ;
#46363=DIRECTION ( 'NONE',  ( 0.000000000000000000, -1.000000000000000000, 0.000000000000000000 ) ) ;
#46367=CIRCLE ( 'NONE', #65262, 15.99999999999999822 ) ;
#46368=CARTESIAN_POINT ( 'NONE',  ( 103.7078221352084881, -28.31921139840152435, 174.8133722090289552 ) ) ;
#46369=CARTESIAN_POINT ( 'NONE',  ( 95.20909952976953150, -35.71394341709248721, 36.25848241876794731 ) ) ;
#46371=ORIENTED_EDGE ( 'NONE', *, *, #60662, .F. ) ;
#46372=EDGE_CURVE ( 'NONE', #15887, #34773, #13337, .T. ) ;
#46374=VERTEX_POINT ( 'NONE', #85335 ) ;
#46376=ADVANCED_FACE ( 'NONE', ( #844 ), #42160, .F. ) ;
#46377=DIRECTION ( 'NONE',  ( -4.299999999999999979E-14, 1.000000000000000000, -4.400000000000000367E-29 ) ) ;
#46378=EDGE_LOOP ( 'NONE', ( #66871, #14905, #57858, #86862 ) ) ;
#46380=CARTESIAN_POINT ( 'NONE',  ( 177.8371591254543489, -47.82818131005477369, 237.4678068554150059 ) ) ;
#46381=CARTESIAN_POINT ( 'NONE',  ( 107.0664832912739968, -36.72944715994100306, -2.364374724089013391 ) ) ;
#46383=ADVANCED_FACE ( 'NONE', ( #44397 ), #87542, .F. ) ;
#46386=CARTESIAN_POINT ( 'NONE',  ( 104.7307148508592007, -47.55717207929887991, 32.41943479972098174 ) ) ;
#46387=CARTESIAN_POINT ( 'NONE',  ( 118.0344259573852810, -38.43289426264998099, 64.69181575210097890 ) ) ;
#46392=DIRECTION ( 'NONE',  ( 0.000000000000000000, -1.000000000000000000, 0.000000000000000000 ) ) ;
#46393=DIRECTION ( 'NONE',  ( 0.000000000000000000, 0.000000000000000000, -1.000000000000000000 ) ) ;
#46394=AXIS2_PLACEMENT_3D ( 'NONE', #44432, #71285, #1791 ) ;
#46396=EDGE_CURVE ( 'NONE', #80032, #74036, #11226, .T. ) ;
#46399=ORIENTED_EDGE ( 'NONE', *, *, #40986, .F. ) ;
#46400=CARTESIAN_POINT ( 'NONE',  ( 115.6098187009959304, -42.78073513203698042, 53.33562527591095659 ) ) ;
#46401=CARTESIAN_POINT ( 'NONE',  ( 103.3035667682879932, -27.00715593367326406, 211.3699109901969848 ) ) ;
#46402=CARTESIAN_POINT ( 'NONE',  ( 107.2325526940309288, -25.65435679020650639, 76.07657765686298035 ) ) ;
#46403=CARTESIAN_POINT ( 'NONE',  ( 115.7842991311344321, -41.80029728880780482, 173.4030991392274643 ) ) ;
#46404=CARTESIAN_POINT ( 'NONE',  ( 41.56648329127398966, -18.82844715994071194, 198.9256252759119832 ) ) ;
#46405=DIRECTION ( 'NONE',  ( 1.000000000000000078E-15, -1.000000000000000083E-30, -1.000000000000000000 ) ) ;
#46406=EDGE_CURVE ( 'NONE', #22588, #89625, #48235, .T. ) ;
#46410=CARTESIAN_POINT ( 'NONE',  ( 117.2073019650708261, -38.89799087863979565, 104.6708633711489824 ) ) ;
#46414=CARTESIAN_POINT ( 'NONE',  ( 95.31970492887387536, -38.09378048407035777, 232.4184824187679794 ) ) ;
#46415=CARTESIAN_POINT ( 'NONE',  ( 163.1543517358493034, -31.62489322948541215, 342.9256252759109884 ) ) ;
#46416=DIRECTION ( 'NONE',  ( 0.000000000000000000, 0.000000000000000000, 1.000000000000000000 ) ) ;
#46418=CARTESIAN_POINT ( 'NONE',  ( 107.0664832912739399, -36.72944715994095333, 292.6356252759106837 ) ) ;
#46419=CARTESIAN_POINT ( 'NONE',  ( 102.0670549762224226, -27.97049805030057712, 81.48979194111957725 ) ) ;
#46420=EDGE_CURVE ( 'NONE', #3477, #25056, #73008, .T. ) ;
#46421=DIRECTION ( 'NONE',  ( 0.000000000000000000, -1.000000000000000000, 0.000000000000000000 ) ) ;
#46422=DIRECTION ( 'NONE',  ( -4.299999999999999979E-14, 1.000000000000000000, -4.400000000000000367E-29 ) ) ;
#46423=CIRCLE ( 'NONE', #63842, 16.00000000000090239 ) ;
#46425=CARTESIAN_POINT ( 'NONE',  ( 116.4077482568849859, -39.73851878533137238, 158.5784824187689708 ) ) ;
#46426=ORIENTED_EDGE ( 'NONE', *, *, #18105, .T. ) ;
#46428=CARTESIAN_POINT ( 'NONE',  ( 112.9789619575112596, -30.12862337550717484, 110.9272975916109658 ) ) ;
#46429=DIRECTION ( 'NONE',  ( -1.000000000000000000, -4.012088370409549976E-14, 0.000000000000000000 ) ) ;
#46430=CARTESIAN_POINT ( 'NONE',  ( 115.6529839569024602, -41.48189714014871043, 259.4241967044819717 ) ) ;
#46432=LINE ( 'NONE', #4678, #55071 ) ;
#46433=CARTESIAN_POINT ( 'NONE',  ( 141.0667039024479834, -58.35344715994099829, 10.91780685541479734 ) ) ;
#46437=FACE_OUTER_BOUND ( 'NONE', #86997, .T. ) ;
#46439=CARTESIAN_POINT ( 'NONE',  ( 104.5678333644583944, -48.28820816006152938, 182.4070538473399665 ) ) ;
#46440=LINE ( 'NONE', #55036, #57613 ) ;
#46442=EDGE_LOOP ( 'NONE', ( #53992, #28183, #31317, #60550 ) ) ;
#46444=CARTESIAN_POINT ( 'NONE',  ( 82.56634656605380940, -19.87725565068429745, 7.080220459968598945 ) ) ;
#46449=CARTESIAN_POINT ( 'NONE',  ( 163.0664832912739826, -18.82844715994099971, 335.9181252759120184 ) ) ;
#46450=ORIENTED_EDGE ( 'NONE', *, *, #51420, .T. ) ;
#46451=CARTESIAN_POINT ( 'NONE',  ( 108.3318470757233030, -46.73504102216281098, 62.67716460038835891 ) ) ;
#46452=CARTESIAN_POINT ( 'NONE',  ( 114.8141470925876462, -29.70096138442027112, 209.4127681330539872 ) ) ;
#46453=CARTESIAN_POINT ( 'NONE',  ( 134.0664828118826506, -39.47944715903992829, 8.225259175038003079 ) ) ;
#46454=ORIENTED_EDGE ( 'NONE', *, *, #81317, .F. ) ;
#46455=VERTEX_POINT ( 'NONE', #3972 ) ;
#46456=VECTOR ( 'NONE', #54359, 1000.000000000000000 ) ;
#46457=CARTESIAN_POINT ( 'NONE',  ( 25.56670390244829250, -48.82844715994168183, 290.7178068554150059 ) ) ;
#46459=CARTESIAN_POINT ( 'NONE',  ( 100.8872385624251535, -44.70003263212168321, 167.0523370925745326 ) ) ;
#46460=CARTESIAN_POINT ( 'NONE',  ( 109.7980830611816714, -44.45091405062262879, 35.66523322673398155 ) ) ;
#46461=CARTESIAN_POINT ( 'NONE',  ( 113.8576076518026383, -28.74447221003411812, 135.5156252759109634 ) ) ;
#46463=CARTESIAN_POINT ( 'NONE',  ( 134.0664832912740110, -39.47944715994100306, 1.625625275910997480 ) ) ;
#46464=ORIENTED_EDGE ( 'NONE', *, *, #68491, .T. ) ;
#46465=FACE_OUTER_BOUND ( 'NONE', #45237, .T. ) ;
#46467=CARTESIAN_POINT ( 'NONE',  ( 81.60736025278326622, -16.45223222829689647, 7.843813999038339979 ) ) ;
#46468=VERTEX_POINT ( 'NONE', #72578 ) ;
#46469=VECTOR ( 'NONE', #79603, 1000.000000000000000 ) ;
#46474=DIRECTION ( 'NONE',  ( 1.000000000000000000, 3.999999999999999995E-14, 1.000000000000000078E-15 ) ) ;
#46475=EDGE_CURVE ( 'NONE', #39210, #71603, #25302, .T. ) ;
#46476=CARTESIAN_POINT ( 'NONE',  ( 111.8977291718574065, -29.68564172797395528, 44.02099125664899049 ) ) ;
#46477=CARTESIAN_POINT ( 'NONE',  ( 98.53312381531716824, -44.98873235655736380, 191.9384824187679612 ) ) ;
#46478=EDGE_CURVE ( 'NONE', #63468, #82506, #52530, .T. ) ;
#46479=CARTESIAN_POINT ( 'NONE',  ( 105.7232414704440941, -24.98023492732636441, 160.1670538473389627 ) ) ;
#46480=CARTESIAN_POINT ( 'NONE',  ( 99.63323364162300777, -43.45394520487258916, 21.91156745383733195 ) ) ;
#46481=CARTESIAN_POINT ( 'NONE',  ( 105.1675567143510364, -46.98732170830142962, 8.429910990196965770 ) ) ;
#46482=DIRECTION ( 'NONE',  ( -0.02150753337723538411, -0.0009076677972193728959, -0.9997682742251812194 ) ) ;
#46483=DIRECTION ( 'NONE',  ( -0.9999999853157766072, -0.0001713722456126752025, 0.000000000000000000 ) ) ;
#46485=ORIENTED_EDGE ( 'NONE', *, *, #30250, .T. ) ;
#46486=EDGE_CURVE ( 'NONE', #24182, #67326, #37850, .T. ) ;
#46488=CARTESIAN_POINT ( 'NONE',  ( 105.1026693892091117, -26.44596034844076371, 235.2270538473399313 ) ) ;
#46489=EDGE_LOOP ( 'NONE', ( #82615, #87173, #26752, #9051 ) ) ;
#46490=CARTESIAN_POINT ( 'NONE',  ( 96.05373888820416539, -35.78152935435744553, 186.2461014663869889 ) ) ;
#46491=DIRECTION ( 'NONE',  ( 1.000000000000000000, 4.163336342344333240E-14, 0.000000000000000000 ) ) ;
#46492=DIRECTION ( 'NONE',  ( -6.524622321627019585E-16, -4.013151879589939944E-16, -1.000000000000000000 ) ) ;
#46494=CARTESIAN_POINT ( 'NONE',  ( 48.16670390244701139, -28.27351298637280408, 313.9678068554150059 ) ) ;
#46495=CARTESIAN_POINT ( 'NONE',  ( 114.9409439400435531, -39.43770971423924721, 277.6356252759110248 ) ) ;
#46496=CARTESIAN_POINT ( 'NONE',  ( 182.2738106836200132, -23.19206098993950604, -5.074374724088000832 ) ) ;
#46497=CARTESIAN_POINT ( 'NONE',  ( 32.24491389930098251, -32.11662333284611748, -5.074374724088000832 ) ) ;
#46498=PLANE ( 'NONE',  #38133 ) ;
#46500=CIRCLE ( 'NONE', #8811, 1.000000000000000888 ) ;
#46502=CONICAL_SURFACE ( 'NONE', #61039, 5.800000000000000711, 0.7853981633974476129 ) ;
#46504=CARTESIAN_POINT ( 'NONE',  ( 83.56670390244801183, -39.24694715994107952, 239.5838068554169809 ) ) ;
#46505=CARTESIAN_POINT ( 'NONE',  ( 45.77381068356854144, -48.62134037881681081, 129.9678068554150911 ) ) ;
#46506=EDGE_CURVE ( 'NONE', #34812, #12195, #40943, .T. ) ;
#46508=ORIENTED_EDGE ( 'NONE', *, *, #40970, .F. ) ;
#46510=CARTESIAN_POINT ( 'NONE',  ( 117.7991783922927738, -31.64581934375353711, 214.1784824187679419 ) ) ;
#46511=CARTESIAN_POINT ( 'NONE',  ( 110.1579320793587442, -46.68562272277494429, 93.81562527591097478 ) ) ;
#46512=CARTESIAN_POINT ( 'NONE',  ( 96.63877784842330243, -35.80427747552585060, 227.2556252759109725 ) ) ;
#46513=CYLINDRICAL_SURFACE ( 'NONE', #7743, 2.500000000000002220 ) ;
#46514=DIRECTION ( 'NONE',  ( 0.7071067811865779928, -0.7071067811865171526, 7.071067811865475333E-16 ) ) ;
#46516=CARTESIAN_POINT ( 'NONE',  ( 172.5664832912729878, -18.82844715994071194, 258.9256252759120116 ) ) ;
#46517=DIRECTION ( 'NONE',  ( 0.0001713722455994027248, -0.9999999853157766072, 0.000000000000000000 ) ) ;
#46518=DIRECTION ( 'NONE',  ( -1.000000000000000078E-15, 1.000000000000000083E-30, 1.000000000000000000 ) ) ;
#46521=B_SPLINE_CURVE_WITH_KNOTS ( 'NONE', 3,
 ( #15641, #50584, #37864, #78324, #51034, #16089, #64674, #43770, #43315, #71060, #36073, #71505, #9266, #56948, #64232, #8833, #65562, #71943 ),
 .UNSPECIFIED., .F., .F.,
 ( 4, 2, 2, 2, 2, 2, 2, 2, 4 ),
 ( 0.4999608178654283974, 0.5624657156322498963, 0.6249706133990713397, 0.6874755111658927831, 0.7499804089327142265, 0.8124853066995356698, 0.8749902044663571132, 0.9374951022331785566, 1.000000000000000000 ),
 .UNSPECIFIED. ) ;
#46522=ORIENTED_EDGE ( 'NONE', *, *, #45745, .F. ) ;
#46525=CARTESIAN_POINT ( 'NONE',  ( 112.9548150380649503, -42.91681406074877003, 157.6038483995049830 ) ) ;
#46527=ORIENTED_EDGE ( 'NONE', *, *, #57624, .T. ) ;
#46529=CARTESIAN_POINT ( 'NONE',  ( 98.47671751366520709, -30.86049585540216711, 116.8499109901969604 ) ) ;
#46530=DIRECTION ( 'NONE',  ( -0.0001211784769825758164, 0.7071067708032326982, -0.7071067811865484609 ) ) ;
#46533=AXIS2_PLACEMENT_3D ( 'NONE', #76153, #40728, #19400 ) ;
#46535=CARTESIAN_POINT ( 'NONE',  ( 101.9936209472876527, -45.44607154236431512, 108.1564586098271405 ) ) ;
#46537=CARTESIAN_POINT ( 'NONE',  ( 101.3196941207356758, -46.24713579373447914, 52.14419670448295108 ) ) ;
#46539=ORIENTED_EDGE ( 'NONE', *, *, #60042, .F. ) ;
#46540=AXIS2_PLACEMENT_3D ( 'NONE', #55766, #46731, #74460 ) ;
#46541=ORIENTED_EDGE ( 'NONE', *, *, #80285, .F. ) ;
#46542=LINE ( 'NONE', #74277, #794 ) ;
#46543=CARTESIAN_POINT ( 'NONE',  ( 117.1372161989436904, -34.25576096370540569, 160.0061014663869798 ) ) ;
#46544=CARTESIAN_POINT ( 'NONE',  ( 125.9611475301394847, -58.72944715994102438, 249.5838068554163840 ) ) ;
#46546=CARTESIAN_POINT ( 'NONE',  ( 172.5664832912740110, -18.82844715994099971, 318.9256252759120116 ) ) ;
#46548=PLANE ( 'NONE',  #83755 ) ;
#46549=CARTESIAN_POINT ( 'NONE',  ( 75.31670390244798341, -50.82844715994100682, 86.31780685541500020 ) ) ;
#46550=CARTESIAN_POINT ( 'NONE',  ( 104.4079121328872617, -46.45803387014570518, 178.3647764060284260 ) ) ;
#46551=CARTESIAN_POINT ( 'NONE',  ( 98.11562048848810491, -31.42749274529980852, 85.90133956162493689 ) ) ;
#46552=VERTEX_POINT ( 'NONE', #55228 ) ;
#46554=VERTEX_POINT ( 'NONE', #12585 ) ;
#46556=LINE ( 'NONE', #13407, #6763 ) ;
#46559=CARTESIAN_POINT ( 'NONE',  ( 112.8577109034250583, -30.29807625619018197, 157.3233284648299559 ) ) ;
#46562=ORIENTED_EDGE ( 'NONE', *, *, #85955, .F. ) ;
#46563=VERTEX_POINT ( 'NONE', #60710 ) ;
#46564=LINE ( 'NONE', #59307, #20673 ) ;
#46567=ORIENTED_EDGE ( 'NONE', *, *, #55124, .F. ) ;
#46568=CARTESIAN_POINT ( 'NONE',  ( 182.4202572930267934, -31.94127993907054019, 193.9678068554150059 ) ) ;
#46569=CARTESIAN_POINT ( 'NONE',  ( 112.2422220273998477, -28.08754728269216372, 201.0787261630399598 ) ) ;
#46570=DIRECTION ( 'NONE',  ( -1.000000000000000000, -1.000000000000000078E-15, -1.000000000000000078E-15 ) ) ;
#46573=FACE_OUTER_BOUND ( 'NONE', #27914, .T. ) ;
#46577=ORIENTED_EDGE ( 'NONE', *, *, #75449, .T. ) ;
#46579=EDGE_CURVE ( 'NONE', #34067, #60619, #20303, .T. ) ;
#46580=CARTESIAN_POINT ( 'NONE',  ( 98.93571844094823575, -36.00806725600566693, 229.0738046553059633 ) ) ;
#46581=CARTESIAN_POINT ( 'NONE',  ( 113.8708677755033847, -44.65703921284106315, 108.1413395616249744 ) ) ;
#46582=EDGE_CURVE ( 'NONE', #25046, #39094, #26648, .T. ) ;
#46583=CARTESIAN_POINT ( 'NONE',  ( 100.3128846869252726, -46.43702735306955276, 87.09276813305393716 ) ) ;
#46584=CARTESIAN_POINT ( 'NONE',  ( 100.4600951037162559, -41.26014358730922282, 249.5838068554172082 ) ) ;
#46585=PRODUCT_DEFINITION_SHAPE ( 'NONE', 'NONE',  #68346 ) ;
#46586=CARTESIAN_POINT ( 'NONE',  ( 117.7221270036566807, -41.68118999199129604, 4.925625275910981316 ) ) ;
#46588=CARTESIAN_POINT ( 'NONE',  ( 114.9778481211559154, -29.01036126763497336, 190.4537205140059655 ) ) ;
#46589=CARTESIAN_POINT ( 'NONE',  ( 103.6782606442165360, -46.19611297174933640, 277.3022125101787765 ) ) ;
#46590=ORIENTED_EDGE ( 'NONE', *, *, #26557, .F. ) ;
#46591=DIRECTION ( 'NONE',  ( 3.999999999999999995E-14, -1.000000000000000000, 4.100000000000000342E-29 ) ) ;
#46592=ORIENTED_EDGE ( 'NONE', *, *, #53863, .F. ) ;
#46593=AXIS2_PLACEMENT_3D ( 'NONE', #56042, #76060, #13839 ) ;
#46600=EDGE_CURVE ( 'NONE', #50719, #87253, #33464, .T. ) ;
#46602=CARTESIAN_POINT ( 'NONE',  ( 98.14942788562998999, -43.26130833009477783, 106.8175300378159704 ) ) ;
#46604=CARTESIAN_POINT ( 'NONE',  ( 168.0371591254543375, -48.62818131005519717, 300.4678068554149490 ) ) ;
#46605=CARTESIAN_POINT ( 'NONE',  ( 181.8884939055948280, -32.11662333283959470, 193.9678068554150059 ) ) ;
#46606=LINE ( 'NONE', #5752, #65043 ) ;
#46608=CARTESIAN_POINT ( 'NONE',  ( 96.07698540226633099, -35.78353028925530310, 182.2461014663869889 ) ) ;
#46609=CARTESIAN_POINT ( 'NONE',  ( 89.06648329127401098, -14.47844715994100007, 17.92562527591199739 ) ) ;
#46610=LINE ( 'NONE', #33447, #56929 ) ;
#46611=ADVANCED_FACE ( 'NONE', ( #76141 ), #34354, .F. ) ;
#46613=AXIS2_PLACEMENT_3D ( 'NONE', #83836, #21611, #15692 ) ;
#46615=CARTESIAN_POINT ( 'NONE',  ( 138.8167039024479834, -67.87844715994100397, 60.91780685541480267 ) ) ;
#46616=CYLINDRICAL_SURFACE ( 'NONE', #67649, 0.9999999999999800160 ) ;
#46618=CARTESIAN_POINT ( 'NONE',  ( 80.06648329127399677, 0.2215528400590013880, 293.6356252759119911 ) ) ;
#46619=CARTESIAN_POINT ( 'NONE',  ( 98.86425576617398292, -29.25038657358478744, 230.7261014663869503 ) ) ;
#46620=ORIENTED_EDGE ( 'NONE', *, *, #68942, .T. ) ;
#46621=DIRECTION ( 'NONE',  ( 1.000000000000000000, 8.673617379883546378E-16, 9.757819552368989676E-16 ) ) ;
#46622=CARTESIAN_POINT ( 'NONE',  ( 111.8740745592753427, -46.04428811464656945, 268.9556252759110180 ) ) ;
#46623=CARTESIAN_POINT ( 'NONE',  ( 98.42274642353920910, -30.82362014679692308, 116.8499109901969604 ) ) ;
#46625=CARTESIAN_POINT ( 'NONE',  ( 82.81648064515525220, -36.72944715939136273, 6.749772901088423538 ) ) ;
#46628=CARTESIAN_POINT ( 'NONE',  ( 193.0371591254585155, -47.82818131005411999, 180.4678068554150343 ) ) ;
#46629=CARTESIAN_POINT ( 'NONE',  ( 73.06648329127396835, -8.729447159941065237, 14.67562527591093513 ) ) ;
#46630=ORIENTED_EDGE ( 'NONE', *, *, #88097, .T. ) ;
#46634=ORIENTED_EDGE ( 'NONE', *, *, #80806, .T. ) ;
#46635=CARTESIAN_POINT ( 'NONE',  ( 107.0664832912739541, -23.72944715994095688, 312.6356252759112522 ) ) ;
#46636=CARTESIAN_POINT ( 'NONE',  ( 96.73636544059199593, -37.96124694896865748, 37.42133956162496844 ) ) ;
#46641=DIRECTION ( 'NONE',  ( 0.000000000000000000, 1.000000000000000000, 0.000000000000000000 ) ) ;
#46644=CARTESIAN_POINT ( 'NONE',  ( 98.63544605819593869, -40.03554478408833006, 246.0343245899819919 ) ) ;
#46648=CIRCLE ( 'NONE', #74225, 9.999999999999994671 ) ;
#46649=DIRECTION ( 'NONE',  ( 0.000000000000000000, 0.000000000000000000, -1.000000000000000000 ) ) ;
#46650=PLANE ( 'NONE',  #49131 ) ;
#46652=DIRECTION ( 'NONE',  ( 0.000000000000000000, 1.000000000000000000, 0.000000000000000000 ) ) ;
#46653=CARTESIAN_POINT ( 'NONE',  ( 142.8832909413445122, -79.11588146349311046, 361.9756252759100335 ) ) ;
#46654=CARTESIAN_POINT ( 'NONE',  ( 115.3146942856800337, -32.23016485065021897, 20.64348806780197521 ) ) ;
#46656=CARTESIAN_POINT ( 'NONE',  ( 102.0657545461937161, -27.97126071411138781, 175.4899107057300967 ) ) ;
#46657=CARTESIAN_POINT ( 'NONE',  ( 101.4562478665867928, -44.74122718545263666, 282.0899109901972110 ) ) ;
#46661=CARTESIAN_POINT ( 'NONE',  ( 113.6361143365868429, -29.10761691970661857, 55.51073420584606311 ) ) ;
#46662=CYLINDRICAL_SURFACE ( 'NONE', #14868, 2.517500000000005844 ) ;
#46663=CARTESIAN_POINT ( 'NONE',  ( 109.7980830611816714, -44.45091405062262879, 35.66523322673398155 ) ) ;
#46664=AXIS2_PLACEMENT_3D ( 'NONE', #20623, #73790, #21067 ) ;
#46665=VECTOR ( 'NONE', #85391, 1000.000000000000000 ) ;
#46666=EDGE_CURVE ( 'NONE', #1484, #19859, #41605, .T. ) ;
#46667=CARTESIAN_POINT ( 'NONE',  ( 135.5773992616618671, -16.43204134599573507, 7.859568798194228378 ) ) ;
#46668=CARTESIAN_POINT ( 'NONE',  ( 25.56670390244797275, -48.82844715994099971, 137.2178068554150059 ) ) ;
#46670=CARTESIAN_POINT ( 'NONE',  ( 19.56648329127400032, 15.62155284005900491, 323.8756252759109202 ) ) ;
#46671=EDGE_LOOP ( 'NONE', ( #46508, #11430, #41127, #45537 ) ) ;
#46673=CARTESIAN_POINT ( 'NONE',  ( 152.0371591254583450, -47.82818131005588214, 249.9678068554149490 ) ) ;
#46674=ORIENTED_EDGE ( 'NONE', *, *, #83021, .T. ) ;
#46675=CARTESIAN_POINT ( 'NONE',  ( 104.9628152733504720, -25.06689740840304381, 125.2184824187689856 ) ) ;
#46677=CARTESIAN_POINT ( 'NONE',  ( 113.7853715510712789, -42.80144937323932908, 82.67622935188595079 ) ) ;
#46680=CARTESIAN_POINT ( 'NONE',  ( 98.97073112826979013, -33.12568863208839076, 97.42444044875497866 ) ) ;
#46681=AXIS2_PLACEMENT_3D ( 'NONE', #10285, #22591, #71633 ) ;
#46683=FACE_OUTER_BOUND ( 'NONE', #41008, .T. ) ;
#46684=CARTESIAN_POINT ( 'NONE',  ( 100.9304087016431453, -28.27451679452656919, 71.57562527591099411 ) ) ;
#46685=LINE ( 'NONE', #70171, #41041 ) ;
#46686=CARTESIAN_POINT ( 'NONE',  ( 105.7153411597131765, -46.72383786517413284, 257.4688385543852291 ) ) ;
#46689=ORIENTED_EDGE ( 'NONE', *, *, #55239, .T. ) ;
#46690=EDGE_LOOP ( 'NONE', ( #29051, #38937, #80690, #9912, #55844, #33924, #47490, #36635, #4562, #28742, #84390, #88096 ) ) ;
#46691=EDGE_CURVE ( 'NONE', #71543, #84928, #81196, .T. ) ;
#46694=CARTESIAN_POINT ( 'NONE',  ( 103.3362402991319442, -47.20309360805218546, 252.3041967044827913 ) ) ;
#46695=DIRECTION ( 'NONE',  ( 0.000000000000000000, 0.000000000000000000, 1.000000000000000000 ) ) ;
#46697=ADVANCED_FACE ( 'NONE', ( #60262 ), #67992, .T. ) ;
#46698=CARTESIAN_POINT ( 'NONE',  ( 101.1417250294410337, -28.10862513908322313, 46.55562527591094835 ) ) ;
#46699=CARTESIAN_POINT ( 'NONE',  ( 105.8025202575843764, -26.72362734506296889, 96.17630429063157749 ) ) ;
#46700=EDGE_LOOP ( 'NONE', ( #69833, #20570, #78429, #22563 ) ) ;
#46701=CARTESIAN_POINT ( 'NONE',  ( 116.3225472244029817, -32.94146556017791738, 114.1356252759109822 ) ) ;
#46702=EDGE_CURVE ( 'NONE', #32451, #40665, #88447, .T. ) ;
#46703=DIRECTION ( 'NONE',  ( -4.237773401492740281E-14, 1.000000000000000000, 0.000000000000000000 ) ) ;
#46704=VECTOR ( 'NONE', #27203, 1000.000000000000000 ) ;
#46709=CARTESIAN_POINT ( 'NONE',  ( 96.27200394136420414, -34.46162041542910970, 261.1737205140064475 ) ) ;
#46710=DIRECTION ( 'NONE',  ( 0.000000000000000000, 0.000000000000000000, 1.000000000000000000 ) ) ;
#46711=DIRECTION ( 'NONE',  ( 0.000000000000000000, 1.000000000000000000, 0.000000000000000000 ) ) ;
#46713=CARTESIAN_POINT ( 'NONE',  ( 113.6113952709150396, -31.24125447920927101, 268.8038483995053411 ) ) ;
#46714=CARTESIAN_POINT ( 'NONE',  ( 97.57298764950955672, -39.87469497683259334, 101.5815513261982943 ) ) ;
#46715=CARTESIAN_POINT ( 'NONE',  ( 117.3497117099303892, -32.73958051198275854, 90.10895860924395606 ) ) ;
#46716=CARTESIAN_POINT ( 'NONE',  ( 41.56648329127499153, -36.32844715994070839, 198.9256252759119832 ) ) ;
#46717=CARTESIAN_POINT ( 'NONE',  ( 114.4941961175866254, -28.48069933791915531, 159.5051490854349652 ) ) ;
#46718=EDGE_LOOP ( 'NONE', ( #43841, #69279, #12330, #70194 ) ) ;
#46719=CARTESIAN_POINT ( 'NONE',  ( 123.6837132603318992, -20.11243780205710507, 239.5838068554165545 ) ) ;
#46720=EDGE_CURVE ( 'NONE', #3377, #31900, #18914, .T. ) ;
#46721=EDGE_LOOP ( 'NONE', ( #88206, #75069, #40202, #51385, #9499, #6598, #55470, #64052, #50138, #79328, #78804, #70692 ) ) ;
#46722=FACE_BOUND ( 'NONE', #64041, .T. ) ;
#46723=CARTESIAN_POINT ( 'NONE',  ( 123.6837132603318992, -16.81243780205710436, 239.5838068554165545 ) ) ;
#46725=CARTESIAN_POINT ( 'NONE',  ( 134.9467300988904128, -34.12360705087674972, 1.744847597651338678 ) ) ;
#46729=CARTESIAN_POINT ( 'NONE',  ( 108.2829496674670224, -47.76277978039057359, 157.6518157521019532 ) ) ;
#46731=DIRECTION ( 'NONE',  ( -1.000000000000000000, -4.554376769437570034E-14, 0.000000000000000000 ) ) ;
#46734=FACE_OUTER_BOUND ( 'NONE', #65424, .T. ) ;
#46735=VERTEX_POINT ( 'NONE', #19394 ) ;
#46737=FACE_OUTER_BOUND ( 'NONE', #15166, .T. ) ;
#46739=VERTEX_POINT ( 'NONE', #21652 ) ;
#46741=VERTEX_POINT ( 'NONE', #7115 ) ;
#46744=CARTESIAN_POINT ( 'NONE',  ( 118.5256205435843526, -36.72944715994100306, 293.2242906452868851 ) ) ;
#46746=DIRECTION ( 'NONE',  ( -0.7071067811865483499, -0.7071067811865466846, -7.071067811865491110E-16 ) ) ;
#46748=DIRECTION ( 'NONE',  ( 0.3818493186865919986, -0.9242245927363031965, 0.000000000000000000 ) ) ;
#46749=VERTEX_POINT ( 'NONE', #29355 ) ;
#46751=CARTESIAN_POINT ( 'NONE',  ( 134.0664832912739826, -18.72944715994100306, 14.92562527591099908 ) ) ;
#46752=EDGE_CURVE ( 'NONE', #70284, #63079, #34806, .T. ) ;
#46753=CARTESIAN_POINT ( 'NONE',  ( 99.07755742602716964, -44.46178485432842109, 187.9384824187679612 ) ) ;
#46755=ORIENTED_EDGE ( 'NONE', *, *, #23777, .F. ) ;
#46756=CARTESIAN_POINT ( 'NONE',  ( 97.35459460924926134, -38.14118110200429612, 62.44133956162495025 ) ) ;
#46757=FACE_OUTER_BOUND ( 'NONE', #2383, .T. ) ;
#46759=LINE ( 'NONE', #45417, #47453 ) ;
#46764=CARTESIAN_POINT ( 'NONE',  ( 101.6018043438793796, -28.26729678577900273, 216.9644404487539475 ) ) ;
#46765=VECTOR ( 'NONE', #81366, 1000.000000000000000 ) ;
#46766=CARTESIAN_POINT ( 'NONE',  ( 97.92313387223457255, -40.78048155489533144, 52.65794466837188992 ) ) ;
#46767=EDGE_CURVE ( 'NONE', #31965, #81124, #16173, .T. ) ;
#46769=CARTESIAN_POINT ( 'NONE',  ( 115.0372574776238110, -42.90846260514542365, 154.3022919387951220 ) ) ;
#46770=CARTESIAN_POINT ( 'NONE',  ( 82.68803181460157248, -37.56139158947667056, 2.921136715972031617 ) ) ;
#46771=ORIENTED_EDGE ( 'NONE', *, *, #72453, .F. ) ;
#46772=LINE ( 'NONE', #39530, #23294 ) ;
#46774=ORIENTED_EDGE ( 'NONE', *, *, #50957, .F. ) ;
#46775=CARTESIAN_POINT ( 'NONE',  ( 97.48652011608379553, -32.61680585812226241, 16.00419670448194154 ) ) ;
#46776=ORIENTED_EDGE ( 'NONE', *, *, #30740, .T. ) ;
#46778=CARTESIAN_POINT ( 'NONE',  ( 106.4091095994060652, -45.35897697767001091, 265.3461856076867207 ) ) ;
#46779=VECTOR ( 'NONE', #41984, 1000.000000000000000 ) ;
#46781=FACE_BOUND ( 'NONE', #45847, .T. ) ;
#46782=CARTESIAN_POINT ( 'NONE',  ( 99.59366209610195142, -44.96145431533982162, 156.9899109901969609 ) ) ;
#46786=CARTESIAN_POINT ( 'NONE',  ( 115.9970180223098311, -30.13831313182449989, 255.3203871806730660 ) ) ;
#46788=EDGE_LOOP ( 'NONE', ( #63588, #66112 ) ) ;
#46789=AXIS2_PLACEMENT_3D ( 'NONE', #66041, #3830, #31523 ) ;
#46790=CARTESIAN_POINT ( 'NONE',  ( 97.22547384517952196, -31.59602418489684084, 86.93181575210095957 ) ) ;
#46791=DIRECTION ( 'NONE',  ( 1.000000000000000000, -1.000000000000000078E-15, 0.000000000000000000 ) ) ;
#46793=EDGE_LOOP ( 'NONE', ( #70121, #15419, #34927, #20320 ) ) ;
#46795=ORIENTED_EDGE ( 'NONE', *, *, #13956, .F. ) ;
#46796=DIRECTION ( 'NONE',  ( -0.7071067811865462405, 0.000000000000000000, 0.7071067811865486830 ) ) ;
#46797=CARTESIAN_POINT ( 'NONE',  ( 41.56648329127499153, -32.07844715994070839, 78.92562527591199739 ) ) ;
#46800=CARTESIAN_POINT ( 'NONE',  ( 103.3443811052163568, -28.91619688769685936, 138.2604713219729717 ) ) ;
#46801=CARTESIAN_POINT ( 'NONE',  ( 111.1359251431956210, -27.10775802199072970, 240.7584824187679544 ) ) ;
#46805=DIRECTION ( 'NONE',  ( 0.000000000000000000, 1.000000000000000000, 0.000000000000000000 ) ) ;
#46807=EDGE_LOOP ( 'NONE', ( #49826, #946, #44135, #29452 ) ) ;
#46808=FACE_OUTER_BOUND ( 'NONE', #85580, .T. ) ;
#46811=CARTESIAN_POINT ( 'NONE',  ( 107.0664832912739399, -36.72944715994095333, 289.6356252759107406 ) ) ;
#46812=DIRECTION ( 'NONE',  ( 0.000000000000000000, 0.000000000000000000, 1.000000000000000000 ) ) ;
#46813=LINE ( 'NONE', #86843, #75088 ) ;
#46814=CARTESIAN_POINT ( 'NONE',  ( 99.46962827726154899, -41.65933777599243371, 146.2190864947439763 ) ) ;
#46815=CARTESIAN_POINT ( 'NONE',  ( 117.4985906579250354, -37.96351766657803495, 53.73276813305394484 ) ) ;
#46819=VECTOR ( 'NONE', #67888, 1000.000000000000000 ) ;
#46820=EDGE_CURVE ( 'NONE', #15124, #51994, #84333, .T. ) ;
#46821=LINE ( 'NONE', #73651, #15115 ) ;
#46822=ORIENTED_EDGE ( 'NONE', *, *, #15090, .T. ) ;
#46823=EDGE_CURVE ( 'NONE', #26639, #13679, #48864, .T. ) ;
#46824=DIRECTION ( 'NONE',  ( 0.000000000000000000, 0.000000000000000000, -1.000000000000000000 ) ) ;
#46832=ORIENTED_EDGE ( 'NONE', *, *, #48267, .F. ) ;
#46833=CARTESIAN_POINT ( 'NONE',  ( 99.12668881670464316, -43.51958910750428089, 31.88991099019594699 ) ) ;
#46834=CARTESIAN_POINT ( 'NONE',  ( 97.77052560236188583, -29.30002703792375485, 41.78991099019596334 ) ) ;
#46838=CARTESIAN_POINT ( 'NONE',  ( 109.7248794765007602, -27.00080882144429140, 145.8651687245758808 ) ) ;
#46839=DIRECTION ( 'NONE',  ( 1.000000000000000000, 0.000000000000000000, 0.000000000000000000 ) ) ;
#46840=DIRECTION ( 'NONE',  ( 0.000000000000000000, 1.000000000000000000, 1.914177628664063178E-15 ) ) ;
#46843=CARTESIAN_POINT ( 'NONE',  ( 118.1222316836501705, -37.72106760768119216, 33.74324432352998571 ) ) ;
#46844=CARTESIAN_POINT ( 'NONE',  ( 117.9485099285917613, -34.79154191225799053, 194.9546728949589749 ) ) ;
#46845=CARTESIAN_POINT ( 'NONE',  ( 106.8407189164991706, -48.60257990303799858, 73.56133956162497611 ) ) ;
#46846=CARTESIAN_POINT ( 'NONE',  ( 98.54792498091607911, -41.97742571765204644, 171.7652816990279234 ) ) ;
#46847=CARTESIAN_POINT ( 'NONE',  ( 126.8164832912740110, -46.47944715994101017, 14.92562527591099020 ) ) ;
#46849=VECTOR ( 'NONE', #49408, 1000.000000000000000 ) ;
#46850=AXIS2_PLACEMENT_3D ( 'NONE', #65927, #18683, #24608 ) ;
#46851=PLANE ( 'NONE',  #63623 ) ;
#46853=EDGE_CURVE ( 'NONE', #24378, #81580, #42952, .T. ) ;
#46854=CARTESIAN_POINT ( 'NONE',  ( 116.0091996907507195, -30.12340400999218559, 105.3327681330529515 ) ) ;
#46856=ORIENTED_EDGE ( 'NONE', *, *, #14554, .T. ) ;
#46857=CARTESIAN_POINT ( 'NONE',  ( 96.79426660377265534, -34.87310936442968057, 237.1841967044819626 ) ) ;
#46858=CARTESIAN_POINT ( 'NONE',  ( 112.0651709148995678, -45.48882515156851269, 253.9919150860570198 ) ) ;
#46860=DIRECTION ( 'NONE',  ( 1.000000000000000000, 6.831565154159360295E-14, 0.000000000000000000 ) ) ;
#46861=CARTESIAN_POINT ( 'NONE',  ( 109.7248659154506640, -27.00080517803650437, 45.86479194305611884 ) ) ;
#46862=CARTESIAN_POINT ( 'NONE',  ( 131.9645448811542678, -38.51222316632535581, 2.376608873922943843 ) ) ;
#46864=CARTESIAN_POINT ( 'NONE',  ( 107.9488082096507213, -26.98745991040259895, 155.0041967044829505 ) ) ;
#46866=ORIENTED_EDGE ( 'NONE', *, *, #74131, .F. ) ;
#46867=CARTESIAN_POINT ( 'NONE',  ( 108.4917517584632236, -27.44263408611272936, 141.3749166392299514 ) ) ;
#46868=CARTESIAN_POINT ( 'NONE',  ( 142.8696205427243626, 0.6543191929522240713, 540.9756252759101471 ) ) ;
#46870=CARTESIAN_POINT ( 'NONE',  ( 116.0161715043949471, -40.67488961668902192, 249.4956252759109532 ) ) ;
#46871=FACE_OUTER_BOUND ( 'NONE', #32994, .T. ) ;
#46872=AXIS2_PLACEMENT_3D ( 'NONE', #57711, #64979, #52206 ) ;
#46876=EDGE_CURVE ( 'NONE', #65403, #27030, #77495, .T. ) ;
#46879=CARTESIAN_POINT ( 'NONE',  ( 162.8913605087219878, -31.76306994223740432, 342.9256252759109884 ) ) ;
#46880=CARTESIAN_POINT ( 'NONE',  ( 21.03689327557619748, -23.42844715994197813, 129.9678068554150627 ) ) ;
#46881=CARTESIAN_POINT ( 'NONE',  ( 101.2129617469312564, -45.32973500739964834, 197.1013395616249966 ) ) ;
#46882=CARTESIAN_POINT ( 'NONE',  ( 107.0664832912739399, -36.72944715994095333, 302.7856252759109452 ) ) ;
#46883=ORIENTED_EDGE ( 'NONE', *, *, #49820, .F. ) ;
#46888=CARTESIAN_POINT ( 'NONE',  ( 82.10313645208317723, -20.57950990142240144, 7.523361336364036589 ) ) ;
#46889=CARTESIAN_POINT ( 'NONE',  ( 112.1401101529673667, -28.01326083308519088, 184.6568239736689350 ) ) ;
#46890=DIRECTION ( 'NONE',  ( -1.000000000000000000, -3.999999999999999995E-14, -1.000000000000000078E-15 ) ) ;
#46891=B_SPLINE_CURVE_WITH_KNOTS ( 'NONE', 3,
 ( #17903, #74664, #73313, #38793, #61026, #66499, #67850, #88755, #54185, #71541, #77903, #77447, #44696, #8872, #64271, #17013, #36569, #50623, #78365, #71981, #2045, #29752, #43806, #78807, #15681, #56990, #22492, #30194, #84283, #57890, #37898, #22056, #65598, #57437, #29307, #16563, #9750, #85178, #72424, #50167, #31070, #44245, #43354, #30636, #10191, #22949, #71098, #16126, #65152, #37452, #3379, #9305 ),
 .UNSPECIFIED., .F., .F.,
 ( 4, 2, 1, 1, 1, 1, 1, 1, 2, 2, 2, 2, 2, 2, 2, 2, 1, 1, 1, 1, 1, 1, 2, 2, 2, 2, 2, 2, 2, 2, 2, 4 ),
 ( 0.5000152423139874180, 0.5001779712831790903, 0.5003407002523706515, 0.5006661581907546621, 0.5013170740675219061, 0.5026189058210562832, 0.5052225693281247043, 0.5104298963422607693, 0.5208445503705330104, 0.5416738584270778256, 0.5833324745401682332, 0.6666497067663494924, 0.7499669389925306406, 0.8332841712187117889, 0.8333655357033079580, 0.8334469001879041272, 0.8335282646725001854, 0.8336909936415386468, 0.8340164515796154587, 0.8346673674557795186, 0.8359691992081024203, 0.8385728627127363444, 0.8437801897220043035, 0.8541948437405375572, 0.8750241517776036204, 0.8958534598146696837, 0.9166827678517357469, 0.9375120758888018102, 0.9583413839258678735, 0.9791706919629339367, 0.9895853459814669684, 1.000000000000000000 ),
 .UNSPECIFIED. ) ;
#46893=AXIS2_PLACEMENT_3D ( 'NONE', #12193, #87162, #81698 ) ;
#46895=ORIENTED_EDGE ( 'NONE', *, *, #29298, .T. ) ;
#46896=CARTESIAN_POINT ( 'NONE',  ( 172.5664832912740110, -18.82844715994099971, 78.92562527591199739 ) ) ;
#46897=EDGE_CURVE ( 'NONE', #50846, #21614, #1654, .T. ) ;
#46898=CARTESIAN_POINT ( 'NONE',  ( 96.19116125691978425, -32.02117184027007113, 211.0013395616249738 ) ) ;
#46899=CARTESIAN_POINT ( 'NONE',  ( 136.7895896102205597, -37.11755991741181759, 6.789748280180922357 ) ) ;
#46901=CARTESIAN_POINT ( 'NONE',  ( 168.5667039024486087, -48.82844715993516616, 129.9678068554150059 ) ) ;
#46902=EDGE_CURVE ( 'NONE', #61996, #48953, #86995, .T. ) ;
#46903=DIRECTION ( 'NONE',  ( 0.000000000000000000, 0.000000000000000000, 1.000000000000000000 ) ) ;
#46905=EDGE_CURVE ( 'NONE', #5529, #59590, #72471, .T. ) ;
#46906=CARTESIAN_POINT ( 'NONE',  ( 100.8503319422675020, -42.75110701849109063, 39.76904275054393878 ) ) ;
#46907=CARTESIAN_POINT ( 'NONE',  ( 114.0955628336689500, -44.50577255156974843, 129.1613395616249704 ) ) ;
#46910=CYLINDRICAL_SURFACE ( 'NONE', #68254, 9.999999999999998224 ) ;
#46911=CARTESIAN_POINT ( 'NONE',  ( 63.03715912545732181, -24.89890238295017966, 300.4678068554150627 ) ) ;
#46912=ORIENTED_EDGE ( 'NONE', *, *, #86638, .F. ) ;
#46914=VECTOR ( 'NONE', #22522, 1000.000000000000000 ) ;
#46918=CARTESIAN_POINT ( 'NONE',  ( 97.31589304778225369, -39.30609602821265725, 157.5312681354445488 ) ) ;
#46920=CARTESIAN_POINT ( 'NONE',  ( 110.1208792074641991, -44.70608788829420632, 62.28956268521896078 ) ) ;
#46921=CARTESIAN_POINT ( 'NONE',  ( 103.8128537583787363, -48.15082670742215498, 217.3556252759109668 ) ) ;
#46922=CARTESIAN_POINT ( 'NONE',  ( 117.2701380961606645, -34.52720868313122082, 183.9956252759109532 ) ) ;
#46923=CARTESIAN_POINT ( 'NONE',  ( 115.9905926440153792, -41.41586665309425541, 23.44146406657679194 ) ) ;
#46924=CARTESIAN_POINT ( 'NONE',  ( 110.9930042498355363, -46.38681234365495953, 278.8841967044824059 ) ) ;
#46927=CARTESIAN_POINT ( 'NONE',  ( 192.5667039024472444, -23.42844715993434335, 300.4678068554149490 ) ) ;
#46928=ORIENTED_EDGE ( 'NONE', *, *, #347, .F. ) ;
#46929=ADVANCED_FACE ( 'NONE', ( #45181 ), #71588, .T. ) ;
#46931=EDGE_CURVE ( 'NONE', #79308, #46344, #52751, .T. ) ;
#46932=CYLINDRICAL_SURFACE ( 'NONE', #51630, 0.2500000000000039968 ) ;
#46933=CARTESIAN_POINT ( 'NONE',  ( 96.07878916947804271, -35.15354693665655361, 226.2251490854349640 ) ) ;
#46934=CIRCLE ( 'NONE', #77446, 10.04999999999999361 ) ;
#46936=CARTESIAN_POINT ( 'NONE',  ( 96.04647588134957914, -35.87007288833441976, 191.2765776568629690 ) ) ;
#46937=CARTESIAN_POINT ( 'NONE',  ( 52.65249034007830176, -49.32844715994059470, 300.4678068554150059 ) ) ;
#46940=CARTESIAN_POINT ( 'NONE',  ( 97.81171347387959258, -40.51745984142272761, 22.63530404563221410 ) ) ;
#46941=CARTESIAN_POINT ( 'NONE',  ( 116.3214877775586018, -32.94188667902410117, 30.13562527591096085 ) ) ;
#46942=CARTESIAN_POINT ( 'NONE',  ( 103.9608317090438874, -29.20111914701857714, 277.6356252759112522 ) ) ;
#46943=CARTESIAN_POINT ( 'NONE',  ( 48.45959712127301344, -26.00627455219131789, -5.074374724088000832 ) ) ;
#46944=CARTESIAN_POINT ( 'NONE',  ( 108.3332299252464708, -46.73488901547833763, 173.6772747286529750 ) ) ;
#46946=DIRECTION ( 'NONE',  ( 0.7071067811865692221, 0.7071067811865259234, 7.071067811865685367E-16 ) ) ;
#46947=CIRCLE ( 'NONE', #81807, 1.571100913904471819 ) ;
#46948=CARTESIAN_POINT ( 'NONE',  ( 25.56670390244797275, -48.82844715994099971, 170.4678068554149775 ) ) ;
#46949=CARTESIAN_POINT ( 'NONE',  ( 34.27258461953899626, -35.55794170701810941, -5.074374724088000832 ) ) ;
#46953=DIRECTION ( 'NONE',  ( -0.7071067811865692221, -0.7071067811865259234, -7.071067811865685367E-16 ) ) ;
#46954=CARTESIAN_POINT ( 'NONE',  ( 107.2435442917537500, -47.21071675017731906, 212.5899109901969837 ) ) ;
#46955=CARTESIAN_POINT ( 'NONE',  ( 103.2788791697577295, -47.11347506355160419, 93.28610146638693834 ) ) ;
#46956=CARTESIAN_POINT ( 'NONE',  ( 112.6870894866849966, -45.56130799126797370, 259.0270538473393458 ) ) ;
#46957=DIRECTION ( 'NONE',  ( 0.000000000000000000, 0.000000000000000000, -1.000000000000000000 ) ) ;
#46958=DIRECTION ( 'NONE',  ( 0.000000000000000000, 0.000000000000000000, 1.000000000000000000 ) ) ;
#46961=DIRECTION ( 'NONE',  ( -1.000000000000000078E-15, 1.000000000000000000, 0.000000000000000000 ) ) ;
#46962=CARTESIAN_POINT ( 'NONE',  ( 133.0522658619956928, -21.28573230649608661, 1.785258109344280975 ) ) ;
#46963=ORIENTED_EDGE ( 'NONE', *, *, #82023, .T. ) ;
#46964=VERTEX_POINT ( 'NONE', #37942 ) ;
#46965=CARTESIAN_POINT ( 'NONE',  ( 112.6189512620115778, -30.20087909038965535, 138.9381341137909658 ) ) ;
#46968=CARTESIAN_POINT ( 'NONE',  ( 100.9546086862564920, -28.70707578211034061, 90.59232038796342579 ) ) ;
#46969=CARTESIAN_POINT ( 'NONE',  ( 97.85535806214043930, -31.89376338832687097, 131.9413395616259947 ) ) ;
#46970=LINE ( 'NONE', #81100, #23660 ) ;
#46971=DIRECTION ( 'NONE',  ( -0.7071067811578587436, 0.7071067812152364018, 0.000000000000000000 ) ) ;
#46972=PLANE ( 'NONE',  #54878 ) ;
#46973=CARTESIAN_POINT ( 'NONE',  ( 117.0608945237148646, -38.08045311927313747, 109.7189586093670215 ) ) ;
#46974=CARTESIAN_POINT ( 'NONE',  ( 116.6363502066643321, -38.74961609181406175, 63.66133956162595098 ) ) ;
#46977=VERTEX_POINT ( 'NONE', #9348 ) ;
#46978=VECTOR ( 'NONE', #38808, 1000.000000000000000 ) ;
#46979=LINE ( 'NONE', #81997, #18102 ) ;
#46980=CARTESIAN_POINT ( 'NONE',  ( 109.6835627966674878, -27.30531164764932939, 170.8613395616249591 ) ) ;
#46981=CARTESIAN_POINT ( 'NONE',  ( 107.0664832912730020, -27.87844715994269862, 361.9756252759109998 ) ) ;
#46984=ADVANCED_FACE ( 'NONE', ( #24755 ), #64757, .T. ) ;
#46986=EDGE_CURVE ( 'NONE', #73517, #41893, #81865, .T. ) ;
#46987=CARTESIAN_POINT ( 'NONE',  ( 72.06648329127401098, -46.47944715994106701, 14.67562527591093513 ) ) ;
#46989=DIRECTION ( 'NONE',  ( 0.000000000000000000, 0.000000000000000000, 1.000000000000000000 ) ) ;
#46991=CARTESIAN_POINT ( 'NONE',  ( 116.9541756933415257, -33.49491404195858735, 89.07848241876791917 ) ) ;
#46995=CARTESIAN_POINT ( 'NONE',  ( 90.44969454456422397, -56.64645651782492308, 249.5838068554174640 ) ) ;
#46999=CARTESIAN_POINT ( 'NONE',  ( 99.97311099609123630, -31.77112186149751949, 158.6471379886389741 ) ) ;
#47000=EDGE_CURVE ( 'NONE', #51570, #5050, #30681, .T. ) ;
#47001=CIRCLE ( 'NONE', #70458, 11.45913725231036118 ) ;
#47003=AXIS2_PLACEMENT_3D ( 'NONE', #18919, #24844, #10323 ) ;
#47004=EDGE_CURVE ( 'NONE', #55605, #770, #32008, .T. ) ;
#47005=CARTESIAN_POINT ( 'NONE',  ( 70.06202783732103967, -36.73691869758536654, 394.9756252759101471 ) ) ;
#47006=ORIENTED_EDGE ( 'NONE', *, *, #26616, .F. ) ;
#47009=AXIS2_PLACEMENT_3D ( 'NONE', #38356, #57913, #37031 ) ;
#47011=VERTEX_POINT ( 'NONE', #51112 ) ;
#47012=ORIENTED_EDGE ( 'NONE', *, *, #74133, .F. ) ;
#47014=EDGE_CURVE ( 'NONE', #50621, #3837, #17501, .T. ) ;
#47015=CARTESIAN_POINT ( 'NONE',  ( 102.2537836627552821, -44.20608088590525853, 218.5530118773259574 ) ) ;
#47020=DIRECTION ( 'NONE',  ( 0.000000000000000000, 0.000000000000000000, -1.000000000000000000 ) ) ;
#47023=B_SPLINE_CURVE_WITH_KNOTS ( 'NONE', 3,
 ( #2775, #86779, #59935, #32237, #10471, #86333, #30910, #18168, #24993, #80866, #38173, #80414, #24550, #24111, #18621, #87224, #87667, #58600 ),
 .UNSPECIFIED., .F., .F.,
 ( 4, 2, 2, 2, 2, 2, 2, 2, 4 ),
 ( 0.000000000000000000, 0.06249999947104563358, 0.1249999989420912672, 0.1874999984131369146, 0.2499999978841825343, 0.3124999973552281540, 0.3749999968262738292, 0.4374999962973194489, 0.4999999957683650686 ),
 .UNSPECIFIED. ) ;
#47024=CARTESIAN_POINT ( 'NONE',  ( 106.8982433325019059, -45.38234380569505788, 225.3671379886389730 ) ) ;
#47025=CARTESIAN_POINT ( 'NONE',  ( 96.61975328461473111, -36.61901104994432643, 111.3184824187679567 ) ) ;
#47026=CARTESIAN_POINT ( 'NONE',  ( 96.73644666290614680, -38.23103596604165944, 66.44133956162495735 ) ) ;
#47027=CARTESIAN_POINT ( 'NONE',  ( 113.4712900281284362, -42.87177457074936626, 249.5838068554168672 ) ) ;
#47030=CARTESIAN_POINT ( 'NONE',  ( 97.40207042353749500, -40.63861732370358482, 202.6327681330539860 ) ) ;
#47031=CARTESIAN_POINT ( 'NONE',  ( 134.0664828118825938, -21.47944715903993540, 8.225259175038406312 ) ) ;
#47033=DIRECTION ( 'NONE',  ( 0.000000000000000000, 0.000000000000000000, -1.000000000000000000 ) ) ;
#47035=ORIENTED_EDGE ( 'NONE', *, *, #55788, .T. ) ;
#47036=DIRECTION ( 'NONE',  ( 0.7071067811866516006, -0.7071067811864434338, 0.000000000000000000 ) ) ;
#47037=VECTOR ( 'NONE', #9852, 1000.000000000000000 ) ;
#47038=ADVANCED_FACE ( 'NONE', ( #2981 ), #85669, .F. ) ;
#47039=ORIENTED_EDGE ( 'NONE', *, *, #81421, .T. ) ;
#47040=CIRCLE ( 'NONE', #26764, 3.000000000000002665 ) ;
#47043=CARTESIAN_POINT ( 'NONE',  ( 108.0341695913198521, -25.71842219955733810, 109.9946728949589811 ) ) ;
#47046=CARTESIAN_POINT ( 'NONE',  ( 37.56670390244716629, -48.82844715994126261, 180.4678068554150911 ) ) ;
#47047=DIRECTION ( 'NONE',  ( 1.000000000000000000, 0.000000000000000000, -2.127927463864879951E-15 ) ) ;
#47049=LINE ( 'NONE', #54304, #78961 ) ;
#47050=CARTESIAN_POINT ( 'NONE',  ( 103.8265608274144398, -48.10271009292816302, 213.3556252759109668 ) ) ;
#47051=DIRECTION ( 'NONE',  ( 0.000000000000000000, 0.000000000000000000, -1.000000000000000000 ) ) ;
#47052=DIRECTION ( 'NONE',  ( 0.7071067811864661934, 0.7071067811866289521, 7.071067811864966518E-16 ) ) ;
#47056=CARTESIAN_POINT ( 'NONE',  ( 19.56670390244648416, -25.42844715994203852, 129.9678068554150627 ) ) ;
#47057=CARTESIAN_POINT ( 'NONE',  ( 172.5664832912729878, -18.82844715994071194, 255.9256252759120684 ) ) ;
#47058=ADVANCED_FACE ( 'NONE', ( #66075 ), #81856, .T. ) ;
#47059=CARTESIAN_POINT ( 'NONE',  ( 100.8220609092773117, -45.17687181127147511, 257.0699109901966608 ) ) ;
#47060=VERTEX_POINT ( 'NONE', #79300 ) ;
#47061=CARTESIAN_POINT ( 'NONE',  ( 101.7228746988208030, -28.24295021050552990, 195.5233366543221223 ) ) ;
#47062=CARTESIAN_POINT ( 'NONE',  ( 117.5122013968931327, -37.28485508719111863, 14.78419670448294454 ) ) ;
#47063=CARTESIAN_POINT ( 'NONE',  ( 108.0108636065302932, -26.30228954677034992, 151.0041967044829505 ) ) ;
#47065=CARTESIAN_POINT ( 'NONE',  ( 97.80783988303282683, -40.50800889367277335, 102.6348159224356920 ) ) ;
#47066=CARTESIAN_POINT ( 'NONE',  ( 51.56670390244799762, -33.35206098992650681, 342.9256252759109884 ) ) ;
#47068=DIRECTION ( 'NONE',  ( -1.000000000000000078E-15, 1.000000000000000083E-30, 1.000000000000000000 ) ) ;
#47070=EDGE_LOOP ( 'NONE', ( #60206, #53459 ) ) ;
#47073=AXIS2_PLACEMENT_3D ( 'NONE', #60485, #75487, #40945 ) ;
#47078=AXIS2_PLACEMENT_3D ( 'NONE', #5646, #89660, #61478 ) ;
#47080=ORIENTED_EDGE ( 'NONE', *, *, #7965, .T. ) ;
#47082=CARTESIAN_POINT ( 'NONE',  ( 114.0759046727995241, -46.25395340493271590, 29.08133956162595268 ) ) ;
#47084=CARTESIAN_POINT ( 'NONE',  ( 116.3212776292293995, -32.94146857471265122, 80.13562527591095375 ) ) ;
#47085=CARTESIAN_POINT ( 'NONE',  ( 107.0620278373210255, -36.73691869758540207, 361.9756252759100903 ) ) ;
#47086=CARTESIAN_POINT ( 'NONE',  ( 22.49541547940852837, 22.69262065192447864, 323.8756252759109202 ) ) ;
#47087=CARTESIAN_POINT ( 'NONE',  ( 98.66229053285113082, -40.10320091580625501, 251.0648007804577730 ) ) ;
#47088=EDGE_LOOP ( 'NONE', ( #3165, #9768 ) ) ;
#47089=ORIENTED_EDGE ( 'NONE', *, *, #52118, .T. ) ;
#47091=LINE ( 'NONE', #12606, #77641 ) ;
#47094=AXIS2_PLACEMENT_3D ( 'NONE', #46937, #33777, #46491 ) ;
#47096=ADVANCED_FACE ( 'NONE', ( #21416 ), #29591, .F. ) ;
#47097=CARTESIAN_POINT ( 'NONE',  ( 114.5680773229086782, -32.01199386431652272, 30.70444044875397793 ) ) ;
#47100=ADVANCED_FACE ( 'NONE', ( #69113 ), #69560, .F. ) ;
#47102=CARTESIAN_POINT ( 'NONE',  ( 115.2378349030890945, -31.35427756934436871, 254.2899109901970292 ) ) ;
#47103=FACE_OUTER_BOUND ( 'NONE', #27421, .T. ) ;
#47104=ORIENTED_EDGE ( 'NONE', *, *, #68168, .T. ) ;
#47105=EDGE_CURVE ( 'NONE', #1366, #37421, #23834, .T. ) ;
#47106=CARTESIAN_POINT ( 'NONE',  ( 188.5667039024479834, -58.35344715994099829, 293.2178068554150627 ) ) ;
#47108=CARTESIAN_POINT ( 'NONE',  ( 99.78939748087903183, -33.03164401141575723, 48.77094751244892734 ) ) ;
#47109=CIRCLE ( 'NONE', #70354, 6.571100913904384555 ) ;
#47111=DIRECTION ( 'NONE',  ( 1.000000000000000000, 0.000000000000000000, 0.000000000000000000 ) ) ;
#47112=VECTOR ( 'NONE', #54759, 1000.000000000000000 ) ;
#47114=ADVANCED_FACE ( 'NONE', ( #28203 ), #55896, .T. ) ;
#47115=CARTESIAN_POINT ( 'NONE',  ( 104.4080392062299012, -46.45807122338121786, 193.3647126831750143 ) ) ;
#47116=EDGE_LOOP ( 'NONE', ( #16907, #16521, #60779, #54058, #81161, #56064, #37502, #24682, #50637, #77238, #64994, #54516 ) ) ;
#47117=FACE_OUTER_BOUND ( 'NONE', #29805, .T. ) ;
#47118=EDGE_LOOP ( 'NONE', ( #73570, #53570, #15829, #22727 ) ) ;
#47119=CARTESIAN_POINT ( 'NONE',  ( 98.83989573471103540, -28.19928051380002287, 115.6870538473389587 ) ) ;
#47120=EDGE_LOOP ( 'NONE', ( #49917, #17209, #44260, #3147 ) ) ;
#47121=CARTESIAN_POINT ( 'NONE',  ( 109.3970511370136904, -44.97690468586920787, 72.21813411379096692 ) ) ;
#47122=FACE_OUTER_BOUND ( 'NONE', #43921, .T. ) ;
#47123=CARTESIAN_POINT ( 'NONE',  ( 100.2558307937446074, -42.39895253252459639, 113.3101547344679574 ) ) ;
#47124=LINE ( 'NONE', #74859, #88123 ) ;
#47125=DIRECTION ( 'NONE',  ( 1.000000000000000000, 4.163336342344333240E-14, 0.000000000000000000 ) ) ;
#47126=CARTESIAN_POINT ( 'NONE',  ( 112.7535375185862705, -27.22457367525289129, 50.65943479972101215 ) ) ;
#47127=CARTESIAN_POINT ( 'NONE',  ( 104.4903241021636973, -26.97870597410075888, 181.2818875591321444 ) ) ;
#47128=DIRECTION ( 'NONE',  ( 0.000000000000000000, 0.000000000000000000, 1.000000000000000000 ) ) ;
#47130=ORIENTED_EDGE ( 'NONE', *, *, #16201, .T. ) ;
#47131=CARTESIAN_POINT ( 'NONE',  ( 77.54412859703678862, -19.82508440162619223, 2.797770139038477044 ) ) ;
#47132=AXIS2_PLACEMENT_3D ( 'NONE', #12250, #40396, #19965 ) ;
#47133=AXIS2_PLACEMENT_3D ( 'NONE', #12152, #41182, #68009 ) ;
#47134=VECTOR ( 'NONE', #23719, 1000.000000000000000 ) ;
#47136=ORIENTED_EDGE ( 'NONE', *, *, #58191, .F. ) ;
#47137=AXIS2_PLACEMENT_3D ( 'NONE', #21863, #35460, #22306 ) ;
#47138=DIRECTION ( 'NONE',  ( 2.900000000000000265E-14, -2.000000000000000155E-15, 1.000000000000000000 ) ) ;
#47139=ORIENTED_EDGE ( 'NONE', *, *, #23176, .T. ) ;
#47140=CARTESIAN_POINT ( 'NONE',  ( 104.5747221139661320, -26.66317121150808944, 240.2575300378159682 ) ) ;
#47141=CARTESIAN_POINT ( 'NONE',  ( 108.5929805111718593, -47.10003145027929605, 138.6927681330539883 ) ) ;
#47142=DIRECTION ( 'NONE',  ( 0.000000000000000000, 1.000000000000000000, 0.000000000000000000 ) ) ;
#47143=DIRECTION ( 'NONE',  ( -1.000000000000000078E-15, 1.000000000000000083E-30, 1.000000000000000000 ) ) ;
#47144=CARTESIAN_POINT ( 'NONE',  ( 112.5142634568524329, -27.84101767465772070, 90.63848241876793566 ) ) ;
#47145=PLANE ( 'NONE',  #74051 ) ;
#47146=ORIENTED_EDGE ( 'NONE', *, *, #83576, .T. ) ;
#47147=CIRCLE ( 'NONE', #76216, 10.04999999999999361 ) ;
#47148=CARTESIAN_POINT ( 'NONE',  ( 97.81168895331838087, -40.51742574516882200, 287.6356252759109680 ) ) ;
#47150=ADVANCED_FACE ( 'NONE', ( #34126 ), #33691, .T. ) ;
#47152=ORIENTED_EDGE ( 'NONE', *, *, #79629, .F. ) ;
#47154=DIRECTION ( 'NONE',  ( 0.000000000000000000, 1.000000000000000000, 0.000000000000000000 ) ) ;
#47155=CARTESIAN_POINT ( 'NONE',  ( 99.34937008002594894, -28.84845824588779095, 270.7051490854348685 ) ) ;
#47159=CARTESIAN_POINT ( 'NONE',  ( 105.8912501276363543, -45.18964566429946217, 256.8895626852198006 ) ) ;
#47160=CARTESIAN_POINT ( 'NONE',  ( 98.43224882071085347, -31.53101443417716254, 100.8965674670191959 ) ) ;
#47161=CARTESIAN_POINT ( 'NONE',  ( 97.59110611908495514, -31.08311649095520934, 126.9108633711489915 ) ) ;
#47162=CARTESIAN_POINT ( 'NONE',  ( 172.5664832912729878, -27.57844715994070484, 198.9256252759119832 ) ) ;
#47163=CARTESIAN_POINT ( 'NONE',  ( 102.0606772939666627, -27.53441096011033906, 145.4727681330539610 ) ) ;
#47164=EDGE_LOOP ( 'NONE', ( #5177, #32025, #18441, #11872 ) ) ;
#47166=ORIENTED_EDGE ( 'NONE', *, *, #62208, .T. ) ;
#47169=CARTESIAN_POINT ( 'NONE',  ( 136.5888380630362633, -35.63381004753313164, 2.797770231024470533 ) ) ;
#47170=ORIENTED_EDGE ( 'NONE', *, *, #6919, .F. ) ;
#47171=CARTESIAN_POINT ( 'NONE',  ( 141.0664832912740394, -46.72944715994099596, 14.67562527591100441 ) ) ;
#47172=CARTESIAN_POINT ( 'NONE',  ( 116.8367917427482467, -32.96809911012589112, 139.1184824187679396 ) ) ;
#47174=CARTESIAN_POINT ( 'NONE',  ( 141.0667039024479834, -50.82844715994100682, 250.9178068554160461 ) ) ;
#47176=CARTESIAN_POINT ( 'NONE',  ( 144.8545562996768012, -1.932463243632626781, 394.9756252759100903 ) ) ;
#47177=AXIS2_PLACEMENT_3D ( 'NONE', #34548, #62253, #21837 ) ;
#47180=ADVANCED_FACE ( 'NONE', ( #19009 ), #88060, .F. ) ;
#47181=CIRCLE ( 'NONE', #22581, 2.749999999999974687 ) ;
#47184=ORIENTED_EDGE ( 'NONE', *, *, #19220, .T. ) ;
#47185=DIRECTION ( 'NONE',  ( 1.000000000000000078E-15, -1.000000000000000083E-30, -1.000000000000000000 ) ) ;
#47187=CARTESIAN_POINT ( 'NONE',  ( 98.30753412437063332, -41.72887537653042500, 156.7397919321415714 ) ) ;
#47188=DIRECTION ( 'NONE',  ( 0.9242245927363031965, 0.3818493186865917766, 0.000000000000000000 ) ) ;
#47189=CARTESIAN_POINT ( 'NONE',  ( 116.3212776292296127, -32.94146857471318413, 287.6356252759109680 ) ) ;
#47191=CARTESIAN_POINT ( 'NONE',  ( 112.1392728139803694, -28.01277785882846061, 179.6564653195408425 ) ) ;
#47192=AXIS2_PLACEMENT_3D ( 'NONE', #68581, #19981, #47663 ) ;
#47193=ORIENTED_EDGE ( 'NONE', *, *, #41072, .F. ) ;
#47197=VECTOR ( 'NONE', #28617, 1000.000000000000000 ) ;
#47198=CARTESIAN_POINT ( 'NONE',  ( 181.8764988495249497, -33.54226604284360036, 117.4678068554150627 ) ) ;
#47199=CARTESIAN_POINT ( 'NONE',  ( 108.5755967597531679, -27.06580334247545494, 185.9527681330529845 ) ) ;
#47200=EDGE_CURVE ( 'NONE', #25576, #752, #26267, .T. ) ;
#47201=DIRECTION ( 'NONE',  ( -0.7071067812159671506, -0.7071067811571278838, -6.612322856129998538E-17 ) ) ;
#47203=VECTOR ( 'NONE', #45069, 1000.000000000000000 ) ;
#47204=B_SPLINE_CURVE_WITH_KNOTS ( 'NONE', 3,
 ( #44234, #9736, #2483, #72416, #10616, #57880, #10180, #79241, #43345, #79688, #85614, #45123, #15668, #17442, #72848, #38321, #37888, #16553, #37441, #58325, #8861, #66019, #36559, #65142, #2034, #29742, #23392, #65587, #43794, #3810, #57429 ),
 .UNSPECIFIED., .F., .F.,
 ( 4, 2, 2, 1, 2, 2, 2, 2, 2, 2, 2, 1, 1, 2, 2, 2, 4 ),
 ( 0.000000000000000000, 0.1249999999999738542, 0.1874999999999520384, 0.2187499999999411304, 0.2343749999999427958, 0.2499999999999444611, 0.3749999999999549805, 0.4374999999999669709, 0.4999999999999790168, 0.6250000000000159872, 0.6875000000000371925, 0.7187500000000494049, 0.7343750000000499600, 0.7421875000000518474, 0.7500000000000536238, 0.8750000000000267564, 1.000000000000000000 ),
 .UNSPECIFIED. ) ;
#47205=CARTESIAN_POINT ( 'NONE',  ( 116.3624975636023322, -33.68846805112529808, 85.07848241876692441 ) ) ;
#47207=LINE ( 'NONE', #67674, #41429 ) ;
#47209=PLANE ( 'NONE',  #74656 ) ;
#47210=AXIS2_PLACEMENT_3D ( 'NONE', #8580, #64881, #50793 ) ;
#47211=DIRECTION ( 'NONE',  ( 9.351236661543306751E-17, -3.725950533538267725E-29, -1.000000000000000000 ) ) ;
#47212=ORIENTED_EDGE ( 'NONE', *, *, #82300, .F. ) ;
#47214=EDGE_CURVE ( 'NONE', #11683, #64730, #74423, .T. ) ;
#47215=ORIENTED_EDGE ( 'NONE', *, *, #53476, .F. ) ;
#47217=AXIS2_PLACEMENT_3D ( 'NONE', #62189, #21777, #89927 ) ;
#47218=CARTESIAN_POINT ( 'NONE',  ( 102.2537836627552821, -44.20608088590525853, 218.5530118773259574 ) ) ;
#47223=EDGE_CURVE ( 'NONE', #21126, #54865, #81260, .T. ) ;
#47224=CARTESIAN_POINT ( 'NONE',  ( 82.16371341589938027, -38.51083119283502754, 2.376725019073457013 ) ) ;
#47226=CARTESIAN_POINT ( 'NONE',  ( 41.56648329127499153, -36.32844715994070839, 18.92562527591200094 ) ) ;
#47229=CARTESIAN_POINT ( 'NONE',  ( 116.1206117333611871, -31.56300607074027909, 289.2384824187681716 ) ) ;
#47230=ORIENTED_EDGE ( 'NONE', *, *, #12172, .F. ) ;
#47231=CARTESIAN_POINT ( 'NONE',  ( 99.19750579858670392, -34.55944272753168889, 248.9309475124489950 ) ) ;
#47233=CARTESIAN_POINT ( 'NONE',  ( 96.69720940280899413, -36.59277893904148726, 156.3280062282929634 ) ) ;
#47236=CARTESIAN_POINT ( 'NONE',  ( 90.44969454456405344, -18.85368780205715566, 218.8274735512160589 ) ) ;
#47237=DIRECTION ( 'NONE',  ( 0.000000000000000000, 0.000000000000000000, -1.000000000000000000 ) ) ;
#47238=AXIS2_PLACEMENT_3D ( 'NONE', #23630, #51289, #57678 ) ;
#47239=CARTESIAN_POINT ( 'NONE',  ( 96.76602677561474763, -40.86443131079876423, 247.6422919425769749 ) ) ;
#47240=DIRECTION ( 'NONE',  ( 0.000000000000000000, 0.000000000000000000, -1.000000000000000000 ) ) ;
#47241=ORIENTED_EDGE ( 'NONE', *, *, #30410, .T. ) ;
#47242=CARTESIAN_POINT ( 'NONE',  ( 102.5393486652204160, -27.29027178147674348, 91.43276813305395478 ) ) ;
#47243=DIRECTION ( 'NONE',  ( -0.7071067811855900054, -0.7071067811875051401, 0.000000000000000000 ) ) ;
#47244=AXIS2_PLACEMENT_3D ( 'NONE', #18435, #67933, #59316 ) ;
#47245=ORIENTED_EDGE ( 'NONE', *, *, #63522, .F. ) ;
#47247=ORIENTED_EDGE ( 'NONE', *, *, #21918, .T. ) ;
#47248=CARTESIAN_POINT ( 'NONE',  ( 112.1371669992055047, -28.01157492980603436, 159.6564172049183412 ) ) ;
#47249=DIRECTION ( 'NONE',  ( 0.000000000000000000, 0.000000000000000000, -1.000000000000000000 ) ) ;
#47252=CARTESIAN_POINT ( 'NONE',  ( 99.76898186052154927, -41.38212431049157658, 139.5842808457819615 ) ) ;
#47253=CARTESIAN_POINT ( 'NONE',  ( 105.1049547281328671, -25.82818065531082041, 271.2061014663873380 ) ) ;
#47254=DIRECTION ( 'NONE',  ( 3.999999999999999995E-14, -1.000000000000000000, 4.100000000000000342E-29 ) ) ;
#47257=CARTESIAN_POINT ( 'NONE',  ( 99.04405175095710945, -42.84124461182535271, 41.84339552792118155 ) ) ;
#47259=EDGE_LOOP ( 'NONE', ( #67995, #31044, #70607, #20462 ) ) ;
#47262=AXIS2_PLACEMENT_3D ( 'NONE', #27337, #13715, #69128 ) ;
#47263=DIRECTION ( 'NONE',  ( 1.000000000000000078E-15, -1.000000000000000083E-30, -1.000000000000000000 ) ) ;
#47266=ORIENTED_EDGE ( 'NONE', *, *, #2061, .T. ) ;
#47267=DIRECTION ( 'NONE',  ( 0.7071067811865295871, -0.7071067811865655584, 7.071067811865303756E-16 ) ) ;
#47268=DIRECTION ( 'NONE',  ( -0.7071067811864691910, -0.7071067811866257324, -7.071067811864685486E-16 ) ) ;
#47269=CIRCLE ( 'NONE', #13897, 10.00000000000000711 ) ;
#47273=CARTESIAN_POINT ( 'NONE',  ( 115.0466524894680731, -42.26004630958951935, 162.7667055423629847 ) ) ;
#47274=CARTESIAN_POINT ( 'NONE',  ( 104.4797840155964082, -46.91084102236943920, 47.37848241876796607 ) ) ;
#47275=DIRECTION ( 'NONE',  ( -0.7071067812162665778, -0.7071067811568285677, -7.071067812162971544E-16 ) ) ;
#47278=ORIENTED_EDGE ( 'NONE', *, *, #45799, .F. ) ;
#47280=VERTEX_POINT ( 'NONE', #40337 ) ;
#47282=CARTESIAN_POINT ( 'NONE',  ( 41.56648329127499153, -36.32844715994070839, 78.92562527591199739 ) ) ;
#47283=CARTESIAN_POINT ( 'NONE',  ( 25.56670390244748603, -48.82844715994178841, 134.7178068554150627 ) ) ;
#47284=CIRCLE ( 'NONE', #42948, 3.250000000000002665 ) ;
#47288=CARTESIAN_POINT ( 'NONE',  ( 102.7461184130007581, -25.66741906146929253, 20.37276813305294354 ) ) ;
#47289=CARTESIAN_POINT ( 'NONE',  ( 115.2412948192700952, -44.23743989039658686, 74.22324432352993995 ) ) ;
#47292=CARTESIAN_POINT ( 'NONE',  ( 177.8371591254545478, -47.82818131005477369, 129.9678068554150059 ) ) ;
#47294=DIRECTION ( 'NONE',  ( 8.755702086949183871E-16, 1.000000000000000000, 0.000000000000000000 ) ) ;
#47295=DIRECTION ( 'NONE',  ( 0.000000000000000000, 0.000000000000000000, -1.000000000000000000 ) ) ;
#47296=ORIENTED_EDGE ( 'NONE', *, *, #9088, .F. ) ;
#47300=VERTEX_POINT ( 'NONE', #72309 ) ;
#47301=CARTESIAN_POINT ( 'NONE',  ( 96.67081033544403113, -37.96906397156782731, 41.42133956162496844 ) ) ;
#47302=CARTESIAN_POINT ( 'NONE',  ( 117.1274056176845733, -39.54282605291903252, 94.60991099019693706 ) ) ;
#47303=CARTESIAN_POINT ( 'NONE',  ( 117.0612810359348543, -38.07772461170434752, 173.7166616957481722 ) ) ;
#47304=DIRECTION ( 'NONE',  ( 4.299999999999999979E-14, -1.000000000000000000, 4.400000000000000367E-29 ) ) ;
#47305=DIRECTION ( 'NONE',  ( 0.0001211784769825749220, -0.7071067708032379162, 0.7071067811865431318 ) ) ;
#47306=LINE ( 'NONE', #61832, #76721 ) ;
#47308=CARTESIAN_POINT ( 'NONE',  ( 107.9743429475490615, -26.39917242597376301, 105.9946728949579864 ) ) ;
#47310=ORIENTED_EDGE ( 'NONE', *, *, #70009, .F. ) ;
#47311=CARTESIAN_POINT ( 'NONE',  ( 114.5897159479185490, -29.54407062678539830, 230.4327681330539690 ) ) ;
#47312=CARTESIAN_POINT ( 'NONE',  ( 97.81213350417895924, -40.51851190632524435, 252.6356759604615547 ) ) ;
#47314=DIRECTION ( 'NONE',  ( 1.000000000000000000, 1.261617073437676668E-15, 9.462128050782575008E-16 ) ) ;
#47316=CARTESIAN_POINT ( 'NONE',  ( 69.25757238336809962, -1.944390235229864539, 394.9756252759101471 ) ) ;
#47319=AXIS2_PLACEMENT_3D ( 'NONE', #29065, #29512, #49025 ) ;
#47320=CARTESIAN_POINT ( 'NONE',  ( 103.1701080265564485, -27.72257962874988024, 155.4013395616259743 ) ) ;
#47323=CIRCLE ( 'NONE', #41550, 0.5000000000000004441 ) ;
#47324=CARTESIAN_POINT ( 'NONE',  ( 98.22997538087754776, -36.06364078424440578, 142.6987261630399644 ) ) ;
#47325=CIRCLE ( 'NONE', #40072, 0.5000000000000172085 ) ;
#47328=CARTESIAN_POINT ( 'NONE',  ( 100.5669465097398358, -44.03830869352244548, 262.9984824187674235 ) ) ;
#47329=CARTESIAN_POINT ( 'NONE',  ( 133.6498166246070127, 12.92155284005802507, 336.5756252759110225 ) ) ;
#47331=DIRECTION ( 'NONE',  ( 0.000000000000000000, -1.000000000000000000, 0.000000000000000000 ) ) ;
#47332=FACE_OUTER_BOUND ( 'NONE', #41950, .T. ) ;
#47333=ADVANCED_FACE ( 'NONE', ( #54389 ), #11292, .T. ) ;
#47334=CARTESIAN_POINT ( 'NONE',  ( 107.0664832912739968, -36.72944715994100306, 287.6356252759109680 ) ) ;
#47335=CARTESIAN_POINT ( 'NONE',  ( 182.0667039024476708, -32.29483332967959086, 237.4678068554150059 ) ) ;
#47336=CARTESIAN_POINT ( 'NONE',  ( 188.5667039024479834, -62.87844715994099687, 254.4678068554150343 ) ) ;
#47338=CARTESIAN_POINT ( 'NONE',  ( 97.78191787992076911, -41.50032452247409509, 196.7041967044819728 ) ) ;
#47339=DIRECTION ( 'NONE',  ( 0.000000000000000000, 0.000000000000000000, -1.000000000000000000 ) ) ;
#47343=CARTESIAN_POINT ( 'NONE',  ( 77.85922577378461540, -17.08568546287367695, 2.471387922356760303 ) ) ;
#47344=CARTESIAN_POINT ( 'NONE',  ( 194.0667039024473581, -24.92844715993408045, 249.9678068554149775 ) ) ;
#47345=CARTESIAN_POINT ( 'NONE',  ( 163.0667039024466192, -32.29483332967941323, 313.9678068554149490 ) ) ;
#47346=VECTOR ( 'NONE', #40570, 1000.000000000000000 ) ;
#47348=ORIENTED_EDGE ( 'NONE', *, *, #39995, .T. ) ;
#47349=DIRECTION ( 'NONE',  ( 0.000000000000000000, 1.000000000000000000, 0.000000000000000000 ) ) ;
#47350=CARTESIAN_POINT ( 'NONE',  ( 96.67388729539801773, -35.53787041403403180, 206.2356252759109623 ) ) ;
#47353=CARTESIAN_POINT ( 'NONE',  ( 76.06670390244796920, -26.72944715994109899, 239.5838068554169809 ) ) ;
#47355=CARTESIAN_POINT ( 'NONE',  ( 109.0838521367681864, -44.63893190664380484, 45.59380465530593796 ) ) ;
#47356=CARTESIAN_POINT ( 'NONE',  ( 105.3125989252256147, -48.47411034989094958, 143.4584824187689662 ) ) ;
#47357=DIRECTION ( 'NONE',  ( 9.351236661543306751E-17, -3.725950533538267725E-29, -1.000000000000000000 ) ) ;
#47358=ORIENTED_EDGE ( 'NONE', *, *, #75222, .T. ) ;
#47359=CIRCLE ( 'NONE', #58969, 0.5000000000000004441 ) ;
#47361=CARTESIAN_POINT ( 'NONE',  ( 107.9967959839596148, -46.76990057558159464, 67.65228226674308587 ) ) ;
#47362=ORIENTED_EDGE ( 'NONE', *, *, #7247, .T. ) ;
#47363=ORIENTED_EDGE ( 'NONE', *, *, #70425, .F. ) ;
#47364=DIRECTION ( 'NONE',  ( 0.7071067811869279351, -0.7071067811861670993, 6.612322855863716074E-17 ) ) ;
#47366=ORIENTED_EDGE ( 'NONE', *, *, #54256, .F. ) ;
#47369=CARTESIAN_POINT ( 'NONE',  ( 104.5191702102720939, -45.41989400652479958, 61.76003887569697781 ) ) ;
#47370=CARTESIAN_POINT ( 'NONE',  ( 99.73754448486663193, -29.28411171159743276, 225.6956252759109702 ) ) ;
#47371=CARTESIAN_POINT ( 'NONE',  ( 117.4047238282099102, -30.98758422922431066, 179.2299109901959753 ) ) ;
#47372=CARTESIAN_POINT ( 'NONE',  ( 117.0412664019691391, -35.29711810607562228, 23.94033278884533544 ) ) ;
#47373=CARTESIAN_POINT ( 'NONE',  ( 98.44183741489698036, -42.05700530801248505, 7.768006228291934434 ) ) ;
#47374=CARTESIAN_POINT ( 'NONE',  ( 41.56648329127398966, -27.57844715994070484, 21.92562527591199739 ) ) ;
#47375=FACE_OUTER_BOUND ( 'NONE', #42682, .T. ) ;
#47377=AXIS2_PLACEMENT_3D ( 'NONE', #61655, #15328, #56639 ) ;
#47378=CARTESIAN_POINT ( 'NONE',  ( 107.0664832912739399, -36.72944715994095333, 293.6369201390379544 ) ) ;
#47379=CIRCLE ( 'NONE', #14027, 0.5000000000000197620 ) ;
#47380=CARTESIAN_POINT ( 'NONE',  ( 116.6462162596975389, -40.95264290462791479, 253.4956252759109532 ) ) ;
#47381=ORIENTED_EDGE ( 'NONE', *, *, #16992, .F. ) ;
#47382=AXIS2_PLACEMENT_3D ( 'NONE', #12396, #60524, #33287 ) ;
#47383=EDGE_CURVE ( 'NONE', #29231, #6135, #80371, .T. ) ;
#47384=CARTESIAN_POINT ( 'NONE',  ( 108.1817894924016770, -47.09492459897622751, 202.6613395616249704 ) ) ;
#47385=CARTESIAN_POINT ( 'NONE',  ( 97.81168895331838087, -40.51742574516882200, 287.6356252759109680 ) ) ;
#47387=VECTOR ( 'NONE', #62555, 1000.000000000000000 ) ;
#47388=CARTESIAN_POINT ( 'NONE',  ( 97.83885977234140796, -40.58323701166357012, 22.64129154176366754 ) ) ;
#47389=CARTESIAN_POINT ( 'NONE',  ( 115.9957689480958720, -41.40556947845971081, 29.44320292253459215 ) ) ;
#47390=EDGE_CURVE ( 'NONE', #1937, #30939, #2046, .T. ) ;
#47391=CARTESIAN_POINT ( 'NONE',  ( 115.1992151880701840, -36.11503712634230823, 277.6356252759109680 ) ) ;
#47393=CARTESIAN_POINT ( 'NONE',  ( 115.7830542439493939, -41.80240532925106578, 174.4064499672970499 ) ) ;
#47394=DIRECTION ( 'NONE',  ( 0.000000000000000000, 0.000000000000000000, 1.000000000000000000 ) ) ;
#47395=CARTESIAN_POINT ( 'NONE',  ( 167.2371591254543262, -47.82818131005522844, 249.9678068554149775 ) ) ;
#47396=ADVANCED_FACE ( 'NONE', ( #800 ), #63470, .T. ) ;
#47397=LINE ( 'NONE', #34228, #67482 ) ;
#47398=DIRECTION ( 'NONE',  ( -1.000000000000000000, -4.299999999999999979E-14, -1.000000000000000078E-15 ) ) ;
#47401=PLANE ( 'NONE',  #63132 ) ;
#47403=EDGE_CURVE ( 'NONE', #1757, #20886, #12212, .T. ) ;
#47404=CARTESIAN_POINT ( 'NONE',  ( 136.8151996730028372, -18.82419990105082519, 6.751707299520380623 ) ) ;
#47405=CARTESIAN_POINT ( 'NONE',  ( 113.1129168750088638, -46.01039980791943407, 223.0480062282919675 ) ) ;
#47406=CARTESIAN_POINT ( 'NONE',  ( 97.22566771925157525, -31.69632393854739760, 91.96229194257693962 ) ) ;
#47407=CARTESIAN_POINT ( 'NONE',  ( 115.0881438103696155, -30.00293675228997614, 265.3813395616251682 ) ) ;
#47410=CARTESIAN_POINT ( 'NONE',  ( 83.06670390244796920, -58.35344715994099829, 207.5838068554149913 ) ) ;
#47411=VECTOR ( 'NONE', #24169, 999.9999999999998863 ) ;
#47412=FACE_OUTER_BOUND ( 'NONE', #13906, .T. ) ;
#47413=DIRECTION ( 'NONE',  ( 2.900000000000000265E-14, -2.000000000000000155E-15, 1.000000000000000000 ) ) ;
#47414=CARTESIAN_POINT ( 'NONE',  ( 134.0664832912740110, -46.72944715994100306, 4.925625275910997303 ) ) ;
#47416=CARTESIAN_POINT ( 'NONE',  ( 131.5565945955665370, -19.85370728022636655, 2.783021134849384737 ) ) ;
#47417=CLOSED_SHELL ( 'NONE', ( #26411, #49379, #4472, #71040, #83124, #18139, #47427 ) ) ;
#47418=EDGE_CURVE ( 'NONE', #40854, #22057, #33979, .T. ) ;
#47419=ORIENTED_EDGE ( 'NONE', *, *, #88928, .F. ) ;
#47420=VERTEX_POINT ( 'NONE', #35305 ) ;
#47421=CARTESIAN_POINT ( 'NONE',  ( 99.32441224009949110, -32.03125536261004669, 125.3028960185529570 ) ) ;
#47423=ORIENTED_EDGE ( 'NONE', *, *, #261, .T. ) ;
#47424=CARTESIAN_POINT ( 'NONE',  ( 108.4173643679176706, -26.73502001125028116, 89.96755253173861888 ) ) ;
#47425=CARTESIAN_POINT ( 'NONE',  ( 117.5859182825551983, -33.41202194707546624, 125.0575300378149706 ) ) ;
#47427=ADVANCED_FACE ( 'NONE', ( #35757 ), #8066, .F. ) ;
#47430=CARTESIAN_POINT ( 'NONE',  ( 109.6430121354276963, -46.48008673386306100, 108.7814586096431100 ) ) ;
#47431=CARTESIAN_POINT ( 'NONE',  ( 97.89279369561084820, -33.33727167892450183, 66.04419670448297097 ) ) ;
#47432=EDGE_LOOP ( 'NONE', ( #72275, #41529, #77434, #19080, #13109, #4593, #48035, #20407, #37985, #49876, #86898, #69067 ) ) ;
#47436=CARTESIAN_POINT ( 'NONE',  ( 108.2029444874845723, -47.03713394308625340, 153.6518157521009584 ) ) ;
#47437=DIRECTION ( 'NONE',  ( 0.000000000000000000, 0.000000000000000000, -1.000000000000000000 ) ) ;
#47438=CYLINDRICAL_SURFACE ( 'NONE', #79900, 9.999999999999998224 ) ;
#47440=CARTESIAN_POINT ( 'NONE',  ( 163.5667039024460223, -18.82844715994111340, -5.074374724088000832 ) ) ;
#47443=CARTESIAN_POINT ( 'NONE',  ( 108.3331690636866256, -46.73489103495947461, 178.6772697487780306 ) ) ;
#47444=CARTESIAN_POINT ( 'NONE',  ( 113.3016265961370408, -28.35762455946448668, 104.5670538473399347 ) ) ;
#47446=VERTEX_POINT ( 'NONE', #42556 ) ;
#47448=EDGE_CURVE ( 'NONE', #49158, #28809, #75768, .T. ) ;
#47450=AXIS2_PLACEMENT_3D ( 'NONE', #53766, #18373, #79738 ) ;
#47451=CARTESIAN_POINT ( 'NONE',  ( 183.6524903400783444, -49.32844715993451956, 300.4678068554149490 ) ) ;
#47453=VECTOR ( 'NONE', #53566, 1000.000000000000000 ) ;
#47455=CARTESIAN_POINT ( 'NONE',  ( 99.48373692063242402, -40.90112338471579534, 174.5328522743529618 ) ) ;
#47456=AXIS2_PLACEMENT_3D ( 'NONE', #26428, #20067, #34576 ) ;
#47458=AXIS2_PLACEMENT_3D ( 'NONE', #83806, #54257, #21580 ) ;
#47459=LINE ( 'NONE', #13413, #79408 ) ;
#47460=EDGE_LOOP ( 'NONE', ( #10598, #16872, #80229, #816 ) ) ;
#47463=DIRECTION ( 'NONE',  ( 0.000000000000000000, 0.000000000000000000, -1.000000000000000000 ) ) ;
#47467=CARTESIAN_POINT ( 'NONE',  ( 77.68755387134090995, -20.11069332325651615, 7.213126773501262967 ) ) ;
#47468=CARTESIAN_POINT ( 'NONE',  ( 104.6178464025351218, -28.18156397322882967, 221.7301547344689823 ) ) ;
#47470=VECTOR ( 'NONE', #57853, 1000.000000000000000 ) ;
#47471=AXIS2_PLACEMENT_3D ( 'NONE', #33977, #6733, #33097 ) ;
#47472=LINE ( 'NONE', #12080, #70490 ) ;
#47473=DIRECTION ( 'NONE',  ( 0.000000000000000000, 0.000000000000000000, 1.000000000000000000 ) ) ;
#47474=VERTEX_POINT ( 'NONE', #83048 ) ;
#47475=ORIENTED_EDGE ( 'NONE', *, *, #36298, .F. ) ;
#47478=ORIENTED_EDGE ( 'NONE', *, *, #87339, .T. ) ;
#47479=CARTESIAN_POINT ( 'NONE',  ( 106.4678557813946043, -44.87017016969328864, 220.3366617981629645 ) ) ;
#47480=CARTESIAN_POINT ( 'NONE',  ( 117.1850550582282580, -34.12927998004249730, 124.0270538473399426 ) ) ;
#47481=CARTESIAN_POINT ( 'NONE',  ( 116.1047473792920357, -29.10330858331343151, 74.38419670448293175 ) ) ;
#47482=CARTESIAN_POINT ( 'NONE',  ( 99.61185357976398791, -39.68090676418853491, 249.5838068554173503 ) ) ;
#47483=CARTESIAN_POINT ( 'NONE',  ( 131.0667039024480118, -61.87844715994100397, 231.5838068554150198 ) ) ;
#47485=CARTESIAN_POINT ( 'NONE',  ( 117.9485099285917613, -34.79154191225799053, 194.9546728949589749 ) ) ;
#47486=DIRECTION ( 'NONE',  ( 0.9963424814100680926, -0.08544974978095712381, 0.000000000000000000 ) ) ;
#47488=CARTESIAN_POINT ( 'NONE',  ( 107.0667039024479834, -36.72944715994100306, 239.5838068554170093 ) ) ;
#47490=ORIENTED_EDGE ( 'NONE', *, *, #19220, .F. ) ;
#47492=VERTEX_POINT ( 'NONE', #61666 ) ;
#47493=VECTOR ( 'NONE', #30677, 1000.000000000000000 ) ;
#47494=CARTESIAN_POINT ( 'NONE',  ( 51.06648329127400388, 12.92155284005902516, 336.6506252759110112 ) ) ;
#47496=CARTESIAN_POINT ( 'NONE',  ( 106.0764471815382279, -48.53877882342441552, 112.5099109901969712 ) ) ;
#47498=CARTESIAN_POINT ( 'NONE',  ( 136.6005499775789076, -35.66120003907548863, 7.039521718172190745 ) ) ;
#47500=ADVANCED_FACE ( 'NONE', ( #56644 ), #89404, .F. ) ;
#47501=CARTESIAN_POINT ( 'NONE',  ( 101.9936209308341262, -45.44607153293747359, 143.1564586083297286 ) ) ;
#47502=CARTESIAN_POINT ( 'NONE',  ( 63.03715912545644784, -24.42818131006026761, 117.4678068554150485 ) ) ;
#47503=CARTESIAN_POINT ( 'NONE',  ( 113.2071528006339918, -45.12711609280817271, 224.0784824187679476 ) ) ;
#47506=ORIENTED_EDGE ( 'NONE', *, *, #60455, .T. ) ;
#47507=LINE ( 'NONE', #33449, #26650 ) ;
#47510=FACE_OUTER_BOUND ( 'NONE', #49812, .T. ) ;
#47511=ADVANCED_FACE ( 'NONE', ( #20799, #34866 ), #28048, .F. ) ;
#47512=DIRECTION ( 'NONE',  ( 0.000000000000000000, -1.000000000000000000, 0.000000000000000000 ) ) ;
#47513=CARTESIAN_POINT ( 'NONE',  ( 105.1026693892091117, -26.44596034844076371, 235.2270538473399313 ) ) ;
#47515=ADVANCED_FACE ( 'NONE', ( #7619, #41280 ), #48092, .F. ) ;
#47516=CARTESIAN_POINT ( 'NONE',  ( 103.7740925671131151, -27.25659402154724020, 195.3423308223554784 ) ) ;
#47517=CARTESIAN_POINT ( 'NONE',  ( 118.1260584382194025, -36.12034675239389259, 269.8822919425776945 ) ) ;
#47518=CARTESIAN_POINT ( 'NONE',  ( 116.8472425118689841, -43.50793233799721094, 159.3441967044829539 ) ) ;
#47524=CARTESIAN_POINT ( 'NONE',  ( 115.8254323939450501, -31.73001883370779552, 189.2397919421528343 ) ) ;
#47527=EDGE_CURVE ( 'NONE', #49825, #78550, #77571, .T. ) ;
#47531=ORIENTED_EDGE ( 'NONE', *, *, #10486, .F. ) ;
#47533=CIRCLE ( 'NONE', #4036, 1.000000000000000888 ) ;
#47535=CARTESIAN_POINT ( 'NONE',  ( 184.5664832912729878, 15.62155284005731204, 361.9756252759109998 ) ) ;
#47536=CARTESIAN_POINT ( 'NONE',  ( 99.99555918775628527, -44.36035129061379934, 42.98133956162492098 ) ) ;
#47538=EDGE_CURVE ( 'NONE', #75765, #59961, #75823, .T. ) ;
#47541=CIRCLE ( 'NONE', #60570, 2.116999999999993776 ) ;
#47543=AXIS2_PLACEMENT_3D ( 'NONE', #45923, #60005, #67744 ) ;
#47544=CARTESIAN_POINT ( 'NONE',  ( 113.7727705757230297, -31.39298644294678908, 243.7838483995059562 ) ) ;
#47545=EDGE_LOOP ( 'NONE', ( #66808, #67458, #62999, #39638 ) ) ;
#47546=ADVANCED_FACE ( 'NONE', ( #20861 ), #25096, .T. ) ;
#47547=VERTEX_POINT ( 'NONE', #20422 ) ;
#47548=ORIENTED_EDGE ( 'NONE', *, *, #57058, .T. ) ;
#47551=LINE ( 'NONE', #25776, #28093 ) ;
#47552=DIRECTION ( 'NONE',  ( 0.7071067811865779928, -0.7071067811865171526, 7.071067811865786933E-16 ) ) ;
#47553=FACE_OUTER_BOUND ( 'NONE', #23396, .T. ) ;
#47554=DIRECTION ( 'NONE',  ( 1.000000000000000078E-15, -1.000000000000000083E-30, -1.000000000000000000 ) ) ;
#47555=CARTESIAN_POINT ( 'NONE',  ( 99.81116105471912192, -29.32005551970541291, 270.7051490854354938 ) ) ;
#47556=CARTESIAN_POINT ( 'NONE',  ( 172.5664832912740110, 0.2215528400590013880, 78.92562527591199739 ) ) ;
#47558=EDGE_CURVE ( 'NONE', #36904, #28057, #49998, .T. ) ;
#47559=DIRECTION ( 'NONE',  ( 1.000000000000000078E-15, -1.000000000000000083E-30, -1.000000000000000000 ) ) ;
#47560=ADVANCED_FACE ( 'NONE', ( #27674 ), #87333, .F. ) ;
#47561=CARTESIAN_POINT ( 'NONE',  ( 131.3164832912740110, -36.72944715994100306, 6.749768910606454675 ) ) ;
#47562=CARTESIAN_POINT ( 'NONE',  ( 99.60924227704973077, -33.40991670024246218, 98.81094751244894780 ) ) ;
#47563=PLANE ( 'NONE',  #69707 ) ;
#47566=EDGE_LOOP ( 'NONE', ( #64520, #80003 ) ) ;
#47567=CARTESIAN_POINT ( 'NONE',  ( 77.96454488115681158, -34.94667115355367315, 7.474641677900894621 ) ) ;
#47568=ORIENTED_EDGE ( 'NONE', *, *, #5094, .F. ) ;
#47569=CARTESIAN_POINT ( 'NONE',  ( 108.6487477603288170, -25.79654920012707109, 149.9737205140059473 ) ) ;
#47570=EDGE_LOOP ( 'NONE', ( #47743, #28456 ) ) ;
#47571=CARTESIAN_POINT ( 'NONE',  ( 98.06038178923066084, -41.07745101822689548, 87.68391174719410230 ) ) ;
#47572=CARTESIAN_POINT ( 'NONE',  ( 115.6007127221643032, -39.11591036577164004, 95.04158330589696391 ) ) ;
#47576=CARTESIAN_POINT ( 'NONE',  ( 98.57234554589554421, -43.83823254894062416, 67.86895860924497015 ) ) ;
#47577=EDGE_CURVE ( 'NONE', #27248, #21233, #31905, .T. ) ;
#47578=DIRECTION ( 'NONE',  ( 0.7071067811987160612, 0.7071067811743789733, 0.000000000000000000 ) ) ;
#47579=ORIENTED_EDGE ( 'NONE', *, *, #36522, .F. ) ;
#47580=CIRCLE ( 'NONE', #63556, 15.69999999999999574 ) ;
#47581=DIRECTION ( 'NONE',  ( 0.000000000000000000, 0.000000000000000000, 1.000000000000000000 ) ) ;
#47583=ORIENTED_EDGE ( 'NONE', *, *, #41558, .T. ) ;
#47585=DIRECTION ( 'NONE',  ( 1.000000000000000000, -3.885780586187990841E-13, 0.000000000000000000 ) ) ;
#47586=ORIENTED_EDGE ( 'NONE', *, *, #80633, .F. ) ;
#47587=CARTESIAN_POINT ( 'NONE',  ( 101.6507727546967175, -27.01955209951621129, 255.4813395616254468 ) ) ;
#47588=CARTESIAN_POINT ( 'NONE',  ( 114.2549023322775383, -45.16142510923258868, 149.1508633711489722 ) ) ;
#47589=CARTESIAN_POINT ( 'NONE',  ( 25.56670390244797275, -67.87844715994100397, 288.3428068554150059 ) ) ;
#47590=CARTESIAN_POINT ( 'NONE',  ( 115.8254323921544682, -31.73001882933136741, 140.2397919425295356 ) ) ;
#47591=CARTESIAN_POINT ( 'NONE',  ( 117.3387810265436144, -32.64853063025485369, 95.13943479972097350 ) ) ;
#47592=DIRECTION ( 'NONE',  ( 0.000000000000000000, 0.000000000000000000, 1.000000000000000000 ) ) ;
#47593=VERTEX_POINT ( 'NONE', #21311 ) ;
#47594=AXIS2_PLACEMENT_3D ( 'NONE', #79041, #17254, #3611 ) ;
#47596=VECTOR ( 'NONE', #53009, 1000.000000000000000 ) ;
#47602=DIRECTION ( 'NONE',  ( -1.000000000000000078E-15, 1.000000000000000083E-30, 1.000000000000000000 ) ) ;
#47603=CARTESIAN_POINT ( 'NONE',  ( 96.58568816239599641, -40.17018292043295702, 286.5908633711491120 ) ) ;
#47605=ADVANCED_FACE ( 'NONE', ( #5896 ), #61286, .F. ) ;
#47606=FACE_OUTER_BOUND ( 'NONE', #42195, .T. ) ;
#47609=CARTESIAN_POINT ( 'NONE',  ( 110.8002668817294847, -46.40403677370081681, 17.85753003781598380 ) ) ;
#47611=CARTESIAN_POINT ( 'NONE',  ( 114.0662423116485229, -44.47333502991302367, 129.1613395616249704 ) ) ;
#47613=CARTESIAN_POINT ( 'NONE',  ( 99.06758658495417080, -45.54097539030503583, 156.9899109901969609 ) ) ;
#47614=CARTESIAN_POINT ( 'NONE',  ( 182.5667039024459939, -22.48495420874030515, 342.9256252759109884 ) ) ;
#47615=EDGE_LOOP ( 'NONE', ( #54015, #359 ) ) ;
#47618=EDGE_CURVE ( 'NONE', #66479, #77917, #16543, .T. ) ;
#47619=CARTESIAN_POINT ( 'NONE',  ( 51.56670390244799762, -33.35206098992650681, 237.4678068554150059 ) ) ;
#47620=CARTESIAN_POINT ( 'NONE',  ( 136.2777084067157887, -35.08426318374723962, 2.472582314376420953 ) ) ;
#47622=CARTESIAN_POINT ( 'NONE',  ( 102.0686427141774999, -27.96957108712200224, 61.48992525579068058 ) ) ;
#47623=EDGE_CURVE ( 'NONE', #21126, #3091, #83544, .T. ) ;
#47624=CARTESIAN_POINT ( 'NONE',  ( 105.7147172347987407, -24.90567422487873017, 160.1670538473389627 ) ) ;
#47625=EDGE_LOOP ( 'NONE', ( #76325, #53569 ) ) ;
#47626=CARTESIAN_POINT ( 'NONE',  ( 71.25580610988301089, -82.12815647064930147, 542.9756252759101471 ) ) ;
#47628=VECTOR ( 'NONE', #42217, 1000.000000000000000 ) ;
#47629=CARTESIAN_POINT ( 'NONE',  ( 31.71315051186898870, -31.94127993907790852, 342.9256252759119548 ) ) ;
#47633=EDGE_CURVE ( 'NONE', #49139, #30320, #47650, .T. ) ;
#47634=ORIENTED_EDGE ( 'NONE', *, *, #49877, .T. ) ;
#47637=ORIENTED_EDGE ( 'NONE', *, *, #59716, .T. ) ;
#47640=CYLINDRICAL_SURFACE ( 'NONE', #9180, 9.999999999999998224 ) ;
#47641=DIRECTION ( 'NONE',  ( -1.000000000000000000, -2.756263715554006823E-15, 0.000000000000000000 ) ) ;
#47643=CARTESIAN_POINT ( 'NONE',  ( 97.06107716906868177, -37.99644359145901973, 106.4272944573947370 ) ) ;
#47645=CARTESIAN_POINT ( 'NONE',  ( 97.78492648218951899, -40.45146748447449170, 181.6299604809356936 ) ) ;
#47646=ORIENTED_EDGE ( 'NONE', *, *, #81057, .T. ) ;
#47650=LINE ( 'NONE', #38719, #10842 ) ;
#47651=DIRECTION ( 'NONE',  ( 1.000000000000000000, 4.299999999999999979E-14, 1.000000000000000078E-15 ) ) ;
#47653=CARTESIAN_POINT ( 'NONE',  ( 115.3120223323505940, -44.18753462406601074, 229.2413395616249545 ) ) ;
#47654=CARTESIAN_POINT ( 'NONE',  ( 107.0664832912750057, -36.72944715993903486, 4.925625275910970657 ) ) ;
#47656=VECTOR ( 'NONE', #56746, 1000.000000000000000 ) ;
#47657=CARTESIAN_POINT ( 'NONE',  ( 109.1197153606379828, -46.32621810461552059, 103.7441967044819791 ) ) ;
#47661=CARTESIAN_POINT ( 'NONE',  ( 97.39131739028603363, -39.27861223437267313, 22.53144478254995420 ) ) ;
#47662=ORIENTED_EDGE ( 'NONE', *, *, #48565, .T. ) ;
#47663=DIRECTION ( 'NONE',  ( 0.000000000000000000, 0.000000000000000000, -1.000000000000000000 ) ) ;
#47664=VECTOR ( 'NONE', #27092, 1000.000000000000000 ) ;
#47665=ORIENTED_EDGE ( 'NONE', *, *, #82236, .F. ) ;
#47667=EDGE_CURVE ( 'NONE', #44045, #70380, #89182, .T. ) ;
#47668=CARTESIAN_POINT ( 'NONE',  ( 115.7948931938460362, -35.19871557519451954, 240.3958690201829427 ) ) ;
#47669=CARTESIAN_POINT ( 'NONE',  ( 50.88849390559460062, -32.11662333284566273, 313.9678068554150059 ) ) ;
#47671=CARTESIAN_POINT ( 'NONE',  ( 97.81170668756638520, -40.51744870325870806, 152.6352702516163902 ) ) ;
#47672=VECTOR ( 'NONE', #33095, 1000.000000000000114 ) ;
#47673=LINE ( 'NONE', #19086, #83615 ) ;
#47676=CARTESIAN_POINT ( 'NONE',  ( 108.3318564647012607, -46.73503994553699670, 183.6777181701287418 ) ) ;
#47678=CARTESIAN_POINT ( 'NONE',  ( 114.8195649486642225, -43.69914982757761379, 38.24419670448192221 ) ) ;
#47680=CARTESIAN_POINT ( 'NONE',  ( 116.1392960594047850, -38.67366927644074082, 256.4766617981626382 ) ) ;
#47682=CARTESIAN_POINT ( 'NONE',  ( 103.1701080265564485, -27.72257962874988024, 155.4013395616259743 ) ) ;
#47685=CARTESIAN_POINT ( 'NONE',  ( 97.81170212845945855, -40.51743756719207568, 176.6354241348688277 ) ) ;
#47687=CARTESIAN_POINT ( 'NONE',  ( 96.97452011921430426, -33.94641660286638540, 247.1127681330539758 ) ) ;
#47688=DIRECTION ( 'NONE',  ( 0.000000000000000000, 1.000000000000000000, 0.000000000000000000 ) ) ;
#47690=EDGE_CURVE ( 'NONE', #5064, #82741, #43074, .T. ) ;
#47691=CARTESIAN_POINT ( 'NONE',  ( 98.42032043187158763, -42.69450228079005427, 122.8070538473389490 ) ) ;
#47693=VERTEX_POINT ( 'NONE', #9040 ) ;
#47694=VERTEX_POINT ( 'NONE', #70356 ) ;
#47695=ORIENTED_EDGE ( 'NONE', *, *, #1527, .T. ) ;
#47697=CARTESIAN_POINT ( 'NONE',  ( 51.06670390244899238, -32.29483332968430886, -5.074374724088000832 ) ) ;
#47698=CARTESIAN_POINT ( 'NONE',  ( 164.9667039024476765, -28.27351298636832055, 193.9678068554149775 ) ) ;
#47699=LINE ( 'NONE', #40453, #33049 ) ;
#47700=CARTESIAN_POINT ( 'NONE',  ( 111.5401709588312116, -43.55702686802507628, 175.8566617981629463 ) ) ;
#47701=CARTESIAN_POINT ( 'NONE',  ( 100.2339645716073164, -28.82666620644582522, 256.6441967044821695 ) ) ;
#47702=CARTESIAN_POINT ( 'NONE',  ( 115.7817526725759336, -41.80460064089260896, 59.40624582981430279 ) ) ;
#47703=ORIENTED_EDGE ( 'NONE', *, *, #47004, .F. ) ;
#47705=VECTOR ( 'NONE', #51421, 1000.000000000000000 ) ;
#47707=ORIENTED_EDGE ( 'NONE', *, *, #20989, .T. ) ;
#47710=CIRCLE ( 'NONE', #79655, 0.5000000000000004441 ) ;
#47711=DIRECTION ( 'NONE',  ( -1.000000000000000000, 0.000000000000000000, 7.043400939473319300E-33 ) ) ;
#47712=ORIENTED_EDGE ( 'NONE', *, *, #1802, .T. ) ;
#47713=ORIENTED_EDGE ( 'NONE', *, *, #80788, .F. ) ;
#47714=CARTESIAN_POINT ( 'NONE',  ( 131.0667039024480118, -43.72944715994093201, 231.5838068554170093 ) ) ;
#47715=CARTESIAN_POINT ( 'NONE',  ( 20.03715912545639100, -24.42818131006202265, 180.4678068554150911 ) ) ;
#47716=DIRECTION ( 'NONE',  ( 1.000000000000000000, 3.999999999999999995E-14, 1.000000000000000078E-15 ) ) ;
#47717=CYLINDRICAL_SURFACE ( 'NONE', #9811, 0.5000000000000129896 ) ;
#47718=EDGE_CURVE ( 'NONE', #49481, #47446, #36285, .T. ) ;
#47719=CARTESIAN_POINT ( 'NONE',  ( 99.99456525420680464, -31.07253584695887483, 195.2000388756959808 ) ) ;
#47720=CARTESIAN_POINT ( 'NONE',  ( 115.7096504343579539, -43.69425479293489900, 43.27467289495795200 ) ) ;
#47723=ORIENTED_EDGE ( 'NONE', *, *, #40845, .T. ) ;
#47725=EDGE_CURVE ( 'NONE', #593, #6607, #31137, .T. ) ;
#47727=ADVANCED_FACE ( 'NONE', ( #56711 ), #63082, .T. ) ;
#47729=CARTESIAN_POINT ( 'NONE',  ( 19.56648329127303043, 25.62155284005700295, 361.9756252759109998 ) ) ;
#47730=EDGE_CURVE ( 'NONE', #39083, #2908, #7680, .T. ) ;
#47732=LINE ( 'NONE', #68647, #18948 ) ;
#47736=ORIENTED_EDGE ( 'NONE', *, *, #26118, .T. ) ;
#47737=EDGE_CURVE ( 'NONE', #69807, #914, #63997, .T. ) ;
#47738=CARTESIAN_POINT ( 'NONE',  ( 106.5169308145888607, -25.66629059357601506, 45.12800622829193742 ) ) ;
#47739=CARTESIAN_POINT ( 'NONE',  ( 172.5664832912740110, -9.303447159940999356, 256.8086252759120498 ) ) ;
#47740=DIRECTION ( 'NONE',  ( 0.000000000000000000, 0.000000000000000000, 1.000000000000000000 ) ) ;
#47741=CARTESIAN_POINT ( 'NONE',  ( 97.33784347520764868, -34.07105638201832676, 147.1152944329917887 ) ) ;
#47743=ORIENTED_EDGE ( 'NONE', *, *, #37824, .T. ) ;
#47744=EDGE_CURVE ( 'NONE', #82504, #51804, #78084, .T. ) ;
#47745=VECTOR ( 'NONE', #27738, 1000.000000000000000 ) ;
#47746=DIRECTION ( 'NONE',  ( -9.073094938289460781E-13, -1.000000000000000000, 0.000000000000000000 ) ) ;
#47750=CARTESIAN_POINT ( 'NONE',  ( 102.5487710710870033, -27.30991770518087591, 91.43276813305395478 ) ) ;
#47752=CYLINDRICAL_SURFACE ( 'NONE', #47073, 2.500000000000002220 ) ;
#47754=CIRCLE ( 'NONE', #56441, 3.249999999999975131 ) ;
#47755=CARTESIAN_POINT ( 'NONE',  ( 51.23005224011641445, -33.89581943344366977, 117.4678068554150485 ) ) ;
#47756=ORIENTED_EDGE ( 'NONE', *, *, #72500, .T. ) ;
#47757=CARTESIAN_POINT ( 'NONE',  ( 96.70615320395842218, -37.17927570127480408, 112.3489586092439652 ) ) ;
#47759=ORIENTED_EDGE ( 'NONE', *, *, #58191, .T. ) ;
#47760=CARTESIAN_POINT ( 'NONE',  ( 110.9847977634195928, -46.36662828626490551, 278.8841967044824059 ) ) ;
#47761=DIRECTION ( 'NONE',  ( 0.000000000000000000, 0.000000000000000000, 1.000000000000000000 ) ) ;
#47762=CARTESIAN_POINT ( 'NONE',  ( 107.0664832912749915, -36.72944715993903486, 25.56312527591096995 ) ) ;
#47763=DIRECTION ( 'NONE',  ( 0.000000000000000000, 0.000000000000000000, -1.000000000000000000 ) ) ;
#47765=VECTOR ( 'NONE', #17277, 1000.000000000000000 ) ;
#47766=CARTESIAN_POINT ( 'NONE',  ( 152.4532657509292335, -72.54478064608022692, 394.9756252759102040 ) ) ;
#47767=DIRECTION ( 'NONE',  ( -1.000000000000000078E-15, 1.000000000000000083E-30, 1.000000000000000000 ) ) ;
#47768=CARTESIAN_POINT ( 'NONE',  ( 115.8019334949658798, -41.12891815432281817, 203.4556252759109611 ) ) ;
#47769=EDGE_LOOP ( 'NONE', ( #44586, #5383, #5051, #58119 ) ) ;
#47772=CIRCLE ( 'NONE', #39091, 2.500000000000002220 ) ;
#47773=CARTESIAN_POINT ( 'NONE',  ( 113.5614835896806625, -43.51851901557028413, 109.6034880678019618 ) ) ;
#47776=CARTESIAN_POINT ( 'NONE',  ( 116.3159835831961857, -41.41832011455023377, 244.4651490854349731 ) ) ;
#47778=DIRECTION ( 'NONE',  ( 0.1811243268507098381, -0.9834602067307437467, 0.000000000000000000 ) ) ;
#47779=ADVANCED_FACE ( 'NONE', ( #23127, #50799 ), #58064, .F. ) ;
#47780=CARTESIAN_POINT ( 'NONE',  ( 142.8679068202682458, 10.65431904611001634, 540.9756252759101471 ) ) ;
#47783=CARTESIAN_POINT ( 'NONE',  ( 97.07207205789896420, -35.37844120677264215, 107.2189586098578076 ) ) ;
#47784=CARTESIAN_POINT ( 'NONE',  ( 20.03715912545645850, -24.95799193693202156, 129.9678068554150627 ) ) ;
#47785=CARTESIAN_POINT ( 'NONE',  ( 114.1099639442526268, -29.07320488188160823, 199.4841967044819739 ) ) ;
#47788=ORIENTED_EDGE ( 'NONE', *, *, #83162, .F. ) ;
#47790=DIRECTION ( 'NONE',  ( 0.000000000000000000, 1.000000000000000000, 0.000000000000000000 ) ) ;
#47791=CARTESIAN_POINT ( 'NONE',  ( 97.81151477712479902, -40.51751189930152464, 186.6359914586728337 ) ) ;
#47793=CARTESIAN_POINT ( 'NONE',  ( 116.3212776292296127, -32.94146857471318413, 287.6356252759109680 ) ) ;
#47795=EDGE_CURVE ( 'NONE', #54206, #51053, #28561, .T. ) ;
#47797=VECTOR ( 'NONE', #31908, 1000.000000000000000 ) ;
#47798=CARTESIAN_POINT ( 'NONE',  ( 96.68196755257399388, -35.80810936406337674, 231.2556252759109725 ) ) ;
#47801=CARTESIAN_POINT ( 'NONE',  ( 142.8698897858160706, -0.9167816978817300289, 394.9756252759102040 ) ) ;
#47803=CARTESIAN_POINT ( 'NONE',  ( 110.8540353023265510, -45.98441608387823720, 167.8855877171093027 ) ) ;
#47804=CARTESIAN_POINT ( 'NONE',  ( 102.2720406957515991, -30.12315877573194101, 73.39380465530592801 ) ) ;
#47805=CARTESIAN_POINT ( 'NONE',  ( 113.6278897941700876, -45.65318799257786964, 179.0689586092439640 ) ) ;
#47806=DIRECTION ( 'NONE',  ( 1.000000000000000078E-15, 1.000000000000000083E-30, -1.000000000000000000 ) ) ;
#47807=ORIENTED_EDGE ( 'NONE', *, *, #78800, .F. ) ;
#47809=VECTOR ( 'NONE', #81456, 1000.000000000000000 ) ;
#47810=CARTESIAN_POINT ( 'NONE',  ( 98.51277055016676343, -41.91915478865436739, 66.76116378984684729 ) ) ;
#47811=ORIENTED_EDGE ( 'NONE', *, *, #83914, .T. ) ;
#47812=VERTEX_POINT ( 'NONE', #49442 ) ;
#47815=ORIENTED_EDGE ( 'NONE', *, *, #18951, .T. ) ;
#47816=LINE ( 'NONE', #55068, #3383 ) ;
#47817=ADVANCED_FACE ( 'NONE', ( #77177 ), #11249, .F. ) ;
#47818=CARTESIAN_POINT ( 'NONE',  ( 98.75426529987753099, -33.13504840779251737, 60.43622935188691514 ) ) ;
#47819=CARTESIAN_POINT ( 'NONE',  ( 111.1360948925329808, -27.10735667079447353, 244.7584824187679544 ) ) ;
#47820=AXIS2_PLACEMENT_3D ( 'NONE', #68696, #59616, #75513 ) ;
#47821=CARTESIAN_POINT ( 'NONE',  ( 115.4997179687694882, -29.61999039777954579, 224.3718157521009573 ) ) ;
#47822=DIRECTION ( 'NONE',  ( 0.000000000000000000, 0.000000000000000000, 1.000000000000000000 ) ) ;
#47823=CARTESIAN_POINT ( 'NONE',  ( 99.16013801855510224, -43.49098322490559809, 27.88991099019694175 ) ) ;
#47826=EDGE_CURVE ( 'NONE', #41907, #17571, #65331, .T. ) ;
#47828=AXIS2_PLACEMENT_3D ( 'NONE', #13366, #54214, #41053 ) ;
#47831=AXIS2_PLACEMENT_3D ( 'NONE', #25841, #27624, #20816 ) ;
#47832=CARTESIAN_POINT ( 'NONE',  ( 106.8551140066829817, -47.84553036069068099, 77.56133956162591403 ) ) ;
#47833=CARTESIAN_POINT ( 'NONE',  ( 97.22485937713641135, -31.59570365635885736, 90.93181575210196854 ) ) ;
#47834=CARTESIAN_POINT ( 'NONE',  ( 100.8220609092773117, -45.17687181127147511, 257.0699109901966608 ) ) ;
#47836=CARTESIAN_POINT ( 'NONE',  ( 109.3369124252947557, -26.55437064873915531, 224.9013395616249511 ) ) ;
#47837=FACE_OUTER_BOUND ( 'NONE', #28961, .T. ) ;
#47838=CARTESIAN_POINT ( 'NONE',  ( 82.81670390244799762, -50.82844715994100682, 250.9178068554150514 ) ) ;
#47839=DIRECTION ( 'NONE',  ( -2.999999999999999839E-15, 1.000000000000000000, -2.999999999999999900E-30 ) ) ;
#47840=LINE ( 'NONE', #89658, #28214 ) ;
#47841=CARTESIAN_POINT ( 'NONE',  ( 98.72346068757417470, -34.40322473509486656, 277.6356252759111385 ) ) ;
#47842=DIRECTION ( 'NONE',  ( 9.912705577010326536E-16, 1.000000000000000000, 0.000000000000000000 ) ) ;
#47843=CARTESIAN_POINT ( 'NONE',  ( 97.92324767642672612, -40.78073790739274074, 172.6583826592236051 ) ) ;
#47846=EDGE_CURVE ( 'NONE', #66586, #56062, #3544, .T. ) ;
#47853=VERTEX_POINT ( 'NONE', #44418 ) ;
#47855=CARTESIAN_POINT ( 'NONE',  ( 97.14868559305091367, -40.01329441332335790, 241.5813395616249863 ) ) ;
#47856=CARTESIAN_POINT ( 'NONE',  ( 102.3127581962668273, -26.75066580571964536, 136.4422919425779526 ) ) ;
#47857=CARTESIAN_POINT ( 'NONE',  ( 97.57588284487002284, -41.14775938459609250, 252.6727681330536655 ) ) ;
#47858=CIRCLE ( 'NONE', #27584, 2.500000000000002220 ) ;
#47859=LINE ( 'NONE', #75596, #20032 ) ;
#47861=DIRECTION ( 'NONE',  ( 0.000000000000000000, 0.000000000000000000, -1.000000000000000000 ) ) ;
#47862=CARTESIAN_POINT ( 'NONE',  ( 176.7738106835053031, -48.62134037887501137, 180.4678068554150059 ) ) ;
#47863=DIRECTION ( 'NONE',  ( -1.000000000000000000, 1.011922027653136551E-15, 0.000000000000000000 ) ) ;
#47864=B_SPLINE_CURVE_WITH_KNOTS ( 'NONE', 3,
 ( #46941, #88322, #6525, #26521, #26080, #47389, #53745, #33780, #12905, #40594, #61476, #68310, #89208, #34222, #43719, #56906, #14696, #48727, #42814, #28767, #21055, #43268, #15595, #84642, #83289, #57349, #16042 ),
 .UNSPECIFIED., .F., .F.,
 ( 4, 2, 2, 2, 2, 2, 2, 2, 2, 2, 1, 1, 1, 2, 4 ),
 ( 0.000000000000000000, 0.06249619433354525883, 0.1249923886670905177, 0.1874885830006357557, 0.2499847773341810353, 0.3124809716677263149, 0.3749771660012715113, 0.4374733603348168187, 0.4687214575015891116, 0.4843455060849753968, 0.4921575303766683729, 0.4960635425225149997, 0.4980165485954382576, 0.4989930516318998310, 0.4999695546683612934 ),
 .UNSPECIFIED. ) ;
#47868=CARTESIAN_POINT ( 'NONE',  ( 115.0376279413645761, -33.66073653188622927, 138.5409912566489652 ) ) ;
#47869=DIRECTION ( 'NONE',  ( 0.000000000000000000, 1.000000000000000000, 0.000000000000000000 ) ) ;
#47870=EDGE_LOOP ( 'NONE', ( #53517, #74378, #52063, #59113, #38315 ) ) ;
#47872=CARTESIAN_POINT ( 'NONE',  ( 113.6005200848514107, -45.61596423689125146, 179.0689586092439640 ) ) ;
#47873=CARTESIAN_POINT ( 'NONE',  ( 97.81219807385008380, -40.51719912245609123, 147.6362401243850115 ) ) ;
#47877=CARTESIAN_POINT ( 'NONE',  ( 98.75024281215304711, -42.92452016420553917, 111.8480062282929737 ) ) ;
#47881=CARTESIAN_POINT ( 'NONE',  ( 46.03715912545433753, -48.62818131006086020, 237.4678068554150059 ) ) ;
#47882=CARTESIAN_POINT ( 'NONE',  ( 116.6769215743979800, -34.91203320259896259, 154.9756252759109714 ) ) ;
#47884=CARTESIAN_POINT ( 'NONE',  ( 115.8259315161528775, -31.73088453253794583, 54.23961552823458021 ) ) ;
#47885=FACE_OUTER_BOUND ( 'NONE', #14046, .T. ) ;
#47886=EDGE_CURVE ( 'NONE', #5969, #46964, #64481, .T. ) ;
#47887=CARTESIAN_POINT ( 'NONE',  ( 48.79742451362098166, -36.32844715994040996, -5.074374724088000832 ) ) ;
#47889=CARTESIAN_POINT ( 'NONE',  ( 73.06670390244801183, -48.82844715994099971, 310.9178068554150514 ) ) ;
#47890=CARTESIAN_POINT ( 'NONE',  ( 97.81169128372820865, -40.51741339292117772, 177.6357569005977268 ) ) ;
#47891=CARTESIAN_POINT ( 'NONE',  ( 110.1514708964275968, -46.66481413883396812, 97.81562527591097478 ) ) ;
#47892=EDGE_LOOP ( 'NONE', ( #21735, #57234 ) ) ;
#47893=ORIENTED_EDGE ( 'NONE', *, *, #11350, .T. ) ;
#47897=CARTESIAN_POINT ( 'NONE',  ( 111.5401709588312116, -43.55702686802507628, 175.8566617981629463 ) ) ;
#47899=ADVANCED_FACE ( 'NONE', ( #72152 ), #67108, .T. ) ;
#47901=ORIENTED_EDGE ( 'NONE', *, *, #45759, .T. ) ;
#47902=VERTEX_POINT ( 'NONE', #52110 ) ;
#47903=ORIENTED_EDGE ( 'NONE', *, *, #25905, .T. ) ;
#47904=VECTOR ( 'NONE', #51279, 1000.000000000000000 ) ;
#47905=FACE_OUTER_BOUND ( 'NONE', #25707, .T. ) ;
#47906=CARTESIAN_POINT ( 'NONE',  ( 134.4433815842287174, -21.47944715994100306, 1.625625275910998813 ) ) ;
#47907=ORIENTED_EDGE ( 'NONE', *, *, #66782, .F. ) ;
#47908=ORIENTED_EDGE ( 'NONE', *, *, #72075, .F. ) ;
#47909=CARTESIAN_POINT ( 'NONE',  ( 77.38816033347450229, -19.35482103167604251, 6.853567712192048411 ) ) ;
#47911=CARTESIAN_POINT ( 'NONE',  ( 114.2010777387499587, -30.61601215110631458, 225.8339642582779447 ) ) ;
#47912=ADVANCED_FACE ( 'NONE', ( #9928 ), #32580, .F. ) ;
#47917=VERTEX_POINT ( 'NONE', #45741 ) ;
#47918=CARTESIAN_POINT ( 'NONE',  ( 31.85959712127300847, -23.19206098994092002, 342.9256252759109884 ) ) ;
#47919=EDGE_LOOP ( 'NONE', ( #22038, #39387 ) ) ;
#47920=ORIENTED_EDGE ( 'NONE', *, *, #35418, .T. ) ;
#47923=CARTESIAN_POINT ( 'NONE',  ( 106.9677948388671069, -45.38341651713141545, 230.3976141791149814 ) ) ;
#47924=CARTESIAN_POINT ( 'NONE',  ( 114.2552021840540846, -45.16177683379865471, 153.1508633711489722 ) ) ;
#47925=VECTOR ( 'NONE', #86105, 999.9999999999998863 ) ;
#47926=CARTESIAN_POINT ( 'NONE',  ( 97.95167206076190780, -31.64175201202206011, 110.9213395616259703 ) ) ;
#47927=CARTESIAN_POINT ( 'NONE',  ( 111.1206699024608753, -28.37365878809221797, 249.5838068554168387 ) ) ;
#47929=CARTESIAN_POINT ( 'NONE',  ( 115.0396333253530230, -29.07419673827904916, 185.4232443235299570 ) ) ;
#47930=EDGE_CURVE ( 'NONE', #37091, #52002, #66659, .T. ) ;
#47932=ORIENTED_EDGE ( 'NONE', *, *, #14718, .T. ) ;
#47933=FACE_OUTER_BOUND ( 'NONE', #89701, .T. ) ;
#47935=VERTEX_POINT ( 'NONE', #78975 ) ;
#47937=VECTOR ( 'NONE', #71727, 1000.000000000000000 ) ;
#47938=ORIENTED_EDGE ( 'NONE', *, *, #41724, .F. ) ;
#47940=CARTESIAN_POINT ( 'NONE',  ( 101.7107321646854246, -27.74380102040660390, 85.50419670448295051 ) ) ;
#47942=CARTESIAN_POINT ( 'NONE',  ( 136.6789756616809655, -35.84952872352904762, 6.945088388040495886 ) ) ;
#47943=CARTESIAN_POINT ( 'NONE',  ( 107.0667039024479834, -36.72944715994099596, 239.5838068554170093 ) ) ;
#47946=CARTESIAN_POINT ( 'NONE',  ( 103.7301789885933943, -26.21598454391068600, 201.3089586092439731 ) ) ;
#47948=DIRECTION ( 'NONE',  ( -1.000000000000000078E-15, 0.000000000000000000, 1.000000000000000000 ) ) ;
#47952=CARTESIAN_POINT ( 'NONE',  ( 151.0371591254575776, -24.42818131005592264, 129.9678068554149775 ) ) ;
#47953=ADVANCED_FACE ( 'NONE', ( #58937, #45309, #37633, #65757, #3109, #58499, #86227 ), #24005, .T. ) ;
#47955=AXIS2_PLACEMENT_3D ( 'NONE', #7915, #7021, #70600 ) ;
#47956=ADVANCED_FACE ( 'NONE', ( #52555 ), #32133, .T. ) ;
#47958=CARTESIAN_POINT ( 'NONE',  ( 141.0664832912740394, -46.72944715994099596, -4.824374724088994704 ) ) ;
#47959=VECTOR ( 'NONE', #55254, 1000.000000000000000 ) ;
#47960=CARTESIAN_POINT ( 'NONE',  ( 112.4772085026190354, -45.73365988577116070, 238.0070538473389377 ) ) ;
#47963=CARTESIAN_POINT ( 'NONE',  ( 96.00433110544545912, -37.29885927265511469, 121.3794347997209684 ) ) ;
#47964=CARTESIAN_POINT ( 'NONE',  ( 104.7356836917145699, -47.53413844247978659, 28.41943479971997988 ) ) ;
#47965=CARTESIAN_POINT ( 'NONE',  ( 97.96923373944615321, -30.37039525599472256, 156.8289586092439549 ) ) ;
#47966=EDGE_CURVE ( 'NONE', #7132, #59432, #88913, .T. ) ;
#47967=DIRECTION ( 'NONE',  ( -0.9254794337955620787, -0.3787978585227822492, 0.000000000000000000 ) ) ;
#47970=DIRECTION ( 'NONE',  ( -4.237773401492740281E-14, 1.000000000000000000, 0.000000000000000000 ) ) ;
#47973=EDGE_LOOP ( 'NONE', ( #71857, #60244, #42003, #45329, #45686, #73234, #24910, #21484, #7279, #38065, #23487, #17670, #39886, #46315 ) ) ;
#47974=VECTOR ( 'NONE', #388, 1000.000000000000000 ) ;
#47975=ORIENTED_EDGE ( 'NONE', *, *, #14644, .F. ) ;
#47976=ORIENTED_EDGE ( 'NONE', *, *, #61192, .T. ) ;
#47977=AXIS2_PLACEMENT_3D ( 'NONE', #21257, #56654, #22167 ) ;
#47978=ORIENTED_EDGE ( 'NONE', *, *, #50186, .T. ) ;
#47979=CARTESIAN_POINT ( 'NONE',  ( 107.0664832912740394, -56.47944715994103149, -5.074374724089029343 ) ) ;
#47980=CARTESIAN_POINT ( 'NONE',  ( 115.9265467165007379, -42.18176083994490000, 14.38705384733995984 ) ) ;
#47981=DIRECTION ( 'NONE',  ( 0.000000000000000000, 1.000000000000000000, 0.000000000000000000 ) ) ;
#47982=AXIS2_PLACEMENT_3D ( 'NONE', #89883, #13124, #61691 ) ;
#47983=DIRECTION ( 'NONE',  ( 1.000000000000000078E-15, -1.000000000000000083E-30, -1.000000000000000000 ) ) ;
#47985=CARTESIAN_POINT ( 'NONE',  ( 115.6071762752661130, -36.01623928086704041, 253.3152769709339793 ) ) ;
#47987=VERTEX_POINT ( 'NONE', #53448 ) ;
#47988=ORIENTED_EDGE ( 'NONE', *, *, #77282, .F. ) ;
#47990=CARTESIAN_POINT ( 'NONE',  ( 114.0075790447407087, -33.88846322102013175, -1.864374724089012947 ) ) ;
#47991=CARTESIAN_POINT ( 'NONE',  ( 172.5664832912729878, -27.57844715994070484, 195.9256252759119832 ) ) ;
#47996=VECTOR ( 'NONE', #57716, 1000.000000000000000 ) ;
#47998=CARTESIAN_POINT ( 'NONE',  ( 97.40014589274343848, -35.23768424668791965, 266.2041967044829676 ) ) ;
#48001=CARTESIAN_POINT ( 'NONE',  ( 41.56648329127399677, -18.82844715994099971, 18.92562527591200094 ) ) ;
#48002=AXIS2_PLACEMENT_3D ( 'NONE', #36911, #77811, #50531 ) ;
#48004=CARTESIAN_POINT ( 'NONE',  ( 100.4744175226576886, -42.33708426910433076, 74.71761417911493197 ) ) ;
#48005=VECTOR ( 'NONE', #30075, 1000.000000000000114 ) ;
#48007=ADVANCED_FACE ( 'NONE', ( #74381 ), #61625, .F. ) ;
#48009=CARTESIAN_POINT ( 'NONE',  ( 97.81169607051373305, -40.51742273377266912, 46.63562653399714009 ) ) ;
#48011=EDGE_CURVE ( 'NONE', #2214, #16775, #47091, .T. ) ;
#48012=CARTESIAN_POINT ( 'NONE',  ( 193.5667039024414464, -48.82844715994099971, 300.4678068554149490 ) ) ;
#48014=CARTESIAN_POINT ( 'NONE',  ( 117.0233241640237338, -39.93681227152024604, 158.5784824187679476 ) ) ;
#48015=ORIENTED_EDGE ( 'NONE', *, *, #72041, .T. ) ;
#48016=EDGE_CURVE ( 'NONE', #48511, #83239, #76145, .T. ) ;
#48017=AXIS2_PLACEMENT_3D ( 'NONE', #63330, #648, #83788 ) ;
#48019=CARTESIAN_POINT ( 'NONE',  ( 97.67976800739046439, -37.13700294324897300, 112.7806309249449441 ) ) ;
#48021=B_SPLINE_CURVE_WITH_KNOTS ( 'NONE', 3,
 ( #36756, #29946, #85373, #23148, #50821, #78557, #43990, #88033, #74398, #80331, #18078, #67581, #47115, #68028, #53922, #60300, #25340, #26684 ),
 .UNSPECIFIED., .F., .F.,
 ( 4, 2, 2, 2, 2, 2, 2, 2, 4 ),
 ( 0.000000000000000000, 0.06250343988587346578, 0.1250068797717469316, 0.1875103196576203834, 0.2500137595434938631, 0.3125171994293673428, 0.3750206393152407669, 0.4375240792011142466, 0.5000275190869877262 ),
 .UNSPECIFIED. ) ;
#48022=DIRECTION ( 'NONE',  ( 0.000000000000000000, 0.000000000000000000, -1.000000000000000000 ) ) ;
#48023=FACE_OUTER_BOUND ( 'NONE', #52106, .T. ) ;
#48024=CARTESIAN_POINT ( 'NONE',  ( 96.31605362642591217, -41.77429727756310740, 57.67562527591096710 ) ) ;
#48026=EDGE_CURVE ( 'NONE', #18171, #2091, #75725, .T. ) ;
#48027=CARTESIAN_POINT ( 'NONE',  ( 116.3199495083284347, -32.94194616109231077, 85.13562527591095375 ) ) ;
#48029=DIRECTION ( 'NONE',  ( 2.900000000000000265E-14, -2.000000000000000155E-15, 1.000000000000000000 ) ) ;
#48034=DIRECTION ( 'NONE',  ( 0.000000000000000000, 0.000000000000000000, -1.000000000000000000 ) ) ;
#48035=ORIENTED_EDGE ( 'NONE', *, *, #25593, .T. ) ;
#48036=CARTESIAN_POINT ( 'NONE',  ( 117.3624379696767335, -35.49166588079122420, 238.9337205140069500 ) ) ;
#48037=CARTESIAN_POINT ( 'NONE',  ( 117.0439256081559165, -39.94344854842797332, 154.5784824187679476 ) ) ;
#48039=CARTESIAN_POINT ( 'NONE',  ( 168.5667039024486087, -48.82844715993516616, 129.9678068554150059 ) ) ;
#48040=CARTESIAN_POINT ( 'NONE',  ( 98.64735160015825954, -43.89130460420365409, 72.89943479972099283 ) ) ;
#48041=CIRCLE ( 'NONE', #8933, 5.599999999999994316 ) ;
#48042=ADVANCED_FACE ( 'NONE', ( #68464, #40296 ), #54345, .T. ) ;
#48046=CARTESIAN_POINT ( 'NONE',  ( 116.3262419368496978, -32.93860311337579105, 160.1356252759109680 ) ) ;
#48047=ORIENTED_EDGE ( 'NONE', *, *, #18499, .T. ) ;
#48048=LINE ( 'NONE', #53506, #86669 ) ;
#48050=CARTESIAN_POINT ( 'NONE',  ( 164.7812970173289955, -35.65087443492610930, -5.074374724088000832 ) ) ;
#48051=CARTESIAN_POINT ( 'NONE',  ( 106.8369185487093063, -47.13021470646874178, 272.5584824187680510 ) ) ;
#48053=DIRECTION ( 'NONE',  ( 1.387778780781444492E-15, 0.000000000000000000, -1.000000000000000000 ) ) ;
#48054=CARTESIAN_POINT ( 'NONE',  ( 104.4095340282210600, -46.45850909292975217, 92.36551864622379071 ) ) ;
#48055=CARTESIAN_POINT ( 'NONE',  ( 116.7468388360755966, -38.12735696270561903, 28.71276813305495423 ) ) ;
#48056=CARTESIAN_POINT ( 'NONE',  ( 111.3508018702361682, -27.66482620347798616, 99.72597377253785567 ) ) ;
#48057=CARTESIAN_POINT ( 'NONE',  ( 103.2134869792596135, -46.43093390711685231, 113.2756252759109827 ) ) ;
#48059=CARTESIAN_POINT ( 'NONE',  ( 97.91784736035330639, -30.44332401329681659, 165.8594347997199634 ) ) ;
#48061=VERTEX_POINT ( 'NONE', #6238 ) ;
#48062=LINE ( 'NONE', #74452, #3378 ) ;
#48063=AXIS2_PLACEMENT_3D ( 'NONE', #62060, #48407, #76140 ) ;
#48065=FACE_OUTER_BOUND ( 'NONE', #15793, .T. ) ;
#48066=ORIENTED_EDGE ( 'NONE', *, *, #23759, .F. ) ;
#48068=LINE ( 'NONE', #75802, #31670 ) ;
#48069=CARTESIAN_POINT ( 'NONE',  ( 97.79690410337100559, -31.86307605613059835, 135.9413395616259947 ) ) ;
#48071=LINE ( 'NONE', #41259, #47974 ) ;
#48072=ADVANCED_FACE ( 'NONE', ( #40738 ), #18964, .T. ) ;
#48073=DIRECTION ( 'NONE',  ( 1.000000000000000000, 4.163336342344333240E-14, 0.000000000000000000 ) ) ;
#48078=AXIS2_PLACEMENT_3D ( 'NONE', #13104, #76666, #61232 ) ;
#48080=VERTEX_POINT ( 'NONE', #67559 ) ;
#48081=VERTEX_POINT ( 'NONE', #82563 ) ;
#48086=CARTESIAN_POINT ( 'NONE',  ( 149.4532656544377289, -72.54365454176046057, 394.9756252759100903 ) ) ;
#48091=EDGE_LOOP ( 'NONE', ( #81557, #82882, #7318, #46485 ) ) ;
#48092=PLANE ( 'NONE',  #39817 ) ;
#48093=LINE ( 'NONE', #89924, #18742 ) ;
#48094=CARTESIAN_POINT ( 'NONE',  ( 99.44473759953889669, -30.59981194223820467, 236.7870538473389388 ) ) ;
#48095=AXIS2_PLACEMENT_3D ( 'NONE', #46719, #34891, #62601 ) ;
#48096=FACE_OUTER_BOUND ( 'NONE', #58272, .T. ) ;
#48097=CARTESIAN_POINT ( 'NONE',  ( 114.7041265136727901, -43.74408836545391921, 74.22324432352993995 ) ) ;
#48098=DIRECTION ( 'NONE',  ( -0.9254794337955620787, -0.3787978585227822492, 0.000000000000000000 ) ) ;
#48099=CARTESIAN_POINT ( 'NONE',  ( 106.5507326060560729, -26.72133602940400721, 21.11751855259041477 ) ) ;
#48106=CARTESIAN_POINT ( 'NONE',  ( 97.88747888210261294, -34.72385408216754143, 252.5749166392305938 ) ) ;
#48109=EDGE_CURVE ( 'NONE', #28751, #56395, #79079, .T. ) ;
#48110=EDGE_CURVE ( 'NONE', #54206, #14514, #33036, .T. ) ;
#48111=DIRECTION ( 'NONE',  ( -8.839355291601565315E-16, -1.000000000000000000, 0.000000000000000000 ) ) ;
#48113=VERTEX_POINT ( 'NONE', #13943 ) ;
#48115=ADVANCED_FACE ( 'NONE', ( #69363 ), #71809, .T. ) ;
#48116=CARTESIAN_POINT ( 'NONE',  ( 95.64925804648841279, -35.75026674902539980, 296.0306255462182321 ) ) ;
#48117=ORIENTED_EDGE ( 'NONE', *, *, #31412, .T. ) ;
#48118=CARTESIAN_POINT ( 'NONE',  ( 96.19295485998075890, -38.71576710077270889, 51.48229194257797303 ) ) ;
#48120=CARTESIAN_POINT ( 'NONE',  ( 99.11752347482735104, -34.75543446931638414, 273.9509475124486357 ) ) ;
#48121=EDGE_CURVE ( 'NONE', #38148, #19807, #77377, .T. ) ;
#48123=CARTESIAN_POINT ( 'NONE',  ( 113.4245949246308243, -29.25360672088980962, 139.5156252759109634 ) ) ;
#48124=FACE_OUTER_BOUND ( 'NONE', #71627, .T. ) ;
#48125=DIRECTION ( 'NONE',  ( 0.000000000000000000, -1.000000000000000000, 0.000000000000000000 ) ) ;
#48126=CARTESIAN_POINT ( 'NONE',  ( 165.2725846195387476, -35.55794170701241796, 313.9678068554149490 ) ) ;
#48127=AXIS2_PLACEMENT_3D ( 'NONE', #41710, #74464, #13141 ) ;
#48129=CARTESIAN_POINT ( 'NONE',  ( 116.9258602667948566, -41.82750404599077854, 239.4346728949589647 ) ) ;
#48130=FACE_OUTER_BOUND ( 'NONE', #11177, .T. ) ;
#48131=EDGE_CURVE ( 'NONE', #28391, #30630, #14857, .T. ) ;
#48133=AXIS2_PLACEMENT_3D ( 'NONE', #30202, #8880, #56549 ) ;
#48134=ORIENTED_EDGE ( 'NONE', *, *, #24575, .T. ) ;
#48135=CARTESIAN_POINT ( 'NONE',  ( 108.3246818025246654, -47.12222909040148267, 113.6727681330539639 ) ) ;
#48138=ORIENTED_EDGE ( 'NONE', *, *, #46478, .F. ) ;
#48143=DIRECTION ( 'NONE',  ( 0.000000000000000000, 0.000000000000000000, 1.000000000000000000 ) ) ;
#48144=CARTESIAN_POINT ( 'NONE',  ( 172.5664832912740110, -36.32844715994070839, 258.9256252759120116 ) ) ;
#48145=CARTESIAN_POINT ( 'NONE',  ( 112.1548083954980939, -43.14751820055241893, 165.9280903695909615 ) ) ;
#48146=CARTESIAN_POINT ( 'NONE',  ( 105.0174007254451567, -25.84429900004466063, 276.2365776568634033 ) ) ;
#48147=AXIS2_PLACEMENT_3D ( 'NONE', #62100, #56165, #27586 ) ;
#48148=ADVANCED_FACE ( 'NONE', ( #8940 ), #36639, .T. ) ;
#48149=CARTESIAN_POINT ( 'NONE',  ( 97.81936407165393632, -40.53612711470664465, 57.63723432799564250 ) ) ;
#48152=CARTESIAN_POINT ( 'NONE',  ( 134.0664832912740110, -8.729447159940999512, 4.925625275911999168 ) ) ;
#48153=EDGE_LOOP ( 'NONE', ( #39243, #64895, #56369, #30955, #76695, #26894, #64920 ) ) ;
#48155=ORIENTED_EDGE ( 'NONE', *, *, #81484, .T. ) ;
#48157=DIRECTION ( 'NONE',  ( 0.000000000000000000, 0.000000000000000000, -1.000000000000000000 ) ) ;
#48159=ORIENTED_EDGE ( 'NONE', *, *, #81492, .T. ) ;
#48163=CARTESIAN_POINT ( 'NONE',  ( 194.0371591254575776, -24.89890238294407254, 129.9678068554150343 ) ) ;
#48164=CARTESIAN_POINT ( 'NONE',  ( 113.5378671157686910, -31.15474330070945541, 183.8152769709339793 ) ) ;
#48166=CARTESIAN_POINT ( 'NONE',  ( 107.8717536863088640, -26.29114242999935769, 70.01562527591099183 ) ) ;
#48167=FACE_OUTER_BOUND ( 'NONE', #258, .T. ) ;
#48170=CIRCLE ( 'NONE', #6128, 15.84999999999999964 ) ;
#48171=EDGE_LOOP ( 'NONE', ( #34862, #57940, #67093, #53941 ) ) ;
#48172=CARTESIAN_POINT ( 'NONE',  ( 104.4889533838145752, -26.97908276471815370, 261.2814877649475989 ) ) ;
#48173=ORIENTED_EDGE ( 'NONE', *, *, #61971, .T. ) ;
#48176=EDGE_CURVE ( 'NONE', #68890, #89686, #73274, .T. ) ;
#48177=DIRECTION ( 'NONE',  ( 0.000000000000000000, 0.000000000000000000, -1.000000000000000000 ) ) ;
#48178=CARTESIAN_POINT ( 'NONE',  ( 147.9173672921288869, -72.54391775211570348, 542.9756252759101471 ) ) ;
#48179=ORIENTED_EDGE ( 'NONE', *, *, #81713, .F. ) ;
#48180=CARTESIAN_POINT ( 'NONE',  ( 115.6294417704117734, -28.50085323451786579, 39.43562527591099354 ) ) ;
#48183=DIRECTION ( 'NONE',  ( 0.000000000000000000, 1.000000000000000000, 0.000000000000000000 ) ) ;
#48184=CARTESIAN_POINT ( 'NONE',  ( 177.0371591254545649, -48.62818131005479927, 180.4678068554150059 ) ) ;
#48185=CARTESIAN_POINT ( 'NONE',  ( 133.6895842087692756, -15.97944715994100839, 1.625625275910996814 ) ) ;
#48186=ORIENTED_EDGE ( 'NONE', *, *, #24770, .T. ) ;
#48193=CARTESIAN_POINT ( 'NONE',  ( 113.3555096308132022, -27.61169779702804306, 85.60800622829195561 ) ) ;
#48194=DIRECTION ( 'NONE',  ( -1.000000000000000000, 0.000000000000000000, 0.000000000000000000 ) ) ;
#48195=DIRECTION ( 'NONE',  ( 0.000000000000000000, 0.000000000000000000, -1.000000000000000000 ) ) ;
#48197=AXIS2_PLACEMENT_3D ( 'NONE', #35516, #84150, #75194 ) ;
#48198=EDGE_CURVE ( 'NONE', #78594, #7132, #35537, .T. ) ;
#48201=CARTESIAN_POINT ( 'NONE',  ( 102.3899016914588884, -28.13915478247121271, 141.4727681330539895 ) ) ;
#48203=ORIENTED_EDGE ( 'NONE', *, *, #71001, .F. ) ;
#48204=CARTESIAN_POINT ( 'NONE',  ( 105.1131368864170526, -25.87365329830177529, 271.2061014663872243 ) ) ;
#48206=DIRECTION ( 'NONE',  ( 0.7071067811865525687, -0.7071067811865425767, 7.071067811865533512E-16 ) ) ;
#48209=AXIS2_PLACEMENT_3D ( 'NONE', #86483, #79676, #9277 ) ;
#48212=CARTESIAN_POINT ( 'NONE',  ( 112.6540662323892263, -44.79745133516141209, 203.0584824187689605 ) ) ;
#48213=VERTEX_POINT ( 'NONE', #69810 ) ;
#48214=ORIENTED_EDGE ( 'NONE', *, *, #87360, .T. ) ;
#48215=CARTESIAN_POINT ( 'NONE',  ( 112.6324721509601545, -29.83393797428842831, 160.9672975916109579 ) ) ;
#48218=CARTESIAN_POINT ( 'NONE',  ( 104.7413546109693527, -27.22895552020974108, 281.2670538473389570 ) ) ;
#48219=DIRECTION ( 'NONE',  ( -0.000000000000000000, -0.000000000000000000, 1.000000000000000000 ) ) ;
#48224=CARTESIAN_POINT ( 'NONE',  ( 107.0664832912739399, -36.72944715994095333, 312.6356252759112522 ) ) ;
#48225=CARTESIAN_POINT ( 'NONE',  ( 104.4899544478337248, -26.97880758572692272, 106.2814586095817333 ) ) ;
#48226=EDGE_CURVE ( 'NONE', #36063, #55559, #57509, .T. ) ;
#48227=CARTESIAN_POINT ( 'NONE',  ( 79.06648329127300201, -36.72944715994189835, 342.9256252759109884 ) ) ;
#48228=CARTESIAN_POINT ( 'NONE',  ( 99.10268845779062019, -29.98093639561593449, 215.7670538473399517 ) ) ;
#48229=CARTESIAN_POINT ( 'NONE',  ( 115.8264358448934246, -31.73174211693571678, 169.2397684523309067 ) ) ;
#48230=ORIENTED_EDGE ( 'NONE', *, *, #61194, .T. ) ;
#48231=EDGE_LOOP ( 'NONE', ( #12302, #27044, #88278, #84406 ) ) ;
#48233=CARTESIAN_POINT ( 'NONE',  ( 118.5256205435842958, -36.72944715994096754, 296.0306255462182321 ) ) ;
#48234=CARTESIAN_POINT ( 'NONE',  ( 81.77795131945210017, -20.88977919473711964, 7.751962620062596621 ) ) ;
#48235=B_SPLINE_CURVE_WITH_KNOTS ( 'NONE', 3,
 ( #32114, #73907, #72129, #87099, #51209, #18041, #31673, #3090, #17168, #45289, #45722, #52973, #23546, #52091, #44850, #37611, #30786, #78952 ),
 .UNSPECIFIED., .F., .F.,
 ( 4, 2, 2, 2, 2, 2, 2, 2, 4 ),
 ( 0.000000000000000000, 0.06250044056969467077, 0.1250008811393893415, 0.1875013217090840123, 0.2500017622787786831, 0.3125022028484733538, 0.3750026434181680246, 0.4375030839878626954, 0.5000035245575573661 ),
 .UNSPECIFIED. ) ;
#48238=DIRECTION ( 'NONE',  ( -0.7071067811985214391, 0.7071067811745735954, 0.000000000000000000 ) ) ;
#48239=VERTEX_POINT ( 'NONE', #16195 ) ;
#48240=CARTESIAN_POINT ( 'NONE',  ( 96.61551125061282619, -32.99117460050268846, 22.06514908543494258 ) ) ;
#48241=CARTESIAN_POINT ( 'NONE',  ( 95.29485650985192535, -38.09666651163277606, 236.4184824187679510 ) ) ;
#48244=VECTOR ( 'NONE', #82885, 1000.000000000000114 ) ;
#48247=CARTESIAN_POINT ( 'NONE',  ( 110.8552107763470644, -45.98393496479614129, 167.8856887709574721 ) ) ;
#48248=CARTESIAN_POINT ( 'NONE',  ( 111.5100823108406587, -29.30278217496053017, 52.47761417911495130 ) ) ;
#48249=CARTESIAN_POINT ( 'NONE',  ( 96.62828407576300549, -37.15518013270143172, 157.3584824187679487 ) ) ;
#48250=DIRECTION ( 'NONE',  ( 0.000000000000000000, -1.000000000000000000, 0.000000000000000000 ) ) ;
#48251=ORIENTED_EDGE ( 'NONE', *, *, #22634, .T. ) ;
#48252=DIRECTION ( 'NONE',  ( 0.000000000000000000, 0.000000000000000000, 1.000000000000000000 ) ) ;
#48255=AXIS2_PLACEMENT_3D ( 'NONE', #33637, #32277, #38653 ) ;
#48257=VERTEX_POINT ( 'NONE', #55684 ) ;
#48259=CARTESIAN_POINT ( 'NONE',  ( 107.0664832912748068, -36.72944715993923381, 14.92562527591097066 ) ) ;
#48260=CARTESIAN_POINT ( 'NONE',  ( 102.5065049712838601, -29.50707016595331567, 109.9467055423629631 ) ) ;
#48261=CARTESIAN_POINT ( 'NONE',  ( 96.10188529952328906, -35.15685947849579662, 226.2251490854349640 ) ) ;
#48262=CARTESIAN_POINT ( 'NONE',  ( 96.87985868497418096, -34.61725761836211035, 216.1641967044819808 ) ) ;
#48263=CARTESIAN_POINT ( 'NONE',  ( 116.4547782460826255, -32.24742764444982157, 15.18133956162492915 ) ) ;
#48264=DIRECTION ( 'NONE',  ( -1.000000000000000000, -3.999999999999999995E-14, -1.000000000000000078E-15 ) ) ;
#48267=EDGE_CURVE ( 'NONE', #72016, #70034, #6194, .T. ) ;
#48268=CARTESIAN_POINT ( 'NONE',  ( 115.9482186066389602, -32.63332544795704138, 104.1699109901969535 ) ) ;
#48270=CARTESIAN_POINT ( 'NONE',  ( 96.67089207319645539, -38.24056507437282448, 66.44133956162495735 ) ) ;
#48271=CARTESIAN_POINT ( 'NONE',  ( 100.2192867603235840, -28.80968922735345927, 260.6441967044821695 ) ) ;
#48272=ORIENTED_EDGE ( 'NONE', *, *, #83540, .F. ) ;
#48273=CARTESIAN_POINT ( 'NONE',  ( 117.3350766552244977, -34.92860824786317409, 243.9641967044819637 ) ) ;
#48274=LINE ( 'NONE', #6974, #23919 ) ;
#48277=EDGE_CURVE ( 'NONE', #14017, #35213, #62977, .T. ) ;
#48279=FACE_OUTER_BOUND ( 'NONE', #29862, .T. ) ;
#48281=CARTESIAN_POINT ( 'NONE',  ( 80.06648329127399677, -8.350947159940998787, 4.925625275911999168 ) ) ;
#48284=VECTOR ( 'NONE', #11761, 1000.000000000000000 ) ;
#48285=CARTESIAN_POINT ( 'NONE',  ( 107.0664832912749915, -36.72944715993903486, 25.56312527591096995 ) ) ;
#48287=CYLINDRICAL_SURFACE ( 'NONE', #76397, 4.750000000000004441 ) ;
#48288=DIRECTION ( 'NONE',  ( 0.000000000000000000, 1.000000000000000000, 0.000000000000000000 ) ) ;
#48292=CARTESIAN_POINT ( 'NONE',  ( 106.8359473341788686, -47.17421700602214685, 272.5584824187680510 ) ) ;
#48293=CARTESIAN_POINT ( 'NONE',  ( 97.79428472817266993, -42.74653246722733257, 142.7965776568629508 ) ) ;
#48294=CARTESIAN_POINT ( 'NONE',  ( 96.22287284433019749, -34.36014117848482385, 252.1432443235303538 ) ) ;
#48295=PLANE ( 'NONE',  #75143 ) ;
#48296=DIRECTION ( 'NONE',  ( 4.194175870806139918E-14, -1.000000000000000000, 0.000000000000000000 ) ) ;
#48298=FACE_OUTER_BOUND ( 'NONE', #20666, .T. ) ;
#48300=EDGE_CURVE ( 'NONE', #27646, #37791, #30702, .T. ) ;
#48301=VECTOR ( 'NONE', #49987, 1000.000000000000000 ) ;
#48304=VERTEX_POINT ( 'NONE', #79319 ) ;
#48305=CARTESIAN_POINT ( 'NONE',  ( 115.5798344143896372, -39.81741137289535004, 172.9600388756959717 ) ) ;
#48306=DIRECTION ( 'NONE',  ( 1.000000000000000078E-15, -1.000000000000000083E-30, -1.000000000000000000 ) ) ;
#48307=ORIENTED_EDGE ( 'NONE', *, *, #66895, .T. ) ;
#48308=VECTOR ( 'NONE', #84568, 1000.000000000000000 ) ;
#48309=DIRECTION ( 'NONE',  ( -1.000000000000000078E-15, 1.000000000000000083E-30, 1.000000000000000000 ) ) ;
#48310=CARTESIAN_POINT ( 'NONE',  ( 95.59354794629810215, -39.59649474372135813, 162.5213395616259788 ) ) ;
#48312=FACE_BOUND ( 'NONE', #78535, .T. ) ;
#48314=FACE_OUTER_BOUND ( 'NONE', #16289, .T. ) ;
#48315=CARTESIAN_POINT ( 'NONE',  ( 113.5922197990811213, -29.44396856740769408, 114.4956252759109816 ) ) ;
#48317=ORIENTED_EDGE ( 'NONE', *, *, #55501, .F. ) ;
#48318=ORIENTED_EDGE ( 'NONE', *, *, #9361, .F. ) ;
#48319=VECTOR ( 'NONE', #87452, 1000.000000000000000 ) ;
#48320=LINE ( 'NONE', #75623, #84989 ) ;
#48321=CARTESIAN_POINT ( 'NONE',  ( 101.5632356570521324, -44.81509498605967678, 193.1013395616249682 ) ) ;
#48325=EDGE_CURVE ( 'NONE', #6628, #79108, #58835, .T. ) ;
#48327=CARTESIAN_POINT ( 'NONE',  ( 53.56670390244749314, -48.82844715994058049, 129.9678068554150911 ) ) ;
#48330=CARTESIAN_POINT ( 'NONE',  ( 111.7842945758856672, -25.88553347519904335, 134.7499109901969518 ) ) ;
#48332=ADVANCED_FACE ( 'NONE', ( #44766 ), #31136, .F. ) ;
#48334=ORIENTED_EDGE ( 'NONE', *, *, #16391, .T. ) ;
#48335=EDGE_CURVE ( 'NONE', #62556, #67090, #2566, .T. ) ;
#48339=CARTESIAN_POINT ( 'NONE',  ( 108.9290709455192570, -28.27771998284391231, 177.7099951314959583 ) ) ;
#48340=VECTOR ( 'NONE', #63398, 1000.000000000000000 ) ;
#48341=CARTESIAN_POINT ( 'NONE',  ( 96.41083957889333078, -31.77770432788677013, 4.925625275910959999 ) ) ;
#48343=CARTESIAN_POINT ( 'NONE',  ( 108.4184404244437019, -26.73515679610073192, 25.96837172698450757 ) ) ;
#48344=ORIENTED_EDGE ( 'NONE', *, *, #76346, .T. ) ;
#48345=ORIENTED_EDGE ( 'NONE', *, *, #38604, .T. ) ;
#48347=ADVANCED_FACE ( 'NONE', ( #37959 ), #17078, .F. ) ;
#48350=VERTEX_POINT ( 'NONE', #24340 ) ;
#48351=EDGE_CURVE ( 'NONE', #15321, #72437, #30266, .T. ) ;
#48353=CARTESIAN_POINT ( 'NONE',  ( 97.87165577458247867, -34.79769342939158605, 257.6053928297065454 ) ) ;
#48354=ORIENTED_EDGE ( 'NONE', *, *, #23285, .T. ) ;
#48357=VERTEX_POINT ( 'NONE', #65226 ) ;
#48359=AXIS2_PLACEMENT_3D ( 'NONE', #41308, #41752, #20446 ) ;
#48360=CARTESIAN_POINT ( 'NONE',  ( 32.25690895537073288, -33.54226604285041446, 237.4678068554150059 ) ) ;
#48362=ORIENTED_EDGE ( 'NONE', *, *, #64163, .F. ) ;
#48364=CARTESIAN_POINT ( 'NONE',  ( 110.1408960893143956, -44.29103306967431308, 280.7023760838771409 ) ) ;
#48365=AXIS2_PLACEMENT_3D ( 'NONE', #74383, #41186, #82113 ) ;
#48366=CARTESIAN_POINT ( 'NONE',  ( 116.9251198095579554, -40.18685225151752860, 133.5584824187679658 ) ) ;
#48367=CARTESIAN_POINT ( 'NONE',  ( 117.0854383170106559, -39.53109055650223524, 98.60991099019594230 ) ) ;
#48368=CARTESIAN_POINT ( 'NONE',  ( 105.2596865451559012, -44.71351967478707223, 249.5838068554171798 ) ) ;
#48369=CARTESIAN_POINT ( 'NONE',  ( 131.5359215223106730, -17.65293368212931568, 7.043713522541953154 ) ) ;
#48370=CARTESIAN_POINT ( 'NONE',  ( 106.4836140971313654, -24.89327890070114435, 191.1156252759109861 ) ) ;
#48371=CARTESIAN_POINT ( 'NONE',  ( 181.9790560690580037, -31.62489322948711035, 193.9678068554150059 ) ) ;
#48372=LINE ( 'NONE', #42023, #85763 ) ;
#48374=CYLINDRICAL_SURFACE ( 'NONE', #20691, 2.999999999999999112 ) ;
#48375=EDGE_LOOP ( 'NONE', ( #31850, #85465, #64943, #14893 ) ) ;
#48379=CIRCLE ( 'NONE', #38229, 15.84999999999999964 ) ;
#48380=CARTESIAN_POINT ( 'NONE',  ( 102.0664873402873809, -27.97083079549564033, 136.4898195177950981 ) ) ;
#48381=CARTESIAN_POINT ( 'NONE',  ( 96.60699139826044757, -36.88735862350505101, 136.3384824187679385 ) ) ;
#48385=CARTESIAN_POINT ( 'NONE',  ( 37.56670390244743629, -48.82844715994126261, 180.4678068554150911 ) ) ;
#48386=DIRECTION ( 'NONE',  ( 0.000000000000000000, 0.000000000000000000, -1.000000000000000000 ) ) ;
#48388=CARTESIAN_POINT ( 'NONE',  ( 101.4165038149807572, -45.50681337102567880, 218.1213395616249784 ) ) ;
#48389=CYLINDRICAL_SURFACE ( 'NONE', #40848, 3.250000000000002665 ) ;
#48391=ORIENTED_EDGE ( 'NONE', *, *, #65904, .T. ) ;
#48393=DIRECTION ( 'NONE',  ( 0.7071067811868657627, 0.7071067811862293828, 7.071067811868650498E-16 ) ) ;
#48394=CARTESIAN_POINT ( 'NONE',  ( 130.1657039024480298, -18.82844715994099971, 199.5838068554170093 ) ) ;
#48395=B_SPLINE_CURVE_WITH_KNOTS ( 'NONE', 3,
 ( #9516, #64925, #2710, #49933, #16779, #65369, #30406, #77668, #3151, #86264, #24047, #51716, #10403, #79468, #17229, #53490, #17669, #60773, #4486, #19448, #24489, #38545, #5835, #47131, #39444, #81255, #52151, #11746, #88509, #74867, #10840 ),
 .UNSPECIFIED., .F., .F.,
 ( 4, 2, 2, 1, 2, 2, 2, 2, 2, 2, 2, 1, 1, 2, 2, 2, 4 ),
 ( 0.000000000000000000, 0.1250000000000227318, 0.1875000000000338618, 0.2187500000000353328, 0.2343750000000360545, 0.2500000000000367484, 0.3750000000000290323, 0.4375000000000245359, 0.5000000000000199840, 0.6250000000000124345, 0.6875000000000107692, 0.7187500000000089928, 0.7343750000000082157, 0.7421875000000077716, 0.7500000000000072164, 0.8750000000000036637, 1.000000000000000000 ),
 .UNSPECIFIED. ) ;
#48396=DIRECTION ( 'NONE',  ( -0.7071067811734105257, 0.7071067811996846197, 0.000000000000000000 ) ) ;
#48397=CARTESIAN_POINT ( 'NONE',  ( 111.4991187713021219, -26.55290587224241960, 284.7375300378155316 ) ) ;
#48398=EDGE_LOOP ( 'NONE', ( #64130, #848, #31947, #13982 ) ) ;
#48399=LINE ( 'NONE', #87985, #10379 ) ;
#48400=CARTESIAN_POINT ( 'NONE',  ( 113.5789493677227711, -44.94383383376451491, 168.1099109901969939 ) ) ;
#48401=CARTESIAN_POINT ( 'NONE',  ( 96.83360046493686468, -38.89957200400883863, 27.49276813305395706 ) ) ;
#48402=CARTESIAN_POINT ( 'NONE',  ( 117.5308098062252498, -40.43017262224169883, 174.5680062282919778 ) ) ;
#48403=CYLINDRICAL_SURFACE ( 'NONE', #59051, 2.116999999999993776 ) ;
#48404=CARTESIAN_POINT ( 'NONE',  ( 115.8252723203762429, -31.72975044166505398, 100.2398416254468714 ) ) ;
#48406=DIRECTION ( 'NONE',  ( -1.000000000000000078E-15, 0.000000000000000000, 1.000000000000000000 ) ) ;
#48407=DIRECTION ( 'NONE',  ( 1.639958061481212836E-42, -4.100000000000000342E-29, -1.000000000000000000 ) ) ;
#48408=CARTESIAN_POINT ( 'NONE',  ( 163.2449138993008262, -32.11662333284039761, 193.9678068554149775 ) ) ;
#48410=VECTOR ( 'NONE', #63287, 1000.000000000000000 ) ;
#48412=AXIS2_PLACEMENT_3D ( 'NONE', #79049, #37712, #85872 ) ;
#48414=ORIENTED_EDGE ( 'NONE', *, *, #1084, .F. ) ;
#48415=ORIENTED_EDGE ( 'NONE', *, *, #65325, .T. ) ;
#48416=DIRECTION ( 'NONE',  ( -1.000000000000000000, -1.000000000000000078E-15, -1.000000000000000078E-15 ) ) ;
#48417=CARTESIAN_POINT ( 'NONE',  ( 104.7644060343265551, -46.87484541886965417, 68.39848241876794077 ) ) ;
#48420=EDGE_CURVE ( 'NONE', #77531, #14756, #25217, .T. ) ;
#48421=CARTESIAN_POINT ( 'NONE',  ( 114.9980252723336207, -29.89690579156949823, 180.3927681330539770 ) ) ;
#48423=CARTESIAN_POINT ( 'NONE',  ( 114.1034101198941215, -31.83723292758831747, 278.7324198280767860 ) ) ;
#48424=ORIENTED_EDGE ( 'NONE', *, *, #53586, .F. ) ;
#48425=ORIENTED_EDGE ( 'NONE', *, *, #15477, .T. ) ;
#48427=VECTOR ( 'NONE', #74401, 1000.000000000000000 ) ;
#48428=DIRECTION ( 'NONE',  ( -1.000000000000000000, -3.201858731750027727E-15, -1.000000000000000078E-15 ) ) ;
#48430=AXIS2_PLACEMENT_3D ( 'NONE', #20715, #47047, #53853 ) ;
#48432=CARTESIAN_POINT ( 'NONE',  ( 105.7964350658723163, -26.72445465374554985, 275.1771098754847458 ) ) ;
#48434=DIRECTION ( 'NONE',  ( 0.000000000000000000, 0.000000000000000000, -1.000000000000000000 ) ) ;
#48436=CARTESIAN_POINT ( 'NONE',  ( 111.4502655420255905, -27.98611277567904310, 279.7070538473400916 ) ) ;
#48439=ORIENTED_EDGE ( 'NONE', *, *, #67842, .T. ) ;
#48440=LINE ( 'NONE', #75290, #40279 ) ;
#48441=LINE ( 'NONE', #63909, #71405 ) ;
#48442=CARTESIAN_POINT ( 'NONE',  ( 114.8246268090051245, -34.19154740317726038, 86.89666179816296676 ) ) ;
#48444=DIRECTION ( 'NONE',  ( 0.000000000000000000, 0.000000000000000000, 1.000000000000000000 ) ) ;
#48445=ORIENTED_EDGE ( 'NONE', *, *, #14483, .F. ) ;
#48448=CARTESIAN_POINT ( 'NONE',  ( 77.67297288197789840, -35.37149612621453088, 7.198162082951554019 ) ) ;
#48450=CARTESIAN_POINT ( 'NONE',  ( 114.2400596693416475, -45.14401474321602592, 153.1508633711489722 ) ) ;
#48453=DIRECTION ( 'NONE',  ( -4.237773401492740281E-14, 1.000000000000000000, 0.000000000000000000 ) ) ;
#48454=CARTESIAN_POINT ( 'NONE',  ( 107.5650335644346569, -45.56823575777373492, 149.0530118773259858 ) ) ;
#48456=CARTESIAN_POINT ( 'NONE',  ( 34.27258461953785229, -35.55794170701850732, 193.9678068554150911 ) ) ;
#48457=CARTESIAN_POINT ( 'NONE',  ( 96.89995799317335923, -32.33320227283598314, 57.01372051400599616 ) ) ;
#48458=VECTOR ( 'NONE', #42506, 1000.000000000000000 ) ;
#48459=CARTESIAN_POINT ( 'NONE',  ( 168.5667039024483813, -48.82844715993517326, 249.9678068554149775 ) ) ;
#48460=ORIENTED_EDGE ( 'NONE', *, *, #52800, .T. ) ;
#48462=ORIENTED_EDGE ( 'NONE', *, *, #20683, .F. ) ;
#48464=DIRECTION ( 'NONE',  ( -0.9068632946707755327, 0.4214249218767993077, 0.000000000000000000 ) ) ;
#48465=EDGE_LOOP ( 'NONE', ( #69510, #12287 ) ) ;
#48466=CARTESIAN_POINT ( 'NONE',  ( 112.0124476237221103, -28.73397683645135814, 289.6356252759109680 ) ) ;
#48467=CARTESIAN_POINT ( 'NONE',  ( 108.8525730979967676, -47.02250997168171409, 163.7127681330539701 ) ) ;
#48468=DIRECTION ( 'NONE',  ( 0.000000000000000000, 0.000000000000000000, -1.000000000000000000 ) ) ;
#48470=CARTESIAN_POINT ( 'NONE',  ( 104.1078173601787995, -46.72588569351386667, 103.3470538473389411 ) ) ;
#48471=CARTESIAN_POINT ( 'NONE',  ( 101.9936209708133248, -45.44607155584300529, 262.1564586119682758 ) ) ;
#48472=ORIENTED_EDGE ( 'NONE', *, *, #15787, .F. ) ;
#48473=CARTESIAN_POINT ( 'NONE',  ( 97.80821801276054828, -40.50893789028450698, 116.6351770529384595 ) ) ;
#48477=VECTOR ( 'NONE', #78892, 1000.000000000000000 ) ;
#48479=VECTOR ( 'NONE', #26875, 1000.000000000000000 ) ;
#48480=AXIS2_PLACEMENT_3D ( 'NONE', #18508, #46194, #80314 ) ;
#48481=LINE ( 'NONE', #13998, #50781 ) ;
#48482=CARTESIAN_POINT ( 'NONE',  ( 115.4447846419100472, -42.99283068281499709, 28.31562527591097123 ) ) ;
#48485=CARTESIAN_POINT ( 'NONE',  ( 141.0235900724604790, -8.833000550534265471, 14.92562527591107369 ) ) ;
#48486=DIRECTION ( 'NONE',  ( 0.000000000000000000, 0.000000000000000000, -1.000000000000000000 ) ) ;
#48487=CARTESIAN_POINT ( 'NONE',  ( 114.6457050300329996, -40.66804080626008044, 287.8667055423626380 ) ) ;
#48488=CARTESIAN_POINT ( 'NONE',  ( 103.2384247724198332, -27.39885374353689329, 100.3865915095992420 ) ) ;
#48489=CARTESIAN_POINT ( 'NONE',  ( 117.1882713363356174, -39.28166824301211335, 119.6299109901969615 ) ) ;
#48490=DIRECTION ( 'NONE',  ( -4.237773401492740281E-14, 1.000000000000000000, 0.000000000000000000 ) ) ;
#48491=CARTESIAN_POINT ( 'NONE',  ( 98.05257159168807846, -42.12399974224388188, 161.7556252759109725 ) ) ;
#48492=CARTESIAN_POINT ( 'NONE',  ( 32.56670390244700997, -22.48495420874110806, -5.074374724088000832 ) ) ;
#48493=EDGE_LOOP ( 'NONE', ( #85958, #39226, #69476, #11160 ) ) ;
#48495=AXIS2_PLACEMENT_3D ( 'NONE', #74124, #53190, #5544 ) ;
#48498=CARTESIAN_POINT ( 'NONE',  ( 136.5763721200418672, -35.60518726037151538, 2.783021291305102896 ) ) ;
#48499=ORIENTED_EDGE ( 'NONE', *, *, #23370, .T. ) ;
#48500=CARTESIAN_POINT ( 'NONE',  ( 41.56648329127398966, -18.82844715994071194, 195.9256252759120684 ) ) ;
#48501=CARTESIAN_POINT ( 'NONE',  ( 117.5013794172148351, -40.51439451343497922, 173.5375300378159693 ) ) ;
#48502=EDGE_LOOP ( 'NONE', ( #11400, #17331 ) ) ;
#48504=CARTESIAN_POINT ( 'NONE',  ( 112.2157656529268763, -45.81911987206276393, 208.9870538473389558 ) ) ;
#48505=CARTESIAN_POINT ( 'NONE',  ( 184.5667039024548615, -48.82844715994099971, 300.4678068554149490 ) ) ;
#48506=DIRECTION ( 'NONE',  ( -0.000000000000000000, -0.000000000000000000, 1.000000000000000000 ) ) ;
#48507=CARTESIAN_POINT ( 'NONE',  ( 143.0664832912740110, -8.729447159940999512, 342.9256252759119548 ) ) ;
#48508=VERTEX_POINT ( 'NONE', #51134 ) ;
#48509=EDGE_CURVE ( 'NONE', #81323, #22750, #78874, .T. ) ;
#48511=VERTEX_POINT ( 'NONE', #60169 ) ;
#48512=ORIENTED_EDGE ( 'NONE', *, *, #68491, .F. ) ;
#48514=ORIENTED_EDGE ( 'NONE', *, *, #22466, .F. ) ;
#48516=CARTESIAN_POINT ( 'NONE',  ( 105.1109661324377811, -26.48940614006117755, 231.2270538473399597 ) ) ;
#48517=DIRECTION ( 'NONE',  ( 3.310531404218880154E-13, -1.000000000000000000, 3.320531404218880632E-28 ) ) ;
#48518=CARTESIAN_POINT ( 'NONE',  ( 135.1485260852034571, -16.20116861174954082, 1.807989644433795728 ) ) ;
#48520=EDGE_CURVE ( 'NONE', #31976, #30939, #10904, .T. ) ;
#48521=DIRECTION ( 'NONE',  ( 0.000000000000000000, 0.000000000000000000, 1.000000000000000000 ) ) ;
#48523=PLANE ( 'NONE',  #54398 ) ;
#48524=CARTESIAN_POINT ( 'NONE',  ( 111.4247116192842810, -46.22429891269226943, 27.91848241876792969 ) ) ;
#48525=VERTEX_POINT ( 'NONE', #19309 ) ;
#48526=EDGE_CURVE ( 'NONE', #69613, #75906, #46979, .T. ) ;
#48527=EDGE_CURVE ( 'NONE', #63937, #70860, #68893, .T. ) ;
#48528=EDGE_LOOP ( 'NONE', ( #20139, #26359 ) ) ;
#48530=CIRCLE ( 'NONE', #76183, 0.4999999999999982236 ) ;
#48531=LINE ( 'NONE', #25885, #60748 ) ;
#48532=EDGE_CURVE ( 'NONE', #83421, #46468, #58816, .T. ) ;
#48533=CARTESIAN_POINT ( 'NONE',  ( 104.4938967476557821, -26.68352342390111787, 241.2880062282909535 ) ) ;
#48534=CARTESIAN_POINT ( 'NONE',  ( 165.2725846195380086, -35.55794170701810941, -5.074374724088000832 ) ) ;
#48535=CARTESIAN_POINT ( 'NONE',  ( 114.6661721138974315, -42.88640786233941782, 84.28419670448195689 ) ) ;
#48538=EDGE_CURVE ( 'NONE', #23155, #21324, #48320, .T. ) ;
#48539=CARTESIAN_POINT ( 'NONE',  ( 97.81170999498195329, -40.51745678363457159, 187.6351607544849287 ) ) ;
#48540=VERTEX_POINT ( 'NONE', #75167 ) ;
#48541=CYLINDRICAL_SURFACE ( 'NONE', #61722, 4.750000000000004441 ) ;
#48542=EDGE_LOOP ( 'NONE', ( #42454, #76707 ) ) ;
#48543=ORIENTED_EDGE ( 'NONE', *, *, #80774, .F. ) ;
#48545=CARTESIAN_POINT ( 'NONE',  ( 115.1162204959661466, -41.57488383322457537, 274.8149166392303755 ) ) ;
#48546=CONICAL_SURFACE ( 'NONE', #57257, 9.571100913904325935, 0.7853981633974543852 ) ;
#48547=CARTESIAN_POINT ( 'NONE',  ( 113.1782937289016218, -44.75186862573180946, 193.0939586049964021 ) ) ;
#48550=CARTESIAN_POINT ( 'NONE',  ( 97.81169952324414396, -40.51743120087827776, 141.6355106266202313 ) ) ;
#48552=CARTESIAN_POINT ( 'NONE',  ( 99.09570908776939291, -30.55043173837237092, 85.80229194108821389 ) ) ;
#48554=AXIS2_PLACEMENT_3D ( 'NONE', #77493, #63873, #14832 ) ;
#48555=VERTEX_POINT ( 'NONE', #12497 ) ;
#48556=CARTESIAN_POINT ( 'NONE',  ( 141.0667039024479834, -50.82844715994100682, 310.9178068554150514 ) ) ;
#48560=EDGE_LOOP ( 'NONE', ( #42050, #5854, #6163, #40936 ) ) ;
#48561=CARTESIAN_POINT ( 'NONE',  ( 107.6068636345326155, -48.56787927409158812, 42.61276813305398292 ) ) ;
#48562=EDGE_LOOP ( 'NONE', ( #55709, #13218, #62420, #44817 ) ) ;
#48564=CARTESIAN_POINT ( 'NONE',  ( 114.3096959184101280, -40.49343719410034481, 286.2623760838771432 ) ) ;
#48565=EDGE_CURVE ( 'NONE', #32414, #9456, #33827, .T. ) ;
#48566=CARTESIAN_POINT ( 'NONE',  ( 108.3347386951206204, -46.73470465874113700, 127.6774649500359828 ) ) ;
#48567=CARTESIAN_POINT ( 'NONE',  ( 102.9676436823273917, -46.25511244710201453, 137.2651490854349561 ) ) ;
#48570=FACE_OUTER_BOUND ( 'NONE', #85732, .T. ) ;
#48571=EDGE_CURVE ( 'NONE', #12725, #79504, #27016, .T. ) ;
#48573=AXIS2_PLACEMENT_3D ( 'NONE', #55006, #34591, #48650 ) ;
#48574=CARTESIAN_POINT ( 'NONE',  ( 104.3994723555534989, -25.95519307775132134, 236.2575300378159682 ) ) ;
#48576=VERTEX_POINT ( 'NONE', #47881 ) ;
#48577=CARTESIAN_POINT ( 'NONE',  ( 63.03715912545735023, -46.82818131006016671, 180.4678068554151196 ) ) ;
#48579=CARTESIAN_POINT ( 'NONE',  ( 95.97749374758174667, -37.21091289986100037, 112.3489586092449599 ) ) ;
#48583=VERTEX_POINT ( 'NONE', #13390 ) ;
#48584=EDGE_LOOP ( 'NONE', ( #67133, #1556, #48307 ) ) ;
#48585=DIRECTION ( 'NONE',  ( 0.000000000000000000, 0.000000000000000000, -1.000000000000000000 ) ) ;
#48587=CARTESIAN_POINT ( 'NONE',  ( 107.0664832912739541, -20.72944715994095333, 357.5272416190308604 ) ) ;
#48588=CARTESIAN_POINT ( 'NONE',  ( 45.76696975232698605, -48.62818131005841593, 129.9678068554150911 ) ) ;
#48589=CARTESIAN_POINT ( 'NONE',  ( 103.7603453811189667, -44.19263536178414142, 175.0623760838769840 ) ) ;
#48590=CARTESIAN_POINT ( 'NONE',  ( 97.19620376612084556, -33.30704266974938577, 282.0613395616252888 ) ) ;
#48591=PLANE ( 'NONE',  #7344 ) ;
#48596=EDGE_LOOP ( 'NONE', ( #70048, #76621, #30650, #49824 ) ) ;
#48597=VECTOR ( 'NONE', #51618, 999.9999999999998863 ) ;
#48598=DIRECTION ( 'NONE',  ( 1.000000000000000000, 4.163336342344333240E-14, 0.000000000000000000 ) ) ;
#48601=VECTOR ( 'NONE', #18602, 1000.000000000000000 ) ;
#48603=DIRECTION ( 'NONE',  ( 3.999999999999999995E-14, -1.000000000000000000, 4.100000000000000342E-29 ) ) ;
#48604=DIRECTION ( 'NONE',  ( 0.9068632946707807507, -0.4214249218767881500, 9.068605531941956314E-16 ) ) ;
#48605=CARTESIAN_POINT ( 'NONE',  ( 103.4754675462218927, -28.97956086136533926, 179.8438483995059869 ) ) ;
#48606=CARTESIAN_POINT ( 'NONE',  ( 116.7859321266972330, -32.83856289285826335, 54.12991099019698282 ) ) ;
#48607=CARTESIAN_POINT ( 'NONE',  ( 25.56670390244816815, -48.82844715994168183, 295.7178068554150059 ) ) ;
#48608=ORIENTED_EDGE ( 'NONE', *, *, #9709, .F. ) ;
#48610=ORIENTED_EDGE ( 'NONE', *, *, #65788, .F. ) ;
#48612=VERTEX_POINT ( 'NONE', #41079 ) ;
#48614=LINE ( 'NONE', #21855, #60369 ) ;
#48615=CARTESIAN_POINT ( 'NONE',  ( 116.7959471365900299, -39.38489853325881285, 274.6145815639363832 ) ) ;
#48618=ORIENTED_EDGE ( 'NONE', *, *, #460, .F. ) ;
#48619=CARTESIAN_POINT ( 'NONE',  ( 113.4731498177359725, -46.72887913999166898, 68.02991099019695298 ) ) ;
#48620=CIRCLE ( 'NONE', #73347, 2.517500000000000071 ) ;
#48621=AXIS2_PLACEMENT_3D ( 'NONE', #29702, #8829, #203 ) ;
#48622=CIRCLE ( 'NONE', #26928, 3.250000000000002665 ) ;
#48626=DIRECTION ( 'NONE',  ( 0.000000000000000000, -1.000000000000000000, 0.000000000000000000 ) ) ;
#48627=EDGE_CURVE ( 'NONE', #79347, #35754, #46542, .T. ) ;
#48629=ORIENTED_EDGE ( 'NONE', *, *, #14660, .F. ) ;
#48631=EDGE_CURVE ( 'NONE', #47902, #66479, #5233, .T. ) ;
#48632=CARTESIAN_POINT ( 'NONE',  ( 116.3212776292293995, -32.94146857471267253, 120.1356252759109537 ) ) ;
#48634=DIRECTION ( 'NONE',  ( 0.000000000000000000, -1.000000000000000000, 0.000000000000000000 ) ) ;
#48637=EDGE_LOOP ( 'NONE', ( #187, #42780, #70941, #37550 ) ) ;
#48638=CARTESIAN_POINT ( 'NONE',  ( 101.6669702799278525, -27.05833217848093497, 101.4937205140059575 ) ) ;
#48641=CARTESIAN_POINT ( 'NONE',  ( 72.06648329127402519, -46.72944715994106701, -5.074374724089063982 ) ) ;
#48645=VECTOR ( 'NONE', #23762, 1000.000000000000000 ) ;
#48647=ADVANCED_FACE ( 'NONE', ( #42859 ), #35611, .F. ) ;
#48649=CARTESIAN_POINT ( 'NONE',  ( 102.6065612795740805, -27.36740250608086100, 136.4422919425769578 ) ) ;
#48650=DIRECTION ( 'NONE',  ( 1.000000000000000000, 0.000000000000000000, 0.000000000000000000 ) ) ;
#48651=ORIENTED_EDGE ( 'NONE', *, *, #81308, .T. ) ;
#48652=CARTESIAN_POINT ( 'NONE',  ( 96.93559702949583823, -34.21358363697174099, 272.1327681330538439 ) ) ;
#48653=CARTESIAN_POINT ( 'NONE',  ( 97.81795488547844286, -40.53270472218247278, 252.6369010203054586 ) ) ;
#48655=DIRECTION ( 'NONE',  ( -1.000000000000000078E-15, 1.000000000000000083E-30, 1.000000000000000000 ) ) ;
#48657=DIRECTION ( 'NONE',  ( 1.000000000000000078E-15, -1.000000000000000083E-30, -1.000000000000000000 ) ) ;
#48658=ADVANCED_FACE ( 'NONE', ( #71055 ), #76055, .T. ) ;
#48659=DIRECTION ( 'NONE',  ( -1.000000000000000078E-15, 1.000000000000000083E-30, 1.000000000000000000 ) ) ;
#48661=CARTESIAN_POINT ( 'NONE',  ( 116.5663773505005310, -40.88766770462213884, 208.4861014663879644 ) ) ;
#48662=ORIENTED_EDGE ( 'NONE', *, *, #40853, .F. ) ;
#48663=VERTEX_POINT ( 'NONE', #7018 ) ;
#48665=AXIS2_PLACEMENT_3D ( 'NONE', #33100, #46710, #52610 ) ;
#48666=CARTESIAN_POINT ( 'NONE',  ( 98.83447963006204873, -41.25831470702095061, 173.1463452106589784 ) ) ;
#48668=CARTESIAN_POINT ( 'NONE',  ( 115.7455327456632403, -41.23958449135837867, 284.4441967044819535 ) ) ;
#48669=DIRECTION ( 'NONE',  ( 0.000000000000000000, 0.000000000000000000, -1.000000000000000000 ) ) ;
#48674=CARTESIAN_POINT ( 'NONE',  ( 99.76842024043810397, -29.31547782932919688, 225.6956252759109702 ) ) ;
#48675=CARTESIAN_POINT ( 'NONE',  ( 97.06386455791596291, -37.34269636115125479, 171.3750780254042070 ) ) ;
#48677=ORIENTED_EDGE ( 'NONE', *, *, #16595, .T. ) ;
#48678=EDGE_CURVE ( 'NONE', #39354, #87937, #36528, .T. ) ;
#48679=CARTESIAN_POINT ( 'NONE',  ( 143.9834832912729894, -1.929447159941392931, 342.9256252759109316 ) ) ;
#48682=CARTESIAN_POINT ( 'NONE',  ( 107.0664832912748068, -36.72944715993923381, -5.074374724089029343 ) ) ;
#48683=EDGE_CURVE ( 'NONE', #50282, #39081, #63326, .T. ) ;
#48685=DIRECTION ( 'NONE',  ( 0.9963424814100680926, -0.08544974978095698503, 0.000000000000000000 ) ) ;
#48687=CARTESIAN_POINT ( 'NONE',  ( 111.1459338097010914, -47.05202348217205355, 18.88800622829195319 ) ) ;
#48689=CIRCLE ( 'NONE', #9567, 1.000000000000000888 ) ;
#48690=CARTESIAN_POINT ( 'NONE',  ( 115.9600293333739387, -30.16561243848903828, 259.3203871806730945 ) ) ;
#48692=CARTESIAN_POINT ( 'NONE',  ( 77.49051321911612433, -37.69637952316315221, 6.988870342670268521 ) ) ;
#48693=CARTESIAN_POINT ( 'NONE',  ( 107.2978958415778123, -24.20855449189627251, 322.4523926293242653 ) ) ;
#48694=CARTESIAN_POINT ( 'NONE',  ( 172.5664832912740110, -27.82844715994070484, 23.67562527591200094 ) ) ;
#48695=CARTESIAN_POINT ( 'NONE',  ( 106.8900815348805509, -46.00655951153972723, 75.37951894101996686 ) ) ;
#48696=CARTESIAN_POINT ( 'NONE',  ( 107.9200411489893412, -47.17696527638128856, 173.6413395616249886 ) ) ;
#48697=CARTESIAN_POINT ( 'NONE',  ( 62.03742497533652767, -23.42844715994041493, 193.9678068554150911 ) ) ;
#48698=VERTEX_POINT ( 'NONE', #42413 ) ;
#48699=ADVANCED_FACE ( 'NONE', ( #34719 ), #27903, .T. ) ;
#48700=VECTOR ( 'NONE', #67386, 1000.000000000000000 ) ;
#48706=VERTEX_POINT ( 'NONE', #1999 ) ;
#48709=AXIS2_PLACEMENT_3D ( 'NONE', #89558, #62734, #33690 ) ;
#48710=CARTESIAN_POINT ( 'NONE',  ( 99.88917683200891418, -30.19057113389683167, 80.16099125664798919 ) ) ;
#48711=CARTESIAN_POINT ( 'NONE',  ( 106.3003094972131208, -47.14862859053906874, 222.5184824187679453 ) ) ;
#48712=CARTESIAN_POINT ( 'NONE',  ( 107.6532706963292725, -47.74396045468181882, 197.6308633711489620 ) ) ;
#48713=CARTESIAN_POINT ( 'NONE',  ( 96.94236579736397630, -32.35154040576534840, 57.01372051400599616 ) ) ;
#48716=ORIENTED_EDGE ( 'NONE', *, *, #9178, .T. ) ;
#48718=CARTESIAN_POINT ( 'NONE',  ( 177.0371591254545649, -48.62818131005479927, 180.4678068554150059 ) ) ;
#48719=ADVANCED_FACE ( 'NONE', ( #50125 ), #43311, .T. ) ;
#48720=CARTESIAN_POINT ( 'NONE',  ( 108.4470127171752125, -27.04659769318750762, 104.9641967044829869 ) ) ;
#48721=CARTESIAN_POINT ( 'NONE',  ( 101.1158648436187235, -27.35912039304959009, 65.51467289495799662 ) ) ;
#48722=CARTESIAN_POINT ( 'NONE',  ( 116.2574608483823226, -41.81646255891691766, 263.4241967044824833 ) ) ;
#48723=VERTEX_POINT ( 'NONE', #45527 ) ;
#48724=CARTESIAN_POINT ( 'NONE',  ( 95.29485650985192535, -38.09666651163277606, 236.4184824187679510 ) ) ;
#48725=DIRECTION ( 'NONE',  ( 0.0001713722455994998422, -0.9999999853157766072, 0.000000000000000000 ) ) ;
#48727=CARTESIAN_POINT ( 'NONE',  ( 98.60354758604864855, -42.06789318863769012, 27.77490799794517073 ) ) ;
#48728=EDGE_CURVE ( 'NONE', #32371, #77722, #50580, .T. ) ;
#48731=CARTESIAN_POINT ( 'NONE',  ( 107.0664832912739541, -36.72944715994095333, 309.2406250056037038 ) ) ;
#48732=ADVANCED_FACE ( 'NONE', ( #71501 ), #24231, .F. ) ;
#48733=DIRECTION ( 'NONE',  ( 0.7071067811865614505, -0.7071067811865336949, 0.000000000000000000 ) ) ;
#48734=DIRECTION ( 'NONE',  ( 0.9068632946707807507, -0.4214249218767881500, 1.031805784967618114E-15 ) ) ;
#48737=CARTESIAN_POINT ( 'NONE',  ( 104.4836948513005552, -26.98053053655335276, 40.28118682077015222 ) ) ;
#48739=CARTESIAN_POINT ( 'NONE',  ( 115.0889047219105663, -30.61763667692697055, 259.3439586095311142 ) ) ;
#48740=ORIENTED_EDGE ( 'NONE', *, *, #32663, .F. ) ;
#48743=CARTESIAN_POINT ( 'NONE',  ( 115.9256476412969192, -30.08033833575881033, 264.3508633711492735 ) ) ;
#48744=CARTESIAN_POINT ( 'NONE',  ( 98.85664311730629095, -30.30429143764317601, 151.7984824187679465 ) ) ;
#48745=CARTESIAN_POINT ( 'NONE',  ( 110.7484172854196629, -26.25849398357808084, 250.8194347997207387 ) ) ;
#48746=VECTOR ( 'NONE', #47578, 1000.000000000000000 ) ;
#48748=CARTESIAN_POINT ( 'NONE',  ( 142.8821648370248170, -72.54478064608022692, 396.9756252759102040 ) ) ;
#48749=CARTESIAN_POINT ( 'NONE',  ( 81.62727349186259573, -34.46583755400396143, 7.833212107640068034 ) ) ;
#48750=CARTESIAN_POINT ( 'NONE',  ( 104.4079917138377454, -46.45806025294579200, 138.3647832575413190 ) ) ;
#48751=DIRECTION ( 'NONE',  ( 0.000000000000000000, 0.000000000000000000, 1.000000000000000000 ) ) ;
#48752=AXIS2_PLACEMENT_3D ( 'NONE', #84008, #31590, #87023 ) ;
#48753=EDGE_CURVE ( 'NONE', #80487, #40161, #29800, .T. ) ;
#48754=VECTOR ( 'NONE', #7764, 1000.000000000000000 ) ;
#48755=AXIS2_PLACEMENT_3D ( 'NONE', #36974, #64684, #83345 ) ;
#48759=ORIENTED_EDGE ( 'NONE', *, *, #14288, .F. ) ;
#48760=EDGE_CURVE ( 'NONE', #20871, #20676, #45095, .T. ) ;
#48761=CARTESIAN_POINT ( 'NONE',  ( 111.5068547175069824, -28.09499701576110198, 169.1209912566479545 ) ) ;
#48764=DIRECTION ( 'NONE',  ( 0.000000000000000000, 0.000000000000000000, -1.000000000000000000 ) ) ;
#48765=CARTESIAN_POINT ( 'NONE',  ( 98.10941331148548272, -42.08998169807667722, 157.7556252759109725 ) ) ;
#48766=PLANE ( 'NONE',  #39574 ) ;
#48767=CARTESIAN_POINT ( 'NONE',  ( 115.8259185139441456, -31.73085971727213916, 149.2400304187415543 ) ) ;
#48768=LINE ( 'NONE', #50116, #33995 ) ;
#48769=CARTESIAN_POINT ( 'NONE',  ( 36.23715912545429063, -47.82818131006125384, 249.9678068554150343 ) ) ;
#48770=LINE ( 'NONE', #35602, #42505 ) ;
#48771=AXIS2_PLACEMENT_3D ( 'NONE', #59548, #38230, #73186 ) ;
#48772=CARTESIAN_POINT ( 'NONE',  ( 102.0841886111852261, -27.63463957783707770, 100.4632443235309580 ) ) ;
#48774=ORIENTED_EDGE ( 'NONE', *, *, #83445, .T. ) ;
#48775=ORIENTED_EDGE ( 'NONE', *, *, #4986, .T. ) ;
#48776=CARTESIAN_POINT ( 'NONE',  ( 109.2565852557048629, -45.31616550848684000, 44.20729759161095984 ) ) ;
#48778=CARTESIAN_POINT ( 'NONE',  ( 113.2095242374419541, -45.08419629851108823, 179.0689586092439640 ) ) ;
#48781=DIRECTION ( 'NONE',  ( 0.000000000000000000, 1.000000000000000000, 0.000000000000000000 ) ) ;
#48783=DIRECTION ( 'NONE',  ( 0.000000000000000000, 0.000000000000000000, -1.000000000000000000 ) ) ;
#48784=CARTESIAN_POINT ( 'NONE',  ( 37.03715912545348488, -48.62818131006127942, 117.4678068554150485 ) ) ;
#48786=CARTESIAN_POINT ( 'NONE',  ( 102.7067583520260712, -46.86140753836549777, 137.2651490854349561 ) ) ;
#48787=ORIENTED_EDGE ( 'NONE', *, *, #4784, .F. ) ;
#48788=ORIENTED_EDGE ( 'NONE', *, *, #71963, .F. ) ;
#48789=VERTEX_POINT ( 'NONE', #79210 ) ;
#48790=CARTESIAN_POINT ( 'NONE',  ( 83.06670390244796920, -58.72944715994099596, 234.8338068554150198 ) ) ;
#48793=EDGE_CURVE ( 'NONE', #2491, #76131, #38290, .T. ) ;
#48794=CARTESIAN_POINT ( 'NONE',  ( 107.9397346479727418, -44.84530559174715592, 200.4795189410199612 ) ) ;
#48795=LINE ( 'NONE', #50146, #40693 ) ;
#48796=CARTESIAN_POINT ( 'NONE',  ( 97.33791405800978680, -34.07076917306103780, 27.11454834448431939 ) ) ;
#48798=ORIENTED_EDGE ( 'NONE', *, *, #69567, .F. ) ;
#48799=ORIENTED_EDGE ( 'NONE', *, *, #4663, .T. ) ;
#48800=CARTESIAN_POINT ( 'NONE',  ( 136.7280559526967920, -19.42731094489385768, 2.974216770160625689 ) ) ;
#48804=CARTESIAN_POINT ( 'NONE',  ( 101.6974430329241272, -44.43982537643711339, 233.5120594963729559 ) ) ;
#48806=VERTEX_POINT ( 'NONE', #58293 ) ;
#48808=FACE_OUTER_BOUND ( 'NONE', #50466, .T. ) ;
#48811=ORIENTED_EDGE ( 'NONE', *, *, #9012, .F. ) ;
#48813=ADVANCED_FACE ( 'NONE', ( #30595 ), #24668, .T. ) ;
#48815=DIRECTION ( 'NONE',  ( 1.000000000000000078E-15, 1.000000000000000083E-30, -1.000000000000000000 ) ) ;
#48817=ORIENTED_EDGE ( 'NONE', *, *, #65605, .F. ) ;
#48818=VERTEX_POINT ( 'NONE', #16967 ) ;
#48819=CARTESIAN_POINT ( 'NONE',  ( 99.35431583021956214, -34.05534528112548287, 283.8795189410199100 ) ) ;
#48820=CARTESIAN_POINT ( 'NONE',  ( 97.96720171806632038, -41.86261760143219846, 136.7356252759109623 ) ) ;
#48821=CARTESIAN_POINT ( 'NONE',  ( 112.5028774994482035, -27.85959465031275784, 94.63848241876793566 ) ) ;
#48823=( LENGTH_UNIT ( ) NAMED_UNIT ( * ) SI_UNIT ( .MILLI., .METRE. ) );
#48824=CARTESIAN_POINT ( 'NONE',  ( 116.5266666817545627, -41.19333145446972821, 224.4756252759109714 ) ) ;
#48825=CYLINDRICAL_SURFACE ( 'NONE', #44304, 0.4999999999999932832 ) ;
#48829=VERTEX_POINT ( 'NONE', #23795 ) ;
#48830=ORIENTED_EDGE ( 'NONE', *, *, #44221, .T. ) ;
#48831=FACE_OUTER_BOUND ( 'NONE', #1253, .T. ) ;
#48832=CARTESIAN_POINT ( 'NONE',  ( 107.8158413964318925, -26.73611026959684267, 136.0168363452475546 ) ) ;
#48835=CARTESIAN_POINT ( 'NONE',  ( 96.67071733825032709, -35.94615501309311156, 146.2670538473399517 ) ) ;
#48840=DIRECTION ( 'NONE',  ( -1.000000000000000078E-15, -1.000000000000000000, 0.000000000000000000 ) ) ;
#48841=CARTESIAN_POINT ( 'NONE',  ( 115.3705510513157009, -30.46277945167186374, 215.3413395616249773 ) ) ;
#48842=CARTESIAN_POINT ( 'NONE',  ( 194.0667039024482392, -40.32844715993407192, 129.9678068554150343 ) ) ;
#48843=EDGE_CURVE ( 'NONE', #31385, #48257, #38735, .T. ) ;
#48846=CARTESIAN_POINT ( 'NONE',  ( 80.06648329127399677, -8.729447159940999512, 311.1531252759119752 ) ) ;
#48847=EDGE_CURVE ( 'NONE', #51938, #56684, #3780, .T. ) ;
#48849=EDGE_CURVE ( 'NONE', #62608, #6901, #31469, .T. ) ;
#48850=FACE_OUTER_BOUND ( 'NONE', #28856, .T. ) ;
#48851=FACE_OUTER_BOUND ( 'NONE', #6069, .T. ) ;
#48852=CARTESIAN_POINT ( 'NONE',  ( 101.0612956599395602, -45.30524461813642745, 282.0899109901967563 ) ) ;
#48855=DIRECTION ( 'NONE',  ( 2.089354330573420398E-14, 0.000000000000000000, 1.000000000000000000 ) ) ;
#48856=CARTESIAN_POINT ( 'NONE',  ( 95.65096329713743728, -33.45531905120653704, 141.1041967044829732 ) ) ;
#48857=CARTESIAN_POINT ( 'NONE',  ( 117.4876440797474828, -37.01562065295904347, 39.80419670448193159 ) ) ;
#48858=CARTESIAN_POINT ( 'NONE',  ( 109.4552518484143206, -25.89010755186295754, 175.8918157521009391 ) ) ;
#48861=DIRECTION ( 'NONE',  ( 1.000000000000000078E-15, 0.000000000000000000, 1.000000000000000000 ) ) ;
#48862=CARTESIAN_POINT ( 'NONE',  ( 191.6375511031381222, 22.69262065192312150, 361.9756252759109998 ) ) ;
#48863=CARTESIAN_POINT ( 'NONE',  ( 57.56670390244832447, -48.82844715994039575, 257.2178068554150627 ) ) ;
#48864=LINE ( 'NONE', #69787, #84494 ) ;
#48865=ORIENTED_EDGE ( 'NONE', *, *, #23759, .T. ) ;
#48866=AXIS2_PLACEMENT_3D ( 'NONE', #3300, #85540, #9656 ) ;
#48867=CARTESIAN_POINT ( 'NONE',  ( 70.14948329127297200, -1.929447159941395817, 342.9256252759109884 ) ) ;
#48868=EDGE_LOOP ( 'NONE', ( #54885, #38714, #20678, #54896 ) ) ;
#48869=ORIENTED_EDGE ( 'NONE', *, *, #48351, .T. ) ;
#48871=ORIENTED_EDGE ( 'NONE', *, *, #42484, .F. ) ;
#48872=CARTESIAN_POINT ( 'NONE',  ( 96.73644666290624627, -38.23103596604165233, 62.44133956162495025 ) ) ;
#48873=LINE ( 'NONE', #76155, #58556 ) ;
#48875=CARTESIAN_POINT ( 'NONE',  ( 108.9530382828359052, -26.39605832486118331, 160.9327681330539690 ) ) ;
#48876=CIRCLE ( 'NONE', #19915, 2.030000000000003801 ) ;
#48877=CARTESIAN_POINT ( 'NONE',  ( 114.3094922386577110, -31.29331878451978355, 263.7733722090294464 ) ) ;
#48878=ORIENTED_EDGE ( 'NONE', *, *, #1399, .F. ) ;
#48880=ORIENTED_EDGE ( 'NONE', *, *, #257, .F. ) ;
#48883=CARTESIAN_POINT ( 'NONE',  ( 112.0659116249482423, -45.48839625912368945, 107.9897919428080684 ) ) ;
#48884=DIRECTION ( 'NONE',  ( -0.7071067811865171526, -0.7071067811865779928, -7.071067811865164719E-16 ) ) ;
#48885=AXIS2_PLACEMENT_3D ( 'NONE', #22474, #86046, #50150 ) ;
#48887=CARTESIAN_POINT ( 'NONE',  ( 99.09610799260327951, -30.54990352127401110, 20.80127292277482098 ) ) ;
#48889=DIRECTION ( 'NONE',  ( 1.000000000000000078E-15, -1.000000000000000083E-30, -1.000000000000000000 ) ) ;
#48891=DIRECTION ( 'NONE',  ( 1.000000000000000000, 0.000000000000000000, 0.000000000000000000 ) ) ;
#48892=CARTESIAN_POINT ( 'NONE',  ( 111.0379167980823496, -47.01981040405703993, 17.85753003781598380 ) ) ;
#48893=DIRECTION ( 'NONE',  ( -0.9999999853157766072, -0.0001713722456133601202, 9.999999853157765648E-16 ) ) ;
#48895=DIRECTION ( 'NONE',  ( 0.000000000000000000, 0.000000000000000000, -1.000000000000000000 ) ) ;
#48897=CIRCLE ( 'NONE', #22813, 2.117000000000007987 ) ;
#48900=CARTESIAN_POINT ( 'NONE',  ( 104.5412336160381273, -44.52083999592182550, 80.14523322673395000 ) ) ;
#48901=ADVANCED_FACE ( 'NONE', ( #31033 ), #78768, .T. ) ;
#48903=CARTESIAN_POINT ( 'NONE',  ( 176.7738106836353325, -48.62134037874481862, 300.4678068554149490 ) ) ;
#48904=ORIENTED_EDGE ( 'NONE', *, *, #38910, .T. ) ;
#48905=ORIENTED_EDGE ( 'NONE', *, *, #347, .T. ) ;
#48906=DIRECTION ( 'NONE',  ( 0.9242245927363031965, 0.3818493186865917766, 0.000000000000000000 ) ) ;
#48907=VERTEX_POINT ( 'NONE', #79656 ) ;
#48909=CARTESIAN_POINT ( 'NONE',  ( 115.7831076793861200, -41.80230949354785253, 69.40645861076393430 ) ) ;
#48910=CARTESIAN_POINT ( 'NONE',  ( 99.14414808984345484, -41.78050036225572228, 138.1977737820869834 ) ) ;
#48912=CARTESIAN_POINT ( 'NONE',  ( 97.52247766716473620, -32.48101032970659219, 96.99276813305395706 ) ) ;
#48913=VECTOR ( 'NONE', #68441, 1000.000000000000000 ) ;
#48915=ORIENTED_EDGE ( 'NONE', *, *, #69352, .F. ) ;
#48917=DIRECTION ( 'NONE',  ( 0.000000000000000000, 1.000000000000000000, 1.541976423090495239E-15 ) ) ;
#48918=VERTEX_POINT ( 'NONE', #33722 ) ;
#48919=ORIENTED_EDGE ( 'NONE', *, *, #7878, .T. ) ;
#48921=EDGE_LOOP ( 'NONE', ( #83972, #14453 ) ) ;
#48922=CARTESIAN_POINT ( 'NONE',  ( 110.6561457788925793, -27.59554888373224557, 269.7784824187687605 ) ) ;
#48923=CARTESIAN_POINT ( 'NONE',  ( 117.3128790654603080, -34.51798396817098080, 179.9956252759109532 ) ) ;
#48924=DIRECTION ( 'NONE',  ( 1.000000000000000078E-15, 1.000000000000000083E-30, -1.000000000000000000 ) ) ;
#48926=CARTESIAN_POINT ( 'NONE',  ( 112.8017646537355176, -47.09965271489118521, 98.97848241876793907 ) ) ;
#48927=CARTESIAN_POINT ( 'NONE',  ( 115.7831076762087577, -41.80230949924659711, 263.4064586102478529 ) ) ;
#48929=CARTESIAN_POINT ( 'NONE',  ( 97.39154043693341123, -39.27946349389958414, 116.5321201934415285 ) ) ;
#48930=ADVANCED_FACE ( 'NONE', ( #60974, #68248, #32355 ), #40529, .T. ) ;
#48932=CARTESIAN_POINT ( 'NONE',  ( 101.9936390655985292, -45.44609458172816119, 133.1574646095896810 ) ) ;
#48934=CIRCLE ( 'NONE', #69341, 13.16666666666670160 ) ;
#48936=AXIS2_PLACEMENT_3D ( 'NONE', #59122, #71891, #38683 ) ;
#48937=CARTESIAN_POINT ( 'NONE',  ( 97.49412692080079523, -39.74150246419772259, 132.5691861445521056 ) ) ;
#48938=CARTESIAN_POINT ( 'NONE',  ( 104.6488677213912695, -47.51528149961286829, 27.38895860924395009 ) ) ;
#48941=DIRECTION ( 'NONE',  ( 1.000000000000000078E-15, -1.000000000000000083E-30, -1.000000000000000000 ) ) ;
#48942=CARTESIAN_POINT ( 'NONE',  ( 104.8797383215544556, -46.86635653470259655, 32.41943479972098174 ) ) ;
#48943=CARTESIAN_POINT ( 'NONE',  ( 109.7246617015826331, -27.00074531322127669, 109.8648087393802086 ) ) ;
#48944=CARTESIAN_POINT ( 'NONE',  ( 99.07096106853141748, -43.38529345585680375, 112.8784824187679732 ) ) ;
#48945=CARTESIAN_POINT ( 'NONE',  ( 115.8254323917127664, -31.73001882825242959, 70.23979194262223302 ) ) ;
#48946=CARTESIAN_POINT ( 'NONE',  ( 177.0371591254545649, -48.62818131005479927, 180.4678068554150059 ) ) ;
#48947=ORIENTED_EDGE ( 'NONE', *, *, #2861, .F. ) ;
#48948=LINE ( 'NONE', #42586, #20755 ) ;
#48950=FACE_BOUND ( 'NONE', #24606, .T. ) ;
#48951=CARTESIAN_POINT ( 'NONE',  ( 136.5970450997408534, -35.65293374834303819, 2.807537076564766920 ) ) ;
#48952=ADVANCED_FACE ( 'NONE', ( #54128 ), #75058, .F. ) ;
#48953=VERTEX_POINT ( 'NONE', #26015 ) ;
#48956=CARTESIAN_POINT ( 'NONE',  ( 101.7470617766046956, -45.74667603143129924, 162.1527681330539679 ) ) ;
#48957=ORIENTED_EDGE ( 'NONE', *, *, #63859, .T. ) ;
#48958=CARTESIAN_POINT ( 'NONE',  ( 91.42390633313587500, -35.38788608837992911, 293.6356252759109680 ) ) ;
#48959=CARTESIAN_POINT ( 'NONE',  ( 96.83718905160354495, -34.60841009949970726, 212.1641967044819808 ) ) ;
#48960=CARTESIAN_POINT ( 'NONE',  ( 105.9839165226978110, -26.31690525417204540, 46.15848241876796720 ) ) ;
#48961=CIRCLE ( 'NONE', #66345, 11.45913725231036118 ) ;
#48963=VECTOR ( 'NONE', #68520, 1000.000000000000000 ) ;
#48965=CARTESIAN_POINT ( 'NONE',  ( 117.0608945238105463, -38.08045311834111146, 78.71895860944069057 ) ) ;
#48971=EDGE_CURVE ( 'NONE', #18271, #68666, #12844, .T. ) ;
#48973=CARTESIAN_POINT ( 'NONE',  ( 184.5667039024485518, -48.82844715993447693, 180.4678068554150343 ) ) ;
#48974=CARTESIAN_POINT ( 'NONE',  ( 97.01652928432748979, -33.95800134492240119, 247.1127681330539758 ) ) ;
#48975=CARTESIAN_POINT ( 'NONE',  ( 97.66492352869934734, -33.15663352981950140, 251.0373582895531399 ) ) ;
#48976=EDGE_CURVE ( 'NONE', #6767, #85401, #73348, .T. ) ;
#48979=CARTESIAN_POINT ( 'NONE',  ( 168.3664380525669912, -48.62818131005477795, 180.4678068554150059 ) ) ;
#48980=FACE_OUTER_BOUND ( 'NONE', #61445, .T. ) ;
#48981=CARTESIAN_POINT ( 'NONE',  ( 115.6914824993820901, -43.67961476919119690, 43.27467289495795200 ) ) ;
#48984=ORIENTED_EDGE ( 'NONE', *, *, #7630, .T. ) ;
#48985=CARTESIAN_POINT ( 'NONE',  ( 172.5664832912729878, -27.82844715994070484, 258.9256252759120116 ) ) ;
#48987=CARTESIAN_POINT ( 'NONE',  ( 100.0046238269857639, -29.91446987444276928, 246.7156252759109520 ) ) ;
#48989=CARTESIAN_POINT ( 'NONE',  ( 109.6029845306728134, -46.78454271877401283, 88.78514908543394313 ) ) ;
#48991=CARTESIAN_POINT ( 'NONE',  ( 103.2779527552481795, -27.47487875237766630, 21.38567362161598595 ) ) ;
#48995=ORIENTED_EDGE ( 'NONE', *, *, #4332, .T. ) ;
#48996=ORIENTED_EDGE ( 'NONE', *, *, #27552, .F. ) ;
#48998=CARTESIAN_POINT ( 'NONE',  ( 99.03278789346684619, -40.46950289042285220, 253.1044404487540760 ) ) ;
#49000=CARTESIAN_POINT ( 'NONE',  ( 179.4595971212720258, -26.00627455219131789, 193.9678068554150059 ) ) ;
#49001=VECTOR ( 'NONE', #7659, 1000.000000000000000 ) ;
#49004=CARTESIAN_POINT ( 'NONE',  ( 115.8254323923647604, -31.73001882984776501, 84.23979194248457247 ) ) ;
#49006=ORIENTED_EDGE ( 'NONE', *, *, #58998, .T. ) ;
#49008=CIRCLE ( 'NONE', #60630, 3.299999999999999822 ) ;
#49010=ORIENTED_EDGE ( 'NONE', *, *, #44435, .F. ) ;
#49011=CARTESIAN_POINT ( 'NONE',  ( 114.0907319755898186, -46.27410096495736269, 33.08133956162495792 ) ) ;
#49013=CARTESIAN_POINT ( 'NONE',  ( 114.3408732721816534, -41.20596775705023163, 17.80956268521999419 ) ) ;
#49014=AXIS2_PLACEMENT_3D ( 'NONE', #54178, #32863, #87844 ) ;
#49015=DIRECTION ( 'NONE',  ( -4.237773401492740281E-14, 1.000000000000000000, 0.000000000000000000 ) ) ;
#49016=CARTESIAN_POINT ( 'NONE',  ( 102.2986265273211188, -45.30740241592388884, 187.1727681330549729 ) ) ;
#49018=DIRECTION ( 'NONE',  ( -1.000000000000000000, -2.756263715554006823E-15, 0.000000000000000000 ) ) ;
#49019=VECTOR ( 'NONE', #76742, 1000.000000000000000 ) ;
#49020=CARTESIAN_POINT ( 'NONE',  ( 32.15435173586061524, -31.62489322948298209, 193.9678068554150911 ) ) ;
#49022=CARTESIAN_POINT ( 'NONE',  ( 112.2081591769286177, -26.91769754996824560, 10.68038718067299087 ) ) ;
#49024=EDGE_LOOP ( 'NONE', ( #19332, #74471, #26409, #15714 ) ) ;
#49025=DIRECTION ( 'NONE',  ( 0.000000000000000000, 0.000000000000000000, -1.000000000000000000 ) ) ;
#49026=ORIENTED_EDGE ( 'NONE', *, *, #36908, .F. ) ;
#49027=CARTESIAN_POINT ( 'NONE',  ( 104.0954500313802527, -46.76767116204542418, 103.3470538473389411 ) ) ;
#49029=DIRECTION ( 'NONE',  ( 0.000000000000000000, 0.000000000000000000, 1.000000000000000000 ) ) ;
#49030=ORIENTED_EDGE ( 'NONE', *, *, #79684, .T. ) ;
#49031=LINE ( 'NONE', #21359, #47037 ) ;
#49032=VERTEX_POINT ( 'NONE', #81450 ) ;
#49034=VECTOR ( 'NONE', #1380, 999.9999999999998863 ) ;
#49035=EDGE_CURVE ( 'NONE', #77239, #11120, #40073, .T. ) ;
#49036=DIRECTION ( 'NONE',  ( 0.000000000000000000, 0.000000000000000000, -1.000000000000000000 ) ) ;
#49038=LINE ( 'NONE', #42674, #29801 ) ;
#49039=CARTESIAN_POINT ( 'NONE',  ( 29.56670390244797630, -48.82844715994099971, 20.91780685541479912 ) ) ;
#49040=DIRECTION ( 'NONE',  ( 1.000000000000000078E-15, -1.000000000000000083E-30, -1.000000000000000000 ) ) ;
#49041=CARTESIAN_POINT ( 'NONE',  ( 112.7646070568428911, -30.84607450481293256, 172.2823760838769829 ) ) ;
#49042=CARTESIAN_POINT ( 'NONE',  ( 115.7943364950945977, -30.98820711043258669, 250.2899109901966028 ) ) ;
#49043=EDGE_CURVE ( 'NONE', #33687, #61833, #5118, .T. ) ;
#49045=VERTEX_POINT ( 'NONE', #61411 ) ;
#49047=EDGE_CURVE ( 'NONE', #63446, #48213, #6460, .T. ) ;
#49048=CARTESIAN_POINT ( 'NONE',  ( 134.4433815842106412, -39.47944715994101017, 1.625625275910999257 ) ) ;
#49049=ORIENTED_EDGE ( 'NONE', *, *, #14554, .F. ) ;
#49051=EDGE_LOOP ( 'NONE', ( #2498, #42916, #75496, #60408 ) ) ;
#49053=CARTESIAN_POINT ( 'NONE',  ( 82.32434691321189746, -20.30306751045458213, 2.518077574347549419 ) ) ;
#49054=FACE_OUTER_BOUND ( 'NONE', #53104, .T. ) ;
#49055=CARTESIAN_POINT ( 'NONE',  ( 98.34981380874698687, -31.65666098073609191, 15.90646538746769778 ) ) ;
#49056=EDGE_CURVE ( 'NONE', #23436, #12855, #89140, .T. ) ;
#49057=DIRECTION ( 'NONE',  ( 0.000000000000000000, 0.000000000000000000, -1.000000000000000000 ) ) ;
#49058=FACE_OUTER_BOUND ( 'NONE', #44537, .T. ) ;
#49059=CARTESIAN_POINT ( 'NONE',  ( 100.0786887504289666, -31.81753722825460429, 205.2609912566479693 ) ) ;
#49060=CARTESIAN_POINT ( 'NONE',  ( 97.18391573584769105, -31.67496972499959895, 95.96229194257799122 ) ) ;
#49061=ORIENTED_EDGE ( 'NONE', *, *, #65373, .F. ) ;
#49062=DIRECTION ( 'NONE',  ( -0.7071067811864634178, 0.7071067811866316166, -7.071067811864642099E-16 ) ) ;
#49064=CARTESIAN_POINT ( 'NONE',  ( 52.65249034007831597, -48.32844715994060181, 249.9678068554150343 ) ) ;
#49071=CARTESIAN_POINT ( 'NONE',  ( 69.26949937496601706, -71.54137415153812185, 394.9756252759101471 ) ) ;
#49072=CARTESIAN_POINT ( 'NONE',  ( 73.17003668186728760, -8.979447159941065237, -5.074374724089063982 ) ) ;
#49075=ORIENTED_EDGE ( 'NONE', *, *, #42716, .T. ) ;
#49076=CIRCLE ( 'NONE', #50513, 0.5000000000000004441 ) ;
#49077=CARTESIAN_POINT ( 'NONE',  ( 97.33091451745008271, -32.84266655496112008, 41.02419670448193045 ) ) ;
#49078=DIRECTION ( 'NONE',  ( 1.000000000000000078E-15, -1.000000000000000083E-30, -1.000000000000000000 ) ) ;
#49080=LINE ( 'NONE', #61821, #13267 ) ;
#49081=CARTESIAN_POINT ( 'NONE',  ( 131.5185316161780804, -17.69475198630851764, 2.828485944707543442 ) ) ;
#49082=EDGE_LOOP ( 'NONE', ( #33734, #81198, #85288, #17579, #71814 ) ) ;
#49083=EDGE_CURVE ( 'NONE', #67881, #49139, #26898, .T. ) ;
#49085=B_SPLINE_CURVE_WITH_KNOTS ( 'NONE', 3,
 ( #7899, #28802, #69686, #62855, #41068, #77393, #35598, #56484, #84229, #15169, #68344, #6126, #6558, #89242, #27007, #54675, #82439, #47873 ),
 .UNSPECIFIED., .F., .F.,
 ( 4, 2, 2, 2, 2, 2, 2, 2, 4 ),
 ( 0.000000000000000000, 0.06249496329388545823, 0.1249899265877709165, 0.1874848898816563747, 0.2499798531755418329, 0.3124748164694273189, 0.3749697797633127494, 0.4374647430571981799, 0.4999597063510836659 ),
 .UNSPECIFIED. ) ;
#49086=CARTESIAN_POINT ( 'NONE',  ( 97.81170669197712186, -40.51744871389600178, 156.6352702525290681 ) ) ;
#49087=ADVANCED_FACE ( 'NONE', ( #80537 ), #66889, .T. ) ;
#49088=AXIS2_PLACEMENT_3D ( 'NONE', #54237, #19757, #47437 ) ;
#49089=CARTESIAN_POINT ( 'NONE',  ( 182.2420472961719895, -31.76306994223730840, 193.9678068554150059 ) ) ;
#49091=CARTESIAN_POINT ( 'NONE',  ( 109.2595486427728559, -46.97979643076451595, 103.7441967044829880 ) ) ;
#49092=EDGE_CURVE ( 'NONE', #12031, #41030, #87789, .T. ) ;
#49093=AXIS2_PLACEMENT_3D ( 'NONE', #59465, #88098, #4966 ) ;
#49095=DIRECTION ( 'NONE',  ( 0.000000000000000000, 0.000000000000000000, 1.000000000000000000 ) ) ;
#49096=CARTESIAN_POINT ( 'NONE',  ( 41.56648329127499153, -32.07844715994070839, 194.1756252759119832 ) ) ;
#49098=DIRECTION ( 'NONE',  ( 0.1858654558203195195, -0.9825752044157765042, 0.000000000000000000 ) ) ;
#49099=CARTESIAN_POINT ( 'NONE',  ( 102.9676436823274202, -46.25511244710193637, 133.2651490854339613 ) ) ;
#49100=AXIS2_PLACEMENT_3D ( 'NONE', #28059, #83487, #63030 ) ;
#49101=CARTESIAN_POINT ( 'NONE',  ( 107.0664832912739968, -36.72944715994100306, 287.6356252759109680 ) ) ;
#49103=CARTESIAN_POINT ( 'NONE',  ( 106.1402962346845982, -47.72062544595559785, 258.4975300378158636 ) ) ;
#49106=LINE ( 'NONE', #8247, #9564 ) ;
#49107=CARTESIAN_POINT ( 'NONE',  ( 25.56670390244797275, -62.87844715994099687, 173.2178068554149775 ) ) ;
#49110=CARTESIAN_POINT ( 'NONE',  ( 98.91665286848242999, -30.31703347128389225, 200.8080062282919869 ) ) ;
#49111=VERTEX_POINT ( 'NONE', #25553 ) ;
#49112=ORIENTED_EDGE ( 'NONE', *, *, #39762, .F. ) ;
#49114=CARTESIAN_POINT ( 'NONE',  ( 113.1089835609813719, -43.92423027677314451, 144.5520594963729764 ) ) ;
#49115=CARTESIAN_POINT ( 'NONE',  ( 21.03689327557706790, -23.42844715994186089, 300.4678068554150059 ) ) ;
#49116=CARTESIAN_POINT ( 'NONE',  ( 105.5822692374337777, -27.99308443639166555, 11.64158330589692980 ) ) ;
#49117=CARTESIAN_POINT ( 'NONE',  ( 71.24189083761808661, -0.9290567490904538817, 396.9756252759102040 ) ) ;
#49118=CARTESIAN_POINT ( 'NONE',  ( 117.0607201049021029, -38.08168303701916813, 268.7191026460068315 ) ) ;
#49121=DIRECTION ( 'NONE',  ( 0.000000000000000000, 0.000000000000000000, -1.000000000000000000 ) ) ;
#49122=CARTESIAN_POINT ( 'NONE',  ( 115.8368392028494185, -44.66223131803950963, 233.2413395616259493 ) ) ;
#49123=DIRECTION ( 'NONE',  ( 1.000000000000000078E-15, 1.000000000000000083E-30, -1.000000000000000000 ) ) ;
#49127=DIRECTION ( 'NONE',  ( 0.000000000000000000, 1.000000000000000000, 0.000000000000000000 ) ) ;
#49128=CARTESIAN_POINT ( 'NONE',  ( 82.81648064515530905, -18.72944715939135207, 6.749772901088279653 ) ) ;
#49129=CYLINDRICAL_SURFACE ( 'NONE', #53375, 0.9999999999999800160 ) ;
#49130=CARTESIAN_POINT ( 'NONE',  ( 25.56670390244797275, -58.35344715994099829, 293.2178068554150627 ) ) ;
#49131=AXIS2_PLACEMENT_3D ( 'NONE', #74382, #33037, #60730 ) ;
#49132=CARTESIAN_POINT ( 'NONE',  ( 62.03742497533751532, -23.42844715994041849, 249.9678068554150343 ) ) ;
#49134=VERTEX_POINT ( 'NONE', #53229 ) ;
#49135=CARTESIAN_POINT ( 'NONE',  ( 100.5706289694924607, -28.47478668554837000, 11.60705384733995515 ) ) ;
#49136=EDGE_CURVE ( 'NONE', #71373, #77225, #5140, .T. ) ;
#49137=CARTESIAN_POINT ( 'NONE',  ( 104.4105186412307944, -25.99981812482467092, 240.2575300378159682 ) ) ;
#49139=VERTEX_POINT ( 'NONE', #49115 ) ;
#49140=CIRCLE ( 'NONE', #89840, 5.799999999999998934 ) ;
#49142=DIRECTION ( 'NONE',  ( 0.000000000000000000, 0.000000000000000000, 1.000000000000000000 ) ) ;
#49143=LINE ( 'NONE', #75978, #74721 ) ;
#49144=DIRECTION ( 'NONE',  ( -4.299999999999999979E-14, 1.000000000000000000, 0.000000000000000000 ) ) ;
#49145=CARTESIAN_POINT ( 'NONE',  ( 109.6546009468767693, -44.98793201169110034, 50.62428084578196774 ) ) ;
#49147=CARTESIAN_POINT ( 'NONE',  ( 95.88671040095643150, -32.72508343906864781, 172.0527681330539735 ) ) ;
#49150=EDGE_LOOP ( 'NONE', ( #42133, #62010 ) ) ;
#49152=AXIS2_PLACEMENT_3D ( 'NONE', #66173, #23974, #52523 ) ;
#49154=ORIENTED_EDGE ( 'NONE', *, *, #86621, .T. ) ;
#49156=EDGE_CURVE ( 'NONE', #71659, #88009, #32753, .T. ) ;
#49158=VERTEX_POINT ( 'NONE', #41849 ) ;
#49159=EDGE_LOOP ( 'NONE', ( #1114, #65251, #43917, #73012 ) ) ;
#49160=CARTESIAN_POINT ( 'NONE',  ( 51.42025729302698522, -31.94127993907710206, -5.074374724088000832 ) ) ;
#49161=EDGE_CURVE ( 'NONE', #52237, #75709, #20551, .T. ) ;
#49162=FACE_OUTER_BOUND ( 'NONE', #41663, .T. ) ;
#49164=CARTESIAN_POINT ( 'NONE',  ( 111.5299334411454311, -29.44702005892069607, 94.06099125664896121 ) ) ;
#49165=CARTESIAN_POINT ( 'NONE',  ( 100.6426946765138695, -44.96845825347062231, 232.0499109901969632 ) ) ;
#49166=CARTESIAN_POINT ( 'NONE',  ( 95.43233898611173061, -38.84956357215551748, 201.4699109901969791 ) ) ;
#49168=CARTESIAN_POINT ( 'NONE',  ( 100.8868098461901610, -44.69967630397148639, 93.05222427096256865 ) ) ;
#49169=EDGE_CURVE ( 'NONE', #20444, #79957, #70510, .T. ) ;
#49170=EDGE_LOOP ( 'NONE', ( #8855, #34897, #19135, #88177, #89797, #50900, #85247, #48512 ) ) ;
#49175=CARTESIAN_POINT ( 'NONE',  ( 98.70071965984708129, -42.85747980491203180, 106.8175300378169652 ) ) ;
#49176=CARTESIAN_POINT ( 'NONE',  ( 116.2704737988580206, -31.74013610724590961, 69.22133956162495849 ) ) ;
#49177=CARTESIAN_POINT ( 'NONE',  ( 100.2183167550744685, -45.46532142855728864, 277.0594347997204068 ) ) ;
#49179=CARTESIAN_POINT ( 'NONE',  ( 118.7903470546216482, -38.45904373001069843, 223.7099109901969598 ) ) ;
#49180=DIRECTION ( 'NONE',  ( 1.000000000000000078E-15, 0.000000000000000000, -1.000000000000000000 ) ) ;
#49186=CARTESIAN_POINT ( 'NONE',  ( 105.2610101554027295, -25.41321098886781016, 321.3089972913614929 ) ) ;
#49187=CYLINDRICAL_SURFACE ( 'NONE', #29458, 0.2500000000000002220 ) ;
#49190=CARTESIAN_POINT ( 'NONE',  ( 97.33784129644996597, -34.07106458208137667, 12.11479194675188253 ) ) ;
#49193=DIRECTION ( 'NONE',  ( 1.000000000000000000, 0.000000000000000000, 0.000000000000000000 ) ) ;
#49194=ORIENTED_EDGE ( 'NONE', *, *, #88153, .T. ) ;
#49195=AXIS2_PLACEMENT_3D ( 'NONE', #62274, #49078, #61819 ) ;
#49197=CARTESIAN_POINT ( 'NONE',  ( 104.8365363718904888, -26.48661066032647327, 260.2470538473397710 ) ) ;
#49198=CARTESIAN_POINT ( 'NONE',  ( 102.6976273654655643, -46.88262786655960923, 133.2651490854349561 ) ) ;
#49199=CARTESIAN_POINT ( 'NONE',  ( 115.9100415161514945, -31.16808610560197224, 30.27276813305396175 ) ) ;
#49200=EDGE_CURVE ( 'NONE', #8807, #63506, #37113, .T. ) ;
#49201=PLANE ( 'NONE',  #86759 ) ;
#49203=CARTESIAN_POINT ( 'NONE',  ( 82.18073802037270070, -34.97076862298165878, 7.459445689453488626 ) ) ;
#49204=CYLINDRICAL_SURFACE ( 'NONE', #37844, 13.16666666666670160 ) ;
#49205=CIRCLE ( 'NONE', #56403, 0.5000000000000004441 ) ;
#49206=AXIS2_PLACEMENT_3D ( 'NONE', #7274, #75420, #61761 ) ;
#49208=DIRECTION ( 'NONE',  ( 0.000000000000000000, 0.000000000000000000, -1.000000000000000000 ) ) ;
#49209=ORIENTED_EDGE ( 'NONE', *, *, #15356, .T. ) ;
#49210=CARTESIAN_POINT ( 'NONE',  ( 113.1264120695652622, -29.99967374510735141, 158.9276579233149391 ) ) ;
#49211=AXIS2_PLACEMENT_3D ( 'NONE', #57053, #29822, #83900 ) ;
#49212=CARTESIAN_POINT ( 'NONE',  ( 94.06648329127393993, -36.72944715994095333, 294.6356252759106837 ) ) ;
#49214=CARTESIAN_POINT ( 'NONE',  ( 188.5667039024484097, -48.82844715993431350, 259.7178068554150059 ) ) ;
#49215=CARTESIAN_POINT ( 'NONE',  ( 112.7681627534586113, -45.43114336468919134, 174.0384824187679556 ) ) ;
#49216=PLANE ( 'NONE',  #72962 ) ;
#49219=CARTESIAN_POINT ( 'NONE',  ( 99.10117237422181802, -30.54315369407227720, 86.80178034974119328 ) ) ;
#49220=LINE ( 'NONE', #70588, #88254 ) ;
#49221=DIRECTION ( 'NONE',  ( 1.000000000000000000, 3.999999999999999995E-14, 1.000000000000000078E-15 ) ) ;
#49222=CARTESIAN_POINT ( 'NONE',  ( 109.1197153606379970, -46.32621810461561296, 107.7441967044829880 ) ) ;
#49224=ORIENTED_EDGE ( 'NONE', *, *, #45610, .T. ) ;
#49226=CARTESIAN_POINT ( 'NONE',  ( 114.2978770801668418, -41.85148020179265416, 49.76729759161096922 ) ) ;
#49227=CARTESIAN_POINT ( 'NONE',  ( 107.0664832912749915, -36.72944715993903486, 25.56312527591096995 ) ) ;
#49228=CARTESIAN_POINT ( 'NONE',  ( 113.3375292005773929, -44.23527279707077042, 189.1299109901959525 ) ) ;
#49230=CARTESIAN_POINT ( 'NONE',  ( 152.4409905591762708, -0.9151414768250908383, 394.9756252759102040 ) ) ;
#49232=CIRCLE ( 'NONE', #30384, 2.029999999999997140 ) ;
#49233=DIRECTION ( 'NONE',  ( 0.000000000000000000, 1.000000000000000000, 0.000000000000000000 ) ) ;
#49234=CARTESIAN_POINT ( 'NONE',  ( 162.7866693523289996, -36.02818131005891189, -5.074374724088000832 ) ) ;
#49235=CARTESIAN_POINT ( 'NONE',  ( 41.56648329127499153, -36.32844715994070839, 18.92562527591200094 ) ) ;
#49236=CARTESIAN_POINT ( 'NONE',  ( 96.66376384204015437, -36.61947630124858932, 111.3184824187679567 ) ) ;
#49238=ORIENTED_EDGE ( 'NONE', *, *, #54366, .F. ) ;
#49241=CARTESIAN_POINT ( 'NONE',  ( 51.34673845256598668, -36.02818131005800950, 342.9256252759119548 ) ) ;
#49242=DIRECTION ( 'NONE',  ( 0.000000000000000000, 0.000000000000000000, -1.000000000000000000 ) ) ;
#49243=CARTESIAN_POINT ( 'NONE',  ( 37.03715912545343514, -48.62818131006108757, 180.4678068554150911 ) ) ;
#49244=CARTESIAN_POINT ( 'NONE',  ( 105.1059768409772062, -45.79875505096494237, 180.2252332267349857 ) ) ;
#49246=ADVANCED_FACE ( 'NONE', ( #62760 ), #51608, .F. ) ;
#49248=LINE ( 'NONE', #21122, #84236 ) ;
#49249=EDGE_CURVE ( 'NONE', #29159, #30966, #87884, .T. ) ;
#49252=ORIENTED_EDGE ( 'NONE', *, *, #46092, .F. ) ;
#49255=CIRCLE ( 'NONE', #52155, 2.500000000000002220 ) ;
#49257=CARTESIAN_POINT ( 'NONE',  ( 162.7131505118551047, -33.70561438051486647, 313.9678068554149490 ) ) ;
#49260=CARTESIAN_POINT ( 'NONE',  ( 78.94219388974397589, -21.23922437001919761, 8.028287874532589186 ) ) ;
#49261=CARTESIAN_POINT ( 'NONE',  ( 98.52374054827556904, -34.37364049580116898, 247.5444404487539600 ) ) ;
#49263=EDGE_CURVE ( 'NONE', #57944, #70541, #6904, .T. ) ;
#49266=FACE_BOUND ( 'NONE', #77337, .T. ) ;
#49269=VERTEX_POINT ( 'NONE', #56831 ) ;
#49271=ORIENTED_EDGE ( 'NONE', *, *, #69116, .F. ) ;
#49272=EDGE_CURVE ( 'NONE', #10481, #67680, #22338, .T. ) ;
#49273=DIRECTION ( 'NONE',  ( 0.000000000000000000, -1.000000000000000000, 0.000000000000000000 ) ) ;
#49275=ORIENTED_EDGE ( 'NONE', *, *, #13395, .T. ) ;
#49277=CARTESIAN_POINT ( 'NONE',  ( 114.5169583807067966, -41.13300932163210177, 281.2318998934008505 ) ) ;
#49279=CARTESIAN_POINT ( 'NONE',  ( 114.0011561472229289, -28.09198494482817310, 119.5261014663869474 ) ) ;
#49280=CARTESIAN_POINT ( 'NONE',  ( 108.9808406375927063, -47.59218431635562041, 122.7032443235299723 ) ) ;
#49282=CYLINDRICAL_SURFACE ( 'NONE', #87325, 0.9999999999999731326 ) ;
#49284=CARTESIAN_POINT ( 'NONE',  ( 96.85852386828889848, -34.61283385893091236, 212.1641967044819808 ) ) ;
#49286=LINE ( 'NONE', #7074, #58237 ) ;
#49287=VERTEX_POINT ( 'NONE', #44091 ) ;
#49291=EDGE_LOOP ( 'NONE', ( #29009, #9272, #68049, #72120 ) ) ;
#49294=CARTESIAN_POINT ( 'NONE',  ( 112.7099490626184206, -28.41643172750246293, 135.6016206186066881 ) ) ;
#49295=VERTEX_POINT ( 'NONE', #16859 ) ;
#49296=CARTESIAN_POINT ( 'NONE',  ( 97.79409093757406879, -42.74665822538010929, 146.7965776568629508 ) ) ;
#49297=CARTESIAN_POINT ( 'NONE',  ( 119.2637946045969954, -42.39761235918182791, 25.56312527591098416 ) ) ;
#49298=B_SPLINE_CURVE_WITH_KNOTS ( 'NONE', 3,
 ( #63606, #49955, #24065, #79931, #65820, #86734, #31751, #39009, #32192, #17686, #73533, #52168, #45366, #79486, #66720, #16799, #4504, #23628 ),
 .UNSPECIFIED., .F., .F.,
 ( 4, 2, 2, 2, 2, 2, 2, 2, 4 ),
 ( 0.000000000000000000, 0.06249510223317854968, 0.1249902044663570994, 0.1874853066995356421, 0.2499804089327141987, 0.3124755111658927276, 0.3749706133990712842, 0.4374657156322498408, 0.4999608178654283974 ),
 .UNSPECIFIED. ) ;
#49301=CARTESIAN_POINT ( 'NONE',  ( 98.77692026739322273, -42.37295007796758739, 56.80169783176815912 ) ) ;
#49302=CARTESIAN_POINT ( 'NONE',  ( 97.24442698086048154, -40.26379795196656630, 262.6013395616254797 ) ) ;
#49303=CARTESIAN_POINT ( 'NONE',  ( 133.5842039024480528, -43.72944715994092491, 207.5838068554170377 ) ) ;
#49307=DIRECTION ( 'NONE',  ( 9.693101022688619289E-16, 0.000000000000000000, -1.000000000000000000 ) ) ;
#49308=CARTESIAN_POINT ( 'NONE',  ( 97.31584372507236935, -39.30597603430089748, 257.5314586121004368 ) ) ;
#49310=CARTESIAN_POINT ( 'NONE',  ( 112.8291378599181485, -28.63395795371034680, 195.5838068554166966 ) ) ;
#49311=EDGE_LOOP ( 'NONE', ( #33569, #7815, #83093, #60996, #87771, #12299, #37747, #54113, #50328, #25363, #53175, #67803, #5724, #60647, #30319, #4555, #38410, #62863, #82931, #6889, #75769, #54629, #66862, #32409, #42744, #27250, #43198, #20265, #86793, #35990, #52331, #8977, #30726, #75923, #25213, #6859, #19809, #87066, #85168, #16469, #10582, #34733, #61210, #82987, #133, #53667, #18846, #44893, #89777, #15113, #18908, #8649, #68178, #6458, #76768, #5808, #22965, #67911, #18682, #22444, #17345, #50956, #62107, #59209, #67439, #51071, #81238, #14726, #3822, #53601, #59955, #5068, #70838, #81019, #74206, #12003, #39317, #81243, #26829, #58063, #30404, #35220, #14303, #62946, #89305, #70732, #68660, #26780, #46115, #3470, #28960, #30051, #38014, #2080, #18591, #15449, #32068, #76517, #75606, #83897, #38854, #18650, #11764, #43407, #63551, #75782, #6319, #5670, #860, #31224, #5901, #54873, #31564, #488, #13863, #8991, #4808, #41279, #59197, #19846, #6270, #72624, #33400, #35410, #77346, #30015, #77925, #46590, #84009, #26276, #70619, #62521, #53162, #43777, #65569, #16793, #26813, #63228, #26198, #4433, #37437, #72337, #63047, #88155, #10538, #4716, #89086, #74096, #17282, #63164, #81306, #59324, #80035 ) ) ;
#49313=CARTESIAN_POINT ( 'NONE',  ( 118.9428397581607442, -36.92852597549882177, 153.8127681330539644 ) ) ;
#49314=CARTESIAN_POINT ( 'NONE',  ( 117.3845446746782386, -38.21944606407609513, 24.71276813305395237 ) ) ;
#49315=CARTESIAN_POINT ( 'NONE',  ( 103.5276745422693523, -26.83930826182397311, 186.3499109901969746 ) ) ;
#49316=CARTESIAN_POINT ( 'NONE',  ( 97.07207202760696418, -35.37844142050483498, 32.21895862687611611 ) ) ;
#49317=EDGE_CURVE ( 'NONE', #61816, #17322, #13894, .T. ) ;
#49318=CYLINDRICAL_SURFACE ( 'NONE', #77956, 3.000000000000002665 ) ;
#49321=DIRECTION ( 'NONE',  ( -4.237773401492740281E-14, 1.000000000000000000, 0.000000000000000000 ) ) ;
#49322=FACE_OUTER_BOUND ( 'NONE', #12334, .T. ) ;
#49326=ORIENTED_EDGE ( 'NONE', *, *, #556, .T. ) ;
#49327=VERTEX_POINT ( 'NONE', #65008 ) ;
#49328=CYLINDRICAL_SURFACE ( 'NONE', #41520, 2.517500000000005844 ) ;
#49330=CARTESIAN_POINT ( 'NONE',  ( 112.7298150101557610, -27.26422151970083263, 50.65943479972101215 ) ) ;
#49331=FACE_OUTER_BOUND ( 'NONE', #23578, .T. ) ;
#49334=EDGE_CURVE ( 'NONE', #11985, #23552, #85478, .T. ) ;
#49335=CARTESIAN_POINT ( 'NONE',  ( 116.7009037750506053, -40.82467873942847802, 164.5070538473399608 ) ) ;
#49336=B_SPLINE_CURVE_WITH_KNOTS ( 'NONE', 3,
 ( #65790, #2699, #58093, #51258, #85829, #24480, #9505, #38099, #31272, #72180, #9956, #64913, #86254, #79001, #44449, #72630, #44000, #65358 ),
 .UNSPECIFIED., .F., .F.,
 ( 4, 2, 2, 2, 2, 2, 2, 2, 4 ),
 ( 0.000000000000000000, 0.06249789214766773848, 0.1249957842953354770, 0.1874936764430032154, 0.2499915685906709539, 0.3124894607383387202, 0.3749873528860064309, 0.4374852450336741416, 0.4999831371813419079 ),
 .UNSPECIFIED. ) ;
#49337=CARTESIAN_POINT ( 'NONE',  ( 113.0872481101271205, -29.11229423309321618, 273.9667055423626039 ) ) ;
#49340=AXIS2_PLACEMENT_3D ( 'NONE', #30096, #1505, #65507 ) ;
#49342=ADVANCED_FACE ( 'NONE', ( #30928 ), #86796, .F. ) ;
#49344=DIRECTION ( 'NONE',  ( 0.000000000000000000, 0.000000000000000000, 1.000000000000000000 ) ) ;
#49345=LINE ( 'NONE', #56611, #86979 ) ;
#49346=CARTESIAN_POINT ( 'NONE',  ( 104.4895514573384077, -26.97891836813563415, 161.2814916280540558 ) ) ;
#49347=CARTESIAN_POINT ( 'NONE',  ( 102.0670549530419606, -27.97049806322867127, 75.48979194321593411 ) ) ;
#49349=CARTESIAN_POINT ( 'NONE',  ( 131.0667039024480403, -43.72944715994093201, 207.5838068554170377 ) ) ;
#49350=CARTESIAN_POINT ( 'NONE',  ( 151.5667039024485518, -48.82844715993590512, 180.4678068554149775 ) ) ;
#49352=CARTESIAN_POINT ( 'NONE',  ( 101.3960830062750063, -28.00733582429760204, 25.53562527591096654 ) ) ;
#49357=DIRECTION ( 'NONE',  ( 1.000000000000000000, 0.000000000000000000, 0.000000000000000000 ) ) ;
#49358=CARTESIAN_POINT ( 'NONE',  ( 106.8900815348805509, -46.00655951153972723, 75.37951894101996686 ) ) ;
#49361=EDGE_CURVE ( 'NONE', #9382, #63793, #85919, .T. ) ;
#49362=AXIS2_PLACEMENT_3D ( 'NONE', #19680, #32391, #53718 ) ;
#49363=CARTESIAN_POINT ( 'NONE',  ( 97.31584371710860637, -39.30597600346539622, 46.53145860958892399 ) ) ;
#49366=CARTESIAN_POINT ( 'NONE',  ( 107.0664832912739968, -36.72944715994100306, 287.6356252759109680 ) ) ;
#49368=ORIENTED_EDGE ( 'NONE', *, *, #71953, .F. ) ;
#49369=EDGE_LOOP ( 'NONE', ( #58708, #20987, #35091, #80707 ) ) ;
#49370=CARTESIAN_POINT ( 'NONE',  ( 111.3621671965809270, -45.84085784651199447, 134.3587261630399894 ) ) ;
#49374=CARTESIAN_POINT ( 'NONE',  ( 96.61744970692362244, -37.56424831167382195, 97.38991099019594344 ) ) ;
#49376=ORIENTED_EDGE ( 'NONE', *, *, #14063, .T. ) ;
#49379=ADVANCED_FACE ( 'NONE', ( #44539 ), #37754, .F. ) ;
#49381=VERTEX_POINT ( 'NONE', #9595 ) ;
#49382=CARTESIAN_POINT ( 'NONE',  ( 111.4502655420255905, -27.98611277567904310, 279.7070538473400916 ) ) ;
#49383=CARTESIAN_POINT ( 'NONE',  ( 99.99340640592768636, -27.19037833420660277, 181.5841967044829630 ) ) ;
#49386=CARTESIAN_POINT ( 'NONE',  ( 98.45872715028987443, -30.84820395253375125, 116.8499109901969604 ) ) ;
#49389=ORIENTED_EDGE ( 'NONE', *, *, #28252, .F. ) ;
#49391=AXIS2_PLACEMENT_3D ( 'NONE', #28669, #70464, #21872 ) ;
#49392=CARTESIAN_POINT ( 'NONE',  ( 104.4082832666847054, -46.45815023090534623, 133.3659487707936364 ) ) ;
#49393=VERTEX_POINT ( 'NONE', #72277 ) ;
#49396=DIRECTION ( 'NONE',  ( -1.000000000000000000, -3.999999999999999995E-14, -1.000000000000000078E-15 ) ) ;
#49397=CARTESIAN_POINT ( 'NONE',  ( 97.07516343140007109, -33.75277822987297327, 31.09562527591097592 ) ) ;
#49400=DIRECTION ( 'NONE',  ( -1.500809167996645702E-15, 0.7071067811865391350, 0.7071067811865560104 ) ) ;
#49401=CARTESIAN_POINT ( 'NONE',  ( 111.8051047218221896, -27.50533234054179843, 19.71086337114996567 ) ) ;
#49402=CARTESIAN_POINT ( 'NONE',  ( 116.3212776292267989, -32.94146857470629186, 109.1356252759109680 ) ) ;
#49403=CARTESIAN_POINT ( 'NONE',  ( 98.29923130492889527, -31.06375673945267124, 141.8699109901969564 ) ) ;
#49405=LINE ( 'NONE', #828, #59706 ) ;
#49406=ORIENTED_EDGE ( 'NONE', *, *, #16879, .F. ) ;
#49408=DIRECTION ( 'NONE',  ( 0.000000000000000000, 0.000000000000000000, 1.000000000000000000 ) ) ;
#49413=CARTESIAN_POINT ( 'NONE',  ( 98.22399452165288380, -42.33453934503185678, 186.7756252759109543 ) ) ;
#49414=ORIENTED_EDGE ( 'NONE', *, *, #86017, .T. ) ;
#49416=CARTESIAN_POINT ( 'NONE',  ( 115.4773891788847067, -29.52237647247901009, 225.4022919425769658 ) ) ;
#49417=CARTESIAN_POINT ( 'NONE',  ( 96.29363189909904008, -41.78481911317979325, 57.67562527591096710 ) ) ;
#49419=EDGE_CURVE ( 'NONE', #2137, #67480, #58616, .T. ) ;
#49421=CARTESIAN_POINT ( 'NONE',  ( 164.9667039024474491, -26.71338133338732845, 237.4678068554150059 ) ) ;
#49422=ORIENTED_EDGE ( 'NONE', *, *, #63338, .F. ) ;
#49427=AXIS2_PLACEMENT_3D ( 'NONE', #10563, #44624, #3755 ) ;
#49428=ORIENTED_EDGE ( 'NONE', *, *, #5142, .F. ) ;
#49430=CARTESIAN_POINT ( 'NONE',  ( 117.4742555207853059, -36.12881027634428222, 224.8727681330539667 ) ) ;
#49432=CARTESIAN_POINT ( 'NONE',  ( 136.4599941731241302, -17.37149686616246669, 2.653088969751947523 ) ) ;
#49433=DIRECTION ( 'NONE',  ( 2.900000000000000265E-14, -2.000000000000000155E-15, 1.000000000000000000 ) ) ;
#49435=CARTESIAN_POINT ( 'NONE',  ( 162.8913605087219878, -31.76306994223740432, -5.074374724088000832 ) ) ;
#49437=CARTESIAN_POINT ( 'NONE',  ( 110.5626142325126153, -46.61202937628593190, 37.84705384733994293 ) ) ;
#49439=VERTEX_POINT ( 'NONE', #9155 ) ;
#49440=AXIS2_PLACEMENT_3D ( 'NONE', #56304, #34072, #54501 ) ;
#49441=EDGE_CURVE ( 'NONE', #73517, #87063, #10487, .T. ) ;
#49442=CARTESIAN_POINT ( 'NONE',  ( 34.67381068360343477, -28.98061976759059988, 117.4678068554150485 ) ) ;
#49444=CARTESIAN_POINT ( 'NONE',  ( 114.9410966442421795, -29.98191058901456074, 225.4022919425769658 ) ) ;
#49446=CARTESIAN_POINT ( 'NONE',  ( 96.37928053093618530, -33.66421044892481262, 137.1041967044819501 ) ) ;
#49447=CARTESIAN_POINT ( 'NONE',  ( 179.1667039024460166, -28.27351298637280408, 342.9256252759109884 ) ) ;
#49450=ORIENTED_EDGE ( 'NONE', *, *, #20201, .F. ) ;
#49451=CYLINDRICAL_SURFACE ( 'NONE', #48752, 3.000000000000002665 ) ;
#49453=ORIENTED_EDGE ( 'NONE', *, *, #59934, .T. ) ;
#49455=CARTESIAN_POINT ( 'NONE',  ( 111.6101215911791087, -44.95330735676063938, 249.3977737820869720 ) ) ;
#49456=VECTOR ( 'NONE', #33120, 1000.000000000000000 ) ;
#49457=CARTESIAN_POINT ( 'NONE',  ( 109.6430120631640079, -46.48008675372654608, 192.7814586037220295 ) ) ;
#49459=CARTESIAN_POINT ( 'NONE',  ( 97.81375517989221180, -40.51659548082960072, 91.63516306087667829 ) ) ;
#49460=ADVANCED_FACE ( 'NONE', ( #65882 ), #3672, .F. ) ;
#49462=CARTESIAN_POINT ( 'NONE',  ( 29.56670390244797630, -67.87844715994100397, 300.9178068554150514 ) ) ;
#49463=ORIENTED_EDGE ( 'NONE', *, *, #50194, .T. ) ;
#49464=LINE ( 'NONE', #22692, #74031 ) ;
#49465=CARTESIAN_POINT ( 'NONE',  ( 97.81493411881378108, -40.51644251795452334, 167.6359250042934264 ) ) ;
#49466=ORIENTED_EDGE ( 'NONE', *, *, #57640, .F. ) ;
#49467=CARTESIAN_POINT ( 'NONE',  ( 118.0833341887621373, -37.62838194956883342, 38.77372051400595865 ) ) ;
#49469=EDGE_CURVE ( 'NONE', #23732, #35180, #7690, .T. ) ;
#49470=CARTESIAN_POINT ( 'NONE',  ( 110.3949268851355328, -45.15168757608171290, 22.31051506617198754 ) ) ;
#49472=CARTESIAN_POINT ( 'NONE',  ( 104.4091555634243349, -46.45838639981014495, 127.3648633746425105 ) ) ;
#49473=CARTESIAN_POINT ( 'NONE',  ( 106.5196382177906855, -25.62481104856546565, 195.1156252759109861 ) ) ;
#49474=DIRECTION ( 'NONE',  ( 0.000000000000000000, 0.000000000000000000, -1.000000000000000000 ) ) ;
#49477=CARTESIAN_POINT ( 'NONE',  ( 107.0664832912739399, -36.72944715994095333, 311.3356252759109566 ) ) ;
#49479=CARTESIAN_POINT ( 'NONE',  ( 99.30088202768328642, -28.79894053213705973, 266.7051490854347549 ) ) ;
#49481=VERTEX_POINT ( 'NONE', #39525 ) ;
#49482=DIRECTION ( 'NONE',  ( -1.806816776397999960E-14, 1.000000000000000000, -1.906816776398000198E-29 ) ) ;
#49483=ORIENTED_EDGE ( 'NONE', *, *, #46478, .T. ) ;
#49484=CARTESIAN_POINT ( 'NONE',  ( 97.50257212865312795, -32.47214954040395440, 96.99276813305395706 ) ) ;
#49485=CARTESIAN_POINT ( 'NONE',  ( 73.06648329127402519, -46.72944715994106701, -5.074374724089063982 ) ) ;
#49486=ORIENTED_EDGE ( 'NONE', *, *, #2764, .T. ) ;
#49487=ORIENTED_EDGE ( 'NONE', *, *, #39487, .F. ) ;
#49488=ORIENTED_EDGE ( 'NONE', *, *, #8233, .F. ) ;
#49489=EDGE_CURVE ( 'NONE', #68501, #35213, #16827, .T. ) ;
#49490=AXIS2_PLACEMENT_3D ( 'NONE', #19509, #60835, #11354 ) ;
#49491=CARTESIAN_POINT ( 'NONE',  ( 152.0368932755770288, -23.42844715993588522, 313.9678068554149490 ) ) ;
#49493=DIRECTION ( 'NONE',  ( 0.000000000000000000, 0.000000000000000000, 1.000000000000000000 ) ) ;
#49494=EDGE_CURVE ( 'NONE', #50110, #32624, #32255, .T. ) ;
#49495=CARTESIAN_POINT ( 'NONE',  ( 107.0664832912730020, -27.87844715994269862, 361.9756252759109998 ) ) ;
#49496=CARTESIAN_POINT ( 'NONE',  ( 107.0664832912739968, 12.92155284005902516, 333.4006252759110112 ) ) ;
#49497=CARTESIAN_POINT ( 'NONE',  ( 110.5551769720564863, -46.59100632561725064, 33.84705384733993583 ) ) ;
#49500=DIRECTION ( 'NONE',  ( 1.000000000000000000, 0.000000000000000000, 0.000000000000000000 ) ) ;
#49501=CARTESIAN_POINT ( 'NONE',  ( 51.56670390244799762, -33.35206098992650681, -5.074374724088000832 ) ) ;
#49502=AXIS2_PLACEMENT_3D ( 'NONE', #81410, #40032, #19157 ) ;
#49505=AXIS2_PLACEMENT_3D ( 'NONE', #16237, #2156, #43913 ) ;
#49506=PLANE ( 'NONE',  #56094 ) ;
#49507=LINE ( 'NONE', #64947, #45488 ) ;
#49510=CARTESIAN_POINT ( 'NONE',  ( 50.88849390559499142, -32.11662333284530746, -5.074374724088000832 ) ) ;
#49511=CARTESIAN_POINT ( 'NONE',  ( 103.1098180292659947, -44.29918505015107399, 211.6152769709339623 ) ) ;
#49514=CARTESIAN_POINT ( 'NONE',  ( 106.6586145429690475, -26.26807492067915462, 85.10705384733896040 ) ) ;
#49518=CYLINDRICAL_SURFACE ( 'NONE', #60017, 0.5000000000000104361 ) ;
#49522=EDGE_LOOP ( 'NONE', ( #88599, #88809, #58931, #42610 ) ) ;
#49523=DIRECTION ( 'NONE',  ( 1.000000000000000078E-15, -1.000000000000000083E-30, -1.000000000000000000 ) ) ;
#49526=AXIS2_PLACEMENT_3D ( 'NONE', #53762, #55104, #26093 ) ;
#49528=EDGE_LOOP ( 'NONE', ( #8557, #53989, #62718, #83167 ) ) ;
#49529=CARTESIAN_POINT ( 'NONE',  ( 104.4852212567679004, -46.88943973524933995, 47.37848241876796607 ) ) ;
#49533=EDGE_CURVE ( 'NONE', #71638, #74855, #54514, .T. ) ;
#49534=DIRECTION ( 'NONE',  ( -0.9999999853157766072, -0.0001713722456143218888, 0.000000000000000000 ) ) ;
#49540=FACE_OUTER_BOUND ( 'NONE', #80916, .T. ) ;
#49541=CARTESIAN_POINT ( 'NONE',  ( 109.0764703591063522, -47.62188296335364157, 123.7337205140059666 ) ) ;
#49542=FACE_OUTER_BOUND ( 'NONE', #69805, .T. ) ;
#49543=CARTESIAN_POINT ( 'NONE',  ( 20.56670390244828184, -48.82844715994187368, 300.4678068554150059 ) ) ;
#49548=CARTESIAN_POINT ( 'NONE',  ( 116.5825849560771417, -39.12894369053751120, 119.6299109901959525 ) ) ;
#49552=CARTESIAN_POINT ( 'NONE',  ( 118.0799254396264786, -36.12288750354066735, 269.8822919425776945 ) ) ;
#49553=DIRECTION ( 'NONE',  ( -0.000000000000000000, 1.000000000000000000, 0.000000000000000000 ) ) ;
#49555=PLANE ( 'NONE',  #63239 ) ;
#49556=CARTESIAN_POINT ( 'NONE',  ( 45.56670390244421753, -48.82844715994099971, 129.9678068554150911 ) ) ;
#49560=CARTESIAN_POINT ( 'NONE',  ( 114.3351522754913674, -30.13549343754558407, 209.4127681330539872 ) ) ;
#49561=VERTEX_POINT ( 'NONE', #66328 ) ;
#49564=CARTESIAN_POINT ( 'NONE',  ( 115.7737780547358710, -35.08282516751891933, 155.4072975916109556 ) ) ;
#49565=VECTOR ( 'NONE', #9757, 1000.000000000000000 ) ;
#49566=DIRECTION ( 'NONE',  ( 0.000000000000000000, 0.000000000000000000, -1.000000000000000000 ) ) ;
#49567=CARTESIAN_POINT ( 'NONE',  ( 115.9456366428866119, -37.20155953748186306, 15.21586902018295895 ) ) ;
#49568=DIRECTION ( 'NONE',  ( -0.0001713722455994998422, 0.9999999853157766072, 0.000000000000000000 ) ) ;
#49570=DIRECTION ( 'NONE',  ( 1.000000000000000000, 4.163336342344333240E-14, 0.000000000000000000 ) ) ;
#49571=CARTESIAN_POINT ( 'NONE',  ( 74.38348329127296665, -71.52944715994142655, 342.9256252759110453 ) ) ;
#49572=LINE ( 'NONE', #542, #78342 ) ;
#49574=CARTESIAN_POINT ( 'NONE',  ( 107.5091008941355994, -47.12332782054438951, 237.6099109901969655 ) ) ;
#49577=EDGE_CURVE ( 'NONE', #57432, #74315, #81776, .T. ) ;
#49579=VECTOR ( 'NONE', #72824, 1000.000000000000000 ) ;
#49584=AXIS2_PLACEMENT_3D ( 'NONE', #89452, #69899, #82653 ) ;
#49585=CARTESIAN_POINT ( 'NONE',  ( 100.8224265971273326, -29.20115443902030705, 36.62705384733894221 ) ) ;
#49586=DIRECTION ( 'NONE',  ( 0.7071067811865513475, -0.7071067811865436870, 7.071067811865519707E-16 ) ) ;
#49589=CARTESIAN_POINT ( 'NONE',  ( 111.3409431244321439, -27.17319409035083666, 20.74133956162494030 ) ) ;
#49590=PLANE ( 'NONE',  #71451 ) ;
#49591=CARTESIAN_POINT ( 'NONE',  ( 106.1383370350330324, -47.74387551462719159, 262.4975300378158636 ) ) ;
#49592=ORIENTED_EDGE ( 'NONE', *, *, #60861, .T. ) ;
#49593=VECTOR ( 'NONE', #77141, 1000.000000000000114 ) ;
#49600=EDGE_CURVE ( 'NONE', #77142, #3395, #80886, .T. ) ;
#49601=CARTESIAN_POINT ( 'NONE',  ( 100.5332814249895108, -41.62301430380158962, 64.65666179816298609 ) ) ;
#49602=CARTESIAN_POINT ( 'NONE',  ( 114.8301775850900128, -29.68641892472961175, 205.4127681330539872 ) ) ;
#49603=LINE ( 'NONE', #87715, #44941 ) ;
#49604=VERTEX_POINT ( 'NONE', #74048 ) ;
#49605=CIRCLE ( 'NONE', #72834, 2.029999999999997140 ) ;
#49607=CYLINDRICAL_SURFACE ( 'NONE', #24799, 0.4999999999999982236 ) ;
#49609=ORIENTED_EDGE ( 'NONE', *, *, #88052, .T. ) ;
#49610=CARTESIAN_POINT ( 'NONE',  ( 163.0664832912739826, 22.62155284005901024, 333.4006252759110112 ) ) ;
#49612=ORIENTED_EDGE ( 'NONE', *, *, #32195, .T. ) ;
#49613=CARTESIAN_POINT ( 'NONE',  ( 179.4595971212723100, -26.00627455218570461, 313.9678068554149490 ) ) ;
#49614=CARTESIAN_POINT ( 'NONE',  ( 107.9985670441620726, -25.30821118569420491, 321.5222355017487530 ) ) ;
#49615=CARTESIAN_POINT ( 'NONE',  ( 114.9386757252747771, -33.34113070369811993, 78.57241982807700253 ) ) ;
#49616=CARTESIAN_POINT ( 'NONE',  ( 97.53973001301494605, -43.81993288943278486, 261.8356252759109566 ) ) ;
#49617=CARTESIAN_POINT ( 'NONE',  ( 177.0664832912730162, 12.92155284005730387, 355.9756252759109998 ) ) ;
#49619=ORIENTED_EDGE ( 'NONE', *, *, #58033, .F. ) ;
#49620=VERTEX_POINT ( 'NONE', #69480 ) ;
#49621=DIRECTION ( 'NONE',  ( 1.000000000000000000, 4.163336342344333240E-14, 0.000000000000000000 ) ) ;
#49622=VECTOR ( 'NONE', #63413, 1000.000000000000000 ) ;
#49623=DIRECTION ( 'NONE',  ( -4.237773401492740281E-14, 1.000000000000000000, 0.000000000000000000 ) ) ;
#49624=CARTESIAN_POINT ( 'NONE',  ( 163.0664832912739826, 12.92155284005902516, 330.1506252759110680 ) ) ;
#49625=AXIS2_PLACEMENT_3D ( 'NONE', #32494, #73842, #66573 ) ;
#49626=CARTESIAN_POINT ( 'NONE',  ( 99.34849973496650932, -28.72665311504486141, 115.6870538473399534 ) ) ;
#49627=CARTESIAN_POINT ( 'NONE',  ( 116.7155050624037926, -32.57635518107161943, 79.14991099019697174 ) ) ;
#49628=DIRECTION ( 'NONE',  ( 1.000000000000000000, 4.163336342344333240E-14, 0.000000000000000000 ) ) ;
#49630=UNCERTAINTY_MEASURE_WITH_UNIT (LENGTH_MEASURE( 1.000000000000000082E-05 ), #38593, 'distance_accuracy_value', 'NONE');
#49631=CARTESIAN_POINT ( 'NONE',  ( 96.51793475972648650, -31.32865002300666646, 245.9499109901969689 ) ) ;
#49632=DIRECTION ( 'NONE',  ( 2.056463827196271584E-15, -0.8571673007021100021, 0.5150380749100580413 ) ) ;
#49634=LINE ( 'NONE', #62822, #73510 ) ;
#49636=FACE_OUTER_BOUND ( 'NONE', #53523, .T. ) ;
#49637=CARTESIAN_POINT ( 'NONE',  ( 105.0850183953499197, -25.44292241093928553, 321.8714993217711822 ) ) ;
#49643=DIRECTION ( 'NONE',  ( 0.000000000000000000, -1.000000000000000000, 0.000000000000000000 ) ) ;
#49644=VECTOR ( 'NONE', #73834, 1000.000000000000000 ) ;
#49645=CARTESIAN_POINT ( 'NONE',  ( 97.07207205388709781, -35.37844123507927918, 261.2189586121116918 ) ) ;
#49648=CARTESIAN_POINT ( 'NONE',  ( 115.2691655829841579, -30.20224515277380917, 244.3613395616249875 ) ) ;
#49649=CARTESIAN_POINT ( 'NONE',  ( 97.74639642956380214, -42.67166664343270099, 137.7661014663869992 ) ) ;
#49650=CARTESIAN_POINT ( 'NONE',  ( 116.1774319148507573, -31.53050193741562524, 285.2384824187680579 ) ) ;
#49653=CARTESIAN_POINT ( 'NONE',  ( 90.44969454456413871, -50.82895651782494895, 229.5838068554169809 ) ) ;
#49654=CARTESIAN_POINT ( 'NONE',  ( 117.0608918343000653, -38.08047937793136128, 139.7189565292726172 ) ) ;
#49655=VECTOR ( 'NONE', #65834, 1000.000000000000000 ) ;
#49658=ADVANCED_FACE ( 'NONE', ( #82679 ), #75843, .T. ) ;
#49659=DIRECTION ( 'NONE',  ( 0.000000000000000000, 0.000000000000000000, -1.000000000000000000 ) ) ;
#49661=AXIS2_PLACEMENT_3D ( 'NONE', #80720, #65294, #54756 ) ;
#49662=CARTESIAN_POINT ( 'NONE',  ( 113.5378671157686910, -31.15474330070945541, 183.8152769709339793 ) ) ;
#49663=EDGE_CURVE ( 'NONE', #29598, #55608, #42200, .T. ) ;
#49665=VERTEX_POINT ( 'NONE', #49000 ) ;
#49666=LINE ( 'NONE', #77848, #82376 ) ;
#49667=CARTESIAN_POINT ( 'NONE',  ( 97.40233316251689644, -42.04621543282986096, 172.7146728949589942 ) ) ;
#49668=DIRECTION ( 'NONE',  ( -4.299999999999999979E-14, 1.000000000000000000, -4.400000000000000367E-29 ) ) ;
#49669=FACE_OUTER_BOUND ( 'NONE', #33018, .T. ) ;
#49671=ADVANCED_FACE ( 'NONE', ( #34494, #7256 ), #52185, .F. ) ;
#49672=EDGE_CURVE ( 'NONE', #10162, #52592, #83121, .T. ) ;
#49673=DIRECTION ( 'NONE',  ( 2.900000000000000265E-14, -2.000000000000000155E-15, 1.000000000000000000 ) ) ;
#49675=CARTESIAN_POINT ( 'NONE',  ( 107.9743429475490615, -26.39917242597363867, 109.9946728949599759 ) ) ;
#49676=ORIENTED_EDGE ( 'NONE', *, *, #51917, .T. ) ;
#49680=CARTESIAN_POINT ( 'NONE',  ( 98.44267559312871185, -33.00030968290830202, 57.44539282970595195 ) ) ;
#49682=( BOUNDED_CURVE ( )  B_SPLINE_CURVE ( 3, ( #4099, #59493, #67671, #25888 ),
 .UNSPECIFIED., .F., .T. ) 
 B_SPLINE_CURVE_WITH_KNOTS ( ( 4, 4 ),
 ( 1.504499544760546481, 1.569169445332449397 ),
 .UNSPECIFIED. ) 
 CURVE ( )  GEOMETRIC_REPRESENTATION_ITEM ( )  RATIONAL_B_SPLINE_CURVE ( ( 1.000000000000000000, 0.9996515140281859724, 0.9996515140281859724, 1.000000000000000000 ) ) 
 REPRESENTATION_ITEM ( '' )  );
#49683=CARTESIAN_POINT ( 'NONE',  ( 118.1473594538625349, -37.63838399483782382, 184.7613395616249647 ) ) ;
#49685=DIRECTION ( 'NONE',  ( 0.000000000000000000, -1.000000000000000000, 0.000000000000000000 ) ) ;
#49686=EDGE_CURVE ( 'NONE', #82238, #19244, #34037, .T. ) ;
#49688=CARTESIAN_POINT ( 'NONE',  ( 162.7131505118539962, -33.70561438052090608, 193.9678068554150059 ) ) ;
#49690=DIRECTION ( 'NONE',  ( 0.000000000000000000, 0.000000000000000000, 1.000000000000000000 ) ) ;
#49691=CARTESIAN_POINT ( 'NONE',  ( 125.0664851986225443, -56.72944715994101728, -4.824374724089012467 ) ) ;
#49692=EDGE_CURVE ( 'NONE', #2723, #18676, #61894, .T. ) ;
#49693=CARTESIAN_POINT ( 'NONE',  ( 113.8422018911647484, -44.62364141802228090, 108.1413395616249744 ) ) ;
#49694=ORIENTED_EDGE ( 'NONE', *, *, #78519, .T. ) ;
#49695=VERTEX_POINT ( 'NONE', #432 ) ;
#49696=EDGE_CURVE ( 'NONE', #69894, #23016, #42637, .T. ) ;
#49697=EDGE_LOOP ( 'NONE', ( #23896, #34762, #26207, #72754, #79602, #25355 ) ) ;
#49700=DIRECTION ( 'NONE',  ( -4.237773401492740281E-14, 1.000000000000000000, 0.000000000000000000 ) ) ;
#49701=DIRECTION ( 'NONE',  ( -0.4214249218767880945, -0.9068632946707806397, -4.214249218767889924E-16 ) ) ;
#49702=CARTESIAN_POINT ( 'NONE',  ( 109.4710126485015280, -28.41565358443893174, 212.6585665600669870 ) ) ;
#49703=CIRCLE ( 'NONE', #70016, 3.299999999999997158 ) ;
#49704=CARTESIAN_POINT ( 'NONE',  ( 31.90335556477799628, -33.89581943344391135, 237.4678068554150059 ) ) ;
#49705=CARTESIAN_POINT ( 'NONE',  ( 19.56670390244734747, -25.42844715994192129, 300.4678068554150059 ) ) ;
#49707=ORIENTED_EDGE ( 'NONE', *, *, #11256, .F. ) ;
#49711=ORIENTED_EDGE ( 'NONE', *, *, #25781, .T. ) ;
#49714=ADVANCED_FACE ( 'NONE', ( #49908 ), #13174, .T. ) ;
#49716=CARTESIAN_POINT ( 'NONE',  ( 115.9273305379513062, -35.98950415022901694, 250.3244404487543022 ) ) ;
#49717=CARTESIAN_POINT ( 'NONE',  ( 154.4532655810165238, -72.54279768053240218, 540.9756252759101471 ) ) ;
#49718=ORIENTED_EDGE ( 'NONE', *, *, #17430, .F. ) ;
#49720=CARTESIAN_POINT ( 'NONE',  ( 179.1667039024460166, -26.71338133339251542, -5.074374724088000832 ) ) ;
#49721=DIRECTION ( 'NONE',  ( 0.000000000000000000, 0.000000000000000000, 1.000000000000000000 ) ) ;
#49722=EDGE_LOOP ( 'NONE', ( #11259, #12401 ) ) ;
#49723=EDGE_LOOP ( 'NONE', ( #28731, #52758, #67366, #7762 ) ) ;
#49724=AXIS2_PLACEMENT_3D ( 'NONE', #75797, #12678, #13563 ) ;
#49729=CARTESIAN_POINT ( 'NONE',  ( 115.8942015304759252, -33.87145029861233070, 281.8938046553057575 ) ) ;
#49730=CARTESIAN_POINT ( 'NONE',  ( 102.0403423364015509, -46.60028036886249225, 172.2137205140059564 ) ) ;
#49731=CARTESIAN_POINT ( 'NONE',  ( 107.6020193903983824, -26.30459096080988246, 95.03562527591097364 ) ) ;
#49733=FACE_OUTER_BOUND ( 'NONE', #63358, .T. ) ;
#49734=CARTESIAN_POINT ( 'NONE',  ( 110.0520154068402263, -26.08705182471624795, 215.8708633711489711 ) ) ;
#49737=ORIENTED_EDGE ( 'NONE', *, *, #17689, .T. ) ;
#49739=ORIENTED_EDGE ( 'NONE', *, *, #2789, .T. ) ;
#49740=ORIENTED_EDGE ( 'NONE', *, *, #49441, .F. ) ;
#49741=CARTESIAN_POINT ( 'NONE',  ( 21.03689327557705369, -23.42844715994186089, 313.9678068554150059 ) ) ;
#49742=VERTEX_POINT ( 'NONE', #52462 ) ;
#49743=CARTESIAN_POINT ( 'NONE',  ( 96.69902036285651548, -37.82614351231516281, 126.4099109901969626 ) ) ;
#49744=CARTESIAN_POINT ( 'NONE',  ( 31.71315051185499811, -33.70561438052111214, -5.074374724088000832 ) ) ;
#49745=CARTESIAN_POINT ( 'NONE',  ( 135.6073602527815183, -34.45223222829677212, 7.843813999039347173 ) ) ;
#49746=FACE_OUTER_BOUND ( 'NONE', #43084, .T. ) ;
#49747=LINE ( 'NONE', #57012, #53394 ) ;
#49749=CARTESIAN_POINT ( 'NONE',  ( 99.34937008002601999, -28.84845824588786911, 266.7051490854347549 ) ) ;
#49754=PLANE ( 'NONE',  #19577 ) ;
#49755=CARTESIAN_POINT ( 'NONE',  ( 165.9667039024459996, -26.71338133339301635, -5.074374724088000832 ) ) ;
#49757=CARTESIAN_POINT ( 'NONE',  ( 118.1498169324930529, -36.11903826555217023, 273.8822919425775808 ) ) ;
#49758=ORIENTED_EDGE ( 'NONE', *, *, #87559, .T. ) ;
#49760=CARTESIAN_POINT ( 'NONE',  ( 117.3318588842742685, -34.78817910010258174, 158.9756252759109714 ) ) ;
#49761=CARTESIAN_POINT ( 'NONE',  ( 115.6112259330891305, -28.51835778375803798, 35.43562527591098643 ) ) ;
#49762=CARTESIAN_POINT ( 'NONE',  ( 115.0729613760110084, -29.04219751930509119, 185.4232443235299570 ) ) ;
#49764=LINE ( 'NONE', #1650, #14133 ) ;
#49767=CARTESIAN_POINT ( 'NONE',  ( 29.56670390244797630, -67.87844715994100397, 20.91780685541479912 ) ) ;
#49769=EDGE_LOOP ( 'NONE', ( #73662, #66214, #27170, #52005 ) ) ;
#49772=ADVANCED_FACE ( 'NONE', ( #65671 ), #72058, .F. ) ;
#49773=ORIENTED_EDGE ( 'NONE', *, *, #19493, .F. ) ;
#49774=EDGE_CURVE ( 'NONE', #43762, #36567, #38857, .T. ) ;
#49776=EDGE_CURVE ( 'NONE', #77006, #11339, #44417, .T. ) ;
#49778=ORIENTED_EDGE ( 'NONE', *, *, #23144, .F. ) ;
#49779=CARTESIAN_POINT ( 'NONE',  ( 115.0059970501926330, -43.50650750775896825, 59.26419670448196086 ) ) ;
#49780=LINE ( 'NONE', #70694, #29534 ) ;
#49783=CARTESIAN_POINT ( 'NONE',  ( 98.05313438099307177, -42.12366292992533801, 157.7556252759109725 ) ) ;
#49784=CARTESIAN_POINT ( 'NONE',  ( 101.3905103160957850, -43.11219441383617124, 266.4209912566481080 ) ) ;
#49786=ORIENTED_EDGE ( 'NONE', *, *, #35730, .F. ) ;
#49787=ORIENTED_EDGE ( 'NONE', *, *, #79758, .T. ) ;
#49789=AXIS2_PLACEMENT_3D ( 'NONE', #34338, #14367, #6643 ) ;
#49791=CARTESIAN_POINT ( 'NONE',  ( 109.6430121338576953, -46.48008673429469439, 107.7814586095166334 ) ) ;
#49792=CARTESIAN_POINT ( 'NONE',  ( 21.03689327557711763, -23.42844715994186089, 249.9678068554150059 ) ) ;
#49793=DIRECTION ( 'NONE',  ( -1.000000000000000000, 0.000000000000000000, 0.000000000000000000 ) ) ;
#49795=DIRECTION ( 'NONE',  ( -1.000000000000000000, 0.000000000000000000, 0.000000000000000000 ) ) ;
#49797=LINE ( 'NONE', #6682, #74176 ) ;
#49801=CARTESIAN_POINT ( 'NONE',  ( 95.28387218206118803, -35.72034718286344201, 36.25848241876794731 ) ) ;
#49803=EDGE_CURVE ( 'NONE', #52054, #46455, #72000, .T. ) ;
#49804=EDGE_LOOP ( 'NONE', ( #71578, #42395, #2598, #56887 ) ) ;
#49807=CARTESIAN_POINT ( 'NONE',  ( 112.4846873277006267, -29.98081840548436006, 117.3442808457819666 ) ) ;
#49809=VECTOR ( 'NONE', #64094, 1000.000000000000000 ) ;
#49810=DIRECTION ( 'NONE',  ( -0.7071067811865165975, -0.7071067811865784369, -7.071067811865158803E-16 ) ) ;
#49812=EDGE_LOOP ( 'NONE', ( #31235, #69274 ) ) ;
#49813=ORIENTED_EDGE ( 'NONE', *, *, #22556, .T. ) ;
#49814=CARTESIAN_POINT ( 'NONE',  ( 97.81316109541715775, -40.52102254706596796, 136.6363148235126630 ) ) ;
#49815=AXIS2_PLACEMENT_3D ( 'NONE', #3767, #11017, #24654 ) ;
#49816=VERTEX_POINT ( 'NONE', #79330 ) ;
#49818=CARTESIAN_POINT ( 'NONE',  ( 99.43677639672335999, -41.29559517668970869, 158.1872975916109567 ) ) ;
#49819=CARTESIAN_POINT ( 'NONE',  ( 80.06648329127402519, -46.72944715994105991, 4.925625275910944012 ) ) ;
#49820=EDGE_CURVE ( 'NONE', #61816, #45134, #17094, .T. ) ;
#49821=CARTESIAN_POINT ( 'NONE',  ( 117.3749687695755171, -38.63058443890392368, 84.68133956162593279 ) ) ;
#49822=VECTOR ( 'NONE', #23822, 1000.000000000000000 ) ;
#49823=CARTESIAN_POINT ( 'NONE',  ( 72.31648329127402519, -56.72944715994105991, 14.67562527591093513 ) ) ;
#49824=ORIENTED_EDGE ( 'NONE', *, *, #16682, .F. ) ;
#49825=VERTEX_POINT ( 'NONE', #33839 ) ;
#49826=ORIENTED_EDGE ( 'NONE', *, *, #72057, .F. ) ;
#49827=CARTESIAN_POINT ( 'NONE',  ( 114.1400169897070924, -40.01656155057797548, 9.125625275910977052 ) ) ;
#49828=ORIENTED_EDGE ( 'NONE', *, *, #60209, .T. ) ;
#49829=CARTESIAN_POINT ( 'NONE',  ( 97.12559377168363994, -39.79659400623925336, 21.56419670448195092 ) ) ;
#49830=CARTESIAN_POINT ( 'NONE',  ( 117.4480285489056683, -30.96353277002295101, 175.2299109901969700 ) ) ;
#49831=FACE_OUTER_BOUND ( 'NONE', #89855, .T. ) ;
#49832=CARTESIAN_POINT ( 'NONE',  ( 51.56670390244899238, -32.29483332968450782, 237.4678068554150059 ) ) ;
#49833=CARTESIAN_POINT ( 'NONE',  ( 95.67524734051724522, -33.46228404877688689, 137.1041967044819501 ) ) ;
#49837=EDGE_CURVE ( 'NONE', #23384, #86581, #41092, .T. ) ;
#49838=EDGE_LOOP ( 'NONE', ( #77371, #5698, #21196, #42352 ) ) ;
#49839=LINE ( 'NONE', #8080, #70929 ) ;
#49841=ORIENTED_EDGE ( 'NONE', *, *, #1912, .F. ) ;
#49842=CIRCLE ( 'NONE', #64391, 12.99999999999999822 ) ;
#49844=LINE ( 'NONE', #43473, #43136 ) ;
#49846=CARTESIAN_POINT ( 'NONE',  ( 111.3232390708907786, -27.21277439355663219, 24.74133956162494030 ) ) ;
#49849=DIRECTION ( 'NONE',  ( 0.000000000000000000, 0.000000000000000000, 1.000000000000000000 ) ) ;
#49851=CARTESIAN_POINT ( 'NONE',  ( 106.9359508110862720, -26.91635713860562973, 60.08705384733998045 ) ) ;
#49852=DIRECTION ( 'NONE',  ( -4.237773401492740281E-14, 1.000000000000000000, 0.000000000000000000 ) ) ;
#49853=CARTESIAN_POINT ( 'NONE',  ( 99.11802762103509679, -45.48540990049882282, 152.9899109901969894 ) ) ;
#49855=CARTESIAN_POINT ( 'NONE',  ( 41.56648329127399677, 0.2215528400590013880, 138.9256252759119832 ) ) ;
#49856=ORIENTED_EDGE ( 'NONE', *, *, #67419, .T. ) ;
#49857=CARTESIAN_POINT ( 'NONE',  ( 89.06648138392552028, -56.72944715994104570, 14.67562527591095289 ) ) ;
#49858=CARTESIAN_POINT ( 'NONE',  ( 142.8698897858160706, -0.9167816978817300289, 394.9756252759102040 ) ) ;
#49860=ORIENTED_EDGE ( 'NONE', *, *, #48026, .T. ) ;
#49861=LINE ( 'NONE', #63504, #50527 ) ;
#49862=CARTESIAN_POINT ( 'NONE',  ( 113.7790015168560558, -44.76367177190390834, 193.1299109901969757 ) ) ;
#49865=CARTESIAN_POINT ( 'NONE',  ( 113.1681127151884141, -26.54159316308081173, 200.6470538473399756 ) ) ;
#49866=CARTESIAN_POINT ( 'NONE',  ( 103.8278507311454177, -46.72190801433284690, 78.32705384733995402 ) ) ;
#49867=LINE ( 'NONE', #77599, #49001 ) ;
#49868=CARTESIAN_POINT ( 'NONE',  ( 22.49541547940886588, 22.69262065192414468, 361.9756252759109998 ) ) ;
#49869=CARTESIAN_POINT ( 'NONE',  ( 156.5667039024481255, -42.82844715993568485, 257.2178068554149490 ) ) ;
#49870=ORIENTED_EDGE ( 'NONE', *, *, #15090, .F. ) ;
#49873=CIRCLE ( 'NONE', #10709, 2.500000000000002220 ) ;
#49874=CIRCLE ( 'NONE', #10711, 9.999999999999998224 ) ;
#49876=ORIENTED_EDGE ( 'NONE', *, *, #44221, .F. ) ;
#49877=EDGE_CURVE ( 'NONE', #60674, #81215, #46556, .T. ) ;
#49878=EDGE_LOOP ( 'NONE', ( #85610, #31054, #23250, #4833, #88548, #52470, #45991, #43456, #19130, #83456, #65208, #38120, #81773, #60760 ) ) ;
#49880=ORIENTED_EDGE ( 'NONE', *, *, #16411, .F. ) ;
#49882=CARTESIAN_POINT ( 'NONE',  ( 115.9598434605651107, -30.16574962093465828, 255.3203871806729524 ) ) ;
#49883=DIRECTION ( 'NONE',  ( -0.7071067811865774377, 0.7071067811865175967, -7.071067811865782003E-16 ) ) ;
#49884=CARTESIAN_POINT ( 'NONE',  ( 135.1249450788499757, -16.19118199975284611, 1.799893109327562524 ) ) ;
#49885=EDGE_CURVE ( 'NONE', #17889, #56291, #60637, .T. ) ;
#49886=CARTESIAN_POINT ( 'NONE',  ( 41.56648329127499153, -32.07844715994070839, 23.67562527591200094 ) ) ;
#49887=DIRECTION ( 'NONE',  ( 0.000000000000000000, 0.000000000000000000, -1.000000000000000000 ) ) ;
#49889=CARTESIAN_POINT ( 'NONE',  ( 118.1065893711158594, -37.63027948749972751, 38.77372051400595865 ) ) ;
#49890=ORIENTED_EDGE ( 'NONE', *, *, #60384, .F. ) ;
#49892=ADVANCED_FACE ( 'NONE', ( #54701 ), #33394, .T. ) ;
#49893=CARTESIAN_POINT ( 'NONE',  ( 115.8264675611344359, -31.73180946705375050, 15.24044151184909168 ) ) ;
#49894=CARTESIAN_POINT ( 'NONE',  ( 110.7503267229639476, -45.78994093226354778, 278.8841967044818375 ) ) ;
#49895=ADVANCED_FACE ( 'NONE', ( #19770, #39748 ), #53806, .F. ) ;
#49896=DIRECTION ( 'NONE',  ( 1.000000000000000078E-15, -1.000000000000000083E-30, -1.000000000000000000 ) ) ;
#49897=CARTESIAN_POINT ( 'NONE',  ( 108.2018929880948548, -26.98138995270375062, 125.9841967044819597 ) ) ;
#49899=CARTESIAN_POINT ( 'NONE',  ( 116.3289480479917017, -32.94026123176625731, 29.13562527591096085 ) ) ;
#49901=CARTESIAN_POINT ( 'NONE',  ( 188.5667039024479834, -65.37844715994100397, 293.2178068554150627 ) ) ;
#49902=CARTESIAN_POINT ( 'NONE',  ( 97.53184938156154260, -39.74897048756918849, 57.57051766616469024 ) ) ;
#49903=ORIENTED_EDGE ( 'NONE', *, *, #36808, .F. ) ;
#49906=CARTESIAN_POINT ( 'NONE',  ( 111.8242684682981718, -44.20552626741085334, 259.4587261630397848 ) ) ;
#49907=AXIS2_PLACEMENT_3D ( 'NONE', #76018, #21973, #26980 ) ;
#49908=FACE_OUTER_BOUND ( 'NONE', #54838, .T. ) ;
#49910=LINE ( 'NONE', #42202, #20075 ) ;
#49911=DIRECTION ( 'NONE',  ( 0.000000000000000000, 1.000000000000000000, 0.000000000000000000 ) ) ;
#49912=ORIENTED_EDGE ( 'NONE', *, *, #35262, .T. ) ;
#49914=DIRECTION ( 'NONE',  ( 0.000000000000000000, 0.000000000000000000, -1.000000000000000000 ) ) ;
#49915=ORIENTED_EDGE ( 'NONE', *, *, #89926, .T. ) ;
#49916=CARTESIAN_POINT ( 'NONE',  ( 106.8411850752606966, -48.57806423327891565, 77.56133956162491927 ) ) ;
#49917=ORIENTED_EDGE ( 'NONE', *, *, #78649, .T. ) ;
#49918=CARTESIAN_POINT ( 'NONE',  ( 99.98530978427844218, -41.10337153935440568, 11.19051506617196878 ) ) ;
#49920=CARTESIAN_POINT ( 'NONE',  ( 116.0678243078411498, -40.55558035091543445, 168.5070538473399608 ) ) ;
#49922=DIRECTION ( 'NONE',  ( -0.000000000000000000, -0.000000000000000000, 1.000000000000000000 ) ) ;
#49923=CARTESIAN_POINT ( 'NONE',  ( 172.5664832912729878, -18.82844715994071194, 315.9256252759120684 ) ) ;
#49924=EDGE_CURVE ( 'NONE', #49695, #12195, #66201, .T. ) ;
#49926=CARTESIAN_POINT ( 'NONE',  ( 105.1008636489907673, -25.80544433381534475, 271.2061014663873380 ) ) ;
#49928=ORIENTED_EDGE ( 'NONE', *, *, #4090, .T. ) ;
#49929=DIRECTION ( 'NONE',  ( 1.000000000000000000, 1.040834085586083310E-14, 0.000000000000000000 ) ) ;
#49930=VECTOR ( 'NONE', #70269, 999.9999999999998863 ) ;
#49932=CARTESIAN_POINT ( 'NONE',  ( 102.5975616584704966, -46.88947854763195267, 128.2346728949589760 ) ) ;
#49933=CARTESIAN_POINT ( 'NONE',  ( 79.41328093380936082, -21.40256188477534494, 1.689562700882486723 ) ) ;
#49935=VECTOR ( 'NONE', #21728, 1000.000000000000000 ) ;
#49936=VERTEX_POINT ( 'NONE', #27472 ) ;
#49937=VERTEX_POINT ( 'NONE', #46995 ) ;
#49938=ORIENTED_EDGE ( 'NONE', *, *, #51912, .F. ) ;
#49939=CIRCLE ( 'NONE', #47009, 11.57110091390437034 ) ;
#49940=DIRECTION ( 'NONE',  ( 0.000000000000000000, 0.000000000000000000, -1.000000000000000000 ) ) ;
#49942=CARTESIAN_POINT ( 'NONE',  ( 105.7995281078892873, -26.72403387351276294, 266.1772911773911119 ) ) ;
#49944=DIRECTION ( 'NONE',  ( 0.000000000000000000, 1.000000000000000000, 0.000000000000000000 ) ) ;
#49946=CARTESIAN_POINT ( 'NONE',  ( 115.8915968718629017, -31.17968520675552924, 30.27276813305396175 ) ) ;
#49947=CARTESIAN_POINT ( 'NONE',  ( 162.7131505118539962, -33.70561438052090608, -5.074374724088000832 ) ) ;
#49948=EDGE_LOOP ( 'NONE', ( #18470, #20197, #12882, #67239 ) ) ;
#49949=CARTESIAN_POINT ( 'NONE',  ( 127.0664832912738973, -54.72944906728955772, -4.970821333495670125 ) ) ;
#49950=CARTESIAN_POINT ( 'NONE',  ( 115.7831080051488613, -41.80230922285955586, 43.40611986575648018 ) ) ;
#49951=ORIENTED_EDGE ( 'NONE', *, *, #55902, .F. ) ;
#49954=CARTESIAN_POINT ( 'NONE',  ( 82.63685198412170507, -19.70758306363565637, 2.855952960430490073 ) ) ;
#49955=CARTESIAN_POINT ( 'NONE',  ( 116.8182998100438965, -34.15748031063536416, 115.0320983290675656 ) ) ;
#49957=B_SPLINE_CURVE_WITH_KNOTS ( 'NONE', 3,
 ( #37366, #65072, #57804, #72342, #10110, #78725, #85982, #2854, #40381, #19047, #5429, #37818, #30107, #79168, #19494, #23318, #60364, #33124 ),
 .UNSPECIFIED., .F., .F.,
 ( 4, 2, 2, 2, 2, 2, 2, 2, 4 ),
 ( 0.000000000000000000, 0.06250000002257644072, 0.1250000000451528814, 0.1875000000677293222, 0.2500000000903057629, 0.3125000001128822036, 0.3750000001354586443, 0.4375000001580350850, 0.5000000001806115257 ),
 .UNSPECIFIED. ) ;
#49958=FACE_BOUND ( 'NONE', #11231, .T. ) ;
#49960=CARTESIAN_POINT ( 'NONE',  ( 100.5279579596103332, -31.18870816475473262, 215.1895626852199541 ) ) ;
#49961=DIRECTION ( 'NONE',  ( -4.299999999999999979E-14, 1.000000000000000000, -4.100000000000000342E-29 ) ) ;
#49962=CARTESIAN_POINT ( 'NONE',  ( 107.0664832912739968, -36.72944715994100306, -1.864374724089012947 ) ) ;
#49963=CARTESIAN_POINT ( 'NONE',  ( 96.03104818302425372, -37.92613241492836806, 81.40038718067299328 ) ) ;
#49964=ORIENTED_EDGE ( 'NONE', *, *, #7693, .T. ) ;
#49965=DIRECTION ( 'NONE',  ( 0.000000000000000000, 0.000000000000000000, 1.000000000000000000 ) ) ;
#49966=ORIENTED_EDGE ( 'NONE', *, *, #3749, .T. ) ;
#49967=CARTESIAN_POINT ( 'NONE',  ( 161.4809174648185888, -48.32844715993547169, 129.9678068554149775 ) ) ;
#49968=CARTESIAN_POINT ( 'NONE',  ( 167.2371591254543546, -47.82818131005522844, 237.4678068554150059 ) ) ;
#49969=ORIENTED_EDGE ( 'NONE', *, *, #62898, .F. ) ;
#49971=ORIENTED_EDGE ( 'NONE', *, *, #78221, .F. ) ;
#49972=CARTESIAN_POINT ( 'NONE',  ( 57.56670390244808289, -42.82844715994040286, 254.7178068554150627 ) ) ;
#49974=AXIS2_PLACEMENT_3D ( 'NONE', #17279, #44957, #38159 ) ;
#49976=VERTEX_POINT ( 'NONE', #20669 ) ;
#49977=CARTESIAN_POINT ( 'NONE',  ( 117.8794170024721240, -39.13275856168890243, 103.6403871806729455 ) ) ;
#49978=CIRCLE ( 'NONE', #9352, 10.04999999999999361 ) ;
#49979=DIRECTION ( 'NONE',  ( 0.08544974978095713769, 0.9963424814100680926, -0.000000000000000000 ) ) ;
#49981=CARTESIAN_POINT ( 'NONE',  ( 134.0664832912740110, -41.22944715994101017, 10.42562527591099553 ) ) ;
#49983=ORIENTED_EDGE ( 'NONE', *, *, #76241, .F. ) ;
#49986=CARTESIAN_POINT ( 'NONE',  ( 83.06670390244796920, -61.87844715994100397, 201.9838068554149970 ) ) ;
#49987=DIRECTION ( 'NONE',  ( 0.000000000000000000, 0.000000000000000000, 1.000000000000000000 ) ) ;
#49988=EDGE_CURVE ( 'NONE', #50110, #23298, #61531, .T. ) ;
#49990=CARTESIAN_POINT ( 'NONE',  ( 103.1665349694895895, -27.03781871365087142, 126.3813395616259783 ) ) ;
#49991=EDGE_CURVE ( 'NONE', #34477, #2880, #51678, .T. ) ;
#49992=CARTESIAN_POINT ( 'NONE',  ( 29.56670390244797630, -48.82844715994099971, 300.9178068554150514 ) ) ;
#49993=DIRECTION ( 'NONE',  ( -0.7071067811865165975, -0.7071067811865784369, -7.071067811865470403E-16 ) ) ;
#49995=CIRCLE ( 'NONE', #6495, 0.5000000000000004441 ) ;
#49996=ORIENTED_EDGE ( 'NONE', *, *, #65477, .F. ) ;
#49998=CIRCLE ( 'NONE', #20966, 13.00000000000000355 ) ;
#49999=AXIS2_PLACEMENT_3D ( 'NONE', #50196, #50647, #35225 ) ;
#50000=CARTESIAN_POINT ( 'NONE',  ( 109.2168187703260998, -26.58475186820039582, 180.9222919425769760 ) ) ;
#50005=CIRCLE ( 'NONE', #20976, 2.117000000000000881 ) ;
#50006=CARTESIAN_POINT ( 'NONE',  ( 111.8803037788896262, -27.54327565145516488, 10.68038718067199078 ) ) ;
#50007=CARTESIAN_POINT ( 'NONE',  ( 179.8585841295800094, -30.08671355700241179, -5.074374724088000832 ) ) ;
#50008=LINE ( 'NONE', #66662, #72212 ) ;
#50010=CARTESIAN_POINT ( 'NONE',  ( 29.56648329127400388, 25.62155284005901379, 328.6381252759109088 ) ) ;
#50011=FACE_BOUND ( 'NONE', #65739, .T. ) ;
#50012=CARTESIAN_POINT ( 'NONE',  ( 111.3277751695583078, -45.53312973143663811, 247.9356252759109509 ) ) ;
#50013=VERTEX_POINT ( 'NONE', #62440 ) ;
#50014=VERTEX_POINT ( 'NONE', #53358 ) ;
#50015=CARTESIAN_POINT ( 'NONE',  ( 108.6634326348915351, -27.98234008310821608, 161.3644404487539816 ) ) ;
#50017=CARTESIAN_POINT ( 'NONE',  ( 113.0371668699568204, -44.84250099658410704, 29.51301187732496700 ) ) ;
#50018=DIRECTION ( 'NONE',  ( 1.000000000000000000, 0.000000000000000000, 0.000000000000000000 ) ) ;
#50019=CARTESIAN_POINT ( 'NONE',  ( 172.5664832912740110, 0.2215528400590013880, 81.04262527591200183 ) ) ;
#50021=DIRECTION ( 'NONE',  ( -2.999999999999999839E-15, 1.000000000000000000, -2.999999999999999900E-30 ) ) ;
#50022=DIRECTION ( 'NONE',  ( -2.900000000000000265E-14, 2.000000000000000155E-15, -1.000000000000000000 ) ) ;
#50023=CARTESIAN_POINT ( 'NONE',  ( 103.3114313307233658, -27.02747569519249993, 215.3699109901969848 ) ) ;
#50026=ORIENTED_EDGE ( 'NONE', *, *, #88043, .T. ) ;
#50029=DIRECTION ( 'NONE',  ( 0.000000000000000000, 0.000000000000000000, -1.000000000000000000 ) ) ;
#50030=FACE_OUTER_BOUND ( 'NONE', #13816, .T. ) ;
#50032=AXIS2_PLACEMENT_3D ( 'NONE', #14106, #63599, #49500 ) ;
#50033=CARTESIAN_POINT ( 'NONE',  ( 101.3196941207357469, -46.24713579373438677, 48.14419670448194211 ) ) ;
#50034=DIRECTION ( 'NONE',  ( -0.7071067811985215501, 0.7071067811745735954, 0.000000000000000000 ) ) ;
#50038=VECTOR ( 'NONE', #75693, 1000.000000000000000 ) ;
#50040=CARTESIAN_POINT ( 'NONE',  ( 98.94247553594858857, -30.19587780982054070, 240.7870538473399620 ) ) ;
#50042=ORIENTED_EDGE ( 'NONE', *, *, #80467, .F. ) ;
#50043=CARTESIAN_POINT ( 'NONE',  ( 78.16547420785481393, -38.71744337668656044, 7.623533105427367396 ) ) ;
#50045=DIRECTION ( 'NONE',  ( -3.999999999999999995E-14, 1.000000000000000000, -4.100000000000000342E-29 ) ) ;
#50046=CARTESIAN_POINT ( 'NONE',  ( 100.7929862627584754, -41.95179922106267156, 114.6966617981629639 ) ) ;
#50047=CARTESIAN_POINT ( 'NONE',  ( 98.51983665003312751, -30.72177789114069313, 201.8384824187679385 ) ) ;
#50048=CARTESIAN_POINT ( 'NONE',  ( 142.8698897858160706, -0.9167816978817300289, 394.9756252759102040 ) ) ;
#50050=DIRECTION ( 'NONE',  ( 4.299999999999999979E-14, -1.000000000000000000, 0.000000000000000000 ) ) ;
#50051=ORIENTED_EDGE ( 'NONE', *, *, #45794, .T. ) ;
#50052=ORIENTED_EDGE ( 'NONE', *, *, #34101, .F. ) ;
#50054=EDGE_CURVE ( 'NONE', #69712, #61365, #27917, .T. ) ;
#50055=CONICAL_SURFACE ( 'NONE', #36981, 1.258749999999999369, 1.029744258676650093 ) ;
#50056=CARTESIAN_POINT ( 'NONE',  ( 107.0664832912750057, -36.72944715993903486, 0.4256252759109709349 ) ) ;
#50060=CARTESIAN_POINT ( 'NONE',  ( 115.0385986129619482, -42.90675649914010137, 169.3030387614307699 ) ) ;
#50062=CARTESIAN_POINT ( 'NONE',  ( 97.33783257808994449, -34.07109485886046230, 42.11472017254328648 ) ) ;
#50063=CARTESIAN_POINT ( 'NONE',  ( 112.2084326156563066, -29.27471527533065299, 89.03051506617198640 ) ) ;
#50064=CIRCLE ( 'NONE', #13840, 18.00000000000000355 ) ;
#50065=CARTESIAN_POINT ( 'NONE',  ( 100.1628669375702714, -45.39175184048325917, 272.0289586092442278 ) ) ;
#50066=FACE_OUTER_BOUND ( 'NONE', #5491, .T. ) ;
#50069=VECTOR ( 'NONE', #29022, 1000.000000000000000 ) ;
#50070=EDGE_CURVE ( 'NONE', #52647, #1233, #14760, .T. ) ;
#50072=DIRECTION ( 'NONE',  ( 1.000000000000000078E-15, -1.000000000000000083E-30, -1.000000000000000000 ) ) ;
#50073=CARTESIAN_POINT ( 'NONE',  ( 156.5667039024484097, -48.82844715993568485, 175.7178068554150059 ) ) ;
#50076=CARTESIAN_POINT ( 'NONE',  ( 113.4367438382844284, -44.15125393826594546, 108.1413395616259692 ) ) ;
#50077=CARTESIAN_POINT ( 'NONE',  ( 104.9539341177782177, -25.01766106605714768, 125.2184824187689856 ) ) ;
#50080=CARTESIAN_POINT ( 'NONE',  ( 109.2120108049357299, -48.38436871983039111, 277.7213395616254843 ) ) ;
#50081=DIRECTION ( 'NONE',  ( 4.299999999999999979E-14, -1.000000000000000000, 4.400000000000000367E-29 ) ) ;
#50083=VECTOR ( 'NONE', #83298, 1000.000000000000000 ) ;
#50084=FACE_OUTER_BOUND ( 'NONE', #52829, .T. ) ;
#50087=DIRECTION ( 'NONE',  ( -1.000000000000000000, 1.011922027653136551E-15, 0.000000000000000000 ) ) ;
#50088=CARTESIAN_POINT ( 'NONE',  ( 132.3477924061170370, -38.87777042261645732, 7.743969477062123019 ) ) ;
#50090=DIRECTION ( 'NONE',  ( 0.000000000000000000, 0.000000000000000000, -1.000000000000000000 ) ) ;
#50091=ADVANCED_FACE ( 'NONE', ( #29718, #57411 ), #9274, .T. ) ;
#50092=LINE ( 'NONE', #84650, #70980 ) ;
#50093=CARTESIAN_POINT ( 'NONE',  ( 49.21437657594998427, -35.91149509761070391, -5.074374724088000832 ) ) ;
#50094=VERTEX_POINT ( 'NONE', #48790 ) ;
#50096=CARTESIAN_POINT ( 'NONE',  ( 104.3185787381473375, -25.99890841748068482, 245.2880062282919482 ) ) ;
#50097=CARTESIAN_POINT ( 'NONE',  ( 109.8559662660393172, -26.68448463234438606, 170.8613395616249591 ) ) ;
#50098=CARTESIAN_POINT ( 'NONE',  ( 116.3557873595856336, -41.55669258580370951, 284.4441967044824082 ) ) ;
#50100=CARTESIAN_POINT ( 'NONE',  ( 82.78382032693660619, -36.30343833343673765, 6.798133076501194694 ) ) ;
#50101=CARTESIAN_POINT ( 'NONE',  ( 97.86667236827629779, -40.64944809824318384, 137.6470064143673255 ) ) ;
#50106=ORIENTED_EDGE ( 'NONE', *, *, #17491, .T. ) ;
#50107=CARTESIAN_POINT ( 'NONE',  ( 112.4896002948435410, -43.98220334580144453, 187.5219436376009696 ) ) ;
#50109=CARTESIAN_POINT ( 'NONE',  ( 117.0599855631655544, -38.08685173747024066, 188.7190441128558120 ) ) ;
#50110=VERTEX_POINT ( 'NONE', #37423 ) ;
#50112=CARTESIAN_POINT ( 'NONE',  ( 98.45302666770176359, -29.83944080489372652, 191.7775300378159784 ) ) ;
#50113=CARTESIAN_POINT ( 'NONE',  ( 41.56648329127398966, -27.82844715994070484, 194.1756252759119832 ) ) ;
#50116=CARTESIAN_POINT ( 'NONE',  ( 180.2121375201600131, -29.73316016639650172, -5.074374724088000832 ) ) ;
#50118=CARTESIAN_POINT ( 'NONE',  ( 110.8563607029707327, -45.98346426043695345, 97.88578756584530538 ) ) ;
#50119=CARTESIAN_POINT ( 'NONE',  ( 102.6819511611810753, -27.33185899950643005, 135.4118157521019441 ) ) ;
#50121=VERTEX_POINT ( 'NONE', #78780 ) ;
#50123=CARTESIAN_POINT ( 'NONE',  ( 105.1055546886446308, -45.37138199117224957, 68.83015473446796761 ) ) ;
#50125=FACE_OUTER_BOUND ( 'NONE', #22172, .T. ) ;
#50127=CARTESIAN_POINT ( 'NONE',  ( 106.9806506443342755, -46.50983917909364607, 183.5699109901959787 ) ) ;
#50130=LINE ( 'NONE', #55584, #43623 ) ;
#50132=CARTESIAN_POINT ( 'NONE',  ( 107.0664832912739399, -36.72944715994095333, 302.6356252759109680 ) ) ;
#50133=DIRECTION ( 'NONE',  ( -1.000000000000000000, 0.000000000000000000, 0.000000000000000000 ) ) ;
#50135=CARTESIAN_POINT ( 'NONE',  ( 108.0321269276242049, -25.74166508409281917, 109.9946728949589811 ) ) ;
#50138=ORIENTED_EDGE ( 'NONE', *, *, #18826, .T. ) ;
#50139=AXIS2_PLACEMENT_3D ( 'NONE', #16076, #76950, #42848 ) ;
#50142=CARTESIAN_POINT ( 'NONE',  ( 117.0608945232069971, -38.08045312423180917, 79.71895860897220132 ) ) ;
#50143=DIRECTION ( 'NONE',  ( -1.000000000000000000, -4.299999999999999979E-14, -1.000000000000000078E-15 ) ) ;
#50144=CIRCLE ( 'NONE', #34191, 0.5000000000000004441 ) ;
#50145=CARTESIAN_POINT ( 'NONE',  ( 111.0898924481313941, -43.83169361959101451, 210.8052332267339750 ) ) ;
#50146=CARTESIAN_POINT ( 'NONE',  ( 34.67381068362099228, -26.00627455219321860, -5.074374724088000832 ) ) ;
#50149=CARTESIAN_POINT ( 'NONE',  ( 102.0817216996469483, -27.57306688727539168, 145.4727681330539610 ) ) ;
#50150=DIRECTION ( 'NONE',  ( 0.000000000000000000, 0.000000000000000000, -1.000000000000000000 ) ) ;
#50152=EDGE_LOOP ( 'NONE', ( #53147, #10405 ) ) ;
#50155=ORIENTED_EDGE ( 'NONE', *, *, #44441, .T. ) ;
#50156=ORIENTED_EDGE ( 'NONE', *, *, #44259, .F. ) ;
#50157=CARTESIAN_POINT ( 'NONE',  ( 78.64532134555092568, -21.08531275930071658, 7.905164235254865446 ) ) ;
#50158=LINE ( 'NONE', #86494, #4906 ) ;
#50159=CARTESIAN_POINT ( 'NONE',  ( 98.34725308318749626, -40.22966859802066608, 248.0739642582779538 ) ) ;
#50160=CARTESIAN_POINT ( 'NONE',  ( 90.06648329127391150, -36.72944715993925513, -5.074374724089047106 ) ) ;
#50162=CARTESIAN_POINT ( 'NONE',  ( 115.6637425838761430, -40.30355366565792252, 9.635625275910941312 ) ) ;
#50163=CARTESIAN_POINT ( 'NONE',  ( 177.0664832912740110, 12.92155284005802685, 349.2756252759111248 ) ) ;
#50164=ORIENTED_EDGE ( 'NONE', *, *, #62518, .F. ) ;
#50165=EDGE_LOOP ( 'NONE', ( #68537, #19665, #89739, #77650 ) ) ;
#50167=CARTESIAN_POINT ( 'NONE',  ( 113.1931473032385185, -44.64809289480323429, 113.1005158354814597 ) ) ;
#50169=ORIENTED_EDGE ( 'NONE', *, *, #14336, .T. ) ;
#50170=CARTESIAN_POINT ( 'NONE',  ( 107.8084489643801334, -27.48037055177216104, 262.8309475124484038 ) ) ;
#50171=EDGE_CURVE ( 'NONE', #26178, #667, #52785, .T. ) ;
#50172=CARTESIAN_POINT ( 'NONE',  ( 114.3594209402202182, -29.19941241435835266, 174.4641967044819637 ) ) ;
#50173=CARTESIAN_POINT ( 'NONE',  ( 105.3199149336540046, -48.42511963160334432, 147.4584824187679715 ) ) ;
#50174=DIRECTION ( 'NONE',  ( 0.000000000000000000, 0.000000000000000000, -1.000000000000000000 ) ) ;
#50175=DIRECTION ( 'NONE',  ( 1.000000000000000078E-15, -1.000000000000000083E-30, -1.000000000000000000 ) ) ;
#50176=CARTESIAN_POINT ( 'NONE',  ( 97.91927484100293100, -41.73055353899491138, 217.7241967044829494 ) ) ;
#50178=CARTESIAN_POINT ( 'NONE',  ( 63.03715912545818156, -46.82818131006018092, 313.9678068554150059 ) ) ;
#50179=ORIENTED_EDGE ( 'NONE', *, *, #44966, .F. ) ;
#50181=EDGE_CURVE ( 'NONE', #60890, #20236, #34306, .T. ) ;
#50182=EDGE_LOOP ( 'NONE', ( #71883, #2997, #28145, #81846 ) ) ;
#50185=CIRCLE ( 'NONE', #47319, 4.875000000000017764 ) ;
#50186=EDGE_CURVE ( 'NONE', #21752, #10255, #13960, .T. ) ;
#50188=CARTESIAN_POINT ( 'NONE',  ( 108.6818361061225602, -26.38549717321916788, 189.9527681330539792 ) ) ;
#50189=VERTEX_POINT ( 'NONE', #86920 ) ;
#50191=CARTESIAN_POINT ( 'NONE',  ( 107.3339538991774447, -26.30757161206916095, 120.0556252759109555 ) ) ;
#50194=EDGE_CURVE ( 'NONE', #13929, #5997, #11047, .T. ) ;
#50195=CARTESIAN_POINT ( 'NONE',  ( 135.5773992616565238, -34.43204134599594113, 7.859568798196992390 ) ) ;
#50196=CARTESIAN_POINT ( 'NONE',  ( 165.9667039024459996, -26.71338133339301635, -5.074374724088000832 ) ) ;
#50197=DIRECTION ( 'NONE',  ( -2.999999999999999839E-15, 1.000000000000000000, -2.999999999999999900E-30 ) ) ;
#50198=CARTESIAN_POINT ( 'NONE',  ( 111.7879433275918473, -45.58683771644975025, 57.96604673916865380 ) ) ;
#50199=CARTESIAN_POINT ( 'NONE',  ( 100.2624651760415873, -28.85963121439202794, 256.6441967044821695 ) ) ;
#50203=DIRECTION ( 'NONE',  ( -1.000000000000000000, -4.299999999999999979E-14, -1.000000000000000078E-15 ) ) ;
#50207=CARTESIAN_POINT ( 'NONE',  ( 112.8675307907708287, -28.58609239232746546, 195.5838076129389833 ) ) ;
#50208=ORIENTED_EDGE ( 'NONE', *, *, #36853, .T. ) ;
#50210=CARTESIAN_POINT ( 'NONE',  ( 103.4607332334527001, -46.53479866174185986, 142.2956252759109645 ) ) ;
#50211=CARTESIAN_POINT ( 'NONE',  ( 107.2322063299336605, -25.67745564896214816, 76.07657765686298035 ) ) ;
#50212=CARTESIAN_POINT ( 'NONE',  ( 95.35923950155199691, -38.86288465644625489, 197.4699109901969791 ) ) ;
#50213=CARTESIAN_POINT ( 'NONE',  ( 194.0371591254572934, -24.42818131005417825, 300.4678068554149490 ) ) ;
#50214=FACE_OUTER_BOUND ( 'NONE', #6321, .T. ) ;
#50218=CARTESIAN_POINT ( 'NONE',  ( 97.07207206176971681, -35.37844117946191602, 71.21895860768269415 ) ) ;
#50222=( BOUNDED_CURVE ( )  B_SPLINE_CURVE ( 3, ( #26610, #5736, #21488, #77340 ),
 .UNSPECIFIED., .F., .T. ) 
 B_SPLINE_CURVE_WITH_KNOTS ( ( 4, 4 ),
 ( 4.646092198350340041, 4.647722573419572178 ),
 .UNSPECIFIED. ) 
 CURVE ( )  GEOMETRIC_REPRESENTATION_ITEM ( )  RATIONAL_B_SPLINE_CURVE ( ( 1.000000000000000000, 0.9999997784897733943, 0.9999997784897733943, 1.000000000000000000 ) ) 
 REPRESENTATION_ITEM ( '' )  );
#50225=EDGE_CURVE ( 'NONE', #39116, #42164, #44211, .T. ) ;
#50226=CARTESIAN_POINT ( 'NONE',  ( 37.06648329127298780, 12.92155284005730387, 361.9756252759109998 ) ) ;
#50227=VERTEX_POINT ( 'NONE', #68266 ) ;
#50228=CARTESIAN_POINT ( 'NONE',  ( 117.9019101119219357, -41.46671778014663801, 54.49848241876792088 ) ) ;
#50229=FACE_OUTER_BOUND ( 'NONE', #21234, .T. ) ;
#50230=EDGE_CURVE ( 'NONE', #54776, #2723, #55039, .T. ) ;
#50231=EDGE_CURVE ( 'NONE', #23923, #77722, #70637, .T. ) ;
#50232=DIRECTION ( 'NONE',  ( 4.299999999999999979E-14, -1.000000000000000000, 4.400000000000000367E-29 ) ) ;
#50233=CARTESIAN_POINT ( 'NONE',  ( 96.00064313654479520, -35.86649870909684523, 187.2765776568629406 ) ) ;
#50235=CARTESIAN_POINT ( 'NONE',  ( 106.3060546692423145, -45.75354925581387278, 261.9200388756959796 ) ) ;
#50236=ORIENTED_EDGE ( 'NONE', *, *, #37803, .F. ) ;
#50240=LINE ( 'NONE', #57510, #21692 ) ;
#50241=DIRECTION ( 'NONE',  ( 1.387778780781444492E-15, 0.000000000000000000, -1.000000000000000000 ) ) ;
#50246=DIRECTION ( 'NONE',  ( -0.7071067811865794361, 0.7071067811865157093, -7.071067811865492096E-16 ) ) ;
#50247=CARTESIAN_POINT ( 'NONE',  ( 115.5933672690474765, -28.53551910654237389, 39.43562527591099354 ) ) ;
#50250=VECTOR ( 'NONE', #791, 1000.000000000000114 ) ;
#50252=CARTESIAN_POINT ( 'NONE',  ( 107.2759047676296120, -28.56943069780466971, 117.8738046553059462 ) ) ;
#50253=AXIS2_PLACEMENT_3D ( 'NONE', #57289, #50022, #2351 ) ;
#50254=VECTOR ( 'NONE', #29042, 1000.000000000000000 ) ;
#50255=CIRCLE ( 'NONE', #35738, 2.999999999999919176 ) ;
#50256=DIRECTION ( 'NONE',  ( 1.000000000000000078E-15, 0.000000000000000000, -1.000000000000000000 ) ) ;
#50257=LINE ( 'NONE', #86145, #79337 ) ;
#50258=ORIENTED_EDGE ( 'NONE', *, *, #86822, .F. ) ;
#50259=ORIENTED_EDGE ( 'NONE', *, *, #73789, .T. ) ;
#50261=ORIENTED_EDGE ( 'NONE', *, *, #18189, .T. ) ;
#50262=VERTEX_POINT ( 'NONE', #67804 ) ;
#50263=CARTESIAN_POINT ( 'NONE',  ( 111.0851542815211985, -27.49251106464650007, 131.1815833058969645 ) ) ;
#50266=CARTESIAN_POINT ( 'NONE',  ( 104.1016336957795261, -46.74677842777965253, 103.3470538473389411 ) ) ;
#50267=CARTESIAN_POINT ( 'NONE',  ( 101.9933438188864159, -45.44590076357884101, 17.15650773109305760 ) ) ;
#50268=ORIENTED_EDGE ( 'NONE', *, *, #73155, .F. ) ;
#50269=AXIS2_PLACEMENT_3D ( 'NONE', #51629, #71658, #24396 ) ;
#50270=ORIENTED_EDGE ( 'NONE', *, *, #86312, .T. ) ;
#50271=VERTEX_POINT ( 'NONE', #48233 ) ;
#50274=CARTESIAN_POINT ( 'NONE',  ( 100.9301527464941444, -28.27416411254235840, 75.57562527591093726 ) ) ;
#50275=EDGE_LOOP ( 'NONE', ( #42990, #22985, #36227, #15132 ) ) ;
#50276=CARTESIAN_POINT ( 'NONE',  ( 114.8131502045276449, -44.70447909941025699, 268.1899109901970633 ) ) ;
#50277=CARTESIAN_POINT ( 'NONE',  ( 115.0562973506820157, -29.05819712879207017, 185.4232443235299570 ) ) ;
#50278=FACE_BOUND ( 'NONE', #59549, .T. ) ;
#50280=CARTESIAN_POINT ( 'NONE',  ( 104.9628592394672069, -25.06714115267218546, 121.2184824187679766 ) ) ;
#50281=LINE ( 'NONE', #2159, #30622 ) ;
#50282=VERTEX_POINT ( 'NONE', #89605 ) ;
#50283=FACE_OUTER_BOUND ( 'NONE', #22678, .T. ) ;
#50285=ADVANCED_FACE ( 'NONE', ( #87804 ), #54142, .T. ) ;
#50286=ORIENTED_EDGE ( 'NONE', *, *, #26504, .T. ) ;
#50287=CARTESIAN_POINT ( 'NONE',  ( 109.6435279985285405, -46.47996157675320461, 133.7827314339946554 ) ) ;
#50290=EDGE_LOOP ( 'NONE', ( #10844, #67224, #62119, #89235 ) ) ;
#50291=VECTOR ( 'NONE', #70096, 1000.000000000000114 ) ;
#50295=CARTESIAN_POINT ( 'NONE',  ( 117.3847603239957635, -38.21947720531817083, 28.71276813305395592 ) ) ;
#50298=LINE ( 'NONE', #56668, #2837 ) ;
#50299=CARTESIAN_POINT ( 'NONE',  ( 57.56670390244829605, -48.82844715994039575, 290.7178068554150627 ) ) ;
#50300=CARTESIAN_POINT ( 'NONE',  ( 97.89279369561084820, -33.33727167892450183, 66.04419670448297097 ) ) ;
#50301=CARTESIAN_POINT ( 'NONE',  ( 97.60806933018331222, -39.98294871649164861, 111.5901086304039751 ) ) ;
#50302=CARTESIAN_POINT ( 'NONE',  ( 105.7232414704440941, -24.98023492732646744, 156.1670538473399574 ) ) ;
#50307=CARTESIAN_POINT ( 'NONE',  ( 156.5667039024485803, -48.82844715993568485, 137.2178068554149775 ) ) ;
#50309=ORIENTED_EDGE ( 'NONE', *, *, #67405, .F. ) ;
#50310=EDGE_CURVE ( 'NONE', #78458, #83951, #3277, .T. ) ;
#50311=CARTESIAN_POINT ( 'NONE',  ( 63.03715912545741418, -46.82818131006016671, 117.4678068554150485 ) ) ;
#50312=CARTESIAN_POINT ( 'NONE',  ( 98.51514891278741004, -45.00612994150532842, 191.9384824187679612 ) ) ;
#50314=DIRECTION ( 'NONE',  ( 0.000000000000000000, 0.000000000000000000, -1.000000000000000000 ) ) ;
#50315=CARTESIAN_POINT ( 'NONE',  ( 109.3416101119966442, -26.53331765884353644, 220.9013395616249795 ) ) ;
#50316=CARTESIAN_POINT ( 'NONE',  ( 97.22547384517952196, -31.59602418489684084, 86.93181575210095957 ) ) ;
#50319=LINE ( 'NONE', #72127, #25663 ) ;
#50320=EDGE_CURVE ( 'NONE', #28372, #59253, #86589, .T. ) ;
#50321=DIRECTION ( 'NONE',  ( -1.000000000000000078E-15, 0.000000000000000000, 1.000000000000000000 ) ) ;
#50322=ORIENTED_EDGE ( 'NONE', *, *, #8102, .T. ) ;
#50327=ORIENTED_EDGE ( 'NONE', *, *, #55049, .T. ) ;
#50328=ORIENTED_EDGE ( 'NONE', *, *, #8287, .F. ) ;
#50329=CARTESIAN_POINT ( 'NONE',  ( 183.6524903400786286, -49.32844715993451956, 129.9678068554150059 ) ) ;
#50330=CARTESIAN_POINT ( 'NONE',  ( 107.2492351517315683, -24.88034519751278850, 226.0641967044829812 ) ) ;
#50331=CARTESIAN_POINT ( 'NONE',  ( 151.5667039024483245, -48.82844715993591223, 300.4678068554149490 ) ) ;
#50332=CARTESIAN_POINT ( 'NONE',  ( 136.6805397534846236, -17.85322261660804699, 2.908039740961557929 ) ) ;
#50335=DIRECTION ( 'NONE',  ( -1.000000000000000000, -3.999999999999999995E-14, -1.000000000000000078E-15 ) ) ;
#50336=CARTESIAN_POINT ( 'NONE',  ( 191.6375511031384633, -78.44951497180814215, 361.9756252759109998 ) ) ;
#50340=CARTESIAN_POINT ( 'NONE',  ( 96.66386919200992622, -42.45828961175909200, 26.72705384733997747 ) ) ;
#50341=ORIENTED_EDGE ( 'NONE', *, *, #9178, .F. ) ;
#50343=ORIENTED_EDGE ( 'NONE', *, *, #42587, .T. ) ;
#50344=VECTOR ( 'NONE', #35966, 1000.000000000000000 ) ;
#50345=DIRECTION ( 'NONE',  ( -1.000000000000000078E-15, 1.000000000000000083E-30, 1.000000000000000000 ) ) ;
#50347=CARTESIAN_POINT ( 'NONE',  ( 115.1619974903459251, -42.21817061296636808, 269.3527681330531891 ) ) ;
#50348=CARTESIAN_POINT ( 'NONE',  ( 107.0664832912739968, -36.72944715994100306, 287.6356252759109680 ) ) ;
#50349=CARTESIAN_POINT ( 'NONE',  ( 105.0928733274061813, -25.78792777683075599, 121.2184824187669818 ) ) ;
#50350=LINE ( 'NONE', #84464, #70698 ) ;
#50351=ORIENTED_EDGE ( 'NONE', *, *, #37362, .F. ) ;
#50352=CARTESIAN_POINT ( 'NONE',  ( 63.03715912545643363, -24.42818131006026761, 129.9678068554150911 ) ) ;
#50353=CARTESIAN_POINT ( 'NONE',  ( 77.45963244950118565, -35.85248396559181572, 2.902015641458088879 ) ) ;
#50354=ORIENTED_EDGE ( 'NONE', *, *, #66094, .T. ) ;
#50356=CARTESIAN_POINT ( 'NONE',  ( 102.6173380888347282, -29.88584920324980487, 23.35380465530695204 ) ) ;
#50357=VECTOR ( 'NONE', #70680, 1000.000000000000000 ) ;
#50359=DIRECTION ( 'NONE',  ( 1.000000000000000000, 1.261617073437676668E-15, 9.462128050782575008E-16 ) ) ;
#50360=CARTESIAN_POINT ( 'NONE',  ( 143.0664832912740110, -18.82844715994099971, 17.92562527591199739 ) ) ;
#50361=DIRECTION ( 'NONE',  ( -0.000000000000000000, -0.000000000000000000, -1.000000000000000000 ) ) ;
#50366=CARTESIAN_POINT ( 'NONE',  ( 114.5675797908445475, -44.02050044317889643, 98.21276813305395592 ) ) ;
#50368=CARTESIAN_POINT ( 'NONE',  ( 115.9627085491522536, -40.61889491704908295, 57.92099125664801562 ) ) ;
#50370=CARTESIAN_POINT ( 'NONE',  ( 98.25516505653058630, -40.97492784622586015, 171.6841967044829573 ) ) ;
#50371=LINE ( 'NONE', #86703, #23060 ) ;
#50372=LINE ( 'NONE', #52143, #51657 ) ;
#50373=DIRECTION ( 'NONE',  ( 0.000000000000000000, 0.000000000000000000, -1.000000000000000000 ) ) ;
#50377=CARTESIAN_POINT ( 'NONE',  ( 117.4730440113279855, -35.59081861377887179, 274.9127681330539872 ) ) ;
#50380=ORIENTED_EDGE ( 'NONE', *, *, #3731, .F. ) ;
#50381=CARTESIAN_POINT ( 'NONE',  ( 102.0609898346451274, -27.53498505803861107, 141.4727681330539895 ) ) ;
#50386=ORIENTED_EDGE ( 'NONE', *, *, #1095, .T. ) ;
#50388=EDGE_CURVE ( 'NONE', #22617, #39335, #62860, .T. ) ;
#50389=VERTEX_POINT ( 'NONE', #48679 ) ;
#50391=EDGE_CURVE ( 'NONE', #31265, #30966, #76411, .T. ) ;
#50392=CYLINDRICAL_SURFACE ( 'NONE', #66589, 2.117000000000007987 ) ;
#50394=DIRECTION ( 'NONE',  ( -0.4214249218767882055, -0.9068632946707806397, -4.214249218767890910E-16 ) ) ;
#50396=CARTESIAN_POINT ( 'NONE',  ( 96.71473009235836571, -37.96382682441392831, 37.42133956162496844 ) ) ;
#50397=CARTESIAN_POINT ( 'NONE',  ( 188.5667039024479834, -62.87844715994099687, 137.2178068554150059 ) ) ;
#50398=ORIENTED_EDGE ( 'NONE', *, *, #77998, .F. ) ;
#50399=CIRCLE ( 'NONE', #79416, 0.4999999999999933387 ) ;
#50401=ADVANCED_FACE ( 'NONE', ( #69604 ), #24137, .T. ) ;
#50408=CARTESIAN_POINT ( 'NONE',  ( 82.62351725430393401, -19.74149216370279802, 2.839569540204898601 ) ) ;
#50412=CARTESIAN_POINT ( 'NONE',  ( 107.0664832912739968, -36.72944715994100306, 287.6356252759109680 ) ) ;
#50413=EDGE_CURVE ( 'NONE', #19054, #15026, #87806, .T. ) ;
#50414=CARTESIAN_POINT ( 'NONE',  ( 101.9513324583280962, -44.20259256747556975, 241.5333722090289825 ) ) ;
#50416=CARTESIAN_POINT ( 'NONE',  ( 96.73636544059199593, -37.96124694896865748, 37.42133956162496844 ) ) ;
#50418=CARTESIAN_POINT ( 'NONE',  ( 98.11178232766683038, -43.28888419983005775, 106.8175300378159704 ) ) ;
#50420=CARTESIAN_POINT ( 'NONE',  ( 165.6738106836042732, -28.98061976758451053, 313.9678068554149490 ) ) ;
#50421=ORIENTED_EDGE ( 'NONE', *, *, #59757, .T. ) ;
#50422=CARTESIAN_POINT ( 'NONE',  ( 97.31584373184972492, -39.30597606054212179, 67.53145861423732299 ) ) ;
#50424=VERTEX_POINT ( 'NONE', #10060 ) ;
#50425=ADVANCED_FACE ( 'NONE', ( #30058 ), #36869, .F. ) ;
#50426=DIRECTION ( 'NONE',  ( 1.000000000000000078E-15, -1.000000000000000083E-30, -1.000000000000000000 ) ) ;
#50428=LINE ( 'NONE', #56792, #72634 ) ;
#50429=DIRECTION ( 'NONE',  ( 4.299999999999999979E-14, -1.000000000000000000, 4.400000000000000367E-29 ) ) ;
#50430=CIRCLE ( 'NONE', #59171, 0.5000000000000004441 ) ;
#50431=CARTESIAN_POINT ( 'NONE',  ( 142.8832909413445122, -79.11588146349311046, 394.9756252759100903 ) ) ;
#50432=EDGE_LOOP ( 'NONE', ( #7759, #52986, #69503, #87887 ) ) ;
#50433=CARTESIAN_POINT ( 'NONE',  ( 109.7758433794879664, -47.46978277150036263, 92.78514908543495210 ) ) ;
#50435=DIRECTION ( 'NONE',  ( 1.000000000000000000, 0.000000000000000000, 0.000000000000000000 ) ) ;
#50436=FACE_OUTER_BOUND ( 'NONE', #55875, .T. ) ;
#50438=ORIENTED_EDGE ( 'NONE', *, *, #38684, .T. ) ;
#50439=CARTESIAN_POINT ( 'NONE',  ( 19.56670390244796920, -67.87844715994100397, 300.9178068554150514 ) ) ;
#50441=CARTESIAN_POINT ( 'NONE',  ( 118.5256205435843526, -36.72944715994100306, 312.6356252759112522 ) ) ;
#50442=VECTOR ( 'NONE', #56650, 1000.000000000000000 ) ;
#50443=CARTESIAN_POINT ( 'NONE',  ( 167.6524903400753885, -49.32844715993521589, 249.9678068554149775 ) ) ;
#50445=ADVANCED_FACE ( 'NONE', ( #24578 ), #65020, .F. ) ;
#50446=CARTESIAN_POINT ( 'NONE',  ( 116.3212776292278363, -32.94146857470881429, 179.1356252759109395 ) ) ;
#50447=AXIS2_PLACEMENT_3D ( 'NONE', #64978, #31787, #86322 ) ;
#50448=ORIENTED_EDGE ( 'NONE', *, *, #51439, .F. ) ;
#50449=VECTOR ( 'NONE', #79197, 1000.000000000000000 ) ;
#50451=CARTESIAN_POINT ( 'NONE',  ( 98.80555182512732415, -41.96590078842027793, 182.7756252759109543 ) ) ;
#50452=CARTESIAN_POINT ( 'NONE',  ( 107.0664832912750057, -36.72944715993903486, 3.024967495036150922 ) ) ;
#50453=ORIENTED_EDGE ( 'NONE', *, *, #70576, .T. ) ;
#50454=VECTOR ( 'NONE', #73941, 1000.000000000000000 ) ;
#50455=CARTESIAN_POINT ( 'NONE',  ( 117.4970320020026406, -36.54623693216563396, 284.8413395616252615 ) ) ;
#50457=CARTESIAN_POINT ( 'NONE',  ( 134.0664832912739826, -18.72944715994100306, -5.074374724089001809 ) ) ;
#50459=CARTESIAN_POINT ( 'NONE',  ( 100.8868523152179364, -44.69971148260871274, 12.05236635724705252 ) ) ;
#50462=CIRCLE ( 'NONE', #18564, 0.5000000000000004441 ) ;
#50464=CARTESIAN_POINT ( 'NONE',  ( 106.8648936900573005, -47.09757847023110600, 227.5489586092449485 ) ) ;
#50466=EDGE_LOOP ( 'NONE', ( #48677, #84424 ) ) ;
#50467=CARTESIAN_POINT ( 'NONE',  ( 113.6520771548495503, -30.75516201018407614, 205.8444404487539714 ) ) ;
#50468=AXIS2_PLACEMENT_3D ( 'NONE', #26671, #74832, #13059 ) ;
#50469=EDGE_CURVE ( 'NONE', #16654, #61996, #8257, .T. ) ;
#50471=CARTESIAN_POINT ( 'NONE',  ( 101.4671292710339117, -29.18466352532158226, 32.02824997256392692 ) ) ;
#50474=VECTOR ( 'NONE', #29979, 1000.000000000000000 ) ;
#50475=CARTESIAN_POINT ( 'NONE',  ( 63.03715912545729338, -24.42818131006027826, 313.9678068554150059 ) ) ;
#50476=EDGE_LOOP ( 'NONE', ( #27398, #37872, #56772, #39667 ) ) ;
#50478=CARTESIAN_POINT ( 'NONE',  ( 97.80893753052176010, -40.51861053356429920, 37.63533870039827178 ) ) ;
#50479=CARTESIAN_POINT ( 'NONE',  ( 96.78489722101812731, -35.14273565208913652, 266.2041967044821149 ) ) ;
#50480=CARTESIAN_POINT ( 'NONE',  ( 92.55667057654251551, -29.98664840991042269, 0.7256252759109563799 ) ) ;
#50481=VERTEX_POINT ( 'NONE', #38204 ) ;
#50482=ORIENTED_EDGE ( 'NONE', *, *, #4088, .F. ) ;
#50483=CARTESIAN_POINT ( 'NONE',  ( 104.4081006417629851, -46.45808913496205861, 87.36479194099514700 ) ) ;
#50484=CARTESIAN_POINT ( 'NONE',  ( 172.5664832912729878, -18.82844715994071194, 135.9256252759120684 ) ) ;
#50485=CARTESIAN_POINT ( 'NONE',  ( 51.34673845256598668, -29.62846900982231446, -5.074374724088000832 ) ) ;
#50488=VECTOR ( 'NONE', #58285, 1000.000000000000000 ) ;
#50489=CARTESIAN_POINT ( 'NONE',  ( 97.72045521349410535, -39.61305637792672485, 17.56419670448195092 ) ) ;
#50492=CARTESIAN_POINT ( 'NONE',  ( 117.3094150574360128, -38.89169797369248727, 59.66133956162595098 ) ) ;
#50494=CARTESIAN_POINT ( 'NONE',  ( 115.0549195170180639, -30.03079676387787345, 269.3813395616251682 ) ) ;
#50496=ADVANCED_FACE ( 'NONE', ( #73614 ), #65900, .T. ) ;
#50498=ADVANCED_FACE ( 'NONE', ( #81790, #59963, #88606, #74512, #5480, #40873, #46781 ), #67697, .T. ) ;
#50503=CARTESIAN_POINT ( 'NONE',  ( 99.36125835269150741, -32.78858003560463175, 93.78047132197198721 ) ) ;
#50504=CARTESIAN_POINT ( 'NONE',  ( 107.5668116379858787, -47.79447663526521239, 188.6003871806729535 ) ) ;
#50506=ORIENTED_EDGE ( 'NONE', *, *, #87734, .F. ) ;
#50508=LINE ( 'NONE', #57315, #63977 ) ;
#50511=AXIS2_PLACEMENT_3D ( 'NONE', #37390, #85116, #50560 ) ;
#50513=AXIS2_PLACEMENT_3D ( 'NONE', #45828, #25408, #48073 ) ;
#50514=CARTESIAN_POINT ( 'NONE',  ( 75.31670390244798341, -50.82844715994100682, 84.20080685541500998 ) ) ;
#50515=ORIENTED_EDGE ( 'NONE', *, *, #41004, .T. ) ;
#50517=CARTESIAN_POINT ( 'NONE',  ( 37.03715912545342093, -48.62818131006128652, 193.9678068554150911 ) ) ;
#50518=CARTESIAN_POINT ( 'NONE',  ( 116.3216976867776964, -32.94060878512167534, 40.13562527591096796 ) ) ;
#50520=CARTESIAN_POINT ( 'NONE',  ( 99.32441224009949110, -32.03125536261004669, 125.3028960185529570 ) ) ;
#50521=CARTESIAN_POINT ( 'NONE',  ( 115.7136949400716333, -42.59221908682786761, 273.3527681330537575 ) ) ;
#50523=EDGE_LOOP ( 'NONE', ( #74109, #18320, #19007, #51183 ) ) ;
#50524=AXIS2_PLACEMENT_3D ( 'NONE', #82452, #12499, #12048 ) ;
#50526=DIRECTION ( 'NONE',  ( 0.000000000000000000, 0.000000000000000000, 1.000000000000000000 ) ) ;
#50527=VECTOR ( 'NONE', #70328, 1000.000000000000000 ) ;
#50528=CARTESIAN_POINT ( 'NONE',  ( 29.77381068363477112, -48.62134037875501491, 300.4678068554150059 ) ) ;
#50529=LINE ( 'NONE', #35555, #45513 ) ;
#50530=CARTESIAN_POINT ( 'NONE',  ( 101.6553708923145649, -27.03755641387271069, 105.4937205140069665 ) ) ;
#50531=DIRECTION ( 'NONE',  ( 1.000000000000000000, 4.163336342344333240E-14, 0.000000000000000000 ) ) ;
#50533=CARTESIAN_POINT ( 'NONE',  ( 117.4299418851264818, -35.59553461117717887, 278.9127681330539872 ) ) ;
#50534=LINE ( 'NONE', #71457, #87770 ) ;
#50536=LINE ( 'NONE', #9222, #50291 ) ;
#50537=CARTESIAN_POINT ( 'NONE',  ( 134.0664832912740110, -8.729447159940999512, 7.443125275912000127 ) ) ;
#50538=CARTESIAN_POINT ( 'NONE',  ( 179.8608231853560255, -35.55794170701751256, -5.074374724088000832 ) ) ;
#50539=CARTESIAN_POINT ( 'NONE',  ( 88.17226027475679473, -58.72944715994100306, 239.5838068554174924 ) ) ;
#50541=CARTESIAN_POINT ( 'NONE',  ( 131.3165200636274790, -36.90534128960221238, 6.749824347015201731 ) ) ;
#50542=AXIS2_PLACEMENT_3D ( 'NONE', #1832, #16349, #77682 ) ;
#50543=CARTESIAN_POINT ( 'NONE',  ( 180.1667039024460166, -28.27351298637340093, -5.074374724088000832 ) ) ;
#50544=CARTESIAN_POINT ( 'NONE',  ( 41.56648329127398966, -27.82844715994070484, 258.9256252759120116 ) ) ;
#50546=LINE ( 'NONE', #64631, #64622 ) ;
#50547=VERTEX_POINT ( 'NONE', #89039 ) ;
#50548=CARTESIAN_POINT ( 'NONE',  ( 116.3168070826688876, -32.94156582961523583, 135.1356252759109680 ) ) ;
#50549=CARTESIAN_POINT ( 'NONE',  ( 100.5702229155400858, -28.47427015469623868, 15.60705384733995871 ) ) ;
#50550=CARTESIAN_POINT ( 'NONE',  ( 108.9451852418780362, -26.43907245703257303, 160.9327681330539690 ) ) ;
#50551=CARTESIAN_POINT ( 'NONE',  ( 116.4941038412854510, -32.22865339830268283, 15.18133956162492915 ) ) ;
#50552=AXIS2_PLACEMENT_3D ( 'NONE', #6365, #89042, #82248 ) ;
#50554=CARTESIAN_POINT ( 'NONE',  ( 82.59705637153234647, -35.65296049054536098, 7.043700149390168974 ) ) ;
#50555=EDGE_CURVE ( 'NONE', #85489, #22788, #39086, .T. ) ;
#50557=AXIS2_PLACEMENT_3D ( 'NONE', #30695, #23460, #72038 ) ;
#50559=VERTEX_POINT ( 'NONE', #11392 ) ;
#50560=DIRECTION ( 'NONE',  ( 0.000000000000000000, 0.000000000000000000, -1.000000000000000000 ) ) ;
#50561=ORIENTED_EDGE ( 'NONE', *, *, #6340, .T. ) ;
#50562=CARTESIAN_POINT ( 'NONE',  ( 116.0809032858470999, -32.84949784884748425, 75.14991099019596277 ) ) ;
#50565=CARTESIAN_POINT ( 'NONE',  ( 100.8873290257058954, -44.70010636051070918, 48.05227766291039160 ) ) ;
#50566=CARTESIAN_POINT ( 'NONE',  ( 116.7748712849171255, -40.56502120445009751, 189.5270538473389479 ) ) ;
#50568=CARTESIAN_POINT ( 'NONE',  ( 110.8561050889767472, -45.98356882364006282, 147.8857656880664422 ) ) ;
#50570=CARTESIAN_POINT ( 'NONE',  ( 105.8095979597606373, -26.72298644015105396, 86.17751431161180165 ) ) ;
#50573=CARTESIAN_POINT ( 'NONE',  ( 110.8524082669982391, -45.98508177266331387, 97.88544780039453030 ) ) ;
#50574=CARTESIAN_POINT ( 'NONE',  ( 105.4244293397738659, -47.72525222749325735, 147.4584824187689662 ) ) ;
#50575=ORIENTED_EDGE ( 'NONE', *, *, #20968, .F. ) ;
#50576=ORIENTED_EDGE ( 'NONE', *, *, #89391, .T. ) ;
#50577=VECTOR ( 'NONE', #1875, 1000.000000000000000 ) ;
#50578=CARTESIAN_POINT ( 'NONE',  ( 97.82387236378413320, -38.41783952554947490, 47.91396425827898753 ) ) ;
#50579=EDGE_CURVE ( 'NONE', #18807, #50606, #77902, .T. ) ;
#50580=LINE ( 'NONE', #10586, #37057 ) ;
#50581=CARTESIAN_POINT ( 'NONE',  ( 101.1405520526760284, -45.23956608920054379, 233.0803871806719769 ) ) ;
#50582=LINE ( 'NONE', #31035, #17217 ) ;
#50583=CARTESIAN_POINT ( 'NONE',  ( 31.90335556477799628, -33.89581943344391135, 342.9256252759119548 ) ) ;
#50584=CARTESIAN_POINT ( 'NONE',  ( 97.31584962811177775, -39.30599893963958635, 112.5320257889539306 ) ) ;
#50585=CARTESIAN_POINT ( 'NONE',  ( 112.8677825012601375, -28.59025478454122648, 249.5838084826162913 ) ) ;
#50586=VECTOR ( 'NONE', #24036, 1000.000000000000000 ) ;
#50587=LINE ( 'NONE', #45102, #60895 ) ;
#50589=CARTESIAN_POINT ( 'NONE',  ( 108.0049669398584911, -26.36739623290726442, 155.0041967044819557 ) ) ;
#50593=AXIS2_PLACEMENT_3D ( 'NONE', #74164, #32357, #40974 ) ;
#50594=ORIENTED_CLOSED_SHELL ( 'NONE', *, #73489, .F. );
#50597=AXIS2_PLACEMENT_3D ( 'NONE', #51201, #24856, #32545 ) ;
#50598=CARTESIAN_POINT ( 'NONE',  ( 152.0368932755772562, -23.42844715993588878, 117.4678068554150485 ) ) ;
#50599=CARTESIAN_POINT ( 'NONE',  ( 117.0719072149801434, -35.46254345245687745, 104.9272870867127665 ) ) ;
#50600=CARTESIAN_POINT ( 'NONE',  ( 114.4736784013144586, -40.22460793573437599, 226.2938046553059621 ) ) ;
#50601=CARTESIAN_POINT ( 'NONE',  ( 98.30752301746520061, -41.72885616756393290, 267.7397901826493580 ) ) ;
#50602=CARTESIAN_POINT ( 'NONE',  ( 99.10121394234140269, -45.50393173043428163, 156.9899109901969609 ) ) ;
#50604=ORIENTED_EDGE ( 'NONE', *, *, #49924, .T. ) ;
#50605=ADVANCED_FACE ( 'NONE', ( #34053, #89492 ), #5025, .F. ) ;
#50606=VERTEX_POINT ( 'NONE', #11844 ) ;
#50608=AXIS2_PLACEMENT_3D ( 'NONE', #31637, #59779, #44368 ) ;
#50611=ORIENTED_EDGE ( 'NONE', *, *, #16381, .F. ) ;
#50613=DIRECTION ( 'NONE',  ( 0.7071067811865431318, -0.7071067811865517916, 7.071067811865425043E-16 ) ) ;
#50614=CARTESIAN_POINT ( 'NONE',  ( 97.00631399252166887, -37.24296311215223909, 267.7987261630397029 ) ) ;
#50618=CARTESIAN_POINT ( 'NONE',  ( 114.3732006581859650, -41.89629318141880532, 9.635625275910941312 ) ) ;
#50619=CIRCLE ( 'NONE', #7059, 12.99999999999999822 ) ;
#50620=CARTESIAN_POINT ( 'NONE',  ( 93.94797395270801132, -35.60435878782501362, 247.7440089327910755 ) ) ;
#50621=VERTEX_POINT ( 'NONE', #20001 ) ;
#50622=ORIENTED_EDGE ( 'NONE', *, *, #45905, .T. ) ;
#50623=CARTESIAN_POINT ( 'NONE',  ( 104.4081753580950505, -46.45811105792077456, 112.3648722168799736 ) ) ;
#50624=ORIENTED_EDGE ( 'NONE', *, *, #22455, .T. ) ;
#50627=CARTESIAN_POINT ( 'NONE',  ( 109.9248237270229680, -44.80917438794489271, 37.26956268521996662 ) ) ;
#50628=CARTESIAN_POINT ( 'NONE',  ( 116.8272927809998123, -43.49410631979629471, 163.3441967044829823 ) ) ;
#50629=CARTESIAN_POINT ( 'NONE',  ( 109.1969564574039282, -26.54663071456422330, 139.9127681330539872 ) ) ;
#50630=EDGE_CURVE ( 'NONE', #84435, #14978, #18202, .T. ) ;
#50632=CARTESIAN_POINT ( 'NONE',  ( 110.2558863881303779, -26.76706588525435748, 230.8299109901969643 ) ) ;
#50633=DIRECTION ( 'NONE',  ( 1.000000000000000078E-15, -1.000000000000000083E-30, -1.000000000000000000 ) ) ;
#50637=ORIENTED_EDGE ( 'NONE', *, *, #12982, .T. ) ;
#50639=ORIENTED_EDGE ( 'NONE', *, *, #82740, .T. ) ;
#50640=AXIS2_PLACEMENT_3D ( 'NONE', #13944, #42970, #83437 ) ;
#50641=AXIS2_PLACEMENT_3D ( 'NONE', #27258, #89043, #69945 ) ;
#50642=CARTESIAN_POINT ( 'NONE',  ( 107.6569944592711607, -47.81385874506208467, 197.6308633711489620 ) ) ;
#50643=EDGE_LOOP ( 'NONE', ( #85046, #6751, #26662, #11282 ) ) ;
#50644=CARTESIAN_POINT ( 'NONE',  ( 117.4265927121613089, -30.97543824232759135, 179.2299109901959753 ) ) ;
#50645=CARTESIAN_POINT ( 'NONE',  ( 194.5667039024479834, -67.87844715994100397, 10.91780685541479734 ) ) ;
#50646=CARTESIAN_POINT ( 'NONE',  ( 135.6382054840678109, -34.47341874818869201, 7.827313014938068747 ) ) ;
#50647=DIRECTION ( 'NONE',  ( -1.000000000000000000, -4.554376769437570034E-14, 0.000000000000000000 ) ) ;
#50649=CARTESIAN_POINT ( 'NONE',  ( 100.7545310429336354, -44.50279142785353770, 57.03342830892890447 ) ) ;
#50650=CARTESIAN_POINT ( 'NONE',  ( 105.6350724880777534, -47.03380199863519806, 253.4670538473393719 ) ) ;
#50651=CARTESIAN_POINT ( 'NONE',  ( 194.5667039024479834, -67.87844715994100397, 10.91780685541479734 ) ) ;
#50653=CARTESIAN_POINT ( 'NONE',  ( 97.33757460489857749, -34.07214903665069272, 272.1144460458409071 ) ) ;
#50655=LINE ( 'NONE', #62940, #15250 ) ;
#50656=AXIS2_PLACEMENT_3D ( 'NONE', #89656, #19265, #5642 ) ;
#50657=CARTESIAN_POINT ( 'NONE',  ( 64.67079002020506096, -0.9301828534102468682, 361.9756252759101471 ) ) ;
#50658=CYLINDRICAL_SURFACE ( 'NONE', #79674, 0.2500000000000039968 ) ;
#50659=CARTESIAN_POINT ( 'NONE',  ( 99.16241280097113986, -32.69931702961348208, 195.5838068554172651 ) ) ;
#50660=ORIENTED_EDGE ( 'NONE', *, *, #67706, .F. ) ;
#50662=CARTESIAN_POINT ( 'NONE',  ( 114.9818473740405835, -29.91084206771912690, 184.3927681330539770 ) ) ;
#50663=CARTESIAN_POINT ( 'NONE',  ( 95.34914990350537778, -34.95780559393485731, 67.20705384733894050 ) ) ;
#50664=CARTESIAN_POINT ( 'NONE',  ( 98.22454660805831850, -42.33418938753942484, 182.7756252759109543 ) ) ;
#50665=DIRECTION ( 'NONE',  ( 1.000000000000000000, 0.000000000000000000, 0.000000000000000000 ) ) ;
#50667=DIRECTION ( 'NONE',  ( 0.000000000000000000, -1.000000000000000000, 0.000000000000000000 ) ) ;
#50669=DIRECTION ( 'NONE',  ( -1.000000000000000078E-15, 1.000000000000000083E-30, 1.000000000000000000 ) ) ;
#50670=CARTESIAN_POINT ( 'NONE',  ( 133.5842039024480812, -58.72944715994091780, 231.5838068554170093 ) ) ;
#50672=ORIENTED_EDGE ( 'NONE', *, *, #33575, .T. ) ;
#50673=LINE ( 'NONE', #72029, #61639 ) ;
#50679=CARTESIAN_POINT ( 'NONE',  ( 101.0184087763112757, -44.32493413285080663, 121.4638483995059630 ) ) ;
#50680=DIRECTION ( 'NONE',  ( -2.900000000000000265E-14, 2.000000000000000155E-15, -1.000000000000000000 ) ) ;
#50682=CARTESIAN_POINT ( 'NONE',  ( 117.8527506973082524, -39.03601561205230297, 104.6708633711489824 ) ) ;
#50683=DIRECTION ( 'NONE',  ( -1.000000000000000000, -2.756263715554006823E-15, 0.000000000000000000 ) ) ;
#50684=LINE ( 'NONE', #748, #71743 ) ;
#50685=DIRECTION ( 'NONE',  ( 2.900000000000000265E-14, -2.000000000000000155E-15, 1.000000000000000000 ) ) ;
#50686=CARTESIAN_POINT ( 'NONE',  ( 100.8863495415024119, -28.40209871822978371, 35.59657765686397113 ) ) ;
#50687=ORIENTED_EDGE ( 'NONE', *, *, #86903, .T. ) ;
#50688=AXIS2_PLACEMENT_3D ( 'NONE', #34274, #61976, #89714 ) ;
#50689=ORIENTED_EDGE ( 'NONE', *, *, #13082, .T. ) ;
#50690=VERTEX_POINT ( 'NONE', #83136 ) ;
#50691=ADVANCED_FACE ( 'NONE', ( #20894 ), #898, .F. ) ;
#50693=DIRECTION ( 'NONE',  ( 0.7071067811864886199, 0.7071067811866064146, 7.071067811864879743E-16 ) ) ;
#50694=CARTESIAN_POINT ( 'NONE',  ( 97.31584371326931659, -39.30597598860000375, 117.5314586083788555 ) ) ;
#50696=DIRECTION ( 'NONE',  ( 1.000000000000000078E-15, -1.000000000000000083E-30, -1.000000000000000000 ) ) ;
#50697=CARTESIAN_POINT ( 'NONE',  ( 97.75827217529801771, -40.38459891742106578, 52.62384772014601708 ) ) ;
#50701=CARTESIAN_POINT ( 'NONE',  ( 99.99555918775621421, -44.36035129061385618, 46.98133956162592284 ) ) ;
#50702=EDGE_CURVE ( 'NONE', #29891, #28724, #70848, .T. ) ;
#50703=ORIENTED_EDGE ( 'NONE', *, *, #16190, .F. ) ;
#50705=EDGE_CURVE ( 'NONE', #66869, #52443, #36316, .T. ) ;
#50706=DIRECTION ( 'NONE',  ( -0.000000000000000000, -0.000000000000000000, -1.000000000000000000 ) ) ;
#50708=CARTESIAN_POINT ( 'NONE',  ( 113.0638415271824897, -42.26672268200739069, 121.0509475124479906 ) ) ;
#50710=VECTOR ( 'NONE', #52797, 1000.000000000000000 ) ;
#50712=CYLINDRICAL_SURFACE ( 'NONE', #36912, 2.116999999999980009 ) ;
#50713=DIRECTION ( 'NONE',  ( 1.000000000000000000, 8.673617379883546378E-16, 9.757819552368989676E-16 ) ) ;
#50714=EDGE_LOOP ( 'NONE', ( #1406, #6595, #43440, #73596 ) ) ;
#50715=VERTEX_POINT ( 'NONE', #41759 ) ;
#50716=VECTOR ( 'NONE', #77440, 1000.000000000000000 ) ;
#50719=VERTEX_POINT ( 'NONE', #14980 ) ;
#50721=EDGE_CURVE ( 'NONE', #29906, #58630, #19921, .T. ) ;
#50722=CARTESIAN_POINT ( 'NONE',  ( 100.4550560919867479, -30.82882778563945791, 187.1787261630399541 ) ) ;
#50723=DIRECTION ( 'NONE',  ( 0.000000000000000000, 0.000000000000000000, 1.000000000000000000 ) ) ;
#50724=AXIS2_PLACEMENT_3D ( 'NONE', #15454, #56301, #35420 ) ;
#50725=CARTESIAN_POINT ( 'NONE',  ( 96.06465719955961902, -38.01203376208108153, 82.43086337114895912 ) ) ;
#50727=CARTESIAN_POINT ( 'NONE',  ( 110.8538278642257779, -45.98450097318836782, 17.88556988677979476 ) ) ;
#50728=ORIENTED_EDGE ( 'NONE', *, *, #57603, .T. ) ;
#50731=CIRCLE ( 'NONE', #52131, 27.99999999999999645 ) ;
#50733=CARTESIAN_POINT ( 'NONE',  ( 98.88612577743202792, -36.32393613343754879, 169.1052332267339580 ) ) ;
#50734=CARTESIAN_POINT ( 'NONE',  ( 117.4766623710874853, -37.96092365070988706, 53.73276813305394484 ) ) ;
#50735=ORIENTED_EDGE ( 'NONE', *, *, #47795, .T. ) ;
#50736=CARTESIAN_POINT ( 'NONE',  ( 111.4063510358307667, -46.18429848020807782, 27.91848241876792969 ) ) ;
#50737=CARTESIAN_POINT ( 'NONE',  ( 117.4353638176713446, -35.45525114565609215, 189.9241967044829664 ) ) ;
#50739=LINE ( 'NONE', #23510, #26313 ) ;
#50741=CARTESIAN_POINT ( 'NONE',  ( 114.7074080197622976, -44.71632701241580321, 109.1718157521009687 ) ) ;
#50742=DIRECTION ( 'NONE',  ( -0.7071067811865753283, 0.7071067811865197061, -7.071067811865760309E-16 ) ) ;
#50746=EDGE_CURVE ( 'NONE', #62066, #19234, #39051, .T. ) ;
#50748=CARTESIAN_POINT ( 'NONE',  ( 116.3168070826688876, -32.94156582961523583, 135.1356252759109680 ) ) ;
#50749=ORIENTED_EDGE ( 'NONE', *, *, #86112, .F. ) ;
#50750=CIRCLE ( 'NONE', #76825, 0.9999999999999731326 ) ;
#50751=ORIENTED_EDGE ( 'NONE', *, *, #41167, .F. ) ;
#50752=B_SPLINE_CURVE_WITH_KNOTS ( 'NONE', 3,
 ( #32716, #80002, #54476, #69037, #28130, #75410, #14068, #27247, #13621, #7703, #47676, #14975, #76297, #438, #54923, #13184, #6801, #55821 ),
 .UNSPECIFIED., .F., .F.,
 ( 4, 2, 2, 2, 2, 2, 2, 2, 4 ),
 ( 0.000000000000000000, 0.06249549862835345609, 0.1249909972567069122, 0.1874864958850603613, 0.2499819945134138244, 0.3124774931417672597, 0.3749729917701207227, 0.4374684903984741857, 0.4999639890268276488 ),
 .UNSPECIFIED. ) ;
#50753=DIRECTION ( 'NONE',  ( 0.000000000000000000, 0.000000000000000000, -1.000000000000000000 ) ) ;
#50754=( BOUNDED_CURVE ( )  B_SPLINE_CURVE ( 3, ( #82742, #75465, #35003, #13235 ),
 .UNSPECIFIED., .F., .T. ) 
 B_SPLINE_CURVE_WITH_KNOTS ( ( 4, 4 ),
 ( 4.712388980377630432, 6.283185307174195877 ),
 .UNSPECIFIED. ) 
 CURVE ( )  GEOMETRIC_REPRESENTATION_ITEM ( )  RATIONAL_B_SPLINE_CURVE ( ( 1.000000000000000000, 0.8047378541227010462, 0.8047378541227010462, 1.000000000000000000 ) ) 
 REPRESENTATION_ITEM ( '' )  );
#50756=CARTESIAN_POINT ( 'NONE',  ( 116.6749405801447921, -32.59381477748385691, 79.14991099019697174 ) ) ;
#50757=DIRECTION ( 'NONE',  ( 0.000000000000000000, 0.000000000000000000, 1.000000000000000000 ) ) ;
#50758=FACE_OUTER_BOUND ( 'NONE', #89489, .T. ) ;
#50760=CARTESIAN_POINT ( 'NONE',  ( 99.23822674327645643, -42.59304969680529496, 66.83848241876894747 ) ) ;
#50761=CARTESIAN_POINT ( 'NONE',  ( 97.07198648724674683, -35.37904510147855319, 111.2190064217568874 ) ) ;
#50762=CARTESIAN_POINT ( 'NONE',  ( 117.7567108552514128, -34.01230579303181401, 165.0365776568629315 ) ) ;
#50763=DIRECTION ( 'NONE',  ( 0.000000000000000000, 0.000000000000000000, 1.000000000000000000 ) ) ;
#50764=DIRECTION ( 'NONE',  ( 0.7071067812152160847, -0.7071067811578790607, 0.000000000000000000 ) ) ;
#50765=ORIENTED_EDGE ( 'NONE', *, *, #71061, .F. ) ;
#50766=FACE_OUTER_BOUND ( 'NONE', #69415, .T. ) ;
#50767=AXIS2_PLACEMENT_3D ( 'NONE', #81889, #82342, #40975 ) ;
#50769=ORIENTED_EDGE ( 'NONE', *, *, #24199, .T. ) ;
#50771=DIRECTION ( 'NONE',  ( -0.000000000000000000, -0.000000000000000000, -1.000000000000000000 ) ) ;
#50772=CARTESIAN_POINT ( 'NONE',  ( 103.7090067442367314, -26.14926592973559138, 205.3089586092439731 ) ) ;
#50774=DIRECTION ( 'NONE',  ( 2.999999999999999839E-15, -1.000000000000000000, 2.999999999999999900E-30 ) ) ;
#50775=CARTESIAN_POINT ( 'NONE',  ( 96.24544184373708333, -34.36507245719054282, 252.1432443235302969 ) ) ;
#50776=CARTESIAN_POINT ( 'NONE',  ( 96.03173718742787912, -37.92605769912402991, 77.40038718067299328 ) ) ;
#50777=CARTESIAN_POINT ( 'NONE',  ( 75.31670390244798341, -67.87844715994100397, 60.91780685541480267 ) ) ;
#50780=ORIENTED_EDGE ( 'NONE', *, *, #20381, .F. ) ;
#50781=VECTOR ( 'NONE', #41681, 1000.000000000000000 ) ;
#50782=ORIENTED_EDGE ( 'NONE', *, *, #13085, .F. ) ;
#50783=VERTEX_POINT ( 'NONE', #56744 ) ;
#50784=CIRCLE ( 'NONE', #82710, 0.5000000000000004441 ) ;
#50787=CARTESIAN_POINT ( 'NONE',  ( 96.53701874497966173, -40.09164955422465937, 277.5603871806729899 ) ) ;
#50788=CYLINDRICAL_SURFACE ( 'NONE', #73660, 4.750000000000004441 ) ;
#50789=DIRECTION ( 'NONE',  ( 1.907762142705490052E-15, 7.167082501179359715E-16, -1.000000000000000000 ) ) ;
#50790=AXIS2_PLACEMENT_3D ( 'NONE', #17703, #53521, #60354 ) ;
#50793=DIRECTION ( 'NONE',  ( 0.000000000000000000, 0.000000000000000000, -1.000000000000000000 ) ) ;
#50794=CARTESIAN_POINT ( 'NONE',  ( 102.4276729374712431, -43.93594010915269621, 221.5438483995059755 ) ) ;
#50799=FACE_OUTER_BOUND ( 'NONE', #66113, .T. ) ;
#50800=CARTESIAN_POINT ( 'NONE',  ( 100.8873721005049475, -44.70014299556108739, 182.0523503870009847 ) ) ;
#50801=EDGE_CURVE ( 'NONE', #41861, #35904, #22855, .T. ) ;
#50802=CARTESIAN_POINT ( 'NONE',  ( 99.18317230595245348, -39.95607890373031523, 8.067297591610955720 ) ) ;
#50804=FACE_OUTER_BOUND ( 'NONE', #81660, .T. ) ;
#50806=CARTESIAN_POINT ( 'NONE',  ( 97.28626111821324685, -36.62605694204433604, 107.3184824187669619 ) ) ;
#50810=DIRECTION ( 'NONE',  ( -4.299999999999999979E-14, 1.000000000000000000, -4.400000000000000367E-29 ) ) ;
#50812=FACE_OUTER_BOUND ( 'NONE', #43416, .T. ) ;
#50814=AXIS2_PLACEMENT_3D ( 'NONE', #66335, #39079, #81350 ) ;
#50815=CARTESIAN_POINT ( 'NONE',  ( 180.2121375201596152, -29.73316016638949577, 313.9678068554149490 ) ) ;
#50816=CARTESIAN_POINT ( 'NONE',  ( 113.9764273654521674, -32.38405892540742315, 32.09094751244895605 ) ) ;
#50817=EDGE_CURVE ( 'NONE', #40235, #40317, #78116, .T. ) ;
#50818=DIRECTION ( 'NONE',  ( -0.7071067811865671127, -0.7071067811865279218, -7.071067811865664660E-16 ) ) ;
#50819=EDGE_CURVE ( 'NONE', #53871, #13694, #41680, .T. ) ;
#50820=CARTESIAN_POINT ( 'NONE',  ( 188.5667039024483529, -48.82844715993431350, 293.2178068554150059 ) ) ;
#50821=CARTESIAN_POINT ( 'NONE',  ( 116.7950807104413684, -39.38798874826055396, 194.6147885282144614 ) ) ;
#50826=CARTESIAN_POINT ( 'NONE',  ( 107.8683683300076837, -26.33502505738635691, 70.01562527591099183 ) ) ;
#50827=ORIENTED_EDGE ( 'NONE', *, *, #42308, .T. ) ;
#50828=CARTESIAN_POINT ( 'NONE',  ( 98.88061221520823096, -34.29066745521690507, 30.51813411379100671 ) ) ;
#50829=ADVANCED_FACE ( 'NONE', ( #15879 ), #3138, .T. ) ;
#50830=AXIS2_PLACEMENT_3D ( 'NONE', #79625, #64636, #73224 ) ;
#50832=CARTESIAN_POINT ( 'NONE',  ( 104.4962338114797262, -45.76661171243296877, 63.79967854399193072 ) ) ;
#50835=CARTESIAN_POINT ( 'NONE',  ( 37.03715912545427358, -48.62818131006112310, 300.4678068554150059 ) ) ;
#50836=CARTESIAN_POINT ( 'NONE',  ( 115.0881438103696155, -30.00293675228997614, 265.3813395616251682 ) ) ;
#50840=LINE ( 'NONE', #65797, #66128 ) ;
#50842=CARTESIAN_POINT ( 'NONE',  ( 108.0108636065302932, -26.30228954677034992, 151.0041967044829505 ) ) ;
#50844=ORIENTED_EDGE ( 'NONE', *, *, #8272, .F. ) ;
#50845=ORIENTED_EDGE ( 'NONE', *, *, #42488, .T. ) ;
#50846=VERTEX_POINT ( 'NONE', #17218 ) ;
#50847=CARTESIAN_POINT ( 'NONE',  ( 117.0718954882821947, -35.46248237174801687, 123.9272919413459562 ) ) ;
#50848=CARTESIAN_POINT ( 'NONE',  ( 41.56670390244804025, -42.82844715994103524, 300.4678068554150059 ) ) ;
#50849=CARTESIAN_POINT ( 'NONE',  ( 101.7545977962314225, -44.98157700518534341, 222.1213395616259731 ) ) ;
#50850=DIRECTION ( 'NONE',  ( -0.9254794337955620787, -0.3787978585227822492, 0.000000000000000000 ) ) ;
#50851=DIRECTION ( 'NONE',  ( 1.000000000000000078E-15, 9.367723249499513438E-31, -1.000000000000000000 ) ) ;
#50853=CARTESIAN_POINT ( 'NONE',  ( 104.6489182489307552, -47.51505607846939938, 23.38895860924494841 ) ) ;
#50855=EDGE_CURVE ( 'NONE', #19111, #84744, #10829, .T. ) ;
#50856=VERTEX_POINT ( 'NONE', #43557 ) ;
#50857=CARTESIAN_POINT ( 'NONE',  ( 103.4067605119645776, -27.42305663254103010, 171.3746256237512569 ) ) ;
#50860=DIRECTION ( 'NONE',  ( 1.000000000000000000, -3.885780586188044357E-13, 0.000000000000000000 ) ) ;
#50861=ORIENTED_EDGE ( 'NONE', *, *, #52896, .F. ) ;
#50863=DIRECTION ( 'NONE',  ( 0.000000000000000000, 0.000000000000000000, -1.000000000000000000 ) ) ;
#50864=CARTESIAN_POINT ( 'NONE',  ( 103.7301789885933658, -26.21598454391059363, 205.3089586092439731 ) ) ;
#50866=FACE_BOUND ( 'NONE', #11149, .T. ) ;
#50868=CARTESIAN_POINT ( 'NONE',  ( 116.0578256703656308, -35.64850657512946697, 238.3562293518859576 ) ) ;
#50870=CARTESIAN_POINT ( 'NONE',  ( 110.7866772467784955, -46.44483816919306207, 58.86705384733998159 ) ) ;
#50872=CARTESIAN_POINT ( 'NONE',  ( 108.5441999379606983, -26.36493947475176114, 104.9641967044819779 ) ) ;
#50873=EDGE_LOOP ( 'NONE', ( #29960, #1206 ) ) ;
#50874=CARTESIAN_POINT ( 'NONE',  ( 131.6875538713323408, -20.11069332324015235, 7.213126773492521515 ) ) ;
#50875=ORIENTED_EDGE ( 'NONE', *, *, #26937, .T. ) ;
#50877=CARTESIAN_POINT ( 'NONE',  ( 134.0664832912739826, -21.47944715994100306, 1.625625275910997480 ) ) ;
#50878=CARTESIAN_POINT ( 'NONE',  ( 105.0465253178684719, -26.92297229278132775, 276.2381595649878818 ) ) ;
#50879=ORIENTED_EDGE ( 'NONE', *, *, #61906, .T. ) ;
#50880=DIRECTION ( 'NONE',  ( 1.000000000000000000, 4.299999999999999979E-14, 1.000000000000000078E-15 ) ) ;
#50883=CARTESIAN_POINT ( 'NONE',  ( 97.81168895331838087, -40.51742574516882200, 287.6356252759109680 ) ) ;
#50884=VECTOR ( 'NONE', #15201, 1000.000000000000000 ) ;
#50885=DIRECTION ( 'NONE',  ( 0.000000000000000000, 0.000000000000000000, 1.000000000000000000 ) ) ;
#50887=CARTESIAN_POINT ( 'NONE',  ( 101.6667450491003706, -27.05792876557581650, 105.4937205140069665 ) ) ;
#50888=( NAMED_UNIT ( * ) SI_UNIT ( $, .STERADIAN. ) SOLID_ANGLE_UNIT ( ) );
#50889=LINE ( 'NONE', #36382, #89891 ) ;
#50890=FACE_OUTER_BOUND ( 'NONE', #3977, .T. ) ;
#50892=ORIENTED_EDGE ( 'NONE', *, *, #35417, .T. ) ;
#50894=CARTESIAN_POINT ( 'NONE',  ( 73.06648329127401098, -46.72944715994106701, 14.67562527591093513 ) ) ;
#50895=DIRECTION ( 'NONE',  ( 0.000000000000000000, 0.000000000000000000, -1.000000000000000000 ) ) ;
#50896=VECTOR ( 'NONE', #86215, 1000.000000000000000 ) ;
#50898=DIRECTION ( 'NONE',  ( 0.000000000000000000, 1.000000000000000000, 0.000000000000000000 ) ) ;
#50899=CARTESIAN_POINT ( 'NONE',  ( 115.8254259877983827, -31.73000318220183047, 179.2397932879499649 ) ) ;
#50900=ORIENTED_EDGE ( 'NONE', *, *, #5793, .T. ) ;
#50902=DIRECTION ( 'NONE',  ( 0.000000000000000000, 0.000000000000000000, 1.000000000000000000 ) ) ;
#50904=CARTESIAN_POINT ( 'NONE',  ( 98.64540312569894809, -41.76920806142280185, 157.7556252759109725 ) ) ;
#50909=CARTESIAN_POINT ( 'NONE',  ( 116.1300133678978170, -31.69047823903422412, 25.24229194257693365 ) ) ;
#50910=CARTESIAN_POINT ( 'NONE',  ( 107.0667039024479834, -48.82844715994099971, 160.9178068554150229 ) ) ;
#50912=CARTESIAN_POINT ( 'NONE',  ( 112.0636370890131985, -45.48966441153708473, 12.99003379025321614 ) ) ;
#50915=DIRECTION ( 'NONE',  ( 1.000000000000000000, 4.163336342344333240E-14, 0.000000000000000000 ) ) ;
#50916=CARTESIAN_POINT ( 'NONE',  ( 116.3159835831962852, -41.41832011455028351, 248.4651490854349731 ) ) ;
#50917=ORIENTED_EDGE ( 'NONE', *, *, #35217, .T. ) ;
#50918=ORIENTED_EDGE ( 'NONE', *, *, #64811, .F. ) ;
#50919=CARTESIAN_POINT ( 'NONE',  ( 97.70553735687687436, -35.92370728225471055, 182.6777737820879679 ) ) ;
#50920=EDGE_CURVE ( 'NONE', #56383, #78468, #64006, .T. ) ;
#50922=CARTESIAN_POINT ( 'NONE',  ( 111.9552019894765493, -28.70592206014574543, 46.06063092494500211 ) ) ;
#50924=EDGE_CURVE ( 'NONE', #87762, #82436, #33514, .T. ) ;
#50925=CARTESIAN_POINT ( 'NONE',  ( 172.5667039024478129, -36.32844715993500273, 300.4678068554149490 ) ) ;
#50927=AXIS2_PLACEMENT_3D ( 'NONE', #55000, #60948, #82317 ) ;
#50929=DIRECTION ( 'NONE',  ( 3.999999999999999995E-14, -1.000000000000000000, 4.100000000000000342E-29 ) ) ;
#50930=CARTESIAN_POINT ( 'NONE',  ( 194.0667039024473297, -24.92844715993408045, 300.4678068554149490 ) ) ;
#50931=CARTESIAN_POINT ( 'NONE',  ( 100.8614382317054776, -45.12360235833661903, 257.0699109901967745 ) ) ;
#50932=LINE ( 'NONE', #24135, #76487 ) ;
#50933=EDGE_LOOP ( 'NONE', ( #34410, #86768, #33853, #13860, #36331 ) ) ;
#50934=ORIENTED_EDGE ( 'NONE', *, *, #16879, .T. ) ;
#50935=EDGE_CURVE ( 'NONE', #62791, #23038, #73958, .T. ) ;
#50936=DIRECTION ( 'NONE',  ( 1.000000000000000078E-15, -1.000000000000000083E-30, -1.000000000000000000 ) ) ;
#50937=CARTESIAN_POINT ( 'NONE',  ( 152.0371591254585155, -47.82818131005588214, 193.9678068554149775 ) ) ;
#50938=CARTESIAN_POINT ( 'NONE',  ( 73.06648329127396835, -8.729447159941065237, 14.67562527591093513 ) ) ;
#50939=FACE_BOUND ( 'NONE', #61657, .T. ) ;
#50940=VECTOR ( 'NONE', #79607, 1000.000000000000114 ) ;
#50941=CARTESIAN_POINT ( 'NONE',  ( 104.7983354005985888, -46.84845355258768507, 23.38895860924395009 ) ) ;
#50945=CARTESIAN_POINT ( 'NONE',  ( 117.9699911065184637, -41.49648292930365301, 54.49848241876792088 ) ) ;
#50946=LINE ( 'NONE', #17333, #88898 ) ;
#50947=CARTESIAN_POINT ( 'NONE',  ( 99.38138666193238180, -29.68485204926252763, 275.7356252759109907 ) ) ;
#50948=ORIENTED_EDGE ( 'NONE', *, *, #81938, .F. ) ;
#50949=CARTESIAN_POINT ( 'NONE',  ( 82.68053975348408358, -17.85322261661534426, 2.908039740960796316 ) ) ;
#50950=FACE_OUTER_BOUND ( 'NONE', #38431, .T. ) ;
#50951=DIRECTION ( 'NONE',  ( -1.000000000000000078E-15, 1.000000000000000083E-30, 1.000000000000000000 ) ) ;
#50952=CARTESIAN_POINT ( 'NONE',  ( 115.1210532203963766, -38.21490719095142197, 86.49951894101998562 ) ) ;
#50953=CARTESIAN_POINT ( 'NONE',  ( 117.2487272683742532, -41.08916198262414099, 209.5165776568640013 ) ) ;
#50955=DIRECTION ( 'NONE',  ( 0.000000000000000000, 0.000000000000000000, -1.000000000000000000 ) ) ;
#50956=ORIENTED_EDGE ( 'NONE', *, *, #57558, .F. ) ;
#50957=EDGE_CURVE ( 'NONE', #78504, #49604, #60489, .T. ) ;
#50958=FACE_OUTER_BOUND ( 'NONE', #71498, .T. ) ;
#50961=ORIENTED_EDGE ( 'NONE', *, *, #42183, .F. ) ;
#50962=DIRECTION ( 'NONE',  ( 0.000000000000000000, 0.000000000000000000, -1.000000000000000000 ) ) ;
#50963=ORIENTED_EDGE ( 'NONE', *, *, #63384, .T. ) ;
#50965=CARTESIAN_POINT ( 'NONE',  ( 193.0374249753377001, -23.42844715993431848, 129.9678068554150343 ) ) ;
#50966=CARTESIAN_POINT ( 'NONE',  ( 112.6855112425771210, -28.39944475707905625, 40.60397405478997968 ) ) ;
#50967=CARTESIAN_POINT ( 'NONE',  ( 100.3264543382982907, -29.74069638407027938, 115.1095626852199558 ) ) ;
#50969=CARTESIAN_POINT ( 'NONE',  ( 96.51457183773001702, -40.09881715592517537, 281.5603871806727625 ) ) ;
#50971=VECTOR ( 'NONE', #71124, 1000.000000000000000 ) ;
#50973=EDGE_CURVE ( 'NONE', #8752, #4393, #87590, .T. ) ;
#50974=CARTESIAN_POINT ( 'NONE',  ( 113.5732777703083229, -29.05103677887047198, 135.5174360739645181 ) ) ;
#50976=DIRECTION ( 'NONE',  ( 0.000000000000000000, 1.000000000000000000, 0.000000000000000000 ) ) ;
#50978=DIRECTION ( 'NONE',  ( 1.000000000000000000, 0.000000000000000000, 0.000000000000000000 ) ) ;
#50979=EDGE_CURVE ( 'NONE', #48918, #66495, #75305, .T. ) ;
#50982=CARTESIAN_POINT ( 'NONE',  ( 114.4151681834755294, -27.43228005255051016, 274.5441967044824878 ) ) ;
#50983=CARTESIAN_POINT ( 'NONE',  ( 101.5861822943782755, -47.29253114347246623, 13.19562527591094891 ) ) ;
#50985=CARTESIAN_POINT ( 'NONE',  ( 19.56648329127400032, -18.82844715994099971, -5.074374724088000832 ) ) ;
#50989=PLANE ( 'NONE',  #71547 ) ;
#50990=CARTESIAN_POINT ( 'NONE',  ( 131.4143329470395827, -37.45719076514804868, 6.889371645759285734 ) ) ;
#50991=CIRCLE ( 'NONE', #7497, 9.999999999999994671 ) ;
#50992=LINE ( 'NONE', #29665, #22792 ) ;
#50993=DIRECTION ( 'NONE',  ( -0.6544127834855474335, -0.2678505344604094618, 0.7071067811865270336 ) ) ;
#50994=DIRECTION ( 'NONE',  ( 4.299999999999999979E-14, -1.000000000000000000, 0.000000000000000000 ) ) ;
#50996=CARTESIAN_POINT ( 'NONE',  ( 115.6735817710496264, -30.74561775548394849, 279.3099109901964994 ) ) ;
#50997=CARTESIAN_POINT ( 'NONE',  ( 117.0170930581839457, -33.62013007832896960, 170.0670538473399631 ) ) ;
#50998=CARTESIAN_POINT ( 'NONE',  ( 116.6217178149748008, -42.37701578139068204, 279.4137205140061724 ) ) ;
#50999=CIRCLE ( 'NONE', #11849, 2.030000000001310312 ) ;
#51000=CARTESIAN_POINT ( 'NONE',  ( 152.0371591254585724, -47.82818131005588214, 129.9678068554149775 ) ) ;
#51002=CARTESIAN_POINT ( 'NONE',  ( 82.54618223951568723, -35.53884010535914229, 2.747932095373032180 ) ) ;
#51003=CIRCLE ( 'NONE', #58212, 0.4999999999999989453 ) ;
#51004=ORIENTED_EDGE ( 'NONE', *, *, #56184, .T. ) ;
#51005=ADVANCED_FACE ( 'NONE', ( #47122 ), #81245, .T. ) ;
#51006=CARTESIAN_POINT ( 'NONE',  ( 41.56648329127399677, 0.2215528400590013880, 198.9256252759119832 ) ) ;
#51009=CARTESIAN_POINT ( 'NONE',  ( 99.23822674327652749, -42.59304969680523101, 62.83848241876793850 ) ) ;
#51010=FACE_OUTER_BOUND ( 'NONE', #36990, .T. ) ;
#51011=VERTEX_POINT ( 'NONE', #74857 ) ;
#51012=CARTESIAN_POINT ( 'NONE',  ( 116.7948932105152835, -39.38865681179672862, 49.61472410800634947 ) ) ;
#51013=EDGE_CURVE ( 'NONE', #41648, #73742, #5826, .T. ) ;
#51014=CARTESIAN_POINT ( 'NONE',  ( 99.30484619187392070, -29.80227926343066613, 186.7470538473389752 ) ) ;
#51015=DIRECTION ( 'NONE',  ( -1.000000000000000000, -4.299999999999999979E-14, -1.000000000000000078E-15 ) ) ;
#51018=CARTESIAN_POINT ( 'NONE',  ( 94.12733899296569007, -42.07533762155323842, 290.1356252759106837 ) ) ;
#51022=EDGE_CURVE ( 'NONE', #1345, #81899, #39434, .T. ) ;
#51023=CARTESIAN_POINT ( 'NONE',  ( 113.8179087694832958, -44.13528601191151068, 98.16463148459392585 ) ) ;
#51024=CARTESIAN_POINT ( 'NONE',  ( 103.6907823165633005, -45.90921117331532741, 142.2956252759109645 ) ) ;
#51025=ORIENTED_EDGE ( 'NONE', *, *, #68817, .F. ) ;
#51028=CARTESIAN_POINT ( 'NONE',  ( 99.62013013265574557, -29.94545647671011679, 77.17015473446797102 ) ) ;
#51029=CIRCLE ( 'NONE', #16421, 13.99999999999999822 ) ;
#51031=CARTESIAN_POINT ( 'NONE',  ( 114.9950743857440756, -30.04541929558971702, 220.3718157521009573 ) ) ;
#51032=LINE ( 'NONE', #78770, #25964 ) ;
#51033=PLANE ( 'NONE',  #59434 ) ;
#51034=CARTESIAN_POINT ( 'NONE',  ( 97.33783612330317681, -34.07108296596891250, 112.1152844433803750 ) ) ;
#51037=DIRECTION ( 'NONE',  ( 0.000000000000000000, 0.000000000000000000, 1.000000000000000000 ) ) ;
#51040=CARTESIAN_POINT ( 'NONE',  ( 95.33621695423326514, -38.27597901479985865, 151.4299109901969871 ) ) ;
#51043=VERTEX_POINT ( 'NONE', #39868 ) ;
#51045=CARTESIAN_POINT ( 'NONE',  ( 77.49614765539782013, -17.75123073099876336, 2.855912073278433994 ) ) ;
#51046=CARTESIAN_POINT ( 'NONE',  ( 50.97905606905900555, -31.62489322948711035, -5.074374724088000832 ) ) ;
#51048=CARTESIAN_POINT ( 'NONE',  ( 113.6383730011278601, -31.09817814777808564, 227.2204713219719565 ) ) ;
#51049=DIRECTION ( 'NONE',  ( 0.000000000000000000, 0.000000000000000000, -1.000000000000000000 ) ) ;
#51050=CARTESIAN_POINT ( 'NONE',  ( 96.64414437497798360, -36.48068628021362514, 196.3070538473399438 ) ) ;
#51051=CARTESIAN_POINT ( 'NONE',  ( 25.56670390244832802, -48.82844715994168183, 254.7178068554150059 ) ) ;
#51052=VERTEX_POINT ( 'NONE', #67589 ) ;
#51053=VERTEX_POINT ( 'NONE', #66689 ) ;
#51054=ORIENTED_EDGE ( 'NONE', *, *, #58686, .T. ) ;
#51055=CARTESIAN_POINT ( 'NONE',  ( 172.5667039024482960, -42.82844715993499563, 180.4678068554150059 ) ) ;
#51057=DIRECTION ( 'NONE',  ( 0.000000000000000000, 0.000000000000000000, 1.000000000000000000 ) ) ;
#51058=CARTESIAN_POINT ( 'NONE',  ( 29.77381068363742855, -48.62134037875159720, 180.4678068554150911 ) ) ;
#51059=CARTESIAN_POINT ( 'NONE',  ( 101.0802515965118573, -30.15484820110618358, 282.0958690201827039 ) ) ;
#51062=VECTOR ( 'NONE', #30893, 1000.000000000000000 ) ;
#51063=ADVANCED_FACE ( 'NONE', ( #5367 ), #59418, .T. ) ;
#51064=CARTESIAN_POINT ( 'NONE',  ( 114.0818748889228402, -42.19149755589351969, 9.635625275910941312 ) ) ;
#51065=DIRECTION ( 'NONE',  ( 1.907762142705490052E-15, 7.167082501179359715E-16, -1.000000000000000000 ) ) ;
#51067=ORIENTED_EDGE ( 'NONE', *, *, #25945, .F. ) ;
#51070=ORIENTED_EDGE ( 'NONE', *, *, #34478, .F. ) ;
#51071=ORIENTED_EDGE ( 'NONE', *, *, #68658, .F. ) ;
#51072=CARTESIAN_POINT ( 'NONE',  ( 116.4921678451845111, -34.41013889705870099, 13.44099125664899219 ) ) ;
#51073=CARTESIAN_POINT ( 'NONE',  ( 112.4976487814606685, -26.16836495570049337, 169.6984824187679521 ) ) ;
#51074=CARTESIAN_POINT ( 'NONE',  ( 109.0680860650138442, -47.57644715601883689, 127.7337205140059382 ) ) ;
#51075=DIRECTION ( 'NONE',  ( -1.000000000000000078E-15, 1.000000000000000083E-30, 1.000000000000000000 ) ) ;
#51076=CARTESIAN_POINT ( 'NONE',  ( 101.2940058763137330, -26.37990030743140224, 251.4813395616249920 ) ) ;
#51085=CARTESIAN_POINT ( 'NONE',  ( 95.35850850670631473, -38.86301786728916596, 201.4699109901969791 ) ) ;
#51086=ORIENTED_EDGE ( 'NONE', *, *, #9684, .T. ) ;
#51087=CARTESIAN_POINT ( 'NONE',  ( 105.7204000585623191, -24.95538135984382677, 160.1670538473389627 ) ) ;
#51089=CARTESIAN_POINT ( 'NONE',  ( 136.0678963112995064, -34.84294903901248830, 7.549690073094341258 ) ) ;
#51090=FACE_BOUND ( 'NONE', #16722, .T. ) ;
#51091=DIRECTION ( 'NONE',  ( 1.000000000000000000, 4.299999999999999979E-14, 1.000000000000000078E-15 ) ) ;
#51093=CARTESIAN_POINT ( 'NONE',  ( 96.54020141486705597, -31.34005042439575561, 241.9499109901969689 ) ) ;
#51094=DIRECTION ( 'NONE',  ( 1.000000000000000000, 0.000000000000000000, 0.000000000000000000 ) ) ;
#51095=CARTESIAN_POINT ( 'NONE',  ( 37.56670390244720892, -48.82844715994099971, 129.9678068554150911 ) ) ;
#51097=CARTESIAN_POINT ( 'NONE',  ( 102.0649443859646794, -27.97173592226305416, 271.4895552763892965 ) ) ;
#51099=CARTESIAN_POINT ( 'NONE',  ( 101.9936209668059348, -45.44607155354699302, 258.1564586116036253 ) ) ;
#51100=CARTESIAN_POINT ( 'NONE',  ( 194.0371591254582881, -46.82818131005407736, 249.9678068554149775 ) ) ;
#51101=CARTESIAN_POINT ( 'NONE',  ( 112.9776102722344007, -29.11574116196578643, 195.5838068554210167 ) ) ;
#51103=CARTESIAN_POINT ( 'NONE',  ( 135.2499210002603718, -21.21189388395679742, 8.006199623929127540 ) ) ;
#51104=CARTESIAN_POINT ( 'NONE',  ( 107.6557532049571932, -47.79055931493532938, 197.6308633711489620 ) ) ;
#51105=CARTESIAN_POINT ( 'NONE',  ( 118.0020517745808633, -38.33796275862062686, 69.72229194257801055 ) ) ;
#51106=CARTESIAN_POINT ( 'NONE',  ( 101.1761829863686160, -45.38377220964024161, 193.1013395616249682 ) ) ;
#51108=DIRECTION ( 'NONE',  ( 1.639958061481212836E-42, -4.100000000000000342E-29, -1.000000000000000000 ) ) ;
#51110=CARTESIAN_POINT ( 'NONE',  ( 116.8019713974398286, -34.34661232220942395, 40.01729125403449672 ) ) ;
#51111=DIRECTION ( 'NONE',  ( 0.000000000000000000, 0.000000000000000000, 1.000000000000000000 ) ) ;
#51112=CARTESIAN_POINT ( 'NONE',  ( 118.5256205435843526, -36.72944715994100306, 294.6356252759106837 ) ) ;
#51114=CARTESIAN_POINT ( 'NONE',  ( 97.33793630998916058, -34.07062831540125813, 66.11592348782718886 ) ) ;
#51115=ORIENTED_EDGE ( 'NONE', *, *, #19235, .F. ) ;
#51117=EDGE_CURVE ( 'NONE', #29858, #35560, #78111, .T. ) ;
#51118=CARTESIAN_POINT ( 'NONE',  ( 104.0317209996959065, -45.26190801010356779, 101.7390864947439724 ) ) ;
#51119=CARTESIAN_POINT ( 'NONE',  ( 130.5667039024479834, -36.72944715994100306, 239.5838068554162987 ) ) ;
#51120=VERTEX_POINT ( 'NONE', #55276 ) ;
#51121=VECTOR ( 'NONE', #23119, 1000.000000000000114 ) ;
#51122=EDGE_CURVE ( 'NONE', #4991, #60356, #7609, .T. ) ;
#51123=CARTESIAN_POINT ( 'NONE',  ( 117.3173117416416744, -32.65705981835812111, 95.13943479972097350 ) ) ;
#51125=EDGE_CURVE ( 'NONE', #64292, #46374, #41207, .T. ) ;
#51126=CARTESIAN_POINT ( 'NONE',  ( 97.81169128372820865, -40.51741339292117772, 177.6357569005977268 ) ) ;
#51129=CARTESIAN_POINT ( 'NONE',  ( 104.7983354006062058, -46.84845355260645761, 27.38895860924495196 ) ) ;
#51130=EDGE_LOOP ( 'NONE', ( #35624, #18314, #33718, #87527 ) ) ;
#51131=ORIENTED_EDGE ( 'NONE', *, *, #33753, .T. ) ;
#51132=ORIENTED_EDGE ( 'NONE', *, *, #51347, .F. ) ;
#51134=CARTESIAN_POINT ( 'NONE',  ( 151.0371591254575492, -24.95799193692592155, 180.4678068554149775 ) ) ;
#51136=CARTESIAN_POINT ( 'NONE',  ( 115.0889047244793488, -30.61763668078588907, 115.3439586091690785 ) ) ;
#51137=DIRECTION ( 'NONE',  ( 1.000000000000000000, 0.000000000000000000, 0.000000000000000000 ) ) ;
#51138=FACE_BOUND ( 'NONE', #85961, .T. ) ;
#51144=CARTESIAN_POINT ( 'NONE',  ( 96.94826409162251935, -39.14818769109204055, 56.51276813305394597 ) ) ;
#51146=VERTEX_POINT ( 'NONE', #54823 ) ;
#51147=CARTESIAN_POINT ( 'NONE',  ( 97.81171235735017433, -40.51746255502365557, 257.6350867217079212 ) ) ;
#51149=CARTESIAN_POINT ( 'NONE',  ( 111.0233670443594463, -45.12224181339347240, 135.7452332267339443 ) ) ;
#51150=AXIS2_PLACEMENT_3D ( 'NONE', #79499, #51750, #39023 ) ;
#51151=CARTESIAN_POINT ( 'NONE',  ( 100.9527330894022299, -28.70853417486769033, 95.59415746019152493 ) ) ;
#51152=AXIS2_PLACEMENT_3D ( 'NONE', #89663, #6096, #26525 ) ;
#51154=EDGE_LOOP ( 'NONE', ( #11135, #68732, #43698, #42327 ) ) ;
#51155=ORIENTED_EDGE ( 'NONE', *, *, #24471, .T. ) ;
#51156=CARTESIAN_POINT ( 'NONE',  ( 112.0661856499390012, -45.48824432087039327, 137.9874038074903240 ) ) ;
#51157=ORIENTED_EDGE ( 'NONE', *, *, #38299, .T. ) ;
#51158=EDGE_LOOP ( 'NONE', ( #48618, #24517 ) ) ;
#51159=CARTESIAN_POINT ( 'NONE',  ( 102.7360552222912418, -45.06754756083040547, 163.6149166392309837 ) ) ;
#51161=CARTESIAN_POINT ( 'NONE',  ( 117.0539910656555094, -30.30509957368958496, 140.2813395616249750 ) ) ;
#51164=CARTESIAN_POINT ( 'NONE',  ( 116.3188053082936051, -32.94429434937755019, 19.13562527591095019 ) ) ;
#51166=VERTEX_POINT ( 'NONE', #33366 ) ;
#51167=VERTEX_POINT ( 'NONE', #39720 ) ;
#51168=EDGE_CURVE ( 'NONE', #39335, #11421, #4415, .T. ) ;
#51169=CARTESIAN_POINT ( 'NONE',  ( 102.6333607924234883, -43.61639954521550067, 219.9395189410199691 ) ) ;
#51170=CARTESIAN_POINT ( 'NONE',  ( 101.1283730419716562, -27.37881681735623829, 65.51467289495799662 ) ) ;
#51172=CARTESIAN_POINT ( 'NONE',  ( 97.09625384711483775, -33.75906160244644383, 31.09562527591097592 ) ) ;
#51174=PLANE ( 'NONE',  #49505 ) ;
#51175=DIRECTION ( 'NONE',  ( 1.000000000000000078E-15, -1.000000000000000000, 0.000000000000000000 ) ) ;
#51176=CARTESIAN_POINT ( 'NONE',  ( 114.2533759015650787, -44.28132150547345702, 154.1813395616249807 ) ) ;
#51177=CARTESIAN_POINT ( 'NONE',  ( 116.3149231129805941, -32.94053081170188335, 174.1356252759109680 ) ) ;
#51178=EDGE_LOOP ( 'NONE', ( #66371, #42255, #9740, #45448 ) ) ;
#51181=CARTESIAN_POINT ( 'NONE',  ( 165.9667039024459996, -28.27351298637401200, -5.074374724088000832 ) ) ;
#51182=ORIENTED_EDGE ( 'NONE', *, *, #58454, .F. ) ;
#51183=ORIENTED_EDGE ( 'NONE', *, *, #50721, .T. ) ;
#51186=CARTESIAN_POINT ( 'NONE',  ( 115.9861642887573367, -32.12167434585060732, 130.2065129988452270 ) ) ;
#51187=CARTESIAN_POINT ( 'NONE',  ( 117.2669906530413186, -38.88274231480306042, 63.66133956162494911 ) ) ;
#51191=CARTESIAN_POINT ( 'NONE',  ( 106.0550521757682816, -27.00111521709620277, 50.15848241876896907 ) ) ;
#51192=CYLINDRICAL_SURFACE ( 'NONE', #2676, 9.999999999999998224 ) ;
#51193=CARTESIAN_POINT ( 'NONE',  ( 102.9221092647374149, -27.14930527916913050, 151.4013395616249511 ) ) ;
#51194=CARTESIAN_POINT ( 'NONE',  ( 112.1355955708808523, -28.01067529516842214, 59.65679988530178690 ) ) ;
#51196=ORIENTED_EDGE ( 'NONE', *, *, #15010, .T. ) ;
#51199=DIRECTION ( 'NONE',  ( 1.000000000000000000, 0.000000000000000000, 0.000000000000000000 ) ) ;
#51200=EDGE_CURVE ( 'NONE', #18271, #44789, #26551, .T. ) ;
#51201=CARTESIAN_POINT ( 'NONE',  ( 107.0664832912739399, -36.72944715994095333, 357.5272416190308604 ) ) ;
#51202=CARTESIAN_POINT ( 'NONE',  ( 100.6103855434584631, -26.73206753375993827, 220.5327681330539633 ) ) ;
#51204=CARTESIAN_POINT ( 'NONE',  ( 97.33774096734804004, -34.07142221982499564, 146.1148210333605562 ) ) ;
#51205=CARTESIAN_POINT ( 'NONE',  ( 95.27050013873164858, -38.09949539013453546, 232.4184824187679794 ) ) ;
#51206=CARTESIAN_POINT ( 'NONE',  ( 103.2630468498471856, -47.15688066943211254, 93.28610146638693834 ) ) ;
#51209=CARTESIAN_POINT ( 'NONE',  ( 116.7948133712559127, -39.38894117706560394, 264.6149338185274473 ) ) ;
#51210=ORIENTED_EDGE ( 'NONE', *, *, #25793, .T. ) ;
#51217=EDGE_LOOP ( 'NONE', ( #34746, #59229 ) ) ;
#51219=CARTESIAN_POINT ( 'NONE',  ( 109.2119659639152047, -48.38412513495681111, 273.7213395616252569 ) ) ;
#51220=LINE ( 'NONE', #38059, #70764 ) ;
#51221=CARTESIAN_POINT ( 'NONE',  ( 131.4050152070336424, -36.03131342368293133, 2.974074870386977931 ) ) ;
#51222=EDGE_CURVE ( 'NONE', #9402, #89894, #14156, .T. ) ;
#51226=CARTESIAN_POINT ( 'NONE',  ( 113.4141308401190287, -30.97102092343966007, 208.8352769709339896 ) ) ;
#51229=ORIENTED_EDGE ( 'NONE', *, *, #66431, .T. ) ;
#51230=DIRECTION ( 'NONE',  ( -0.000000000000000000, 1.000000000000000000, 0.000000000000000000 ) ) ;
#51231=VECTOR ( 'NONE', #72697, 1000.000000000000000 ) ;
#51232=CARTESIAN_POINT ( 'NONE',  ( 111.0152562398575213, -45.91716645315732848, 182.8994882387802932 ) ) ;
#51233=CARTESIAN_POINT ( 'NONE',  ( 97.54182784564409303, -34.36413255805981493, 272.1327681330532755 ) ) ;
#51235=EDGE_CURVE ( 'NONE', #62232, #77142, #26111, .T. ) ;
#51237=PLANE ( 'NONE',  #89815 ) ;
#51238=EDGE_CURVE ( 'NONE', #43116, #48706, #32940, .T. ) ;
#51241=CARTESIAN_POINT ( 'NONE',  ( 78.92334784196830810, -34.22821065591988798, 1.829869330583619558 ) ) ;
#51242=ORIENTED_EDGE ( 'NONE', *, *, #40558, .F. ) ;
#51244=CARTESIAN_POINT ( 'NONE',  ( 115.1453852183930593, -37.89609606526670404, 26.53094751244894312 ) ) ;
#51245=VECTOR ( 'NONE', #47581, 1000.000000000000000 ) ;
#51246=PLANE ( 'NONE',  #43546 ) ;
#51248=CARTESIAN_POINT ( 'NONE',  ( 57.56670390244747892, -48.82844715994040286, 134.7178068554150911 ) ) ;
#51249=EDGE_LOOP ( 'NONE', ( #82877, #69969, #5914, #8990, #35505, #87548, #989 ) ) ;
#51251=FACE_BOUND ( 'NONE', #72833, .T. ) ;
#51252=VERTEX_POINT ( 'NONE', #68342 ) ;
#51253=CARTESIAN_POINT ( 'NONE',  ( 114.3532617768494504, -44.18530993788802874, 73.19276813305397411 ) ) ;
#51255=CARTESIAN_POINT ( 'NONE',  ( 104.9561144943094035, -45.03597746244296474, 46.80099125664899162 ) ) ;
#51257=CARTESIAN_POINT ( 'NONE',  ( 112.4631721614844651, -29.03839555594388955, 81.00920235351600240 ) ) ;
#51258=CARTESIAN_POINT ( 'NONE',  ( 117.0606442662038091, -38.08221774826209582, 14.71881810016104275 ) ) ;
#51259=CARTESIAN_POINT ( 'NONE',  ( 151.0371591254572934, -24.42818131005592974, 300.4678068554149490 ) ) ;
#51261=CARTESIAN_POINT ( 'NONE',  ( 105.9861696881796860, -26.33857706295247070, 46.15848241876796720 ) ) ;
#51262=DIRECTION ( 'NONE',  ( 0.7071067811865101582, 0.7071067811865849873, 0.000000000000000000 ) ) ;
#51266=ORIENTED_EDGE ( 'NONE', *, *, #81886, .T. ) ;
#51267=CARTESIAN_POINT ( 'NONE',  ( 97.75552660847078812, -42.77168409777202385, 142.7965776568629508 ) ) ;
#51268=DIRECTION ( 'NONE',  ( 1.147230458779309805E-16, 0.000000000000000000, 1.000000000000000000 ) ) ;
#51269=CIRCLE ( 'NONE', #75930, 5.599999999999994316 ) ;
#51270=ORIENTED_EDGE ( 'NONE', *, *, #84663, .F. ) ;
#51271=EDGE_LOOP ( 'NONE', ( #19257, #12575 ) ) ;
#51272=CYLINDRICAL_SURFACE ( 'NONE', #62330, 13.44999999999999396 ) ;
#51273=LINE ( 'NONE', #44017, #28948 ) ;
#51274=CARTESIAN_POINT ( 'NONE',  ( 102.5357197525641766, -45.39752751535337438, 212.1927681330539599 ) ) ;
#51276=LINE ( 'NONE', #1373, #62621 ) ;
#51277=PLANE ( 'NONE',  #80931 ) ;
#51278=CARTESIAN_POINT ( 'NONE',  ( 96.68599849774213340, -42.44610274171655817, 22.72705384733997391 ) ) ;
#51279=DIRECTION ( 'NONE',  ( 0.000000000000000000, 0.000000000000000000, 1.000000000000000000 ) ) ;
#51281=CARTESIAN_POINT ( 'NONE',  ( 116.0758788059830096, -32.34242916441947813, 170.1871404008558670 ) ) ;
#51282=FACE_OUTER_BOUND ( 'NONE', #38987, .T. ) ;
#51283=VERTEX_POINT ( 'NONE', #66989 ) ;
#51284=CARTESIAN_POINT ( 'NONE',  ( 172.5664832912740110, -9.303447159940999356, 321.0426252759119734 ) ) ;
#51286=AXIS2_PLACEMENT_3D ( 'NONE', #35812, #63527, #89913 ) ;
#51288=CARTESIAN_POINT ( 'NONE',  ( 115.9412561796928429, -30.17946786548967353, 259.3203871806730945 ) ) ;
#51289=DIRECTION ( 'NONE',  ( -1.000000000000000078E-15, 0.000000000000000000, -1.000000000000000000 ) ) ;
#51291=FACE_BOUND ( 'NONE', #86047, .T. ) ;
#51292=CARTESIAN_POINT ( 'NONE',  ( 106.0039306387646860, -11.55185827894094786, 322.0356252759110021 ) ) ;
#51293=CARTESIAN_POINT ( 'NONE',  ( 99.20650695390740736, -40.14600596985821568, 231.0752769709339418 ) ) ;
#51294=CARTESIAN_POINT ( 'NONE',  ( 107.0664832912739399, -36.72944715994095333, 294.6356252759106837 ) ) ;
#51295=CARTESIAN_POINT ( 'NONE',  ( 106.5192459994187715, -25.71289806663804711, 41.12800622829193742 ) ) ;
#51297=CARTESIAN_POINT ( 'NONE',  ( 96.59774800590200527, -36.61877842429220209, 111.3184824187679567 ) ) ;
#51299=DIRECTION ( 'NONE',  ( 1.000000000000000000, 4.163336342344333240E-14, 0.000000000000000000 ) ) ;
#51301=EDGE_CURVE ( 'NONE', #16063, #48612, #89240, .T. ) ;
#51302=VECTOR ( 'NONE', #67110, 1000.000000000000000 ) ;
#51303=CARTESIAN_POINT ( 'NONE',  ( 123.0664832912750057, -36.72944715993921960, 9.125625275910985934 ) ) ;
#51304=CARTESIAN_POINT ( 'NONE',  ( 103.2913588842583721, -27.46939931803447976, 276.3845213361897777 ) ) ;
#51305=VERTEX_POINT ( 'NONE', #13379 ) ;
#51306=EDGE_CURVE ( 'NONE', #72479, #52459, #41065, .T. ) ;
#51308=DIRECTION ( 'NONE',  ( 0.7071067708032375831, 0.0001211784769776684463, -0.7071067811865434649 ) ) ;
#51310=DIRECTION ( 'NONE',  ( 1.387778780781444492E-15, 0.000000000000000000, -1.000000000000000000 ) ) ;
#51311=DIRECTION ( 'NONE',  ( 1.000000000000000000, 4.299999999999999979E-14, 1.000000000000000078E-15 ) ) ;
#51313=DIRECTION ( 'NONE',  ( 0.000000000000000000, 1.000000000000000000, 0.000000000000000000 ) ) ;
#51316=CARTESIAN_POINT ( 'NONE',  ( 100.9301527464941444, -28.27416411254235840, 75.57562527591093726 ) ) ;
#51318=EDGE_CURVE ( 'NONE', #67326, #16018, #82883, .T. ) ;
#51319=CARTESIAN_POINT ( 'NONE',  ( 116.3265979651016409, -32.94445627519164077, 14.13562527591094664 ) ) ;
#51320=CARTESIAN_POINT ( 'NONE',  ( 50.56670390244699576, -22.48495420874030515, -5.074374724088000832 ) ) ;
#51321=CARTESIAN_POINT ( 'NONE',  ( 99.04406183884522363, -42.84125761427707602, 141.8439586067010509 ) ) ;
#51322=VERTEX_POINT ( 'NONE', #1088 ) ;
#51324=CARTESIAN_POINT ( 'NONE',  ( 83.06670390244806867, -58.72944715994108122, 231.5838068554169524 ) ) ;
#51325=CARTESIAN_POINT ( 'NONE',  ( 142.0664832912740394, -45.72944715994099596, -5.074374724088994704 ) ) ;
#51326=ADVANCED_FACE ( 'NONE', ( #83316 ), #76494, .T. ) ;
#51327=DIRECTION ( 'NONE',  ( 0.000000000000000000, 1.000000000000000000, 0.000000000000000000 ) ) ;
#51328=DIRECTION ( 'NONE',  ( 0.7071067811865460184, 0.000000000000000000, 0.7071067811865487940 ) ) ;
#51330=DIRECTION ( 'NONE',  ( 6.745093096447288888E-17, 1.000000000000000000, 0.000000000000000000 ) ) ;
#51332=ORIENTED_EDGE ( 'NONE', *, *, #43553, .F. ) ;
#51333=VECTOR ( 'NONE', #21850, 1000.000000000000000 ) ;
#51334=DIRECTION ( 'NONE',  ( 0.000000000000000000, 0.000000000000000000, 1.000000000000000000 ) ) ;
#51335=CARTESIAN_POINT ( 'NONE',  ( 116.4500618263485592, -39.48841239489304655, 179.5984824187679294 ) ) ;
#51336=DIRECTION ( 'NONE',  ( -0.9068632946707807507, 0.4214249218767881500, -9.028300618466658994E-16 ) ) ;
#51338=EDGE_CURVE ( 'NONE', #51651, #48080, #19988, .T. ) ;
#51339=CARTESIAN_POINT ( 'NONE',  ( 105.5226833586260966, -46.38761039419742360, 33.44991099019595282 ) ) ;
#51340=FACE_OUTER_BOUND ( 'NONE', #36719, .T. ) ;
#51342=ADVANCED_FACE ( 'NONE', ( #7005 ), #56482, .T. ) ;
#51343=DIRECTION ( 'NONE',  ( -0.7071067811865171526, -0.7071067811865779928, -7.071067811865164719E-16 ) ) ;
#51346=CARTESIAN_POINT ( 'NONE',  ( 31.71315051186713418, -31.94127993907761009, 117.4678068554150485 ) ) ;
#51347=EDGE_CURVE ( 'NONE', #65933, #62770, #41505, .T. ) ;
#51348=CARTESIAN_POINT ( 'NONE',  ( 109.1965444620390571, -27.18343884754219886, 224.9013395616259459 ) ) ;
#51351=CARTESIAN_POINT ( 'NONE',  ( 108.4337774161041921, -27.97394686652187090, 186.3844404487539634 ) ) ;
#51352=AXIS2_PLACEMENT_3D ( 'NONE', #21920, #42323, #63236 ) ;
#51353=DIRECTION ( 'NONE',  ( -0.9834602067153815907, -0.1811243269341220596, 0.000000000000000000 ) ) ;
#51354=CARTESIAN_POINT ( 'NONE',  ( 114.2978770801668418, -41.85148020179265416, 49.76729759161096922 ) ) ;
#51356=VECTOR ( 'NONE', #74781, 1000.000000000000000 ) ;
#51357=CARTESIAN_POINT ( 'NONE',  ( 188.5667039024479834, -62.87844715994099687, 257.2178068554150059 ) ) ;
#51358=PLANE ( 'NONE',  #2370 ) ;
#51359=AXIS2_PLACEMENT_3D ( 'NONE', #70665, #63850, #48840 ) ;
#51361=CARTESIAN_POINT ( 'NONE',  ( 97.80791547859365664, -40.51903635482080546, 112.6360621818907077 ) ) ;
#51363=ORIENTED_EDGE ( 'NONE', *, *, #9115, .T. ) ;
#51364=CARTESIAN_POINT ( 'NONE',  ( 110.8846227072672121, -27.01418920731891404, 269.7784824187681920 ) ) ;
#51366=VERTEX_POINT ( 'NONE', #41951 ) ;
#51368=DIRECTION ( 'NONE',  ( 0.000000000000000000, 0.000000000000000000, 1.000000000000000000 ) ) ;
#51371=CARTESIAN_POINT ( 'NONE',  ( 97.30224646444959546, -33.23681714887386818, 22.06514908543394426 ) ) ;
#51373=ORIENTED_EDGE ( 'NONE', *, *, #26453, .F. ) ;
#51374=CARTESIAN_POINT ( 'NONE',  ( 99.11046098610404442, -43.53346720896296773, 27.88991099019694175 ) ) ;
#51375=CARTESIAN_POINT ( 'NONE',  ( 125.0664851986225159, -56.72944715994101728, 14.67562527591098842 ) ) ;
#51376=CARTESIAN_POINT ( 'NONE',  ( 111.7737306318703361, -46.73355046572731908, 287.9146728949587555 ) ) ;
#51378=CARTESIAN_POINT ( 'NONE',  ( 82.80042800423676397, -18.38432671279261754, 3.076561810303517497 ) ) ;
#51381=CARTESIAN_POINT ( 'NONE',  ( 114.9276189159122907, -38.92769025571944042, 96.42809036959192781 ) ) ;
#51382=CARTESIAN_POINT ( 'NONE',  ( 101.1884425732228436, -45.36575980889334403, 193.1013395616249682 ) ) ;
#51384=CARTESIAN_POINT ( 'NONE',  ( 134.0664832912740110, -46.72944715994100306, 8.225625275910998013 ) ) ;
#51385=ORIENTED_EDGE ( 'NONE', *, *, #71358, .F. ) ;
#51386=DIRECTION ( 'NONE',  ( 0.000000000000000000, 1.000000000000000000, 0.000000000000000000 ) ) ;
#51387=VERTEX_POINT ( 'NONE', #42844 ) ;
#51388=ORIENTED_EDGE ( 'NONE', *, *, #26937, .F. ) ;
#51389=AXIS2_PLACEMENT_3D ( 'NONE', #3744, #59133, #24630 ) ;
#51392=EDGE_LOOP ( 'NONE', ( #55471, #64501, #67569, #16098 ) ) ;
#51393=LINE ( 'NONE', #50517, #77358 ) ;
#51394=TOROIDAL_SURFACE ( 'NONE', #67351, 15.69999999999999929, 0.2999999999999999889 ) ;
#51396=EDGE_CURVE ( 'NONE', #65745, #75765, #49666, .T. ) ;
#51397=CARTESIAN_POINT ( 'NONE',  ( 103.2789150993301774, -27.47448485603423407, 41.38559085328053300 ) ) ;
#51398=CARTESIAN_POINT ( 'NONE',  ( 112.6791402994794709, -29.62235551608389628, 123.9790864947439815 ) ) ;
#51399=CARTESIAN_POINT ( 'NONE',  ( 96.22633597390384352, -34.45202597047101278, 261.1737205140064475 ) ) ;
#51400=EDGE_CURVE ( 'NONE', #47935, #65138, #70583, .T. ) ;
#51401=CYLINDRICAL_SURFACE ( 'NONE', #83268, 15.99999999999999822 ) ;
#51403=EDGE_CURVE ( 'NONE', #50559, #26343, #76946, .T. ) ;
#51405=CARTESIAN_POINT ( 'NONE',  ( 110.9938485345201258, -27.48116441456390646, 135.7571480591466582 ) ) ;
#51406=ORIENTED_EDGE ( 'NONE', *, *, #37503, .F. ) ;
#51407=DIRECTION ( 'NONE',  ( 0.000000000000000000, 1.000000000000000000, 0.000000000000000000 ) ) ;
#51408=CARTESIAN_POINT ( 'NONE',  ( 116.3219235766278672, -32.94275373074044211, 34.13562527591096085 ) ) ;
#51409=CARTESIAN_POINT ( 'NONE',  ( 30.48091746481831166, -48.32844715994148999, 249.9678068554150059 ) ) ;
#51411=CARTESIAN_POINT ( 'NONE',  ( 97.17500156396280886, -33.29969143728342829, 286.0613395616251751 ) ) ;
#51412=VECTOR ( 'NONE', #14394, 1000.000000000000000 ) ;
#51414=CARTESIAN_POINT ( 'NONE',  ( 97.61519122654028990, -41.12945951998310790, 256.6727681330537507 ) ) ;
#51416=CARTESIAN_POINT ( 'NONE',  ( 99.73159624296292236, -44.24858557630691536, 17.96133956162493206 ) ) ;
#51420=EDGE_CURVE ( 'NONE', #52361, #73456, #34495, .T. ) ;
#51421=DIRECTION ( 'NONE',  ( -1.000000000000000078E-15, 1.000000000000000083E-30, 1.000000000000000000 ) ) ;
#51423=CARTESIAN_POINT ( 'NONE',  ( 106.1313900203587366, -25.30815840704239150, 323.4690612957397775 ) ) ;
#51426=AXIS2_PLACEMENT_3D ( 'NONE', #48281, #57352, #63738 ) ;
#51427=CIRCLE ( 'NONE', #57268, 1.000000000000000888 ) ;
#51428=DIRECTION ( 'NONE',  ( -0.7071067811607679721, 0.7071067812123270624, 0.000000000000000000 ) ) ;
#51430=EDGE_CURVE ( 'NONE', #51167, #76957, #43183, .T. ) ;
#51432=CARTESIAN_POINT ( 'NONE',  ( 134.0664832912740110, -46.72944715994100306, 1.625625275910997480 ) ) ;
#51433=CARTESIAN_POINT ( 'NONE',  ( 96.29878009220107060, -39.42515072222565209, 16.53372051400597798 ) ) ;
#51434=CARTESIAN_POINT ( 'NONE',  ( 117.4872506282070503, -40.41476785070875621, 174.5680062282919778 ) ) ;
#51435=CARTESIAN_POINT ( 'NONE',  ( 106.9270610292626742, -26.24804662171751346, 56.08705384733997334 ) ) ;
#51437=CARTESIAN_POINT ( 'NONE',  ( 115.7831076706773388, -41.80230950916739374, 48.40645860934917977 ) ) ;
#51438=DIRECTION ( 'NONE',  ( 0.000000000000000000, 0.000000000000000000, 1.000000000000000000 ) ) ;
#51439=EDGE_CURVE ( 'NONE', #28273, #16229, #43296, .T. ) ;
#51443=CARTESIAN_POINT ( 'NONE',  ( 116.8124865092210456, -37.88235468918157522, 49.73276813305294297 ) ) ;
#51444=PLANE ( 'NONE',  #750 ) ;
#51447=CARTESIAN_POINT ( 'NONE',  ( 117.2062538965839309, -41.07097622818925942, 209.5165776568640013 ) ) ;
#51448=CARTESIAN_POINT ( 'NONE',  ( 162.8913605087219878, -31.76306994223740432, -5.074374724088000832 ) ) ;
#51449=CARTESIAN_POINT ( 'NONE',  ( 97.81556513139278763, -40.52688310217321543, 146.6364384312551294 ) ) ;
#51452=EDGE_CURVE ( 'NONE', #26493, #38746, #63487, .T. ) ;
#51454=CARTESIAN_POINT ( 'NONE',  ( 41.56648329127499153, -32.07844715994070839, 18.92562527591200094 ) ) ;
#51456=CARTESIAN_POINT ( 'NONE',  ( 113.4935171807054246, -28.59114140144088623, 124.5565776568639507 ) ) ;
#51457=ORIENTED_EDGE ( 'NONE', *, *, #77128, .F. ) ;
#51458=VERTEX_POINT ( 'NONE', #58709 ) ;
#51460=CARTESIAN_POINT ( 'NONE',  ( 112.3776303481765950, -29.59825886299321951, 100.9987261630399757 ) ) ;
#51462=CARTESIAN_POINT ( 'NONE',  ( 114.8736367985562623, -30.83777597042988106, 215.3413395616249773 ) ) ;
#51463=DIRECTION ( 'NONE',  ( 5.512527431108029424E-15, -1.000000000000000000, 0.000000000000000000 ) ) ;
#51464=VECTOR ( 'NONE', #89779, 1000.000000000000114 ) ;
#51465=DIRECTION ( 'NONE',  ( 1.000000000000000000, -8.545435842250265406E-15, 0.000000000000000000 ) ) ;
#51469=DIRECTION ( 'NONE',  ( 1.000000000000000000, 6.493183223601999383E-14, 9.351236661543306751E-17 ) ) ;
#51471=CARTESIAN_POINT ( 'NONE',  ( 117.2167691715783064, -39.01263929987995027, 148.6499109901969859 ) ) ;
#51472=ORIENTED_EDGE ( 'NONE', *, *, #67116, .T. ) ;
#51474=DIRECTION ( 'NONE',  ( 1.000000000000000000, 0.000000000000000000, 0.000000000000000000 ) ) ;
#51475=CARTESIAN_POINT ( 'NONE',  ( 134.0664832912740110, -8.350947159940998787, 291.1181252759119502 ) ) ;
#51477=CYLINDRICAL_SURFACE ( 'NONE', #383, 3.000000000000002665 ) ;
#51479=AXIS2_PLACEMENT_3D ( 'NONE', #51454, #43759, #71495 ) ;
#51481=CARTESIAN_POINT ( 'NONE',  ( 116.3115597373110290, -32.94279827685361539, 270.1356252759109680 ) ) ;
#51483=VECTOR ( 'NONE', #85509, 1000.000000000000000 ) ;
#51484=CARTESIAN_POINT ( 'NONE',  ( 113.5652313304969567, -44.92653082429684730, 168.1099109901969939 ) ) ;
#51485=CARTESIAN_POINT ( 'NONE',  ( 83.73314995793998605, 12.92155284005730387, 355.9756252759109998 ) ) ;
#51487=ORIENTED_EDGE ( 'NONE', *, *, #73563, .F. ) ;
#51488=ORIENTED_EDGE ( 'NONE', *, *, #29676, .F. ) ;
#51489=CARTESIAN_POINT ( 'NONE',  ( 115.4190912951222288, -42.26680109789320028, 64.36133032379248675 ) ) ;
#51491=PLANE ( 'NONE',  #9260 ) ;
#51492=CARTESIAN_POINT ( 'NONE',  ( 105.6993345102559942, -28.68213381844667609, 13.02809036959096112 ) ) ;
#51493=CARTESIAN_POINT ( 'NONE',  ( 104.4080996569733770, -46.45808887385236829, 272.3647918606883991 ) ) ;
#51494=ORIENTED_EDGE ( 'NONE', *, *, #50935, .T. ) ;
#51495=AXIS2_PLACEMENT_3D ( 'NONE', #45077, #10571, #73233 ) ;
#51496=CARTESIAN_POINT ( 'NONE',  ( 115.1675060414467993, -40.96806874415090505, 9.635625275910943088 ) ) ;
#51497=EDGE_CURVE ( 'NONE', #58643, #57294, #53036, .T. ) ;
#51499=VERTEX_POINT ( 'NONE', #72368 ) ;
#51502=ORIENTED_EDGE ( 'NONE', *, *, #83670, .F. ) ;
#51503=ORIENTED_EDGE ( 'NONE', *, *, #39436, .F. ) ;
#51504=AXIS2_PLACEMENT_3D ( 'NONE', #85549, #2864, #3748 ) ;
#51505=ADVANCED_FACE ( 'NONE', ( #65098 ), #59159, .T. ) ;
#51507=CARTESIAN_POINT ( 'NONE',  ( 100.5751258508236674, -42.28088033547287949, 31.31241982807697610 ) ) ;
#51508=CARTESIAN_POINT ( 'NONE',  ( 117.0443417989465758, -39.94358261462815562, 158.5784824187679476 ) ) ;
#51509=EDGE_CURVE ( 'NONE', #34951, #73279, #24652, .T. ) ;
#51510=CARTESIAN_POINT ( 'NONE',  ( 118.8928063919343998, -36.92768728534039724, 153.8127681330539644 ) ) ;
#51511=FACE_OUTER_BOUND ( 'NONE', #74032, .T. ) ;
#51512=CARTESIAN_POINT ( 'NONE',  ( 103.0905057572046672, -47.89305850247227880, 248.3041967044829619 ) ) ;
#51513=CARTESIAN_POINT ( 'NONE',  ( 41.56670390244689628, -36.32844715994109208, 180.4678068554150911 ) ) ;
#51514=LINE ( 'NONE', #58344, #10382 ) ;
#51517=EDGE_CURVE ( 'NONE', #43446, #52666, #80082, .T. ) ;
#51518=ORIENTED_EDGE ( 'NONE', *, *, #18409, .F. ) ;
#51521=CARTESIAN_POINT ( 'NONE',  ( 115.0734612967709722, -29.04171753102041365, 189.4232443235299570 ) ) ;
#51522=ORIENTED_EDGE ( 'NONE', *, *, #57996, .T. ) ;
#51523=CARTESIAN_POINT ( 'NONE',  ( 113.6143417880574020, -45.63476223351307226, 183.0689586092439640 ) ) ;
#51524=DIRECTION ( 'NONE',  ( 0.7071067811869279351, -0.7071067811861670993, 6.612322855863716074E-17 ) ) ;
#51525=AXIS2_PLACEMENT_3D ( 'NONE', #18152, #31337, #87211 ) ;
#51528=CARTESIAN_POINT ( 'NONE',  ( 123.6837132603318707, -20.11243780205705534, 219.5838068554170093 ) ) ;
#51529=DIRECTION ( 'NONE',  ( 0.000000000000000000, 0.000000000000000000, -1.000000000000000000 ) ) ;
#51530=CARTESIAN_POINT ( 'NONE',  ( 104.5933598291445605, -26.62426044571802208, 281.2670538473395823 ) ) ;
#51532=CARTESIAN_POINT ( 'NONE',  ( 130.0664832912740110, -18.82844715994099971, 226.9256252759120116 ) ) ;
#51533=ADVANCED_FACE ( 'NONE', ( #2437 ), #38278, .T. ) ;
#51534=CARTESIAN_POINT ( 'NONE',  ( 105.7964350658774180, -26.72445465374488549, 271.1771098916634628 ) ) ;
#51538=CARTESIAN_POINT ( 'NONE',  ( 99.65405756092035006, -40.29016652223857164, 195.5838068554173219 ) ) ;
#51539=VERTEX_POINT ( 'NONE', #57831 ) ;
#51540=CYLINDRICAL_SURFACE ( 'NONE', #52424, 0.9999999999999731326 ) ;
#51541=CARTESIAN_POINT ( 'NONE',  ( 97.36144725414590084, -42.06870896796115034, 176.7146728949589658 ) ) ;
#51542=CARTESIAN_POINT ( 'NONE',  ( 103.8413319783160489, -46.68031304110885316, 78.32705384733995402 ) ) ;
#51543=CARTESIAN_POINT ( 'NONE',  ( 118.0865697951701350, -35.40461063965730659, 234.9337205140059552 ) ) ;
#51545=CARTESIAN_POINT ( 'NONE',  ( 19.56670390244648416, -25.42844715994203852, 129.9678068554150627 ) ) ;
#51546=FACE_OUTER_BOUND ( 'NONE', #79990, .T. ) ;
#51547=CARTESIAN_POINT ( 'NONE',  ( 117.0736645660960988, -36.55483027940629626, 39.84004045961177809 ) ) ;
#51550=EDGE_LOOP ( 'NONE', ( #5498, #57307, #43239, #68394 ) ) ;
#51551=CARTESIAN_POINT ( 'NONE',  ( 100.9557301351062932, -28.70619097067474002, 65.59534030220335410 ) ) ;
#51555=AXIS2_PLACEMENT_3D ( 'NONE', #47556, #14867, #56159 ) ;
#51556=ORIENTED_EDGE ( 'NONE', *, *, #55362, .T. ) ;
#51557=ORIENTED_EDGE ( 'NONE', *, *, #10248, .F. ) ;
#51558=VECTOR ( 'NONE', #77380, 1000.000000000000000 ) ;
#51559=CARTESIAN_POINT ( 'NONE',  ( 114.8760577754623569, -30.96046336120327069, 108.7552769709339771 ) ) ;
#51562=CARTESIAN_POINT ( 'NONE',  ( 101.6894933626720245, -27.09867346898214180, 101.4937205140059575 ) ) ;
#51563=CARTESIAN_POINT ( 'NONE',  ( 71.25529199314597406, -79.12815651470191369, 361.9756252759101471 ) ) ;
#51564=CARTESIAN_POINT ( 'NONE',  ( 79.05226586200201666, -16.17316201338597637, 8.065992442479700486 ) ) ;
#51567=VECTOR ( 'NONE', #86782, 1000.000000000000000 ) ;
#51568=CARTESIAN_POINT ( 'NONE',  ( 104.8797383215544556, -46.86635653470259655, 32.41943479972098174 ) ) ;
#51570=VERTEX_POINT ( 'NONE', #65542 ) ;
#51572=CARTESIAN_POINT ( 'NONE',  ( 125.0664851986225159, -56.72944715994084675, -4.970821333495647920 ) ) ;
#51573=CARTESIAN_POINT ( 'NONE',  ( 34.27482367531361973, -30.08671355700341010, 193.9678068554150911 ) ) ;
#51578=DIRECTION ( 'NONE',  ( 0.000000000000000000, 1.000000000000000000, 0.000000000000000000 ) ) ;
#51581=CARTESIAN_POINT ( 'NONE',  ( 107.6057229598026339, -48.54288983744056907, 42.61276813305398292 ) ) ;
#51586=LINE ( 'NONE', #52892, #24543 ) ;
#51587=B_SPLINE_CURVE_WITH_KNOTS ( 'NONE', 3,
 ( #64685, #73266, #86481, #66451, #3357, #31047, #51914, #58737, #25125, #72402, #11048, #4240, #45109, #10601, #37875, #59186, #79673, #38307 ),
 .UNSPECIFIED., .F., .F.,
 ( 4, 2, 2, 2, 2, 2, 2, 2, 4 ),
 ( 0.5000000022694898183, 0.5625000019858036326, 0.6250000017021173360, 0.6875000014184311503, 0.7500000011347449647, 0.8125000008510586680, 0.8750000005673724823, 0.9375000002836861857, 1.000000000000000000 ),
 .UNSPECIFIED. ) ;
#51589=CARTESIAN_POINT ( 'NONE',  ( 113.0992926495536182, -42.93477843977468922, 116.0204713219719679 ) ) ;
#51600=CARTESIAN_POINT ( 'NONE',  ( 104.2961655698287302, -28.31198801876947613, 161.7615833058969486 ) ) ;
#51602=CARTESIAN_POINT ( 'NONE',  ( 96.58534993179142703, -36.88768535406505578, 132.3384824187679669 ) ) ;
#51603=DIRECTION ( 'NONE',  ( -0.7071067811865270336, 0.7071067811865680008, -7.071067811865277132E-16 ) ) ;
#51604=CARTESIAN_POINT ( 'NONE',  ( 108.3328101825627385, -46.73493184262017763, 17.67728433966769686 ) ) ;
#51605=AXIS2_PLACEMENT_3D ( 'NONE', #46096, #5241, #75176 ) ;
#51606=ORIENTED_EDGE ( 'NONE', *, *, #54427, .T. ) ;
#51607=CIRCLE ( 'NONE', #87883, 1.000000000000000888 ) ;
#51608=CONICAL_SURFACE ( 'NONE', #61791, 1.258750000000002922, 1.029744258676650093 ) ;
#51609=AXIS2_PLACEMENT_3D ( 'NONE', #27800, #55480, #15078 ) ;
#51611=ORIENTED_EDGE ( 'NONE', *, *, #79771, .T. ) ;
#51612=EDGE_CURVE ( 'NONE', #67030, #2296, #44602, .T. ) ;
#51613=CARTESIAN_POINT ( 'NONE',  ( 98.90610402553750191, -36.53467484046868208, 194.1252332267349630 ) ) ;
#51614=CARTESIAN_POINT ( 'NONE',  ( 104.0363141061766186, -47.38371934748259662, 67.36800622829191809 ) ) ;
#51615=ORIENTED_EDGE ( 'NONE', *, *, #56459, .T. ) ;
#51616=EDGE_CURVE ( 'NONE', #752, #34034, #6948, .T. ) ;
#51617=CARTESIAN_POINT ( 'NONE',  ( 100.9539191370901960, -46.85292318231938680, 52.14419670448194921 ) ) ;
#51618=DIRECTION ( 'NONE',  ( 0.7071067811869841124, -0.7071067811861110330, 0.000000000000000000 ) ) ;
#51620=CARTESIAN_POINT ( 'NONE',  ( 107.3661318999371161, -25.27282818541385367, 323.3302093749328492 ) ) ;
#51621=EDGE_CURVE ( 'NONE', #26492, #85897, #57719, .T. ) ;
#51622=CARTESIAN_POINT ( 'NONE',  ( 97.67470816545109358, -41.25460433215529577, 167.6841967044829573 ) ) ;
#51623=CARTESIAN_POINT ( 'NONE',  ( 162.7131505118549057, -33.70561438051511516, 237.4678068554150059 ) ) ;
#51624=ORIENTED_EDGE ( 'NONE', *, *, #85077, .F. ) ;
#51626=ADVANCED_FACE ( 'NONE', ( #45046 ), #30984, .T. ) ;
#51628=DIRECTION ( 'NONE',  ( 0.000000000000000000, 0.000000000000000000, 1.000000000000000000 ) ) ;
#51629=CARTESIAN_POINT ( 'NONE',  ( 138.8167039024479834, -50.82844715994100682, 35.51780685541480409 ) ) ;
#51630=AXIS2_PLACEMENT_3D ( 'NONE', #60573, #24726, #86965 ) ;
#51634=CARTESIAN_POINT ( 'NONE',  ( 117.9889986865933196, -38.42583888725547325, 68.69181575210198787 ) ) ;
#51635=CARTESIAN_POINT ( 'NONE',  ( 32.06670390244800473, -33.35206098992711077, -5.074374724088000832 ) ) ;
#51636=AXIS2_PLACEMENT_3D ( 'NONE', #36626, #15733, #26758 ) ;
#51637=CARTESIAN_POINT ( 'NONE',  ( 100.1253875378088338, -39.57043109886122778, 9.125625275910969947 ) ) ;
#51639=CARTESIAN_POINT ( 'NONE',  ( 117.4022237771662276, -37.57280582802028590, 38.77372051400595865 ) ) ;
#51640=CARTESIAN_POINT ( 'NONE',  ( 126.8164832912740394, -54.72944906728950798, -5.074374724089010691 ) ) ;
#51641=CARTESIAN_POINT ( 'NONE',  ( 112.7681627534586113, -45.43114336468919134, 174.0384824187679556 ) ) ;
#51642=LINE ( 'NONE', #82962, #16117 ) ;
#51644=EDGE_CURVE ( 'NONE', #74639, #53210, #59566, .T. ) ;
#51645=ORIENTED_EDGE ( 'NONE', *, *, #75928, .T. ) ;
#51646=CARTESIAN_POINT ( 'NONE',  ( 83.06670390244796920, -67.87844715994100397, 225.9838068554150254 ) ) ;
#51647=DIRECTION ( 'NONE',  ( 1.000000000000000000, 4.299999999999999979E-14, 1.000000000000000078E-15 ) ) ;
#51649=DIRECTION ( 'NONE',  ( 0.000000000000000000, 0.000000000000000000, -1.000000000000000000 ) ) ;
#51650=CARTESIAN_POINT ( 'NONE',  ( 113.0507064547910829, -46.07834852625790489, 218.0175300378159591 ) ) ;
#51651=VERTEX_POINT ( 'NONE', #17363 ) ;
#51652=DIRECTION ( 'NONE',  ( -4.237773401492740281E-14, 1.000000000000000000, 0.000000000000000000 ) ) ;
#51653=CARTESIAN_POINT ( 'NONE',  ( 116.9459113946819286, -41.73765103896904805, 244.4651490854349731 ) ) ;
#51654=CARTESIAN_POINT ( 'NONE',  ( 99.47006920962783738, -43.93274313109116491, 77.92991099019597812 ) ) ;
#51655=DIRECTION ( 'NONE',  ( 0.000000000000000000, 0.000000000000000000, 1.000000000000000000 ) ) ;
#51656=CARTESIAN_POINT ( 'NONE',  ( 98.34933868204893770, -31.65751815772215849, 191.9063711284184706 ) ) ;
#51657=VECTOR ( 'NONE', #31273, 1000.000000000000000 ) ;
#51658=CARTESIAN_POINT ( 'NONE',  ( 172.5667039024480118, -36.32844715993499563, 180.4678068554150059 ) ) ;
#51659=CARTESIAN_POINT ( 'NONE',  ( 25.56670390244832447, -48.82844715994168183, 257.2178068554150059 ) ) ;
#51662=ORIENTED_EDGE ( 'NONE', *, *, #54163, .F. ) ;
#51664=CARTESIAN_POINT ( 'NONE',  ( 167.2371591254544967, -47.82818131005522133, 180.4678068554150059 ) ) ;
#51665=CARTESIAN_POINT ( 'NONE',  ( 116.2186307022408727, -41.79497087860992366, 259.4241967044825969 ) ) ;
#51670=AXIS2_PLACEMENT_3D ( 'NONE', #6267, #40326, #82148 ) ;
#51673=CARTESIAN_POINT ( 'NONE',  ( 115.3666750469823938, -34.71377145672549602, 208.4381341137909658 ) ) ;
#51674=EDGE_LOOP ( 'NONE', ( #57103, #1513 ) ) ;
#51675=ORIENTED_EDGE ( 'NONE', *, *, #87176, .T. ) ;
#51676=AXIS2_PLACEMENT_3D ( 'NONE', #1001, #42311, #6467 ) ;
#51677=ORIENTED_EDGE ( 'NONE', *, *, #22142, .F. ) ;
#51678=CIRCLE ( 'NONE', #12532, 3.249999999999975131 ) ;
#51679=CARTESIAN_POINT ( 'NONE',  ( 107.0667039024479834, -48.82844715994099971, 160.9178068554150229 ) ) ;
#51680=CIRCLE ( 'NONE', #61857, 2.500000000000002220 ) ;
#51681=CARTESIAN_POINT ( 'NONE',  ( 98.15099777509990986, -41.26165302448119121, 181.7007408304860689 ) ) ;
#51683=CARTESIAN_POINT ( 'NONE',  ( 114.8131502045275880, -44.70447909941016462, 264.1899109901960401 ) ) ;
#51684=CARTESIAN_POINT ( 'NONE',  ( 176.7669697523286061, -48.62818131005462163, 300.4678068554149490 ) ) ;
#51685=DIRECTION ( 'NONE',  ( 0.000000000000000000, 0.000000000000000000, 1.000000000000000000 ) ) ;
#51686=CARTESIAN_POINT ( 'NONE',  ( 97.81170495107971874, -40.51745053935989915, 26.63526479160227112 ) ) ;
#51687=ORIENTED_EDGE ( 'NONE', *, *, #74397, .F. ) ;
#51688=CARTESIAN_POINT ( 'NONE',  ( 103.2843211798393241, -27.47227357675608772, 56.38512623260010770 ) ) ;
#51690=AXIS2_PLACEMENT_3D ( 'NONE', #9200, #85521, #50962 ) ;
#51692=CARTESIAN_POINT ( 'NONE',  ( 98.94126815719160106, -33.74921318831734851, 18.85285227435401367 ) ) ;
#51693=EDGE_CURVE ( 'NONE', #228, #10278, #86860, .T. ) ;
#51694=CARTESIAN_POINT ( 'NONE',  ( 36.65249034007526063, -48.32844715994123419, 300.4678068554150059 ) ) ;
#51695=CARTESIAN_POINT ( 'NONE',  ( 20.03715912545735023, -46.82818131006202123, 180.4678068554150911 ) ) ;
#51697=ORIENTED_EDGE ( 'NONE', *, *, #2200, .T. ) ;
#51699=DIRECTION ( 'NONE',  ( 0.000000000000000000, 1.000000000000000000, 0.000000000000000000 ) ) ;
#51700=VERTEX_POINT ( 'NONE', #24185 ) ;
#51701=CARTESIAN_POINT ( 'NONE',  ( 99.50153220775246155, -43.90290835836871253, 81.92991099019597812 ) ) ;
#51703=CARTESIAN_POINT ( 'NONE',  ( 115.5775591941339542, -37.73626844564258676, 53.15527697093397563 ) ) ;
#51704=CARTESIAN_POINT ( 'NONE',  ( 105.2997058862832347, -46.60644133428081659, 88.43476079292317138 ) ) ;
#51705=CARTESIAN_POINT ( 'NONE',  ( 104.3250142303409831, -45.18796221723782480, 78.75872616303996665 ) ) ;
#51706=FACE_BOUND ( 'NONE', #68144, .T. ) ;
#51709=CIRCLE ( 'NONE', #67682, 5.599999999999994316 ) ;
#51710=CARTESIAN_POINT ( 'NONE',  ( 111.0545523236672807, -47.06291463499678684, 13.85753003781498016 ) ) ;
#51711=DIRECTION ( 'NONE',  ( 0.7071067811866377228, -0.7071067811864573116, 0.000000000000000000 ) ) ;
#51712=ORIENTED_EDGE ( 'NONE', *, *, #76659, .F. ) ;
#51713=DIRECTION ( 'NONE',  ( 0.0001713722456133526934, -0.9999999853157766072, 0.000000000000000000 ) ) ;
#51714=ORIENTED_EDGE ( 'NONE', *, *, #85853, .F. ) ;
#51715=CARTESIAN_POINT ( 'NONE',  ( 96.62748084391311920, -35.94289726309906996, 142.2670538473399517 ) ) ;
#51716=CARTESIAN_POINT ( 'NONE',  ( 78.64593636901959428, -21.09121833381964706, 1.942446336658495643 ) ) ;
#51717=ORIENTED_EDGE ( 'NONE', *, *, #8569, .T. ) ;
#51718=ORIENTED_EDGE ( 'NONE', *, *, #977, .F. ) ;
#51721=CARTESIAN_POINT ( 'NONE',  ( 109.8674951572811551, -26.74480306206631397, 219.8708633711499658 ) ) ;
#51722=CARTESIAN_POINT ( 'NONE',  ( 115.5869760628213214, -31.41147761708738173, 124.2698573529066977 ) ) ;
#51723=CARTESIAN_POINT ( 'NONE',  ( 71.25614885437424562, -84.12815644128085069, 396.9756252759102040 ) ) ;
#51724=EDGE_CURVE ( 'NONE', #34970, #79915, #30168, .T. ) ;
#51725=CARTESIAN_POINT ( 'NONE',  ( 96.95674990518240577, -32.26097187787489418, 51.98324432352996638 ) ) ;
#51726=CARTESIAN_POINT ( 'NONE',  ( 72.06648329127399677, -8.729447159941065237, -4.824374724089063982 ) ) ;
#51728=CARTESIAN_POINT ( 'NONE',  ( 107.8824949288598987, -26.74133428231821696, 171.0115286325450654 ) ) ;
#51729=CIRCLE ( 'NONE', #77834, 4.875000000000017764 ) ;
#51730=DIRECTION ( 'NONE',  ( 0.7071067811865475727, -0.7071067811865475727, 0.000000000000000000 ) ) ;
#51731=EDGE_LOOP ( 'NONE', ( #25095, #74508, #62894, #76125, #63210, #85474, #6274, #64724, #72261, #43573, #89526, #5675 ) ) ;
#51733=PLANE ( 'NONE',  #79351 ) ;
#51734=VECTOR ( 'NONE', #33624, 1000.000000000000000 ) ;
#51735=CARTESIAN_POINT ( 'NONE',  ( 83.06670390244796920, -58.72944715994093201, 204.3338068554149913 ) ) ;
#51736=CARTESIAN_POINT ( 'NONE',  ( 96.14807755961376756, -35.16348456217429685, 226.2251490854349640 ) ) ;
#51737=LINE ( 'NONE', #67166, #9536 ) ;
#51741=CARTESIAN_POINT ( 'NONE',  ( 104.8904560483511545, -27.93868065388478428, 239.6800388756959705 ) ) ;
#51743=CARTESIAN_POINT ( 'NONE',  ( 117.0329088946582630, -32.00354160957723337, 60.19086337114898555 ) ) ;
#51745=CARTESIAN_POINT ( 'NONE',  ( 96.65525155030036331, -37.83077348759547220, 126.4099109901969626 ) ) ;
#51747=CARTESIAN_POINT ( 'NONE',  ( 46.03715912545348488, -48.62818131006090283, 129.9678068554150911 ) ) ;
#51748=ADVANCED_FACE ( 'NONE', ( #38246 ), #78719, .F. ) ;
#51750=DIRECTION ( 'NONE',  ( 1.000000000000000078E-15, -1.000000000000000083E-30, -1.000000000000000000 ) ) ;
#51751=LINE ( 'NONE', #64517, #1467 ) ;
#51753=CARTESIAN_POINT ( 'NONE',  ( 134.0664832912740110, -33.97944715994100306, 1.625625275910997480 ) ) ;
#51755=CARTESIAN_POINT ( 'NONE',  ( 97.39139531738810263, -39.27891137106568920, 51.53149185393750287 ) ) ;
#51756=EDGE_LOOP ( 'NONE', ( #18330, #11801 ) ) ;
#51759=AXIS2_PLACEMENT_3D ( 'NONE', #6844, #75890, #13660 ) ;
#51761=ORIENTED_EDGE ( 'NONE', *, *, #33896, .F. ) ;
#51763=CARTESIAN_POINT ( 'NONE',  ( 99.48556355041279176, -43.91805062995148745, 81.92991099019597812 ) ) ;
#51765=DIRECTION ( 'NONE',  ( 0.7071067811739204512, -0.7071067811991745833, 0.000000000000000000 ) ) ;
#51768=ORIENTED_EDGE ( 'NONE', *, *, #70371, .F. ) ;
#51769=DIRECTION ( 'NONE',  ( -2.999999999999999839E-15, 1.000000000000000000, -2.999999999999999900E-30 ) ) ;
#51771=CARTESIAN_POINT ( 'NONE',  ( 141.9629299006807059, -45.68655394112752077, 14.92562527591105415 ) ) ;
#51772=CARTESIAN_POINT ( 'NONE',  ( 90.44969454456405344, -20.11243780205715481, 219.5838068554169809 ) ) ;
#51773=CARTESIAN_POINT ( 'NONE',  ( 184.5667039024480118, -67.87844715994100397, 310.9178068554150514 ) ) ;
#51774=CARTESIAN_POINT ( 'NONE',  ( 107.0664832912739399, -36.72944715994095333, 312.1356252759112522 ) ) ;
#51777=CARTESIAN_POINT ( 'NONE',  ( 164.9212702847350158, -29.73316016639540749, 193.9678068554150059 ) ) ;
#51778=EDGE_CURVE ( 'NONE', #79496, #11556, #86713, .T. ) ;
#51779=CARTESIAN_POINT ( 'NONE',  ( 108.7386892141029335, -46.36620816325528693, 163.7127681330539701 ) ) ;
#51781=ORIENTED_EDGE ( 'NONE', *, *, #40637, .T. ) ;
#51782=CARTESIAN_POINT ( 'NONE',  ( 104.7983354005985888, -46.84845355258768507, 23.38895860924395009 ) ) ;
#51784=CARTESIAN_POINT ( 'NONE',  ( 182.3467384525650061, -36.02818131005800950, -5.074374724088000832 ) ) ;
#51785=PLANE ( 'NONE',  #86272 ) ;
#51786=EDGE_LOOP ( 'NONE', ( #86407, #59516 ) ) ;
#51787=CARTESIAN_POINT ( 'NONE',  ( 107.0664832912739968, -36.72944715994100306, 293.2242906452868851 ) ) ;
#51788=AXIS2_PLACEMENT_3D ( 'NONE', #42946, #57484, #85223 ) ;
#51791=ORIENTED_EDGE ( 'NONE', *, *, #15338, .F. ) ;
#51792=CARTESIAN_POINT ( 'NONE',  ( 97.69936372639945432, -35.99897019620807725, 187.7082499725639764 ) ) ;
#51793=VECTOR ( 'NONE', #29564, 1000.000000000000000 ) ;
#51794=CARTESIAN_POINT ( 'NONE',  ( 51.06648329127330044, -0.7548456658612000547, 335.0256252759120343 ) ) ;
#51795=AXIS2_PLACEMENT_3D ( 'NONE', #17657, #24478, #37658 ) ;
#51796=EDGE_CURVE ( 'NONE', #30264, #88540, #76606, .T. ) ;
#51797=CARTESIAN_POINT ( 'NONE',  ( 109.8762032759827321, -45.69504804023497968, 49.23777378208799149 ) ) ;
#51799=CARTESIAN_POINT ( 'NONE',  ( 100.9546728179205815, -28.70702572233378191, 80.59395860859407890 ) ) ;
#51800=CARTESIAN_POINT ( 'NONE',  ( 63.03715912545825262, -46.82818131006018092, 249.9678068554150343 ) ) ;
#51803=DIRECTION ( 'NONE',  ( 0.000000000000000000, 0.000000000000000000, 1.000000000000000000 ) ) ;
#51804=VERTEX_POINT ( 'NONE', #64615 ) ;
#51805=CARTESIAN_POINT ( 'NONE',  ( 100.1919508713739049, -45.35525880799018239, 272.0289586092443415 ) ) ;
#51808=EDGE_CURVE ( 'NONE', #79084, #25402, #80051, .T. ) ;
#51813=FACE_OUTER_BOUND ( 'NONE', #27719, .T. ) ;
#51814=VECTOR ( 'NONE', #62873, 1000.000000000000000 ) ;
#51815=LINE ( 'NONE', #16877, #63626 ) ;
#51816=CARTESIAN_POINT ( 'NONE',  ( 116.5662105847193999, -41.21199064955116143, 224.4756252759109714 ) ) ;
#51819=CARTESIAN_POINT ( 'NONE',  ( 117.4979393226723516, -37.96344061660173708, 49.73276813305393773 ) ) ;
#51820=DIRECTION ( 'NONE',  ( -0.7071067811865434649, -0.7071067811865516806, -7.071067811865440820E-16 ) ) ;
#51821=EDGE_CURVE ( 'NONE', #64957, #8036, #68213, .T. ) ;
#51822=CARTESIAN_POINT ( 'NONE',  ( 112.3383795496262820, -28.20708685789894687, 289.6356252759109680 ) ) ;
#51823=VERTEX_POINT ( 'NONE', #47283 ) ;
#51824=CARTESIAN_POINT ( 'NONE',  ( 78.82227874342571283, -39.18254450372162978, 7.982620440113867843 ) ) ;
#51827=EDGE_CURVE ( 'NONE', #49032, #47693, #40275, .T. ) ;
#51828=CARTESIAN_POINT ( 'NONE',  ( 114.4788834064733862, -33.31096057238692509, 101.9880903695909780 ) ) ;
#51829=CARTESIAN_POINT ( 'NONE',  ( 104.4050232528787774, -25.97761772452189888, 236.2575300378159682 ) ) ;
#51830=CARTESIAN_POINT ( 'NONE',  ( 50.88849390559499142, -32.11662333284530746, -5.074374724088000832 ) ) ;
#51832=CARTESIAN_POINT ( 'NONE',  ( 136.4640758026458229, -38.08864647353156130, 2.654395117668909343 ) ) ;
#51833=ORIENTED_EDGE ( 'NONE', *, *, #86343, .F. ) ;
#51834=AXIS2_PLACEMENT_3D ( 'NONE', #21648, #36155, #63870 ) ;
#51835=ORIENTED_EDGE ( 'NONE', *, *, #47886, .T. ) ;
#51836=LINE ( 'NONE', #12319, #67722 ) ;
#51838=ORIENTED_EDGE ( 'NONE', *, *, #63740, .T. ) ;
#51839=DIRECTION ( 'NONE',  ( -0.7071067811865671127, -0.7071067811865279218, -7.071067811865664660E-16 ) ) ;
#51840=CARTESIAN_POINT ( 'NONE',  ( 103.2785405023565346, -27.47463817066477532, 41.38562306036225635 ) ) ;
#51841=CARTESIAN_POINT ( 'NONE',  ( 111.9909297607753160, -29.75048171432638355, 129.0095626852189525 ) ) ;
#51842=CARTESIAN_POINT ( 'NONE',  ( 117.5565198162756104, -37.28721152219886648, 18.78419670448294809 ) ) ;
#51844=ADVANCED_FACE ( 'NONE', ( #5985 ), #89094, .F. ) ;
#51846=ORIENTED_EDGE ( 'NONE', *, *, #35315, .T. ) ;
#51848=CARTESIAN_POINT ( 'NONE',  ( 164.9667039024459996, -28.27351298637401200, -5.074374724088000832 ) ) ;
#51849=ORIENTED_EDGE ( 'NONE', *, *, #60873, .F. ) ;
#51851=ADVANCED_FACE ( 'NONE', ( #75469 ), #89546, .T. ) ;
#51852=DIRECTION ( 'NONE',  ( -0.04216478779797398074, 0.9991106698809455455, 0.000000000000000000 ) ) ;
#51853=DIRECTION ( 'NONE',  ( 0.000000000000000000, 0.000000000000000000, -1.000000000000000000 ) ) ;
#51856=VECTOR ( 'NONE', #66388, 1000.000000000000000 ) ;
#51857=CARTESIAN_POINT ( 'NONE',  ( 118.3411383306134468, -33.07924694129162901, 284.0756252759109657 ) ) ;
#51858=CARTESIAN_POINT ( 'NONE',  ( 115.9284861604400731, -31.15648700444841879, 30.27276813305396175 ) ) ;
#51862=CARTESIAN_POINT ( 'NONE',  ( 172.5664832912729878, -18.82844715994071194, 318.9256252759120116 ) ) ;
#51864=CARTESIAN_POINT ( 'NONE',  ( 139.7494832912729805, -71.52944715994142655, 352.4506252759077825 ) ) ;
#51865=CARTESIAN_POINT ( 'NONE',  ( 107.0958534276316527, -25.26768445413491904, 322.6018878585615539 ) ) ;
#51866=CARTESIAN_POINT ( 'NONE',  ( 108.3338011049130785, -46.73481928183232270, 162.6771430053029519 ) ) ;
#51868=CARTESIAN_POINT ( 'NONE',  ( 193.0371591254585724, -47.82818131005411999, 129.9678068554150343 ) ) ;
#51869=CARTESIAN_POINT ( 'NONE',  ( 111.3412100197261765, -27.17259740239810739, 24.74133956162494030 ) ) ;
#51870=CARTESIAN_POINT ( 'NONE',  ( 111.4172602844868862, -47.75239391268459599, 168.8756252759109486 ) ) ;
#51871=CARTESIAN_POINT ( 'NONE',  ( 117.5094244910773114, -37.01621876064744754, 39.80419670448193159 ) ) ;
#51873=FACE_OUTER_BOUND ( 'NONE', #51271, .T. ) ;
#51874=CARTESIAN_POINT ( 'NONE',  ( 116.7951252716678425, -39.38782978912111332, 48.61479194265253057 ) ) ;
#51875=CARTESIAN_POINT ( 'NONE',  ( 82.60038231476902126, -35.66080131299400335, 2.811527311783414973 ) ) ;
#51876=VECTOR ( 'NONE', #18511, 1000.000000000000000 ) ;
#51877=ORIENTED_EDGE ( 'NONE', *, *, #80695, .T. ) ;
#51878=CARTESIAN_POINT ( 'NONE',  ( 134.0664832912739826, -9.029447159941003775, 4.925625275910997303 ) ) ;
#51880=CARTESIAN_POINT ( 'NONE',  ( 101.4370486012140589, -28.02035706366318379, 66.54514908543396245 ) ) ;
#51883=CARTESIAN_POINT ( 'NONE',  ( 96.21411768969888101, -32.03111041547180804, 207.0013395616249738 ) ) ;
#51884=DIRECTION ( 'NONE',  ( 0.000000000000000000, -1.000000000000000000, 0.000000000000000000 ) ) ;
#51885=FACE_OUTER_BOUND ( 'NONE', #88837, .T. ) ;
#51887=DIRECTION ( 'NONE',  ( 0.000000000000000000, 1.000000000000000000, 0.000000000000000000 ) ) ;
#51889=CARTESIAN_POINT ( 'NONE',  ( 97.86670531118147665, -40.64952528798283993, 96.64701509883359165 ) ) ;
#51890=CARTESIAN_POINT ( 'NONE',  ( 116.9310496459150244, -33.53114825773879915, 134.0880062282919880 ) ) ;
#51893=EDGE_LOOP ( 'NONE', ( #36333, #86207 ) ) ;
#51894=CIRCLE ( 'NONE', #44648, 2.750000000000002665 ) ;
#51895=CARTESIAN_POINT ( 'NONE',  ( 99.44206372185087162, -32.21319818083724584, 82.33301187732594428 ) ) ;
#51896=DIRECTION ( 'NONE',  ( -1.000000000000000000, -3.360405532702990443E-14, 0.000000000000000000 ) ) ;
#51898=CARTESIAN_POINT ( 'NONE',  ( 112.1213531720969883, -45.14146623880446185, 234.0070538473389377 ) ) ;
#51901=FACE_OUTER_BOUND ( 'NONE', #32496, .T. ) ;
#51904=EDGE_CURVE ( 'NONE', #62846, #78275, #62269, .T. ) ;
#51906=DIRECTION ( 'NONE',  ( 0.000000000000000000, 1.000000000000000000, 0.000000000000000000 ) ) ;
#51907=DIRECTION ( 'NONE',  ( -0.7071067708032388044, -0.0001211784769776682566, -0.7071067811865423547 ) ) ;
#51908=CARTESIAN_POINT ( 'NONE',  ( 96.69266148864264210, -35.94780844399461017, 146.2670538473399517 ) ) ;
#51912=EDGE_CURVE ( 'NONE', #5603, #34522, #15116, .T. ) ;
#51914=CARTESIAN_POINT ( 'NONE',  ( 99.09570913538954073, -30.55043167795444248, 151.8022919350126756 ) ) ;
#51916=CARTESIAN_POINT ( 'NONE',  ( 101.9931138818980259, -45.44578100715379776, 103.1564127035998695 ) ) ;
#51917=EDGE_CURVE ( 'NONE', #39822, #6347, #43161, .T. ) ;
#51920=EDGE_CURVE ( 'NONE', #5997, #55129, #57238, .T. ) ;
#51921=CARTESIAN_POINT ( 'NONE',  ( 101.9844316336549070, -45.87267731258258152, 187.1727681330539781 ) ) ;
#51922=CARTESIAN_POINT ( 'NONE',  ( 135.7779513194176957, -38.88977919476615597, 7.751962620083525657 ) ) ;
#51925=ORIENTED_EDGE ( 'NONE', *, *, #65282, .F. ) ;
#51926=CARTESIAN_POINT ( 'NONE',  ( 100.9418374907563276, -44.69577378954579672, 63.05520604563989906 ) ) ;
#51928=LINE ( 'NONE', #64261, #49822 ) ;
#51929=EDGE_CURVE ( 'NONE', #41258, #75328, #16016, .T. ) ;
#51930=CARTESIAN_POINT ( 'NONE',  ( 111.0677264286952521, -45.23305914580045339, 284.3463452106589102 ) ) ;
#51933=ORIENTED_EDGE ( 'NONE', *, *, #39232, .T. ) ;
#51936=CARTESIAN_POINT ( 'NONE',  ( 116.1871362286084235, -39.57816415692806089, 9.635625275910941312 ) ) ;
#51937=CARTESIAN_POINT ( 'NONE',  ( 82.79786375350293781, -18.40984252624906858, 6.777538624683209889 ) ) ;
#51938=VERTEX_POINT ( 'NONE', #13677 ) ;
#51939=EDGE_LOOP ( 'NONE', ( #9366, #16114, #36092, #40541 ) ) ;
#51941=ORIENTED_EDGE ( 'NONE', *, *, #88960, .T. ) ;
#51942=ORIENTED_EDGE ( 'NONE', *, *, #68524, .T. ) ;
#51943=DIRECTION ( 'NONE',  ( 1.000000000000000078E-15, -1.000000000000000083E-30, -1.000000000000000000 ) ) ;
#51944=CIRCLE ( 'NONE', #54866, 13.16666666666670160 ) ;
#51945=CARTESIAN_POINT ( 'NONE',  ( 101.6581149080599573, -43.36298066831790265, 11.45527697093296027 ) ) ;
#51946=CARTESIAN_POINT ( 'NONE',  ( 116.8159443494545826, -40.58124828358739222, 193.5270538473389479 ) ) ;
#51947=CARTESIAN_POINT ( 'NONE',  ( 96.62907006607237292, -36.88702529232764249, 136.3384824187679385 ) ) ;
#51949=CARTESIAN_POINT ( 'NONE',  ( 110.8167803534805813, -26.33188723323253910, 245.7889586092439629 ) ) ;
#51950=CYLINDRICAL_SURFACE ( 'NONE', #54263, 2.117000000000007987 ) ;
#51953=EDGE_CURVE ( 'NONE', #51387, #29395, #10448, .T. ) ;
#51954=VERTEX_POINT ( 'NONE', #4074 ) ;
#51956=VECTOR ( 'NONE', #53133, 1000.000000000000000 ) ;
#51957=CIRCLE ( 'NONE', #17184, 29.00000000000000000 ) ;
#51958=CARTESIAN_POINT ( 'NONE',  ( 110.7116931949060614, -48.05822654157750407, 207.8241967044819489 ) ) ;
#51959=VERTEX_POINT ( 'NONE', #31775 ) ;
#51960=CARTESIAN_POINT ( 'NONE',  ( 102.0509295376110117, -46.57948817496540528, 172.2137205140059564 ) ) ;
#51961=CARTESIAN_POINT ( 'NONE',  ( 113.2442291481513053, -28.75770190615245170, 264.5523025444954897 ) ) ;
#51966=CARTESIAN_POINT ( 'NONE',  ( 25.56670390244797275, -62.87844715994099687, 173.2178068554149775 ) ) ;
#51967=CARTESIAN_POINT ( 'NONE',  ( 111.4711666614668673, -26.61707918639095993, 280.7375300378156453 ) ) ;
#51970=PLANE ( 'NONE',  #6350 ) ;
#51971=DIRECTION ( 'NONE',  ( -0.7071067811855900054, -0.7071067811875051401, 0.000000000000000000 ) ) ;
#51972=CARTESIAN_POINT ( 'NONE',  ( 162.8595971212720031, -23.19206098994090581, -5.074374724088000832 ) ) ;
#51973=CARTESIAN_POINT ( 'NONE',  ( 127.0664832912738405, -46.72944715994102438, -4.970821333495669236 ) ) ;
#51974=CARTESIAN_POINT ( 'NONE',  ( 108.0557358071366423, -44.68002202782491139, 195.5838068554168103 ) ) ;
#51975=ORIENTED_EDGE ( 'NONE', *, *, #71848, .F. ) ;
#51977=CARTESIAN_POINT ( 'NONE',  ( 135.5597725514459171, -21.04085022828651930, 7.869587501222441439 ) ) ;
#51978=CARTESIAN_POINT ( 'NONE',  ( 117.0895389762686136, -39.67643183956238317, 183.5984824187679578 ) ) ;
#51979=CARTESIAN_POINT ( 'NONE',  ( 96.08760325403525826, -38.00935872415581684, 82.43086337114895912 ) ) ;
#51980=CARTESIAN_POINT ( 'NONE',  ( 96.09249528944252461, -35.06539016137039511, 217.1946728949589840 ) ) ;
#51981=PLANE ( 'NONE',  #47450 ) ;
#51982=FACE_OUTER_BOUND ( 'NONE', #62170, .T. ) ;
#51983=FACE_OUTER_BOUND ( 'NONE', #86625, .T. ) ;
#51984=CARTESIAN_POINT ( 'NONE',  ( 117.0243171429062556, -35.72162122982938826, 39.90646649224381548 ) ) ;
#51987=CARTESIAN_POINT ( 'NONE',  ( 116.3283240494693160, -32.94276334974209419, 64.13562527591099638 ) ) ;
#51989=VERTEX_POINT ( 'NONE', #64524 ) ;
#51990=ORIENTED_EDGE ( 'NONE', *, *, #17537, .F. ) ;
#51991=CARTESIAN_POINT ( 'NONE',  ( 115.3391490808644875, -34.60362203641794565, 123.4495626852199734 ) ) ;
#51994=VERTEX_POINT ( 'NONE', #38151 ) ;
#51995=CARTESIAN_POINT ( 'NONE',  ( 117.3497117099303892, -32.73958051198275854, 90.10895860924395606 ) ) ;
#51996=CARTESIAN_POINT ( 'NONE',  ( 62.03742497533659872, -23.42844715994041493, 129.9678068554150911 ) ) ;
#51998=CARTESIAN_POINT ( 'NONE',  ( 77.58678459498788982, -17.53883969337279680, 7.103318745423876202 ) ) ;
#51999=LINE ( 'NONE', #31130, #5576 ) ;
#52000=VECTOR ( 'NONE', #50771, 1000.000000000000000 ) ;
#52001=CARTESIAN_POINT ( 'NONE',  ( 116.8666057829012033, -37.25052826422871277, 18.78419670448294809 ) ) ;
#52002=VERTEX_POINT ( 'NONE', #24087 ) ;
#52005=ORIENTED_EDGE ( 'NONE', *, *, #62910, .F. ) ;
#52008=CARTESIAN_POINT ( 'NONE',  ( 105.7995184923274792, -26.72403496536887246, 116.1772919422014070 ) ) ;
#52009=LINE ( 'NONE', #58401, #42609 ) ;
#52010=LINE ( 'NONE', #79770, #55008 ) ;
#52011=EDGE_CURVE ( 'NONE', #26172, #31238, #54832, .T. ) ;
#52012=CARTESIAN_POINT ( 'NONE',  ( 100.9550256842345703, -28.70674946826466467, 51.59535640286041058 ) ) ;
#52013=ADVANCED_FACE ( 'NONE', ( #10886 ), #79055, .T. ) ;
#52016=ADVANCED_FACE ( 'NONE', ( #71789 ), #45390, .F. ) ;
#52018=CARTESIAN_POINT ( 'NONE',  ( 101.9712125536870957, -27.65933791914790874, 60.48419670448296159 ) ) ;
#52019=EDGE_LOOP ( 'NONE', ( #84079, #79411 ) ) ;
#52021=EDGE_CURVE ( 'NONE', #39595, #73742, #1200, .T. ) ;
#52025=CARTESIAN_POINT ( 'NONE',  ( 115.4543170047500098, -34.59750657913997429, 166.8547570362579506 ) ) ;
#52027=EDGE_CURVE ( 'NONE', #79315, #50547, #66456, .T. ) ;
#52029=CARTESIAN_POINT ( 'NONE',  ( 87.06648329127403940, -54.72944906728955061, -4.824374724089049771 ) ) ;
#52030=ORIENTED_EDGE ( 'NONE', *, *, #35, .T. ) ;
#52032=DIRECTION ( 'NONE',  ( 1.000000000000000000, 4.299999999999999979E-14, 1.000000000000000078E-15 ) ) ;
#52033=EDGE_LOOP ( 'NONE', ( #72028, #76432, #28337, #66149 ) ) ;
#52034=ORIENTED_EDGE ( 'NONE', *, *, #39717, .F. ) ;
#52035=CARTESIAN_POINT ( 'NONE',  ( 107.0664832912739968, -36.72944715994100306, 287.6356252759109680 ) ) ;
#52036=EDGE_CURVE ( 'NONE', #8519, #3245, #3626, .T. ) ;
#52037=CARTESIAN_POINT ( 'NONE',  ( 97.58318307924886881, -33.33272491023742390, 172.4844404487539578 ) ) ;
#52038=AXIS2_PLACEMENT_3D ( 'NONE', #55091, #82852, #76014 ) ;
#52040=CARTESIAN_POINT ( 'NONE',  ( 32.06670390244800473, -33.35206098992711077, 342.9256252759119548 ) ) ;
#52042=EDGE_LOOP ( 'NONE', ( #14350, #82025, #61116 ) ) ;
#52045=CARTESIAN_POINT ( 'NONE',  ( 109.4710126485015280, -28.41565358443893174, 212.6585665600669870 ) ) ;
#52047=CARTESIAN_POINT ( 'NONE',  ( 117.3857798876165788, -38.35993227889734669, 113.7013395616249767 ) ) ;
#52048=CARTESIAN_POINT ( 'NONE',  ( 115.7104945841387718, -43.58108136993647719, 48.30514908543492680 ) ) ;
#52049=CARTESIAN_POINT ( 'NONE',  ( 100.8867414696376272, -44.69961926644128170, 252.0525101340111860 ) ) ;
#52050=DIRECTION ( 'NONE',  ( 0.9068632946707755327, -0.4214249218767993077, 0.000000000000000000 ) ) ;
#52051=CARTESIAN_POINT ( 'NONE',  ( 131.0667039024480971, -58.72944715994092491, 207.5838068554170377 ) ) ;
#52052=CARTESIAN_POINT ( 'NONE',  ( 117.7791004155048853, -34.00661502546044801, 165.0365776568629315 ) ) ;
#52054=VERTEX_POINT ( 'NONE', #2304 ) ;
#52056=LINE ( 'NONE', #17570, #71414 ) ;
#52057=ORIENTED_EDGE ( 'NONE', *, *, #51452, .T. ) ;
#52058=ORIENTED_EDGE ( 'NONE', *, *, #85735, .F. ) ;
#52059=AXIS2_PLACEMENT_3D ( 'NONE', #18823, #74240, #39699 ) ;
#52061=CARTESIAN_POINT ( 'NONE',  ( 22.49541547940750519, -78.44951497180814215, 342.9256252759109884 ) ) ;
#52062=EDGE_CURVE ( 'NONE', #74183, #70165, #69396, .T. ) ;
#52063=ORIENTED_EDGE ( 'NONE', *, *, #87734, .T. ) ;
#52066=CARTESIAN_POINT ( 'NONE',  ( 99.04406183770223038, -42.84125761279484124, 176.8439586068464280 ) ) ;
#52067=CARTESIAN_POINT ( 'NONE',  ( 112.7599586733956727, -27.95389904326713904, 69.61848241876793963 ) ) ;
#52068=DIRECTION ( 'NONE',  ( 0.000000000000000000, 0.000000000000000000, 1.000000000000000000 ) ) ;
#52069=DIRECTION ( 'NONE',  ( 0.7071067811865171526, 0.7071067811865779928, 7.071067811865164719E-16 ) ) ;
#52071=CARTESIAN_POINT ( 'NONE',  ( 107.5699729851651938, -26.92841289699908458, 95.03562527591097364 ) ) ;
#52073=CARTESIAN_POINT ( 'NONE',  ( 98.39792771585426578, -29.90889243069713288, 196.8080062282919869 ) ) ;
#52074=DIRECTION ( 'NONE',  ( 0.000000000000000000, 0.000000000000000000, -1.000000000000000000 ) ) ;
#52076=ORIENTED_EDGE ( 'NONE', *, *, #76553, .F. ) ;
#52077=AXIS2_PLACEMENT_3D ( 'NONE', #29537, #15915, #24069 ) ;
#52078=DIRECTION ( 'NONE',  ( 0.000000000000000000, 0.000000000000000000, -1.000000000000000000 ) ) ;
#52080=CARTESIAN_POINT ( 'NONE',  ( 97.79672674250161890, -40.48067604376981166, 136.6328479018905284 ) ) ;
#52081=CARTESIAN_POINT ( 'NONE',  ( 107.0664832912739968, -36.72944715994100306, 277.6356252759110248 ) ) ;
#52082=EDGE_CURVE ( 'NONE', #13607, #88437, #79955, .T. ) ;
#52083=CARTESIAN_POINT ( 'NONE',  ( 97.99847537351134008, -44.43658864837386346, 226.8870538473399563 ) ) ;
#52086=CARTESIAN_POINT ( 'NONE',  ( 110.7407540106703010, -26.28028736477551419, 250.8194347997206819 ) ) ;
#52087=CARTESIAN_POINT ( 'NONE',  ( 109.2103426150987104, -26.48265019188898606, 135.9127681330539872 ) ) ;
#52088=CARTESIAN_POINT ( 'NONE',  ( 108.4212757395327174, -26.73551752249970548, 250.9740451590128316 ) ) ;
#52089=CARTESIAN_POINT ( 'NONE',  ( 81.20964327716589537, -39.23067567606557304, 8.021372095561080329 ) ) ;
#52090=DIRECTION ( 'NONE',  ( 9.073094938289460781E-13, 1.000000000000000000, 0.000000000000000000 ) ) ;
#52091=CARTESIAN_POINT ( 'NONE',  ( 101.9933639039164035, -45.44591285733346098, 263.1565428173477130 ) ) ;
#52092=ORIENTED_EDGE ( 'NONE', *, *, #80203, .F. ) ;
#52094=ORIENTED_EDGE ( 'NONE', *, *, #12315, .F. ) ;
#52095=ORIENTED_EDGE ( 'NONE', *, *, #33789, .F. ) ;
#52096=ORIENTED_EDGE ( 'NONE', *, *, #74640, .T. ) ;
#52097=PLANE ( 'NONE',  #77042 ) ;
#52098=CARTESIAN_POINT ( 'NONE',  ( 96.88896422860915436, -30.65880273170215276, 276.8984824187680829 ) ) ;
#52100=CARTESIAN_POINT ( 'NONE',  ( 51.06670390244899238, -32.29483332968430886, -5.074374724088000832 ) ) ;
#52104=CARTESIAN_POINT ( 'NONE',  ( 99.14828105993673546, -39.93229045078558670, 206.0552769709339884 ) ) ;
#52106=EDGE_LOOP ( 'NONE', ( #13618, #80648, #19422, #77906 ) ) ;
#52107=AXIS2_PLACEMENT_3D ( 'NONE', #38397, #79768, #72046 ) ;
#52108=CIRCLE ( 'NONE', #17388, 11.57110091390437034 ) ;
#52109=ORIENTED_EDGE ( 'NONE', *, *, #10521, .T. ) ;
#52110=CARTESIAN_POINT ( 'NONE',  ( 87.31648329127402519, -54.62589567669624557, 14.92562527591095112 ) ) ;
#52111=PLANE ( 'NONE',  #75294 ) ;
#52112=CARTESIAN_POINT ( 'NONE',  ( 63.31670390244797630, -58.72944715994110254, 310.9178068554150514 ) ) ;
#52114=CARTESIAN_POINT ( 'NONE',  ( 101.4092135025303776, -29.90862777007100703, 37.05872616303995670 ) ) ;
#52115=EDGE_CURVE ( 'NONE', #48663, #4991, #67898, .T. ) ;
#52117=CIRCLE ( 'NONE', #1398, 9.999999999999994671 ) ;
#52118=EDGE_CURVE ( 'NONE', #64715, #1134, #9876, .T. ) ;
#52119=LINE ( 'NONE', #72607, #85416 ) ;
#52121=DIRECTION ( 'NONE',  ( -1.000200923085726652E-15, -1.000000000000000000, 0.000000000000000000 ) ) ;
#52122=EDGE_LOOP ( 'NONE', ( #43467, #36737, #64975, #20954 ) ) ;
#52123=ADVANCED_FACE ( 'NONE', ( #18145 ), #80845, .F. ) ;
#52125=ORIENTED_EDGE ( 'NONE', *, *, #44685, .T. ) ;
#52127=CARTESIAN_POINT ( 'NONE',  ( 115.6864120445923163, -37.50259225211298286, 31.56142370292397459 ) ) ;
#52130=EDGE_CURVE ( 'NONE', #21819, #32172, #47580, .T. ) ;
#52131=AXIS2_PLACEMENT_3D ( 'NONE', #5298, #4847, #25730 ) ;
#52133=ORIENTED_EDGE ( 'NONE', *, *, #22841, .T. ) ;
#52134=DIRECTION ( 'NONE',  ( -0.7071067811865431318, 0.7071067811865517916, -7.071067811865425043E-16 ) ) ;
#52136=ORIENTED_EDGE ( 'NONE', *, *, #23831, .T. ) ;
#52137=CARTESIAN_POINT ( 'NONE',  ( 101.6781192058861762, -27.07830111727894362, 105.4937205140069665 ) ) ;
#52138=ORIENTED_EDGE ( 'NONE', *, *, #85798, .F. ) ;
#52139=CARTESIAN_POINT ( 'NONE',  ( 101.7280645633873775, -29.41412380334073973, 29.98861030426797214 ) ) ;
#52141=CARTESIAN_POINT ( 'NONE',  ( 112.5007446479794453, -45.21116328700192355, 64.46158330589696561 ) ) ;
#52143=CARTESIAN_POINT ( 'NONE',  ( 71.06648329127399677, -8.729447159940999512, 323.8756252759120002 ) ) ;
#52145=AXIS2_PLACEMENT_3D ( 'NONE', #30155, #23802, #51906 ) ;
#52146=CARTESIAN_POINT ( 'NONE',  ( 111.1374431767090414, -47.03053892029802796, 18.88800622829195319 ) ) ;
#52147=CARTESIAN_POINT ( 'NONE',  ( 162.5667039024460223, -19.82844715994111340, -5.074374724088000832 ) ) ;
#52149=CARTESIAN_POINT ( 'NONE',  ( 19.56648329127400032, -18.82844715994099971, -5.074374724088000832 ) ) ;
#52150=ORIENTED_EDGE ( 'NONE', *, *, #82033, .F. ) ;
#52151=CARTESIAN_POINT ( 'NONE',  ( 77.45242755740704865, -19.60567372264617703, 2.908038864009607316 ) ) ;
#52155=AXIS2_PLACEMENT_3D ( 'NONE', #12847, #80541, #60977 ) ;
#52156=CARTESIAN_POINT ( 'NONE',  ( 97.99937763885726838, -40.39701179870337455, 206.6327681330539860 ) ) ;
#52157=LINE ( 'NONE', #25372, #11795 ) ;
#52159=CARTESIAN_POINT ( 'NONE',  ( 110.7944688027788658, -46.46518603654068613, 58.86705384733998159 ) ) ;
#52160=LINE ( 'NONE', #23622, #47904 ) ;
#52162=DIRECTION ( 'NONE',  ( 1.000000000000000000, 4.163336342344333240E-14, 0.000000000000000000 ) ) ;
#52164=LINE ( 'NONE', #39458, #79618 ) ;
#52167=LINE ( 'NONE', #51284, #38729 ) ;
#52168=CARTESIAN_POINT ( 'NONE',  ( 105.7138707427173898, -46.72361436802630408, 113.4695631962065505 ) ) ;
#52169=CARTESIAN_POINT ( 'NONE',  ( 115.8368392028494185, -44.66223131803950963, 233.2413395616259493 ) ) ;
#52171=EDGE_CURVE ( 'NONE', #35753, #834, #88279, .T. ) ;
#52172=LINE ( 'NONE', #33101, #7121 ) ;
#52173=CARTESIAN_POINT ( 'NONE',  ( 77.67297288197859473, -38.08739819366309121, 2.653088468869586602 ) ) ;
#52174=CARTESIAN_POINT ( 'NONE',  ( 110.9972015515846238, -44.34532242709460093, 272.3781341137911909 ) ) ;
#52175=DIRECTION ( 'NONE',  ( 4.194175870806139918E-14, -1.000000000000000000, 0.000000000000000000 ) ) ;
#52176=CARTESIAN_POINT ( 'NONE',  ( 117.3173117416416744, -32.65705981835812111, 95.13943479972097350 ) ) ;
#52178=CARTESIAN_POINT ( 'NONE',  ( 102.5972826210866060, -46.89011293525640411, 132.2346728949579528 ) ) ;
#52179=EDGE_LOOP ( 'NONE', ( #32714, #11969, #30697, #88480, #4432, #64848, #26809, #60910, #25059, #5882, #19363, #3153, #10824, #32507, #7208, #80918, #52805, #5780, #15781, #74623, #21633, #59282, #51363, #28652, #85777, #81732, #43869, #19980, #88909, #83936, #26595, #25915, #78981, #65093, #17768, #50051, #24832, #46630, #32603, #61713, #66823, #68341, #60202, #25599, #38324, #637, #49890, #80422, #66291, #66186, #23028, #46244, #57451, #69236, #39681, #41845, #22462, #80332, #5163, #3776, #10980, #20223, #84019, #32342, #48159, #29633, #29107, #39563, #6028, #34716, #33596, #67729, #31604, #41024, #85380, #15105, #1878, #68091, #36432, #5982, #28964, #18716, #76698, #43586, #56296, #9979, #46329, #51157, #60441, #33859, #59856, #56262, #88298, #3705, #25548, #89560 ) ) ;
#52180=CARTESIAN_POINT ( 'NONE',  ( 132.7628207310606854, -21.15113447712359473, 7.957506268076239841 ) ) ;
#52181=ORIENTED_EDGE ( 'NONE', *, *, #60777, .F. ) ;
#52185=PLANE ( 'NONE',  #41431 ) ;
#52187=ORIENTED_EDGE ( 'NONE', *, *, #46406, .F. ) ;
#52188=CARTESIAN_POINT ( 'NONE',  ( 99.09552584949113907, -30.55066422794973136, 50.80231514688692585 ) ) ;
#52189=CARTESIAN_POINT ( 'NONE',  ( 99.02022134730059122, -43.42753157066677261, 116.8784824187679732 ) ) ;
#52190=ORIENTED_EDGE ( 'NONE', *, *, #10511, .F. ) ;
#52191=CARTESIAN_POINT ( 'NONE',  ( 25.56670390244797275, -65.37844715994100397, 293.2178068554150627 ) ) ;
#52192=AXIS2_PLACEMENT_3D ( 'NONE', #71782, #15926, #72674 ) ;
#52194=LINE ( 'NONE', #72236, #6082 ) ;
#52196=EDGE_CURVE ( 'NONE', #78219, #11954, #49076, .T. ) ;
#52197=CARTESIAN_POINT ( 'NONE',  ( 113.8708677755033847, -44.65703921284106315, 108.1413395616249744 ) ) ;
#52199=LINE ( 'NONE', #37270, #66649 ) ;
#52200=CARTESIAN_POINT ( 'NONE',  ( 167.2371591254545535, -47.82818131005522133, 129.9678068554149775 ) ) ;
#52201=DIRECTION ( 'NONE',  ( -1.000000000000000078E-15, 0.000000000000000000, -1.000000000000000000 ) ) ;
#52203=VECTOR ( 'NONE', #45157, 1000.000000000000000 ) ;
#52204=EDGE_LOOP ( 'NONE', ( #46689, #16995 ) ) ;
#52205=CARTESIAN_POINT ( 'NONE',  ( 172.5664832912729878, -27.57844715994070484, 318.9256252759120116 ) ) ;
#52206=DIRECTION ( 'NONE',  ( 0.000000000000000000, 0.000000000000000000, 1.000000000000000000 ) ) ;
#52208=CARTESIAN_POINT ( 'NONE',  ( 142.8838050580813785, -82.11588141944041297, 542.9756252759101471 ) ) ;
#52209=FACE_OUTER_BOUND ( 'NONE', #51756, .T. ) ;
#52210=LINE ( 'NONE', #65432, #47996 ) ;
#52212=ORIENTED_EDGE ( 'NONE', *, *, #74885, .F. ) ;
#52213=FACE_OUTER_BOUND ( 'NONE', #69694, .T. ) ;
#52214=CARTESIAN_POINT ( 'NONE',  ( 106.3491918589965763, -46.48387837312645132, 218.5184824187679453 ) ) ;
#52218=CIRCLE ( 'NONE', #36308, 2.517500000000005844 ) ;
#52219=CARTESIAN_POINT ( 'NONE',  ( 116.4365193811696457, -32.28633913640747011, 60.19086337114898555 ) ) ;
#52221=CARTESIAN_POINT ( 'NONE',  ( 97.83900272812365984, -40.58357929434716738, 51.64132164664623303 ) ) ;
#52224=VECTOR ( 'NONE', #85108, 1000.000000000000000 ) ;
#52225=ORIENTED_EDGE ( 'NONE', *, *, #41669, .T. ) ;
#52227=EDGE_CURVE ( 'NONE', #63620, #11064, #22198, .T. ) ;
#52228=ORIENTED_EDGE ( 'NONE', *, *, #14533, .T. ) ;
#52230=CARTESIAN_POINT ( 'NONE',  ( 98.55918112442081735, -40.71722039560211925, 208.0949166392299787 ) ) ;
#52234=DIRECTION ( 'NONE',  ( 0.7071067811874257591, -0.7071067811856692753, 2.899137802861360256E-29 ) ) ;
#52235=EDGE_CURVE ( 'NONE', #88986, #56291, #55769, .T. ) ;
#52237=VERTEX_POINT ( 'NONE', #15382 ) ;
#52238=CARTESIAN_POINT ( 'NONE',  ( 134.0664832912739826, -33.97944715994100306, 8.225625275910998013 ) ) ;
#52239=DIRECTION ( 'NONE',  ( 1.000000000000000000, 0.000000000000000000, 0.000000000000000000 ) ) ;
#52241=ORIENTED_EDGE ( 'NONE', *, *, #60023, .F. ) ;
#52242=CARTESIAN_POINT ( 'NONE',  ( 101.3840881871039272, -27.98888560156178329, 25.53562527591096654 ) ) ;
#52248=DIRECTION ( 'NONE',  ( -2.981567257902526681E-15, 0.8571673007021100021, 0.5150380749100580413 ) ) ;
#52249=CARTESIAN_POINT ( 'NONE',  ( 103.6242938494280423, -26.17725164406494542, 206.3394347997209763 ) ) ;
#52251=VERTEX_POINT ( 'NONE', #48505 ) ;
#52252=CARTESIAN_POINT ( 'NONE',  ( 99.26130681012091372, -43.75918647830361863, 52.90991099019698396 ) ) ;
#52253=DIRECTION ( 'NONE',  ( -0.7071067812160284349, 0.7071067811570665995, -7.071067812160292375E-16 ) ) ;
#52255=EDGE_LOOP ( 'NONE', ( #7614, #52310 ) ) ;
#52256=AXIS2_PLACEMENT_3D ( 'NONE', #28848, #34754, #76545 ) ;
#52257=CARTESIAN_POINT ( 'NONE',  ( 81.91153210826661279, -16.68812259376749907, 2.188418746631556999 ) ) ;
#52258=CARTESIAN_POINT ( 'NONE',  ( 90.44969454456416713, -53.34645651782494724, 219.5838068554169809 ) ) ;
#52259=CARTESIAN_POINT ( 'NONE',  ( 41.56670390244783420, -36.32844715994104234, 249.9678068554150343 ) ) ;
#52260=CARTESIAN_POINT ( 'NONE',  ( 98.22859028455410169, -39.55567757615634861, 129.3909475124479798 ) ) ;
#52261=CARTESIAN_POINT ( 'NONE',  ( 113.2328747769256410, -45.16229216617723097, 224.0784824187679476 ) ) ;
#52264=CARTESIAN_POINT ( 'NONE',  ( 136.8165183345649041, -36.90056224777460159, 3.101534470964323553 ) ) ;
#52266=EDGE_CURVE ( 'NONE', #28614, #84277, #49867, .T. ) ;
#52267=ORIENTED_EDGE ( 'NONE', *, *, #32866, .F. ) ;
#52268=VERTEX_POINT ( 'NONE', #1297 ) ;
#52269=FACE_OUTER_BOUND ( 'NONE', #4394, .T. ) ;
#52270=ORIENTED_EDGE ( 'NONE', *, *, #75210, .F. ) ;
#52272=LINE ( 'NONE', #73189, #39604 ) ;
#52275=DIRECTION ( 'NONE',  ( -1.000000000000000078E-15, -9.367723249499513438E-31, 1.000000000000000000 ) ) ;
#52276=CARTESIAN_POINT ( 'NONE',  ( 115.3767887321059789, -38.82490071601502990, 123.0524198280769639 ) ) ;
#52277=CARTESIAN_POINT ( 'NONE',  ( 115.9290394997688480, -31.15613903141374763, 34.27276813305396530 ) ) ;
#52283=DIRECTION ( 'NONE',  ( 0.7071067811575828532, -0.7071067812155121812, 0.000000000000000000 ) ) ;
#52285=CARTESIAN_POINT ( 'NONE',  ( 97.80162807463898389, -40.49275734879226718, 167.6337774318473350 ) ) ;
#52287=DIRECTION ( 'NONE',  ( 1.000000000000000000, 0.000000000000000000, 0.000000000000000000 ) ) ;
#52288=CONICAL_SURFACE ( 'NONE', #81408, 1.258750000000002922, 1.029744258676650093 ) ;
#52289=CARTESIAN_POINT ( 'NONE',  ( 89.33314995793998037, 12.92155284005730387, 355.9756252759109998 ) ) ;
#52290=EDGE_LOOP ( 'NONE', ( #75873, #48869, #47548, #82059, #59705, #56655, #19006, #43776 ) ) ;
#52291=EDGE_CURVE ( 'NONE', #65644, #18741, #78950, .T. ) ;
#52292=CARTESIAN_POINT ( 'NONE',  ( 111.7737306318703361, -46.73355046572731908, 287.9146728949587555 ) ) ;
#52293=CARTESIAN_POINT ( 'NONE',  ( 117.4276745381585556, -38.22567431247780689, 24.71276813305395237 ) ) ;
#52294=CARTESIAN_POINT ( 'NONE',  ( 107.0664832912739399, -36.72944715994095333, 302.4856252759109907 ) ) ;
#52296=DIRECTION ( 'NONE',  ( 4.299999999999999979E-14, -1.000000000000000000, 0.000000000000000000 ) ) ;
#52297=CARTESIAN_POINT ( 'NONE',  ( 132.8827458516741160, -39.21170328187210430, 8.006085407568425794 ) ) ;
#52298=AXIS2_PLACEMENT_3D ( 'NONE', #88410, #32515, #47486 ) ;
#52299=CARTESIAN_POINT ( 'NONE',  ( 116.3212776292296127, -32.94146857471318413, 287.6356252759109680 ) ) ;
#52300=FACE_OUTER_BOUND ( 'NONE', #4657, .T. ) ;
#52303=CARTESIAN_POINT ( 'NONE',  ( 101.3600985487617692, -27.95198515609010315, 25.53562527591096654 ) ) ;
#52304=CARTESIAN_POINT ( 'NONE',  ( 102.2372498927960720, -45.96854842739928415, 208.1927681330539599 ) ) ;
#52305=CARTESIAN_POINT ( 'NONE',  ( 98.70509129169590778, -42.99238438483101987, 62.83848241876793850 ) ) ;
#52306=DIRECTION ( 'NONE',  ( 1.000000000000000078E-15, -1.000000000000000083E-30, -1.000000000000000000 ) ) ;
#52307=CARTESIAN_POINT ( 'NONE',  ( 107.0664832912730020, -36.72944715994189835, 342.9256252759119548 ) ) ;
#52308=FACE_OUTER_BOUND ( 'NONE', #30637, .T. ) ;
#52310=ORIENTED_EDGE ( 'NONE', *, *, #1334, .T. ) ;
#52311=CARTESIAN_POINT ( 'NONE',  ( 90.44969454456405344, -22.62993780205708916, 219.5838068554169809 ) ) ;
#52312=ORIENTED_EDGE ( 'NONE', *, *, #973, .F. ) ;
#52313=AXIS2_PLACEMENT_3D ( 'NONE', #1485, #58227, #64599 ) ;
#52314=CARTESIAN_POINT ( 'NONE',  ( 113.1080853710607528, -29.03773216254920797, 75.54705384733895812 ) ) ;
#52317=VECTOR ( 'NONE', #16839, 999.9999999999998863 ) ;
#52318=CARTESIAN_POINT ( 'NONE',  ( 172.5667039024480687, -36.32844715993499563, 129.9678068554150059 ) ) ;
#52319=CARTESIAN_POINT ( 'NONE',  ( 100.6510976905702393, -26.79511100149722935, 216.5327681330539633 ) ) ;
#52320=CARTESIAN_POINT ( 'NONE',  ( 41.56648329127499153, -36.32844715994070839, 318.9256252759120116 ) ) ;
#52321=CARTESIAN_POINT ( 'NONE',  ( 97.81218034145919660, -40.51862630628952644, 146.6357281275130902 ) ) ;
#52322=DIRECTION ( 'NONE',  ( -1.000000000000000000, -4.299999999999999979E-14, -1.000000000000000078E-15 ) ) ;
#52324=EDGE_CURVE ( 'NONE', #19093, #24119, #9016, .T. ) ;
#52325=LINE ( 'NONE', #58714, #54460 ) ;
#52326=CARTESIAN_POINT ( 'NONE',  ( 132.6459363690134978, -39.09121833381820466, 1.942446336661487027 ) ) ;
#52328=CARTESIAN_POINT ( 'NONE',  ( 107.6167445103326230, -46.48501816386551866, 152.6213395616259731 ) ) ;
#52331=ORIENTED_EDGE ( 'NONE', *, *, #18209, .F. ) ;
#52332=CARTESIAN_POINT ( 'NONE',  ( 117.0765951205083439, -35.60322954364740156, 80.34729759161096752 ) ) ;
#52333=AXIS2_PLACEMENT_3D ( 'NONE', #16445, #85510, #56866 ) ;
#52335=CARTESIAN_POINT ( 'NONE',  ( 112.8396959964675972, -44.62460075896464673, 224.0784824187679476 ) ) ;
#52341=CARTESIAN_POINT ( 'NONE',  ( 34.96670390244699433, -28.27351298637401200, -5.074374724088000832 ) ) ;
#52344=EDGE_CURVE ( 'NONE', #29169, #73752, #70833, .T. ) ;
#52345=CARTESIAN_POINT ( 'NONE',  ( 96.67182511810079859, -37.15340426533111895, 161.3584824187679487 ) ) ;
#52346=ORIENTED_EDGE ( 'NONE', *, *, #34011, .F. ) ;
#52348=EDGE_CURVE ( 'NONE', #62712, #73560, #43949, .T. ) ;
#52352=ADVANCED_FACE ( 'NONE', ( #86650 ), #17606, .T. ) ;
#52353=CARTESIAN_POINT ( 'NONE',  ( 51.03742451361238608, -23.42844715994066362, 313.9678068554150059 ) ) ;
#52356=FACE_OUTER_BOUND ( 'NONE', #79047, .T. ) ;
#52357=CARTESIAN_POINT ( 'NONE',  ( 109.4453579932576872, -25.93500217162640453, 179.8918157521019339 ) ) ;
#52358=LINE ( 'NONE', #38314, #926 ) ;
#52360=VERTEX_POINT ( 'NONE', #57129 ) ;
#52361=VERTEX_POINT ( 'NONE', #15824 ) ;
#52362=AXIS2_PLACEMENT_3D ( 'NONE', #5526, #61801, #34998 ) ;
#52364=DIRECTION ( 'NONE',  ( 0.08544974978095713769, 0.9963424814100680926, -0.000000000000000000 ) ) ;
#52365=CARTESIAN_POINT ( 'NONE',  ( 108.3327054655748469, -46.73494365500790337, 163.6772328748223231 ) ) ;
#52366=VECTOR ( 'NONE', #79834, 1000.000000000000000 ) ;
#52367=CARTESIAN_POINT ( 'NONE',  ( 99.81817287040931319, -30.93652672145504567, 43.60809036959195595 ) ) ;
#52368=DIRECTION ( 'NONE',  ( 1.000000000000000000, 4.163336342344333240E-14, 0.000000000000000000 ) ) ;
#52369=ORIENTED_EDGE ( 'NONE', *, *, #73667, .F. ) ;
#52370=CARTESIAN_POINT ( 'NONE',  ( 194.0371591254572650, -24.42818131005417825, 313.9678068554149490 ) ) ;
#52371=CARTESIAN_POINT ( 'NONE',  ( 82.60054997757899287, -17.66120003907535363, 7.039521718172035314 ) ) ;
#52372=ORIENTED_EDGE ( 'NONE', *, *, #7597, .T. ) ;
#52373=EDGE_LOOP ( 'NONE', ( #70320, #62966, #6175 ) ) ;
#52375=ORIENTED_EDGE ( 'NONE', *, *, #24377, .T. ) ;
#52376=ORIENTED_EDGE ( 'NONE', *, *, #77339, .F. ) ;
#52377=DIRECTION ( 'NONE',  ( 0.000000000000000000, 1.000000000000000000, 0.000000000000000000 ) ) ;
#52379=CARTESIAN_POINT ( 'NONE',  ( 114.9815630121539272, -32.32897180620768296, 28.66480078045796631 ) ) ;
#52380=CARTESIAN_POINT ( 'NONE',  ( 114.8305014334234642, -29.68612513766509053, 209.4127681330539872 ) ) ;
#52382=CARTESIAN_POINT ( 'NONE',  ( 103.5497706991576905, -26.90106182813401503, 190.3499109901969746 ) ) ;
#52383=DIRECTION ( 'NONE',  ( 0.7071067811865171526, 0.7071067811865779928, 7.071067811865164719E-16 ) ) ;
#52384=CARTESIAN_POINT ( 'NONE',  ( 103.9393079366161032, -26.78443525705497663, 246.3184824187679567 ) ) ;
#52387=ORIENTED_EDGE ( 'NONE', *, *, #298, .F. ) ;
#52388=ORIENTED_EDGE ( 'NONE', *, *, #26504, .F. ) ;
#52390=CARTESIAN_POINT ( 'NONE',  ( 97.88046564956832185, -41.75177191353013484, 221.7241967044819546 ) ) ;
#52391=ORIENTED_EDGE ( 'NONE', *, *, #32299, .F. ) ;
#52392=EDGE_CURVE ( 'NONE', #6148, #84235, #16090, .T. ) ;
#52393=CARTESIAN_POINT ( 'NONE',  ( 108.9452245070828411, -26.43885738637160543, 164.9327681330529742 ) ) ;
#52394=CARTESIAN_POINT ( 'NONE',  ( 99.09532346180453999, -30.55094594714533329, 265.8023343502491684 ) ) ;
#52395=DIRECTION ( 'NONE',  ( 0.9068632946707755327, -0.4214249218767993077, 0.000000000000000000 ) ) ;
#52396=CARTESIAN_POINT ( 'NONE',  ( 188.5667039024484097, -48.82844715993431350, 254.7178068554150059 ) ) ;
#52398=ADVANCED_FACE ( 'NONE', ( #64414 ), #25747, .T. ) ;
#52399=LINE ( 'NONE', #45159, #57837 ) ;
#52400=DIRECTION ( 'NONE',  ( 0.000000000000000000, 0.000000000000000000, -1.000000000000000000 ) ) ;
#52401=CARTESIAN_POINT ( 'NONE',  ( 96.99990081654259200, -39.35482002063352525, 272.5299109901966972 ) ) ;
#52402=LINE ( 'NONE', #30224, #80045 ) ;
#52405=ADVANCED_FACE ( 'NONE', ( #59366 ), #57778, .T. ) ;
#52406=PLANE ( 'NONE',  #64587 ) ;
#52409=CARTESIAN_POINT ( 'NONE',  ( 97.33784131552974372, -34.07106451407344139, 77.11479194128529002 ) ) ;
#52410=CIRCLE ( 'NONE', #13296, 1.000000000000000888 ) ;
#52411=CARTESIAN_POINT ( 'NONE',  ( 115.5168658168125830, -36.45974858580882483, 195.5838068554167819 ) ) ;
#52414=LINE ( 'NONE', #31105, #42266 ) ;
#52415=CARTESIAN_POINT ( 'NONE',  ( 98.51948014227190242, -30.72152729218522538, 205.8384824187679669 ) ) ;
#52416=CARTESIAN_POINT ( 'NONE',  ( 118.9036788419121962, -36.16782713317093112, 114.8641967044819694 ) ) ;
#52417=CARTESIAN_POINT ( 'NONE',  ( 115.4949314580552624, -29.50734498268579387, 225.4022919425769658 ) ) ;
#52418=FACE_OUTER_BOUND ( 'NONE', #38421, .T. ) ;
#52419=CARTESIAN_POINT ( 'NONE',  ( 31.89136050872298966, -31.76306994223740432, -5.074374724088000832 ) ) ;
#52420=CARTESIAN_POINT ( 'NONE',  ( 162.5667039024470171, -32.29483332968611364, -5.074374724088000832 ) ) ;
#52421=CARTESIAN_POINT ( 'NONE',  ( 98.52126951539199240, -41.93296859720368985, 37.76142964116910861 ) ) ;
#52422=LINE ( 'NONE', #78852, #47925 ) ;
#52423=DIRECTION ( 'NONE',  ( -1.000000000000000000, -4.237773401492740281E-14, 0.000000000000000000 ) ) ;
#52424=AXIS2_PLACEMENT_3D ( 'NONE', #86545, #80178, #85659 ) ;
#52425=ADVANCED_FACE ( 'NONE', ( #12126 ), #67086, .F. ) ;
#52426=CARTESIAN_POINT ( 'NONE',  ( 172.5664832912740110, -36.32844715994070839, 258.9256252759120116 ) ) ;
#52428=ADVANCED_FACE ( 'NONE', ( #59805 ), #87539, .T. ) ;
#52429=VERTEX_POINT ( 'NONE', #31669 ) ;
#52430=VERTEX_POINT ( 'NONE', #12580 ) ;
#52431=CARTESIAN_POINT ( 'NONE',  ( 116.7648798213666623, -36.26930322673007367, 118.2867055423629807 ) ) ;
#52434=CARTESIAN_POINT ( 'NONE',  ( 116.5783909117431136, -29.70293872869714846, 105.3327681330539463 ) ) ;
#52437=AXIS2_PLACEMENT_3D ( 'NONE', #50651, #2073, #84314 ) ;
#52438=EDGE_CURVE ( 'NONE', #65413, #57074, #53876, .T. ) ;
#52439=CARTESIAN_POINT ( 'NONE',  ( 79.18623681048846663, -16.12360705087681367, 8.106403045240202943 ) ) ;
#52440=CARTESIAN_POINT ( 'NONE',  ( 76.06670390244796920, -26.72944715994109899, 239.5838068554169809 ) ) ;
#52441=CARTESIAN_POINT ( 'NONE',  ( 99.04406186382159660, -42.84125764666617897, 107.8439586099191700 ) ) ;
#52442=CARTESIAN_POINT ( 'NONE',  ( 99.63325261332695959, -43.08637385293071986, 31.88991099019694531 ) ) ;
#52443=VERTEX_POINT ( 'NONE', #5768 ) ;
#52447=CARTESIAN_POINT ( 'NONE',  ( 108.8662857618680846, -46.94215964495589333, 118.7032443235299723 ) ) ;
#52448=CARTESIAN_POINT ( 'NONE',  ( 63.56670390244824631, -47.82844715994016127, 300.4678068554150627 ) ) ;
#52449=CARTESIAN_POINT ( 'NONE',  ( 31.56670390244720892, -33.35206098992784263, 193.9678068554150911 ) ) ;
#52451=DIRECTION ( 'NONE',  ( 1.000000000000000000, 0.000000000000000000, -0.000000000000000000 ) ) ;
#52453=ADVANCED_FACE ( 'NONE', ( #40267, #25299 ), #33459, .T. ) ;
#52456=B_SPLINE_CURVE_WITH_KNOTS ( 'NONE', 3,
 ( #87168, #10853, #51722, #66247, #88063, #73975, #80807, #59875, #72646, #18557, #10412, #39890, #5386, #11295, #3595, #58981, #11754, #4039, #38115, #59437, #87608, #39452, #46240, #67153, #31740, #25828, #86275, #4935, #38998, #24934, #24054, #52598, #4494, #53497, #65807, #80359 ),
 .UNSPECIFIED., .F., .F.,
 ( 4, 2, 2, 2, 2, 2, 2, 2, 2, 2, 2, 2, 2, 2, 1, 1, 1, 1, 2, 4 ),
 ( 0.000000000000000000, 0.06249359649563903524, 0.1249871929912780705, 0.1874807894869170988, 0.2499743859825561410, 0.2812211842303752873, 0.3124679824781944060, 0.3437147807260135246, 0.3749615789738326432, 0.4062083772216517619, 0.4374551754694708805, 0.4687019737172900546, 0.4843253728411998082, 0.4921370724031547961, 0.4960429221841324288, 0.4979958470746210786, 0.4989723095198653202, 0.4994605407424874133, 0.4997046563537985708, 0.4999487719651097284 ),
 .UNSPECIFIED. ) ;
#52458=CARTESIAN_POINT ( 'NONE',  ( 103.6060256796756534, -46.54035428658124118, 57.30705384733997221 ) ) ;
#52459=VERTEX_POINT ( 'NONE', #75256 ) ;
#52460=ORIENTED_EDGE ( 'NONE', *, *, #68923, .T. ) ;
#52462=CARTESIAN_POINT ( 'NONE',  ( 97.95250717983367394, -32.49412669507731266, 6.826283056785781511 ) ) ;
#52464=EDGE_CURVE ( 'NONE', #21130, #28780, #34366, .T. ) ;
#52466=CARTESIAN_POINT ( 'NONE',  ( 112.3727512366848487, -30.49036002617200936, 137.3338046553059826 ) ) ;
#52467=VECTOR ( 'NONE', #43361, 1000.000000000000000 ) ;
#52468=LINE ( 'NONE', #41990, #18489 ) ;
#52470=ORIENTED_EDGE ( 'NONE', *, *, #70006, .F. ) ;
#52471=LINE ( 'NONE', #79792, #25008 ) ;
#52474=CYLINDRICAL_SURFACE ( 'NONE', #89836, 9.999999999999998224 ) ;
#52475=AXIS2_PLACEMENT_3D ( 'NONE', #773, #42538, #83449 ) ;
#52476=CARTESIAN_POINT ( 'NONE',  ( 104.0709181822855243, -28.35754658334662182, 186.7815833058969872 ) ) ;
#52477=CYLINDRICAL_SURFACE ( 'NONE', #39979, 0.4999999999999933387 ) ;
#52479=AXIS2_PLACEMENT_3D ( 'NONE', #35359, #41717, #54888 ) ;
#52481=ORIENTED_EDGE ( 'NONE', *, *, #61804, .F. ) ;
#52482=VERTEX_POINT ( 'NONE', #11223 ) ;
#52483=VECTOR ( 'NONE', #30313, 1000.000000000000000 ) ;
#52486=CARTESIAN_POINT ( 'NONE',  ( 115.0224139972512063, -40.13592505470528238, 211.3347570362579404 ) ) ;
#52487=CARTESIAN_POINT ( 'NONE',  ( 99.03713458771083822, -43.41345219906346387, 116.8784824187679732 ) ) ;
#52488=CARTESIAN_POINT ( 'NONE',  ( 116.2124334422530865, -31.77159869865914388, 69.22133956162495849 ) ) ;
#52490=DIRECTION ( 'NONE',  ( 0.9068632946707808618, -0.4214249218767877059, 0.000000000000000000 ) ) ;
#52492=CARTESIAN_POINT ( 'NONE',  ( 102.9134293080737450, -27.12924067693381502, 151.4013395616249511 ) ) ;
#52493=CIRCLE ( 'NONE', #74266, 2.999999999999947153 ) ;
#52495=ORIENTED_EDGE ( 'NONE', *, *, #1328, .F. ) ;
#52498=ORIENTED_EDGE ( 'NONE', *, *, #87045, .F. ) ;
#52501=ORIENTED_EDGE ( 'NONE', *, *, #11642, .T. ) ;
#52502=CARTESIAN_POINT ( 'NONE',  ( 49.21437657594911741, -35.91149509761154945, 193.9678068554150911 ) ) ;
#52504=CARTESIAN_POINT ( 'NONE',  ( 99.82429199452421642, -29.71057280230317232, 131.7142967403817124 ) ) ;
#52505=CARTESIAN_POINT ( 'NONE',  ( 116.2317802277880787, -31.76111116818806224, 69.22133956162495849 ) ) ;
#52508=CARTESIAN_POINT ( 'NONE',  ( 165.9667039024475059, -28.27351298636806831, 237.4678068554150059 ) ) ;
#52509=FACE_OUTER_BOUND ( 'NONE', #57448, .T. ) ;
#52510=EDGE_CURVE ( 'NONE', #27981, #57293, #24757, .T. ) ;
#52511=CARTESIAN_POINT ( 'NONE',  ( 112.9545114599701918, -28.19305977888944525, 89.60800622829296458 ) ) ;
#52513=CARTESIAN_POINT ( 'NONE',  ( 112.4747680694540293, -26.21285726233897506, 165.6984824187679521 ) ) ;
#52514=LINE ( 'NONE', #80719, #52366 ) ;
#52515=DIRECTION ( 'NONE',  ( -1.000000000000000078E-15, 0.000000000000000000, 1.000000000000000000 ) ) ;
#52519=AXIS2_PLACEMENT_3D ( 'NONE', #73019, #52547, #10789 ) ;
#52520=CARTESIAN_POINT ( 'NONE',  ( 75.31670390244798341, -57.40094715994099772, 84.20080685541500998 ) ) ;
#52521=CARTESIAN_POINT ( 'NONE',  ( 143.0664832912740110, -18.82844715994099971, 246.4006252759120059 ) ) ;
#52522=EDGE_CURVE ( 'NONE', #11886, #70782, #45945, .T. ) ;
#52523=DIRECTION ( 'NONE',  ( 1.387778780781444492E-15, 0.000000000000000000, -1.000000000000000000 ) ) ;
#52524=CARTESIAN_POINT ( 'NONE',  ( 113.2461215947159161, -45.18040784396236376, 228.0784824187679760 ) ) ;
#52526=LINE ( 'NONE', #18034, #85750 ) ;
#52527=CARTESIAN_POINT ( 'NONE',  ( 112.4656099449901916, -45.71435824391657832, 234.0070538473389377 ) ) ;
#52528=CARTESIAN_POINT ( 'NONE',  ( 113.1020477030913582, -28.17579636167772605, 125.5870538473399591 ) ) ;
#52529=CARTESIAN_POINT ( 'NONE',  ( 51.23005224011598102, -33.89581943344511217, -5.074374724088000832 ) ) ;
#52530=CIRCLE ( 'NONE', #14849, 1.571100913904416307 ) ;
#52531=CARTESIAN_POINT ( 'NONE',  ( 82.45326694837886805, -38.09809895854016304, 7.205238605739220148 ) ) ;
#52532=LINE ( 'NONE', #18483, #19606 ) ;
#52535=EDGE_CURVE ( 'NONE', #77006, #26329, #82538, .T. ) ;
#52537=B_SPLINE_CURVE_WITH_KNOTS ( 'NONE', 3,
 ( #45967, #57836, #2886, #30585, #86015, #72374, #10143, #65547, #25543, #33261, #32348, #39177, #46861, #89133, #67322, #40961, #60051, #75048 ),
 .UNSPECIFIED., .F., .F.,
 ( 4, 2, 2, 2, 2, 2, 2, 2, 4 ),
 ( 0.4999914309044427019, 0.5624925020413873433, 0.6249935731783320403, 0.6874946443152767372, 0.7499957154522214342, 0.8124967865891661312, 0.8749978577261107171, 0.9374989288630553030, 1.000000000000000000 ),
 .UNSPECIFIED. ) ;
#52539=ORIENTED_EDGE ( 'NONE', *, *, #32258, .F. ) ;
#52540=ORIENTED_EDGE ( 'NONE', *, *, #54810, .T. ) ;
#52541=CARTESIAN_POINT ( 'NONE',  ( 116.8171228669039721, -34.15291832155635632, 74.03145860916620791 ) ) ;
#52542=CARTESIAN_POINT ( 'NONE',  ( 100.4791399132689236, -44.80881982087480964, 8.032768133053981074 ) ) ;
#52543=CARTESIAN_POINT ( 'NONE',  ( 49.35031423293201414, -29.99615139349890569, -5.074374724088000832 ) ) ;
#52544=CARTESIAN_POINT ( 'NONE',  ( 131.3325396840767212, -36.38436945697923619, 3.076560175367943906 ) ) ;
#52546=EDGE_CURVE ( 'NONE', #28680, #22667, #72121, .T. ) ;
#52547=DIRECTION ( 'NONE',  ( 0.000000000000000000, -1.000000000000000000, 0.000000000000000000 ) ) ;
#52548=CARTESIAN_POINT ( 'NONE',  ( 109.7255615593723377, -27.00098969710095886, 149.8651129182388217 ) ) ;
#52549=CARTESIAN_POINT ( 'NONE',  ( 100.5279579596103332, -31.18870816475473262, 215.1895626852199541 ) ) ;
#52550=ORIENTED_EDGE ( 'NONE', *, *, #67080, .T. ) ;
#52551=ADVANCED_FACE ( 'NONE', ( #42497 ), #27987, .T. ) ;
#52555=FACE_OUTER_BOUND ( 'NONE', #83145, .T. ) ;
#52556=CARTESIAN_POINT ( 'NONE',  ( 110.8745347144050015, -45.97600918556555882, 182.8873507977141628 ) ) ;
#52557=DIRECTION ( 'NONE',  ( 0.000000000000000000, 0.000000000000000000, -1.000000000000000000 ) ) ;
#52558=CARTESIAN_POINT ( 'NONE',  ( 97.02995690277612084, -35.86988738539728416, 32.69015473446795994 ) ) ;
#52559=AXIS2_PLACEMENT_3D ( 'NONE', #86089, #43832, #23861 ) ;
#52561=DIRECTION ( 'NONE',  ( 1.000000000000000078E-15, -1.000000000000000083E-30, -1.000000000000000000 ) ) ;
#52562=DIRECTION ( 'NONE',  ( 0.000000000000000000, 0.000000000000000000, -1.000000000000000000 ) ) ;
#52565=CARTESIAN_POINT ( 'NONE',  ( 108.7002376003399178, -26.83066989546479775, 55.94644779129590972 ) ) ;
#52566=ORIENTED_EDGE ( 'NONE', *, *, #35655, .F. ) ;
#52568=DIRECTION ( 'NONE',  ( 1.000000000000000078E-15, 1.000000000000000083E-30, -1.000000000000000000 ) ) ;
#52569=CARTESIAN_POINT ( 'NONE',  ( 104.6989491262461769, -45.05385146434951338, 65.18618560768597092 ) ) ;
#52570=CARTESIAN_POINT ( 'NONE',  ( 136.5970563715337391, -17.65296049054856553, 7.043700149388504528 ) ) ;
#52574=CARTESIAN_POINT ( 'NONE',  ( 142.8821648370248170, -72.54478064608022692, 394.9756252759100903 ) ) ;
#52577=ORIENTED_EDGE ( 'NONE', *, *, #59034, .F. ) ;
#52578=CARTESIAN_POINT ( 'NONE',  ( 117.2096823498778662, -39.28706705594211712, 123.6299109901969615 ) ) ;
#52579=ORIENTED_EDGE ( 'NONE', *, *, #57404, .F. ) ;
#52580=CARTESIAN_POINT ( 'NONE',  ( 98.06318007301436523, -37.70576754076741821, 80.82289601855296723 ) ) ;
#52581=DIRECTION ( 'NONE',  ( 0.000000000000000000, 0.000000000000000000, 1.000000000000000000 ) ) ;
#52582=CARTESIAN_POINT ( 'NONE',  ( 115.7370193921850898, -38.55977017368898174, 60.09301187732596361 ) ) ;
#52584=LINE ( 'NONE', #60310, #40107 ) ;
#52585=DIRECTION ( 'NONE',  ( 0.000000000000000000, -1.000000000000000000, 0.000000000000000000 ) ) ;
#52586=CARTESIAN_POINT ( 'NONE',  ( 96.63726304471626349, -32.99895513370901057, 22.06514908543494258 ) ) ;
#52588=ORIENTED_EDGE ( 'NONE', *, *, #48627, .F. ) ;
#52591=LINE ( 'NONE', #61222, #60362 ) ;
#52592=VERTEX_POINT ( 'NONE', #56118 ) ;
#52594=VERTEX_POINT ( 'NONE', #62952 ) ;
#52596=ORIENTED_EDGE ( 'NONE', *, *, #52717, .F. ) ;
#52597=CARTESIAN_POINT ( 'NONE',  ( 106.8648936900573005, -47.09757847023110600, 227.5489586092449485 ) ) ;
#52598=CARTESIAN_POINT ( 'NONE',  ( 97.79342564157622064, -40.47254066486753743, 126.6313135746393357 ) ) ;
#52600=CARTESIAN_POINT ( 'NONE',  ( 117.0537825276303749, -31.99364369613817161, 60.19086337114898555 ) ) ;
#52601=CARTESIAN_POINT ( 'NONE',  ( 116.7950950855014156, -39.38795255544770413, 44.61478202052061448 ) ) ;
#52602=ORIENTED_EDGE ( 'NONE', *, *, #75316, .F. ) ;
#52603=LINE ( 'NONE', #47148, #42391 ) ;
#52604=CARTESIAN_POINT ( 'NONE',  ( 51.42025729302567072, -31.94127993907664020, 193.9678068554150911 ) ) ;
#52609=CARTESIAN_POINT ( 'NONE',  ( 117.3134009501235795, -34.93240959161192194, 243.9641967044819637 ) ) ;
#52610=DIRECTION ( 'NONE',  ( -1.000000000000000000, 0.000000000000000000, 0.000000000000000000 ) ) ;
#52611=AXIS2_PLACEMENT_3D ( 'NONE', #49160, #21032, #138 ) ;
#52614=CARTESIAN_POINT ( 'NONE',  ( 79.18623681048256913, -39.33528726900532746, 1.744847506583331098 ) ) ;
#52615=ADVANCED_FACE ( 'NONE', ( #20733 ), #48403, .F. ) ;
#52616=CARTESIAN_POINT ( 'NONE',  ( 116.0913394378304702, -33.14858145062638073, 248.5495626852199678 ) ) ;
#52618=CARTESIAN_POINT ( 'NONE',  ( 194.5664832912729878, -71.37844715994266664, 342.9256252759109884 ) ) ;
#52619=CARTESIAN_POINT ( 'NONE',  ( 109.9050689397999605, -46.77468768478695438, 68.79562527591099297 ) ) ;
#52621=CARTESIAN_POINT ( 'NONE',  ( 117.6526747975261458, -33.39096950974673916, 129.0575300378159795 ) ) ;
#52622=ORIENTED_EDGE ( 'NONE', *, *, #4895, .T. ) ;
#52623=CARTESIAN_POINT ( 'NONE',  ( 132.2449836194477655, -20.78962918509812496, 7.677444906557659543 ) ) ;
#52624=ORIENTED_EDGE ( 'NONE', *, *, #70185, .T. ) ;
#52627=DIRECTION ( 'NONE',  ( 0.000000000000000000, 0.000000000000000000, -1.000000000000000000 ) ) ;
#52628=DIRECTION ( 'NONE',  ( 4.299999999999999979E-14, -1.000000000000000000, 4.400000000000000367E-29 ) ) ;
#52632=CARTESIAN_POINT ( 'NONE',  ( 117.3823636748946058, -32.63121637840519895, 99.13943479972098771 ) ) ;
#52635=CARTESIAN_POINT ( 'NONE',  ( 107.0664832912739968, -36.72944715994100306, 394.9756252759102040 ) ) ;
#52636=DIRECTION ( 'NONE',  ( -1.000000000000000078E-15, 1.000000000000000083E-30, 1.000000000000000000 ) ) ;
#52638=EDGE_CURVE ( 'NONE', #54865, #38542, #9342, .T. ) ;
#52639=CARTESIAN_POINT ( 'NONE',  ( 114.0369391955824483, -28.94747385925965943, 114.4956252759109816 ) ) ;
#52641=AXIS2_PLACEMENT_3D ( 'NONE', #4757, #19284, #60141 ) ;
#52647=VERTEX_POINT ( 'NONE', #16168 ) ;
#52652=CARTESIAN_POINT ( 'NONE',  ( 33.96670390244654669, -26.71338133339342136, 117.4678068554150485 ) ) ;
#52653=CARTESIAN_POINT ( 'NONE',  ( 97.39138678773666413, -39.27887895447691591, 181.5314891877281127 ) ) ;
#52654=AXIS2_PLACEMENT_3D ( 'NONE', #80202, #67436, #81990 ) ;
#52656=DIRECTION ( 'NONE',  ( 1.000000000000000000, 3.999999999999999995E-14, 1.000000000000000078E-15 ) ) ;
#52657=CARTESIAN_POINT ( 'NONE',  ( 108.1128363339379490, -46.45408497333508535, 198.6613395616249989 ) ) ;
#52658=DIRECTION ( 'NONE',  ( 0.9068632946707805287, -0.4214249218767882055, 8.896017825522093530E-16 ) ) ;
#52659=VERTEX_POINT ( 'NONE', #9788 ) ;
#52660=CARTESIAN_POINT ( 'NONE',  ( 101.3196941207357469, -46.24713579373438677, 48.14419670448194211 ) ) ;
#52661=CARTESIAN_POINT ( 'NONE',  ( 110.8553855737280003, -45.98386346395795243, 52.88570380872458543 ) ) ;
#52662=CARTESIAN_POINT ( 'NONE',  ( 107.0664832912739968, -8.979447159941031487, -4.824374724089029343 ) ) ;
#52663=DIRECTION ( 'NONE',  ( -4.012088370409549976E-14, 1.000000000000000000, 0.000000000000000000 ) ) ;
#52664=ORIENTED_EDGE ( 'NONE', *, *, #57558, .T. ) ;
#52665=CARTESIAN_POINT ( 'NONE',  ( 130.5667039024480118, -39.24694715994093741, 229.5838068554170093 ) ) ;
#52666=VERTEX_POINT ( 'NONE', #8916 ) ;
#52668=EDGE_CURVE ( 'NONE', #76240, #74866, #69190, .T. ) ;
#52669=CARTESIAN_POINT ( 'NONE',  ( 117.0318879909729048, -38.19962202173364574, 220.1415833058969724 ) ) ;
#52670=CIRCLE ( 'NONE', #29511, 1.000000000000000888 ) ;
#52674=VECTOR ( 'NONE', #47602, 1000.000000000000000 ) ;
#52675=CARTESIAN_POINT ( 'NONE',  ( 41.56648329127399677, -18.82844715994099971, 78.92562527591199739 ) ) ;
#52676=CARTESIAN_POINT ( 'NONE',  ( 81.19087023417370119, -39.23918067504817486, 1.822998012175015559 ) ) ;
#52677=EDGE_LOOP ( 'NONE', ( #22389, #65137, #52387, #9531 ) ) ;
#52678=DIRECTION ( 'NONE',  ( 0.000000000000000000, 1.000000000000000000, 0.000000000000000000 ) ) ;
#52679=CARTESIAN_POINT ( 'NONE',  ( 97.39144547896158599, -39.27908535653673994, 37.53121822511904782 ) ) ;
#52681=CARTESIAN_POINT ( 'NONE',  ( 104.6488677213912695, -47.51528149961286829, 27.38895860924395009 ) ) ;
#52683=ORIENTED_EDGE ( 'NONE', *, *, #2706, .T. ) ;
#52684=CARTESIAN_POINT ( 'NONE',  ( 104.9869425053901892, -28.32846893322983917, 238.0757094172099642 ) ) ;
#52685=CARTESIAN_POINT ( 'NONE',  ( 194.0667039024475287, -24.92844715993407334, 180.4678068554150343 ) ) ;
#52688=LINE ( 'NONE', #18205, #65171 ) ;
#52689=CARTESIAN_POINT ( 'NONE',  ( 96.63066398506619237, -35.53291458860860530, 202.2356252759109623 ) ) ;
#52693=CARTESIAN_POINT ( 'NONE',  ( 102.9539626486510713, -46.35650038051790744, 88.25562527591095829 ) ) ;
#52694=FACE_OUTER_BOUND ( 'NONE', #17732, .T. ) ;
#52695=AXIS2_PLACEMENT_3D ( 'NONE', #78865, #43865, #10681 ) ;
#52696=ORIENTED_EDGE ( 'NONE', *, *, #18183, .T. ) ;
#52697=ORIENTED_EDGE ( 'NONE', *, *, #22653, .F. ) ;
#52700=CARTESIAN_POINT ( 'NONE',  ( 63.56670390244708813, -40.82844715994014706, 180.4678068554151196 ) ) ;
#52701=CARTESIAN_POINT ( 'NONE',  ( 181.8764988495240118, -33.54226604284930602, -5.074374724088000832 ) ) ;
#52703=CARTESIAN_POINT ( 'NONE',  ( 114.8702562078425160, -31.70976148532177064, 142.0995189410209605 ) ) ;
#52704=CARTESIAN_POINT ( 'NONE',  ( 100.6429626219512983, -44.96811459249982335, 228.0499109901969348 ) ) ;
#52705=CARTESIAN_POINT ( 'NONE',  ( 116.3279290549545806, -32.94269076977911226, 60.13562527591098927 ) ) ;
#52706=ORIENTED_EDGE ( 'NONE', *, *, #51200, .F. ) ;
#52707=DIRECTION ( 'NONE',  ( 0.000000000000000000, 0.000000000000000000, -1.000000000000000000 ) ) ;
#52708=ORIENTED_EDGE ( 'NONE', *, *, #7042, .F. ) ;
#52709=VERTEX_POINT ( 'NONE', #43847 ) ;
#52710=CIRCLE ( 'NONE', #1997, 0.5000000000000004441 ) ;
#52711=CARTESIAN_POINT ( 'NONE',  ( 90.44969454456405344, -20.11243780205715481, 218.8274735512160589 ) ) ;
#52712=VERTEX_POINT ( 'NONE', #3420 ) ;
#52714=CARTESIAN_POINT ( 'NONE',  ( 113.1798478553082248, -44.75070311407051094, 169.0948016189585417 ) ) ;
#52715=CARTESIAN_POINT ( 'NONE',  ( 184.5667039024480118, -67.87844715994100397, 20.91780685541479912 ) ) ;
#52716=CARTESIAN_POINT ( 'NONE',  ( 97.81170495107971874, -40.51745053935989915, 26.63526479160227112 ) ) ;
#52717=EDGE_CURVE ( 'NONE', #22746, #12675, #70697, .T. ) ;
#52718=CARTESIAN_POINT ( 'NONE',  ( 102.9572487778789878, -44.79956872283601399, 171.6362293518859587 ) ) ;
#52719=CARTESIAN_POINT ( 'NONE',  ( 111.1461885285858671, -47.05266801877174032, 22.88800622829195675 ) ) ;
#52720=ORIENTED_EDGE ( 'NONE', *, *, #8866, .F. ) ;
#52724=VERTEX_POINT ( 'NONE', #23874 ) ;
#52725=CARTESIAN_POINT ( 'NONE',  ( 167.2371591254544967, -47.82818131005522133, 180.4678068554150059 ) ) ;
#52727=VERTEX_POINT ( 'NONE', #79293 ) ;
#52728=CYLINDRICAL_SURFACE ( 'NONE', #8774, 3.249999999999975131 ) ;
#52730=DIRECTION ( 'NONE',  ( -1.000000000000000078E-15, 1.000000000000000083E-30, 1.000000000000000000 ) ) ;
#52733=CARTESIAN_POINT ( 'NONE',  ( 100.4512775726424820, -44.84301714363712676, 12.03276813305398463 ) ) ;
#52734=CARTESIAN_POINT ( 'NONE',  ( 106.5158076061070460, -25.64367904723916780, 41.12800622829193742 ) ) ;
#52737=DIRECTION ( 'NONE',  ( 0.9068632946707806397, -0.4214249218767879279, 9.068632946707804446E-16 ) ) ;
#52739=LINE ( 'NONE', #87756, #78625 ) ;
#52740=DIRECTION ( 'NONE',  ( 1.000000000000000000, 4.163336342344333240E-14, 0.000000000000000000 ) ) ;
#52741=EDGE_CURVE ( 'NONE', #28724, #58384, #17053, .T. ) ;
#52742=CARTESIAN_POINT ( 'NONE',  ( 106.6019379103756535, -25.27972995136449441, 322.9014499992877631 ) ) ;
#52743=DIRECTION ( 'NONE',  ( 0.08544974978095713769, 0.9963424814100680926, -0.000000000000000000 ) ) ;
#52744=CARTESIAN_POINT ( 'NONE',  ( 99.09377177006922466, -44.45270778143659385, 41.95086337114900488 ) ) ;
#52745=CARTESIAN_POINT ( 'NONE',  ( 100.6376613383881704, -26.77430457650146423, 216.5327681330539633 ) ) ;
#52746=CARTESIAN_POINT ( 'NONE',  ( 113.4728825864854116, -46.72846204934055692, 64.02991099019695298 ) ) ;
#52748=CARTESIAN_POINT ( 'NONE',  ( 116.8171228664610766, -34.15291832047437026, 49.03145860925929611 ) ) ;
#52749=CARTESIAN_POINT ( 'NONE',  ( 81.77561474850375589, -34.57277681850425211, 2.101554741571703744 ) ) ;
#52750=AXIS2_PLACEMENT_3D ( 'NONE', #30830, #23152, #37205 ) ;
#52751=CIRCLE ( 'NONE', #28151, 1.000000000000000888 ) ;
#52752=VECTOR ( 'NONE', #69315, 1000.000000000000000 ) ;
#52756=CARTESIAN_POINT ( 'NONE',  ( 114.2351621074132026, -44.22269940884944361, 109.1718157521009687 ) ) ;
#52758=ORIENTED_EDGE ( 'NONE', *, *, #3650, .T. ) ;
#52760=CARTESIAN_POINT ( 'NONE',  ( 115.3705510513157009, -30.46277945167186374, 215.3413395616249773 ) ) ;
#52762=CARTESIAN_POINT ( 'NONE',  ( 110.9557970953006247, -45.94221351776628381, 147.8943543333864739 ) ) ;
#52764=DIRECTION ( 'NONE',  ( 1.017460296392624983E-15, 1.000000000000000000, 0.000000000000000000 ) ) ;
#52765=CARTESIAN_POINT ( 'NONE',  ( 131.5325842222575830, -37.79809288067819040, 2.811527366592918575 ) ) ;
#52766=CARTESIAN_POINT ( 'NONE',  ( 172.5664832912740110, -18.82844715994099971, 78.92562527591199739 ) ) ;
#52767=CARTESIAN_POINT ( 'NONE',  ( 96.69720940280899413, -36.59277893904148726, 156.3280062282929634 ) ) ;
#52771=CARTESIAN_POINT ( 'NONE',  ( 115.4437480007128443, -33.74891607059462473, 110.5301547344689794 ) ) ;
#52773=CARTESIAN_POINT ( 'NONE',  ( 97.83217745605955429, -40.05230289513912822, 262.6013395616248545 ) ) ;
#52779=DIRECTION ( 'NONE',  ( 1.639958061481212836E-42, -4.100000000000000342E-29, -1.000000000000000000 ) ) ;
#52780=LINE ( 'NONE', #5125, #23235 ) ;
#52782=CARTESIAN_POINT ( 'NONE',  ( 97.42226921825827901, -40.63044708855872500, 206.6327681330539860 ) ) ;
#52783=ORIENTED_EDGE ( 'NONE', *, *, #45745, .T. ) ;
#52785=LINE ( 'NONE', #23807, #73472 ) ;
#52786=LINE ( 'NONE', #51475, #30251 ) ;
#52788=CARTESIAN_POINT ( 'NONE',  ( 116.1804594027163517, -40.96476762480074996, 0.4256252759109800388 ) ) ;
#52790=EDGE_CURVE ( 'NONE', #70380, #78000, #36615, .T. ) ;
#52791=CARTESIAN_POINT ( 'NONE',  ( 115.0356604027599587, -42.91048835123673655, 63.30208818923281910 ) ) ;
#52792=CARTESIAN_POINT ( 'NONE',  ( 116.7954078171858896, -40.57313474401875197, 193.5270538473389479 ) ) ;
#52793=CARTESIAN_POINT ( 'NONE',  ( 135.9139897988364112, -38.77444411304905714, 7.664507283842826979 ) ) ;
#52797=DIRECTION ( 'NONE',  ( 0.000000000000000000, 0.000000000000000000, 1.000000000000000000 ) ) ;
#52798=CARTESIAN_POINT ( 'NONE',  ( 116.7947413403456522, -39.38919790731562642, 164.6146797249617748 ) ) ;
#52799=CARTESIAN_POINT ( 'NONE',  ( 98.54061126669880366, -38.21619907818254802, 44.26999513149598897 ) ) ;
#52800=EDGE_CURVE ( 'NONE', #36112, #44764, #75029, .T. ) ;
#52801=FACE_OUTER_BOUND ( 'NONE', #78766, .T. ) ;
#52802=ORIENTED_EDGE ( 'NONE', *, *, #33163, .T. ) ;
#52804=CARTESIAN_POINT ( 'NONE',  ( 82.06789631129603890, -16.84294903901377793, 7.549690073096890330 ) ) ;
#52805=ORIENTED_EDGE ( 'NONE', *, *, #1943, .T. ) ;
#52806=VERTEX_POINT ( 'NONE', #73338 ) ;
#52808=AXIS2_PLACEMENT_3D ( 'NONE', #7782, #29569, #36396 ) ;
#52809=LINE ( 'NONE', #66030, #77855 ) ;
#52810=VECTOR ( 'NONE', #64439, 1000.000000000000000 ) ;
#52811=ORIENTED_EDGE ( 'NONE', *, *, #54264, .T. ) ;
#52812=VERTEX_POINT ( 'NONE', #25639 ) ;
#52813=CARTESIAN_POINT ( 'NONE',  ( 97.06112134132963831, -37.99667316087620605, 157.4271097502474390 ) ) ;
#52814=AXIS2_PLACEMENT_3D ( 'NONE', #21169, #34783, #33885 ) ;
#52815=CARTESIAN_POINT ( 'NONE',  ( 101.2610328325635010, -42.99465878394229179, 46.40384839950495177 ) ) ;
#52816=AXIS2_PLACEMENT_3D ( 'NONE', #2521, #58359, #25174 ) ;
#52817=CARTESIAN_POINT ( 'NONE',  ( 103.6313148537710305, -26.19877486694289459, 210.3394347997209763 ) ) ;
#52819=CARTESIAN_POINT ( 'NONE',  ( 103.8142050530422438, -26.84757730287814326, 165.3299109901969643 ) ) ;
#52820=CARTESIAN_POINT ( 'NONE',  ( 98.05739576140550184, -41.07564549115163288, 21.68389642371685255 ) ) ;
#52821=CARTESIAN_POINT ( 'NONE',  ( 97.55999611477783162, -43.80484941858547643, 257.8356252759109566 ) ) ;
#52822=LINE ( 'NONE', #26960, #39058 ) ;
#52823=ADVANCED_FACE ( 'NONE', ( #11580 ), #51981, .T. ) ;
#52826=VERTEX_POINT ( 'NONE', #52852 ) ;
#52828=CARTESIAN_POINT ( 'NONE',  ( 115.4232488078209258, -30.42301107085752321, 219.3413395616249773 ) ) ;
#52829=EDGE_LOOP ( 'NONE', ( #86502, #10083, #27244, #24455 ) ) ;
#52830=CARTESIAN_POINT ( 'NONE',  ( 113.6857051329922683, -45.58184738042410800, 188.0994347997199725 ) ) ;
#52831=CARTESIAN_POINT ( 'NONE',  ( 115.8245126124504907, -31.72842839644106405, 264.2397945930570700 ) ) ;
#52833=FACE_OUTER_BOUND ( 'NONE', #42629, .T. ) ;
#52837=CARTESIAN_POINT ( 'NONE',  ( 105.4283309587863613, -27.08694620864308789, 11.20991099019597037 ) ) ;
#52838=DIRECTION ( 'NONE',  ( -1.639958061481212836E-42, 4.100000000000000342E-29, 1.000000000000000000 ) ) ;
#52839=FACE_OUTER_BOUND ( 'NONE', #23640, .T. ) ;
#52840=CARTESIAN_POINT ( 'NONE',  ( 180.3521107875639871, -35.65087443492551245, -5.074374724088000832 ) ) ;
#52841=EDGE_CURVE ( 'NONE', #56941, #82390, #66070, .T. ) ;
#52842=CARTESIAN_POINT ( 'NONE',  ( 73.06670390244801183, -48.82844715994099971, 198.9178068554149945 ) ) ;
#52843=ADVANCED_FACE ( 'NONE', ( #59259 ), #24749, .F. ) ;
#52848=CARTESIAN_POINT ( 'NONE',  ( 136.5663465660592806, -19.87725565066165956, 7.080220459962397683 ) ) ;
#52849=CARTESIAN_POINT ( 'NONE',  ( 99.73754448486663193, -29.28411171159743276, 225.6956252759109702 ) ) ;
#52850=CARTESIAN_POINT ( 'NONE',  ( 117.3712488531672165, -32.73122415481606851, 90.10895860924395606 ) ) ;
#52851=CARTESIAN_POINT ( 'NONE',  ( 116.5662105847193999, -41.21199064955116143, 224.4756252759109714 ) ) ;
#52852=CARTESIAN_POINT ( 'NONE',  ( 172.5664832912740110, -18.82844715994099971, 256.8086252759120498 ) ) ;
#52853=B_SPLINE_CURVE_WITH_KNOTS ( 'NONE', 3,
 ( #18796, #4726, #12431, #25607, #5169, #66489, #52820, #32405, #81941, #60563, #80593, #46480, #73759, #18339, #74217, #11542, #39237, #26064, #53732, #81498, #19250, #46923, #40120, #19692, #47372, #40579, #75103 ),
 .UNSPECIFIED., .F., .F.,
 ( 4, 2, 1, 1, 1, 2, 2, 2, 2, 2, 2, 2, 2, 2, 4 ),
 ( 0.4999367561938997673, 0.5009134422169587708, 0.5018901282400176633, 0.5038435002861353373, 0.5077502443783706854, 0.5155637325628411594, 0.5311907089317821073, 0.5624446616696634482, 0.6249525671454257969, 0.6874604726211881456, 0.7499683780969504943, 0.8124762835727128429, 0.8749841890484753026, 0.9374920945242376513, 1.000000000000000000 ),
 .UNSPECIFIED. ) ;
#52854=PLANE ( 'NONE',  #60529 ) ;
#52856=CARTESIAN_POINT ( 'NONE',  ( 107.0664832912739968, 19.62155284005901024, 333.4006252759110112 ) ) ;
#52862=CARTESIAN_POINT ( 'NONE',  ( 103.6638222329471262, -28.86385020797125733, 154.8238483995059767 ) ) ;
#52863=CARTESIAN_POINT ( 'NONE',  ( 21.03689327557619748, -23.42844715994197813, 129.9678068554150627 ) ) ;
#52864=ORIENTED_EDGE ( 'NONE', *, *, #48843, .T. ) ;
#52865=CARTESIAN_POINT ( 'NONE',  ( 109.7247368277677424, -27.00077089589298751, 89.86349248373032594 ) ) ;
#52866=CARTESIAN_POINT ( 'NONE',  ( 114.4965984691700953, -29.44205611023144087, 145.4441967044819819 ) ) ;
#52867=DIRECTION ( 'NONE',  ( 0.000000000000000000, 0.000000000000000000, -1.000000000000000000 ) ) ;
#52868=CARTESIAN_POINT ( 'NONE',  ( 77.61460381940085540, -17.48272374588778533, 7.134497377255414108 ) ) ;
#52871=CARTESIAN_POINT ( 'NONE',  ( 101.4370486012140020, -28.02035706366309853, 70.54514908543596619 ) ) ;
#52872=ORIENTED_EDGE ( 'NONE', *, *, #50320, .T. ) ;
#52874=ORIENTED_EDGE ( 'NONE', *, *, #37476, .T. ) ;
#52878=CARTESIAN_POINT ( 'NONE',  ( 97.29384000864243376, -37.12803473146956890, 157.3584824187679487 ) ) ;
#52879=CARTESIAN_POINT ( 'NONE',  ( 83.06670390244796920, -58.35344715994099829, 228.3338068554150198 ) ) ;
#52881=DIRECTION ( 'NONE',  ( -0.04216478779797398074, 0.9991106698809455455, 0.000000000000000000 ) ) ;
#52882=LINE ( 'NONE', #87462, #3115 ) ;
#52888=CARTESIAN_POINT ( 'NONE',  ( 98.32466564902610173, -28.76522518762216052, 80.73848241876795839 ) ) ;
#52889=ORIENTED_EDGE ( 'NONE', *, *, #17313, .T. ) ;
#52892=CARTESIAN_POINT ( 'NONE',  ( 142.0664832912740394, -46.72944715994099596, 14.67562527591100441 ) ) ;
#52894=AXIS2_PLACEMENT_3D ( 'NONE', #63311, #27888, #63767 ) ;
#52895=CARTESIAN_POINT ( 'NONE',  ( 99.71285092336476907, -40.27258376677666263, 169.5023760838769817 ) ) ;
#52896=EDGE_CURVE ( 'NONE', #68461, #38148, #32898, .T. ) ;
#52898=DIRECTION ( 'NONE',  ( -4.237773401492740281E-14, 1.000000000000000000, 0.000000000000000000 ) ) ;
#52899=ORIENTED_EDGE ( 'NONE', *, *, #82614, .T. ) ;
#52900=ORIENTED_EDGE ( 'NONE', *, *, #26841, .F. ) ;
#52901=EDGE_CURVE ( 'NONE', #57610, #83459, #21556, .T. ) ;
#52902=DIRECTION ( 'NONE',  ( 1.000000000000000078E-15, -1.000000000000000083E-30, -1.000000000000000000 ) ) ;
#52903=ORIENTED_EDGE ( 'NONE', *, *, #37415, .F. ) ;
#52906=EDGE_CURVE ( 'NONE', #8522, #44708, #87493, .T. ) ;
#52907=CARTESIAN_POINT ( 'NONE',  ( 113.6520771548495503, -30.75516201018407614, 205.8444404487539714 ) ) ;
#52908=EDGE_CURVE ( 'NONE', #6901, #85061, #81081, .T. ) ;
#52909=DIRECTION ( 'NONE',  ( 0.000000000000000000, 0.000000000000000000, -1.000000000000000000 ) ) ;
#52911=EDGE_CURVE ( 'NONE', #11918, #86172, #39706, .T. ) ;
#52915=VERTEX_POINT ( 'NONE', #86989 ) ;
#52916=VECTOR ( 'NONE', #25180, 1000.000000000000000 ) ;
#52918=EDGE_LOOP ( 'NONE', ( #63368, #15108, #60400, #13777 ) ) ;
#52919=ADVANCED_FACE ( 'NONE', ( #52418 ), #46513, .F. ) ;
#52920=B_SPLINE_CURVE_WITH_KNOTS ( 'NONE', 3,
 ( #82523, #85653, #22978, #3409, #50653, #64304, #3852, #72452, #51097, #16157, #51534, #30226, #2964, #8902, #43834, #57917, #58364, #37925 ),
 .UNSPECIFIED., .F., .F.,
 ( 4, 2, 2, 2, 2, 2, 2, 2, 4 ),
 ( 0.5000723104273193664, 0.5625632716239044040, 0.6250542328204895526, 0.6875451940170745901, 0.7500361552136596277, 0.8125271164102447763, 0.8750180776068298139, 0.9375090388034148514, 1.000000000000000000 ),
 .UNSPECIFIED. ) ;
#52921=CARTESIAN_POINT ( 'NONE',  ( 114.9986391697397607, -34.80314782265816831, 206.8338046553059826 ) ) ;
#52922=CARTESIAN_POINT ( 'NONE',  ( 117.3606796971436523, -32.63983085838949449, 99.13943479972098771 ) ) ;
#52923=CARTESIAN_POINT ( 'NONE',  ( 116.6546583390153131, -32.60254457568996855, 79.14991099019697174 ) ) ;
#52924=CARTESIAN_POINT ( 'NONE',  ( 112.8677825012601375, -28.59025478454122648, 249.5838084826162913 ) ) ;
#52925=FACE_BOUND ( 'NONE', #15769, .T. ) ;
#52927=CARTESIAN_POINT ( 'NONE',  ( 100.8865061632069882, -45.89117093204367137, 148.0918157521009562 ) ) ;
#52928=EDGE_CURVE ( 'NONE', #42715, #64265, #17852, .T. ) ;
#52931=DIRECTION ( 'NONE',  ( -1.000000000000000000, 0.000000000000000000, 0.000000000000000000 ) ) ;
#52934=PLANE ( 'NONE',  #62154 ) ;
#52935=DIRECTION ( 'NONE',  ( 1.000000000000000000, 0.000000000000000000, 0.000000000000000000 ) ) ;
#52937=VECTOR ( 'NONE', #47767, 1000.000000000000000 ) ;
#52938=DIRECTION ( 'NONE',  ( 0.000000000000000000, 1.000000000000000000, 1.598363122120870523E-15 ) ) ;
#52939=VERTEX_POINT ( 'NONE', #33352 ) ;
#52940=VECTOR ( 'NONE', #12371, 1000.000000000000000 ) ;
#52941=AXIS2_PLACEMENT_3D ( 'NONE', #73712, #45979, #6032 ) ;
#52943=CARTESIAN_POINT ( 'NONE',  ( 115.1669806615814622, -43.29214270484202132, 88.28419670448195689 ) ) ;
#52945=VECTOR ( 'NONE', #10804, 1000.000000000000000 ) ;
#52946=CARTESIAN_POINT ( 'NONE',  ( 48.16670390244701139, -28.27351298637280408, -5.074374724088000832 ) ) ;
#52948=CARTESIAN_POINT ( 'NONE',  ( 116.7039036015866031, -32.90075090702271865, 99.13943479972198247 ) ) ;
#52950=CARTESIAN_POINT ( 'NONE',  ( 96.64068249873270133, -36.21262657180042766, 167.2870538473399620 ) ) ;
#52952=DIRECTION ( 'NONE',  ( 3.340531404218880531E-13, -1.000000000000000000, 3.350531404218880242E-28 ) ) ;
#52953=ORIENTED_EDGE ( 'NONE', *, *, #26850, .F. ) ;
#52954=CARTESIAN_POINT ( 'NONE',  ( 49.21213752016101495, -29.73316016639650172, -5.074374724088000832 ) ) ;
#52955=AXIS2_PLACEMENT_3D ( 'NONE', #26863, #47740, #75475 ) ;
#52959=DIRECTION ( 'NONE',  ( 0.000000000000000000, 1.000000000000000000, 1.914177628664063178E-15 ) ) ;
#52960=ADVANCED_FACE ( 'NONE', ( #66976 ), #1918, .T. ) ;
#52961=VECTOR ( 'NONE', #56705, 1000.000000000000000 ) ;
#52963=CARTESIAN_POINT ( 'NONE',  ( 116.9264758816979537, -41.82782236628663242, 243.4346728949589647 ) ) ;
#52964=ORIENTED_EDGE ( 'NONE', *, *, #73583, .F. ) ;
#52965=CARTESIAN_POINT ( 'NONE',  ( 97.07201709675129564, -35.37882905153811208, 146.2189892174000363 ) ) ;
#52966=CARTESIAN_POINT ( 'NONE',  ( 96.86769303131731590, -30.64611497598638579, 276.8984824187680829 ) ) ;
#52967=CARTESIAN_POINT ( 'NONE',  ( 114.7580948764747291, -43.83100269166961027, 119.2327681330539804 ) ) ;
#52968=EDGE_CURVE ( 'NONE', #84350, #17132, #39271, .T. ) ;
#52969=DIRECTION ( 'NONE',  ( -0.7071067811865671127, -0.7071067811865279218, -7.071067811865664660E-16 ) ) ;
#52972=CYLINDRICAL_SURFACE ( 'NONE', #10912, 2.117000000000000881 ) ;
#52973=CARTESIAN_POINT ( 'NONE',  ( 105.7149977036519459, -46.72378562122258927, 263.4690551747434597 ) ) ;
#52978=VERTEX_POINT ( 'NONE', #17496 ) ;
#52980=CARTESIAN_POINT ( 'NONE',  ( 100.4250012405661607, -28.72198927997979823, 36.62705384733894221 ) ) ;
#52981=DIRECTION ( 'NONE',  ( -2.279500465453769633E-16, 3.512896218562319948E-31, 1.000000000000000000 ) ) ;
#52985=CARTESIAN_POINT ( 'NONE',  ( 97.42200983434074146, -37.84960760947268454, 235.8409912566479818 ) ) ;
#52986=ORIENTED_EDGE ( 'NONE', *, *, #40841, .F. ) ;
#52987=VERTEX_POINT ( 'NONE', #56806 ) ;
#52989=ORIENTED_EDGE ( 'NONE', *, *, #77080, .F. ) ;
#52990=DIRECTION ( 'NONE',  ( -0.7071067811864671926, -0.7071067811866279529, -7.071067811864976379E-16 ) ) ;
#52991=CIRCLE ( 'NONE', #13874, 3.300000000000000711 ) ;
#52992=CARTESIAN_POINT ( 'NONE',  ( 116.3216177720312317, -32.94249360885015676, 184.1356252759109680 ) ) ;
#52993=CARTESIAN_POINT ( 'NONE',  ( 34.33598329127499227, -36.32844715994100682, -5.074374724088000832 ) ) ;
#52994=CARTESIAN_POINT ( 'NONE',  ( 109.8015415646094226, -45.15840846867854452, 9.258726163039964874 ) ) ;
#52996=DIRECTION ( 'NONE',  ( 4.299999999999999979E-14, -1.000000000000000000, 0.000000000000000000 ) ) ;
#52997=CARTESIAN_POINT ( 'NONE',  ( 104.4938967476557536, -26.68352342390101128, 245.2880062282919482 ) ) ;
#53001=DIRECTION ( 'NONE',  ( 1.000000000000000078E-15, -1.000000000000000083E-30, -1.000000000000000000 ) ) ;
#53002=CARTESIAN_POINT ( 'NONE',  ( 115.5682441604615178, -40.44643428488449644, 56.31666179816296847 ) ) ;
#53005=AXIS2_PLACEMENT_3D ( 'NONE', #14521, #1340, #6351 ) ;
#53007=AXIS2_PLACEMENT_3D ( 'NONE', #68919, #20768, #7145 ) ;
#53008=EDGE_CURVE ( 'NONE', #67672, #16139, #37796, .T. ) ;
#53009=DIRECTION ( 'NONE',  ( 1.000000000000000000, 4.299999999999999979E-14, 1.000000000000000078E-15 ) ) ;
#53011=EDGE_LOOP ( 'NONE', ( #6072, #13756, #80412, #55737 ) ) ;
#53012=CARTESIAN_POINT ( 'NONE',  ( 33.78129701732998313, -35.65087443492610930, -5.074374724088000832 ) ) ;
#53015=ORIENTED_EDGE ( 'NONE', *, *, #22019, .F. ) ;
#53016=CARTESIAN_POINT ( 'NONE',  ( 116.5335121716806981, -32.36339692672488155, 104.1699109901969535 ) ) ;
#53017=VERTEX_POINT ( 'NONE', #28663 ) ;
#53018=CARTESIAN_POINT ( 'NONE',  ( 97.46629167631436985, -35.27791395320982559, 70.62956268521996606 ) ) ;
#53020=DIRECTION ( 'NONE',  ( 1.000000000000000078E-15, 0.000000000000000000, 1.000000000000000000 ) ) ;
#53021=CARTESIAN_POINT ( 'NONE',  ( 99.74759560186635099, -41.77880479991928553, 123.2387261630399564 ) ) ;
#53023=LINE ( 'NONE', #25350, #31485 ) ;
#53025=CARTESIAN_POINT ( 'NONE',  ( 117.5094244910773114, -37.01621876064744754, 39.80419670448193159 ) ) ;
#53026=DIRECTION ( 'NONE',  ( 0.000000000000000000, 0.000000000000000000, 1.000000000000000000 ) ) ;
#53027=EDGE_CURVE ( 'NONE', #81179, #60711, #21868, .T. ) ;
#53028=ORIENTED_EDGE ( 'NONE', *, *, #74295, .T. ) ;
#53029=CARTESIAN_POINT ( 'NONE',  ( 115.0370918404214393, -42.90867283834190715, 258.3021863231967927 ) ) ;
#53033=AXIS2_PLACEMENT_3D ( 'NONE', #30021, #29566, #29124 ) ;
#53035=ADVANCED_FACE ( 'NONE', ( #77272 ), #42718, .F. ) ;
#53036=B_SPLINE_CURVE_WITH_KNOTS ( 'NONE', 3,
 ( #43750, #16509, #86450, #71487, #51012, #72806, #85568, #57379, #23782, #9687, #85122, #79638, #9249, #22889, #50565, #2881, #86009, #30580 ),
 .UNSPECIFIED., .F., .F.,
 ( 4, 2, 2, 2, 2, 2, 2, 2, 4 ),
 ( 0.000000000000000000, 0.06249892886305533773, 0.1249978577261106755, 0.1874967865891660201, 0.2499957154522213509, 0.3124946443152766817, 0.3749935731783320403, 0.4374925020413873433, 0.4999914309044427019 ),
 .UNSPECIFIED. ) ;
#53039=CARTESIAN_POINT ( 'NONE',  ( 112.3177584634463244, -44.98096486020163098, 263.0270538473400279 ) ) ;
#53042=CARTESIAN_POINT ( 'NONE',  ( 109.6429888323185224, -46.83113546657025950, 43.77562527591094721 ) ) ;
#53043=EDGE_CURVE ( 'NONE', #48663, #36108, #40611, .T. ) ;
#53044=CARTESIAN_POINT ( 'NONE',  ( 97.92315705725079056, -40.78053340632050094, 42.65836484899426040 ) ) ;
#53046=CARTESIAN_POINT ( 'NONE',  ( 105.7993578692051244, -26.72404692965724848, 115.1793930805829547 ) ) ;
#53050=ORIENTED_EDGE ( 'NONE', *, *, #5508, .T. ) ;
#53053=CARTESIAN_POINT ( 'NONE',  ( 118.0177608886754967, -35.41288285714057338, 238.9337205140059552 ) ) ;
#53054=CARTESIAN_POINT ( 'NONE',  ( 48.79742451362098166, -36.32844715994040996, -5.074374724088000832 ) ) ;
#53056=CARTESIAN_POINT ( 'NONE',  ( 79.87807227642889529, -39.47944715994105280, 1.625625275910943301 ) ) ;
#53057=CARTESIAN_POINT ( 'NONE',  ( 101.3905103160957850, -43.11219441383617124, 266.4209912566481080 ) ) ;
#53059=CARTESIAN_POINT ( 'NONE',  ( 116.9541756933414263, -33.49491404195861577, 85.07848241876791917 ) ) ;
#53061=CARTESIAN_POINT ( 'NONE',  ( 103.1581569894456294, -27.01699888143334860, 130.3813395616259925 ) ) ;
#53062=VERTEX_POINT ( 'NONE', #71366 ) ;
#53065=DIRECTION ( 'NONE',  ( 1.000000000000000000, 4.163336342344333240E-14, 0.000000000000000000 ) ) ;
#53066=PLANE ( 'NONE',  #75445 ) ;
#53067=CARTESIAN_POINT ( 'NONE',  ( 20.03715912545730760, -24.42818131006189830, 300.4678068554150059 ) ) ;
#53069=ADVANCED_FACE ( 'NONE', ( #35465 ), #35921, .F. ) ;
#53070=CARTESIAN_POINT ( 'NONE',  ( 97.60797852784317286, -39.98268459812312869, 51.59008640786052524 ) ) ;
#53071=CARTESIAN_POINT ( 'NONE',  ( 108.3247603638532865, -47.12287801086134920, 117.6727681330539639 ) ) ;
#53072=ORIENTED_EDGE ( 'NONE', *, *, #81519, .F. ) ;
#53074=EDGE_CURVE ( 'NONE', #79111, #39595, #14602, .T. ) ;
#53075=VECTOR ( 'NONE', #3148, 1000.000000000000000 ) ;
#53077=DIRECTION ( 'NONE',  ( -1.000000000000000000, -1.000000000000000078E-15, -1.000000000000000078E-15 ) ) ;
#53079=EDGE_LOOP ( 'NONE', ( #67667, #15582, #66175, #20142 ) ) ;
#53080=CARTESIAN_POINT ( 'NONE',  ( 97.81638875629413121, -31.87330516686267501, 135.9413395616259947 ) ) ;
#53084=DIRECTION ( 'NONE',  ( 0.9963424814100680926, -0.08544974978095691565, 0.000000000000000000 ) ) ;
#53085=DIRECTION ( 'NONE',  ( -1.424786214935630051E-15, 0.000000000000000000, 1.000000000000000000 ) ) ;
#53091=DIRECTION ( 'NONE',  ( -2.106816776397999944E-14, 1.000000000000000000, -2.206816776398000223E-29 ) ) ;
#53093=CARTESIAN_POINT ( 'NONE',  ( 109.7246038384062246, -27.00073569414776387, 104.8648133147524391 ) ) ;
#53096=AXIS2_PLACEMENT_3D ( 'NONE', #42901, #23833, #85624 ) ;
#53097=EDGE_CURVE ( 'NONE', #58575, #38868, #36739, .T. ) ;
#53099=( BOUNDED_CURVE ( )  B_SPLINE_CURVE ( 3, ( #54051, #74978, #45900, #4145 ),
 .UNSPECIFIED., .F., .F. ) 
 B_SPLINE_CURVE_WITH_KNOTS ( ( 4, 4 ),
 ( 1.570796326781801477, 3.141592653579262873 ),
 .UNSPECIFIED. ) 
 CURVE ( )  GEOMETRIC_REPRESENTATION_ITEM ( )  RATIONAL_B_SPLINE_CURVE ( ( 1.000000000000000000, 0.8047378541237604210, 0.8047378541237604210, 1.000000000000000000 ) ) 
 REPRESENTATION_ITEM ( '' )  );
#53101=DIRECTION ( 'NONE',  ( -1.000000000000000078E-15, 0.000000000000000000, -1.000000000000000000 ) ) ;
#53102=CARTESIAN_POINT ( 'NONE',  ( 107.5349099188610893, -47.08895302312297559, 188.6003871806719587 ) ) ;
#53104=EDGE_LOOP ( 'NONE', ( #42026, #34649, #27333, #2294, #83025, #3228, #19775, #26029 ) ) ;
#53105=CARTESIAN_POINT ( 'NONE',  ( 104.9021620152489476, -46.26774620671717031, 68.39848241876694601 ) ) ;
#53111=ORIENTED_EDGE ( 'NONE', *, *, #51301, .F. ) ;
#53112=ORIENTED_EDGE ( 'NONE', *, *, #42484, .T. ) ;
#53113=VECTOR ( 'NONE', #57642, 1000.000000000000000 ) ;
#53114=EDGE_CURVE ( 'NONE', #63918, #46374, #57251, .T. ) ;
#53115=CARTESIAN_POINT ( 'NONE',  ( 103.8678987209337947, -28.46522696937008945, 211.8015833058969690 ) ) ;
#53116=CARTESIAN_POINT ( 'NONE',  ( 104.4090465223629707, -46.45838000546697089, 53.36450883979372151 ) ) ;
#53121=DIRECTION ( 'NONE',  ( -0.7071067812159671506, -0.7071067811571278838, -6.612322856129998538E-17 ) ) ;
#53122=ORIENTED_EDGE ( 'NONE', *, *, #60114, .T. ) ;
#53123=DIRECTION ( 'NONE',  ( 0.000000000000000000, 0.000000000000000000, -1.000000000000000000 ) ) ;
#53124=ADVANCED_FACE ( 'NONE', ( #24102 ), #19347, .T. ) ;
#53125=DIRECTION ( 'NONE',  ( -1.000000000000000000, 0.000000000000000000, 0.000000000000000000 ) ) ;
#53127=CARTESIAN_POINT ( 'NONE',  ( 115.9452887564414851, -42.19329433630747417, 18.38705384733896153 ) ) ;
#53128=ORIENTED_EDGE ( 'NONE', *, *, #24256, .F. ) ;
#53129=ORIENTED_EDGE ( 'NONE', *, *, #11783, .T. ) ;
#53130=CARTESIAN_POINT ( 'NONE',  ( 99.03493788190004921, -39.95360648959476180, 249.4604713219719656 ) ) ;
#53133=DIRECTION ( 'NONE',  ( -1.000000000000000078E-15, 1.000000000000000083E-30, 1.000000000000000000 ) ) ;
#53134=CARTESIAN_POINT ( 'NONE',  ( 49.16670390244661348, -28.27351298637376686, 117.4678068554150485 ) ) ;
#53136=CARTESIAN_POINT ( 'NONE',  ( 104.4428039971878803, -26.59488813107328653, 196.2784824187679362 ) ) ;
#53139=ADVANCED_FACE ( 'NONE', ( #37275 ), #85453, .F. ) ;
#53142=CARTESIAN_POINT ( 'NONE',  ( 98.05938055883913762, -31.39417958322244218, 81.90133956162493689 ) ) ;
#53144=DIRECTION ( 'NONE',  ( -1.042183321081676705E-15, -1.000000000000000000, 0.000000000000000000 ) ) ;
#53145=CIRCLE ( 'NONE', #32879, 0.5000000000000004441 ) ;
#53147=ORIENTED_EDGE ( 'NONE', *, *, #45253, .T. ) ;
#53148=VERTEX_POINT ( 'NONE', #50894 ) ;
#53149=EDGE_CURVE ( 'NONE', #83508, #68103, #17726, .T. ) ;
#53150=CARTESIAN_POINT ( 'NONE',  ( 97.31589304778262317, -39.30609602821370174, 161.5312681493450668 ) ) ;
#53152=CARTESIAN_POINT ( 'NONE',  ( 97.81219835445369881, -40.51719899421586746, 151.6362400511890769 ) ) ;
#53153=CARTESIAN_POINT ( 'NONE',  ( 100.3267271402381624, -32.12451360540737255, 118.6680903695919653 ) ) ;
#53154=CARTESIAN_POINT ( 'NONE',  ( 116.9053397700284478, -41.81689336946376301, 239.4346728949589647 ) ) ;
#53156=CARTESIAN_POINT ( 'NONE',  ( 71.06648329127399677, -18.82844715994099971, 17.92562527591199739 ) ) ;
#53157=ORIENTED_EDGE ( 'NONE', *, *, #6065, .T. ) ;
#53161=VERTEX_POINT ( 'NONE', #78637 ) ;
#53162=ORIENTED_EDGE ( 'NONE', *, *, #64251, .F. ) ;
#53166=EDGE_LOOP ( 'NONE', ( #68688, #801, #48334, #16014 ) ) ;
#53167=CARTESIAN_POINT ( 'NONE',  ( 180.1667039024460166, -28.27351298637340093, -5.074374724088000832 ) ) ;
#53170=CARTESIAN_POINT ( 'NONE',  ( 107.8370078009992028, -28.22187835749811313, 154.4267055423619581 ) ) ;
#53171=CARTESIAN_POINT ( 'NONE',  ( 106.2486884972880432, -26.25648168547507311, 25.13848241876792855 ) ) ;
#53172=CARTESIAN_POINT ( 'NONE',  ( 112.1373864550455153, -28.01170058494273718, 125.6566369152155005 ) ) ;
#53173=ORIENTED_EDGE ( 'NONE', *, *, #34620, .T. ) ;
#53175=ORIENTED_EDGE ( 'NONE', *, *, #42801, .F. ) ;
#53177=VERTEX_POINT ( 'NONE', #38165 ) ;
#53182=VECTOR ( 'NONE', #71300, 1000.000000000000000 ) ;
#53183=VECTOR ( 'NONE', #25864, 1000.000000000000000 ) ;
#53184=CARTESIAN_POINT ( 'NONE',  ( 83.06670390244804025, -51.22944715994108122, 231.5838068554169524 ) ) ;
#53185=ORIENTED_EDGE ( 'NONE', *, *, #55044, .T. ) ;
#53186=CARTESIAN_POINT ( 'NONE',  ( 109.6173639926175269, -25.13086864565549661, 29.90419670448196854 ) ) ;
#53187=CARTESIAN_POINT ( 'NONE',  ( 98.68765228159747949, -43.00544673443933874, 62.83848241876793850 ) ) ;
#53190=DIRECTION ( 'NONE',  ( 0.000000000000000000, 0.000000000000000000, 1.000000000000000000 ) ) ;
#53191=LINE ( 'NONE', #32783, #55430 ) ;
#53192=CARTESIAN_POINT ( 'NONE',  ( 134.0664832912740110, -46.72944715994100306, 1.625625275910997480 ) ) ;
#53193=DIRECTION ( 'NONE',  ( 1.000000000000000000, 0.000000000000000000, 0.000000000000000000 ) ) ;
#53198=CARTESIAN_POINT ( 'NONE',  ( 100.3828542815028015, -28.67117381486349004, 40.62705384733894221 ) ) ;
#53199=CARTESIAN_POINT ( 'NONE',  ( 113.1553867986010857, -26.56284154956258092, 200.6470538473399756 ) ) ;
#53200=CARTESIAN_POINT ( 'NONE',  ( 104.4853289249099362, -46.88901594738546663, 43.37848241876896083 ) ) ;
#53203=CARTESIAN_POINT ( 'NONE',  ( 100.8878723336333536, -44.70055754049414531, 172.0502159399892150 ) ) ;
#53204=DIRECTION ( 'NONE',  ( 0.000000000000000000, 0.000000000000000000, 1.000000000000000000 ) ) ;
#53207=AXIS2_PLACEMENT_3D ( 'NONE', #12813, #40499, #61382 ) ;
#53209=CARTESIAN_POINT ( 'NONE',  ( 115.0889047302471369, -30.61763668945012995, 185.3439586083565871 ) ) ;
#53210=VERTEX_POINT ( 'NONE', #80405 ) ;
#53211=CARTESIAN_POINT ( 'NONE',  ( 108.4470127171751983, -27.04659769318761775, 100.9641967044819779 ) ) ;
#53214=CARTESIAN_POINT ( 'NONE',  ( 97.19046783542286505, -39.99946004141659017, 237.5813395616249579 ) ) ;
#53215=CARTESIAN_POINT ( 'NONE',  ( 172.5664832912740110, -32.07844715994070839, 203.6756252759119832 ) ) ;
#53217=CARTESIAN_POINT ( 'NONE',  ( 116.7487619956327052, -34.15501469173477744, 149.0333341547117527 ) ) ;
#53218=CARTESIAN_POINT ( 'NONE',  ( 134.0664832912739826, -18.72944715994100306, -5.074374724089001809 ) ) ;
#53219=CARTESIAN_POINT ( 'NONE',  ( 107.0667039024479834, -48.82844715994099971, 160.9178068554150229 ) ) ;
#53220=CARTESIAN_POINT ( 'NONE',  ( 133.0080215814357700, -39.26771232012913515, 1.799893082726756965 ) ) ;
#53223=VECTOR ( 'NONE', #47711, 1000.000000000000000 ) ;
#53224=CARTESIAN_POINT ( 'NONE',  ( 105.8036208730406003, -25.68330614323999228, 160.1670538473399574 ) ) ;
#53225=ORIENTED_EDGE ( 'NONE', *, *, #37600, .T. ) ;
#53226=ORIENTED_EDGE ( 'NONE', *, *, #26398, .T. ) ;
#53227=CARTESIAN_POINT ( 'NONE',  ( 108.3613424580152724, -45.52634895430261253, 139.1244404487539725 ) ) ;
#53228=CIRCLE ( 'NONE', #34392, 5.599999999999994316 ) ;
#53229=CARTESIAN_POINT ( 'NONE',  ( 100.1253875378072848, -39.57043109886186727, -1.864374724089012947 ) ) ;
#53230=CARTESIAN_POINT ( 'NONE',  ( 96.91794407517411969, -34.59732685048010126, 257.1737205140059928 ) ) ;
#53231=PLANE ( 'NONE',  #50593 ) ;
#53233=PLANE ( 'NONE',  #88774 ) ;
#53234=EDGE_CURVE ( 'NONE', #27248, #58422, #30953, .T. ) ;
#53237=CARTESIAN_POINT ( 'NONE',  ( 32.15435173583699680, -31.62489322948790971, -5.074374724088000832 ) ) ;
#53238=ADVANCED_FACE ( 'NONE', ( #86770 ), #44514, .T. ) ;
#53239=CARTESIAN_POINT ( 'NONE',  ( 151.0371591254585155, -46.82818131005592477, 129.9678068554149775 ) ) ;
#53240=CARTESIAN_POINT ( 'NONE',  ( 99.30484619187383544, -29.80227926343058797, 190.7470538473399415 ) ) ;
#53241=DIRECTION ( 'NONE',  ( 1.000000000000000078E-15, 1.000000000000000083E-30, -1.000000000000000000 ) ) ;
#53246=CARTESIAN_POINT ( 'NONE',  ( 82.51464772712792239, -19.98222059079053636, 7.138441653514920660 ) ) ;
#53247=CARTESIAN_POINT ( 'NONE',  ( 48.16670390244738797, -26.71338133339277476, 313.9678068554150059 ) ) ;
#53248=DIRECTION ( 'NONE',  ( 1.000000000000000000, 4.163336342344333240E-14, 0.000000000000000000 ) ) ;
#53249=CIRCLE ( 'NONE', #25725, 3.299999999999999822 ) ;
#53250=CARTESIAN_POINT ( 'NONE',  ( 113.2420556116021260, -28.75603552117033956, 94.55263669061166354 ) ) ;
#53251=EDGE_CURVE ( 'NONE', #18458, #48525, #73572, .T. ) ;
#53254=CARTESIAN_POINT ( 'NONE',  ( 118.0511761103140316, -35.49834556997346624, 233.9032443235299752 ) ) ;
#53255=LINE ( 'NONE', #86930, #74908 ) ;
#53257=ORIENTED_EDGE ( 'NONE', *, *, #17723, .T. ) ;
#53258=EDGE_CURVE ( 'NONE', #73498, #686, #24542, .T. ) ;
#53261=CARTESIAN_POINT ( 'NONE',  ( 99.08974868363957000, -42.79574995047337183, 166.8439877233610105 ) ) ;
#53262=CARTESIAN_POINT ( 'NONE',  ( 102.6173380888347282, -29.88584920324980487, 23.35380465530695204 ) ) ;
#53263=CARTESIAN_POINT ( 'NONE',  ( 97.96758126215280527, -41.86240348953004542, 132.7356252759109623 ) ) ;
#53264=CARTESIAN_POINT ( 'NONE',  ( 63.56670390244745050, -47.82844715994014706, 129.9678068554150911 ) ) ;
#53267=CARTESIAN_POINT ( 'NONE',  ( 188.5667039024479834, -62.87844715994099687, 262.0928068554150059 ) ) ;
#53268=DIRECTION ( 'NONE',  ( 0.7071067811864676367, 0.7071067811866273978, 7.071067811864669709E-16 ) ) ;
#53269=ORIENTED_EDGE ( 'NONE', *, *, #67092, .T. ) ;
#53270=ORIENTED_EDGE ( 'NONE', *, *, #72773, .T. ) ;
#53271=CIRCLE ( 'NONE', #12660, 29.00000000000000000 ) ;
#53272=AXIS2_PLACEMENT_3D ( 'NONE', #59858, #52581, #26253 ) ;
#53273=DIRECTION ( 'NONE',  ( 0.000000000000000000, 0.000000000000000000, 1.000000000000000000 ) ) ;
#53274=AXIS2_PLACEMENT_3D ( 'NONE', #58746, #5144, #26039 ) ;
#53278=CARTESIAN_POINT ( 'NONE',  ( 98.15782025887804707, -38.35683565110198145, 50.90480078045794698 ) ) ;
#53279=CARTESIAN_POINT ( 'NONE',  ( 113.1683672335202431, -26.54116819535108363, 204.6470538473399756 ) ) ;
#53280=CARTESIAN_POINT ( 'NONE',  ( 102.8528367378537496, -46.24122135049443472, 177.2441967044819648 ) ) ;
#53281=LINE ( 'NONE', #60110, #8406 ) ;
#53282=CARTESIAN_POINT ( 'NONE',  ( 114.0759046727995241, -46.25395340493271590, 29.08133956162595268 ) ) ;
#53285=ORIENTED_EDGE ( 'NONE', *, *, #57793, .F. ) ;
#53286=AXIS2_PLACEMENT_3D ( 'NONE', #38564, #59449, #18123 ) ;
#53287=ORIENTED_EDGE ( 'NONE', *, *, #85969, .F. ) ;
#53289=VECTOR ( 'NONE', #22618, 1000.000000000000000 ) ;
#53290=EDGE_CURVE ( 'NONE', #60678, #25804, #4087, .T. ) ;
#53291=AXIS2_PLACEMENT_3D ( 'NONE', #86679, #24450, #81219 ) ;
#53292=DIRECTION ( 'NONE',  ( -0.8571673007021110013, 1.917331853055865018E-16, 0.5150380749100563760 ) ) ;
#53293=CARTESIAN_POINT ( 'NONE',  ( 98.86425576617398292, -29.25038657358478744, 230.7261014663869503 ) ) ;
#53295=CARTESIAN_POINT ( 'NONE',  ( 96.64414437497798360, -36.48068628021362514, 196.3070538473399438 ) ) ;
#53296=DIRECTION ( 'NONE',  ( 4.299999999999999979E-14, -1.000000000000000000, 4.400000000000000367E-29 ) ) ;
#53297=CYLINDRICAL_SURFACE ( 'NONE', #74063, 2.117000000000007987 ) ;
#53299=DIRECTION ( 'NONE',  ( 0.000000000000000000, 0.000000000000000000, 1.000000000000000000 ) ) ;
#53301=CARTESIAN_POINT ( 'NONE',  ( 107.0280868098776210, -28.61744286730494125, 277.6356252759110816 ) ) ;
#53303=DIRECTION ( 'NONE',  ( -0.7071067812123270624, -0.7071067811607679721, 0.000000000000000000 ) ) ;
#53306=DIRECTION ( 'NONE',  ( 2.900000000000000265E-14, -2.000000000000000155E-15, 1.000000000000000000 ) ) ;
#53311=CARTESIAN_POINT ( 'NONE',  ( 62.03715912545726496, -23.42818131006022142, 300.4678068554150627 ) ) ;
#53312=CARTESIAN_POINT ( 'NONE',  ( 109.3417050147583041, -26.53289234591626311, 224.9013395616249511 ) ) ;
#53313=CARTESIAN_POINT ( 'NONE',  ( 113.9864041344766861, -28.11035927269328738, 115.5261014663869474 ) ) ;
#53314=CARTESIAN_POINT ( 'NONE',  ( 111.1444126100616927, -27.08769046218140986, 240.7584824187679544 ) ) ;
#53315=DIRECTION ( 'NONE',  ( -1.000000000000000000, 6.036837696399408848E-13, 0.000000000000000000 ) ) ;
#53316=CARTESIAN_POINT ( 'NONE',  ( 156.5667039024482676, -48.82844715993569196, 259.7178068554149490 ) ) ;
#53318=PLANE ( 'NONE',  #21109 ) ;
#53322=EDGE_CURVE ( 'NONE', #21597, #89871, #11349, .T. ) ;
#53325=CARTESIAN_POINT ( 'NONE',  ( 98.49703967840136443, -36.85882374884989332, 135.7609912566479409 ) ) ;
#53329=CARTESIAN_POINT ( 'NONE',  ( 117.6568287320715882, -39.81301747186223139, 134.5889586092439743 ) ) ;
#53330=CARTESIAN_POINT ( 'NONE',  ( 116.3214453605167478, -32.94026287388232532, 159.1356252759109680 ) ) ;
#53331=DIRECTION ( 'NONE',  ( 1.000000000000000000, 1.261617073437676668E-15, 1.261617073437676668E-15 ) ) ;
#53334=LINE ( 'NONE', #73814, #88943 ) ;
#53336=CARTESIAN_POINT ( 'NONE',  ( 107.8187922529720026, -26.97765417004747945, 70.01562527591099183 ) ) ;
#53337=ORIENTED_EDGE ( 'NONE', *, *, #88036, .F. ) ;
#53339=ORIENTED_EDGE ( 'NONE', *, *, #27021, .F. ) ;
#53342=DIRECTION ( 'NONE',  ( 0.000000000000000000, 0.000000000000000000, -1.000000000000000000 ) ) ;
#53343=CARTESIAN_POINT ( 'NONE',  ( 114.0519814166326995, -29.87813257090978070, 145.4441967044819819 ) ) ;
#53344=CARTESIAN_POINT ( 'NONE',  ( 50.97905606905900555, -31.62489322948711035, 313.9678068554150059 ) ) ;
#53346=CARTESIAN_POINT ( 'NONE',  ( 172.5667039024482960, -42.82844715993499563, 180.4678068554150059 ) ) ;
#53348=CARTESIAN_POINT ( 'NONE',  ( 154.4409905298078058, -0.9147987323338667709, 540.9756252759101471 ) ) ;
#53349=CIRCLE ( 'NONE', #31658, 6.571100913904396101 ) ;
#53352=CARTESIAN_POINT ( 'NONE',  ( 103.2867953297129588, -47.09177226061144239, 97.28610146638693834 ) ) ;
#53353=VERTEX_POINT ( 'NONE', #54890 ) ;
#53357=EDGE_CURVE ( 'NONE', #74086, #29576, #62845, .T. ) ;
#53358=CARTESIAN_POINT ( 'NONE',  ( 33.78129701732998313, -35.65087443492610930, -5.074374724088000832 ) ) ;
#53360=AXIS2_PLACEMENT_3D ( 'NONE', #434, #42640, #63558 ) ;
#53361=DIRECTION ( 'NONE',  ( -0.7071067812160284349, 0.7071067811570665995, -7.071067812159980775E-16 ) ) ;
#53362=CARTESIAN_POINT ( 'NONE',  ( 104.2492358271959603, -44.39057208814350020, 140.1138046553059837 ) ) ;
#53364=VERTEX_POINT ( 'NONE', #33135 ) ;
#53365=ORIENTED_EDGE ( 'NONE', *, *, #63519, .F. ) ;
#53366=ADVANCED_FACE ( 'NONE', ( #27212 ), #20413, .T. ) ;
#53367=AXIS2_PLACEMENT_3D ( 'NONE', #43137, #36345, #85415 ) ;
#53368=DIRECTION ( 'NONE',  ( 1.000000000000000000, 0.000000000000000000, 0.000000000000000000 ) ) ;
#53369=EDGE_LOOP ( 'NONE', ( #16747, #51624, #65313, #49773 ) ) ;
#53370=EDGE_LOOP ( 'NONE', ( #27700, #70082, #51388 ) ) ;
#53371=EDGE_CURVE ( 'NONE', #47011, #50271, #26321, .T. ) ;
#53372=DIRECTION ( 'NONE',  ( 0.000000000000000000, 0.000000000000000000, 1.000000000000000000 ) ) ;
#53373=CARTESIAN_POINT ( 'NONE',  ( 107.2166699364993292, -45.61986748510933865, 209.0215833058969963 ) ) ;
#53374=CARTESIAN_POINT ( 'NONE',  ( 172.5664832912729878, -18.82844715994071194, 198.9256252759119832 ) ) ;
#53375=AXIS2_PLACEMENT_3D ( 'NONE', #35063, #76867, #7376 ) ;
#53376=FACE_BOUND ( 'NONE', #42078, .T. ) ;
#53377=AXIS2_PLACEMENT_3D ( 'NONE', #62415, #49673, #77397 ) ;
#53379=ORIENTED_EDGE ( 'NONE', *, *, #34809, .F. ) ;
#53381=ORIENTED_EDGE ( 'NONE', *, *, #65763, .F. ) ;
#53382=ORIENTED_EDGE ( 'NONE', *, *, #20870, .T. ) ;
#53383=CARTESIAN_POINT ( 'NONE',  ( 113.8860208566381544, -32.24350986527421981, 252.1080903695913662 ) ) ;
#53384=CARTESIAN_POINT ( 'NONE',  ( 97.20468889015201341, -31.68559423518837193, 95.96229194257799122 ) ) ;
#53385=CARTESIAN_POINT ( 'NONE',  ( 115.2499566122393588, -44.12502604085376134, 83.25372051400698581 ) ) ;
#53386=CARTESIAN_POINT ( 'NONE',  ( 107.1343666215160937, -28.01736584179905876, 249.5838068554171230 ) ) ;
#53387=DIRECTION ( 'NONE',  ( -0.0001713722456120069274, 0.9999999853157766072, 0.000000000000000000 ) ) ;
#53388=CARTESIAN_POINT ( 'NONE',  ( 181.5667039024459939, -18.82844715994031048, 342.9256252759119548 ) ) ;
#53389=CARTESIAN_POINT ( 'NONE',  ( 113.6142049395107421, -45.63457611473454989, 179.0689586092439640 ) ) ;
#53392=CARTESIAN_POINT ( 'NONE',  ( 91.06648329127500574, -36.72944715993925513, 0.7256252759109548256 ) ) ;
#53394=VECTOR ( 'NONE', #50197, 1000.000000000000000 ) ;
#53395=VERTEX_POINT ( 'NONE', #75817 ) ;
#53396=DIRECTION ( 'NONE',  ( 1.000000000000000078E-15, -1.000000000000000083E-30, -1.000000000000000000 ) ) ;
#53397=CARTESIAN_POINT ( 'NONE',  ( 139.7494832912729805, -1.929447159941395817, 352.4506252759079530 ) ) ;
#53399=CARTESIAN_POINT ( 'NONE',  ( 152.0371591254585155, -47.82818131005588214, 180.4678068554149775 ) ) ;
#53400=AXIS2_PLACEMENT_3D ( 'NONE', #86309, #26307, #13139 ) ;
#53401=CARTESIAN_POINT ( 'NONE',  ( 116.3228127852087113, -32.93589129790882453, 90.13562527591095375 ) ) ;
#53402=CARTESIAN_POINT ( 'NONE',  ( 116.5335121716806981, -32.36339692672488155, 104.1699109901969535 ) ) ;
#53403=FACE_OUTER_BOUND ( 'NONE', #55965, .T. ) ;
#53405=PLANE ( 'NONE',  #56502 ) ;
#53406=CARTESIAN_POINT ( 'NONE',  ( 83.73314995793998605, 12.92155284005730387, 355.9756252759109998 ) ) ;
#53408=CARTESIAN_POINT ( 'NONE',  ( 97.81577456866601494, -40.52739464819840265, 56.63606675467388385 ) ) ;
#53409=CARTESIAN_POINT ( 'NONE',  ( 114.9485010938853122, -29.93956786141553295, 180.3927681330539770 ) ) ;
#53411=CARTESIAN_POINT ( 'NONE',  ( 179.1667039024460166, -26.71338133339251542, 342.9256252759119548 ) ) ;
#53412=ORIENTED_EDGE ( 'NONE', *, *, #67007, .F. ) ;
#53413=DIRECTION ( 'NONE',  ( 0.000000000000000000, 0.000000000000000000, 1.000000000000000000 ) ) ;
#53414=AXIS2_PLACEMENT_3D ( 'NONE', #54265, #55158, #54714 ) ;
#53416=CARTESIAN_POINT ( 'NONE',  ( 99.09586653601625983, -30.55018848384835550, 135.8022601447096633 ) ) ;
#53417=LINE ( 'NONE', #68434, #82539 ) ;
#53418=CARTESIAN_POINT ( 'NONE',  ( 117.5348925983358583, -35.85526142194976273, 253.8927681330537780 ) ) ;
#53419=ORIENTED_EDGE ( 'NONE', *, *, #65287, .F. ) ;
#53420=CARTESIAN_POINT ( 'NONE',  ( 108.2708916590322019, -26.77333427660188292, 194.9803191584221622 ) ) ;
#53421=CARTESIAN_POINT ( 'NONE',  ( 102.3694487442499934, -47.63304195565743981, 283.2527681330539053 ) ) ;
#53422=CARTESIAN_POINT ( 'NONE',  ( 96.62748084391311920, -35.94289726309906996, 142.2670538473399517 ) ) ;
#53423=DIRECTION ( 'NONE',  ( 1.000000000000000000, 4.299999999999999979E-14, 1.000000000000000078E-15 ) ) ;
#53424=VECTOR ( 'NONE', #83081, 1000.000000000000000 ) ;
#53430=EDGE_CURVE ( 'NONE', #16139, #54231, #65523, .T. ) ;
#53432=ORIENTED_EDGE ( 'NONE', *, *, #59277, .T. ) ;
#53434=ORIENTED_EDGE ( 'NONE', *, *, #12068, .T. ) ;
#53435=LINE ( 'NONE', #81202, #4671 ) ;
#53436=CARTESIAN_POINT ( 'NONE',  ( 115.7104945841387007, -43.58108136993639903, 44.30514908543492680 ) ) ;
#53437=DIRECTION ( 'NONE',  ( 0.000000000000000000, 0.000000000000000000, -1.000000000000000000 ) ) ;
#53439=ADVANCED_FACE ( 'NONE', ( #6324 ), #33579, .T. ) ;
#53440=ADVANCED_FACE ( 'NONE', ( #80859 ), #47640, .T. ) ;
#53443=CARTESIAN_POINT ( 'NONE',  ( 99.66831329903114067, -43.01734891331329891, 226.3095626852189639 ) ) ;
#53445=AXIS2_PLACEMENT_3D ( 'NONE', #42296, #75944, #68241 ) ;
#53448=CARTESIAN_POINT ( 'NONE',  ( 77.31648329127399677, -18.72944715994106346, 3.101481641215480867 ) ) ;
#53451=DIRECTION ( 'NONE',  ( 4.299999999999999979E-14, -1.000000000000000000, 0.000000000000000000 ) ) ;
#53452=CARTESIAN_POINT ( 'NONE',  ( 112.1356898331015657, -28.01072921633452850, 274.6563675756979137 ) ) ;
#53453=CARTESIAN_POINT ( 'NONE',  ( 101.5678104218880549, -29.74196420480149072, 12.03872616303996956 ) ) ;
#53455=CARTESIAN_POINT ( 'NONE',  ( 112.1370916094985546, -28.01153175057062228, 174.6566637475011419 ) ) ;
#53456=CARTESIAN_POINT ( 'NONE',  ( 117.4208826026019779, -36.15918394850536544, 273.8822919425783198 ) ) ;
#53458=CARTESIAN_POINT ( 'NONE',  ( 134.0664832912740110, -8.729447159940999512, 293.6356252759119911 ) ) ;
#53459=ORIENTED_EDGE ( 'NONE', *, *, #73126, .F. ) ;
#53460=CARTESIAN_POINT ( 'NONE',  ( 103.2774713272750233, -27.47507576204077040, 56.38571505098142467 ) ) ;
#53462=CARTESIAN_POINT ( 'NONE',  ( 104.2561231690431782, -27.88649476002280636, 53.13951894101997908 ) ) ;
#53464=VECTOR ( 'NONE', #31938, 1000.000000000000000 ) ;
#53465=CARTESIAN_POINT ( 'NONE',  ( 136.6789756616833813, -17.84952872354597275, 6.945088388037557792 ) ) ;
#53467=CARTESIAN_POINT ( 'NONE',  ( 152.0371591254583450, -47.82818131005587503, 237.4678068554150059 ) ) ;
#53468=VERTEX_POINT ( 'NONE', #35362 ) ;
#53469=LINE ( 'NONE', #45326, #72613 ) ;
#53471=VECTOR ( 'NONE', #78571, 1000.000000000000000 ) ;
#53474=CARTESIAN_POINT ( 'NONE',  ( 96.02763272632168423, -37.29765984735794859, 121.3794347997209684 ) ) ;
#53475=ORIENTED_EDGE ( 'NONE', *, *, #35769, .F. ) ;
#53476=EDGE_CURVE ( 'NONE', #45997, #33402, #54191, .T. ) ;
#53477=CARTESIAN_POINT ( 'NONE',  ( 102.6785256587874926, -29.36752282311925200, 84.92670554236298130 ) ) ;
#53479=CARTESIAN_POINT ( 'NONE',  ( 98.34084657651359862, -41.62045863392593503, 87.73252430093928922 ) ) ;
#53480=CARTESIAN_POINT ( 'NONE',  ( 115.6990777838195186, -41.92069145011852527, 124.8272975916109573 ) ) ;
#53483=AXIS2_PLACEMENT_3D ( 'NONE', #75250, #39802, #89782 ) ;
#53485=CARTESIAN_POINT ( 'NONE',  ( 99.27755186283980038, -43.74455535675208040, 52.90991099019698396 ) ) ;
#53488=FACE_OUTER_BOUND ( 'NONE', #55019, .T. ) ;
#53490=CARTESIAN_POINT ( 'NONE',  ( 78.15700282949087807, -20.71057579843893492, 2.232988688762077345 ) ) ;
#53491=EDGE_LOOP ( 'NONE', ( #22854, #65802 ) ) ;
#53493=CIRCLE ( 'NONE', #25979, 2.517500000000005844 ) ;
#53495=ORIENTED_EDGE ( 'NONE', *, *, #35418, .F. ) ;
#53496=CARTESIAN_POINT ( 'NONE',  ( 105.7207279102414077, -46.41719084699269615, 257.4670538473400825 ) ) ;
#53497=CARTESIAN_POINT ( 'NONE',  ( 97.80667890149351251, -40.50516858506785667, 126.6341183413926217 ) ) ;
#53498=CARTESIAN_POINT ( 'NONE',  ( 117.0718954874529345, -35.46248236743199556, 189.9272919416899015 ) ) ;
#53499=CARTESIAN_POINT ( 'NONE',  ( 116.3875994391314634, -31.98201348113981268, 40.20133956162496958 ) ) ;
#53500=FACE_OUTER_BOUND ( 'NONE', #83474, .T. ) ;
#53502=CARTESIAN_POINT ( 'NONE',  ( 168.3595971213390499, -48.62134037882588444, 300.4678068554149490 ) ) ;
#53504=AXIS2_PLACEMENT_3D ( 'NONE', #46549, #87910, #25672 ) ;
#53506=CARTESIAN_POINT ( 'NONE',  ( 45.76696975232824371, -48.62818131006036992, 300.4678068554150059 ) ) ;
#53508=CARTESIAN_POINT ( 'NONE',  ( 118.3173389373707920, -33.08695204176926552, 284.0756252759109657 ) ) ;
#53511=CARTESIAN_POINT ( 'NONE',  ( 78.64593636900363549, -39.09121833381438904, 1.942446336666123985 ) ) ;
#53512=CARTESIAN_POINT ( 'NONE',  ( 113.8315610999352714, -43.69395359880221719, 267.6124198280766677 ) ) ;
#53513=CARTESIAN_POINT ( 'NONE',  ( 152.4409905591762993, -0.9151414768251351362, 394.9756252759102040 ) ) ;
#53514=CARTESIAN_POINT ( 'NONE',  ( 113.3292761056178648, -27.64973082387879444, 85.60800622829195561 ) ) ;
#53516=CARTESIAN_POINT ( 'NONE',  ( 108.3716159000525039, -47.75258262280652843, 162.6822919425769669 ) ) ;
#53517=ORIENTED_EDGE ( 'NONE', *, *, #76452, .F. ) ;
#53520=CARTESIAN_POINT ( 'NONE',  ( 29.56670390244789459, -48.82844715994099971, 129.9678068554150627 ) ) ;
#53521=DIRECTION ( 'NONE',  ( -4.237773401492740281E-14, 1.000000000000000000, 0.000000000000000000 ) ) ;
#53522=DIRECTION ( 'NONE',  ( 0.000000000000000000, 0.000000000000000000, -1.000000000000000000 ) ) ;
#53523=EDGE_LOOP ( 'NONE', ( #35746, #30342, #57375, #79355 ) ) ;
#53524=VECTOR ( 'NONE', #16170, 1000.000000000000000 ) ;
#53525=DIRECTION ( 'NONE',  ( -4.237773401492740281E-14, 1.000000000000000000, 0.000000000000000000 ) ) ;
#53526=CARTESIAN_POINT ( 'NONE',  ( 114.4941961175866254, -28.48069933791915531, 159.5051490854349652 ) ) ;
#53527=ORIENTED_EDGE ( 'NONE', *, *, #71441, .T. ) ;
#53531=CARTESIAN_POINT ( 'NONE',  ( 32.56670390244700997, -22.48495420874110806, -5.074374724088000832 ) ) ;
#53533=CYLINDRICAL_SURFACE ( 'NONE', #87321, 0.2500000000000002220 ) ;
#53534=ORIENTED_EDGE ( 'NONE', *, *, #42294, .F. ) ;
#53538=CARTESIAN_POINT ( 'NONE',  ( 172.5667039024480118, -36.32844715993499563, 180.4678068554150059 ) ) ;
#53539=EDGE_CURVE ( 'NONE', #78479, #59669, #87564, .T. ) ;
#53540=CARTESIAN_POINT ( 'NONE',  ( 37.03715912545342093, -48.62818131006128652, 193.9678068554150911 ) ) ;
#53544=ORIENTED_EDGE ( 'NONE', *, *, #87438, .F. ) ;
#53545=DIRECTION ( 'NONE',  ( 0.000000000000000000, 0.000000000000000000, 1.000000000000000000 ) ) ;
#53548=DIRECTION ( 'NONE',  ( 0.000000000000000000, 1.000000000000000000, 0.000000000000000000 ) ) ;
#53549=EDGE_CURVE ( 'NONE', #72641, #13444, #14532, .T. ) ;
#53551=CARTESIAN_POINT ( 'NONE',  ( 99.09563243660048215, -30.55053396421687850, 105.8023020003378178 ) ) ;
#53553=CARTESIAN_POINT ( 'NONE',  ( 97.06384305289986969, -37.34228284162757205, 181.3752372158707828 ) ) ;
#53554=EDGE_CURVE ( 'NONE', #62031, #41740, #21301, .T. ) ;
#53555=ORIENTED_EDGE ( 'NONE', *, *, #39326, .T. ) ;
#53558=CARTESIAN_POINT ( 'NONE',  ( 116.2522929705882859, -40.08866370952546987, 214.5470538473389581 ) ) ;
#53559=AXIS2_PLACEMENT_3D ( 'NONE', #70770, #23960, #16253 ) ;
#53560=DIRECTION ( 'NONE',  ( -1.000000000000000078E-15, 1.000000000000000000, 0.000000000000000000 ) ) ;
#53561=VERTEX_POINT ( 'NONE', #9030 ) ;
#53562=CARTESIAN_POINT ( 'NONE',  ( 107.5734549334945314, -47.83597508069280480, 38.61276813305297395 ) ) ;
#53563=CARTESIAN_POINT ( 'NONE',  ( 113.6628025804010775, -44.27377612063442314, 53.14812363029078313 ) ) ;
#53565=EDGE_CURVE ( 'NONE', #72320, #34580, #31008, .T. ) ;
#53566=DIRECTION ( 'NONE',  ( 0.000000000000000000, 0.000000000000000000, 1.000000000000000000 ) ) ;
#53569=ORIENTED_EDGE ( 'NONE', *, *, #14720, .F. ) ;
#53570=ORIENTED_EDGE ( 'NONE', *, *, #22428, .T. ) ;
#53572=CARTESIAN_POINT ( 'NONE',  ( 104.8088860400571463, -27.60915219823615985, 236.6892023535159808 ) ) ;
#53575=CARTESIAN_POINT ( 'NONE',  ( 98.34985891762011079, -31.65658480093746974, 80.90645860845471304 ) ) ;
#53576=FACE_OUTER_BOUND ( 'NONE', #34843, .T. ) ;
#53578=VECTOR ( 'NONE', #86471, 1000.000000000000114 ) ;
#53579=DIRECTION ( 'NONE',  ( -4.237773401492740281E-14, 1.000000000000000000, 0.000000000000000000 ) ) ;
#53582=CARTESIAN_POINT ( 'NONE',  ( 117.3847603239957635, -38.21947720531817083, 28.71276813305395592 ) ) ;
#53583=ORIENTED_EDGE ( 'NONE', *, *, #2014, .T. ) ;
#53585=CARTESIAN_POINT ( 'NONE',  ( 99.35983957736841887, -39.50259174935074213, 264.4195189410201579 ) ) ;
#53586=EDGE_CURVE ( 'NONE', #72918, #52237, #59974, .T. ) ;
#53587=VECTOR ( 'NONE', #83873, 1000.000000000000000 ) ;
#53588=DIRECTION ( 'NONE',  ( -0.000000000000000000, 1.000000000000000000, 0.000000000000000000 ) ) ;
#53589=CARTESIAN_POINT ( 'NONE',  ( 102.0969121991172557, -45.15362633196983211, 162.1527681330539679 ) ) ;
#53591=CARTESIAN_POINT ( 'NONE',  ( 63.56670390244796920, -40.82844715994016127, 300.4678068554150627 ) ) ;
#53592=DIRECTION ( 'NONE',  ( 0.000000000000000000, 0.000000000000000000, 1.000000000000000000 ) ) ;
#53594=CARTESIAN_POINT ( 'NONE',  ( 117.9780035659441495, -34.69567636304840619, 199.9851490854349549 ) ) ;
#53595=VECTOR ( 'NONE', #22183, 1000.000000000000000 ) ;
#53597=CIRCLE ( 'NONE', #2873, 6.571100913904396990 ) ;
#53598=EDGE_LOOP ( 'NONE', ( #78652, #83921, #72163, #40005, #53128, #13688, #74431, #13041, #81386, #84717, #16413, #82532 ) ) ;
#53599=CARTESIAN_POINT ( 'NONE',  ( 95.30017103329034001, -34.95040006919153086, 67.20705384733894050 ) ) ;
#53601=ORIENTED_EDGE ( 'NONE', *, *, #37722, .F. ) ;
#53602=EDGE_LOOP ( 'NONE', ( #64871, #23123, #55967, #73137 ) ) ;
#53603=ORIENTED_EDGE ( 'NONE', *, *, #56785, .T. ) ;
#53604=CIRCLE ( 'NONE', #37707, 1.000000000000000888 ) ;
#53608=CARTESIAN_POINT ( 'NONE',  ( 112.9083776113003665, -30.34675141079074834, 152.2928522743529527 ) ) ;
#53609=CARTESIAN_POINT ( 'NONE',  ( 96.10234264863321130, -35.15692507338371087, 222.2251490854349640 ) ) ;
#53613=VECTOR ( 'NONE', #48815, 1000.000000000000000 ) ;
#53614=CARTESIAN_POINT ( 'NONE',  ( 136.8164832912740110, -36.72944715994100306, 3.101481641215515950 ) ) ;
#53615=ORIENTED_EDGE ( 'NONE', *, *, #74212, .T. ) ;
#53618=VERTEX_POINT ( 'NONE', #15835 ) ;
#53619=ORIENTED_EDGE ( 'NONE', *, *, #67211, .T. ) ;
#53620=CARTESIAN_POINT ( 'NONE',  ( 127.0664832912740394, -54.72944906728950798, -4.824374724089008915 ) ) ;
#53621=DIRECTION ( 'NONE',  ( 0.000000000000000000, 1.000000000000000000, 0.000000000000000000 ) ) ;
#53624=CARTESIAN_POINT ( 'NONE',  ( 108.6057327191364976, -28.29838476132584191, 164.3552769709339714 ) ) ;
#53625=CARTESIAN_POINT ( 'NONE',  ( 103.4619715496438630, -25.38765309446003116, 55.32133956162594046 ) ) ;
#53627=ORIENTED_EDGE ( 'NONE', *, *, #642, .F. ) ;
#53628=LINE ( 'NONE', #81835, #81849 ) ;
#53629=VERTEX_POINT ( 'NONE', #66190 ) ;
#53630=DIRECTION ( 'NONE',  ( 1.000000000000000000, -9.104347601086962483E-12, 0.000000000000000000 ) ) ;
#53632=CARTESIAN_POINT ( 'NONE',  ( 104.4230182660072472, -27.06115666640247852, 166.2882327781027527 ) ) ;
#53634=CARTESIAN_POINT ( 'NONE',  ( 111.5308273356922797, -45.68399439548272056, 132.9444956965449194 ) ) ;
#53636=DIRECTION ( 'NONE',  ( -1.000000000000000000, -2.756263715554006823E-15, 0.000000000000000000 ) ) ;
#53638=CARTESIAN_POINT ( 'NONE',  ( 97.05407301568530443, -33.74649485729950271, 31.09562527591097592 ) ) ;
#53639=CARTESIAN_POINT ( 'NONE',  ( 118.7813114821712901, -34.63805691389952557, 44.96705384733895272 ) ) ;
#53640=( BOUNDED_CURVE ( )  B_SPLINE_CURVE ( 3, ( #73273, #72840, #23381, #24248 ),
 .UNSPECIFIED., .F., .F. ) 
 B_SPLINE_CURVE_WITH_KNOTS ( ( 4, 4 ),
 ( 1.570796326806955134, 3.141592653599507123 ),
 .UNSPECIFIED. ) 
 CURVE ( )  GEOMETRIC_REPRESENTATION_ITEM ( )  RATIONAL_B_SPLINE_CURVE ( ( 1.000000000000000000, 0.8047378541249177175, 0.8047378541249177175, 1.000000000000000000 ) ) 
 REPRESENTATION_ITEM ( '' )  );
#53641=EDGE_CURVE ( 'NONE', #33706, #48061, #57602, .T. ) ;
#53642=DIRECTION ( 'NONE',  ( -1.000000000000000000, -4.299999999999999979E-14, -1.000000000000000078E-15 ) ) ;
#53646=FACE_OUTER_BOUND ( 'NONE', #15390, .T. ) ;
#53647=VECTOR ( 'NONE', #64013, 1000.000000000000000 ) ;
#53649=CARTESIAN_POINT ( 'NONE',  ( 103.5958499319329036, -27.24642460418891687, 121.3544414785948788 ) ) ;
#53652=ORIENTED_EDGE ( 'NONE', *, *, #54670, .T. ) ;
#53653=CARTESIAN_POINT ( 'NONE',  ( 115.9290394997688480, -31.15613903141374763, 34.27276813305396530 ) ) ;
#53654=CARTESIAN_POINT ( 'NONE',  ( 96.19138854833354912, -32.02127024200479610, 207.0013395616249738 ) ) ;
#53655=CARTESIAN_POINT ( 'NONE',  ( 99.48587976144928291, -43.91775078298940116, 77.92991099019597812 ) ) ;
#53658=DIRECTION ( 'NONE',  ( 0.000000000000000000, 1.000000000000000000, 0.000000000000000000 ) ) ;
#53659=AXIS2_PLACEMENT_3D ( 'NONE', #19021, #12213, #39902 ) ;
#53660=EDGE_CURVE ( 'NONE', #21597, #16304, #30796, .T. ) ;
#53661=DIRECTION ( 'NONE',  ( 1.000000000000000000, 0.000000000000000000, 0.000000000000000000 ) ) ;
#53663=EDGE_CURVE ( 'NONE', #30378, #67268, #77437, .T. ) ;
#53664=CARTESIAN_POINT ( 'NONE',  ( 114.1038288540492687, -43.56973530630599356, 94.21276813305296116 ) ) ;
#53667=ORIENTED_EDGE ( 'NONE', *, *, #50388, .F. ) ;
#53668=CARTESIAN_POINT ( 'NONE',  ( 99.55514648348079731, -29.48070623161996551, 246.7156252759109520 ) ) ;
#53669=CARTESIAN_POINT ( 'NONE',  ( 115.0368136288728067, -42.90904383531166388, 254.3042057836352114 ) ) ;
#53670=CARTESIAN_POINT ( 'NONE',  ( 116.3173461584868278, -32.93718857426866720, 59.13562527591098217 ) ) ;
#53672=PLANE ( 'NONE',  #2235 ) ;
#53673=CYLINDRICAL_SURFACE ( 'NONE', #16642, 11.45913725231036118 ) ;
#53674=EDGE_CURVE ( 'NONE', #19968, #36283, #4890, .T. ) ;
#53678=CARTESIAN_POINT ( 'NONE',  ( 108.2857792741417882, -47.02760743735412063, 162.6822919425779617 ) ) ;
#53681=CARTESIAN_POINT ( 'NONE',  ( 105.2783438540041061, -26.81616000048136428, 121.6501547344689698 ) ) ;
#53683=CARTESIAN_POINT ( 'NONE',  ( 103.3362402991319584, -47.20309360805207177, 248.3041967044819387 ) ) ;
#53684=CARTESIAN_POINT ( 'NONE',  ( 172.5664832912740110, -9.303447159940999356, 258.9256252759120116 ) ) ;
#53686=CONICAL_SURFACE ( 'NONE', #72605, 1.258749999999999369, 1.029744258676650093 ) ;
#53687=CARTESIAN_POINT ( 'NONE',  ( 37.03715912545347777, -48.62818131006128652, 129.9678068554150911 ) ) ;
#53689=LINE ( 'NONE', #19207, #5770 ) ;
#53691=CARTESIAN_POINT ( 'NONE',  ( 100.0229104548316172, -27.23016881827663127, 185.5841967044829630 ) ) ;
#53693=ORIENTED_EDGE ( 'NONE', *, *, #73320, .T. ) ;
#53694=VERTEX_POINT ( 'NONE', #68000 ) ;
#53697=CARTESIAN_POINT ( 'NONE',  ( 41.56648329127399677, 0.2215528400590013880, 81.04262527591200183 ) ) ;
#53698=CARTESIAN_POINT ( 'NONE',  ( 194.0371591254582313, -46.82818131005407736, 313.9678068554149490 ) ) ;
#53699=DIRECTION ( 'NONE',  ( 4.194175870806139918E-14, -1.000000000000000000, 0.000000000000000000 ) ) ;
#53700=EDGE_CURVE ( 'NONE', #86147, #74870, #16501, .T. ) ;
#53701=AXIS2_PLACEMENT_3D ( 'NONE', #56057, #7932, #62446 ) ;
#53703=ORIENTED_EDGE ( 'NONE', *, *, #30229, .F. ) ;
#53705=CARTESIAN_POINT ( 'NONE',  ( 97.09604340039788895, -41.50117806558871791, 216.6937205140059461 ) ) ;
#53706=DIRECTION ( 'NONE',  ( -0.9254794337955620787, -0.3787978585227822492, 0.000000000000000000 ) ) ;
#53710=FACE_OUTER_BOUND ( 'NONE', #51154, .T. ) ;
#53712=CARTESIAN_POINT ( 'NONE',  ( 114.4327864602578870, -33.21273682179715792, 16.99951894101997496 ) ) ;
#53713=CARTESIAN_POINT ( 'NONE',  ( 98.44073678691454177, -30.83591204966533894, 116.8499109901969604 ) ) ;
#53714=VECTOR ( 'NONE', #46746, 1000.000000000000000 ) ;
#53718=DIRECTION ( 'NONE',  ( 0.000000000000000000, 0.000000000000000000, -1.000000000000000000 ) ) ;
#53719=CARTESIAN_POINT ( 'NONE',  ( 82.81181082189912956, -18.54506369575707225, 6.756870620000345440 ) ) ;
#53720=ORIENTED_EDGE ( 'NONE', *, *, #11642, .F. ) ;
#53724=CARTESIAN_POINT ( 'NONE',  ( 167.6524903400755875, -48.32844715993520879, 129.9678068554150059 ) ) ;
#53725=ORIENTED_EDGE ( 'NONE', *, *, #78526, .F. ) ;
#53727=CARTESIAN_POINT ( 'NONE',  ( 97.81136857581559241, -40.51756142658395987, 157.6353372204761456 ) ) ;
#53728=CARTESIAN_POINT ( 'NONE',  ( 116.6246688045503248, -35.02307164793359107, 48.38956268521998538 ) ) ;
#53729=AXIS2_PLACEMENT_3D ( 'NONE', #30862, #87611, #2722 ) ;
#53730=CARTESIAN_POINT ( 'NONE',  ( 117.2491520020922451, -41.08934384016853869, 213.5165776568629781 ) ) ;
#53731=CARTESIAN_POINT ( 'NONE',  ( 107.9164806882189396, -47.13338536194959971, 177.6413395616249886 ) ) ;
#53732=CARTESIAN_POINT ( 'NONE',  ( 112.5159765079568928, -45.21572303546594895, 23.03180688963041689 ) ) ;
#53733=CARTESIAN_POINT ( 'NONE',  ( 102.7643194828038702, -25.71402177940534983, 16.37276813305293999 ) ) ;
#53734=DIRECTION ( 'NONE',  ( 4.299999999999999979E-14, -1.000000000000000000, 4.400000000000000367E-29 ) ) ;
#53735=CARTESIAN_POINT ( 'NONE',  ( 181.9694315774339941, -34.03355364505720360, -5.074374724088000832 ) ) ;
#53737=ORIENTED_EDGE ( 'NONE', *, *, #52638, .T. ) ;
#53739=CARTESIAN_POINT ( 'NONE',  ( 116.0932472193867966, -42.03267250216092776, 238.4041967044829562 ) ) ;
#53741=CARTESIAN_POINT ( 'NONE',  ( 98.55109871784688380, -44.97133477160940629, 191.9384824187679612 ) ) ;
#53742=DIRECTION ( 'NONE',  ( -4.237773401492740281E-14, 1.000000000000000000, 0.000000000000000000 ) ) ;
#53744=CARTESIAN_POINT ( 'NONE',  ( 112.0650724570131018, -45.48886861298491624, 23.98971456471283048 ) ) ;
#53745=CARTESIAN_POINT ( 'NONE',  ( 115.3228590304952519, -42.51629437446412396, 29.34178388814013516 ) ) ;
#53747=CARTESIAN_POINT ( 'NONE',  ( 98.00444231558566344, -38.77556477352123920, 277.6356252759110248 ) ) ;
#53748=FACE_OUTER_BOUND ( 'NONE', #23747, .T. ) ;
#53749=CARTESIAN_POINT ( 'NONE',  ( 104.4078422938526387, -46.45802063222308931, 173.3647710761513281 ) ) ;
#53753=LINE ( 'NONE', #39259, #83263 ) ;
#53754=CIRCLE ( 'NONE', #62469, 2.517500000000005844 ) ;
#53755=EDGE_CURVE ( 'NONE', #27930, #12659, #26213, .T. ) ;
#53757=LINE ( 'NONE', #89217, #80819 ) ;
#53759=CARTESIAN_POINT ( 'NONE',  ( 101.1484327817356927, -28.92773574981692164, 195.5838068554168672 ) ) ;
#53760=ORIENTED_EDGE ( 'NONE', *, *, #55194, .F. ) ;
#53761=EDGE_CURVE ( 'NONE', #47300, #87803, #53891, .T. ) ;
#53762=CARTESIAN_POINT ( 'NONE',  ( 83.06670390244796920, -67.87844715994100397, 207.5838068554149913 ) ) ;
#53763=CARTESIAN_POINT ( 'NONE',  ( 115.8739437555936718, -44.69579237430344421, 233.2413395616259493 ) ) ;
#53764=CARTESIAN_POINT ( 'NONE',  ( 117.1635299909640082, -34.13481127188234865, 120.0270538473389479 ) ) ;
#53765=CARTESIAN_POINT ( 'NONE',  ( 109.2209341577003698, -48.43284210327079364, 273.7213395616253706 ) ) ;
#53766=CARTESIAN_POINT ( 'NONE',  ( 21.03715912545744615, -47.82818131006197149, 129.9678068554150627 ) ) ;
#53767=DIRECTION ( 'NONE',  ( 0.000000000000000000, -1.000000000000000000, 0.000000000000000000 ) ) ;
#53768=AXIS2_PLACEMENT_3D ( 'NONE', #11052, #17433, #23813 ) ;
#53769=FACE_OUTER_BOUND ( 'NONE', #83910, .T. ) ;
#53771=DIRECTION ( 'NONE',  ( 1.000000000000000000, -4.238735976179846264E-15, 0.000000000000000000 ) ) ;
#53772=CARTESIAN_POINT ( 'NONE',  ( 133.1862368104746110, -21.33528726900525641, 1.744847506585589292 ) ) ;
#53773=EDGE_CURVE ( 'NONE', #14469, #33687, #25168, .T. ) ;
#53774=VECTOR ( 'NONE', #26379, 1000.000000000000000 ) ;
#53778=CARTESIAN_POINT ( 'NONE',  ( 98.54925023078828872, -36.08769725913535353, 145.6895626852199541 ) ) ;
#53781=CARTESIAN_POINT ( 'NONE',  ( 97.07206807804939785, -35.37847778407284949, 91.21778693248904801 ) ) ;
#53782=CARTESIAN_POINT ( 'NONE',  ( 117.1424269838422987, -34.14023410701943817, 120.0270538473389479 ) ) ;
#53783=CARTESIAN_POINT ( 'NONE',  ( 64.68306507141296890, -72.55818180160879649, 361.9756252759101471 ) ) ;
#53784=CARTESIAN_POINT ( 'NONE',  ( 90.44969454456405344, -17.59493780205721691, 219.5838068554169809 ) ) ;
#53785=AXIS2_PLACEMENT_3D ( 'NONE', #27557, #39827, #67544 ) ;
#53788=CARTESIAN_POINT ( 'NONE',  ( 111.6283393632454448, -28.07768985461828848, 59.68991099019693536 ) ) ;
#53789=ORIENTED_EDGE ( 'NONE', *, *, #67919, .F. ) ;
#53790=ORIENTED_EDGE ( 'NONE', *, *, #6225, .T. ) ;
#53791=VECTOR ( 'NONE', #24966, 1000.000000000000000 ) ;
#53792=ORIENTED_EDGE ( 'NONE', *, *, #54280, .T. ) ;
#53794=CARTESIAN_POINT ( 'NONE',  ( 98.82386243697619932, -31.40279086140556331, 141.8699109901959616 ) ) ;
#53796=DIRECTION ( 'NONE',  ( -0.9254794337955620787, -0.3787978585227822492, 0.000000000000000000 ) ) ;
#53799=DIRECTION ( 'NONE',  ( 1.000000000000000000, 4.299999999999999979E-14, 1.000000000000000078E-15 ) ) ;
#53800=DIRECTION ( 'NONE',  ( 1.000000000000000078E-15, -1.000000000000000083E-30, -1.000000000000000000 ) ) ;
#53802=CARTESIAN_POINT ( 'NONE',  ( 96.05879824974435621, -41.05137697672059716, 96.62419670448197451 ) ) ;
#53804=CIRCLE ( 'NONE', #55240, 0.5000000000000004441 ) ;
#53805=ORIENTED_EDGE ( 'NONE', *, *, #63562, .F. ) ;
#53806=PLANE ( 'NONE',  #80753 ) ;
#53810=CARTESIAN_POINT ( 'NONE',  ( 115.3951208896509399, -39.08203659613434411, 141.4376141791150019 ) ) ;
#53812=ORIENTED_EDGE ( 'NONE', *, *, #70518, .F. ) ;
#53813=ORIENTED_EDGE ( 'NONE', *, *, #77936, .T. ) ;
#53815=AXIS2_PLACEMENT_3D ( 'NONE', #68670, #61831, #74578 ) ;
#53816=CARTESIAN_POINT ( 'NONE',  ( 135.4847699230876117, -21.08750326149013077, 1.944748881540630858 ) ) ;
#53817=EDGE_LOOP ( 'NONE', ( #22844, #72860, #74976, #39336 ) ) ;
#53818=ORIENTED_EDGE ( 'NONE', *, *, #80261, .F. ) ;
#53820=CARTESIAN_POINT ( 'NONE',  ( 101.6018043438793796, -28.26729678577900273, 216.9644404487539475 ) ) ;
#53822=VECTOR ( 'NONE', #8675, 1000.000000000000000 ) ;
#53824=DIRECTION ( 'NONE',  ( 0.000000000000000000, 0.000000000000000000, -1.000000000000000000 ) ) ;
#53825=ORIENTED_EDGE ( 'NONE', *, *, #15451, .F. ) ;
#53826=ORIENTED_EDGE ( 'NONE', *, *, #8261, .T. ) ;
#53829=DIRECTION ( 'NONE',  ( -1.000000000000000000, -4.163336342344275811E-14, 0.000000000000000000 ) ) ;
#53830=VERTEX_POINT ( 'NONE', #28449 ) ;
#53832=CARTESIAN_POINT ( 'NONE',  ( 102.0474437309886184, -43.16675777147634108, 229.8680903695919540 ) ) ;
#53833=CARTESIAN_POINT ( 'NONE',  ( 108.0362122550155135, -25.69517931502184993, 109.9946728949589811 ) ) ;
#53834=CARTESIAN_POINT ( 'NONE',  ( 117.9659426345832713, -38.42225801833666310, 68.69181575210198787 ) ) ;
#53835=CARTESIAN_POINT ( 'NONE',  ( 99.04747455419412461, -37.07517787504866646, 249.5838068554172651 ) ) ;
#53836=CARTESIAN_POINT ( 'NONE',  ( 132.4277392773762472, -16.51875925607410167, 7.791169830161673637 ) ) ;
#53837=CARTESIAN_POINT ( 'NONE',  ( 97.81168895331838087, -40.51742574516882200, 287.6356252759109680 ) ) ;
#53838=CARTESIAN_POINT ( 'NONE',  ( 116.3502490628398647, -44.09465650233049416, 194.2927681330539542 ) ) ;
#53839=CARTESIAN_POINT ( 'NONE',  ( 97.81252181335722184, -40.51708140359354360, 276.6353344664656220 ) ) ;
#53841=DIRECTION ( 'NONE',  ( 2.900000000000000265E-14, -2.000000000000000155E-15, 1.000000000000000000 ) ) ;
#53843=CIRCLE ( 'NONE', #68347, 0.5000000000000079936 ) ;
#53844=ORIENTED_EDGE ( 'NONE', *, *, #28959, .T. ) ;
#53845=FACE_OUTER_BOUND ( 'NONE', #22951, .T. ) ;
#53846=EDGE_LOOP ( 'NONE', ( #24042, #46289, #32455, #24957 ) ) ;
#53848=DIRECTION ( 'NONE',  ( 8.755702086949183871E-16, 1.000000000000000000, 0.000000000000000000 ) ) ;
#53849=CARTESIAN_POINT ( 'NONE',  ( 99.09478958797689074, -30.55165821669924497, 91.80241262291944793 ) ) ;
#53850=CARTESIAN_POINT ( 'NONE',  ( 98.33613682261365341, -42.42752411612296015, 101.7870538473399620 ) ) ;
#53852=CARTESIAN_POINT ( 'NONE',  ( 172.5664832912729878, -27.82844715994070484, 74.17562527591199739 ) ) ;
#53853=DIRECTION ( 'NONE',  ( -2.127927463864879951E-15, 0.000000000000000000, -1.000000000000000000 ) ) ;
#53854=CARTESIAN_POINT ( 'NONE',  ( 116.3212776292299253, -32.94146857471393730, 145.1356252759109680 ) ) ;
#53856=CARTESIAN_POINT ( 'NONE',  ( 100.6510976905702393, -26.79511100149722935, 216.5327681330539633 ) ) ;
#53857=DIRECTION ( 'NONE',  ( 0.000000000000000000, 1.000000000000000000, 0.000000000000000000 ) ) ;
#53859=FACE_OUTER_BOUND ( 'NONE', #1849, .T. ) ;
#53860=VERTEX_POINT ( 'NONE', #20747 ) ;
#53862=DIRECTION ( 'NONE',  ( -2.108538789381372925E-16, 0.5150380749100580413, 0.8571673007021100021 ) ) ;
#53863=EDGE_CURVE ( 'NONE', #26572, #81096, #69349, .T. ) ;
#53864=LINE ( 'NONE', #55210, #16665 ) ;
#53865=EDGE_CURVE ( 'NONE', #55247, #61174, #23773, .T. ) ;
#53866=FACE_OUTER_BOUND ( 'NONE', #23586, .T. ) ;
#53867=B_SPLINE_CURVE_WITH_KNOTS ( 'NONE', 3,
 ( #38658, #79575, #59536, #45017, #10514, #38219, #65912, #80460, #3699, #87271, #25037, #31392, #59089, #86824, #52257, #80022, #17776, #10952, #72304, #45454, #18219, #45899, #2373, #9623, #30073, #57767, #50949, #65035, #51378, #23718, #79127 ),
 .UNSPECIFIED., .F., .F.,
 ( 4, 2, 2, 1, 2, 2, 2, 2, 2, 2, 2, 1, 1, 2, 2, 2, 4 ),
 ( 0.000000000000000000, 0.06250000000002874090, 0.09375000000004299339, 0.1093750000000480727, 0.1171875000000508066, 0.1250000000000535405, 0.1875000000000552891, 0.2187500000000547895, 0.2500000000000542899, 0.3125000000000500711, 0.3437500000000475175, 0.3593750000000461853, 0.3671875000000460187, 0.3710937500000459077, 0.3750000000000457967, 0.4375000000000229261, 0.5000000000000000000 ),
 .UNSPECIFIED. ) ;
#53870=CARTESIAN_POINT ( 'NONE',  ( 111.6277637875740538, -46.15289590646231943, 247.9356252759109509 ) ) ;
#53871=VERTEX_POINT ( 'NONE', #42513 ) ;
#53873=CARTESIAN_POINT ( 'NONE',  ( 113.1467068653160908, -28.75413120684047996, 194.5579722171665082 ) ) ;
#53874=CARTESIAN_POINT ( 'NONE',  ( 112.3492874949901932, -28.18945346073204306, 285.6356252759109680 ) ) ;
#53875=CARTESIAN_POINT ( 'NONE',  ( 118.9531587402301511, -36.16547954148851574, 114.8641967044819694 ) ) ;
#53876=LINE ( 'NONE', #60257, #17139 ) ;
#53877=CARTESIAN_POINT ( 'NONE',  ( 82.53070037946083914, -37.95069274173288676, 7.120636252906606956 ) ) ;
#53879=CARTESIAN_POINT ( 'NONE',  ( 25.56670390244748248, -48.82844715994178841, 137.2178068554150627 ) ) ;
#53880=CARTESIAN_POINT ( 'NONE',  ( 97.81170999939396893, -40.51745679428447744, 191.6351607553995393 ) ) ;
#53881=CARTESIAN_POINT ( 'NONE',  ( 73.06648329127401098, -8.729447159940974643, 14.82207188531764608 ) ) ;
#53885=EDGE_CURVE ( 'NONE', #76504, #6713, #48873, .T. ) ;
#53889=CARTESIAN_POINT ( 'NONE',  ( 111.4063510358307241, -46.18429848020799255, 23.91848241876792969 ) ) ;
#53891=LINE ( 'NONE', #19402, #80315 ) ;
#53893=DIRECTION ( 'NONE',  ( 0.000000000000000000, 0.000000000000000000, -1.000000000000000000 ) ) ;
#53896=CARTESIAN_POINT ( 'NONE',  ( 98.83240126976802742, -34.45875894154226415, 250.5352769709339782 ) ) ;
#53899=ORIENTED_EDGE ( 'NONE', *, *, #20668, .T. ) ;
#53900=AXIS2_PLACEMENT_3D ( 'NONE', #88642, #26399, #66038 ) ;
#53902=FACE_OUTER_BOUND ( 'NONE', #43053, .T. ) ;
#53904=CARTESIAN_POINT ( 'NONE',  ( 36.23715912545344509, -47.82818131006131779, 129.9678068554150911 ) ) ;
#53905=CARTESIAN_POINT ( 'NONE',  ( 98.57375871705461634, -34.19924797442281772, 27.52729759161093170 ) ) ;
#53908=CARTESIAN_POINT ( 'NONE',  ( 99.87094702832891358, -29.26198151734318742, 265.6746728949591443 ) ) ;
#53909=CARTESIAN_POINT ( 'NONE',  ( 177.8371591254545194, -47.82818131005477369, 180.4678068554150343 ) ) ;
#53911=VERTEX_POINT ( 'NONE', #35711 ) ;
#53912=LINE ( 'NONE', #40753, #21429 ) ;
#53913=LINE ( 'NONE', #84812, #30797 ) ;
#53914=EDGE_CURVE ( 'NONE', #36668, #75973, #15288, .T. ) ;
#53915=CARTESIAN_POINT ( 'NONE',  ( 102.4274780401303531, -29.97946060242000144, 48.37380465530593909 ) ) ;
#53917=VECTOR ( 'NONE', #40795, 1000.000000000000000 ) ;
#53919=EDGE_CURVE ( 'NONE', #24368, #6819, #34817, .T. ) ;
#53920=DIRECTION ( 'NONE',  ( 0.000000000000000000, 0.000000000000000000, 1.000000000000000000 ) ) ;
#53922=CARTESIAN_POINT ( 'NONE',  ( 100.8874379353258064, -44.70019678655637563, 193.0521937219151312 ) ) ;
#53927=CARTESIAN_POINT ( 'NONE',  ( 114.7075677164476986, -44.71649393962480445, 113.1718157521009687 ) ) ;
#53928=EDGE_LOOP ( 'NONE', ( #5849, #32764, #75443, #42522 ) ) ;
#53929=CARTESIAN_POINT ( 'NONE',  ( 100.2301541646454552, -41.85006585248910937, 66.26099125664796929 ) ) ;
#53930=AXIS2_PLACEMENT_3D ( 'NONE', #46497, #81960, #12011 ) ;
#53931=CARTESIAN_POINT ( 'NONE',  ( 97.83394025066695576, -40.57137221588841669, 87.63980401892214900 ) ) ;
#53932=CARTESIAN_POINT ( 'NONE',  ( 99.64559906019141522, -41.57287113897975672, 98.21872616303994619 ) ) ;
#53934=DIRECTION ( 'NONE',  ( -0.9254794337955620787, -0.3787978585227822492, 0.000000000000000000 ) ) ;
#53935=CARTESIAN_POINT ( 'NONE',  ( 116.6948211927369812, -32.58525784656897883, 75.14991099019697174 ) ) ;
#53936=CARTESIAN_POINT ( 'NONE',  ( 97.33787651319606482, -34.07092125289876350, 182.1152721348323666 ) ) ;
#53937=CARTESIAN_POINT ( 'NONE',  ( 104.4079846621045107, -46.45805526528280183, 257.3646764449513853 ) ) ;
#53938=EDGE_LOOP ( 'NONE', ( #33620, #53270, #52706, #27616, #43893, #60319, #56186, #10269, #78208, #8703, #32721, #59017, #45319, #57182, #3170, #64162, #89521, #33157, #61424, #41267, #24723, #34097, #66571, #33119, #18382, #44400, #21210, #546, #61721, #35197, #11089, #79091, #49238, #28294, #3806, #12948, #86881, #37632, #69231, #14257, #81869, #6158, #56900, #60521, #75868, #61803, #50561, #41594 ) ) ;
#53939=EDGE_CURVE ( 'NONE', #58383, #49742, #42605, .T. ) ;
#53941=ORIENTED_EDGE ( 'NONE', *, *, #57358, .F. ) ;
#53943=CARTESIAN_POINT ( 'NONE',  ( 194.0371591254572650, -24.42818131005417825, 313.9678068554149490 ) ) ;
#53944=ORIENTED_EDGE ( 'NONE', *, *, #62706, .T. ) ;
#53945=CARTESIAN_POINT ( 'NONE',  ( 117.9377692877172450, -39.05906590213767515, 258.6584824187686422 ) ) ;
#53946=CARTESIAN_POINT ( 'NONE',  ( 100.8735899011331014, -45.91031909761725416, 148.0918157521009562 ) ) ;
#53949=CARTESIAN_POINT ( 'NONE',  ( 113.8563929230154912, -44.64017497981368621, 104.1413395616249744 ) ) ;
#53951=ORIENTED_EDGE ( 'NONE', *, *, #56980, .T. ) ;
#53954=AXIS2_PLACEMENT_3D ( 'NONE', #40824, #61707, #89442 ) ;
#53955=ORIENTED_EDGE ( 'NONE', *, *, #53097, .T. ) ;
#53956=AXIS2_PLACEMENT_3D ( 'NONE', #8961, #16655, #36660 ) ;
#53957=DIRECTION ( 'NONE',  ( -0.000000000000000000, -0.000000000000000000, -1.000000000000000000 ) ) ;
#53958=LINE ( 'NONE', #5857, #61452 ) ;
#53959=CARTESIAN_POINT ( 'NONE',  ( 106.1402962346845982, -47.72062544595571154, 262.4975300378158636 ) ) ;
#53962=CARTESIAN_POINT ( 'NONE',  ( 95.60734603896362671, -36.72944715994100306, 293.2242906452868851 ) ) ;
#53963=CARTESIAN_POINT ( 'NONE',  ( 151.0371591254573218, -24.95799193692592866, 300.4678068554149490 ) ) ;
#53964=CARTESIAN_POINT ( 'NONE',  ( 114.3094922386577110, -31.29331878451978355, 263.7733722090294464 ) ) ;
#53965=CARTESIAN_POINT ( 'NONE',  ( 179.1667039024460166, -28.27351298637280408, -5.074374724088000832 ) ) ;
#53966=CARTESIAN_POINT ( 'NONE',  ( 108.0321269276242049, -25.74166508409292220, 105.9946728949589811 ) ) ;
#53968=CARTESIAN_POINT ( 'NONE',  ( 96.57452018799374116, -36.20934681947932177, 171.2870538473399620 ) ) ;
#53969=ORIENTED_EDGE ( 'NONE', *, *, #52062, .T. ) ;
#53972=B_SPLINE_CURVE_WITH_KNOTS ( 'NONE', 3,
 ( #6381, #11861, #19559, #54945, #47248, #82711, #74977, #5041, #59980, #87710, #68170, #25479, #5951, #33641, #61332, #89059, #53150, #80919 ),
 .UNSPECIFIED., .F., .F.,
 ( 4, 2, 2, 2, 2, 2, 2, 2, 4 ),
 ( 0.000000000000000000, 0.06249602157272145242, 0.1249920431454429048, 0.1874880647181643711, 0.2499840862908858097, 0.3124801078636072482, 0.3749761294363287423, 0.4374721510090504584, 0.4999681725817722855 ),
 .UNSPECIFIED. ) ;
#53973=DIRECTION ( 'NONE',  ( -4.237773401492740281E-14, 1.000000000000000000, 0.000000000000000000 ) ) ;
#53974=CARTESIAN_POINT ( 'NONE',  ( 116.3201542697790529, -32.94256427661516540, 65.13562527591099638 ) ) ;
#53976=EDGE_CURVE ( 'NONE', #85218, #60508, #7572, .T. ) ;
#53977=EDGE_LOOP ( 'NONE', ( #48919, #56862, #13432, #12417 ) ) ;
#53978=CARTESIAN_POINT ( 'NONE',  ( 25.56670390244797275, -67.87844715994100397, 252.3428068554150059 ) ) ;
#53979=CARTESIAN_POINT ( 'NONE',  ( 109.0807882705640139, -47.64528240413121551, 127.7337205140059382 ) ) ;
#53980=ORIENTED_EDGE ( 'NONE', *, *, #17918, .T. ) ;
#53984=FACE_OUTER_BOUND ( 'NONE', #70629, .T. ) ;
#53985=ORIENTED_EDGE ( 'NONE', *, *, #41478, .T. ) ;
#53986=CIRCLE ( 'NONE', #58350, 1.000000000000000888 ) ;
#53988=CARTESIAN_POINT ( 'NONE',  ( 172.5664832912728457, -18.82844715994071194, 321.9256252759119548 ) ) ;
#53989=ORIENTED_EDGE ( 'NONE', *, *, #1203, .T. ) ;
#53990=CIRCLE ( 'NONE', #26463, 11.45913725231036118 ) ;
#53991=ADVANCED_FACE ( 'NONE', ( #49331 ), #28000, .T. ) ;
#53992=ORIENTED_EDGE ( 'NONE', *, *, #15855, .F. ) ;
#53995=EDGE_CURVE ( 'NONE', #14566, #15500, #49780, .T. ) ;
#53996=CARTESIAN_POINT ( 'NONE',  ( 99.04406178140811789, -42.84125753979320450, 156.8439585992620096 ) ) ;
#53998=CARTESIAN_POINT ( 'NONE',  ( 97.33782221849729410, -34.07114218142883288, 106.1147982288662774 ) ) ;
#54002=ORIENTED_EDGE ( 'NONE', *, *, #38346, .F. ) ;
#54003=DIRECTION ( 'NONE',  ( 1.000000000000000078E-15, 1.000000000000000083E-30, -1.000000000000000000 ) ) ;
#54004=CARTESIAN_POINT ( 'NONE',  ( 98.48461633480667388, -41.42146110206439147, 217.7241967044819546 ) ) ;
#54005=FACE_BOUND ( 'NONE', #67712, .T. ) ;
#54007=AXIS2_PLACEMENT_3D ( 'NONE', #73921, #11701, #53893 ) ;
#54008=CARTESIAN_POINT ( 'NONE',  ( 112.3909220325769382, -27.83061929752864572, 50.65943479972001739 ) ) ;
#54009=DIRECTION ( 'NONE',  ( 0.000000000000000000, 0.000000000000000000, -1.000000000000000000 ) ) ;
#54015=ORIENTED_EDGE ( 'NONE', *, *, #43112, .T. ) ;
#54016=CARTESIAN_POINT ( 'NONE',  ( 109.7775653660112596, -28.26114369521987868, 231.2615833058969770 ) ) ;
#54018=DIRECTION ( 'NONE',  ( 0.000000000000000000, 0.000000000000000000, -1.000000000000000000 ) ) ;
#54019=DIRECTION ( 'NONE',  ( -1.000000000000000078E-15, 1.000000000000000000, 0.000000000000000000 ) ) ;
#54020=EDGE_CURVE ( 'NONE', #48304, #31161, #41171, .T. ) ;
#54021=CARTESIAN_POINT ( 'NONE',  ( 34.96670390244699433, -26.71338133339301635, 313.9678068554150059 ) ) ;
#54022=CARTESIAN_POINT ( 'NONE',  ( 82.60909586547556671, -37.77717416134770190, 2.822018739140996324 ) ) ;
#54025=CARTESIAN_POINT ( 'NONE',  ( 112.1310759968675654, -28.00808910187714673, 35.65652423099695056 ) ) ;
#54027=CARTESIAN_POINT ( 'NONE',  ( 105.3203727031265373, -26.45150370518939198, 15.20991099019697401 ) ) ;
#54028=VERTEX_POINT ( 'NONE', #68902 ) ;
#54029=CARTESIAN_POINT ( 'NONE',  ( 98.61142602524013512, -34.88203500400037882, 253.9614237029248613 ) ) ;
#54032=CARTESIAN_POINT ( 'NONE',  ( 109.3575602964533431, -46.23809593081423941, 132.7641967044829698 ) ) ;
#54034=DIRECTION ( 'NONE',  ( -0.9254794337955620787, -0.3787978585227822492, 0.000000000000000000 ) ) ;
#54036=LINE ( 'NONE', #12750, #55174 ) ;
#54037=CARTESIAN_POINT ( 'NONE',  ( 111.6274790011277247, -46.15230754745154940, 243.9356252759109509 ) ) ;
#54041=CARTESIAN_POINT ( 'NONE',  ( 109.9229042994399492, -46.83780379245977343, 68.79562527591099297 ) ) ;
#54042=EDGE_CURVE ( 'NONE', #63582, #83770, #49873, .T. ) ;
#54043=DIRECTION ( 'NONE',  ( 0.000000000000000000, -1.000000000000000000, 0.000000000000000000 ) ) ;
#54045=ORIENTED_EDGE ( 'NONE', *, *, #25584, .F. ) ;
#54046=EDGE_CURVE ( 'NONE', #35135, #27298, #55238, .T. ) ;
#54049=EDGE_CURVE ( 'NONE', #69845, #88931, #79755, .T. ) ;
#54050=CARTESIAN_POINT ( 'NONE',  ( 182.5667039024480118, -32.29483332968450782, 193.9678068554150059 ) ) ;
#54051=CARTESIAN_POINT ( 'NONE',  ( 140.9629299006806775, -8.979447159940995959, -5.074374724088994704 ) ) ;
#54053=PLANE ( 'NONE',  #11265 ) ;
#54054=CARTESIAN_POINT ( 'NONE',  ( 105.4193742293517460, -27.59801994936882252, 123.0366617981629673 ) ) ;
#54055=CARTESIAN_POINT ( 'NONE',  ( 117.5131067102741582, -36.80237174509009179, 259.8213395616249386 ) ) ;
#54056=EDGE_CURVE ( 'NONE', #15222, #5926, #44303, .T. ) ;
#54057=CARTESIAN_POINT ( 'NONE',  ( 152.0371591254582881, -47.82818131005588214, 313.9678068554149490 ) ) ;
#54058=ORIENTED_EDGE ( 'NONE', *, *, #86324, .F. ) ;
#54060=ADVANCED_FACE ( 'NONE', ( #16185 ), #72482, .F. ) ;
#54064=ADVANCED_FACE ( 'NONE', ( #10247 ), #16622, .F. ) ;
#54066=DIRECTION ( 'NONE',  ( 0.000000000000000000, 1.000000000000000000, 0.000000000000000000 ) ) ;
#54068=ORIENTED_EDGE ( 'NONE', *, *, #77614, .F. ) ;
#54072=CARTESIAN_POINT ( 'NONE',  ( 71.24076473329807868, 5.642044068322332961, 361.9756252759101471 ) ) ;
#54073=CARTESIAN_POINT ( 'NONE',  ( 102.8311628264132906, -45.84342327138038087, 9.425625275910965328 ) ) ;
#54074=CARTESIAN_POINT ( 'NONE',  ( 99.71244791179715605, -41.13061414147755812, 161.1781341137909465 ) ) ;
#54075=CARTESIAN_POINT ( 'NONE',  ( 114.3840247170090407, -44.21678670926648635, 73.19276813305397411 ) ) ;
#54076=ORIENTED_EDGE ( 'NONE', *, *, #35303, .F. ) ;
#54079=AXIS2_PLACEMENT_3D ( 'NONE', #41507, #89693, #27892 ) ;
#54082=EDGE_LOOP ( 'NONE', ( #69191, #53129 ) ) ;
#54083=CARTESIAN_POINT ( 'NONE',  ( 102.0662944402450876, -27.97094399344484117, 261.4898263993179626 ) ) ;
#54087=CARTESIAN_POINT ( 'NONE',  ( 113.7395804989182579, -44.20594635639993442, 133.1562568519375418 ) ) ;
#54089=LINE ( 'NONE', #54534, #45149 ) ;
#54091=CARTESIAN_POINT ( 'NONE',  ( 104.6437644399306635, -47.53804903515802494, 27.38895860924395009 ) ) ;
#54092=CARTESIAN_POINT ( 'NONE',  ( 96.61310803562074057, -37.29506674262550803, 72.36991099019596163 ) ) ;
#54093=LINE ( 'NONE', #81850, #66578 ) ;
#54096=CARTESIAN_POINT ( 'NONE',  ( 36.65249034007531037, -48.32844715994123419, 249.9678068554150343 ) ) ;
#54097=EDGE_CURVE ( 'NONE', #25485, #8128, #71507, .T. ) ;
#54102=DIRECTION ( 'NONE',  ( 0.000000000000000000, 0.000000000000000000, -1.000000000000000000 ) ) ;
#54104=CARTESIAN_POINT ( 'NONE',  ( 110.3859512856231788, -47.32161482583386913, 52.80610146638697699 ) ) ;
#54105=CARTESIAN_POINT ( 'NONE',  ( 115.2842354651272814, -44.15600456922878436, 79.25372051400697160 ) ) ;
#54106=ADVANCED_FACE ( 'NONE', ( #38386 ), #84787, .T. ) ;
#54107=CARTESIAN_POINT ( 'NONE',  ( 182.4202572930259976, -31.94127993907710206, -5.074374724088000832 ) ) ;
#54110=CIRCLE ( 'NONE', #14990, 2.500000000000002220 ) ;
#54112=DIRECTION ( 'NONE',  ( 1.000000000000000078E-15, -1.000000000000000083E-30, -1.000000000000000000 ) ) ;
#54113=ORIENTED_EDGE ( 'NONE', *, *, #63194, .F. ) ;
#54114=CARTESIAN_POINT ( 'NONE',  ( 97.87212830949614784, -31.93334231290201330, 86.93181575210095957 ) ) ;
#54115=DIRECTION ( 'NONE',  ( -4.237773401492740281E-14, 1.000000000000000000, 0.000000000000000000 ) ) ;
#54116=ORIENTED_EDGE ( 'NONE', *, *, #78228, .F. ) ;
#54117=CARTESIAN_POINT ( 'NONE',  ( 106.8520627977276973, -47.75749532952657006, 223.5489586092439538 ) ) ;
#54118=CARTESIAN_POINT ( 'NONE',  ( 101.9925926974754731, -45.44547922718067667, 253.1577994238472513 ) ) ;
#54119=CARTESIAN_POINT ( 'NONE',  ( 113.2118005416166682, -44.63368877937661239, 148.1023887368787086 ) ) ;
#54120=DIRECTION ( 'NONE',  ( 0.000000000000000000, 0.000000000000000000, -1.000000000000000000 ) ) ;
#54121=CARTESIAN_POINT ( 'NONE',  ( 141.8664832912729992, -1.929447159941394263, 361.9756252759109998 ) ) ;
#54122=LINE ( 'NONE', #81879, #2726 ) ;
#54124=CARTESIAN_POINT ( 'NONE',  ( 98.02110346605346081, -41.80092515478916937, 181.7451490854359974 ) ) ;
#54125=VERTEX_POINT ( 'NONE', #15736 ) ;
#54127=CARTESIAN_POINT ( 'NONE',  ( 117.1284314671335665, -36.25205438732766083, 115.2958690201829626 ) ) ;
#54128=FACE_OUTER_BOUND ( 'NONE', #27403, .T. ) ;
#54129=CARTESIAN_POINT ( 'NONE',  ( 105.2300248619054344, -26.52326248388681051, 271.2061014663865990 ) ) ;
#54130=DIRECTION ( 'NONE',  ( 1.639958061481212836E-42, -4.100000000000000342E-29, -1.000000000000000000 ) ) ;
#54131=AXIS2_PLACEMENT_3D ( 'NONE', #82655, #53091, #25875 ) ;
#54133=DIRECTION ( 'NONE',  ( -0.0001713722456133526934, 0.9999999853157766072, 0.000000000000000000 ) ) ;
#54136=DIRECTION ( 'NONE',  ( 1.000000000000000078E-15, 1.000000000000000083E-30, -1.000000000000000000 ) ) ;
#54137=CARTESIAN_POINT ( 'NONE',  ( 177.4809174648216299, -49.32844715993478246, 129.9678068554150059 ) ) ;
#54138=CARTESIAN_POINT ( 'NONE',  ( 113.6717327907684165, -45.56316108038149082, 188.0994347997199725 ) ) ;
#54139=CARTESIAN_POINT ( 'NONE',  ( 108.4185240248554720, -26.73515827628457231, 169.9680643324088862 ) ) ;
#54140=ORIENTED_EDGE ( 'NONE', *, *, #69446, .F. ) ;
#54141=ORIENTED_EDGE ( 'NONE', *, *, #23869, .F. ) ;
#54142=CYLINDRICAL_SURFACE ( 'NONE', #35802, 9.999999999999998224 ) ;
#54144=CARTESIAN_POINT ( 'NONE',  ( 98.35001644836999901, -31.65630223862054393, 185.9069172308759335 ) ) ;
#54146=CIRCLE ( 'NONE', #78904, 4.750000000000004441 ) ;
#54147=DIRECTION ( 'NONE',  ( 0.000000000000000000, 0.000000000000000000, 1.000000000000000000 ) ) ;
#54148=VERTEX_POINT ( 'NONE', #23007 ) ;
#54149=CARTESIAN_POINT ( 'NONE',  ( 116.8180511536208712, -34.15651531693190179, 64.03116570955137377 ) ) ;
#54151=CARTESIAN_POINT ( 'NONE',  ( 109.3369124252947557, -26.55437064873915531, 224.9013395616249511 ) ) ;
#54153=ORIENTED_EDGE ( 'NONE', *, *, #68982, .T. ) ;
#54154=EDGE_CURVE ( 'NONE', #65985, #976, #29410, .T. ) ;
#54156=DIRECTION ( 'NONE',  ( 0.000000000000000000, 1.000000000000000000, 0.000000000000000000 ) ) ;
#54157=DIRECTION ( 'NONE',  ( 0.000000000000000000, 0.000000000000000000, -1.000000000000000000 ) ) ;
#54158=CARTESIAN_POINT ( 'NONE',  ( 113.8053744393198485, -42.15975756917345763, 41.09285227435299959 ) ) ;
#54159=CARTESIAN_POINT ( 'NONE',  ( 108.7467188015556729, -25.78131109771034701, 140.9432443235299672 ) ) ;
#54160=ADVANCED_FACE ( 'NONE', ( #50229 ), #71154, .F. ) ;
#54161=DIRECTION ( 'NONE',  ( 0.7071067811873675835, 0.7071067811857274510, 7.071067811873980240E-16 ) ) ;
#54163=EDGE_CURVE ( 'NONE', #37451, #61450, #14959, .T. ) ;
#54165=CARTESIAN_POINT ( 'NONE',  ( 98.03114200176756299, -41.01962003592631589, 66.67980080132694809 ) ) ;
#54167=ORIENTED_EDGE ( 'NONE', *, *, #50171, .F. ) ;
#54168=EDGE_CURVE ( 'NONE', #64389, #32858, #31570, .T. ) ;
#54170=EDGE_LOOP ( 'NONE', ( #5788, #240 ) ) ;
#54172=DIRECTION ( 'NONE',  ( -1.000000000000000078E-15, -1.000000000000000083E-30, 1.000000000000000000 ) ) ;
#54173=VECTOR ( 'NONE', #39463, 1000.000000000000000 ) ;
#54174=EDGE_CURVE ( 'NONE', #39224, #66807, #46970, .T. ) ;
#54175=CARTESIAN_POINT ( 'NONE',  ( 98.75910798445569583, -38.71530899645634349, 55.93527697093397677 ) ) ;
#54176=CARTESIAN_POINT ( 'NONE',  ( 103.0820296961932456, -47.91685729158425744, 252.3041967044823366 ) ) ;
#54177=CARTESIAN_POINT ( 'NONE',  ( 98.18688568738947708, -31.30898482519904036, 170.8899109901960003 ) ) ;
#54178=CARTESIAN_POINT ( 'NONE',  ( 41.56648329127398966, -27.57844715994070484, 198.9256252759119832 ) ) ;
#54179=CARTESIAN_POINT ( 'NONE',  ( 97.21679027376985971, -33.31418093018012172, 282.0613395616252888 ) ) ;
#54181=CARTESIAN_POINT ( 'NONE',  ( 115.7812481455904390, -41.80544854195400717, 94.40617102049091613 ) ) ;
#54183=VERTEX_POINT ( 'NONE', #74265 ) ;
#54184=ADVANCED_FACE ( 'NONE', ( #32459 ), #74705, .T. ) ;
#54185=CARTESIAN_POINT ( 'NONE',  ( 97.92339830869723016, -40.78107783808657416, 111.6584168148213223 ) ) ;
#54186=CARTESIAN_POINT ( 'NONE',  ( 100.6291634319263864, -44.98581313249158598, 232.0499109901969632 ) ) ;
#54187=VECTOR ( 'NONE', #4467, 1000.000000000000000 ) ;
#54188=VERTEX_POINT ( 'NONE', #12037 ) ;
#54189=CARTESIAN_POINT ( 'NONE',  ( 101.9844316336549070, -45.87267731258258152, 187.1727681330539781 ) ) ;
#54190=CARTESIAN_POINT ( 'NONE',  ( 116.3219235766278672, -32.94275373074044211, 34.13562527591096085 ) ) ;
#54191=CIRCLE ( 'NONE', #35354, 0.5000000000000004441 ) ;
#54193=CARTESIAN_POINT ( 'NONE',  ( 105.7147421359655795, -46.72375322334213621, 23.46889897272690106 ) ) ;
#54195=CARTESIAN_POINT ( 'NONE',  ( 100.9356538695852663, -31.07395776800294485, 277.6356252759110248 ) ) ;
#54196=LINE ( 'NONE', #46943, #79017 ) ;
#54199=LINE ( 'NONE', #87418, #2021 ) ;
#54200=VECTOR ( 'NONE', #39405, 1000.000000000000000 ) ;
#54201=CARTESIAN_POINT ( 'NONE',  ( 41.56648329127399677, -18.82844715994099971, 196.8086252759119645 ) ) ;
#54202=CARTESIAN_POINT ( 'NONE',  ( 97.06125986173157116, -37.99738863349521978, 41.42674836562936491 ) ) ;
#54203=DIRECTION ( 'NONE',  ( 0.000000000000000000, 1.000000000000000000, 0.000000000000000000 ) ) ;
#54204=EDGE_CURVE ( 'NONE', #41893, #46749, #80641, .T. ) ;
#54205=CARTESIAN_POINT ( 'NONE',  ( 160.7738106836385441, -48.62134037874550074, 180.4678068554150059 ) ) ;
#54206=VERTEX_POINT ( 'NONE', #12487 ) ;
#54207=DIRECTION ( 'NONE',  ( 9.351236661543306751E-17, -3.725950533538267725E-29, -1.000000000000000000 ) ) ;
#54208=CARTESIAN_POINT ( 'NONE',  ( 96.83676235526975518, -34.60832162431106696, 216.1641967044819808 ) ) ;
#54209=CARTESIAN_POINT ( 'NONE',  ( 116.5983126044778402, -29.68822244385183140, 105.3327681330539463 ) ) ;
#54210=CARTESIAN_POINT ( 'NONE',  ( 112.4341072229889136, -46.44469865882210513, 248.9661014663869878 ) ) ;
#54211=CARTESIAN_POINT ( 'NONE',  ( 100.9546728758785150, -28.70702567901418689, 155.5939586028919450 ) ) ;
#54212=ADVANCED_FACE ( 'NONE', ( #19299 ), #26114, .F. ) ;
#54213=LINE ( 'NONE', #19721, #8432 ) ;
#54214=DIRECTION ( 'NONE',  ( 0.7071067811865171526, 0.7071067811865779928, 7.071067811865164719E-16 ) ) ;
#54215=DIRECTION ( 'NONE',  ( -3.360405532702990443E-14, 1.000000000000000000, 0.000000000000000000 ) ) ;
#54216=CARTESIAN_POINT ( 'NONE',  ( 123.6837132603319418, -50.82895651782485658, 239.5838068554170377 ) ) ;
#54217=CARTESIAN_POINT ( 'NONE',  ( 131.6729728819825311, -20.08739819367843182, 2.653088468865466787 ) ) ;
#54220=CARTESIAN_POINT ( 'NONE',  ( 100.5405518937255209, -43.91836718856000488, 156.4124198280769917 ) ) ;
#54223=CARTESIAN_POINT ( 'NONE',  ( 183.6524903400783160, -48.32844715993452667, 300.4678068554149490 ) ) ;
#54224=CARTESIAN_POINT ( 'NONE',  ( 112.1095002620001253, -47.42599740258504681, 133.9270538473399768 ) ) ;
#54225=DIRECTION ( 'NONE',  ( 0.000000000000000000, 0.000000000000000000, -1.000000000000000000 ) ) ;
#54226=CARTESIAN_POINT ( 'NONE',  ( 164.7830935719630361, -29.99615139349950965, -5.074374724088000832 ) ) ;
#54227=DIRECTION ( 'NONE',  ( 1.000000000000000078E-15, -1.000000000000000083E-30, -1.000000000000000000 ) ) ;
#54228=CARTESIAN_POINT ( 'NONE',  ( 107.0664832912748068, -36.72944715993923381, 14.92562527591097066 ) ) ;
#54229=CARTESIAN_POINT ( 'NONE',  ( 116.8124865092211451, -37.88235468918158944, 53.73276813305394484 ) ) ;
#54231=VERTEX_POINT ( 'NONE', #53330 ) ;
#54232=ORIENTED_EDGE ( 'NONE', *, *, #619, .F. ) ;
#54233=AXIS2_PLACEMENT_3D ( 'NONE', #66513, #46946, #12455 ) ;
#54234=EDGE_CURVE ( 'NONE', #41446, #42554, #66541, .T. ) ;
#54236=CARTESIAN_POINT ( 'NONE',  ( 116.4171719250472137, -30.71472603919677624, 140.2813395616249750 ) ) ;
#54237=CARTESIAN_POINT ( 'NONE',  ( 41.56648329127398966, -27.82844715994070484, 318.9256252759120116 ) ) ;
#54239=CARTESIAN_POINT ( 'NONE',  ( 191.6375511031384633, -78.44951497180814215, 342.9256252759109884 ) ) ;
#54241=CARTESIAN_POINT ( 'NONE',  ( 127.0664832912740110, -46.72944715994101017, 14.67562527591099197 ) ) ;
#54243=CARTESIAN_POINT ( 'NONE',  ( 100.8873815386462809, -44.70014985875308611, 178.0522830632788214 ) ) ;
#54244=CARTESIAN_POINT ( 'NONE',  ( 104.2200364793041274, -25.25138339198301907, 90.26991099019693365 ) ) ;
#54246=ORIENTED_EDGE ( 'NONE', *, *, #57164, .T. ) ;
#54249=DIRECTION ( 'NONE',  ( 0.000000000000000000, 0.000000000000000000, -1.000000000000000000 ) ) ;
#54251=CARTESIAN_POINT ( 'NONE',  ( 115.1781387256201725, -32.22423048609648788, 177.0480903695909660 ) ) ;
#54252=EDGE_CURVE ( 'NONE', #4156, #43071, #39722, .T. ) ;
#54254=CIRCLE ( 'NONE', #84736, 3.250000000000002665 ) ;
#54255=EDGE_CURVE ( 'NONE', #61899, #18226, #58434, .T. ) ;
#54256=EDGE_CURVE ( 'NONE', #6148, #22550, #46074, .T. ) ;
#54257=DIRECTION ( 'NONE',  ( -1.000000000000000078E-15, 0.000000000000000000, -1.000000000000000000 ) ) ;
#54260=ORIENTED_EDGE ( 'NONE', *, *, #26450, .T. ) ;
#54263=AXIS2_PLACEMENT_3D ( 'NONE', #3389, #45143, #2505 ) ;
#54264=EDGE_CURVE ( 'NONE', #770, #58384, #87003, .T. ) ;
#54265=CARTESIAN_POINT ( 'NONE',  ( 107.3678158256761179, -26.30747296201684549, 321.5865679059475610 ) ) ;
#54267=ORIENTED_EDGE ( 'NONE', *, *, #18026, .T. ) ;
#54268=CARTESIAN_POINT ( 'NONE',  ( 77.31648329127399677, -18.72944715994106346, 6.749768910606400496 ) ) ;
#54269=CARTESIAN_POINT ( 'NONE',  ( 102.0804048320179618, -44.05524405925518039, 193.5330118773259755 ) ) ;
#54271=DIRECTION ( 'NONE',  ( 0.000000000000000000, 0.000000000000000000, 1.000000000000000000 ) ) ;
#54277=FACE_OUTER_BOUND ( 'NONE', #39294, .T. ) ;
#54278=ORIENTED_EDGE ( 'NONE', *, *, #36542, .F. ) ;
#54280=EDGE_CURVE ( 'NONE', #72232, #77895, #80197, .T. ) ;
#54281=CARTESIAN_POINT ( 'NONE',  ( 115.6591437269271694, -35.69643618062379176, 236.7518998934009460 ) ) ;
#54282=CARTESIAN_POINT ( 'NONE',  ( 113.9315101381565682, -28.03652776953382286, 124.5565776568629559 ) ) ;
#54283=CARTESIAN_POINT ( 'NONE',  ( 111.9186950350130303, -27.52701776748434170, 59.68991099019693536 ) ) ;
#54284=CARTESIAN_POINT ( 'NONE',  ( 99.40430160516557123, -34.20253528913899999, 249.5838068554174356 ) ) ;
#54285=CARTESIAN_POINT ( 'NONE',  ( 162.9033555647770015, -33.89581943344391135, 342.9256252759119548 ) ) ;
#54286=CARTESIAN_POINT ( 'NONE',  ( 107.3114696520656395, -25.27148101547330228, 320.7096034169829863 ) ) ;
#54287=CARTESIAN_POINT ( 'NONE',  ( 108.6750115452441747, -26.42919841034747819, 185.9527681330539792 ) ) ;
#54288=DIRECTION ( 'NONE',  ( 4.299999999999999979E-14, -1.000000000000000000, 4.400000000000000367E-29 ) ) ;
#54289=ORIENTED_EDGE ( 'NONE', *, *, #53357, .T. ) ;
#54290=CARTESIAN_POINT ( 'NONE',  ( 72.26949937496598864, -71.54137415153812185, 361.9756252759101471 ) ) ;
#54292=ORIENTED_EDGE ( 'NONE', *, *, #37388, .F. ) ;
#54293=DIRECTION ( 'NONE',  ( 0.000000000000000000, 0.000000000000000000, 1.000000000000000000 ) ) ;
#54296=CARTESIAN_POINT ( 'NONE',  ( 116.3192736897089645, -32.94707975126958388, 130.1356252759109680 ) ) ;
#54298=CARTESIAN_POINT ( 'NONE',  ( 98.20221454234541625, -43.33276655250838871, 111.8480062282919647 ) ) ;
#54299=CARTESIAN_POINT ( 'NONE',  ( 105.8028369410636316, -26.72358438641067124, 255.1772342916230798 ) ) ;
#54300=VECTOR ( 'NONE', #79948, 1000.000000000000000 ) ;
#54301=CARTESIAN_POINT ( 'NONE',  ( 136.7727304466901899, -36.23917853418728185, 6.814128304792808066 ) ) ;
#54302=DIRECTION ( 'NONE',  ( -1.000000000000000078E-15, 1.000000000000000083E-30, 1.000000000000000000 ) ) ;
#54303=CARTESIAN_POINT ( 'NONE',  ( 117.0718954855416172, -35.46248235747613364, 144.9272919424813892 ) ) ;
#54304=CARTESIAN_POINT ( 'NONE',  ( 194.5667039024485234, -47.82844715993405060, 180.4678068554150343 ) ) ;
#54305=CARTESIAN_POINT ( 'NONE',  ( 110.2492204789523100, -26.78788743924354065, 230.8299109901969643 ) ) ;
#54306=DIRECTION ( 'NONE',  ( -4.237773401492740281E-14, 1.000000000000000000, 0.000000000000000000 ) ) ;
#54307=CARTESIAN_POINT ( 'NONE',  ( 90.44969454456416713, -54.60520651782495349, 218.8274735512160589 ) ) ;
#54308=ORIENTED_EDGE ( 'NONE', *, *, #81184, .F. ) ;
#54309=DIRECTION ( 'NONE',  ( -1.000200923085726652E-15, -1.000000000000000000, 0.000000000000000000 ) ) ;
#54313=CARTESIAN_POINT ( 'NONE',  ( 97.57529025620152652, -41.14803526195210992, 256.6727681330537507 ) ) ;
#54314=VERTEX_POINT ( 'NONE', #32016 ) ;
#54315=DIRECTION ( 'NONE',  ( -0.9254794337955620787, -0.3787978585227822492, 0.000000000000000000 ) ) ;
#54316=CARTESIAN_POINT ( 'NONE',  ( 97.10477362122047396, -39.80301782323012105, 17.56419670448195092 ) ) ;
#54317=CARTESIAN_POINT ( 'NONE',  ( 114.2834173682332732, -44.31288860877327807, 154.1813395616249807 ) ) ;
#54318=DIRECTION ( 'NONE',  ( 1.000000000000000000, 2.999999999999999839E-15, 1.000000000000000078E-15 ) ) ;
#54320=CARTESIAN_POINT ( 'NONE',  ( 97.33785231244870317, -34.07101398346973298, 102.1147137487239718 ) ) ;
#54321=CARTESIAN_POINT ( 'NONE',  ( 107.0664832912739541, -23.41337547937445862, 305.7141315223800007 ) ) ;
#54323=DIRECTION ( 'NONE',  ( 0.000000000000000000, 0.000000000000000000, -1.000000000000000000 ) ) ;
#54328=VECTOR ( 'NONE', #23569, 1000.000000000000000 ) ;
#54329=VECTOR ( 'NONE', #62037, 1000.000000000000000 ) ;
#54331=EDGE_LOOP ( 'NONE', ( #13132, #12772, #14976, #78364 ) ) ;
#54332=CIRCLE ( 'NONE', #47078, 4.875000000000017764 ) ;
#54333=AXIS2_PLACEMENT_3D ( 'NONE', #7795, #48657, #43193 ) ;
#54334=VERTEX_POINT ( 'NONE', #55123 ) ;
#54336=CARTESIAN_POINT ( 'NONE',  ( 115.6551466294303054, -43.65033472170370032, 39.27467289495895386 ) ) ;
#54338=DIRECTION ( 'NONE',  ( 1.000000000000000078E-15, 0.000000000000000000, 1.000000000000000000 ) ) ;
#54339=FACE_OUTER_BOUND ( 'NONE', #49838, .T. ) ;
#54340=CARTESIAN_POINT ( 'NONE',  ( 116.5602560931381220, -38.76387722282552062, 258.0809912566484741 ) ) ;
#54341=VERTEX_POINT ( 'NONE', #20200 ) ;
#54342=ORIENTED_EDGE ( 'NONE', *, *, #406, .T. ) ;
#54345=PLANE ( 'NONE',  #47133 ) ;
#54346=LINE ( 'NONE', #40297, #15843 ) ;
#54349=LINE ( 'NONE', #27126, #69290 ) ;
#54350=CARTESIAN_POINT ( 'NONE',  ( 142.8821648370248170, -72.54478064608022692, 540.9756252759101471 ) ) ;
#54352=CARTESIAN_POINT ( 'NONE',  ( 98.14754276252327259, -43.36755551587079083, 261.8356252759109566 ) ) ;
#54353=CARTESIAN_POINT ( 'NONE',  ( 188.5667039024479834, -62.87844715994099687, 168.3428068554150059 ) ) ;
#54356=CARTESIAN_POINT ( 'NONE',  ( 107.0664832912749915, -36.72944715993903486, 25.56312527591096995 ) ) ;
#54357=CARTESIAN_POINT ( 'NONE',  ( 110.2109830224615052, -27.99972479296931382, 97.61951894101994753 ) ) ;
#54359=DIRECTION ( 'NONE',  ( 0.000000000000000000, 1.000000000000000000, 0.000000000000000000 ) ) ;
#54360=AXIS2_PLACEMENT_3D ( 'NONE', #1639, #57019, #21636 ) ;
#54361=CARTESIAN_POINT ( 'NONE',  ( 49.35211078756498893, -35.65087443492551245, 313.9678068554150059 ) ) ;
#54362=ADVANCED_FACE ( 'NONE', ( #21088 ), #38161, .T. ) ;
#54363=DIRECTION ( 'NONE',  ( -1.000000000000000078E-15, 0.000000000000000000, -1.000000000000000000 ) ) ;
#54364=ORIENTED_EDGE ( 'NONE', *, *, #11171, .T. ) ;
#54366=EDGE_CURVE ( 'NONE', #70797, #64389, #33817, .T. ) ;
#54368=CARTESIAN_POINT ( 'NONE',  ( 98.09046607155295305, -42.10132104613245474, 161.7556252759109725 ) ) ;
#54370=EDGE_CURVE ( 'NONE', #75722, #26617, #13381, .T. ) ;
#54372=CARTESIAN_POINT ( 'NONE',  ( 115.6492561437540445, -34.52393389210755004, 120.4587261630399837 ) ) ;
#54373=ADVANCED_FACE ( 'NONE', ( #68791 ), #48766, .T. ) ;
#54374=DIRECTION ( 'NONE',  ( 0.000000000000000000, 0.000000000000000000, -1.000000000000000000 ) ) ;
#54376=CARTESIAN_POINT ( 'NONE',  ( 101.0536616762676374, -27.42723333900414318, 66.54514908543495721 ) ) ;
#54378=DIRECTION ( 'NONE',  ( 0.000000000000000000, 1.000000000000000000, 0.000000000000000000 ) ) ;
#54381=CARTESIAN_POINT ( 'NONE',  ( 130.5667039024479834, -36.72944715994100306, 239.5838068554162987 ) ) ;
#54382=VECTOR ( 'NONE', #2210, 1000.000000000000000 ) ;
#54383=AXIS2_PLACEMENT_3D ( 'NONE', #58398, #10690, #23900 ) ;
#54384=VECTOR ( 'NONE', #84156, 1000.000000000000000 ) ;
#54385=ORIENTED_EDGE ( 'NONE', *, *, #35366, .T. ) ;
#54386=ORIENTED_EDGE ( 'NONE', *, *, #64159, .F. ) ;
#54387=ADVANCED_FACE ( 'NONE', ( #7007 ), #49216, .T. ) ;
#54389=FACE_OUTER_BOUND ( 'NONE', #66819, .T. ) ;
#54391=CARTESIAN_POINT ( 'NONE',  ( 110.8764511561472546, -27.72125199330407241, 244.7584824187689492 ) ) ;
#54392=CARTESIAN_POINT ( 'NONE',  ( 117.7257289732168744, -39.74036323029751117, 139.6194347997199827 ) ) ;
#54393=CARTESIAN_POINT ( 'NONE',  ( 49.35031423293199282, -29.99615139349890924, 342.9256252759109884 ) ) ;
#54394=CARTESIAN_POINT ( 'NONE',  ( 112.1393456442706196, -28.01282278279440519, 140.6564586090036357 ) ) ;
#54395=CARTESIAN_POINT ( 'NONE',  ( 114.5674230198705317, -44.02034806205370643, 94.21276813305395592 ) ) ;
#54398=AXIS2_PLACEMENT_3D ( 'NONE', #69907, #42618, #41723 ) ;
#54399=LINE ( 'NONE', #82163, #53917 ) ;
#54400=DIRECTION ( 'NONE',  ( 4.194175870806139918E-14, -1.000000000000000000, 0.000000000000000000 ) ) ;
#54403=CARTESIAN_POINT ( 'NONE',  ( 107.0664832912739399, -36.72944715994095333, 311.6356252759109680 ) ) ;
#54405=CARTESIAN_POINT ( 'NONE',  ( 115.0380569359702463, -30.04493676975920380, 269.3813395616251682 ) ) ;
#54407=TOROIDAL_SURFACE ( 'NONE', #87840, 15.84999999999999964, 0.1499999999999999944 ) ;
#54408=CARTESIAN_POINT ( 'NONE',  ( 131.3164832912739826, -18.72944715994100662, -5.074374724089004474 ) ) ;
#54409=CARTESIAN_POINT ( 'NONE',  ( 165.6738106836199904, -26.00627455219321860, -5.074374724088000832 ) ) ;
#54410=CARTESIAN_POINT ( 'NONE',  ( 99.63325261332695959, -43.08637385293071986, 31.88991099019694531 ) ) ;
#54411=CARTESIAN_POINT ( 'NONE',  ( 114.3025730761101357, -29.78814224338164962, 99.43545738674667689 ) ) ;
#54412=CARTESIAN_POINT ( 'NONE',  ( 113.9719413768824126, -28.12837331961977938, 115.5261014663869474 ) ) ;
#54413=DIRECTION ( 'NONE',  ( 0.0001211784769804374580, -0.7071067708032349186, 0.7071067811865462405 ) ) ;
#54414=CARTESIAN_POINT ( 'NONE',  ( 97.96866571142417968, -30.36999819975766357, 160.8289586092449497 ) ) ;
#54418=CARTESIAN_POINT ( 'NONE',  ( 130.5667039024480118, -36.72944715994093912, 219.5838068554170093 ) ) ;
#54419=DIRECTION ( 'NONE',  ( 1.000000000000000078E-15, -1.000000000000000083E-30, -1.000000000000000000 ) ) ;
#54420=CARTESIAN_POINT ( 'NONE',  ( 136.8004280042375740, -36.38432671277701758, 3.076561810304699218 ) ) ;
#54421=VERTEX_POINT ( 'NONE', #70129 ) ;
#54422=CARTESIAN_POINT ( 'NONE',  ( 164.9190312289439930, -35.91149509761220315, -5.074374724088000832 ) ) ;
#54423=CARTESIAN_POINT ( 'NONE',  ( 118.9678564412739092, -36.92894532057803758, 153.8127681330539644 ) ) ;
#54424=ORIENTED_EDGE ( 'NONE', *, *, #36217, .F. ) ;
#54425=CARTESIAN_POINT ( 'NONE',  ( 116.3183049785035195, -32.94379174720932468, 54.13562527591098217 ) ) ;
#54427=EDGE_CURVE ( 'NONE', #41221, #85162, #80249, .T. ) ;
#54429=CARTESIAN_POINT ( 'NONE',  ( 101.9936209511393486, -45.44607154457114007, 77.15645861017721074 ) ) ;
#54432=VECTOR ( 'NONE', #59477, 1000.000000000000000 ) ;
#54433=ADVANCED_FACE ( 'NONE', ( #75612 ), #76496, .T. ) ;
#54434=ORIENTED_EDGE ( 'NONE', *, *, #78635, .T. ) ;
#54437=CARTESIAN_POINT ( 'NONE',  ( 123.6837132603318992, -53.34645651782490461, 239.5838068554164693 ) ) ;
#54439=DIRECTION ( 'NONE',  ( -2.900000000000000265E-14, 2.000000000000000155E-15, -1.000000000000000000 ) ) ;
#54441=LINE ( 'NONE', #33138, #24768 ) ;
#54443=CARTESIAN_POINT ( 'NONE',  ( 97.33775388477235424, -34.07137617144550035, 181.1148172561750869 ) ) ;
#54444=VERTEX_POINT ( 'NONE', #42402 ) ;
#54447=EDGE_CURVE ( 'NONE', #17557, #89449, #49085, .T. ) ;
#54448=CIRCLE ( 'NONE', #29799, 3.299999999999997158 ) ;
#54449=VECTOR ( 'NONE', #20211, 1000.000000000000000 ) ;
#54450=CARTESIAN_POINT ( 'NONE',  ( 188.5667039024479834, -65.37844715994100397, 262.0928068554150059 ) ) ;
#54453=CARTESIAN_POINT ( 'NONE',  ( 110.5849939505706487, -26.97450646431661880, 245.7889586092439629 ) ) ;
#54454=CARTESIAN_POINT ( 'NONE',  ( 162.5667039024460223, -22.48495420874110806, 342.9256252759119548 ) ) ;
#54455=ORIENTED_EDGE ( 'NONE', *, *, #24447, .T. ) ;
#54457=CARTESIAN_POINT ( 'NONE',  ( 113.1080853710607528, -29.03773216254920797, 75.54705384733895812 ) ) ;
#54458=CARTESIAN_POINT ( 'NONE',  ( 115.9438631943473723, -41.40486966552543890, 53.44085822901627125 ) ) ;
#54460=VECTOR ( 'NONE', #80089, 1000.000000000000000 ) ;
#54461=CARTESIAN_POINT ( 'NONE',  ( 103.2784135495991222, -27.47469012475126604, 21.38563400800847347 ) ) ;
#54463=DIRECTION ( 'NONE',  ( -1.000000000000000078E-15, 1.000000000000000083E-30, 1.000000000000000000 ) ) ;
#54465=ORIENTED_EDGE ( 'NONE', *, *, #66487, .F. ) ;
#54467=CARTESIAN_POINT ( 'NONE',  ( 104.3066903214637620, -46.41728735870637479, 213.7872975916119458 ) ) ;
#54468=CARTESIAN_POINT ( 'NONE',  ( 112.0680535738694488, -45.48720938564293448, 53.98962239635005034 ) ) ;
#54470=AXIS2_PLACEMENT_3D ( 'NONE', #64538, #35922, #84555 ) ;
#54471=FACE_OUTER_BOUND ( 'NONE', #22807, .T. ) ;
#54473=CARTESIAN_POINT ( 'NONE',  ( 82.10314251156871990, -38.57949487819261236, 2.327894807235353802 ) ) ;
#54474=VERTEX_POINT ( 'NONE', #8358 ) ;
#54475=DIRECTION ( 'NONE',  ( 1.387778780781444492E-15, 0.000000000000000000, -1.000000000000000000 ) ) ;
#54476=CARTESIAN_POINT ( 'NONE',  ( 117.0723176125373044, -35.46598533043084700, 184.9276149807092509 ) ) ;
#54477=ORIENTED_EDGE ( 'NONE', *, *, #29283, .T. ) ;
#54478=CARTESIAN_POINT ( 'NONE',  ( 100.4109522542116650, -28.70505079160765760, 40.62705384733894221 ) ) ;
#54481=CARTESIAN_POINT ( 'NONE',  ( 113.3211896355758057, -31.48460449655562954, 267.1995189410199600 ) ) ;
#54482=DIRECTION ( 'NONE',  ( 0.7071067811865460184, 0.000000000000000000, 0.7071067811865487940 ) ) ;
#54483=CARTESIAN_POINT ( 'NONE',  ( 116.4171719250473984, -30.71472603919669098, 144.2813395616259697 ) ) ;
#54486=CARTESIAN_POINT ( 'NONE',  ( 172.5664832912729878, -27.57844715994070484, 255.9256252759120116 ) ) ;
#54487=CARTESIAN_POINT ( 'NONE',  ( 120.0056275895821898, -31.38355669832866468, 293.6369201390379544 ) ) ;
#54488=CARTESIAN_POINT ( 'NONE',  ( 118.0865697951701350, -35.40461063965730659, 234.9337205140059552 ) ) ;
#54490=EDGE_LOOP ( 'NONE', ( #13157, #53969 ) ) ;
#54491=CARTESIAN_POINT ( 'NONE',  ( 96.03173718742787912, -37.92605769912402991, 77.40038718067299328 ) ) ;
#54492=CYLINDRICAL_SURFACE ( 'NONE', #68586, 0.4999999999999982236 ) ;
#54494=EDGE_LOOP ( 'NONE', ( #77295, #28171, #63149, #12644, #14439, #21848, #39912, #32026 ) ) ;
#54495=ORIENTED_EDGE ( 'NONE', *, *, #61280, .T. ) ;
#54496=VERTEX_POINT ( 'NONE', #65544 ) ;
#54497=EDGE_CURVE ( 'NONE', #64498, #29605, #77323, .T. ) ;
#54499=CARTESIAN_POINT ( 'NONE',  ( 32.06670390244800473, -32.29483332968611364, -5.074374724088000832 ) ) ;
#54500=EDGE_CURVE ( 'NONE', #38055, #19567, #40996, .T. ) ;
#54501=DIRECTION ( 'NONE',  ( 0.000000000000000000, 0.000000000000000000, -1.000000000000000000 ) ) ;
#54502=CARTESIAN_POINT ( 'NONE',  ( 21.03715912545823130, -47.82818131006186491, 313.9678068554150059 ) ) ;
#54503=CARTESIAN_POINT ( 'NONE',  ( 107.7334136049453406, -44.89265071023657327, 175.4595189410199509 ) ) ;
#54504=CARTESIAN_POINT ( 'NONE',  ( 118.6781471654015689, -39.21772221756580734, 254.6584824187681022 ) ) ;
#54505=CARTESIAN_POINT ( 'NONE',  ( 116.7943317353957440, -39.39066265141695311, 59.61455726299030999 ) ) ;
#54506=VERTEX_POINT ( 'NONE', #50113 ) ;
#54508=DIRECTION ( 'NONE',  ( 1.000000000000000000, 6.208581945447490230E-14, 1.000000000000000078E-15 ) ) ;
#54512=CIRCLE ( 'NONE', #26998, 11.57110091390434192 ) ;
#54514=CIRCLE ( 'NONE', #89378, 1.000000000002049694 ) ;
#54515=VERTEX_POINT ( 'NONE', #64652 ) ;
#54516=ORIENTED_EDGE ( 'NONE', *, *, #59388, .T. ) ;
#54520=DIRECTION ( 'NONE',  ( 9.351236661543306751E-17, -3.725950533538267725E-29, -1.000000000000000000 ) ) ;
#54522=CARTESIAN_POINT ( 'NONE',  ( 112.9437820074331569, -43.62348782359368471, 152.5733722090289746 ) ) ;
#54523=CARTESIAN_POINT ( 'NONE',  ( 117.9706719164645250, -41.49678058079525300, 58.49848241876792798 ) ) ;
#54524=CARTESIAN_POINT ( 'NONE',  ( 107.0664832912739968, -36.72944715994100306, 293.2242906452868851 ) ) ;
#54528=CARTESIAN_POINT ( 'NONE',  ( 108.4162223138228285, -26.73487509133866524, 260.9689798133920249 ) ) ;
#54529=ORIENTED_EDGE ( 'NONE', *, *, #57709, .F. ) ;
#54530=CARTESIAN_POINT ( 'NONE',  ( 25.56670390244797275, -65.37844715994100397, 168.3428068554150059 ) ) ;
#54532=CARTESIAN_POINT ( 'NONE',  ( 116.3197976069899795, -32.94561274469138112, 134.1356252759109680 ) ) ;
#54533=VECTOR ( 'NONE', #53292, 1000.000000000000000 ) ;
#54534=CARTESIAN_POINT ( 'NONE',  ( 19.56648329127400032, 0.2215528400590013880, -5.074374724088000832 ) ) ;
#54535=ORIENTED_EDGE ( 'NONE', *, *, #15294, .F. ) ;
#54536=CARTESIAN_POINT ( 'NONE',  ( 105.9861246248700439, -26.33814362677674836, 50.15848241876796720 ) ) ;
#54542=DIRECTION ( 'NONE',  ( 0.9963424814100679816, -0.08544974978095716545, 0.000000000000000000 ) ) ;
#54544=ORIENTED_EDGE ( 'NONE', *, *, #77754, .F. ) ;
#54545=DIRECTION ( 'NONE',  ( 0.000000000000000000, 0.000000000000000000, 1.000000000000000000 ) ) ;
#54546=CARTESIAN_POINT ( 'NONE',  ( 123.6837132603318565, -22.62993780205705718, 239.5838068554170377 ) ) ;
#54548=EDGE_LOOP ( 'NONE', ( #51488, #25090, #17800, #58974 ) ) ;
#54549=CARTESIAN_POINT ( 'NONE',  ( 114.3683386633632324, -44.20073667237542026, 69.19276813305397411 ) ) ;
#54550=CARTESIAN_POINT ( 'NONE',  ( 99.08999158803118235, -42.79608037983736324, 171.8429505068361891 ) ) ;
#54553=ADVANCED_FACE ( 'NONE', ( #1988 ), #30137, .T. ) ;
#54554=DIRECTION ( 'NONE',  ( 1.000000000000000078E-15, -1.000000000000000083E-30, -1.000000000000000000 ) ) ;
#54556=CARTESIAN_POINT ( 'NONE',  ( 112.4472966703648780, -46.45872411559670212, 98.97848241876694431 ) ) ;
#54558=VERTEX_POINT ( 'NONE', #56935 ) ;
#54559=CARTESIAN_POINT ( 'NONE',  ( 105.7790678824445223, -26.40611305247087870, 266.1756252759109884 ) ) ;
#54560=DIRECTION ( 'NONE',  ( 0.000000000000000000, 1.000000000000000000, 0.000000000000000000 ) ) ;
#54561=CARTESIAN_POINT ( 'NONE',  ( 113.6616400493835357, -44.27479244131740899, 148.1480010436838768 ) ) ;
#54563=LINE ( 'NONE', #32805, #71816 ) ;
#54565=EDGE_CURVE ( 'NONE', #57694, #53468, #9129, .T. ) ;
#54568=CARTESIAN_POINT ( 'NONE',  ( 113.3375292005774639, -44.23527279707086279, 193.1299109901969757 ) ) ;
#54569=ORIENTED_EDGE ( 'NONE', *, *, #64888, .T. ) ;
#54571=CARTESIAN_POINT ( 'NONE',  ( 115.6990777838195186, -41.92069145011852527, 124.8272975916109573 ) ) ;
#54573=CARTESIAN_POINT ( 'NONE',  ( 162.5667039024460223, -19.82844715994111340, -5.074374724088000832 ) ) ;
#54575=CARTESIAN_POINT ( 'NONE',  ( 106.5981863181247604, -46.53222597210204725, 243.5384824187679556 ) ) ;
#54576=FACE_OUTER_BOUND ( 'NONE', #54494, .T. ) ;
#54578=CARTESIAN_POINT ( 'NONE',  ( 188.5667039024483529, -42.82844715993430640, 137.2178068554150059 ) ) ;
#54579=EDGE_CURVE ( 'NONE', #57891, #68568, #37397, .T. ) ;
#54580=B_SPLINE_CURVE_WITH_KNOTS ( 'NONE', 3,
 ( #65332, #24007, #37634, #17631, #45310, #9474, #16295, #65758, #11250, #59833, #51681, #3110, #58501, #31693, #38502, #50800, #17188, #3994, #3545, #86228, #78539, #43974, #23570, #66204, #79876, #59390, #24890, #2671, #30371, #72602, #52556, #80316, #18062, #51232, #78976, #81217, #61626, #18965, #32581, #62085, #40739, #12154, #88014, #6678, #67561, #34377, #25775, #19414, #25325, #68911, #52992 ),
 .UNSPECIFIED., .F., .F.,
 ( 4, 2, 1, 1, 1, 1, 1, 1, 2, 2, 2, 2, 2, 2, 2, 1, 1, 1, 1, 1, 1, 1, 2, 2, 2, 2, 2, 2, 2, 2, 2, 4 ),
 ( 0.5000148990659494252, 0.5001369657410288383, 0.5002590324161083624, 0.5005031657662670774, 0.5009914324665847296, 0.5019679658672203670, 0.5039210326684915309, 0.5078271662710340806, 0.5156394334761188469, 0.5312639678862881576, 0.5625130367066264458, 0.6250111743473033554, 0.6875093119879802650, 0.7500074496286570636, 0.7500684829661968811, 0.7501295163037366986, 0.7502515829787583801, 0.7504957163287344635, 0.7509839830286886286, 0.7519605164285885213, 0.7539135832283616612, 0.7578197168279081630, 0.7656319840270084942, 0.7812565184252078243, 0.8125055872216067065, 0.8437546560180054778, 0.8750037248144043600, 0.9062527936108031312, 0.9375018624072020135, 0.9687509312036008957, 0.9843754656018004479, 1.000000000000000000 ),
 .UNSPECIFIED. ) ;
#54582=B_SPLINE_CURVE_WITH_KNOTS ( 'NONE', 3,
 ( #20214, #47884, #13393, #41082, #27458, #43314, #69252, #56500, #29706, #20659, #71059, #36072, #1107, #21560, #56041, #69703, #83787, #14295 ),
 .UNSPECIFIED., .F., .F.,
 ( 4, 2, 2, 2, 2, 2, 2, 2, 4 ),
 ( 0.000000000000000000, 0.06249194833952455286, 0.1249838966790491057, 0.1874758450185736725, 0.2499677933580982114, 0.3124597416976227504, 0.3749516900371473449, 0.4374436383766718839, 0.4999355867161964229 ),
 .UNSPECIFIED. ) ;
#54584=CARTESIAN_POINT ( 'NONE',  ( 182.0374245136174522, -23.42844715993458848, 117.4678068554150627 ) ) ;
#54585=DIRECTION ( 'NONE',  ( -0.7071067811865101582, -0.7071067811865849873, 0.000000000000000000 ) ) ;
#54586=CARTESIAN_POINT ( 'NONE',  ( 98.55548742614587354, -30.74683778668241985, 205.8384824187679669 ) ) ;
#54587=DIRECTION ( 'NONE',  ( -2.900000000000000265E-14, 2.000000000000000155E-15, -1.000000000000000000 ) ) ;
#54589=EDGE_CURVE ( 'NONE', #33523, #57034, #23348, .T. ) ;
#54590=VERTEX_POINT ( 'NONE', #29250 ) ;
#54592=CARTESIAN_POINT ( 'NONE',  ( 82.16007929298940837, -20.51483178663177398, 7.477467810856416541 ) ) ;
#54593=CARTESIAN_POINT ( 'NONE',  ( 100.1253875378072848, -39.57043109886186727, 9.635625275910941312 ) ) ;
#54594=CARTESIAN_POINT ( 'NONE',  ( 41.56648329127398966, -27.57844715994070484, 141.9256252759119832 ) ) ;
#54595=CARTESIAN_POINT ( 'NONE',  ( 182.4202572930269923, -31.94127993907680718, -5.074374724088000832 ) ) ;
#54596=ORIENTED_EDGE ( 'NONE', *, *, #81395, .T. ) ;
#54597=DIRECTION ( 'NONE',  ( 0.000000000000000000, 0.000000000000000000, -1.000000000000000000 ) ) ;
#54598=CARTESIAN_POINT ( 'NONE',  ( 117.4744730450754560, -36.12879772292662039, 228.8727681330539667 ) ) ;
#54601=PLANE ( 'NONE',  #60756 ) ;
#54602=LINE ( 'NONE', #20128, #23195 ) ;
#54603=EDGE_CURVE ( 'NONE', #34812, #8195, #23784, .T. ) ;
#54605=ADVANCED_FACE ( 'NONE', ( #57381 ), #58711, .T. ) ;
#54606=CARTESIAN_POINT ( 'NONE',  ( 104.5412336160381273, -44.52083999592182550, 80.14523322673395000 ) ) ;
#54607=CARTESIAN_POINT ( 'NONE',  ( 117.4480285489056683, -30.96353277002295101, 175.2299109901969700 ) ) ;
#54608=LINE ( 'NONE', #48697, #71103 ) ;
#54612=CYLINDRICAL_SURFACE ( 'NONE', #21899, 14.00000000000000888 ) ;
#54613=CARTESIAN_POINT ( 'NONE',  ( 117.0906974882439755, -35.57082847448015883, 68.91926238958696160 ) ) ;
#54616=VERTEX_POINT ( 'NONE', #10138 ) ;
#54619=EDGE_LOOP ( 'NONE', ( #44593, #15320, #9497, #10004, #11191 ) ) ;
#54620=DIRECTION ( 'NONE',  ( 0.000000000000000000, 0.000000000000000000, -1.000000000000000000 ) ) ;
#54621=CARTESIAN_POINT ( 'NONE',  ( 102.1503607674210343, -29.12389592045764530, 69.96765792331494538 ) ) ;
#54622=CARTESIAN_POINT ( 'NONE',  ( 110.2626856154920603, -26.74582790018529366, 234.8299109901969643 ) ) ;
#54623=CARTESIAN_POINT ( 'NONE',  ( 114.1099639442526268, -29.07320488188160823, 199.4841967044819739 ) ) ;
#54624=LINE ( 'NONE', #88306, #59140 ) ;
#54625=CARTESIAN_POINT ( 'NONE',  ( 117.5188882057536830, -36.54585972124053939, 284.8413395616252615 ) ) ;
#54627=DIRECTION ( 'NONE',  ( 0.000000000000000000, 0.000000000000000000, -1.000000000000000000 ) ) ;
#54628=ORIENTED_EDGE ( 'NONE', *, *, #46475, .F. ) ;
#54629=ORIENTED_EDGE ( 'NONE', *, *, #4689, .F. ) ;
#54630=AXIS2_PLACEMENT_3D ( 'NONE', #3375, #9300, #56986 ) ;
#54631=CARTESIAN_POINT ( 'NONE',  ( 97.30000116515907393, -37.25789978020652882, 76.36991099019796536 ) ) ;
#54632=CARTESIAN_POINT ( 'NONE',  ( 104.2019728789896078, -25.17854340234507760, 90.26991099019693365 ) ) ;
#54633=AXIS2_PLACEMENT_3D ( 'NONE', #67404, #59687, #5195 ) ;
#54634=CARTESIAN_POINT ( 'NONE',  ( 117.4736937924436688, -35.59074751853778196, 278.9127681330539872 ) ) ;
#54635=ORIENTED_EDGE ( 'NONE', *, *, #6504, .F. ) ;
#54636=VECTOR ( 'NONE', #59628, 1000.000000000000000 ) ;
#54637=CARTESIAN_POINT ( 'NONE',  ( 118.8775732333442647, -37.69828162312832376, 188.7613395616259595 ) ) ;
#54638=CARTESIAN_POINT ( 'NONE',  ( 108.4174892093325440, -26.73503592116915684, 34.96895861265306138 ) ) ;
#54639=VECTOR ( 'NONE', #37980, 1000.000000000000000 ) ;
#54640=LINE ( 'NONE', #89207, #8745 ) ;
#54642=CARTESIAN_POINT ( 'NONE',  ( 98.57600492221074262, -34.82225168922051495, 277.6356252759111953 ) ) ;
#54643=CARTESIAN_POINT ( 'NONE',  ( 131.0667039024480118, -64.87844715994098976, 201.9838068554149970 ) ) ;
#54648=CARTESIAN_POINT ( 'NONE',  ( 75.31670390244798341, -50.82844715994100682, 86.31780685541500020 ) ) ;
#54649=CARTESIAN_POINT ( 'NONE',  ( 99.09570908462971772, -30.55043174235573034, 76.80229194148932947 ) ) ;
#54652=DIRECTION ( 'NONE',  ( 0.000000000000000000, 0.000000000000000000, 1.000000000000000000 ) ) ;
#54653=CARTESIAN_POINT ( 'NONE',  ( 98.01753632367962155, -44.42038823906860756, 226.8870538473399563 ) ) ;
#54654=CARTESIAN_POINT ( 'NONE',  ( 117.2221417514105610, -42.83659189374058940, 124.3956252759109731 ) ) ;
#54655=CARTESIAN_POINT ( 'NONE',  ( 100.1487569102796300, -45.40945638099971404, 268.0289586092443415 ) ) ;
#54657=AXIS2_PLACEMENT_3D ( 'NONE', #30708, #11145, #79773 ) ;
#54658=CYLINDRICAL_SURFACE ( 'NONE', #73639, 3.250000000000002665 ) ;
#54660=CARTESIAN_POINT ( 'NONE',  ( 188.5667039024479834, -48.82844715994099971, 290.4678068554150627 ) ) ;
#54662=FACE_OUTER_BOUND ( 'NONE', #41623, .T. ) ;
#54663=CARTESIAN_POINT ( 'NONE',  ( 131.5359215223111278, -19.80596063775375626, 2.807537029279443708 ) ) ;
#54666=EDGE_LOOP ( 'NONE', ( #86378, #65314, #2563, #54943 ) ) ;
#54667=EDGE_CURVE ( 'NONE', #5006, #75208, #78309, .T. ) ;
#54669=CARTESIAN_POINT ( 'NONE',  ( 107.5470202762386549, -45.24887850357546171, 152.0438483995049523 ) ) ;
#54670=EDGE_CURVE ( 'NONE', #10572, #12659, #78836, .T. ) ;
#54673=CARTESIAN_POINT ( 'NONE',  ( 98.34983002861665113, -31.65663634061341369, 90.90496632418863499 ) ) ;
#54674=CARTESIAN_POINT ( 'NONE',  ( 102.4028819069269645, -26.73371583578780886, 131.4118157521009778 ) ) ;
#54675=CARTESIAN_POINT ( 'NONE',  ( 99.04382043865727780, -42.84089565470306837, 147.8445008508561216 ) ) ;
#54677=EDGE_CURVE ( 'NONE', #24616, #49620, #80525, .T. ) ;
#54678=EDGE_CURVE ( 'NONE', #67341, #58630, #18278, .T. ) ;
#54679=CARTESIAN_POINT ( 'NONE',  ( 34.96670390244699433, -28.27351298637401200, -5.074374724088000832 ) ) ;
#54680=FACE_OUTER_BOUND ( 'NONE', #15929, .T. ) ;
#54681=CARTESIAN_POINT ( 'NONE',  ( 103.8130989789263197, -45.95327097697902730, 57.30705384734097407 ) ) ;
#54682=ORIENTED_EDGE ( 'NONE', *, *, #2580, .F. ) ;
#54683=ORIENTED_EDGE ( 'NONE', *, *, #77095, .F. ) ;
#54686=EDGE_CURVE ( 'NONE', #17571, #58627, #19187, .T. ) ;
#54688=CARTESIAN_POINT ( 'NONE',  ( 96.03815445040697796, -38.18343476501374312, 147.4299109901959923 ) ) ;
#54690=CARTESIAN_POINT ( 'NONE',  ( 125.0664832912740110, -18.82844715994099971, 284.9256252759119548 ) ) ;
#54694=CARTESIAN_POINT ( 'NONE',  ( 152.5667039024471592, -23.42844715993585325, 180.4678068554149775 ) ) ;
#54695=CARTESIAN_POINT ( 'NONE',  ( 113.1779779702134903, -44.75210462311810744, 179.0939275391108936 ) ) ;
#54696=CARTESIAN_POINT ( 'NONE',  ( 102.5676158828201352, -27.34920955258903419, 95.43276813305395478 ) ) ;
#54697=ORIENTED_EDGE ( 'NONE', *, *, #16751, .T. ) ;
#54698=ORIENTED_EDGE ( 'NONE', *, *, #45028, .T. ) ;
#54699=EDGE_CURVE ( 'NONE', #62015, #67197, #86889, .T. ) ;
#54700=VERTEX_POINT ( 'NONE', #45081 ) ;
#54701=FACE_OUTER_BOUND ( 'NONE', #75650, .T. ) ;
#54702=CARTESIAN_POINT ( 'NONE',  ( 142.8821648370248170, -72.54478064608022692, 540.9756252759101471 ) ) ;
#54705=CARTESIAN_POINT ( 'NONE',  ( 98.33113000137380766, -33.60062404821446336, 173.8709475124489359 ) ) ;
#54708=CIRCLE ( 'NONE', #43120, 5.599999999999994316 ) ;
#54711=ORIENTED_EDGE ( 'NONE', *, *, #50579, .T. ) ;
#54714=DIRECTION ( 'NONE',  ( -0.04216478779797398074, 0.9991106698809455455, 0.000000000000000000 ) ) ;
#54718=EDGE_CURVE ( 'NONE', #27069, #21321, #1922, .T. ) ;
#54719=CARTESIAN_POINT ( 'NONE',  ( 104.1527054293246550, -27.79712248444839773, 206.7711071154209606 ) ) ;
#54721=AXIS2_PLACEMENT_3D ( 'NONE', #66896, #40978, #6037 ) ;
#54724=DIRECTION ( 'NONE',  ( 4.299999999999999979E-14, -1.000000000000000000, 4.400000000000000367E-29 ) ) ;
#54730=ORIENTED_EDGE ( 'NONE', *, *, #9088, .T. ) ;
#54731=ORIENTED_EDGE ( 'NONE', *, *, #76149, .F. ) ;
#54732=CARTESIAN_POINT ( 'NONE',  ( 100.6247221172615127, -30.94977259965520844, 233.5747570362579495 ) ) ;
#54733=CARTESIAN_POINT ( 'NONE',  ( 107.6542440074338458, -47.14984605634950299, 152.6213395616249500 ) ) ;
#54734=CARTESIAN_POINT ( 'NONE',  ( 117.8527506973083518, -39.03601561205234560, 108.6708633711489824 ) ) ;
#54735=CARTESIAN_POINT ( 'NONE',  ( 99.32188085270527722, -38.83570505065259937, 249.5838068554172935 ) ) ;
#54737=CARTESIAN_POINT ( 'NONE',  ( 114.9650091533680722, -29.92534717146685708, 180.3927681330539770 ) ) ;
#54738=CARTESIAN_POINT ( 'NONE',  ( 98.75905348231658820, -42.39375861569092052, 276.8019443637107884 ) ) ;
#54739=VERTEX_POINT ( 'NONE', #80084 ) ;
#54742=ORIENTED_EDGE ( 'NONE', *, *, #70246, .T. ) ;
#54743=DIRECTION ( 'NONE',  ( 0.000000000000000000, 0.000000000000000000, 1.000000000000000000 ) ) ;
#54744=VECTOR ( 'NONE', #33953, 1000.000000000000000 ) ;
#54746=AXIS2_PLACEMENT_3D ( 'NONE', #28435, #74800, #728 ) ;
#54748=CARTESIAN_POINT ( 'NONE',  ( 101.5007711604877159, -27.91412646590841362, 110.5241967044819944 ) ) ;
#54750=DIRECTION ( 'NONE',  ( -0.7071067811865516806, 0.7071067811865433539, -7.071067811865510832E-16 ) ) ;
#54751=CYLINDRICAL_SURFACE ( 'NONE', #71690, 2.517499999999998739 ) ;
#54752=DIRECTION ( 'NONE',  ( 0.000000000000000000, 0.000000000000000000, -1.000000000000000000 ) ) ;
#54754=CARTESIAN_POINT ( 'NONE',  ( 113.1426608820137716, -26.58408993604434301, 200.6470538473399756 ) ) ;
#54756=DIRECTION ( 'NONE',  ( 1.000000000000000000, 4.299999999999999979E-14, 1.000000000000000078E-15 ) ) ;
#54757=ORIENTED_EDGE ( 'NONE', *, *, #83553, .F. ) ;
#54759=DIRECTION ( 'NONE',  ( -1.000000000000000078E-15, 1.000000000000000083E-30, 1.000000000000000000 ) ) ;
#54760=LINE ( 'NONE', #75694, #13959 ) ;
#54762=CARTESIAN_POINT ( 'NONE',  ( 106.1344186357298867, -47.79037565197016590, 262.4975300378158067 ) ) ;
#54763=ORIENTED_EDGE ( 'NONE', *, *, #64465, .F. ) ;
#54765=CARTESIAN_POINT ( 'NONE',  ( 112.1308356434906273, -47.47125106351535351, 137.9270538473389820 ) ) ;
#54766=CARTESIAN_POINT ( 'NONE',  ( 96.71473009235836571, -37.96382682441392831, 37.42133956162496844 ) ) ;
#54767=CARTESIAN_POINT ( 'NONE',  ( 99.06808600115306263, -45.54042523694053557, 152.9899109901969894 ) ) ;
#54768=AXIS2_PLACEMENT_3D ( 'NONE', #17126, #72091, #45680 ) ;
#54773=CARTESIAN_POINT ( 'NONE',  ( 51.56670390244699576, -19.82844715994031048, -5.074374724088000832 ) ) ;
#54775=DIRECTION ( 'NONE',  ( 1.000000000000000078E-15, -1.000000000000000083E-30, -1.000000000000000000 ) ) ;
#54776=VERTEX_POINT ( 'NONE', #38280 ) ;
#54778=AXIS2_PLACEMENT_3D ( 'NONE', #40926, #68649, #48177 ) ;
#54779=EDGE_CURVE ( 'NONE', #2705, #54188, #59599, .T. ) ;
#54780=VERTEX_POINT ( 'NONE', #46415 ) ;
#54783=AXIS2_PLACEMENT_3D ( 'NONE', #47106, #12618, #41197 ) ;
#54784=EDGE_CURVE ( 'NONE', #30635, #6148, #88041, .T. ) ;
#54787=CARTESIAN_POINT ( 'NONE',  ( 100.5643946202652756, -27.81952766013699119, 26.56610146638793779 ) ) ;
#54790=CARTESIAN_POINT ( 'NONE',  ( 115.3189361407783480, -42.43561143203083930, 118.3469642877515327 ) ) ;
#54792=AXIS2_PLACEMENT_3D ( 'NONE', #46668, #60299, #33052 ) ;
#54793=CARTESIAN_POINT ( 'NONE',  ( 162.5667039024460223, -22.48495420874110806, -5.074374724088000832 ) ) ;
#54794=VECTOR ( 'NONE', #32308, 1000.000000000000000 ) ;
#54795=CARTESIAN_POINT ( 'NONE',  ( 100.4104977919876802, -31.37650509455747283, 240.2095626852199928 ) ) ;
#54796=VERTEX_POINT ( 'NONE', #34141 ) ;
#54798=ORIENTED_EDGE ( 'NONE', *, *, #16895, .F. ) ;
#54800=EDGE_CURVE ( 'NONE', #23215, #7800, #55565, .T. ) ;
#54802=CARTESIAN_POINT ( 'NONE',  ( 116.7952057194422224, -39.38754349606188754, 103.6145979094304721 ) ) ;
#54804=CARTESIAN_POINT ( 'NONE',  ( 63.56670390244739366, -47.82844715994014706, 180.4678068554151196 ) ) ;
#54807=FACE_OUTER_BOUND ( 'NONE', #48091, .T. ) ;
#54808=CARTESIAN_POINT ( 'NONE',  ( 101.2327472597881552, -44.62129728587218835, 257.0699109901973998 ) ) ;
#54810=EDGE_CURVE ( 'NONE', #68056, #79637, #80320, .T. ) ;
#54813=LINE ( 'NONE', #80771, #8964 ) ;
#54814=CARTESIAN_POINT ( 'NONE',  ( 115.5148531418241191, -38.60720430987922214, 101.4585665600679647 ) ) ;
#54815=VECTOR ( 'NONE', #55849, 1000.000000000000000 ) ;
#54817=CARTESIAN_POINT ( 'NONE',  ( 25.56670390244797275, -48.82844715994099971, 175.9678068554150059 ) ) ;
#54818=ORIENTED_EDGE ( 'NONE', *, *, #809, .T. ) ;
#54820=ORIENTED_EDGE ( 'NONE', *, *, #86404, .T. ) ;
#54821=CARTESIAN_POINT ( 'NONE',  ( 96.64983689172015602, -37.15430107835312157, 161.3584824187679487 ) ) ;
#54823=CARTESIAN_POINT ( 'NONE',  ( 184.5664832912729878, -81.37844715994266664, 342.9256252759109884 ) ) ;
#54824=CARTESIAN_POINT ( 'NONE',  ( 112.9789619575112596, -30.12862337550717484, 110.9272975916109658 ) ) ;
#54826=ADVANCED_FACE ( 'NONE', ( #61839 ), #64305, .T. ) ;
#54827=CARTESIAN_POINT ( 'NONE',  ( 80.06648329127401098, -41.22944715994105280, 4.925625275910944012 ) ) ;
#54828=CARTESIAN_POINT ( 'NONE',  ( 111.9390199320367145, -27.48847072138506320, 55.68991099019693536 ) ) ;
#54829=CARTESIAN_POINT ( 'NONE',  ( 117.0608945229798081, -38.08045312644978964, 84.71895860879563145 ) ) ;
#54831=ORIENTED_EDGE ( 'NONE', *, *, #5335, .T. ) ;
#54832=CIRCLE ( 'NONE', #30246, 11.45913725231036118 ) ;
#54833=FACE_OUTER_BOUND ( 'NONE', #55365, .T. ) ;
#54835=VERTEX_POINT ( 'NONE', #89130 ) ;
#54838=EDGE_LOOP ( 'NONE', ( #30890, #7077, #37254, #63976 ) ) ;
#54839=CARTESIAN_POINT ( 'NONE',  ( 98.19951187208806687, -40.85743130997450834, 256.6727681330542623 ) ) ;
#54840=CARTESIAN_POINT ( 'NONE',  ( 117.8230732226064532, -34.08729308082334342, 160.0061014663869798 ) ) ;
#54841=CARTESIAN_POINT ( 'NONE',  ( 107.0664832912739968, -36.72944715994100306, 287.6356252759109680 ) ) ;
#54842=CARTESIAN_POINT ( 'NONE',  ( 20.56670390244828184, -48.82844715994187368, 300.4678068554150059 ) ) ;
#54843=CARTESIAN_POINT ( 'NONE',  ( 98.30635682897023742, -28.74854496012902771, 76.73848241876795839 ) ) ;
#54844=DIRECTION ( 'NONE',  ( -1.000000000000000078E-15, 1.000000000000000083E-30, 1.000000000000000000 ) ) ;
#54847=CARTESIAN_POINT ( 'NONE',  ( 99.09536660752770842, -30.55085998965113347, 115.8042979613130399 ) ) ;
#54852=ADVANCED_FACE ( 'NONE', ( #40515 ), #34594, .T. ) ;
#54855=CARTESIAN_POINT ( 'NONE',  ( 96.78489722101812731, -35.14273565208913652, 266.2041967044821149 ) ) ;
#54858=DIRECTION ( 'NONE',  ( 4.299999999999999979E-14, -1.000000000000000000, 0.000000000000000000 ) ) ;
#54859=CARTESIAN_POINT ( 'NONE',  ( 100.8732324256648951, -44.32512360075851632, 12.03276813305398463 ) ) ;
#54861=CARTESIAN_POINT ( 'NONE',  ( 101.6894933626720245, -27.09867346898214180, 101.4937205140059575 ) ) ;
#54862=CARTESIAN_POINT ( 'NONE',  ( 116.6018603435394141, -39.73108032723776972, 249.5838075904518121 ) ) ;
#54863=CARTESIAN_POINT ( 'NONE',  ( 95.26177648276406273, -38.28579333248966776, 151.4299109901969871 ) ) ;
#54864=CARTESIAN_POINT ( 'NONE',  ( 161.4809174648183898, -48.32844715993547879, 249.9678068554149490 ) ) ;
#54865=VERTEX_POINT ( 'NONE', #979 ) ;
#54866=AXIS2_PLACEMENT_3D ( 'NONE', #75887, #13657, #26387 ) ;
#54867=CARTESIAN_POINT ( 'NONE',  ( 41.56648329127398966, -27.82844715994070484, 18.92562527591200094 ) ) ;
#54868=CARTESIAN_POINT ( 'NONE',  ( 150.5667039024475571, -25.42844715993593852, 180.4678068554149775 ) ) ;
#54871=CARTESIAN_POINT ( 'NONE',  ( 45.56670390244743629, -48.82844715994092866, 180.4678068554150911 ) ) ;
#54872=CARTESIAN_POINT ( 'NONE',  ( 113.1024245609201984, -28.17526227570857955, 129.5870538473399449 ) ) ;
#54873=ORIENTED_EDGE ( 'NONE', *, *, #26669, .F. ) ;
#54874=DIRECTION ( 'NONE',  ( 0.000000000000000000, 0.000000000000000000, -1.000000000000000000 ) ) ;
#54876=AXIS2_PLACEMENT_3D ( 'NONE', #20004, #34056, #80447 ) ;
#54878=AXIS2_PLACEMENT_3D ( 'NONE', #52440, #12942, #67890 ) ;
#54880=ORIENTED_EDGE ( 'NONE', *, *, #34190, .T. ) ;
#54882=EDGE_CURVE ( 'NONE', #88430, #2245, #62298, .T. ) ;
#54885=ORIENTED_EDGE ( 'NONE', *, *, #72075, .T. ) ;
#54887=ORIENTED_EDGE ( 'NONE', *, *, #71521, .F. ) ;
#54888=DIRECTION ( 'NONE',  ( 1.000000000000000000, 4.163336342344333240E-14, 0.000000000000000000 ) ) ;
#54890=CARTESIAN_POINT ( 'NONE',  ( 167.2371591254542693, -47.82818131005522844, 300.4678068554149490 ) ) ;
#54892=EDGE_CURVE ( 'NONE', #36690, #2932, #10655, .T. ) ;
#54894=CARTESIAN_POINT ( 'NONE',  ( 36.74138383868169910, -48.33240602328862678, 249.9678068554150343 ) ) ;
#54895=CARTESIAN_POINT ( 'NONE',  ( 64.67079002020506096, -0.9301828534102468682, 361.9756252759101471 ) ) ;
#54896=ORIENTED_EDGE ( 'NONE', *, *, #24591, .T. ) ;
#54897=VECTOR ( 'NONE', #59491, 1000.000000000000000 ) ;
#54898=CIRCLE ( 'NONE', #83932, 2.030000000002086580 ) ;
#54900=DIRECTION ( 'NONE',  ( 1.387778780781444492E-15, 0.000000000000000000, -1.000000000000000000 ) ) ;
#54901=DIRECTION ( 'NONE',  ( 0.000000000000000000, 1.000000000000000000, 0.000000000000000000 ) ) ;
#54902=CARTESIAN_POINT ( 'NONE',  ( 106.8648936900573148, -47.09757847023101363, 223.5489586092439538 ) ) ;
#54903=EDGE_CURVE ( 'NONE', #41003, #59850, #67198, .T. ) ;
#54905=CARTESIAN_POINT ( 'NONE',  ( 98.70071965984716655, -42.85747980491196074, 102.8175300378149899 ) ) ;
#54906=CARTESIAN_POINT ( 'NONE',  ( 165.3359832912740046, -36.32844715994100682, -5.074374724088000832 ) ) ;
#54908=CARTESIAN_POINT ( 'NONE',  ( 179.4595971212889935, -28.98061976758940617, 193.9678068554150059 ) ) ;
#54909=VERTEX_POINT ( 'NONE', #21431 ) ;
#54910=DIRECTION ( 'NONE',  ( 0.000000000000000000, 1.000000000000000000, 1.914177628664063178E-15 ) ) ;
#54911=CIRCLE ( 'NONE', #14379, 16.00000000000000000 ) ;
#54912=EDGE_LOOP ( 'NONE', ( #2984, #63995 ) ) ;
#54915=CARTESIAN_POINT ( 'NONE',  ( 105.3283384058428851, -27.49606390364131414, 276.6682499725636717 ) ) ;
#54918=CARTESIAN_POINT ( 'NONE',  ( 97.33784131412605234, -34.07106451907700517, 81.11479194169517370 ) ) ;
#54921=ORIENTED_EDGE ( 'NONE', *, *, #79066, .T. ) ;
#54923=CARTESIAN_POINT ( 'NONE',  ( 100.8869759769006578, -44.69981387740176615, 183.0527697648384731 ) ) ;
#54925=CARTESIAN_POINT ( 'NONE',  ( 99.12728904495253346, -44.42023919799950704, 41.95086337114900488 ) ) ;
#54926=ORIENTED_EDGE ( 'NONE', *, *, #57344, .F. ) ;
#54927=CARTESIAN_POINT ( 'NONE',  ( 110.0622958990556839, -29.10660024649327227, 267.5966617981628701 ) ) ;
#54929=CARTESIAN_POINT ( 'NONE',  ( 113.7965574739370993, -44.62378898692907825, 153.1508633711499670 ) ) ;
#54931=FACE_OUTER_BOUND ( 'NONE', #9556, .T. ) ;
#54932=FACE_OUTER_BOUND ( 'NONE', #39914, .T. ) ;
#54935=CARTESIAN_POINT ( 'NONE',  ( 106.9399153568602259, -47.82816235210678002, 228.5794347997199907 ) ) ;
#54936=LINE ( 'NONE', #61324, #15199 ) ;
#54937=EDGE_LOOP ( 'NONE', ( #36687, #61884, #81252, #23968 ) ) ;
#54939=CARTESIAN_POINT ( 'NONE',  ( 116.5728860035299164, -32.34523831224304047, 100.1699109901969535 ) ) ;
#54942=ORIENTED_EDGE ( 'NONE', *, *, #47930, .T. ) ;
#54943=ORIENTED_EDGE ( 'NONE', *, *, #38610, .T. ) ;
#54945=CARTESIAN_POINT ( 'NONE',  ( 113.2433956935260113, -28.75706466399002537, 159.5522588191168154 ) ) ;
#54948=PLANE ( 'NONE',  #34476 ) ;
#54949=CARTESIAN_POINT ( 'NONE',  ( 115.0870346033256055, -35.21269407640084381, 156.7938046553059905 ) ) ;
#54950=CARTESIAN_POINT ( 'NONE',  ( 112.5006845157638651, -46.38111348219169372, 253.9965776568635647 ) ) ;
#54951=CYLINDRICAL_SURFACE ( 'NONE', #66785, 2.750000000000002665 ) ;
#54952=EDGE_LOOP ( 'NONE', ( #22108, #58307 ) ) ;
#54958=VECTOR ( 'NONE', #74304, 1000.000000000000000 ) ;
#54960=DIRECTION ( 'NONE',  ( 0.000000000000000000, 0.000000000000000000, -1.000000000000000000 ) ) ;
#54961=ORIENTED_EDGE ( 'NONE', *, *, #11778, .T. ) ;
#54962=ORIENTED_EDGE ( 'NONE', *, *, #29187, .T. ) ;
#54963=CARTESIAN_POINT ( 'NONE',  ( 63.03715912545637678, -24.42818131006026761, 193.9678068554150911 ) ) ;
#54964=CARTESIAN_POINT ( 'NONE',  ( 97.39131799614082752, -39.27861749894243815, 16.53146768276753420 ) ) ;
#54966=CARTESIAN_POINT ( 'NONE',  ( 125.0235919798090833, -56.62589376934762697, 14.92562527591091204 ) ) ;
#54967=CARTESIAN_POINT ( 'NONE',  ( 102.9027671602101037, -44.22047980607887752, 186.5952769709339805 ) ) ;
#54968=CARTESIAN_POINT ( 'NONE',  ( 105.9838489277333480, -26.31625509990853828, 50.15848241876796720 ) ) ;
#54969=LINE ( 'NONE', #41799, #55288 ) ;
#54973=ORIENTED_EDGE ( 'NONE', *, *, #449, .T. ) ;
#54975=EDGE_LOOP ( 'NONE', ( #16534, #35640, #43651, #83939 ) ) ;
#54977=DIRECTION ( 'NONE',  ( 0.000000000000000000, 0.000000000000000000, -1.000000000000000000 ) ) ;
#54978=CARTESIAN_POINT ( 'NONE',  ( 115.9858208431400044, -41.32354544834976906, 133.4481121647361306 ) ) ;
#54979=LINE ( 'NONE', #83189, #13277 ) ;
#54980=ORIENTED_EDGE ( 'NONE', *, *, #7536, .T. ) ;
#54981=CARTESIAN_POINT ( 'NONE',  ( 97.26762016986505444, -33.10609988230974920, 66.04419670448297097 ) ) ;
#54983=CARTESIAN_POINT ( 'NONE',  ( 115.8250108040429467, -31.72928582533900865, 164.2398587763299531 ) ) ;
#54985=PLANE ( 'NONE',  #81495 ) ;
#54986=DIRECTION ( 'NONE',  ( 1.000000000000000078E-15, -1.000000000000000000, 0.000000000000000000 ) ) ;
#54987=VERTEX_POINT ( 'NONE', #8245 ) ;
#54988=ADVANCED_FACE ( 'NONE', ( #23244 ), #43642, .T. ) ;
#54989=CIRCLE ( 'NONE', #66624, 1.000000000000000888 ) ;
#54990=ADVANCED_FACE ( 'NONE', ( #77286 ), #70476, .T. ) ;
#54992=ADVANCED_FACE ( 'NONE', ( #51340 ), #43190, .T. ) ;
#54993=LINE ( 'NONE', #82761, #9580 ) ;
#54995=ORIENTED_EDGE ( 'NONE', *, *, #37415, .T. ) ;
#54996=CARTESIAN_POINT ( 'NONE',  ( 96.01268936646508223, -41.06948063400285776, 92.62419670448296927 ) ) ;
#54997=EDGE_CURVE ( 'NONE', #33634, #61676, #30477, .T. ) ;
#55000=CARTESIAN_POINT ( 'NONE',  ( 163.0667039024470171, -33.35206098992711077, -5.074374724088000832 ) ) ;
#55001=AXIS2_PLACEMENT_3D ( 'NONE', #49234, #29268, #84694 ) ;
#55002=CYLINDRICAL_SURFACE ( 'NONE', #4158, 1.000000000000000888 ) ;
#55003=ORIENTED_EDGE ( 'NONE', *, *, #42514, .F. ) ;
#55004=CARTESIAN_POINT ( 'NONE',  ( 116.5944731948637809, -42.45914096480943556, 124.3956252759109731 ) ) ;
#55006=CARTESIAN_POINT ( 'NONE',  ( 130.3998166246059895, 12.92155284005730387, 355.9756252759109998 ) ) ;
#55008=VECTOR ( 'NONE', #80212, 1000.000000000000000 ) ;
#55009=CARTESIAN_POINT ( 'NONE',  ( 106.8369185487093063, -47.13021470646864941, 268.5584824187679374 ) ) ;
#55010=CARTESIAN_POINT ( 'NONE',  ( 97.83847648579691736, -40.58231914350135838, 252.6411887015405000 ) ) ;
#55012=ADVANCED_FACE ( 'NONE', ( #56819, #71818, #42736, #1438 ), #63656, .F. ) ;
#55013=DIRECTION ( 'NONE',  ( -2.900000000000000265E-14, 2.000000000000000155E-15, -1.000000000000000000 ) ) ;
#55014=CARTESIAN_POINT ( 'NONE',  ( 97.06107109349493101, -37.99641193259417093, 82.42729194011009497 ) ) ;
#55018=CARTESIAN_POINT ( 'NONE',  ( 101.7740290765682403, -45.64733444449330335, 207.1622919425779514 ) ) ;
#55019=EDGE_LOOP ( 'NONE', ( #33033, #36431, #70353, #62602 ) ) ;
#55022=CARTESIAN_POINT ( 'NONE',  ( 107.5650335644346569, -45.56823575777373492, 149.0530118773259858 ) ) ;
#55024=DIRECTION ( 'NONE',  ( -4.237773401492740281E-14, 1.000000000000000000, 0.000000000000000000 ) ) ;
#55025=CARTESIAN_POINT ( 'NONE',  ( 111.3597915011938539, -28.37217101237177985, 16.14253568684992501 ) ) ;
#55026=CARTESIAN_POINT ( 'NONE',  ( 97.80782663584228942, -40.50797902753792101, 57.63481331718827505 ) ) ;
#55027=DIRECTION ( 'NONE',  ( -0.7071067811865753283, 0.7071067811865197061, -7.071067811865760309E-16 ) ) ;
#55028=B_SPLINE_CURVE_WITH_KNOTS ( 'NONE', 3,
 ( #72243, #15040, #51321, #21865, #42714, #2762, #3205, #30459, #30899, #84092, #70456, #8228, #35918, #63633, #84550, #11344, #87654, #3637 ),
 .UNSPECIFIED., .F., .F.,
 ( 4, 2, 2, 2, 2, 2, 2, 2, 4 ),
 ( 0.4999949742048476198, 0.5624956024292416812, 0.6249962306536357426, 0.6874968588780296930, 0.7499974871024237544, 0.8124981153268178158, 0.8749987435512118772, 0.9374993717756059386, 1.000000000000000000 ),
 .UNSPECIFIED. ) ;
#55030=AXIS2_PLACEMENT_3D ( 'NONE', #83436, #48884, #76623 ) ;
#55031=DIRECTION ( 'NONE',  ( 0.000000000000000000, 0.000000000000000000, -1.000000000000000000 ) ) ;
#55032=CARTESIAN_POINT ( 'NONE',  ( 97.33784130911575971, -34.07106453693553760, 107.1147919431604834 ) ) ;
#55034=STYLED_ITEM ( 'NONE', ( #29559 ), #56477 ) ;
#55035=CARTESIAN_POINT ( 'NONE',  ( 96.21411768969875311, -32.03111041547175120, 211.0013395616249738 ) ) ;
#55036=CARTESIAN_POINT ( 'NONE',  ( 51.56670390244699576, -19.82844715994031048, 342.9256252759119548 ) ) ;
#55039=LINE ( 'NONE', #20564, #64866 ) ;
#55040=CARTESIAN_POINT ( 'NONE',  ( 78.21890182792367341, -16.68450975841368233, 2.186797062523622159 ) ) ;
#55041=AXIS2_PLACEMENT_3D ( 'NONE', #16338, #49940, #8181 ) ;
#55044=EDGE_CURVE ( 'NONE', #8645, #21680, #8706, .T. ) ;
#55045=CARTESIAN_POINT ( 'NONE',  ( 107.0664832912739399, -36.72944715994095333, 293.9356252759109793 ) ) ;
#55046=EDGE_LOOP ( 'NONE', ( #5252, #64423, #20786, #69477 ) ) ;
#55049=EDGE_CURVE ( 'NONE', #66156, #46554, #16406, .T. ) ;
#55050=CARTESIAN_POINT ( 'NONE',  ( 99.39677155223240845, -28.76988628678374837, 265.6746728949588032 ) ) ;
#55051=ORIENTED_EDGE ( 'NONE', *, *, #13213, .F. ) ;
#55054=PLANE ( 'NONE',  #66010 ) ;
#55055=CARTESIAN_POINT ( 'NONE',  ( 110.8627678800837657, -45.98083881433460363, 167.8863385848088399 ) ) ;
#55056=CARTESIAN_POINT ( 'NONE',  ( 100.0434009169665757, -32.56939427797095021, 83.71951894101997027 ) ) ;
#55057=CARTESIAN_POINT ( 'NONE',  ( 104.5573670441197720, -48.33662538491821437, 178.4070538473399665 ) ) ;
#55058=CARTESIAN_POINT ( 'NONE',  ( 173.8164832912740394, 12.92155284005802685, 336.5756252759111362 ) ) ;
#55061=AXIS2_PLACEMENT_3D ( 'NONE', #89598, #82797, #35501 ) ;
#55062=ORIENTED_EDGE ( 'NONE', *, *, #67127, .F. ) ;
#55063=ORIENTED_EDGE ( 'NONE', *, *, #5444, .T. ) ;
#55064=EDGE_CURVE ( 'NONE', #38655, #41295, #2333, .T. ) ;
#55067=ORIENTED_EDGE ( 'NONE', *, *, #41464, .T. ) ;
#55068=CARTESIAN_POINT ( 'NONE',  ( 73.06670390244801183, -58.35344715994099829, 310.9178068554150514 ) ) ;
#55069=CARTESIAN_POINT ( 'NONE',  ( 112.6295607727957133, -43.21082823627408231, 107.5638483995059715 ) ) ;
#55070=CARTESIAN_POINT ( 'NONE',  ( 113.1129168750088638, -46.01039980791943407, 223.0480062282919675 ) ) ;
#55071=VECTOR ( 'NONE', #32359, 1000.000000000000000 ) ;
#55072=CARTESIAN_POINT ( 'NONE',  ( 117.1759530674219860, -34.27439392744687296, 209.0156252759109634 ) ) ;
#55074=CARTESIAN_POINT ( 'NONE',  ( 97.50674219252222485, -32.62548708300533207, 12.00419670448293985 ) ) ;
#55075=DIRECTION ( 'NONE',  ( 1.000000000000000078E-15, 1.000000000000000083E-30, -1.000000000000000000 ) ) ;
#55077=ADVANCED_FACE ( 'NONE', ( #44083, #37289 ), #64110, .T. ) ;
#55078=ORIENTED_EDGE ( 'NONE', *, *, #16864, .F. ) ;
#55080=CARTESIAN_POINT ( 'NONE',  ( 114.6661721138975025, -42.88640786233948887, 88.28419670448295165 ) ) ;
#55081=CARTESIAN_POINT ( 'NONE',  ( 101.0407447616467351, -27.40725005837418138, 70.54514908543497143 ) ) ;
#55082=CARTESIAN_POINT ( 'NONE',  ( 96.97388998173752839, -33.94624283173551049, 251.1127681330538337 ) ) ;
#55083=VERTEX_POINT ( 'NONE', #64997 ) ;
#55084=CARTESIAN_POINT ( 'NONE',  ( 98.94247553594858857, -30.19587780982054070, 240.7870538473399620 ) ) ;
#55087=EDGE_CURVE ( 'NONE', #83503, #81882, #72264, .T. ) ;
#55088=DIRECTION ( 'NONE',  ( 0.000000000000000000, 0.000000000000000000, 1.000000000000000000 ) ) ;
#55091=CARTESIAN_POINT ( 'NONE',  ( 181.8884939055940038, -32.11662333284530746, -5.074374724088000832 ) ) ;
#55092=DIRECTION ( 'NONE',  ( 0.000000000000000000, 0.000000000000000000, -1.000000000000000000 ) ) ;
#55093=FACE_OUTER_BOUND ( 'NONE', #53079, .T. ) ;
#55095=CARTESIAN_POINT ( 'NONE',  ( 107.0664832912739399, -36.72944715994095333, 293.6356252759106837 ) ) ;
#55096=AXIS2_PLACEMENT_3D ( 'NONE', #56871, #35989, #15563 ) ;
#55098=CARTESIAN_POINT ( 'NONE',  ( 98.41530666024773666, -31.56922914487509502, 277.3301547344686355 ) ) ;
#55099=CARTESIAN_POINT ( 'NONE',  ( 97.07187113119439914, -35.38041075382983536, 41.21846444838222823 ) ) ;
#55100=EDGE_CURVE ( 'NONE', #61174, #52592, #78202, .T. ) ;
#55104=DIRECTION ( 'NONE',  ( 0.000000000000000000, 1.000000000000000000, 0.000000000000000000 ) ) ;
#55105=CARTESIAN_POINT ( 'NONE',  ( 106.2251211966456879, -47.77424462129209815, 267.5280062282920994 ) ) ;
#55106=CARTESIAN_POINT ( 'NONE',  ( 95.67524734051724522, -33.46228404877688689, 137.1041967044819501 ) ) ;
#55107=CARTESIAN_POINT ( 'NONE',  ( 103.9262362324350590, -26.74286475366834281, 246.3184824187679567 ) ) ;
#55109=DIRECTION ( 'NONE',  ( 0.000000000000000000, 0.000000000000000000, -1.000000000000000000 ) ) ;
#55113=ORIENTED_EDGE ( 'NONE', *, *, #43647, .T. ) ;
#55117=CARTESIAN_POINT ( 'NONE',  ( 99.37165735872611094, -40.43697808898449608, 171.1067055423629597 ) ) ;
#55118=EDGE_CURVE ( 'NONE', #68275, #63748, #44527, .T. ) ;
#55120=ORIENTED_EDGE ( 'NONE', *, *, #34231, .T. ) ;
#55121=DIRECTION ( 'NONE',  ( -0.0001713722456133601202, 0.9999999853157766072, 1.713722456133601401E-19 ) ) ;
#55122=CARTESIAN_POINT ( 'NONE',  ( 102.6926969729870507, -27.29023857175978662, 176.4213395616249898 ) ) ;
#55123=CARTESIAN_POINT ( 'NONE',  ( 63.03715912545740707, -46.82818131006016671, 129.9678068554150911 ) ) ;
#55124=EDGE_CURVE ( 'NONE', #40542, #77354, #75282, .T. ) ;
#55125=CARTESIAN_POINT ( 'NONE',  ( 182.0667039024477276, -33.35206098992059509, 237.4678068554150059 ) ) ;
#55126=CARTESIAN_POINT ( 'NONE',  ( 112.8675307907708287, -28.58609239232746546, 195.5838076129389833 ) ) ;
#55128=CARTESIAN_POINT ( 'NONE',  ( 114.2351621074132879, -44.22269940884951467, 113.1718157521019776 ) ) ;
#55129=VERTEX_POINT ( 'NONE', #33485 ) ;
#55131=VERTEX_POINT ( 'NONE', #12155 ) ;
#55132=ORIENTED_EDGE ( 'NONE', *, *, #38990, .T. ) ;
#55133=DIRECTION ( 'NONE',  ( 1.000000000000000000, 0.000000000000000000, 0.000000000000000000 ) ) ;
#55134=CARTESIAN_POINT ( 'NONE',  ( 99.18511857479145988, -30.88155312011797804, 176.8184824187669619 ) ) ;
#55135=CARTESIAN_POINT ( 'NONE',  ( 138.8167039024479834, -57.40094715994099772, 86.31780685541500020 ) ) ;
#55137=DIRECTION ( 'NONE',  ( -4.237773401492740281E-14, 1.000000000000000000, 0.000000000000000000 ) ) ;
#55139=AXIS2_PLACEMENT_3D ( 'NONE', #31709, #4907, #47111 ) ;
#55142=CARTESIAN_POINT ( 'NONE',  ( 109.5033840998384136, -46.84330794493983774, 132.7641967044819751 ) ) ;
#55144=ORIENTED_EDGE ( 'NONE', *, *, #35121, .F. ) ;
#55146=AXIS2_PLACEMENT_3D ( 'NONE', #71912, #9672, #17384 ) ;
#55147=DIRECTION ( 'NONE',  ( 1.000000000000000078E-15, 0.000000000000000000, -1.000000000000000000 ) ) ;
#55149=CARTESIAN_POINT ( 'NONE',  ( 86.06670390244804025, -16.72944715994094622, 239.5838068554176346 ) ) ;
#55150=CARTESIAN_POINT ( 'NONE',  ( 115.2023469127646820, -39.68048904007974897, 171.3557094172109885 ) ) ;
#55151=AXIS2_PLACEMENT_3D ( 'NONE', #30451, #77708, #15490 ) ;
#55153=CARTESIAN_POINT ( 'NONE',  ( 99.09599905102065520, -30.55004517099500561, 26.80180474063285345 ) ) ;
#55155=VERTEX_POINT ( 'NONE', #88915 ) ;
#55156=ORIENTED_EDGE ( 'NONE', *, *, #26310, .F. ) ;
#55157=VECTOR ( 'NONE', #64051, 1000.000000000000000 ) ;
#55158=DIRECTION ( 'NONE',  ( 0.4808135048159887792, 0.02029144519433677407, -0.8765880622267739897 ) ) ;
#55159=ORIENTED_EDGE ( 'NONE', *, *, #17970, .T. ) ;
#55160=ORIENTED_EDGE ( 'NONE', *, *, #82620, .F. ) ;
#55161=LINE ( 'NONE', #21131, #34758 ) ;
#55162=CARTESIAN_POINT ( 'NONE',  ( 116.3948728625927060, -35.60798670905003860, 235.3653928297059679 ) ) ;
#55165=DIRECTION ( 'NONE',  ( 1.000000000000000000, -9.073094938289460781E-13, 0.000000000000000000 ) ) ;
#55167=ORIENTED_EDGE ( 'NONE', *, *, #40278, .F. ) ;
#55170=DIRECTION ( 'NONE',  ( -1.000000000000000078E-15, 1.000000000000000083E-30, 1.000000000000000000 ) ) ;
#55173=EDGE_CURVE ( 'NONE', #22477, #2950, #7810, .T. ) ;
#55174=VECTOR ( 'NONE', #40879, 1000.000000000000000 ) ;
#55175=CARTESIAN_POINT ( 'NONE',  ( 101.6421866332951396, -42.82917926744636361, 264.8166617981626700 ) ) ;
#55176=EDGE_CURVE ( 'NONE', #73698, #82549, #58570, .T. ) ;
#55177=CARTESIAN_POINT ( 'NONE',  ( 107.3345184958865275, -26.28557234761613159, 120.0556252759109555 ) ) ;
#55178=AXIS2_PLACEMENT_3D ( 'NONE', #89231, #5207, #53771 ) ;
#55179=CARTESIAN_POINT ( 'NONE',  ( 108.0321269276242049, -25.74166508409281917, 109.9946728949589811 ) ) ;
#55180=CARTESIAN_POINT ( 'NONE',  ( 103.0103351263445859, -43.74012547698517750, 249.5838068554171514 ) ) ;
#55181=CARTESIAN_POINT ( 'NONE',  ( 132.2214349158033713, -16.68812225916125058, 7.662832107305504792 ) ) ;
#55182=CARTESIAN_POINT ( 'NONE',  ( 97.42522746746806206, -42.13501527293522742, 177.7451490854349743 ) ) ;
#55184=CARTESIAN_POINT ( 'NONE',  ( 142.8687636814963184, 5.654319119531167281, 394.9756252759100903 ) ) ;
#55185=ORIENTED_EDGE ( 'NONE', *, *, #68062, .F. ) ;
#55188=ORIENTED_EDGE ( 'NONE', *, *, #873, .F. ) ;
#55189=EDGE_CURVE ( 'NONE', #25661, #47060, #88015, .T. ) ;
#55190=VERTEX_POINT ( 'NONE', #68011 ) ;
#55191=LINE ( 'NONE', #49741, #43141 ) ;
#55194=EDGE_CURVE ( 'NONE', #75223, #32339, #74528, .T. ) ;
#55195=EDGE_CURVE ( 'NONE', #82764, #14401, #47551, .T. ) ;
#55196=DIRECTION ( 'NONE',  ( -1.000000000000000078E-15, 1.000000000000000083E-30, 1.000000000000000000 ) ) ;
#55197=CARTESIAN_POINT ( 'NONE',  ( 116.7957173713512873, -32.98391181527420457, 139.1184824187679396 ) ) ;
#55199=EDGE_CURVE ( 'NONE', #48508, #71603, #60731, .T. ) ;
#55200=CARTESIAN_POINT ( 'NONE',  ( 136.8118108218990869, -36.54506369575593538, 6.756870620000529293 ) ) ;
#55201=FACE_OUTER_BOUND ( 'NONE', #30210, .T. ) ;
#55204=CARTESIAN_POINT ( 'NONE',  ( 114.7977927517517855, -29.71579763117551565, 205.4127681330539872 ) ) ;
#55205=CARTESIAN_POINT ( 'NONE',  ( 194.5667039024479834, -48.82844715994099971, 20.91780685541479912 ) ) ;
#55206=CYLINDRICAL_SURFACE ( 'NONE', #39499, 5.600000000000000533 ) ;
#55209=EDGE_CURVE ( 'NONE', #16685, #89473, #3468, .T. ) ;
#55210=CARTESIAN_POINT ( 'NONE',  ( 177.4809174648215162, -48.32844715993478246, 180.4678068554150059 ) ) ;
#55211=DIRECTION ( 'NONE',  ( 0.9068632946707805287, -0.4214249218767880389, 9.068632946707802473E-16 ) ) ;
#55215=CARTESIAN_POINT ( 'NONE',  ( 49.16670390244701139, -26.71338133339240528, 342.9256252759119548 ) ) ;
#55216=CIRCLE ( 'NONE', #18995, 3.250000000000002665 ) ;
#55217=CARTESIAN_POINT ( 'NONE',  ( 111.0096634661633885, -46.42778601040829045, 282.8841967044824628 ) ) ;
#55220=CARTESIAN_POINT ( 'NONE',  ( 107.3345184958865275, -26.28557234761613159, 120.0556252759109555 ) ) ;
#55221=CARTESIAN_POINT ( 'NONE',  ( 96.92707254288593788, -39.15325348941441064, 52.51276813305394597 ) ) ;
#55222=CARTESIAN_POINT ( 'NONE',  ( 105.3089409210114269, -48.49860570903479129, 143.4584824187689662 ) ) ;
#55223=CARTESIAN_POINT ( 'NONE',  ( 107.0664832912739968, -36.72944715994100306, 9.635625275910941312 ) ) ;
#55224=LINE ( 'NONE', #19390, #41655 ) ;
#55225=LINE ( 'NONE', #12128, #79711 ) ;
#55227=CARTESIAN_POINT ( 'NONE',  ( 113.2454987145582663, -28.75867295845091576, 189.5522919408784333 ) ) ;
#55228=CARTESIAN_POINT ( 'NONE',  ( 131.0667039024480118, -67.87844715994100397, 201.9838068554149970 ) ) ;
#55229=VERTEX_POINT ( 'NONE', #58606 ) ;
#55230=VECTOR ( 'NONE', #38149, 1000.000000000000000 ) ;
#55232=EDGE_LOOP ( 'NONE', ( #51131, #7542 ) ) ;
#55235=ORIENTED_EDGE ( 'NONE', *, *, #11947, .T. ) ;
#55236=CARTESIAN_POINT ( 'NONE',  ( 164.7830935719583181, -29.99615139351723769, 313.9678068554149490 ) ) ;
#55237=CARTESIAN_POINT ( 'NONE',  ( 98.32466564902617279, -28.76522518762223157, 76.73848241876795839 ) ) ;
#55238=LINE ( 'NONE', #82993, #61473 ) ;
#55239=EDGE_CURVE ( 'NONE', #50389, #10149, #80387, .T. ) ;
#55240=AXIS2_PLACEMENT_3D ( 'NONE', #39910, #88536, #19479 ) ;
#55243=CARTESIAN_POINT ( 'NONE',  ( 117.4569897637122011, -35.45259360763351708, 189.9241967044829664 ) ) ;
#55245=EDGE_CURVE ( 'NONE', #2317, #62004, #89364, .T. ) ;
#55246=CARTESIAN_POINT ( 'NONE',  ( 113.8315610999352714, -43.69395359880221719, 267.6124198280766677 ) ) ;
#55247=VERTEX_POINT ( 'NONE', #74831 ) ;
#55250=CARTESIAN_POINT ( 'NONE',  ( 76.06670390244805446, -58.72944715994109544, 239.5838068554169809 ) ) ;
#55251=FACE_OUTER_BOUND ( 'NONE', #46718, .T. ) ;
#55252=DIRECTION ( 'NONE',  ( 0.000000000000000000, 0.000000000000000000, -1.000000000000000000 ) ) ;
#55254=DIRECTION ( 'NONE',  ( 0.000000000000000000, 0.000000000000000000, -1.000000000000000000 ) ) ;
#55255=CIRCLE ( 'NONE', #40742, 5.599999999999994316 ) ;
#55257=AXIS2_PLACEMENT_3D ( 'NONE', #51774, #72252, #3648 ) ;
#55259=CARTESIAN_POINT ( 'NONE',  ( 105.8561066403587176, -27.02385992090109568, 270.1756252759109884 ) ) ;
#55261=ORIENTED_EDGE ( 'NONE', *, *, #76862, .F. ) ;
#55262=DIRECTION ( 'NONE',  ( -0.7071067811874389708, 0.7071067811856560636, 0.000000000000000000 ) ) ;
#55263=AXIS2_PLACEMENT_3D ( 'NONE', #71961, #65578, #38755 ) ;
#55264=FACE_OUTER_BOUND ( 'NONE', #38573, .T. ) ;
#55265=CARTESIAN_POINT ( 'NONE',  ( 100.0434009169665757, -32.56939427797095021, 83.71951894101997027 ) ) ;
#55271=CARTESIAN_POINT ( 'NONE',  ( 77.31651901074903321, -36.55810522839829702, 6.749822759741121558 ) ) ;
#55273=CARTESIAN_POINT ( 'NONE',  ( 108.0069521509713297, -26.34547698190780451, 155.0041967044819557 ) ) ;
#55276=CARTESIAN_POINT ( 'NONE',  ( 149.4430470701762488, -12.91565541735124256, 361.9756252759100335 ) ) ;
#55277=CARTESIAN_POINT ( 'NONE',  ( 112.3917779585437131, -43.81249117439911345, 139.5215833058969679 ) ) ;
#55279=CARTESIAN_POINT ( 'NONE',  ( 83.06670390244796920, -61.87844715994100397, 225.9838068554150254 ) ) ;
#55280=CARTESIAN_POINT ( 'NONE',  ( 116.2507439086588761, -31.75083131158774918, 65.22133956162595325 ) ) ;
#55281=CARTESIAN_POINT ( 'NONE',  ( 116.8171228670677806, -34.15291832195875799, 85.03145860913214449 ) ) ;
#55282=EDGE_LOOP ( 'NONE', ( #6432, #61754, #2779, #33877, #57773 ) ) ;
#55286=EDGE_CURVE ( 'NONE', #75364, #31678, #27125, .T. ) ;
#55287=EDGE_CURVE ( 'NONE', #1937, #44152, #38277, .T. ) ;
#55288=VECTOR ( 'NONE', #49062, 1000.000000000000000 ) ;
#55289=ADVANCED_FACE ( 'NONE', ( #69365 ), #89058, .T. ) ;
#55292=CARTESIAN_POINT ( 'NONE',  ( 115.5786047259628759, -31.87203575477177964, 289.2384824187686263 ) ) ;
#55293=CARTESIAN_POINT ( 'NONE',  ( 97.81677459100555438, -31.87350772351088679, 131.9413395616259947 ) ) ;
#55295=CARTESIAN_POINT ( 'NONE',  ( 108.3316104892186189, -46.73506784959683102, 128.6771457822665354 ) ) ;
#55296=CARTESIAN_POINT ( 'NONE',  ( 117.8564148307409596, -39.12764603782969886, 99.64038718067195077 ) ) ;
#55297=AXIS2_PLACEMENT_3D ( 'NONE', #86088, #86536, #17041 ) ;
#55298=LINE ( 'NONE', #88520, #66858 ) ;
#55300=CARTESIAN_POINT ( 'NONE',  ( 100.9543326502937504, -28.70727443998947592, 115.5961036648878775 ) ) ;
#55302=CARTESIAN_POINT ( 'NONE',  ( 172.5664832912740110, -32.07844715994070839, 23.67562527591200094 ) ) ;
#55304=EDGE_CURVE ( 'NONE', #55351, #9306, #55689, .T. ) ;
#55305=CARTESIAN_POINT ( 'NONE',  ( 41.56648329127399677, -18.82844715994099971, 258.9256252759120116 ) ) ;
#55306=LINE ( 'NONE', #48050, #41164 ) ;
#55307=CARTESIAN_POINT ( 'NONE',  ( 105.4209491665783105, -47.02406944081578644, 37.44991099019695469 ) ) ;
#55308=DIRECTION ( 'NONE',  ( -6.524622321627019585E-16, -4.013151879589939944E-16, -1.000000000000000000 ) ) ;
#55310=CARTESIAN_POINT ( 'NONE',  ( 140.9629299006806491, -8.979447159940995959, 14.92562527591100618 ) ) ;
#55311=CARTESIAN_POINT ( 'NONE',  ( 117.0713329378632039, -35.45783045783232978, 93.92760797587766319 ) ) ;
#55312=CARTESIAN_POINT ( 'NONE',  ( 98.99648076951073961, -33.93126856627920773, 285.4838483995053480 ) ) ;
#55314=CARTESIAN_POINT ( 'NONE',  ( 107.9437834512411314, -25.73425880284256095, 111.0251490854349754 ) ) ;
#55315=CARTESIAN_POINT ( 'NONE',  ( 62.03715912545824551, -47.82818131006021645, 300.4678068554150627 ) ) ;
#55316=CARTESIAN_POINT ( 'NONE',  ( 96.62682903746573970, -35.94284815129010013, 146.2670538473399517 ) ) ;
#55317=DIRECTION ( 'NONE',  ( 4.299999999999999979E-14, -1.000000000000000000, 4.400000000000000367E-29 ) ) ;
#55318=VERTEX_POINT ( 'NONE', #34832 ) ;
#55320=AXIS2_PLACEMENT_3D ( 'NONE', #6870, #21864, #70001 ) ;
#55321=FACE_BOUND ( 'NONE', #11602, .T. ) ;
#55324=EDGE_CURVE ( 'NONE', #77063, #48698, #6380, .T. ) ;
#55326=CARTESIAN_POINT ( 'NONE',  ( 100.8602861511969024, -45.93004170815812159, 152.0918157521009562 ) ) ;
#55327=EDGE_LOOP ( 'NONE', ( #54763, #15225, #8211 ) ) ;
#55329=CARTESIAN_POINT ( 'NONE',  ( 110.5060411634814557, -26.86503128786541694, 205.8099109901969541 ) ) ;
#55331=VECTOR ( 'NONE', #10888, 1000.000000000000000 ) ;
#55336=AXIS2_PLACEMENT_3D ( 'NONE', #78020, #81155, #52050 ) ;
#55337=ORIENTED_EDGE ( 'NONE', *, *, #88777, .T. ) ;
#55340=DIRECTION ( 'NONE',  ( 0.000000000000000000, -1.000000000000000000, 0.000000000000000000 ) ) ;
#55341=CARTESIAN_POINT ( 'NONE',  ( 117.4137378716304738, -35.45790868367866722, 189.9241967044829664 ) ) ;
#55342=CARTESIAN_POINT ( 'NONE',  ( 151.5667039024483813, -48.82844715993591223, 249.9678068554149490 ) ) ;
#55344=VECTOR ( 'NONE', #11943, 1000.000000000000000 ) ;
#55347=CARTESIAN_POINT ( 'NONE',  ( 94.86917197795301604, -31.06128196069623471, 6.826283056785777958 ) ) ;
#55348=EDGE_CURVE ( 'NONE', #68797, #2099, #37037, .T. ) ;
#55350=ORIENTED_EDGE ( 'NONE', *, *, #77303, .T. ) ;
#55351=VERTEX_POINT ( 'NONE', #69813 ) ;
#55352=AXIS2_PLACEMENT_3D ( 'NONE', #44611, #52296, #86868 ) ;
#55354=CARTESIAN_POINT ( 'NONE',  ( 162.5667039024460223, -22.48495420874110806, -5.074374724088000832 ) ) ;
#55355=CARTESIAN_POINT ( 'NONE',  ( 107.4826147187165333, -46.50135945624614209, 233.6099109901959707 ) ) ;
#55356=CARTESIAN_POINT ( 'NONE',  ( 134.0664832912739826, -9.029447159941003775, 4.925625275910997303 ) ) ;
#55357=CARTESIAN_POINT ( 'NONE',  ( 116.8058161338297509, -37.62879752186919546, 74.75276813305298163 ) ) ;
#55362=EDGE_CURVE ( 'NONE', #49327, #44506, #33818, .T. ) ;
#55365=EDGE_LOOP ( 'NONE', ( #53339, #6946, #10566, #6255 ) ) ;
#55367=CARTESIAN_POINT ( 'NONE',  ( 98.11614316284976667, -39.58741349592436620, 277.9920594963732015 ) ) ;
#55370=CARTESIAN_POINT ( 'NONE',  ( 104.4896222497930864, -26.97889890500220034, 140.2814858277504015 ) ) ;
#55373=ORIENTED_EDGE ( 'NONE', *, *, #52021, .T. ) ;
#55375=CARTESIAN_POINT ( 'NONE',  ( 116.3268456006857718, -32.93825467094161752, 164.1356252759109680 ) ) ;
#55377=CARTESIAN_POINT ( 'NONE',  ( 118.0757533234433083, -37.71689883586016379, 33.74324432352998571 ) ) ;
#55379=CARTESIAN_POINT ( 'NONE',  ( 101.5523784292199991, -30.67338203694697185, 283.4823760838770568 ) ) ;
#55380=CARTESIAN_POINT ( 'NONE',  ( 117.0716382134925340, -35.46038279169101060, 128.9272686535105379 ) ) ;
#55381=CARTESIAN_POINT ( 'NONE',  ( 113.7357275853186991, -44.67049210939298831, 148.1203871806729353 ) ) ;
#55383=LINE ( 'NONE', #83139, #32795 ) ;
#55384=CARTESIAN_POINT ( 'NONE',  ( 164.9190312289449878, -35.91149509761320502, 342.9256252759109884 ) ) ;
#55387=CARTESIAN_POINT ( 'NONE',  ( 97.52025866034094292, -43.83442485161933178, 257.8356252759109566 ) ) ;
#55392=ORIENTED_EDGE ( 'NONE', *, *, #64625, .T. ) ;
#55393=CARTESIAN_POINT ( 'NONE',  ( 98.16534761909046836, -43.36023007783336425, 107.8480062282919647 ) ) ;
#55394=CARTESIAN_POINT ( 'NONE',  ( 48.16670390244701139, -28.27351298637280408, -5.074374724088000832 ) ) ;
#55395=ORIENTED_EDGE ( 'NONE', *, *, #51693, .T. ) ;
#55396=VERTEX_POINT ( 'NONE', #86130 ) ;
#55397=ADVANCED_FACE ( 'NONE', ( #2116 ), #79322, .T. ) ;
#55398=ADVANCED_FACE ( 'NONE', ( #10262 ), #64344, .T. ) ;
#55401=DIRECTION ( 'NONE',  ( 4.299999999999999979E-14, -1.000000000000000000, 0.000000000000000000 ) ) ;
#55402=CARTESIAN_POINT ( 'NONE',  ( 165.2725846195390602, -35.55794170701241086, 117.4678068554150485 ) ) ;
#55404=CARTESIAN_POINT ( 'NONE',  ( 25.56670390244797275, -62.87844715994099687, 173.2178068554149775 ) ) ;
#55405=CARTESIAN_POINT ( 'NONE',  ( 101.5399107887468944, -29.27606352979315574, 183.4023760838769590 ) ) ;
#55406=CARTESIAN_POINT ( 'NONE',  ( 115.9784307414374780, -30.15203137637957909, 255.3203871806729524 ) ) ;
#55412=DIRECTION ( 'NONE',  ( 0.000000000000000000, 1.000000000000000000, 0.000000000000000000 ) ) ;
#55413=EDGE_LOOP ( 'NONE', ( #20208, #68271, #76662, #48203 ) ) ;
#55414=VECTOR ( 'NONE', #88903, 1000.000000000000000 ) ;
#55415=ORIENTED_EDGE ( 'NONE', *, *, #76983, .T. ) ;
#55417=CIRCLE ( 'NONE', #27882, 29.00000000000000000 ) ;
#55418=DIRECTION ( 'NONE',  ( -1.000000000000000000, -3.360405532702990443E-14, 0.000000000000000000 ) ) ;
#55419=FACE_OUTER_BOUND ( 'NONE', #59008, .T. ) ;
#55420=CARTESIAN_POINT ( 'NONE',  ( 97.60787735695338085, -39.98239029230723673, 16.59006164541757755 ) ) ;
#55422=DIRECTION ( 'NONE',  ( 0.000000000000000000, 0.000000000000000000, 1.000000000000000000 ) ) ;
#55424=CARTESIAN_POINT ( 'NONE',  ( 104.9258105463076873, -28.46061097091046577, 199.7009912566479386 ) ) ;
#55426=CARTESIAN_POINT ( 'NONE',  ( 100.9172270114722494, -28.25635367234391992, 75.57562527591093726 ) ) ;
#55427=CARTESIAN_POINT ( 'NONE',  ( 182.2300522401149863, -33.89581943344511217, 342.9256252759109884 ) ) ;
#55429=FACE_OUTER_BOUND ( 'NONE', #54975, .T. ) ;
#55430=VECTOR ( 'NONE', #62276, 1000.000000000000000 ) ;
#55434=DIRECTION ( 'NONE',  ( -0.9834602067153815907, -0.1811243269341220596, 0.000000000000000000 ) ) ;
#55435=CARTESIAN_POINT ( 'NONE',  ( 37.56670390244814683, -48.82844715994099971, 249.9678068554150343 ) ) ;
#55436=CARTESIAN_POINT ( 'NONE',  ( 116.8161993950274535, -34.14934549342144976, 275.0312959239825545 ) ) ;
#55439=CARTESIAN_POINT ( 'NONE',  ( 117.2885226371813872, -38.88728764921428649, 63.66133956162494911 ) ) ;
#55440=CARTESIAN_POINT ( 'NONE',  ( 97.81186544543886896, -40.51730612966257183, 271.6361395295153898 ) ) ;
#55441=LINE ( 'NONE', #27311, #80567 ) ;
#55442=LINE ( 'NONE', #76366, #37967 ) ;
#55443=DIRECTION ( 'NONE',  ( 3.999999999999999995E-14, -1.000000000000000000, 4.100000000000000342E-29 ) ) ;
#55445=AXIS2_PLACEMENT_3D ( 'NONE', #84447, #49433, #14947 ) ;
#55446=DIRECTION ( 'NONE',  ( 2.900000000000000265E-14, -2.000000000000000155E-15, 1.000000000000000000 ) ) ;
#55449=ORIENTED_EDGE ( 'NONE', *, *, #50391, .T. ) ;
#55450=CARTESIAN_POINT ( 'NONE',  ( 106.6594888599963298, -26.29050016388675104, 81.10705384733896040 ) ) ;
#55451=DIRECTION ( 'NONE',  ( 0.000000000000000000, 0.000000000000000000, 1.000000000000000000 ) ) ;
#55453=ADVANCED_FACE ( 'NONE', ( #57512 ), #65229, .F. ) ;
#55454=DIRECTION ( 'NONE',  ( 1.000000000000000000, 0.000000000000000000, 0.000000000000000000 ) ) ;
#55455=AXIS2_PLACEMENT_3D ( 'NONE', #26587, #77320, #82028 ) ;
#55457=EDGE_LOOP ( 'NONE', ( #85272, #76972 ) ) ;
#55458=CARTESIAN_POINT ( 'NONE',  ( 113.7965574739370140, -44.62378898692899298, 149.1508633711479774 ) ) ;
#55459=LINE ( 'NONE', #14160, #2255 ) ;
#55461=CARTESIAN_POINT ( 'NONE',  ( 115.3062145713271747, -45.21207857638179917, 264.1899109901965517 ) ) ;
#55463=CARTESIAN_POINT ( 'NONE',  ( 107.0664832912739541, -20.87944715994095546, 302.6356252759109680 ) ) ;
#55464=LINE ( 'NONE', #69576, #13893 ) ;
#55469=CARTESIAN_POINT ( 'NONE',  ( 110.4719531740380347, -47.31314961125950447, 207.8241967044829721 ) ) ;
#55470=ORIENTED_EDGE ( 'NONE', *, *, #49200, .T. ) ;
#55471=ORIENTED_EDGE ( 'NONE', *, *, #48683, .F. ) ;
#55472=CARTESIAN_POINT ( 'NONE',  ( 112.5904859203986206, -43.69705252635404236, 164.5415833058969781 ) ) ;
#55473=VECTOR ( 'NONE', #25158, 1000.000000000000000 ) ;
#55474=EDGE_CURVE ( 'NONE', #38746, #76506, #52009, .T. ) ;
#55476=CARTESIAN_POINT ( 'NONE',  ( 98.21984324360056462, -33.56503799257626497, 22.49682140113501561 ) ) ;
#55479=CARTESIAN_POINT ( 'NONE',  ( 101.9933586085964805, -45.44590959077525127, 267.1565423270654378 ) ) ;
#55480=DIRECTION ( 'NONE',  ( 0.000000000000000000, 1.000000000000000000, 0.000000000000000000 ) ) ;
#55481=CARTESIAN_POINT ( 'NONE',  ( 97.81169789812091153, -40.51742632959496859, 107.6355761348045519 ) ) ;
#55482=CARTESIAN_POINT ( 'NONE',  ( 86.98314995794061133, 12.92155284005802507, 336.5756252759109657 ) ) ;
#55483=CARTESIAN_POINT ( 'NONE',  ( 100.7633749303630850, -45.78122309449486949, 237.0803871806729717 ) ) ;
#55484=FACE_BOUND ( 'NONE', #55728, .T. ) ;
#55485=ORIENTED_EDGE ( 'NONE', *, *, #60344, .T. ) ;
#55486=ORIENTED_EDGE ( 'NONE', *, *, #49600, .F. ) ;
#55489=CARTESIAN_POINT ( 'NONE',  ( 176.5667039024483245, -48.82844715993483220, 300.4678068554149490 ) ) ;
#55493=CARTESIAN_POINT ( 'NONE',  ( 105.3131098409624542, -26.40875552125079295, 11.20991099019697046 ) ) ;
#55494=CARTESIAN_POINT ( 'NONE',  ( 97.22365000156210613, -40.27127430222545001, 266.6013395616254797 ) ) ;
#55495=EDGE_CURVE ( 'NONE', #81124, #70274, #46947, .T. ) ;
#55497=AXIS2_PLACEMENT_3D ( 'NONE', #16511, #24219, #70585 ) ;
#55499=CARTESIAN_POINT ( 'NONE',  ( 77.43081253121034990, -37.51428458727112769, 6.911392308671570284 ) ) ;
#55500=LINE ( 'NONE', #14659, #36984 ) ;
#55501=EDGE_CURVE ( 'NONE', #61365, #23550, #17526, .T. ) ;
#55502=CARTESIAN_POINT ( 'NONE',  ( 116.3170820643562564, -32.94538914428453324, 169.1356252759109680 ) ) ;
#55503=CARTESIAN_POINT ( 'NONE',  ( 114.2426363300227763, -32.83938885940727204, 67.03951894101994924 ) ) ;
#55504=CARTESIAN_POINT ( 'NONE',  ( 117.4790109288255309, -40.50628101140208770, 169.5375300378159693 ) ) ;
#55505=CARTESIAN_POINT ( 'NONE',  ( 118.5256205435843526, -36.72944715994100306, 293.2242906452868851 ) ) ;
#55506=VERTEX_POINT ( 'NONE', #36642 ) ;
#55507=EDGE_CURVE ( 'NONE', #89573, #73333, #10716, .T. ) ;
#55508=LINE ( 'NONE', #7393, #32050 ) ;
#55509=VERTEX_POINT ( 'NONE', #28289 ) ;
#55510=ORIENTED_EDGE ( 'NONE', *, *, #54020, .F. ) ;
#55513=ORIENTED_EDGE ( 'NONE', *, *, #63979, .T. ) ;
#55517=CARTESIAN_POINT ( 'NONE',  ( 110.3568814055478242, -27.59468345507334064, 99.22384839950498758 ) ) ;
#55518=CARTESIAN_POINT ( 'NONE',  ( 116.0742729640735007, -42.02152512393894312, 238.4041967044829562 ) ) ;
#55519=CARTESIAN_POINT ( 'NONE',  ( 102.2473430764596714, -45.94923854148477460, 212.1927681330539599 ) ) ;
#55520=CARTESIAN_POINT ( 'NONE',  ( 96.94826409162261882, -39.14818769109201213, 52.51276813305394597 ) ) ;
#55521=CARTESIAN_POINT ( 'NONE',  ( 162.7131505118683208, -31.94127993907824958, 342.9256252759109884 ) ) ;
#55522=CARTESIAN_POINT ( 'NONE',  ( 104.4066637080126867, -46.45766777219723309, 93.36467352085369953 ) ) ;
#55524=DIRECTION ( 'NONE',  ( 0.000000000000000000, 0.000000000000000000, -1.000000000000000000 ) ) ;
#55525=CARTESIAN_POINT ( 'NONE',  ( 31.90335556477799628, -33.89581943344391135, -5.074374724088000832 ) ) ;
#55526=CARTESIAN_POINT ( 'NONE',  ( 98.49710108934563380, -31.94619897774420636, 110.9213395616259703 ) ) ;
#55527=CIRCLE ( 'NONE', #23688, 2.500000000000002220 ) ;
#55528=CARTESIAN_POINT ( 'NONE',  ( 96.03104818302425372, -37.92613241492836806, 81.40038718067299328 ) ) ;
#55529=CARTESIAN_POINT ( 'NONE',  ( 111.6277637875740538, -46.15289590646231943, 247.9356252759109509 ) ) ;
#55531=CARTESIAN_POINT ( 'NONE',  ( 96.13794759894150843, -35.07228238994858316, 221.1946728949589840 ) ) ;
#55533=AXIS2_PLACEMENT_3D ( 'NONE', #67273, #32756, #86841 ) ;
#55534=CARTESIAN_POINT ( 'NONE',  ( 104.4074300115074294, -46.45789994007284918, 23.36473591763067503 ) ) ;
#55538=CARTESIAN_POINT ( 'NONE',  ( 106.1642028280447363, -25.30548797942247674, 320.5922460209141605 ) ) ;
#55542=FACE_OUTER_BOUND ( 'NONE', #72410, .T. ) ;
#55543=CARTESIAN_POINT ( 'NONE',  ( 168.3664380525667639, -48.62818131005518296, 300.4678068554149490 ) ) ;
#55545=CARTESIAN_POINT ( 'NONE',  ( 115.8254323912423303, -31.73001882710328658, 259.2397919427208990 ) ) ;
#55546=EDGE_LOOP ( 'NONE', ( #49880, #51975, #56695, #15355 ) ) ;
#55548=CARTESIAN_POINT ( 'NONE',  ( 99.31672145811513985, -28.81511631862888123, 270.7051490854347549 ) ) ;
#55549=CARTESIAN_POINT ( 'NONE',  ( 102.9134293080737450, -27.12924067693381502, 151.4013395616249511 ) ) ;
#55550=CARTESIAN_POINT ( 'NONE',  ( 115.3579863298411254, -45.26537652146382840, 264.1899109901965517 ) ) ;
#55551=DIRECTION ( 'NONE',  ( -9.073094938289460781E-13, -1.000000000000000000, 0.000000000000000000 ) ) ;
#55553=CARTESIAN_POINT ( 'NONE',  ( 82.51738923908165191, -35.48112160757226263, 7.135585143033805977 ) ) ;
#55554=ADVANCED_FACE ( 'NONE', ( #16031 ), #85081, .F. ) ;
#55556=DIRECTION ( 'NONE',  ( 0.000000000000000000, 0.000000000000000000, 1.000000000000000000 ) ) ;
#55557=AXIS2_PLACEMENT_3D ( 'NONE', #26097, #38820, #31556 ) ;
#55558=EDGE_CURVE ( 'NONE', #10820, #32414, #50529, .T. ) ;
#55559=VERTEX_POINT ( 'NONE', #70085 ) ;
#55562=CARTESIAN_POINT ( 'NONE',  ( 98.03781028509631312, -36.02536330594374192, 190.6990864947429998 ) ) ;
#55563=CARTESIAN_POINT ( 'NONE',  ( 113.1746683643167728, -44.75457706286819359, 188.0941723682731208 ) ) ;
#55565=CIRCLE ( 'NONE', #491, 0.2999999999999943823 ) ;
#55566=DIRECTION ( 'NONE',  ( -0.7071067812152160847, 0.7071067811578790607, 0.000000000000000000 ) ) ;
#55567=CARTESIAN_POINT ( 'NONE',  ( 101.9826776100855881, -46.51815199768660847, 163.1832443235299763 ) ) ;
#55569=CARTESIAN_POINT ( 'NONE',  ( 116.3221839001005264, -32.94216875276463696, 149.1356252759109680 ) ) ;
#55570=CARTESIAN_POINT ( 'NONE',  ( 109.3845169419079042, -26.99633185450459649, 85.89096953987156269 ) ) ;
#55571=DIRECTION ( 'NONE',  ( -1.094868876412250136E-15, -2.588449845256440170E-31, -1.000000000000000000 ) ) ;
#55573=CARTESIAN_POINT ( 'NONE',  ( 99.34849973496650932, -28.72665311504486141, 115.6870538473399534 ) ) ;
#55574=ORIENTED_EDGE ( 'NONE', *, *, #87943, .F. ) ;
#55578=B_SPLINE_CURVE_WITH_KNOTS ( 'NONE', 3,
 ( #101, #27799, #57284, #85028, #55479, #22799, #83231, #20994, #7363, #76403, #14180, #83677, #56389, #21450, #49118, #76851, #14635, #65888 ),
 .UNSPECIFIED., .F., .F.,
 ( 4, 2, 2, 2, 2, 2, 2, 2, 4 ),
 ( 0.4999967102254601614, 0.5624971214472775927, 0.6249975326690950794, 0.6874979438909125662, 0.7499983551127300530, 0.8124987663345475397, 0.8749991775563650265, 0.9374995887781825132, 1.000000000000000000 ),
 .UNSPECIFIED. ) ;
#55579=CARTESIAN_POINT ( 'NONE',  ( 115.5559677222042154, -32.70388140663459353, 60.62253568684894134 ) ) ;
#55580=EDGE_CURVE ( 'NONE', #30145, #86172, #29211, .T. ) ;
#55581=DIRECTION ( 'NONE',  ( 0.7071067811865516806, -0.7071067811865434649, 7.071067811865510832E-16 ) ) ;
#55582=CARTESIAN_POINT ( 'NONE',  ( 107.8656169629272341, -46.51081515578102454, 173.6413395616249886 ) ) ;
#55584=CARTESIAN_POINT ( 'NONE',  ( 138.8167039024479834, -57.40094715994099772, 84.20080685541500998 ) ) ;
#55589=CARTESIAN_POINT ( 'NONE',  ( 109.0680860650138442, -47.57644715601883689, 127.7337205140059382 ) ) ;
#55590=EDGE_LOOP ( 'NONE', ( #26779, #69683 ) ) ;
#55591=EDGE_LOOP ( 'NONE', ( #52057, #85880 ) ) ;
#55592=VERTEX_POINT ( 'NONE', #22850 ) ;
#55595=DIRECTION ( 'NONE',  ( 4.299999999999999979E-14, -1.000000000000000000, 4.400000000000000367E-29 ) ) ;
#55597=CARTESIAN_POINT ( 'NONE',  ( 114.8576755932693487, -34.29489411463138282, 171.8852332267339591 ) ) ;
#55598=VECTOR ( 'NONE', #22087, 1000.000000000000114 ) ;
#55600=DIRECTION ( 'NONE',  ( 1.000000000000000000, 3.999999999999999995E-14, 1.000000000000000078E-15 ) ) ;
#55602=CARTESIAN_POINT ( 'NONE',  ( 116.3274949261486881, -32.94048995676258329, 25.13562527591095375 ) ) ;
#55603=EDGE_LOOP ( 'NONE', ( #39838, #37946, #42889, #66642 ) ) ;
#55604=VERTEX_POINT ( 'NONE', #55525 ) ;
#55605=VERTEX_POINT ( 'NONE', #48718 ) ;
#55606=CARTESIAN_POINT ( 'NONE',  ( 136.1031425115596392, -20.57949487819923462, 2.327894807228624074 ) ) ;
#55608=VERTEX_POINT ( 'NONE', #76451 ) ;
#55609=CARTESIAN_POINT ( 'NONE',  ( 77.86687873446965114, -20.38871026388561347, 7.389079501618835089 ) ) ;
#55611=CARTESIAN_POINT ( 'NONE',  ( 102.4628740603001233, -44.30143901548009211, 243.5730118773259676 ) ) ;
#55616=EDGE_LOOP ( 'NONE', ( #4016, #63587, #24491, #68165 ) ) ;
#55617=CIRCLE ( 'NONE', #71622, 2.116999999999980009 ) ;
#55618=CARTESIAN_POINT ( 'NONE',  ( 193.5667039024416738, -48.82844715994099971, 129.9678068554150343 ) ) ;
#55620=ORIENTED_EDGE ( 'NONE', *, *, #53043, .F. ) ;
#55621=ORIENTED_EDGE ( 'NONE', *, *, #41987, .T. ) ;
#55623=CARTESIAN_POINT ( 'NONE',  ( 101.5523784292199991, -30.67338203694697185, 283.4823760838770568 ) ) ;
#55624=AXIS2_PLACEMENT_3D ( 'NONE', #70999, #77349, #35103 ) ;
#55625=CARTESIAN_POINT ( 'NONE',  ( 102.0711994968067984, -27.55373892369285826, 145.4727681330539610 ) ) ;
#55626=CARTESIAN_POINT ( 'NONE',  ( 98.35456548258453324, -42.41549619454043096, 101.7870538473399620 ) ) ;
#55629=CARTESIAN_POINT ( 'NONE',  ( 132.9844404253383630, -16.20116865955289143, 8.043260881866483913 ) ) ;
#55630=CARTESIAN_POINT ( 'NONE',  ( 116.8848192732620390, -41.80628269293674748, 239.4346728949589647 ) ) ;
#55631=DIRECTION ( 'NONE',  ( 1.000000000000000000, 3.999999999999999995E-14, 1.000000000000000078E-15 ) ) ;
#55637=CYLINDRICAL_SURFACE ( 'NONE', #59080, 2.030000000001872529 ) ;
#55639=CARTESIAN_POINT ( 'NONE',  ( 103.9236440166535687, -27.23036313016521248, 136.3307465375340541 ) ) ;
#55640=CARTESIAN_POINT ( 'NONE',  ( 116.9043533071046568, -40.17956947857189220, 133.5584824187679658 ) ) ;
#55642=DIRECTION ( 'NONE',  ( -4.237773401492740281E-14, 1.000000000000000000, 0.000000000000000000 ) ) ;
#55643=PLANE ( 'NONE',  #12277 ) ;
#55645=CARTESIAN_POINT ( 'NONE',  ( 114.0300661836957090, -43.96678976627357827, 58.18600423541299449 ) ) ;
#55646=CARTESIAN_POINT ( 'NONE',  ( 110.0457755916377494, -26.10929462018219382, 215.8708633711489711 ) ) ;
#55647=LINE ( 'NONE', #48842, #58240 ) ;
#55649=ORIENTED_EDGE ( 'NONE', *, *, #46269, .T. ) ;
#55650=DIRECTION ( 'NONE',  ( 0.000000000000000000, 0.000000000000000000, -1.000000000000000000 ) ) ;
#55651=LINE ( 'NONE', #67975, #51464 ) ;
#55652=DIRECTION ( 'NONE',  ( 0.000000000000000000, 0.000000000000000000, -1.000000000000000000 ) ) ;
#55654=CARTESIAN_POINT ( 'NONE',  ( 117.4736937924436688, -35.59074751853778196, 278.9127681330539872 ) ) ;
#55655=VERTEX_POINT ( 'NONE', #47502 ) ;
#55656=DIRECTION ( 'NONE',  ( 1.000000000000000000, 0.000000000000000000, -2.089354330573420398E-14 ) ) ;
#55657=CARTESIAN_POINT ( 'NONE',  ( 98.83914123113804351, -30.29059417415423638, 155.7984824187679465 ) ) ;
#55658=CARTESIAN_POINT ( 'NONE',  ( 105.4209835578153189, -47.02385428587647453, 33.44991099019695469 ) ) ;
#55659=CARTESIAN_POINT ( 'NONE',  ( 107.9218213793745633, -47.19875523359718983, 173.6413395616249886 ) ) ;
#55663=FACE_OUTER_BOUND ( 'NONE', #28922, .T. ) ;
#55666=ORIENTED_EDGE ( 'NONE', *, *, #85297, .T. ) ;
#55667=AXIS2_PLACEMENT_3D ( 'NONE', #85545, #10114, #37823 ) ;
#55669=AXIS2_PLACEMENT_3D ( 'NONE', #31413, #40024, #60921 ) ;
#55670=EDGE_CURVE ( 'NONE', #61557, #59994, #83233, .T. ) ;
#55674=CARTESIAN_POINT ( 'NONE',  ( 106.9276426037745011, -26.29176787048590214, 56.08705384733997334 ) ) ;
#55675=DIRECTION ( 'NONE',  ( 1.000000000000000000, 3.999999999999999995E-14, 1.000000000000000078E-15 ) ) ;
#55677=CARTESIAN_POINT ( 'NONE',  ( 98.13109353019112291, -31.27492705589930821, 166.8899109901969950 ) ) ;
#55678=CARTESIAN_POINT ( 'NONE',  ( 105.3911398957759076, -27.82967838469355115, 279.6590864947435762 ) ) ;
#55679=ORIENTED_EDGE ( 'NONE', *, *, #20314, .F. ) ;
#55680=ORIENTED_EDGE ( 'NONE', *, *, #14229, .T. ) ;
#55681=ORIENTED_EDGE ( 'NONE', *, *, #47886, .F. ) ;
#55682=AXIS2_PLACEMENT_3D ( 'NONE', #61430, #26476, #82358 ) ;
#55684=CARTESIAN_POINT ( 'NONE',  ( 87.06670390244778446, -15.72944715994119669, 239.5838068554169809 ) ) ;
#55686=FACE_OUTER_BOUND ( 'NONE', #85084, .T. ) ;
#55687=CARTESIAN_POINT ( 'NONE',  ( 80.06648329127402519, -46.42944715994105565, -0.5743747240890559880 ) ) ;
#55689=LINE ( 'NONE', #8487, #65835 ) ;
#55691=DIRECTION ( 'NONE',  ( -0.7071067811865175967, -0.7071067811865774377, -7.071067811865480264E-16 ) ) ;
#55694=VECTOR ( 'NONE', #74783, 1000.000000000000000 ) ;
#55696=CARTESIAN_POINT ( 'NONE',  ( 115.5786047259628759, -31.87203575477177964, 289.2384824187686263 ) ) ;
#55700=ADVANCED_FACE ( 'NONE', ( #74340 ), #82960, .T. ) ;
#55701=DIRECTION ( 'NONE',  ( 0.000000000000000000, 0.000000000000000000, 1.000000000000000000 ) ) ;
#55703=CARTESIAN_POINT ( 'NONE',  ( 107.4866789999374390, -28.54983079893278486, 92.85380465530596439 ) ) ;
#55705=B_SPLINE_CURVE_WITH_KNOTS ( 'NONE', 3,
 ( #59120, #18696, #60007, #52285, #73200, #60464, #4178, #11440, #80049, #80488, #10981, #87299, #25063, #17361, #18247, #39139, #45044, #66844, #4626, #5532, #88207, #80948, #72775, #25967, #53632, #19154, #12335, #40028, #67747, #69095, #83184, #89092, #75467, #20508, #76353 ),
 .UNSPECIFIED., .F., .F.,
 ( 4, 2, 1, 1, 1, 1, 1, 2, 2, 2, 2, 2, 2, 2, 2, 2, 2, 2, 2, 4 ),
 ( 0.4999644244176295604, 0.5002085824135195091, 0.5004527404094094578, 0.5009410564011892442, 0.5019176883847487058, 0.5038709523518675182, 0.5077774802861049208, 0.5155905361545793930, 0.5312166478915285595, 0.5624688713654264482, 0.5937210948393243370, 0.6249733183132222258, 0.6562255417871201146, 0.6874777652610181145, 0.7187299887349160032, 0.7499822122088140031, 0.8124866591566104468, 0.8749911061044071126, 0.9374955530522035563, 1.000000000000000000 ),
 .UNSPECIFIED. ) ;
#55706=EDGE_CURVE ( 'NONE', #18234, #2491, #47049, .T. ) ;
#55708=CARTESIAN_POINT ( 'NONE',  ( 115.8254323918504696, -31.73001882859116662, 44.23979194259261760 ) ) ;
#55709=ORIENTED_EDGE ( 'NONE', *, *, #87127, .F. ) ;
#55711=CARTESIAN_POINT ( 'NONE',  ( 41.56648329127398966, -27.57844715994070484, 138.9256252759119832 ) ) ;
#55712=EDGE_LOOP ( 'NONE', ( #83029, #6626, #53122, #46464 ) ) ;
#55714=EDGE_CURVE ( 'NONE', #3629, #21597, #89321, .T. ) ;
#55715=CARTESIAN_POINT ( 'NONE',  ( 117.0608945246740973, -38.08045310990723920, 69.71895861011263662 ) ) ;
#55716=CARTESIAN_POINT ( 'NONE',  ( 108.4114243528872095, -27.43637152299345061, 146.4053928297069547 ) ) ;
#55718=CARTESIAN_POINT ( 'NONE',  ( 115.1837411929738977, -43.30572140991047547, 84.28419670448195689 ) ) ;
#55720=CARTESIAN_POINT ( 'NONE',  ( 53.56670390244743629, -48.82844715994058049, 180.4678068554151196 ) ) ;
#55723=VECTOR ( 'NONE', #52628, 1000.000000000000000 ) ;
#55724=ORIENTED_EDGE ( 'NONE', *, *, #64766, .F. ) ;
#55726=EDGE_CURVE ( 'NONE', #11190, #58495, #6200, .T. ) ;
#55727=DIRECTION ( 'NONE',  ( 1.000000000000000078E-15, 0.000000000000000000, -1.000000000000000000 ) ) ;
#55728=EDGE_LOOP ( 'NONE', ( #81636, #17683 ) ) ;
#55729=CARTESIAN_POINT ( 'NONE',  ( 95.96284676697203508, -37.29622633765243478, 271.3670538473399461 ) ) ;
#55730=CARTESIAN_POINT ( 'NONE',  ( 116.8158478801051530, -32.97616202413719577, 135.1184824187679396 ) ) ;
#55734=CARTESIAN_POINT ( 'NONE',  ( 109.2549746569086437, -46.95841770046993702, 103.7441967044829880 ) ) ;
#55737=ORIENTED_EDGE ( 'NONE', *, *, #54667, .F. ) ;
#55738=CARTESIAN_POINT ( 'NONE',  ( 97.06387421237998581, -37.34281635329717375, 116.3762687914366722 ) ) ;
#55741=ORIENTED_EDGE ( 'NONE', *, *, #63545, .F. ) ;
#55744=AXIS2_PLACEMENT_3D ( 'NONE', #49543, #1871, #75926 ) ;
#55746=DIRECTION ( 'NONE',  ( 9.351236661543306751E-17, -3.725950533538267725E-29, -1.000000000000000000 ) ) ;
#55747=CARTESIAN_POINT ( 'NONE',  ( 96.17734138947662359, -38.62830894954290528, 46.45181575210094138 ) ) ;
#55750=CARTESIAN_POINT ( 'NONE',  ( 112.0683309827296767, -45.48704644034171451, 92.99083554691495124 ) ) ;
#55751=CARTESIAN_POINT ( 'NONE',  ( 97.46604185887800043, -38.76544784714115366, 31.49276813305495892 ) ) ;
#55752=CARTESIAN_POINT ( 'NONE',  ( 112.1392154949572841, -28.01274250318494197, 109.6564706139660075 ) ) ;
#55753=CARTESIAN_POINT ( 'NONE',  ( 102.3122812202564802, -27.43633205498518635, 116.4527681330539650 ) ) ;
#55754=DIRECTION ( 'NONE',  ( -0.7071067811578587436, 0.7071067812152364018, 0.000000000000000000 ) ) ;
#55755=FACE_OUTER_BOUND ( 'NONE', #38288, .T. ) ;
#55756=ORIENTED_EDGE ( 'NONE', *, *, #5669, .T. ) ;
#55757=DIRECTION ( 'NONE',  ( 0.000000000000000000, 0.000000000000000000, 1.000000000000000000 ) ) ;
#55758=AXIS2_PLACEMENT_3D ( 'NONE', #70098, #27859, #41475 ) ;
#55761=LINE ( 'NONE', #5873, #84829 ) ;
#55764=CARTESIAN_POINT ( 'NONE',  ( 108.9531560784502915, -26.39541311287850434, 164.9327681330529742 ) ) ;
#55765=ORIENTED_EDGE ( 'NONE', *, *, #47200, .F. ) ;
#55766=CARTESIAN_POINT ( 'NONE',  ( 165.9667039024459996, -26.71338133339301635, -5.074374724088000832 ) ) ;
#55767=CARTESIAN_POINT ( 'NONE',  ( 98.01791376823749147, -44.42006743888428133, 222.8870538473399563 ) ) ;
#55768=CARTESIAN_POINT ( 'NONE',  ( 110.3678327243794541, -25.29650332976257943, 60.85276813305395649 ) ) ;
#55769=LINE ( 'NONE', #56226, #33075 ) ;
#55771=FACE_OUTER_BOUND ( 'NONE', #41825, .T. ) ;
#55772=ORIENTED_EDGE ( 'NONE', *, *, #20432, .T. ) ;
#55775=ORIENTED_EDGE ( 'NONE', *, *, #32299, .T. ) ;
#55778=CARTESIAN_POINT ( 'NONE',  ( 107.0664832912739399, -48.18858441225130917, 305.0306255462182321 ) ) ;
#55779=CARTESIAN_POINT ( 'NONE',  ( 96.80890382254112581, -40.84721887859184619, 247.6422919425769749 ) ) ;
#55780=CARTESIAN_POINT ( 'NONE',  ( 97.81085527707094229, -40.51777768585955641, 251.6359959587111064 ) ) ;
#55781=CARTESIAN_POINT ( 'NONE',  ( 136.5888380630391339, -17.63381004753921033, 2.797770231027887800 ) ) ;
#55782=DIRECTION ( 'NONE',  ( -1.000000000000000000, -4.163336342344275811E-14, 0.000000000000000000 ) ) ;
#55783=LINE ( 'NONE', #1313, #77640 ) ;
#55784=CARTESIAN_POINT ( 'NONE',  ( 181.9694315774203233, -34.03355364505981129, 342.9256252759109884 ) ) ;
#55785=CARTESIAN_POINT ( 'NONE',  ( 100.4651824673786393, -27.83460210401261747, 35.59657765686397113 ) ) ;
#55787=ORIENTED_EDGE ( 'NONE', *, *, #43160, .F. ) ;
#55788=EDGE_CURVE ( 'NONE', #55509, #4752, #38164, .T. ) ;
#55789=CARTESIAN_POINT ( 'NONE',  ( 89.06648138392552028, -56.72944715994104570, 14.67562527591095289 ) ) ;
#55790=CIRCLE ( 'NONE', #21011, 5.599999999999994316 ) ;
#55791=CARTESIAN_POINT ( 'NONE',  ( 32.06670390244800473, -32.29483332968611364, -5.074374724088000832 ) ) ;
#55792=EDGE_CURVE ( 'NONE', #53468, #14978, #35227, .T. ) ;
#55793=CARTESIAN_POINT ( 'NONE',  ( 104.1325824198641783, -27.39908484284276469, 246.3184824187669619 ) ) ;
#55794=DIRECTION ( 'NONE',  ( 0.000000000000000000, 0.000000000000000000, 1.000000000000000000 ) ) ;
#55796=CARTESIAN_POINT ( 'NONE',  ( 98.87588542518402335, -42.07524381596787322, 97.78705384733893879 ) ) ;
#55797=CARTESIAN_POINT ( 'NONE',  ( 73.06648329127396835, -8.979447159941065237, 14.92562527591093691 ) ) ;
#55798=CARTESIAN_POINT ( 'NONE',  ( 112.7336434204684252, -28.43300400972322350, 20.59933406696459457 ) ) ;
#55799=EDGE_CURVE ( 'NONE', #11998, #29962, #87636, .T. ) ;
#55801=DIRECTION ( 'NONE',  ( 0.000000000000000000, 0.000000000000000000, -1.000000000000000000 ) ) ;
#55803=ORIENTED_EDGE ( 'NONE', *, *, #54020, .T. ) ;
#55806=CARTESIAN_POINT ( 'NONE',  ( 115.1751221500829701, -40.30411560180680652, 249.9272975916113637 ) ) ;
#55808=CIRCLE ( 'NONE', #87809, 2.500000000000002220 ) ;
#55809=CARTESIAN_POINT ( 'NONE',  ( 98.30753412859742468, -41.72887538384050288, 191.7397919328074636 ) ) ;
#55810=AXIS2_PLACEMENT_3D ( 'NONE', #35365, #69906, #855 ) ;
#55814=ADVANCED_FACE ( 'NONE', ( #28880, #15255 ), #42928, .T. ) ;
#55815=CARTESIAN_POINT ( 'NONE',  ( 91.06648329127393993, -36.72944715994093912, 311.6356252759109680 ) ) ;
#55817=VECTOR ( 'NONE', #11689, 1000.000000000000000 ) ;
#55818=ORIENTED_EDGE ( 'NONE', *, *, #69897, .T. ) ;
#55819=LINE ( 'NONE', #48556, #39202 ) ;
#55820=AXIS2_PLACEMENT_3D ( 'NONE', #49350, #85259, #16641 ) ;
#55821=CARTESIAN_POINT ( 'NONE',  ( 97.81151460250711693, -40.51751193867107759, 182.6359910548048333 ) ) ;
#55823=CARTESIAN_POINT ( 'NONE',  ( 117.9248307134361937, -41.47673871369620002, 58.49848241876792798 ) ) ;
#55825=CARTESIAN_POINT ( 'NONE',  ( 101.6581149080599573, -43.36298066831790265, 11.45527697093296027 ) ) ;
#55826=EDGE_CURVE ( 'NONE', #15646, #4014, #9311, .T. ) ;
#55827=DIRECTION ( 'NONE',  ( -4.237773401492740281E-14, 1.000000000000000000, 0.000000000000000000 ) ) ;
#55828=CARTESIAN_POINT ( 'NONE',  ( 115.7764676695378512, -43.63945112744040955, 198.2927681330539542 ) ) ;
#55829=CARTESIAN_POINT ( 'NONE',  ( 165.3359832912740046, -36.32844715994100682, -5.074374724088000832 ) ) ;
#55830=FACE_OUTER_BOUND ( 'NONE', #50714, .T. ) ;
#55831=DIRECTION ( 'NONE',  ( -0.7071067811578587436, 0.7071067812152364018, 0.000000000000000000 ) ) ;
#55834=CARTESIAN_POINT ( 'NONE',  ( 110.2692182064865420, -26.72542277727598403, 230.8299109901969643 ) ) ;
#55835=CARTESIAN_POINT ( 'NONE',  ( 107.7544711540019478, -46.72718120385261642, 117.6331727250829715 ) ) ;
#55837=DIRECTION ( 'NONE',  ( 0.000000000000000000, 0.000000000000000000, -1.000000000000000000 ) ) ;
#55839=CARTESIAN_POINT ( 'NONE',  ( 114.7580948764747291, -43.83100269166961027, 119.2327681330539804 ) ) ;
#55842=CIRCLE ( 'NONE', #3674, 2.116999999999980009 ) ;
#55844=ORIENTED_EDGE ( 'NONE', *, *, #14435, .T. ) ;
#55845=DIRECTION ( 'NONE',  ( -2.734539469520093702E-14, -1.000000000000000000, 0.000000000000000000 ) ) ;
#55847=LINE ( 'NONE', #27271, #6572 ) ;
#55849=DIRECTION ( 'NONE',  ( 0.000000000000000000, 0.000000000000000000, 1.000000000000000000 ) ) ;
#55850=CARTESIAN_POINT ( 'NONE',  ( 111.3099657731024337, -28.47785412639777647, 167.5166617981629713 ) ) ;
#55851=CARTESIAN_POINT ( 'NONE',  ( 102.3694487442499934, -47.63304195565743981, 283.2527681330539053 ) ) ;
#55853=EDGE_CURVE ( 'NONE', #58766, #54444, #12228, .T. ) ;
#55856=EDGE_CURVE ( 'NONE', #48806, #241, #20913, .T. ) ;
#55857=LINE ( 'NONE', #69971, #82478 ) ;
#55864=CARTESIAN_POINT ( 'NONE',  ( 105.7994668797627185, -26.72404082623033972, 15.17729597880891390 ) ) ;
#55865=FACE_OUTER_BOUND ( 'NONE', #22744, .T. ) ;
#55866=DIRECTION ( 'NONE',  ( -1.000000000000000000, -3.999999999999999995E-14, -1.000000000000000078E-15 ) ) ;
#55867=CARTESIAN_POINT ( 'NONE',  ( 115.2610577610831655, -39.13882072599808026, 183.0209912566479602 ) ) ;
#55868=CARTESIAN_POINT ( 'NONE',  ( 116.7155050624037926, -32.57635518107161943, 79.14991099019697174 ) ) ;
#55869=ORIENTED_EDGE ( 'NONE', *, *, #30837, .F. ) ;
#55871=ORIENTED_EDGE ( 'NONE', *, *, #87642, .T. ) ;
#55873=ORIENTED_EDGE ( 'NONE', *, *, #67275, .T. ) ;
#55875=EDGE_LOOP ( 'NONE', ( #37910, #57734, #9286, #30820 ) ) ;
#55876=LINE ( 'NONE', #54530, #63893 ) ;
#55881=VERTEX_POINT ( 'NONE', #45160 ) ;
#55882=CARTESIAN_POINT ( 'NONE',  ( 112.7719768816358936, -27.93537496831996592, 69.61848241876793963 ) ) ;
#55888=DIRECTION ( 'NONE',  ( 1.000000000000000000, 0.000000000000000000, 0.000000000000000000 ) ) ;
#55890=LINE ( 'NONE', #14598, #23881 ) ;
#55893=CARTESIAN_POINT ( 'NONE',  ( 29.56670390244864777, -48.82844715994099971, 249.9678068554150059 ) ) ;
#55896=CYLINDRICAL_SURFACE ( 'NONE', #10776, 0.4999999999999989453 ) ;
#55897=CARTESIAN_POINT ( 'NONE',  ( 99.66919142226757344, -46.01935155626545537, 118.0413395616259606 ) ) ;
#55898=CARTESIAN_POINT ( 'NONE',  ( 193.5667039024415033, -48.82844715994099971, 249.9678068554149775 ) ) ;
#55899=CARTESIAN_POINT ( 'NONE',  ( 21.03715912545739641, -47.82818131006197149, 180.4678068554150911 ) ) ;
#55902=EDGE_CURVE ( 'NONE', #10820, #64140, #49939, .T. ) ;
#55903=CONICAL_SURFACE ( 'NONE', #29825, 1.219499999999975159, 1.047197551196598297 ) ;
#55905=CARTESIAN_POINT ( 'NONE',  ( 172.5664832912740110, 0.2215528400590013880, 321.0426252759119734 ) ) ;
#55906=EDGE_CURVE ( 'NONE', #39283, #70136, #23839, .T. ) ;
#55907=CARTESIAN_POINT ( 'NONE',  ( 113.4245949246307532, -29.25360672088989489, 135.5156252759109634 ) ) ;
#55909=ORIENTED_EDGE ( 'NONE', *, *, #84881, .F. ) ;
#55911=CARTESIAN_POINT ( 'NONE',  ( 97.23737678141888807, -33.32131919061086478, 282.0613395616252888 ) ) ;
#55914=DIRECTION ( 'NONE',  ( 1.000000000000000078E-15, 1.000000000000000083E-30, -1.000000000000000000 ) ) ;
#55915=CIRCLE ( 'NONE', #28380, 10.00000000000002665 ) ;
#55921=CARTESIAN_POINT ( 'NONE',  ( 97.71246005893821973, -41.20616857227592789, 216.6937205140069409 ) ) ;
#55922=ORIENTED_EDGE ( 'NONE', *, *, #84891, .T. ) ;
#55924=AXIS2_PLACEMENT_3D ( 'NONE', #17688, #73088, #81277 ) ;
#55925=CARTESIAN_POINT ( 'NONE',  ( 113.3535730310440215, -29.74740315656111989, 155.9368214011359726 ) ) ;
#55926=EDGE_CURVE ( 'NONE', #20086, #1937, #86213, .T. ) ;
#55927=DIRECTION ( 'NONE',  ( 0.000000000000000000, 1.000000000000000000, 0.000000000000000000 ) ) ;
#55928=CARTESIAN_POINT ( 'NONE',  ( 116.5375268006221319, -40.16019621794498562, 19.98158330589694387 ) ) ;
#55930=CARTESIAN_POINT ( 'NONE',  ( 151.0371591254573502, -24.42818131005592974, 249.9678068554149490 ) ) ;
#55936=CARTESIAN_POINT ( 'NONE',  ( 107.2488531970940073, -24.90511003128400347, 230.0641967044819580 ) ) ;
#55939=ORIENTED_EDGE ( 'NONE', *, *, #27432, .T. ) ;
#55943=CARTESIAN_POINT ( 'NONE',  ( 107.0664832912739968, -36.72944715994100306, 287.6356252759109680 ) ) ;
#55946=DIRECTION ( 'NONE',  ( 0.000000000000000000, 0.000000000000000000, -1.000000000000000000 ) ) ;
#55948=AXIS2_PLACEMENT_3D ( 'NONE', #7350, #55914, #21433 ) ;
#55949=DIRECTION ( 'NONE',  ( 0.000000000000000000, 0.000000000000000000, -1.000000000000000000 ) ) ;
#55950=AXIS2_PLACEMENT_3D ( 'NONE', #61196, #6248, #41195 ) ;
#55951=CARTESIAN_POINT ( 'NONE',  ( 111.6085881668573450, -46.11327973307566452, 247.9356252759109509 ) ) ;
#55953=CARTESIAN_POINT ( 'NONE',  ( 77.46225723383157913, -37.61690131752746424, 6.952852217891951625 ) ) ;
#55954=B_SPLINE_CURVE_WITH_KNOTS ( 'NONE', 3,
 ( #51753, #19037, #88095, #25857, #59463, #46725, #24961, #67635, #5418, #79501, #80389, #45821, #73551, #13565, #20831, #88981, #75351, #47620, #13131, #26741, #89889, #12681, #48498, #47169, #48951, #69878, #75799, #33558, #54420, #41698, #82183 ),
 .UNSPECIFIED., .F., .F.,
 ( 4, 2, 2, 1, 2, 2, 2, 2, 2, 2, 2, 1, 1, 2, 2, 2, 4 ),
 ( 0.000000000000000000, 0.06249999999996883049, 0.09374999999995763111, 0.1093749999999479305, 0.1171874999999430872, 0.1249999999999382161, 0.1874999999999378275, 0.2187499999999375777, 0.2499999999999373834, 0.3124999999999420464, 0.3437499999999465428, 0.3593749999999497624, 0.3671874999999486522, 0.3710937499999490963, 0.3749999999999495404, 0.4374999999999747424, 0.5000000000000000000 ),
 .UNSPECIFIED. ) ;
#55955=DIRECTION ( 'NONE',  ( 0.000000000000000000, -1.000000000000000000, 4.100000000000000342E-29 ) ) ;
#55957=CARTESIAN_POINT ( 'NONE',  ( 113.4874516948114547, -42.53221286317273098, 81.07189989340096758 ) ) ;
#55958=CARTESIAN_POINT ( 'NONE',  ( 108.8525730979967676, -47.02250997168171409, 163.7127681330539701 ) ) ;
#55959=DIRECTION ( 'NONE',  ( 0.000000000000000000, 0.000000000000000000, -1.000000000000000000 ) ) ;
#55960=ORIENTED_EDGE ( 'NONE', *, *, #4813, .F. ) ;
#55962=VECTOR ( 'NONE', #64000, 1000.000000000000114 ) ;
#55963=FACE_OUTER_BOUND ( 'NONE', #67014, .T. ) ;
#55964=ORIENTED_EDGE ( 'NONE', *, *, #14348, .F. ) ;
#55965=EDGE_LOOP ( 'NONE', ( #76252, #69548, #59319, #53269 ) ) ;
#55967=ORIENTED_EDGE ( 'NONE', *, *, #67009, .F. ) ;
#55969=DIRECTION ( 'NONE',  ( 0.000000000000000000, 0.000000000000000000, 1.000000000000000000 ) ) ;
#55970=AXIS2_PLACEMENT_3D ( 'NONE', #61384, #48634, #82309 ) ;
#55972=CARTESIAN_POINT ( 'NONE',  ( 115.1845888671227556, -34.07379402343466523, 88.50099125664800681 ) ) ;
#55973=CARTESIAN_POINT ( 'NONE',  ( 106.9401735163927611, -47.80552439772274909, 232.5794347997199907 ) ) ;
#55974=CARTESIAN_POINT ( 'NONE',  ( 97.11708974113231818, -41.49110554365062598, 216.6937205140059461 ) ) ;
#55975=DIRECTION ( 'NONE',  ( 1.000000000000000000, 0.000000000000000000, 2.283216351027200160E-14 ) ) ;
#55978=EDGE_LOOP ( 'NONE', ( #69024, #59305 ) ) ;
#55979=CARTESIAN_POINT ( 'NONE',  ( 115.8232288109526991, -31.72620974502509483, 90.24013890756648948 ) ) ;
#55980=DIRECTION ( 'NONE',  ( 0.000000000000000000, -1.000000000000000000, 0.000000000000000000 ) ) ;
#55982=CARTESIAN_POINT ( 'NONE',  ( 103.4440497394145808, -45.85039829771051245, 117.2756252759109543 ) ) ;
#55983=ADVANCED_FACE ( 'NONE', ( #2959 ), #44270, .T. ) ;
#55984=CARTESIAN_POINT ( 'NONE',  ( 108.9933628702935238, -47.01991853554855538, 82.72419670448194040 ) ) ;
#55985=CARTESIAN_POINT ( 'NONE',  ( 111.8844023637430638, -46.06429852124467317, 272.9556252759110180 ) ) ;
#55986=ORIENTED_EDGE ( 'NONE', *, *, #65777, .T. ) ;
#55987=CARTESIAN_POINT ( 'NONE',  ( 116.8850244782298091, -41.80638879970206290, 243.4346728949589647 ) ) ;
#55993=CARTESIAN_POINT ( 'NONE',  ( 105.8056005331014688, -25.33960583424948965, 320.7503373063622689 ) ) ;
#55994=DIRECTION ( 'NONE',  ( 1.000000000000000000, 1.000000000000000078E-15, 1.000000000000000078E-15 ) ) ;
#55999=CARTESIAN_POINT ( 'NONE',  ( 120.1849926298398685, -37.85453553205689303, 247.7440089327910755 ) ) ;
#56000=ORIENTED_EDGE ( 'NONE', *, *, #80365, .T. ) ;
#56002=CARTESIAN_POINT ( 'NONE',  ( 110.7409072761653306, -26.27985149715145496, 254.8194347997204545 ) ) ;
#56003=CARTESIAN_POINT ( 'NONE',  ( 108.2778103265350893, -47.71616603169876214, 153.6518157521009584 ) ) ;
#56004=CARTESIAN_POINT ( 'NONE',  ( 109.6172575917244529, -25.13135243900233817, 25.90419670448196143 ) ) ;
#56005=AXIS2_PLACEMENT_3D ( 'NONE', #45343, #78578, #72187 ) ;
#56006=CARTESIAN_POINT ( 'NONE',  ( 107.0664832912739968, -18.82844715994099971, 168.9256252759119832 ) ) ;
#56009=CARTESIAN_POINT ( 'NONE',  ( 98.04148634841929777, -41.04178939192217968, 137.6811862625705487 ) ) ;
#56010=DIRECTION ( 'NONE',  ( 1.000000000000000000, 4.299999999999999979E-14, 1.000000000000000078E-15 ) ) ;
#56012=AXIS2_PLACEMENT_3D ( 'NONE', #87531, #25291, #52959 ) ;
#56013=VECTOR ( 'NONE', #26576, 1000.000000000000000 ) ;
#56014=ORIENTED_EDGE ( 'NONE', *, *, #26606, .F. ) ;
#56016=EDGE_LOOP ( 'NONE', ( #65052, #10826, #73545, #9273 ) ) ;
#56018=CARTESIAN_POINT ( 'NONE',  ( 113.0289883941274525, -30.57309799635150682, 173.8867055423629608 ) ) ;
#56019=CARTESIAN_POINT ( 'NONE',  ( 142.0664832912740394, -45.72944715994099596, 14.67562527591100441 ) ) ;
#56021=DIRECTION ( 'NONE',  ( 0.000000000000000000, 1.000000000000000000, 0.000000000000000000 ) ) ;
#56023=CARTESIAN_POINT ( 'NONE',  ( 102.8528367378537922, -46.24122135049434235, 173.2441967044829596 ) ) ;
#56030=AXIS2_PLACEMENT_3D ( 'NONE', #56876, #21940, #64603 ) ;
#56031=CARTESIAN_POINT ( 'NONE',  ( 117.1895451461017643, -38.97942580829906944, 103.6403871806739545 ) ) ;
#56032=VERTEX_POINT ( 'NONE', #24300 ) ;
#56034=EDGE_LOOP ( 'NONE', ( #23463, #16277, #26440, #12320 ) ) ;
#56035=CARTESIAN_POINT ( 'NONE',  ( 113.8294273123088374, -42.50220367264088139, 59.69586902018298247 ) ) ;
#56037=( BOUNDED_CURVE ( )  B_SPLINE_CURVE ( 3, ( #5945, #67710, #18212, #73170 ),
 .UNSPECIFIED., .F., .T. ) 
 B_SPLINE_CURVE_WITH_KNOTS ( ( 4, 4 ),
 ( 6.634086817347963434E-13, 1.570796326796151110 ),
 .UNSPECIFIED. ) 
 CURVE ( )  GEOMETRIC_REPRESENTATION_ITEM ( )  RATIONAL_B_SPLINE_CURVE ( ( 1.000000000000000000, 0.8047378541242256045, 0.8047378541242256045, 1.000000000000000000 ) ) 
 REPRESENTATION_ITEM ( '' )  );
#56038=CARTESIAN_POINT ( 'NONE',  ( 117.2759483237919085, -34.91131378075003511, 194.9546728949579517 ) ) ;
#56039=CARTESIAN_POINT ( 'NONE',  ( 113.1782938136983603, -44.75186855938550679, 38.09395861350527213 ) ) ;
#56041=CARTESIAN_POINT ( 'NONE',  ( 97.07211459577071366, -35.37809379564900070, 56.21790486657103258 ) ) ;
#56042=CARTESIAN_POINT ( 'NONE',  ( 41.56648329127399677, -18.82844715994099971, 258.9256252759120116 ) ) ;
#56043=EDGE_CURVE ( 'NONE', #2932, #36690, #45573, .T. ) ;
#56047=CARTESIAN_POINT ( 'NONE',  ( 102.3703197837810279, -46.01248081495484854, 127.2041967044829960 ) ) ;
#56048=ORIENTED_EDGE ( 'NONE', *, *, #24940, .T. ) ;
#56049=ORIENTED_EDGE ( 'NONE', *, *, #70026, .T. ) ;
#56050=ORIENTED_EDGE ( 'NONE', *, *, #62547, .T. ) ;
#56053=CARTESIAN_POINT ( 'NONE',  ( 117.0718954856374552, -35.46248235797460779, 79.92729194244158464 ) ) ;
#56055=CARTESIAN_POINT ( 'NONE',  ( 107.4574165340472263, -45.37514529517124373, 190.4185665600669779 ) ) ;
#56056=VECTOR ( 'NONE', #18091, 1000.000000000000000 ) ;
#56057=CARTESIAN_POINT ( 'NONE',  ( 72.06648329127396835, -9.729447159941065237, 14.92562527591093691 ) ) ;
#56058=B_SPLINE_CURVE_WITH_KNOTS ( 'NONE', 3,
 ( #1968, #71466, #9228, #36928, #49190, #76926, #64629, #85547, #21522, #14704, #42375, #70104, #7879, #30561, #4193, #10554, #85988, #25077 ),
 .UNSPECIFIED., .F., .F.,
 ( 4, 2, 2, 2, 2, 2, 2, 2, 4 ),
 ( 0.4999831371813419079, 0.5624852450336741416, 0.6249873528860063754, 0.6874894607383387202, 0.7499915685906709539, 0.8124936764430031877, 0.8749957842953355325, 0.9374978921476677662, 1.000000000000000000 ),
 .UNSPECIFIED. ) ;
#56059=CARTESIAN_POINT ( 'NONE',  ( 112.1403329462429639, -28.01338855262134686, 25.65604057059988108 ) ) ;
#56060=ORIENTED_EDGE ( 'NONE', *, *, #66928, .F. ) ;
#56062=VERTEX_POINT ( 'NONE', #80166 ) ;
#56064=ORIENTED_EDGE ( 'NONE', *, *, #52227, .F. ) ;
#56066=CARTESIAN_POINT ( 'NONE',  ( 79.68962695804320617, -21.47945062089174684, 8.225625248534930378 ) ) ;
#56067=CARTESIAN_POINT ( 'NONE',  ( 106.9593448401346620, -46.12439510495315886, 229.0111071154209696 ) ) ;
#56069=ORIENTED_EDGE ( 'NONE', *, *, #67431, .T. ) ;
#56070=ADVANCED_FACE ( 'NONE', ( #45592 ), #64487, .F. ) ;
#56071=LINE ( 'NONE', #49720, #1542 ) ;
#56074=ORIENTED_EDGE ( 'NONE', *, *, #78887, .T. ) ;
#56077=CARTESIAN_POINT ( 'NONE',  ( 21.03715912545739641, -47.82818131006197149, 180.4678068554150911 ) ) ;
#56080=ADVANCED_FACE ( 'NONE', ( #31987 ), #44099, .F. ) ;
#56081=CARTESIAN_POINT ( 'NONE',  ( 111.4490224358278994, -43.61588866942526721, 260.8452332267341376 ) ) ;
#56082=CARTESIAN_POINT ( 'NONE',  ( 103.4607332334527001, -46.53479866174185986, 142.2956252759109645 ) ) ;
#56083=CARTESIAN_POINT ( 'NONE',  ( 97.28692064948100438, -31.62807703868913833, 90.93181575210196854 ) ) ;
#56084=CARTESIAN_POINT ( 'NONE',  ( 194.0371591254575492, -24.42818131005417115, 129.9678068554150343 ) ) ;
#56085=DIRECTION ( 'NONE',  ( 3.999999999999999995E-14, -1.000000000000000000, 4.100000000000000342E-29 ) ) ;
#56086=CARTESIAN_POINT ( 'NONE',  ( 97.09625178000921153, -41.50107833764869980, 212.6937205140059461 ) ) ;
#56088=DIRECTION ( 'NONE',  ( 0.000000000000000000, 0.000000000000000000, 1.000000000000000000 ) ) ;
#56089=ORIENTED_EDGE ( 'NONE', *, *, #88236, .T. ) ;
#56090=LINE ( 'NONE', #20263, #26458 ) ;
#56091=ORIENTED_EDGE ( 'NONE', *, *, #68276, .F. ) ;
#56092=EDGE_LOOP ( 'NONE', ( #81394, #87229, #67469, #7691 ) ) ;
#56093=DIRECTION ( 'NONE',  ( 0.000000000000000000, 0.000000000000000000, -1.000000000000000000 ) ) ;
#56094=AXIS2_PLACEMENT_3D ( 'NONE', #29985, #58124, #21378 ) ;
#56095=CARTESIAN_POINT ( 'NONE',  ( 97.70649186885867721, -40.25113332959050183, 137.6128355545769466 ) ) ;
#56096=ADVANCED_FACE ( 'NONE', ( #53748 ), #33338, .T. ) ;
#56097=EDGE_LOOP ( 'NONE', ( #73769, #44591, #65731, #11899 ) ) ;
#56098=CARTESIAN_POINT ( 'NONE',  ( 108.9848901524495801, -47.61516268848960465, 122.7032443235299723 ) ) ;
#56099=CARTESIAN_POINT ( 'NONE',  ( 167.7413838386819691, -48.33240602328260849, 129.9678068554150059 ) ) ;
#56101=LINE ( 'NONE', #2518, #60104 ) ;
#56102=FACE_OUTER_BOUND ( 'NONE', #28113, .T. ) ;
#56103=CARTESIAN_POINT ( 'NONE',  ( 116.7787425647057091, -34.05740579004297075, 59.03918106495919460 ) ) ;
#56104=CARTESIAN_POINT ( 'NONE',  ( 117.3134009501234658, -34.93240959161192905, 239.9641967044819637 ) ) ;
#56109=DIRECTION ( 'NONE',  ( 0.000000000000000000, 0.000000000000000000, -1.000000000000000000 ) ) ;
#56110=LINE ( 'NONE', #82527, #45891 ) ;
#56112=DIRECTION ( 'NONE',  ( -0.04216478779797398074, 0.9991106698809455455, 0.000000000000000000 ) ) ;
#56114=CARTESIAN_POINT ( 'NONE',  ( 107.0667039024479834, -36.72944715994099596, 239.5838068554170093 ) ) ;
#56115=CARTESIAN_POINT ( 'NONE',  ( 113.6284486023480724, -28.60005753680112761, 164.5356252759109736 ) ) ;
#56116=CARTESIAN_POINT ( 'NONE',  ( 112.8177273059790764, -27.29031728650405597, 45.62895860924398761 ) ) ;
#56117=CARTESIAN_POINT ( 'NONE',  ( 114.1542194384027908, -29.02509929289194801, 195.4841967044819739 ) ) ;
#56118=CARTESIAN_POINT ( 'NONE',  ( 51.42025729304101844, -33.70561438051982606, 342.9256252759109884 ) ) ;
#56119=LINE ( 'NONE', #83872, #27156 ) ;
#56120=CARTESIAN_POINT ( 'NONE',  ( 25.56670390244797275, -65.37844715994100397, 257.2178068554150059 ) ) ;
#56121=DIRECTION ( 'NONE',  ( 0.000000000000000000, 0.000000000000000000, 1.000000000000000000 ) ) ;
#56123=CARTESIAN_POINT ( 'NONE',  ( 37.03715912545433042, -48.62818131006122258, 249.9678068554150343 ) ) ;
#56125=AXIS2_PLACEMENT_3D ( 'NONE', #1298, #43950, #78513 ) ;
#56126=FACE_BOUND ( 'NONE', #69094, .T. ) ;
#56128=VERTEX_POINT ( 'NONE', #60582 ) ;
#56129=EDGE_CURVE ( 'NONE', #39780, #28327, #74674, .T. ) ;
#56130=CARTESIAN_POINT ( 'NONE',  ( 184.5667039024480118, -67.87844715994100397, 20.91780685541479912 ) ) ;
#56131=ORIENTED_EDGE ( 'NONE', *, *, #71944, .F. ) ;
#56132=CARTESIAN_POINT ( 'NONE',  ( 110.3650187231686601, -47.25482062520513438, 48.80610146638797175 ) ) ;
#56133=DIRECTION ( 'NONE',  ( 0.4214249218767882055, 0.9068632946707806397, 4.214249218767890910E-16 ) ) ;
#56136=CARTESIAN_POINT ( 'NONE',  ( 117.1100247017212723, -39.68245506451066262, 179.5984824187679294 ) ) ;
#56137=EDGE_CURVE ( 'NONE', #60854, #69462, #7939, .T. ) ;
#56138=AXIS2_PLACEMENT_3D ( 'NONE', #55223, #76136, #89789 ) ;
#56139=VECTOR ( 'NONE', #68060, 1000.000000000000000 ) ;
#56140=CARTESIAN_POINT ( 'NONE',  ( 106.8780034376490278, -45.26880352128168283, 271.9809912566482808 ) ) ;
#56141=VERTEX_POINT ( 'NONE', #39693 ) ;
#56142=ORIENTED_EDGE ( 'NONE', *, *, #32195, .F. ) ;
#56143=ORIENTED_EDGE ( 'NONE', *, *, #80691, .T. ) ;
#56144=VECTOR ( 'NONE', #32325, 1000.000000000000000 ) ;
#56150=DIRECTION ( 'NONE',  ( -1.000000000000000078E-15, 0.000000000000000000, -1.000000000000000000 ) ) ;
#56153=CARTESIAN_POINT ( 'NONE',  ( 177.0371591254545933, -48.62818131005479927, 129.9678068554150059 ) ) ;
#56155=CARTESIAN_POINT ( 'NONE',  ( 48.16670390244647137, -26.71338133339281029, 193.9678068554150911 ) ) ;
#56157=EDGE_CURVE ( 'NONE', #36065, #73817, #54196, .T. ) ;
#56158=CARTESIAN_POINT ( 'NONE',  ( 100.6111884388666766, -28.52632756463403751, 15.60705384733995871 ) ) ;
#56159=DIRECTION ( 'NONE',  ( 0.000000000000000000, 0.000000000000000000, -1.000000000000000000 ) ) ;
#56160=VERTEX_POINT ( 'NONE', #61929 ) ;
#56161=AXIS2_PLACEMENT_3D ( 'NONE', #29882, #78929, #2622 ) ;
#56162=CARTESIAN_POINT ( 'NONE',  ( 97.07207223047387856, -35.37843998912999410, 271.2189585129040097 ) ) ;
#56165=DIRECTION ( 'NONE',  ( -3.999999999999999995E-14, 1.000000000000000000, -4.100000000000000342E-29 ) ) ;
#56166=CARTESIAN_POINT ( 'NONE',  ( 99.36125835269150741, -32.78858003560463175, 93.78047132197198721 ) ) ;
#56168=CARTESIAN_POINT ( 'NONE',  ( 182.4202572930406916, -33.70561438051399961, 313.9678068554149490 ) ) ;
#56169=CARTESIAN_POINT ( 'NONE',  ( 112.1393456408476510, -28.01282278068320508, 44.65645860931923750 ) ) ;
#56171=ORIENTED_EDGE ( 'NONE', *, *, #4171, .T. ) ;
#56172=CARTESIAN_POINT ( 'NONE',  ( 97.81553679132888135, -40.52681664444901344, 136.6368110416782145 ) ) ;
#56173=ORIENTED_EDGE ( 'NONE', *, *, #40737, .F. ) ;
#56174=ORIENTED_EDGE ( 'NONE', *, *, #277, .T. ) ;
#56175=CARTESIAN_POINT ( 'NONE',  ( 99.22037001696983793, -32.61037140242165577, 132.3730118773259790 ) ) ;
#56177=CONICAL_SURFACE ( 'NONE', #25788, 5.799999999999998934, 0.7853981633974369547 ) ;
#56178=CARTESIAN_POINT ( 'NONE',  ( 114.0366484478682310, -28.94779845652852757, 110.4956252759109816 ) ) ;
#56179=AXIS2_PLACEMENT_3D ( 'NONE', #2086, #70226, #8000 ) ;
#56180=DIRECTION ( 'NONE',  ( 0.000000000000000000, 0.000000000000000000, 1.000000000000000000 ) ) ;
#56181=ORIENTED_EDGE ( 'NONE', *, *, #69384, .T. ) ;
#56182=ORIENTED_EDGE ( 'NONE', *, *, #85526, .F. ) ;
#56183=ORIENTED_EDGE ( 'NONE', *, *, #6513, .T. ) ;
#56184=EDGE_CURVE ( 'NONE', #46552, #69245, #87861, .T. ) ;
#56185=DIRECTION ( 'NONE',  ( 6.745093096447288888E-17, 1.000000000000000000, 0.000000000000000000 ) ) ;
#56186=ORIENTED_EDGE ( 'NONE', *, *, #68222, .T. ) ;
#56187=CARTESIAN_POINT ( 'NONE',  ( 117.4903696573864522, -37.28369426754697002, 18.78419670448294809 ) ) ;
#56188=CARTESIAN_POINT ( 'NONE',  ( 98.64836624540230048, -30.48328824330908660, 176.8184824187679567 ) ) ;
#56189=CYLINDRICAL_SURFACE ( 'NONE', #80016, 16.00000000000090239 ) ;
#56190=CARTESIAN_POINT ( 'NONE',  ( 83.56670390244801183, -37.98819715994108037, 218.8274735512160589 ) ) ;
#56191=CARTESIAN_POINT ( 'NONE',  ( 116.9041476981693677, -40.17949737190902937, 129.5584824187679658 ) ) ;
#56193=ORIENTED_EDGE ( 'NONE', *, *, #51022, .T. ) ;
#56196=DIRECTION ( 'NONE',  ( -1.000000000000000000, -3.999999999999999995E-14, 4.193851878741028267E-47 ) ) ;
#56198=AXIS2_PLACEMENT_3D ( 'NONE', #35811, #8573, #63526 ) ;
#56200=VECTOR ( 'NONE', #16954, 1000.000000000000000 ) ;
#56201=EDGE_CURVE ( 'NONE', #33687, #14469, #39823, .T. ) ;
#56203=CARTESIAN_POINT ( 'NONE',  ( 96.34404753607181249, -39.41381804822120216, 16.53372051400597798 ) ) ;
#56205=LINE ( 'NONE', #34436, #24611 ) ;
#56207=CARTESIAN_POINT ( 'NONE',  ( 110.2835424219824034, -44.64187515646635518, 282.3067055423625789 ) ) ;
#56208=DIRECTION ( 'NONE',  ( -1.000000000000000078E-15, 1.000000000000000083E-30, 1.000000000000000000 ) ) ;
#56209=CARTESIAN_POINT ( 'NONE',  ( 95.33621695423336462, -38.27597901479983733, 147.4299109901969871 ) ) ;
#56210=CARTESIAN_POINT ( 'NONE',  ( 105.7995184819918535, -26.72403496654249011, 71.17729194302346230 ) ) ;
#56211=DIRECTION ( 'NONE',  ( 0.000000000000000000, 1.000000000000000000, 0.000000000000000000 ) ) ;
#56212=ORIENTED_EDGE ( 'NONE', *, *, #73056, .F. ) ;
#56213=CYLINDRICAL_SURFACE ( 'NONE', #62813, 3.000000000000002665 ) ;
#56214=CARTESIAN_POINT ( 'NONE',  ( 75.31670390244798341, -57.40094715994099772, 35.51780685541480409 ) ) ;
#56216=ORIENTED_EDGE ( 'NONE', *, *, #36217, .T. ) ;
#56218=EDGE_CURVE ( 'NONE', #71147, #18287, #54332, .T. ) ;
#56220=CARTESIAN_POINT ( 'NONE',  ( 102.8260968645185045, -46.30158323273214904, 177.2441967044819648 ) ) ;
#56221=ORIENTED_EDGE ( 'NONE', *, *, #81708, .T. ) ;
#56222=FACE_OUTER_BOUND ( 'NONE', #45822, .T. ) ;
#56223=CARTESIAN_POINT ( 'NONE',  ( 113.0346028865331363, -45.34691455509256031, 199.0584824187679374 ) ) ;
#56224=CARTESIAN_POINT ( 'NONE',  ( 96.13205292066136565, -38.63620640773733328, 42.45181575210199298 ) ) ;
#56225=AXIS2_PLACEMENT_3D ( 'NONE', #41414, #19644, #67796 ) ;
#56226=CARTESIAN_POINT ( 'NONE',  ( 63.06670390244736524, -24.92844715994017690, 249.9678068554150343 ) ) ;
#56229=DIRECTION ( 'NONE',  ( -6.524622321627019585E-16, -4.013151879589939944E-16, -1.000000000000000000 ) ) ;
#56232=EDGE_CURVE ( 'NONE', #21135, #17509, #89189, .T. ) ;
#56233=VERTEX_POINT ( 'NONE', #81959 ) ;
#56235=VERTEX_POINT ( 'NONE', #41038 ) ;
#56236=DIRECTION ( 'NONE',  ( 0.7071067809773464719, -0.7071067813957485626, 7.071067809773160819E-16 ) ) ;
#56237=CARTESIAN_POINT ( 'NONE',  ( 101.2940058763137330, -26.37990030743140224, 251.4813395616249920 ) ) ;
#56240=EDGE_CURVE ( 'NONE', #44500, #59691, #75123, .T. ) ;
#56241=LINE ( 'NONE', #14040, #87376 ) ;
#56242=CARTESIAN_POINT ( 'NONE',  ( 182.4202572930259976, -31.94127993907710206, -5.074374724088000832 ) ) ;
#56244=CARTESIAN_POINT ( 'NONE',  ( 111.3322245453084918, -27.19268589797737334, 24.74133956162494030 ) ) ;
#56246=CIRCLE ( 'NONE', #15697, 10.00000000000000355 ) ;
#56248=CARTESIAN_POINT ( 'NONE',  ( 151.0371591254575776, -24.42818131005592264, 129.9678068554149775 ) ) ;
#56249=CARTESIAN_POINT ( 'NONE',  ( 97.53179058352803565, -39.74878676319904969, 17.57055365400502822 ) ) ;
#56250=CARTESIAN_POINT ( 'NONE',  ( 115.4995704134666141, -41.68388727776409297, 234.4041967044819899 ) ) ;
#56253=CARTESIAN_POINT ( 'NONE',  ( 116.0809032858470999, -32.84949784884748425, 75.14991099019596277 ) ) ;
#56255=EDGE_CURVE ( 'NONE', #7616, #19968, #40596, .T. ) ;
#56259=LINE ( 'NONE', #73376, #5135 ) ;
#56261=CIRCLE ( 'NONE', #62055, 5.599999999999994316 ) ;
#56262=ORIENTED_EDGE ( 'NONE', *, *, #56951, .F. ) ;
#56265=CARTESIAN_POINT ( 'NONE',  ( 106.3528233092926740, -46.09786297945525035, 263.9596785439923678 ) ) ;
#56266=AXIS2_PLACEMENT_3D ( 'NONE', #4206, #25089, #87328 ) ;
#56270=DIRECTION ( 'NONE',  ( -0.7071067812164788524, 0.7071067811566160710, 0.000000000000000000 ) ) ;
#56271=FACE_OUTER_BOUND ( 'NONE', #53817, .T. ) ;
#56272=VERTEX_POINT ( 'NONE', #74234 ) ;
#56274=AXIS2_PLACEMENT_3D ( 'NONE', #28829, #55595, #56512 ) ;
#56277=CARTESIAN_POINT ( 'NONE',  ( 96.92686062739846875, -39.15330414739766240, 56.51276813305394597 ) ) ;
#56278=ORIENTED_EDGE ( 'NONE', *, *, #69074, .F. ) ;
#56279=CARTESIAN_POINT ( 'NONE',  ( 105.6358988306284346, -28.30874812457275524, 14.63241982807694797 ) ) ;
#56280=CIRCLE ( 'NONE', #5611, 2.030000000000003801 ) ;
#56282=CARTESIAN_POINT ( 'NONE',  ( 96.28008679191512442, -39.42493101749853679, 166.5213395616259788 ) ) ;
#56283=DIRECTION ( 'NONE',  ( 1.607304094387810152E-29, -0.7071067811865555663, 0.7071067811865394681 ) ) ;
#56284=CARTESIAN_POINT ( 'NONE',  ( 168.3664380525666218, -48.62818131005518296, 249.9678068554149775 ) ) ;
#56285=VECTOR ( 'NONE', #36755, 1000.000000000000000 ) ;
#56286=PLANE ( 'NONE',  #36128 ) ;
#56288=DIRECTION ( 'NONE',  ( -1.000000000000000078E-15, 1.000000000000000083E-30, 1.000000000000000000 ) ) ;
#56289=CARTESIAN_POINT ( 'NONE',  ( 112.3603056216204550, -28.17164194844215430, 285.6356252759109680 ) ) ;
#56291=VERTEX_POINT ( 'NONE', #36025 ) ;
#56292=CARTESIAN_POINT ( 'NONE',  ( 136.8151996730033204, -36.82419990104954621, 6.751707299519810412 ) ) ;
#56293=ORIENTED_EDGE ( 'NONE', *, *, #77938, .F. ) ;
#56294=CARTESIAN_POINT ( 'NONE',  ( 103.1892778894433320, -46.49189014610453086, 113.2756252759109827 ) ) ;
#56296=ORIENTED_EDGE ( 'NONE', *, *, #36764, .T. ) ;
#56297=CARTESIAN_POINT ( 'NONE',  ( 115.8254323948531095, -31.73001883592735339, 119.2397919419617551 ) ) ;
#56300=VECTOR ( 'NONE', #54508, 1000.000000000000000 ) ;
#56301=DIRECTION ( 'NONE',  ( 1.000000000000000078E-15, 0.000000000000000000, 1.000000000000000000 ) ) ;
#56302=CARTESIAN_POINT ( 'NONE',  ( 108.4174969398134323, -26.73503709278844198, 265.9689579970951172 ) ) ;
#56304=CARTESIAN_POINT ( 'NONE',  ( 179.7974245136200011, -36.32844715994040996, -5.074374724088000832 ) ) ;
#56305=CARTESIAN_POINT ( 'NONE',  ( 194.0371591254584587, -46.82818131005407736, 193.9678068554150343 ) ) ;
#56306=CARTESIAN_POINT ( 'NONE',  ( 105.4209835578153189, -47.02385428587647453, 33.44991099019695469 ) ) ;
#56308=ORIENTED_EDGE ( 'NONE', *, *, #84455, .F. ) ;
#56311=DIRECTION ( 'NONE',  ( 0.000000000000000000, -1.000000000000000000, 0.000000000000000000 ) ) ;
#56313=CIRCLE ( 'NONE', #30212, 0.5000000000000073275 ) ;
#56314=ORIENTED_EDGE ( 'NONE', *, *, #49200, .F. ) ;
#56315=DIRECTION ( 'NONE',  ( 0.000000000000000000, -1.000000000000000000, 0.000000000000000000 ) ) ;
#56316=ADVANCED_FACE ( 'NONE', ( #8785 ), #21058, .F. ) ;
#56320=DIRECTION ( 'NONE',  ( -2.981567257902526681E-15, 0.8571673007021100021, 0.5150380749100580413 ) ) ;
#56321=LINE ( 'NONE', #62705, #76523 ) ;
#56322=CARTESIAN_POINT ( 'NONE',  ( 97.51448592794399417, -38.47012922887837760, 200.8924198280769815 ) ) ;
#56323=DIRECTION ( 'NONE',  ( -0.7071067811865165975, -0.7071067811865784369, -7.071067811865158803E-16 ) ) ;
#56324=CARTESIAN_POINT ( 'NONE',  ( 113.4422559937560777, -27.64306140573813408, 84.57753003781698453 ) ) ;
#56325=ORIENTED_EDGE ( 'NONE', *, *, #14940, .F. ) ;
#56326=CARTESIAN_POINT ( 'NONE',  ( 162.5667039024460223, -19.82844715994111340, -5.074374724088000832 ) ) ;
#56327=ORIENTED_EDGE ( 'NONE', *, *, #54234, .F. ) ;
#56328=ADVANCED_FACE ( 'NONE', ( #21970 ), #62378, .T. ) ;
#56332=CIRCLE ( 'NONE', #17197, 0.5000000000000004441 ) ;
#56333=EDGE_CURVE ( 'NONE', #1134, #85218, #3591, .T. ) ;
#56334=CARTESIAN_POINT ( 'NONE',  ( 112.1392665423922210, -28.01277399031326709, 49.65646589883106543 ) ) ;
#56336=DIRECTION ( 'NONE',  ( -0.7071067811865274777, 0.7071067811865675568, -7.071067811865283048E-16 ) ) ;
#56338=CARTESIAN_POINT ( 'NONE',  ( 112.0677311185675649, -45.48738121332133488, 273.9895100238672399 ) ) ;
#56339=EDGE_CURVE ( 'NONE', #10437, #33219, #6978, .T. ) ;
#56344=CARTESIAN_POINT ( 'NONE',  ( 104.7546666864753320, -46.91776733316893200, 72.39848241876795498 ) ) ;
#56346=ADVANCED_FACE ( 'NONE', ( #49636 ), #28300, .F. ) ;
#56347=DIRECTION ( 'NONE',  ( 0.000000000000000000, 0.000000000000000000, -1.000000000000000000 ) ) ;
#56348=FACE_OUTER_BOUND ( 'NONE', #52122, .T. ) ;
#56349=LINE ( 'NONE', #27762, #14770 ) ;
#56350=CARTESIAN_POINT ( 'NONE',  ( 80.06648329127402519, -46.72944715994105991, 4.925625275910944012 ) ) ;
#56351=ORIENTED_EDGE ( 'NONE', *, *, #69793, .F. ) ;
#56352=AXIS2_PLACEMENT_3D ( 'NONE', #4020, #89282, #88835 ) ;
#56353=ADVANCED_FACE ( 'NONE', ( #56451 ), #13791, .T. ) ;
#56354=DIRECTION ( 'NONE',  ( 0.000000000000000000, -1.000000000000000000, 0.000000000000000000 ) ) ;
#56356=EDGE_CURVE ( 'NONE', #51043, #18192, #61612, .T. ) ;
#56357=VECTOR ( 'NONE', #17955, 999.9999999999998863 ) ;
#56358=DIRECTION ( 'NONE',  ( -1.000000000000000000, -4.299999999999999979E-14, -1.000000000000000078E-15 ) ) ;
#56359=CARTESIAN_POINT ( 'NONE',  ( 108.0361718062294614, -25.69563957016125855, 105.9946728949589811 ) ) ;
#56360=VECTOR ( 'NONE', #5762, 1000.000000000000000 ) ;
#56362=LINE ( 'NONE', #70014, #89180 ) ;
#56364=ORIENTED_EDGE ( 'NONE', *, *, #41027, .F. ) ;
#56366=CARTESIAN_POINT ( 'NONE',  ( 108.9483104351207174, -46.92736419409149562, 123.7337205140059666 ) ) ;
#56368=CARTESIAN_POINT ( 'NONE',  ( 130.3998166246059895, 12.92155284005730387, 361.9756252759109998 ) ) ;
#56369=ORIENTED_EDGE ( 'NONE', *, *, #36602, .T. ) ;
#56370=ADVANCED_FACE ( 'NONE', ( #64189 ), #15141, .F. ) ;
#56371=CARTESIAN_POINT ( 'NONE',  ( 118.0844448206163833, -36.21142561920247971, 264.8518157521014587 ) ) ;
#56373=CARTESIAN_POINT ( 'NONE',  ( 95.60734603896362671, -36.72944715994100306, 394.9756252759102040 ) ) ;
#56381=CARTESIAN_POINT ( 'NONE',  ( 114.4768422515204946, -30.34587328852055066, 184.3927681330539770 ) ) ;
#56382=ORIENTED_EDGE ( 'NONE', *, *, #60636, .F. ) ;
#56383=VERTEX_POINT ( 'NONE', #44162 ) ;
#56385=CARTESIAN_POINT ( 'NONE',  ( 113.4085779730985166, -29.80024602262787425, 150.9063452106589693 ) ) ;
#56387=CARTESIAN_POINT ( 'NONE',  ( 115.5794671477453761, -31.87256924526127477, 285.2384824187676600 ) ) ;
#56389=CARTESIAN_POINT ( 'NONE',  ( 115.7825698381208213, -41.80321761809266690, 268.4065905822184845 ) ) ;
#56390=LINE ( 'NONE', #84132, #80632 ) ;
#56391=CARTESIAN_POINT ( 'NONE',  ( 168.0371591254546217, -48.62818131005519007, 129.9678068554150059 ) ) ;
#56392=CARTESIAN_POINT ( 'NONE',  ( 176.7669697523285208, -48.62818131005431610, 180.4678068554150059 ) ) ;
#56393=CARTESIAN_POINT ( 'NONE',  ( 116.5068947302722222, -41.18400185692905069, 228.4756252759109714 ) ) ;
#56394=CARTESIAN_POINT ( 'NONE',  ( 97.80437445726883539, -40.49951938081226643, 171.6343582250473787 ) ) ;
#56395=VERTEX_POINT ( 'NONE', #31883 ) ;
#56396=ORIENTED_EDGE ( 'NONE', *, *, #35430, .F. ) ;
#56400=CARTESIAN_POINT ( 'NONE',  ( 98.54754732716219223, -41.97681284361367204, 122.7650852229510576 ) ) ;
#56401=DIRECTION ( 'NONE',  ( -4.237773401492740281E-14, 1.000000000000000000, 0.000000000000000000 ) ) ;
#56402=CARTESIAN_POINT ( 'NONE',  ( 95.98894198207693762, -35.78073158428682632, 32.25848241876694544 ) ) ;
#56403=AXIS2_PLACEMENT_3D ( 'NONE', #87565, #45743, #24449 ) ;
#56404=FACE_OUTER_BOUND ( 'NONE', #49804, .T. ) ;
#56405=VERTEX_POINT ( 'NONE', #30109 ) ;
#56407=CARTESIAN_POINT ( 'NONE',  ( 37.03715912545427358, -48.62818131006101652, 300.4678068554150059 ) ) ;
#56408=CARTESIAN_POINT ( 'NONE',  ( 96.24916995763402383, -34.45682319295006124, 261.1737205140064475 ) ) ;
#56409=ORIENTED_EDGE ( 'NONE', *, *, #19630, .T. ) ;
#56410=AXIS2_PLACEMENT_3D ( 'NONE', #83253, #15099, #49142 ) ;
#56412=CARTESIAN_POINT ( 'NONE',  ( 172.5664832912729878, -27.82844715994070484, 75.92562527591199739 ) ) ;
#56414=CARTESIAN_POINT ( 'NONE',  ( 102.4269143325283835, -29.42360532460997291, 63.33285227435298026 ) ) ;
#56416=CARTESIAN_POINT ( 'NONE',  ( 96.59701100649584760, -36.21046171878319342, 167.2870538473399620 ) ) ;
#56418=ORIENTED_EDGE ( 'NONE', *, *, #73056, .T. ) ;
#56420=CARTESIAN_POINT ( 'NONE',  ( 46.48091746482131015, -48.32844715994084339, 249.9678068554150343 ) ) ;
#56421=ORIENTED_EDGE ( 'NONE', *, *, #20414, .F. ) ;
#56423=DIRECTION ( 'NONE',  ( 1.000000000000000078E-15, 1.000000000000000083E-30, -1.000000000000000000 ) ) ;
#56424=ORIENTED_EDGE ( 'NONE', *, *, #19432, .T. ) ;
#56429=CARTESIAN_POINT ( 'NONE',  ( 97.81170003938157720, -40.51743348276853851, 42.63567940883270069 ) ) ;
#56430=CIRCLE ( 'NONE', #24552, 10.00000000000000888 ) ;
#56431=CARTESIAN_POINT ( 'NONE',  ( 99.76075522406560481, -42.08098971643298825, 106.2400388756959728 ) ) ;
#56432=CARTESIAN_POINT ( 'NONE',  ( 111.4898014013570560, -26.57429697695857129, 284.7375300378155316 ) ) ;
#56433=ADVANCED_FACE ( 'NONE', ( #9658 ), #22478, .F. ) ;
#56436=ADVANCED_FACE ( 'NONE', ( #72784 ), #37368, .T. ) ;
#56437=ORIENTED_EDGE ( 'NONE', *, *, #41289, .T. ) ;
#56439=FACE_OUTER_BOUND ( 'NONE', #14788, .T. ) ;
#56441=AXIS2_PLACEMENT_3D ( 'NONE', #28017, #57063, #28932 ) ;
#56442=ADVANCED_FACE ( 'NONE', ( #30556 ), #85542, .F. ) ;
#56443=CARTESIAN_POINT ( 'NONE',  ( 98.75024281215304711, -42.92452016420553917, 111.8480062282929737 ) ) ;
#56444=CARTESIAN_POINT ( 'NONE',  ( 98.55409819730274990, -43.85350384415066571, 71.86895860924397539 ) ) ;
#56447=CARTESIAN_POINT ( 'NONE',  ( 116.9255123305063222, -41.72731008894000837, 248.4651490854349731 ) ) ;
#56448=DIRECTION ( 'NONE',  ( 0.000000000000000000, 0.000000000000000000, -1.000000000000000000 ) ) ;
#56451=FACE_OUTER_BOUND ( 'NONE', #14105, .T. ) ;
#56452=CARTESIAN_POINT ( 'NONE',  ( 106.0697754944390994, -25.31338314874918538, 320.6231843933491064 ) ) ;
#56453=CARTESIAN_POINT ( 'NONE',  ( 125.8897075496517317, -55.55267141831851774, -4.824374724089010691 ) ) ;
#56456=DIRECTION ( 'NONE',  ( -1.000000000000000000, 6.036837696399451257E-13, 0.000000000000000000 ) ) ;
#56458=CARTESIAN_POINT ( 'NONE',  ( 29.56648329127400388, 15.62155284005900491, 323.8756252759109202 ) ) ;
#56459=EDGE_CURVE ( 'NONE', #57152, #48829, #18106, .T. ) ;
#56460=CARTESIAN_POINT ( 'NONE',  ( 33.92127028473601769, -29.73316016639540749, -5.074374724088000832 ) ) ;
#56461=ORIENTED_EDGE ( 'NONE', *, *, #49161, .T. ) ;
#56464=CARTESIAN_POINT ( 'NONE',  ( 115.7136949400716333, -42.59221908682786761, 273.3527681330537575 ) ) ;
#56465=CARTESIAN_POINT ( 'NONE',  ( 117.6790090996954632, -39.81947568642139856, 134.5889586092439743 ) ) ;
#56466=CARTESIAN_POINT ( 'NONE',  ( 102.7462986198438273, -25.66788047019655394, 16.37276813305293999 ) ) ;
#56467=DIRECTION ( 'NONE',  ( 1.000000000000000000, 0.000000000000000000, 0.000000000000000000 ) ) ;
#56468=FACE_OUTER_BOUND ( 'NONE', #68941, .T. ) ;
#56469=CARTESIAN_POINT ( 'NONE',  ( 82.67897566168164758, -35.84952872354146791, 6.945088388039701854 ) ) ;
#56471=ADVANCED_FACE ( 'NONE', ( #59130 ), #76150, .T. ) ;
#56472=VECTOR ( 'NONE', #30768, 1000.000000000000000 ) ;
#56473=AXIS2_PLACEMENT_3D ( 'NONE', #31495, #37440, #59203 ) ;
#56474=ORIENTED_EDGE ( 'NONE', *, *, #79233, .F. ) ;
#56476=ORIENTED_EDGE ( 'NONE', *, *, #60790, .F. ) ;
#56477=ADVANCED_BREP_SHAPE_REPRESENTATION ( '', ( #18841, #50656 ), #27505 ) ;
#56478=CARTESIAN_POINT ( 'NONE',  ( 115.4440039095595409, -34.92134030032634939, 183.4181341137909556 ) ) ;
#56479=AXIS2_PLACEMENT_3D ( 'NONE', #84799, #70255, #77974 ) ;
#56480=FACE_BOUND ( 'NONE', #67253, .T. ) ;
#56482=PLANE ( 'NONE',  #70766 ) ;
#56483=CARTESIAN_POINT ( 'NONE',  ( 116.6407469026008243, -40.79910830432089597, 164.5070538473399608 ) ) ;
#56484=CARTESIAN_POINT ( 'NONE',  ( 113.1759050958252004, -44.75365348611187244, 149.0944250870025769 ) ) ;
#56485=B_SPLINE_CURVE_WITH_KNOTS ( 'NONE', 3,
 ( #12559, #40247, #55200, #67964, #88869, #26625, #82514, #54301, #82068, #47942, #47498, #40698, #33884, #61581, #56566, #2517, #23423, #9325, #15702, #70662, #72004, #29773, #42475, #9771, #51089, #1630, #14809, #50646, #71564, #49745, #50195, #77469, #78827, #37028, #36595, #22971, #28877 ),
 .UNSPECIFIED., .F., .F.,
 ( 4, 2, 2, 1, 2, 2, 2, 1, 1, 2, 2, 2, 2, 1, 2, 2, 2, 1, 1, 1, 2, 4 ),
 ( 0.6666501603260894804, 0.6874845253057108030, 0.6926931165506157173, 0.6979017077955206316, 0.7083188902853314595, 0.7499876202445696638, 0.7525919158670218989, 0.7551962114894742450, 0.7604048027343788263, 0.7708219852241890990, 0.7916563502038072020, 0.8124907151834253050, 0.8176993064283285539, 0.8229078976732318029, 0.8333250801630380789, 0.8749938101222534126, 0.8775981057447067579, 0.8802024013671601033, 0.8854109926120669050, 0.8958281751018802863, 0.9166625400815033853, 1.000000000000000000 ),
 .UNSPECIFIED. ) ;
#56486=CARTESIAN_POINT ( 'NONE',  ( 97.33789316567710159, -34.07085429710922142, 151.1152779172331861 ) ) ;
#56490=AXIS2_PLACEMENT_3D ( 'NONE', #71017, #8794, #49643 ) ;
#56492=CARTESIAN_POINT ( 'NONE',  ( 115.9482186066389602, -32.63332544795704138, 104.1699109901969535 ) ) ;
#56493=ORIENTED_EDGE ( 'NONE', *, *, #79874, .F. ) ;
#56495=ORIENTED_EDGE ( 'NONE', *, *, #22542, .F. ) ;
#56496=CARTESIAN_POINT ( 'NONE',  ( 107.7480938161759951, -27.89408153625565845, 66.44729759161194238 ) ) ;
#56498=CARTESIAN_POINT ( 'NONE',  ( 98.33750497493211640, -41.21483588869658377, 192.7041967044819728 ) ) ;
#56500=CARTESIAN_POINT ( 'NONE',  ( 105.8002047024404106, -26.72394367052961428, 55.17592173170812231 ) ) ;
#56502=AXIS2_PLACEMENT_3D ( 'NONE', #46604, #52069, #38457 ) ;
#56503=CARTESIAN_POINT ( 'NONE',  ( 63.56670390244714497, -40.82844715994014706, 129.9678068554150911 ) ) ;
#56504=PLANE ( 'NONE',  #50688 ) ;
#56506=CARTESIAN_POINT ( 'NONE',  ( 108.9808406375927063, -47.59218431635562041, 122.7032443235299723 ) ) ;
#56507=ORIENTED_EDGE ( 'NONE', *, *, #9405, .F. ) ;
#56508=EDGE_LOOP ( 'NONE', ( #24867, #47104, #87284, #87740 ) ) ;
#56509=ORIENTED_EDGE ( 'NONE', *, *, #26914, .T. ) ;
#56512=DIRECTION ( 'NONE',  ( 1.000000000000000000, 4.299999999999999979E-14, 1.000000000000000078E-15 ) ) ;
#56513=CARTESIAN_POINT ( 'NONE',  ( 99.09507197483526397, -30.55126955676270839, 130.8023766919142474 ) ) ;
#56515=CARTESIAN_POINT ( 'NONE',  ( 98.49961498605385657, -35.50075171889626091, 224.0433284648299548 ) ) ;
#56516=VECTOR ( 'NONE', #57855, 1000.000000000000000 ) ;
#56519=DIRECTION ( 'NONE',  ( 0.000000000000000000, 0.000000000000000000, 1.000000000000000000 ) ) ;
#56522=VERTEX_POINT ( 'NONE', #33683 ) ;
#56523=AXIS2_PLACEMENT_3D ( 'NONE', #3341, #72823, #44203 ) ;
#56528=CARTESIAN_POINT ( 'NONE',  ( 101.6176986403717279, -43.71793944654686470, 228.4815833058969758 ) ) ;
#56530=PLANE ( 'NONE',  #66665 ) ;
#56531=ORIENTED_EDGE ( 'NONE', *, *, #55474, .F. ) ;
#56532=FACE_OUTER_BOUND ( 'NONE', #22503, .T. ) ;
#56535=ORIENTED_EDGE ( 'NONE', *, *, #89360, .T. ) ;
#56537=ORIENTED_EDGE ( 'NONE', *, *, #19737, .T. ) ;
#56538=CARTESIAN_POINT ( 'NONE',  ( 180.1667039024477504, -28.27351298636767041, 117.4678068554150627 ) ) ;
#56539=ORIENTED_EDGE ( 'NONE', *, *, #474, .T. ) ;
#56541=EDGE_CURVE ( 'NONE', #48789, #43538, #87688, .T. ) ;
#56543=CARTESIAN_POINT ( 'NONE',  ( 108.7463670854851756, -45.85490172528324138, 275.5395189410199919 ) ) ;
#56544=AXIS2_PLACEMENT_3D ( 'NONE', #53156, #72751, #30962 ) ;
#56545=CARTESIAN_POINT ( 'NONE',  ( 97.36144725414590084, -42.06870896796115034, 176.7146728949589658 ) ) ;
#56546=EDGE_CURVE ( 'NONE', #70798, #77857, #60106, .T. ) ;
#56547=CARTESIAN_POINT ( 'NONE',  ( 99.70004787478420383, -45.98060041612311721, 122.0413395616249659 ) ) ;
#56548=DIRECTION ( 'NONE',  ( 0.000000000000000000, 0.000000000000000000, 1.000000000000000000 ) ) ;
#56549=DIRECTION ( 'NONE',  ( 0.000000000000000000, 0.000000000000000000, -1.000000000000000000 ) ) ;
#56551=CARTESIAN_POINT ( 'NONE',  ( 109.3368649739139187, -26.55458330520283994, 220.9013395616249795 ) ) ;
#56552=LINE ( 'NONE', #89756, #8017 ) ;
#56553=CARTESIAN_POINT ( 'NONE',  ( 88.17226027475679473, -14.72944715994100484, 239.5838068554175777 ) ) ;
#56555=DIRECTION ( 'NONE',  ( -4.237773401492740281E-14, 1.000000000000000000, 0.000000000000000000 ) ) ;
#56560=DIRECTION ( 'NONE',  ( 0.000000000000000000, 0.000000000000000000, -1.000000000000000000 ) ) ;
#56561=CARTESIAN_POINT ( 'NONE',  ( 103.3256077877525030, -27.45548614628576445, 136.3815795745832133 ) ) ;
#56563=ORIENTED_EDGE ( 'NONE', *, *, #69276, .F. ) ;
#56564=CARTESIAN_POINT ( 'NONE',  ( 96.02763272632168423, -37.29765984735794859, 121.3794347997209684 ) ) ;
#56566=CARTESIAN_POINT ( 'NONE',  ( 136.5456844410060455, -35.53793914063654569, 7.103892432653868383 ) ) ;
#56567=CYLINDRICAL_SURFACE ( 'NONE', #81934, 1.000000000000000888 ) ;
#56569=CARTESIAN_POINT ( 'NONE',  ( 99.75293322724810707, -43.56396968085568489, 56.92422635920629403 ) ) ;
#56570=CARTESIAN_POINT ( 'NONE',  ( 116.9047011640239759, -41.71676023082950735, 244.4651490854349731 ) ) ;
#56572=CARTESIAN_POINT ( 'NONE',  ( 182.0667039024478413, -32.29483332967958376, 193.9678068554150059 ) ) ;
#56574=DIRECTION ( 'NONE',  ( 0.000000000000000000, 0.000000000000000000, -1.000000000000000000 ) ) ;
#56576=LINE ( 'NONE', #84318, #44478 ) ;
#56577=DIRECTION ( 'NONE',  ( 1.000000000000000000, 4.299999999999999979E-14, 1.000000000000000078E-15 ) ) ;
#56578=CARTESIAN_POINT ( 'NONE',  ( 115.3585040474263508, -45.26590950091470233, 268.1899109901965517 ) ) ;
#56580=CARTESIAN_POINT ( 'NONE',  ( 134.0664832912740110, 0.2215528400590013880, 293.6356252759119911 ) ) ;
#56581=CARTESIAN_POINT ( 'NONE',  ( 114.1902268275144507, -45.21166270573645107, 148.1203871806719405 ) ) ;
#56582=CARTESIAN_POINT ( 'NONE',  ( 109.6119375470732109, -25.15554210634138954, 25.90419670448196143 ) ) ;
#56583=CARTESIAN_POINT ( 'NONE',  ( 117.8211145215647946, -31.63542911875440211, 210.1784824187679703 ) ) ;
#56584=CARTESIAN_POINT ( 'NONE',  ( 108.4174891635765619, -26.73503591423436276, 30.96895861629700519 ) ) ;
#56585=DIRECTION ( 'NONE',  ( -1.000000000000000078E-15, 1.000000000000000083E-30, 1.000000000000000000 ) ) ;
#56586=CIRCLE ( 'NONE', #30469, 4.750000000000000888 ) ;
#56587=DIRECTION ( 'NONE',  ( 0.1811243268507098381, -0.9834602067307437467, 0.000000000000000000 ) ) ;
#56589=CARTESIAN_POINT ( 'NONE',  ( 41.56648329127398966, -18.82844715994071194, 258.9256252759120116 ) ) ;
#56591=ORIENTED_EDGE ( 'NONE', *, *, #8757, .F. ) ;
#56592=CARTESIAN_POINT ( 'NONE',  ( 165.3359832912740046, -36.32844715994100682, -5.074374724088000832 ) ) ;
#56593=( BOUNDED_CURVE ( )  B_SPLINE_CURVE ( 3, ( #68190, #54966, #14576, #484 ),
 .UNSPECIFIED., .F., .T. ) 
 B_SPLINE_CURVE_WITH_KNOTS ( ( 4, 4 ),
 ( 1.570796326790817377, 3.141592653586014805 ),
 .UNSPECIFIED. ) 
 CURVE ( )  GEOMETRIC_REPRESENTATION_ITEM ( )  RATIONAL_B_SPLINE_CURVE ( ( 1.000000000000000000, 0.8047378541242942163, 0.8047378541242942163, 1.000000000000000000 ) ) 
 REPRESENTATION_ITEM ( '' )  );
#56594=VERTEX_POINT ( 'NONE', #61378 ) ;
#56596=AXIS2_PLACEMENT_3D ( 'NONE', #29043, #61745, #83122 ) ;
#56597=CARTESIAN_POINT ( 'NONE',  ( 107.0664832912739399, -36.72944715994095333, 290.1356252759106837 ) ) ;
#56599=CARTESIAN_POINT ( 'NONE',  ( 110.7866772467784955, -46.44483816919306207, 58.86705384733998159 ) ) ;
#56600=DIRECTION ( 'NONE',  ( 1.000000000000000000, 4.299999999999999979E-14, 1.000000000000000078E-15 ) ) ;
#56601=VECTOR ( 'NONE', #83758, 1000.000000000000000 ) ;
#56602=CARTESIAN_POINT ( 'NONE',  ( 121.3042370176062548, -43.34581843340460239, 0.7256252759109850237 ) ) ;
#56603=CARTESIAN_POINT ( 'NONE',  ( 108.6817352505430705, -26.38614300430984372, 185.9527681330539792 ) ) ;
#56605=CARTESIAN_POINT ( 'NONE',  ( 111.6523633261645188, -43.93540552976629243, 262.4495626852196892 ) ) ;
#56607=EDGE_LOOP ( 'NONE', ( #23935, #30900, #46883, #83354 ) ) ;
#56608=VERTEX_POINT ( 'NONE', #74566 ) ;
#56610=DIRECTION ( 'NONE',  ( -0.0001713722456129692653, 0.9999999853157764962, 0.000000000000000000 ) ) ;
#56611=CARTESIAN_POINT ( 'NONE',  ( 48.16670390244701139, -26.71338133339251542, -5.074374724088000832 ) ) ;
#56613=CARTESIAN_POINT ( 'NONE',  ( 113.2466443085970553, -28.75955056167441271, 19.55182030042092478 ) ) ;
#56619=CARTESIAN_POINT ( 'NONE',  ( 96.68076663292303863, -33.01451620012163346, 26.06514908543494613 ) ) ;
#56621=ORIENTED_EDGE ( 'NONE', *, *, #61535, .T. ) ;
#56624=DIRECTION ( 'NONE',  ( -0.000000000000000000, -0.000000000000000000, 1.000000000000000000 ) ) ;
#56625=CARTESIAN_POINT ( 'NONE',  ( 112.5126453671185942, -30.64922967528412556, 112.3138046553059723 ) ) ;
#56626=EDGE_CURVE ( 'NONE', #810, #15908, #12349, .T. ) ;
#56628=DIRECTION ( 'NONE',  ( 0.000000000000000000, 0.000000000000000000, -1.000000000000000000 ) ) ;
#56629=ORIENTED_EDGE ( 'NONE', *, *, #25475, .T. ) ;
#56631=CARTESIAN_POINT ( 'NONE',  ( 115.7833298848688344, -41.80193538969286493, 138.4043975589790705 ) ) ;
#56632=AXIS2_PLACEMENT_3D ( 'NONE', #59151, #86879, #24641 ) ;
#56635=CARTESIAN_POINT ( 'NONE',  ( 105.9222987080832752, -26.72137021301569959, 156.5987261630399701 ) ) ;
#56638=CARTESIAN_POINT ( 'NONE',  ( 117.3853494549534844, -38.35986426902426416, 109.7013395616249767 ) ) ;
#56639=DIRECTION ( 'NONE',  ( 0.9834602067019604377, 0.1811243270069963496, 0.000000000000000000 ) ) ;
#56640=ORIENTED_EDGE ( 'NONE', *, *, #13742, .F. ) ;
#56641=EDGE_LOOP ( 'NONE', ( #62808, #52964, #7954, #72074 ) ) ;
#56642=ORIENTED_EDGE ( 'NONE', *, *, #42381, .T. ) ;
#56643=ADVANCED_FACE ( 'NONE', ( #5994 ), #6424, .F. ) ;
#56644=FACE_OUTER_BOUND ( 'NONE', #37436, .T. ) ;
#56647=CARTESIAN_POINT ( 'NONE',  ( 116.4547782460827250, -32.24742764444978604, 19.18133956162493092 ) ) ;
#56648=CARTESIAN_POINT ( 'NONE',  ( 98.14969091592392658, -31.28627964566590336, 166.8899109901969950 ) ) ;
#56649=PLANE ( 'NONE',  #3108 ) ;
#56650=DIRECTION ( 'NONE',  ( 0.000000000000000000, -1.000000000000000000, 0.000000000000000000 ) ) ;
#56652=CARTESIAN_POINT ( 'NONE',  ( 117.6079501356808947, -33.40507394795707796, 125.0575300378149706 ) ) ;
#56653=VECTOR ( 'NONE', #26566, 1000.000000000000000 ) ;
#56654=DIRECTION ( 'NONE',  ( 1.000000000000000078E-15, 1.000000000000000083E-30, -1.000000000000000000 ) ) ;
#56655=ORIENTED_EDGE ( 'NONE', *, *, #14348, .T. ) ;
#56656=CARTESIAN_POINT ( 'NONE',  ( 97.70685139758691662, -40.25208905359860267, 116.6132694511275218 ) ) ;
#56657=AXIS2_PLACEMENT_3D ( 'NONE', #86326, #64984, #17288 ) ;
#56658=ADVANCED_FACE ( 'NONE', ( #56348 ), #14595, .F. ) ;
#56659=ORIENTED_EDGE ( 'NONE', *, *, #66675, .F. ) ;
#56660=CARTESIAN_POINT ( 'NONE',  ( 99.08970696490817431, -42.79570318340363855, 132.8446165289294356 ) ) ;
#56663=VECTOR ( 'NONE', #8672, 1000.000000000000000 ) ;
#56664=FACE_OUTER_BOUND ( 'NONE', #17267, .T. ) ;
#56665=CARTESIAN_POINT ( 'NONE',  ( 97.25147018216796369, -38.86936842998233033, 132.4977133313580850 ) ) ;
#56666=CARTESIAN_POINT ( 'NONE',  ( 107.6068636345326155, -48.56787927409158812, 42.61276813305398292 ) ) ;
#56668=CARTESIAN_POINT ( 'NONE',  ( 22.49563609058249725, -67.87844715994100397, 13.84673904354931651 ) ) ;
#56669=LINE ( 'NONE', #83957, #23837 ) ;
#56670=CARTESIAN_POINT ( 'NONE',  ( 110.5640613610538168, -45.86347053068967483, 62.86705384733992474 ) ) ;
#56671=CARTESIAN_POINT ( 'NONE',  ( 97.06386015463802153, -37.34256901384676297, 111.3752599851678298 ) ) ;
#56672=CARTESIAN_POINT ( 'NONE',  ( 98.02603654163385727, -30.41010087969375775, 156.8289586092439549 ) ) ;
#56673=CARTESIAN_POINT ( 'NONE',  ( 109.7248659175985779, -27.00080517866619800, 70.86479194288972394 ) ) ;
#56674=DIRECTION ( 'NONE',  ( 1.000000000000000078E-15, 0.000000000000000000, -1.000000000000000000 ) ) ;
#56677=AXIS2_PLACEMENT_3D ( 'NONE', #41126, #6185, #34317 ) ;
#56679=DIRECTION ( 'NONE',  ( 0.000000000000000000, 0.000000000000000000, -1.000000000000000000 ) ) ;
#56682=DIRECTION ( 'NONE',  ( 1.387778780781444492E-15, 0.000000000000000000, -1.000000000000000000 ) ) ;
#56683=CARTESIAN_POINT ( 'NONE',  ( 97.91784736035330639, -30.44332401329681659, 165.8594347997199634 ) ) ;
#56684=VERTEX_POINT ( 'NONE', #69104 ) ;
#56685=DIRECTION ( 'NONE',  ( 1.000000000000000078E-15, -1.000000000000000083E-30, -1.000000000000000000 ) ) ;
#56686=CARTESIAN_POINT ( 'NONE',  ( 96.16865940696823145, -32.01143006853777706, 207.0013395616249738 ) ) ;
#56687=CARTESIAN_POINT ( 'NONE',  ( 95.43962894333766656, -34.19422119854147013, 102.1556252759109640 ) ) ;
#56690=DIRECTION ( 'NONE',  ( 0.7071067811868696484, 0.7071067811862253860, 7.071067811868689941E-16 ) ) ;
#56695=ORIENTED_EDGE ( 'NONE', *, *, #55124, .T. ) ;
#56696=CONICAL_SURFACE ( 'NONE', #69818, 1.624999999999987566, 1.029744258676650093 ) ;
#56697=VERTEX_POINT ( 'NONE', #83193 ) ;
#56698=CARTESIAN_POINT ( 'NONE',  ( 188.5667039024479834, -62.87844715994099687, 288.3428068554150059 ) ) ;
#56699=CARTESIAN_POINT ( 'NONE',  ( 110.7330907359209107, -26.30208074597294754, 250.8194347997206819 ) ) ;
#56700=DIRECTION ( 'NONE',  ( 1.000000000000000000, -1.581013800890250371E-15, 0.000000000000000000 ) ) ;
#56701=CARTESIAN_POINT ( 'NONE',  ( 134.2548946453563303, -15.97944715994100484, 1.625625275910998147 ) ) ;
#56702=VECTOR ( 'NONE', #87994, 1000.000000000000000 ) ;
#56703=DIRECTION ( 'NONE',  ( -1.000000000000000078E-15, 1.000000000000000083E-30, 1.000000000000000000 ) ) ;
#56704=DIRECTION ( 'NONE',  ( 0.000000000000000000, -1.000000000000000000, 0.000000000000000000 ) ) ;
#56705=DIRECTION ( 'NONE',  ( 0.000000000000000000, 0.000000000000000000, 1.000000000000000000 ) ) ;
#56706=VECTOR ( 'NONE', #80954, 1000.000000000000000 ) ;
#56707=ADVANCED_FACE ( 'NONE', ( #27761 ), #21408, .T. ) ;
#56708=CARTESIAN_POINT ( 'NONE',  ( 114.8359307259106856, -43.71386199060815869, 38.24419670448192221 ) ) ;
#56711=FACE_OUTER_BOUND ( 'NONE', #58462, .T. ) ;
#56712=CARTESIAN_POINT ( 'NONE',  ( 112.1408248370476741, -28.01367038444149316, 15.65874614011077881 ) ) ;
#56713=EDGE_CURVE ( 'NONE', #56395, #31400, #8226, .T. ) ;
#56714=CARTESIAN_POINT ( 'NONE',  ( 116.7892270756567967, -35.66563809766837778, 274.9127681330532482 ) ) ;
#56715=CARTESIAN_POINT ( 'NONE',  ( 181.8764988495246655, -33.54226604284360747, 313.9678068554149490 ) ) ;
#56716=CARTESIAN_POINT ( 'NONE',  ( 103.6907823165633289, -45.90921117331522083, 138.2956252759109645 ) ) ;
#56718=DIRECTION ( 'NONE',  ( 1.000000000000000078E-15, 1.000000000000000083E-30, -1.000000000000000000 ) ) ;
#56721=CARTESIAN_POINT ( 'NONE',  ( 62.03715912545732181, -23.42818131006021432, 237.4678068554150059 ) ) ;
#56722=CARTESIAN_POINT ( 'NONE',  ( 97.81168895331838087, -40.51742574516882200, 287.6356252759109680 ) ) ;
#56723=ORIENTED_EDGE ( 'NONE', *, *, #50555, .T. ) ;
#56726=CARTESIAN_POINT ( 'NONE',  ( 98.69997382787508400, -39.74003663468293013, 263.0330118773257482 ) ) ;
#56729=EDGE_CURVE ( 'NONE', #66807, #83508, #55441, .T. ) ;
#56730=CARTESIAN_POINT ( 'NONE',  ( 98.34976866985373078, -31.65674666536116888, 140.9064732640824502 ) ) ;
#56732=CARTESIAN_POINT ( 'NONE',  ( 105.7995184992940381, -26.72403496457788563, 85.17729194164677153 ) ) ;
#56735=ORIENTED_EDGE ( 'NONE', *, *, #34190, .F. ) ;
#56736=DIRECTION ( 'NONE',  ( 1.000000000000000000, 4.299999999999999979E-14, 1.000000000000000078E-15 ) ) ;
#56737=LINE ( 'NONE', #64906, #36851 ) ;
#56738=ORIENTED_EDGE ( 'NONE', *, *, #42269, .F. ) ;
#56739=CARTESIAN_POINT ( 'NONE',  ( 109.7701363090614990, -47.44715903388583200, 92.78514908543495210 ) ) ;
#56740=ORIENTED_EDGE ( 'NONE', *, *, #24898, .T. ) ;
#56741=CARTESIAN_POINT ( 'NONE',  ( 115.0166753900997065, -32.39272993814809354, 23.63432458998199337 ) ) ;
#56742=AXIS2_PLACEMENT_3D ( 'NONE', #38462, #44832, #52074 ) ;
#56744=CARTESIAN_POINT ( 'NONE',  ( 123.0664832912750057, -36.72944715993921960, 0.7256252759109869110 ) ) ;
#56745=CARTESIAN_POINT ( 'NONE',  ( 102.9544237342423969, -27.85507949283293527, 180.4213395616259845 ) ) ;
#56746=DIRECTION ( 'NONE',  ( 3.999999999999999995E-14, -1.000000000000000000, 4.100000000000000342E-29 ) ) ;
#56747=CARTESIAN_POINT ( 'NONE',  ( 107.0664832912739968, -36.72944715994100306, 293.2242906452868851 ) ) ;
#56750=CARTESIAN_POINT ( 'NONE',  ( 105.7709788128635182, -26.34124963128569163, 266.1756252759109884 ) ) ;
#56755=CARTESIAN_POINT ( 'NONE',  ( 104.9540660161283370, -25.01839229886434524, 121.2184824187679766 ) ) ;
#56757=ORIENTED_EDGE ( 'NONE', *, *, #25900, .T. ) ;
#56761=FACE_OUTER_BOUND ( 'NONE', #14870, .T. ) ;
#56762=FACE_OUTER_BOUND ( 'NONE', #79304, .T. ) ;
#56763=CARTESIAN_POINT ( 'NONE',  ( 177.4809174648213741, -48.32844715993478957, 249.9678068554149775 ) ) ;
#56764=DIRECTION ( 'NONE',  ( -0.7071067811607679721, 0.7071067812123270624, 0.000000000000000000 ) ) ;
#56765=ADVANCED_FACE ( 'NONE', ( #24865 ), #38050, .F. ) ;
#56766=CARTESIAN_POINT ( 'NONE',  ( 116.1584918543541960, -31.54133664852386332, 285.2384824187680579 ) ) ;
#56767=DIRECTION ( 'NONE',  ( -0.7071067811862239427, -0.7071067811868709807, 0.000000000000000000 ) ) ;
#56768=ORIENTED_EDGE ( 'NONE', *, *, #54589, .T. ) ;
#56770=DIRECTION ( 'NONE',  ( 0.7071067811865779928, -0.7071067811865171526, 7.071067811865786933E-16 ) ) ;
#56772=ORIENTED_EDGE ( 'NONE', *, *, #60762, .T. ) ;
#56773=AXIS2_PLACEMENT_3D ( 'NONE', #78590, #2719, #77676 ) ;
#56775=LINE ( 'NONE', #22732, #78877 ) ;
#56776=DIRECTION ( 'NONE',  ( 0.000000000000000000, 1.000000000000000000, 0.000000000000000000 ) ) ;
#56777=FACE_BOUND ( 'NONE', #13596, .T. ) ;
#56779=CARTESIAN_POINT ( 'NONE',  ( 107.4298862253102698, -45.26314917194000742, 237.0324198280769679 ) ) ;
#56781=CARTESIAN_POINT ( 'NONE',  ( 177.0371591254543375, -48.62818131005480637, 300.4678068554149490 ) ) ;
#56782=CARTESIAN_POINT ( 'NONE',  ( 101.7334424669833339, -26.99437863453528408, 100.4632443235299633 ) ) ;
#56783=EDGE_LOOP ( 'NONE', ( #47506, #10792, #15874, #47278 ) ) ;
#56784=CARTESIAN_POINT ( 'NONE',  ( 131.3881603334746160, -19.35482103166650703, 6.853567712192263350 ) ) ;
#56785=EDGE_CURVE ( 'NONE', #23292, #17303, #52532, .T. ) ;
#56788=CARTESIAN_POINT ( 'NONE',  ( 103.4155122767169388, -27.41960725263014709, 276.3738772456573543 ) ) ;
#56789=ORIENTED_EDGE ( 'NONE', *, *, #25792, .T. ) ;
#56790=CARTESIAN_POINT ( 'NONE',  ( 83.06670390244796920, -64.87844715994098976, 213.1838068554149856 ) ) ;
#56792=CARTESIAN_POINT ( 'NONE',  ( 151.5667039024486087, -48.82844715993590512, 129.9678068554149775 ) ) ;
#56794=AXIS2_PLACEMENT_3D ( 'NONE', #61490, #74245, #75591 ) ;
#56795=DIRECTION ( 'NONE',  ( 0.000000000000000000, 0.000000000000000000, -1.000000000000000000 ) ) ;
#56796=ORIENTED_EDGE ( 'NONE', *, *, #41781, .T. ) ;
#56797=CARTESIAN_POINT ( 'NONE',  ( 117.3932167392688655, -32.72270067050601483, 94.10895860924395606 ) ) ;
#56799=CARTESIAN_POINT ( 'NONE',  ( 116.3268456006857718, -32.93825467094161752, 164.1356252759109680 ) ) ;
#56804=CIRCLE ( 'NONE', #10459, 0.5000000000000004441 ) ;
#56805=DIRECTION ( 'NONE',  ( 1.000000000000000078E-15, -1.000000000000000083E-30, -1.000000000000000000 ) ) ;
#56806=CARTESIAN_POINT ( 'NONE',  ( 80.06648329127399677, -8.729447159940999512, 291.1181252759119502 ) ) ;
#56808=CARTESIAN_POINT ( 'NONE',  ( 117.3853494549534844, -38.35986426902426416, 109.7013395616249767 ) ) ;
#56813=CYLINDRICAL_SURFACE ( 'NONE', #2754, 0.4999999999999994449 ) ;
#56814=CARTESIAN_POINT ( 'NONE',  ( 99.89458030379221043, -28.23347241844150091, 146.6356252759109395 ) ) ;
#56815=DIRECTION ( 'NONE',  ( -0.9254794337955620787, -0.3787978585227822492, 0.000000000000000000 ) ) ;
#56816=ORIENTED_EDGE ( 'NONE', *, *, #12050, .T. ) ;
#56818=CARTESIAN_POINT ( 'NONE',  ( 111.7637953458031745, -46.71243375810358600, 283.9146728949585849 ) ) ;
#56819=FACE_BOUND ( 'NONE', #78854, .T. ) ;
#56820=DIRECTION ( 'NONE',  ( 1.000000000000000078E-15, -1.000000000000000000, 0.000000000000000000 ) ) ;
#56821=DIRECTION ( 'NONE',  ( 0.000000000000000000, 0.000000000000000000, 1.000000000000000000 ) ) ;
#56824=LINE ( 'NONE', #57730, #18163 ) ;
#56825=CARTESIAN_POINT ( 'NONE',  ( 109.8674951572811551, -26.74480306206631397, 219.8708633711499658 ) ) ;
#56826=ORIENTED_EDGE ( 'NONE', *, *, #69689, .T. ) ;
#56827=AXIS2_PLACEMENT_3D ( 'NONE', #12238, #20840, #7218 ) ;
#56829=CARTESIAN_POINT ( 'NONE',  ( 97.07454461617307118, -38.04679588918885713, 147.8615833058969713 ) ) ;
#56831=CARTESIAN_POINT ( 'NONE',  ( 162.9033555647770015, -33.89581943344391135, 193.9678068554150059 ) ) ;
#56832=ADVANCED_FACE ( 'NONE', ( #18040 ), #58915, .F. ) ;
#56833=CARTESIAN_POINT ( 'NONE',  ( 111.4502655538902758, -27.98611278301861560, 275.7070538473389547 ) ) ;
#56835=EDGE_CURVE ( 'NONE', #78594, #628, #44849, .T. ) ;
#56837=EDGE_CURVE ( 'NONE', #944, #32467, #63106, .T. ) ;
#56838=CARTESIAN_POINT ( 'NONE',  ( 107.3428450438784694, -25.27364292152175551, 322.4523926293242653 ) ) ;
#56840=CARTESIAN_POINT ( 'NONE',  ( 97.78482738069629931, -40.45122027033047374, 37.62964898729292429 ) ) ;
#56841=CARTESIAN_POINT ( 'NONE',  ( 110.1310368924891350, -26.13358316477604504, 214.8403871806729342 ) ) ;
#56843=VERTEX_POINT ( 'NONE', #67088 ) ;
#56844=ORIENTED_EDGE ( 'NONE', *, *, #73147, .T. ) ;
#56846=VECTOR ( 'NONE', #10273, 1000.000000000000000 ) ;
#56847=EDGE_CURVE ( 'NONE', #65495, #74787, #38930, .T. ) ;
#56851=DIRECTION ( 'NONE',  ( 0.000000000000000000, 0.000000000000000000, -1.000000000000000000 ) ) ;
#56852=AXIS2_PLACEMENT_3D ( 'NONE', #36726, #23114, #21759 ) ;
#56853=ADVANCED_FACE ( 'NONE', ( #4866 ), #52972, .F. ) ;
#56854=CARTESIAN_POINT ( 'NONE',  ( 116.1702204287673794, -31.76348745224625958, 20.21181575210096071 ) ) ;
#56855=LINE ( 'NONE', #49132, #71688 ) ;
#56857=VECTOR ( 'NONE', #26173, 1000.000000000000000 ) ;
#56858=CARTESIAN_POINT ( 'NONE',  ( 112.2188834189205409, -26.89723471487287654, 10.68038718067299087 ) ) ;
#56861=CARTESIAN_POINT ( 'NONE',  ( 100.7500417190893245, -45.80037066963202363, 237.0803871806729717 ) ) ;
#56862=ORIENTED_EDGE ( 'NONE', *, *, #35417, .F. ) ;
#56864=CARTESIAN_POINT ( 'NONE',  ( 77.42411991178801145, -37.49143581486279686, 6.902478035881912000 ) ) ;
#56866=DIRECTION ( 'NONE',  ( 0.000000000000000000, 0.000000000000000000, -1.000000000000000000 ) ) ;
#56867=CIRCLE ( 'NONE', #78638, 5.599999999999994316 ) ;
#56869=CARTESIAN_POINT ( 'NONE',  ( 115.3104451506078192, -40.98773602117310588, 91.26523322673496352 ) ) ;
#56870=CARTESIAN_POINT ( 'NONE',  ( 117.2182995153958132, -34.26411022451439692, 205.0156252759109634 ) ) ;
#56871=CARTESIAN_POINT ( 'NONE',  ( 107.0620278373210255, -36.73691869758540207, 361.9756252759100903 ) ) ;
#56873=DIRECTION ( 'NONE',  ( 0.9242245927363033076, 0.3818493186865917766, 0.000000000000000000 ) ) ;
#56874=ORIENTED_EDGE ( 'NONE', *, *, #12315, .T. ) ;
#56876=CARTESIAN_POINT ( 'NONE',  ( 51.34673845256598668, -36.02818131005800950, -5.074374724088000832 ) ) ;
#56879=CARTESIAN_POINT ( 'NONE',  ( 116.8163745243374194, -34.15002972185388330, 170.0315280845597670 ) ) ;
#56880=CARTESIAN_POINT ( 'NONE',  ( 103.2785698053728396, -27.47462617712415422, 41.38562054109723221 ) ) ;
#56881=CARTESIAN_POINT ( 'NONE',  ( 113.2121186763659040, -42.70299450126940144, 97.63527697093398672 ) ) ;
#56882=CARTESIAN_POINT ( 'NONE',  ( 111.0013748985821422, -46.40740010236051916, 282.8841967044824628 ) ) ;
#56884=EDGE_CURVE ( 'NONE', #51252, #45127, #61602, .T. ) ;
#56885=LINE ( 'NONE', #70993, #13681 ) ;
#56887=ORIENTED_EDGE ( 'NONE', *, *, #44249, .T. ) ;
#56889=ORIENTED_EDGE ( 'NONE', *, *, #58090, .T. ) ;
#56891=ADVANCED_FACE ( 'NONE', ( #55663 ), #88894, .T. ) ;
#56895=AXIS2_PLACEMENT_3D ( 'NONE', #63693, #1017, #47463 ) ;
#56896=CARTESIAN_POINT ( 'NONE',  ( 108.9483104351207317, -46.92736419409159510, 127.7337205140069472 ) ) ;
#56898=CARTESIAN_POINT ( 'NONE',  ( 96.59774800590200527, -36.61877842429220209, 111.3184824187679567 ) ) ;
#56900=ORIENTED_EDGE ( 'NONE', *, *, #74749, .F. ) ;
#56902=CARTESIAN_POINT ( 'NONE',  ( 115.9600293333739387, -30.16561243848903828, 259.3203871806730945 ) ) ;
#56903=DIRECTION ( 'NONE',  ( -1.000000000000000000, -5.512527431108013646E-15, 0.000000000000000000 ) ) ;
#56906=CARTESIAN_POINT ( 'NONE',  ( 99.63728152159639251, -43.45851683074288019, 27.91285964145581033 ) ) ;
#56909=CARTESIAN_POINT ( 'NONE',  ( 105.1452543958526178, -25.43249337517275066, 322.4561491387724459 ) ) ;
#56911=CARTESIAN_POINT ( 'NONE',  ( 132.2601441849014918, -38.80290789369895066, 7.687431601935594827 ) ) ;
#56913=CARTESIAN_POINT ( 'NONE',  ( 163.2569089553700223, -33.54226604285010893, -5.074374724088000832 ) ) ;
#56914=DIRECTION ( 'NONE',  ( -0.9254794337955620787, -0.3787978585227822492, 0.000000000000000000 ) ) ;
#56915=AXIS2_PLACEMENT_3D ( 'NONE', #47345, #12861, #75073 ) ;
#56916=CARTESIAN_POINT ( 'NONE',  ( 41.56648329127399677, -18.82844715994099971, 318.9256252759120116 ) ) ;
#56919=CARTESIAN_POINT ( 'NONE',  ( 118.6786315247609167, -39.21782601141705271, 258.6584824187679033 ) ) ;
#56920=CARTESIAN_POINT ( 'NONE',  ( 98.55127668717894096, -44.97116251829300637, 187.9384824187679612 ) ) ;
#56921=CARTESIAN_POINT ( 'NONE',  ( 111.7933198282062364, -46.77516514641244783, 283.9146728949586418 ) ) ;
#56923=CARTESIAN_POINT ( 'NONE',  ( 100.8874678875339583, -44.70022137742768109, 47.05229194287733208 ) ) ;
#56924=DIRECTION ( 'NONE',  ( 0.000000000000000000, 0.000000000000000000, 1.000000000000000000 ) ) ;
#56925=VECTOR ( 'NONE', #22388, 1000.000000000000000 ) ;
#56926=EDGE_LOOP ( 'NONE', ( #34031, #82201 ) ) ;
#56927=FACE_BOUND ( 'NONE', #3989, .T. ) ;
#56929=VECTOR ( 'NONE', #67970, 1000.000000000000000 ) ;
#56930=CARTESIAN_POINT ( 'NONE',  ( 115.8611420101186269, -34.56920459637935750, 163.4286103042669822 ) ) ;
#56933=CARTESIAN_POINT ( 'NONE',  ( 177.0664832912730162, 12.92155284005730387, 355.9756252759109998 ) ) ;
#56934=CARTESIAN_POINT ( 'NONE',  ( 117.7782040715256926, -34.09831434418946827, 160.0061014663869798 ) ) ;
#56935=CARTESIAN_POINT ( 'NONE',  ( 31.90335556477799628, -33.89581943344391135, 313.9678068554150059 ) ) ;
#56937=CARTESIAN_POINT ( 'NONE',  ( 110.9162716161081477, -27.50018748410121106, 85.76213040958664635 ) ) ;
#56939=DIRECTION ( 'NONE',  ( -0.9254794337955620787, -0.3787978585227822492, 0.000000000000000000 ) ) ;
#56940=CARTESIAN_POINT ( 'NONE',  ( 103.2241971045484092, -45.72390501747114655, 92.25562527591097250 ) ) ;
#56941=VERTEX_POINT ( 'NONE', #40270 ) ;
#56943=CARTESIAN_POINT ( 'NONE',  ( 97.10642131522254772, -35.22350214559244819, 67.63872616303994789 ) ) ;
#56945=CARTESIAN_POINT ( 'NONE',  ( 103.9298229712114363, -26.84510867568836545, 201.3089586092439731 ) ) ;
#56946=CARTESIAN_POINT ( 'NONE',  ( 116.7951252779109552, -39.38782976372972655, 38.61479194470811649 ) ) ;
#56948=CARTESIAN_POINT ( 'NONE',  ( 112.1393427418982611, -28.01282092607783625, 110.6566897338729234 ) ) ;
#56951=EDGE_CURVE ( 'NONE', #51146, #1529, #86338, .T. ) ;
#56952=VECTOR ( 'NONE', #24880, 1000.000000000000000 ) ;
#56954=LINE ( 'NONE', #49691, #60366 ) ;
#56955=CARTESIAN_POINT ( 'NONE',  ( 103.1828028919049558, -27.07824557232541807, 130.3813395616259925 ) ) ;
#56959=ADVANCED_FACE ( 'NONE', ( #74359 ), #6218, .F. ) ;
#56961=DIRECTION ( 'NONE',  ( 1.000000000000000078E-15, -1.000000000000000083E-30, -1.000000000000000000 ) ) ;
#56962=CARTESIAN_POINT ( 'NONE',  ( 62.03742497533659872, -23.42844715994041493, 129.9678068554150911 ) ) ;
#56963=CARTESIAN_POINT ( 'NONE',  ( 112.0659116142514762, -45.48839626539587755, 78.98979194182945207 ) ) ;
#56965=CARTESIAN_POINT ( 'NONE',  ( 111.7322531227442681, -44.01858407219413039, 215.8357094172109782 ) ) ;
#56966=EDGE_CURVE ( 'NONE', #28336, #23638, #19392, .T. ) ;
#56968=DIRECTION ( 'NONE',  ( 1.000000000000000078E-15, -1.000000000000000083E-30, -1.000000000000000000 ) ) ;
#56969=ADVANCED_FACE ( 'NONE', ( #27103 ), #82542, .F. ) ;
#56970=CARTESIAN_POINT ( 'NONE',  ( 112.1201679527454047, -47.44862423305024635, 137.9270538473389820 ) ) ;
#56971=CARTESIAN_POINT ( 'NONE',  ( 20.03715912545826328, -46.82818131006190043, 237.4678068554150059 ) ) ;
#56977=VERTEX_POINT ( 'NONE', #6658 ) ;
#56978=DIRECTION ( 'NONE',  ( 1.000000000000000078E-15, 0.000000000000000000, 1.000000000000000000 ) ) ;
#56980=EDGE_CURVE ( 'NONE', #61833, #51166, #66016, .T. ) ;
#56981=CARTESIAN_POINT ( 'NONE',  ( 98.23953817868523686, -35.94630056370082372, 227.6872975916109567 ) ) ;
#56982=CARTESIAN_POINT ( 'NONE',  ( 117.0718955085710746, -35.46248247742748561, 273.9272919329436036 ) ) ;
#56983=ORIENTED_EDGE ( 'NONE', *, *, #9182, .T. ) ;
#56984=CARTESIAN_POINT ( 'NONE',  ( 114.1129555325863549, -42.16089393588610079, 9.635625275910941312 ) ) ;
#56986=DIRECTION ( 'NONE',  ( 0.000000000000000000, 0.000000000000000000, 1.000000000000000000 ) ) ;
#56989=VECTOR ( 'NONE', #86193, 1000.000000000000000 ) ;
#56990=CARTESIAN_POINT ( 'NONE',  ( 110.8545929532096608, -45.98418784724056252, 112.8856356861517725 ) ) ;
#56991=ORIENTED_EDGE ( 'NONE', *, *, #29044, .F. ) ;
#56993=CONICAL_SURFACE ( 'NONE', #3321, 13.31607168056649115, 0.1047197551196538678 ) ;
#56994=CARTESIAN_POINT ( 'NONE',  ( 101.0114332956932088, -30.54581597779692359, 268.5233284648295466 ) ) ;
#56995=CARTESIAN_POINT ( 'NONE',  ( 95.54500964991285628, -39.60862429916534211, 166.5213395616259788 ) ) ;
#56996=CARTESIAN_POINT ( 'NONE',  ( 112.1095002620001821, -47.42599740258513208, 137.9270538473389820 ) ) ;
#56998=CARTESIAN_POINT ( 'NONE',  ( 102.2372498927960720, -45.96854842739928415, 208.1927681330539599 ) ) ;
#56999=DIRECTION ( 'NONE',  ( 1.000000000000000000, 4.299999999999999979E-14, 1.000000000000000078E-15 ) ) ;
#57001=DIRECTION ( 'NONE',  ( 1.000000000000000000, -6.745093096447288888E-17, 0.000000000000000000 ) ) ;
#57003=EDGE_CURVE ( 'NONE', #69055, #68920, #50064, .T. ) ;
#57005=EDGE_CURVE ( 'NONE', #38670, #48540, #9438, .T. ) ;
#57006=CARTESIAN_POINT ( 'NONE',  ( 108.1864980337677764, -47.13868502929719284, 202.6613395616249704 ) ) ;
#57007=ORIENTED_EDGE ( 'NONE', *, *, #47448, .F. ) ;
#57008=CARTESIAN_POINT ( 'NONE',  ( 113.0770494671172628, -28.21122406429266150, 129.5870538473399449 ) ) ;
#57009=LINE ( 'NONE', #28413, #76169 ) ;
#57011=DIRECTION ( 'NONE',  ( 1.000000000000000078E-15, -1.000000000000000083E-30, -1.000000000000000000 ) ) ;
#57012=CARTESIAN_POINT ( 'NONE',  ( 85.58420390244806697, -51.22944715994107412, 207.5838068554169809 ) ) ;
#57013=CARTESIAN_POINT ( 'NONE',  ( 103.6783103676969233, -46.16071442410667913, 57.30167220430897856 ) ) ;
#57014=CARTESIAN_POINT ( 'NONE',  ( 111.5990003564989479, -46.09347164638224825, 243.9356252759109509 ) ) ;
#57018=AXIS2_PLACEMENT_3D ( 'NONE', #59275, #54225, #40168 ) ;
#57019=DIRECTION ( 'NONE',  ( 0.000000000000000000, 1.000000000000000000, 0.000000000000000000 ) ) ;
#57020=DIRECTION ( 'NONE',  ( 0.000000000000000000, 0.000000000000000000, 1.000000000000000000 ) ) ;
#57021=PLANE ( 'NONE',  #79604 ) ;
#57022=CARTESIAN_POINT ( 'NONE',  ( 111.7936012040045597, -46.77578388097458628, 287.9146728949587555 ) ) ;
#57025=CARTESIAN_POINT ( 'NONE',  ( 108.0089373620841826, -26.32355773090834816, 155.0041967044819557 ) ) ;
#57026=CARTESIAN_POINT ( 'NONE',  ( 104.2140748950419464, -25.22734379144252870, 86.26991099019699050 ) ) ;
#57027=CARTESIAN_POINT ( 'NONE',  ( 106.4811776831737262, -24.84380329649774666, 191.1156252759109861 ) ) ;
#57029=FACE_OUTER_BOUND ( 'NONE', #88560, .T. ) ;
#57030=DIRECTION ( 'NONE',  ( 0.000000000000000000, 0.000000000000000000, -1.000000000000000000 ) ) ;
#57032=CARTESIAN_POINT ( 'NONE',  ( 98.34985892109634165, -31.65658479506688039, 70.90645860791694588 ) ) ;
#57034=VERTEX_POINT ( 'NONE', #12129 ) ;
#57038=ORIENTED_EDGE ( 'NONE', *, *, #43712, .F. ) ;
#57041=ORIENTED_EDGE ( 'NONE', *, *, #45559, .T. ) ;
#57042=CARTESIAN_POINT ( 'NONE',  ( 112.8057071037347185, -27.31004523576153886, 45.62895860924398761 ) ) ;
#57043=DIRECTION ( 'NONE',  ( -1.000000000000000078E-15, 0.000000000000000000, 1.000000000000000000 ) ) ;
#57044=CARTESIAN_POINT ( 'NONE',  ( 76.06670390244796920, -26.72944715994109899, 239.5838068554169809 ) ) ;
#57045=CARTESIAN_POINT ( 'NONE',  ( 103.0329776526464087, -26.38883157761164000, 166.3603871806729444 ) ) ;
#57046=CARTESIAN_POINT ( 'NONE',  ( 116.1125752699382048, -36.30413522796790460, 268.2743245899816884 ) ) ;
#57048=ADVANCED_FACE ( 'NONE', ( #88445 ), #26205, .F. ) ;
#57049=ORIENTED_EDGE ( 'NONE', *, *, #69893, .T. ) ;
#57050=ORIENTED_EDGE ( 'NONE', *, *, #81421, .F. ) ;
#57051=CIRCLE ( 'NONE', #25146, 16.72999999999999332 ) ;
#57053=CARTESIAN_POINT ( 'NONE',  ( 51.42025729302698522, -31.94127993907710206, -5.074374724088000832 ) ) ;
#57054=DIRECTION ( 'NONE',  ( 4.299999999999999979E-14, -1.000000000000000000, 4.400000000000000367E-29 ) ) ;
#57056=CARTESIAN_POINT ( 'NONE',  ( 102.0677952829802706, -27.97006589295626711, 20.48873420085072539 ) ) ;
#57058=EDGE_CURVE ( 'NONE', #72437, #25185, #8458, .T. ) ;
#57059=CARTESIAN_POINT ( 'NONE',  ( 115.8259566582697175, -31.73092551245608561, 50.24009526075410292 ) ) ;
#57061=CARTESIAN_POINT ( 'NONE',  ( 72.26949937496601706, -71.54137415153812185, 394.9756252759101471 ) ) ;
#57063=DIRECTION ( 'NONE',  ( 0.000000000000000000, -1.000000000000000000, 0.000000000000000000 ) ) ;
#57064=CARTESIAN_POINT ( 'NONE',  ( 111.4063510358307667, -46.18429848020807782, 27.91848241876792969 ) ) ;
#57065=ORIENTED_EDGE ( 'NONE', *, *, #80976, .T. ) ;
#57066=EDGE_CURVE ( 'NONE', #87632, #43121, #61665, .T. ) ;
#57067=CARTESIAN_POINT ( 'NONE',  ( 125.9611475301391721, -58.72944715994100306, 239.5838068554164124 ) ) ;
#57069=CARTESIAN_POINT ( 'NONE',  ( 99.63185314732805864, -32.29918761127225224, 128.7290427505439823 ) ) ;
#57071=CARTESIAN_POINT ( 'NONE',  ( 112.1357519924663819, -28.01076024733613679, 94.65678908386330193 ) ) ;
#57072=ADVANCED_FACE ( 'NONE', ( #30240 ), #69785, .T. ) ;
#57073=DIRECTION ( 'NONE',  ( 1.387778780781444492E-15, 0.000000000000000000, -1.000000000000000000 ) ) ;
#57074=VERTEX_POINT ( 'NONE', #14383 ) ;
#57077=VECTOR ( 'NONE', #25540, 1000.000000000000000 ) ;
#57078=ORIENTED_EDGE ( 'NONE', *, *, #5497, .T. ) ;
#57079=VERTEX_POINT ( 'NONE', #57934 ) ;
#57081=CARTESIAN_POINT ( 'NONE',  ( 102.8293847037436421, -28.94642981657014147, 141.9044404487549684 ) ) ;
#57083=CARTESIAN_POINT ( 'NONE',  ( 116.5531001583795216, -32.35436324414348519, 100.1699109901969535 ) ) ;
#57085=CARTESIAN_POINT ( 'NONE',  ( 110.9644701411503718, -45.93855847050220120, 17.89510309453403991 ) ) ;
#57087=ORIENTED_EDGE ( 'NONE', *, *, #24559, .T. ) ;
#57089=CARTESIAN_POINT ( 'NONE',  ( 99.48556355041279176, -43.91805062995148745, 81.92991099019597812 ) ) ;
#57091=CARTESIAN_POINT ( 'NONE',  ( 97.54182784580959265, -34.36413255816223966, 276.1327681330543555 ) ) ;
#57092=CARTESIAN_POINT ( 'NONE',  ( 109.4502800619034417, -25.91266766229690433, 175.8918157521009391 ) ) ;
#57094=FACE_OUTER_BOUND ( 'NONE', #16292, .T. ) ;
#57095=CARTESIAN_POINT ( 'NONE',  ( 107.9456208643995012, -25.71123053419755422, 111.0251490854349754 ) ) ;
#57097=ORIENTED_EDGE ( 'NONE', *, *, #58920, .F. ) ;
#57099=EDGE_LOOP ( 'NONE', ( #50611, #73206, #25271, #53475 ) ) ;
#57100=CARTESIAN_POINT ( 'NONE',  ( 97.83885989710027786, -40.58323732884709045, 132.6416815133410694 ) ) ;
#57102=EDGE_CURVE ( 'NONE', #69894, #51700, #44228, .T. ) ;
#57103=ORIENTED_EDGE ( 'NONE', *, *, #61886, .T. ) ;
#57104=AXIS2_PLACEMENT_3D ( 'NONE', #3305, #1966, #84647 ) ;
#57107=CARTESIAN_POINT ( 'NONE',  ( 115.9452887564414851, -42.19329433630747417, 18.38705384733896153 ) ) ;
#57110=CARTESIAN_POINT ( 'NONE',  ( 172.5667039024478413, -36.32844715993500273, 249.9678068554149775 ) ) ;
#57112=CARTESIAN_POINT ( 'NONE',  ( 115.1932381579440943, -43.17108053757048935, 48.30514908543492680 ) ) ;
#57113=CARTESIAN_POINT ( 'NONE',  ( 97.31316628587843809, -38.96101710005021346, 111.5054712859669053 ) ) ;
#57114=CARTESIAN_POINT ( 'NONE',  ( 108.3633857348901159, -47.68307073960293963, 158.6822919425779617 ) ) ;
#57119=DIRECTION ( 'NONE',  ( 1.000000000000000078E-15, -1.000000000000000083E-30, -1.000000000000000000 ) ) ;
#57121=ORIENTED_EDGE ( 'NONE', *, *, #84378, .T. ) ;
#57124=CARTESIAN_POINT ( 'NONE',  ( 117.4703304800641206, -30.95114626853415984, 179.2299109901959753 ) ) ;
#57126=CARTESIAN_POINT ( 'NONE',  ( 25.56670390244797275, -48.82844715994099971, 254.4678068554150343 ) ) ;
#57127=CARTESIAN_POINT ( 'NONE',  ( 117.2487272683742532, -41.08916198262414099, 209.5165776568640013 ) ) ;
#57128=CARTESIAN_POINT ( 'NONE',  ( 113.3686263934108780, -27.59268128360266914, 85.60800622829195561 ) ) ;
#57129=CARTESIAN_POINT ( 'NONE',  ( 34.33598329127389093, -36.32844715994141893, 117.4678068554150485 ) ) ;
#57130=CARTESIAN_POINT ( 'NONE',  ( 108.4150567101785896, -26.73472737019633172, 190.9689174417968616 ) ) ;
#57134=VECTOR ( 'NONE', #64460, 1000.000000000000000 ) ;
#57138=EDGE_LOOP ( 'NONE', ( #4796, #14992, #82230, #3910 ) ) ;
#57142=CARTESIAN_POINT ( 'NONE',  ( 112.4117637605556297, -46.40425760712833636, 248.9661014663869878 ) ) ;
#57143=DIRECTION ( 'NONE',  ( -0.000000000000000000, -0.000000000000000000, -1.000000000000000000 ) ) ;
#57146=LINE ( 'NONE', #16285, #16316 ) ;
#57147=CARTESIAN_POINT ( 'NONE',  ( 97.81193015299326987, -40.51731617131004271, 31.63594527021773573 ) ) ;
#57149=CARTESIAN_POINT ( 'NONE',  ( 99.11053040751089327, -44.43647348971805400, 41.95086337114900488 ) ) ;
#57150=ORIENTED_EDGE ( 'NONE', *, *, #65706, .F. ) ;
#57151=VERTEX_POINT ( 'NONE', #48862 ) ;
#57152=VERTEX_POINT ( 'NONE', #35246 ) ;
#57154=CARTESIAN_POINT ( 'NONE',  ( 97.70647924652797656, -40.25110015705713096, 17.61264076450902039 ) ) ;
#57155=CARTESIAN_POINT ( 'NONE',  ( 111.5675350091814266, -45.45035926415653194, 268.9556252759110180 ) ) ;
#57156=ADVANCED_FACE ( 'NONE', ( #36618 ), #84331, .F. ) ;
#57157=DIRECTION ( 'NONE',  ( -3.999999999999999995E-14, 1.000000000000000000, -4.100000000000000342E-29 ) ) ;
#57158=CARTESIAN_POINT ( 'NONE',  ( 113.5922197990810645, -29.44396856740777224, 110.4956252759109816 ) ) ;
#57161=CARTESIAN_POINT ( 'NONE',  ( 100.8872389986638041, -44.70003178514691911, 27.05226840473932626 ) ) ;
#57164=EDGE_CURVE ( 'NONE', #61470, #63620, #64319, .T. ) ;
#57165=CARTESIAN_POINT ( 'NONE',  ( 77.48363092588479617, -35.78502016655541951, 2.871594975604034872 ) ) ;
#57169=CARTESIAN_POINT ( 'NONE',  ( 99.26659991834783625, -39.13601125124746716, 19.38237608387593980 ) ) ;
#57171=EDGE_CURVE ( 'NONE', #36108, #60356, #5146, .T. ) ;
#57172=FACE_OUTER_BOUND ( 'NONE', #29047, .T. ) ;
#57174=DIRECTION ( 'NONE',  ( 0.7071067811864656383, 0.7071067811866295072, 7.071067811864962574E-16 ) ) ;
#57176=DIRECTION ( 'NONE',  ( 0.9834602067019598826, 0.1811243270069988198, 0.000000000000000000 ) ) ;
#57178=CARTESIAN_POINT ( 'NONE',  ( 163.0959832912770082, -23.42844715993521021, 313.9678068554149490 ) ) ;
#57179=CARTESIAN_POINT ( 'NONE',  ( 25.56670390244797275, -62.87844715994099687, 257.2178068554150059 ) ) ;
#57181=CARTESIAN_POINT ( 'NONE',  ( 98.72235591169328472, -42.97945265871884857, 66.83848241876793850 ) ) ;
#57182=ORIENTED_EDGE ( 'NONE', *, *, #15852, .F. ) ;
#57183=CARTESIAN_POINT ( 'NONE',  ( 106.6898958108015307, -27.68119582636871456, 39.52003887569599527 ) ) ;
#57185=CARTESIAN_POINT ( 'NONE',  ( 116.6595528204499601, -34.65899032542078118, 183.9956252759109532 ) ) ;
#57187=CARTESIAN_POINT ( 'NONE',  ( 62.03715912545828814, -47.82818131006021645, 237.4678068554150059 ) ) ;
#57190=CARTESIAN_POINT ( 'NONE',  ( 118.1491249375158645, -36.11907637682050165, 269.8822919425776945 ) ) ;
#57191=CARTESIAN_POINT ( 'NONE',  ( 112.4702123878613804, -45.17926194093625014, 118.0310380580964420 ) ) ;
#57193=CARTESIAN_POINT ( 'NONE',  ( 116.3212776292296127, -32.94146857471318413, 287.6356252759109680 ) ) ;
#57195=ORIENTED_EDGE ( 'NONE', *, *, #7117, .F. ) ;
#57196=CARTESIAN_POINT ( 'NONE',  ( 108.5961642634028692, -47.12166094979025388, 138.6927681330539883 ) ) ;
#57198=VECTOR ( 'NONE', #49993, 1000.000000000000000 ) ;
#57202=ORIENTED_EDGE ( 'NONE', *, *, #12257, .T. ) ;
#57203=ORIENTED_EDGE ( 'NONE', *, *, #30644, .F. ) ;
#57209=CARTESIAN_POINT ( 'NONE',  ( 107.0664832912739399, -36.72944715994095333, 311.6343304127839815 ) ) ;
#57210=CARTESIAN_POINT ( 'NONE',  ( 100.5507766775973835, -27.80086676837388637, 26.56610146638793779 ) ) ;
#57211=CYLINDRICAL_SURFACE ( 'NONE', #24716, 3.000000000000002665 ) ;
#57212=VERTEX_POINT ( 'NONE', #59263 ) ;
#57214=PLANE ( 'NONE',  #25854 ) ;
#57215=EDGE_CURVE ( 'NONE', #81490, #78010, #80245, .T. ) ;
#57216=ORIENTED_EDGE ( 'NONE', *, *, #19222, .F. ) ;
#57218=FACE_OUTER_BOUND ( 'NONE', #31225, .T. ) ;
#57219=DIRECTION ( 'NONE',  ( 0.000000000000000000, 0.000000000000000000, -1.000000000000000000 ) ) ;
#57222=FACE_BOUND ( 'NONE', #64926, .T. ) ;
#57223=FACE_OUTER_BOUND ( 'NONE', #35378, .T. ) ;
#57224=CARTESIAN_POINT ( 'NONE',  ( 106.9632158956753756, -45.78494306966059924, 232.0019436376009594 ) ) ;
#57225=DIRECTION ( 'NONE',  ( 0.000000000000000000, 0.000000000000000000, 1.000000000000000000 ) ) ;
#57226=CARTESIAN_POINT ( 'NONE',  ( 110.3650187231686601, -47.25482062520513438, 48.80610146638797175 ) ) ;
#57227=DIRECTION ( 'NONE',  ( 0.000000000000000000, 1.000000000000000000, 0.000000000000000000 ) ) ;
#57228=CARTESIAN_POINT ( 'NONE',  ( 117.3971137516355014, -38.63466851614541753, 88.68133956162493803 ) ) ;
#57230=DIRECTION ( 'NONE',  ( -0.000000000000000000, -0.000000000000000000, -1.000000000000000000 ) ) ;
#57232=CARTESIAN_POINT ( 'NONE',  ( 99.09570904887901577, -30.55043178771423129, 66.80229194605105647 ) ) ;
#57234=ORIENTED_EDGE ( 'NONE', *, *, #65361, .T. ) ;
#57238=LINE ( 'NONE', #84983, #78097 ) ;
#57239=CIRCLE ( 'NONE', #50032, 5.599999999999994316 ) ;
#57240=DIRECTION ( 'NONE',  ( -1.000000000000000078E-15, 1.000000000000000083E-30, 1.000000000000000000 ) ) ;
#57241=ORIENTED_EDGE ( 'NONE', *, *, #33598, .T. ) ;
#57242=EDGE_CURVE ( 'NONE', #70634, #6412, #82077, .T. ) ;
#57243=CARTESIAN_POINT ( 'NONE',  ( 96.63442969565970486, -37.29391305320381633, 76.36991099019697060 ) ) ;
#57245=CIRCLE ( 'NONE', #64454, 3.250000000000002665 ) ;
#57246=CARTESIAN_POINT ( 'NONE',  ( 97.81168895331838087, -40.51742574516882200, 287.6356252759109680 ) ) ;
#57248=DIRECTION ( 'NONE',  ( -1.000000000000000000, 0.000000000000000000, 0.000000000000000000 ) ) ;
#57251=LINE ( 'NONE', #84998, #77382 ) ;
#57253=CARTESIAN_POINT ( 'NONE',  ( 98.43831584450654759, -42.68208710540699258, 122.8070538473389490 ) ) ;
#57255=DIRECTION ( 'NONE',  ( -1.000000000000000078E-15, 1.000000000000000083E-30, 1.000000000000000000 ) ) ;
#57256=CARTESIAN_POINT ( 'NONE',  ( 151.0371591254582597, -46.82818131005593187, 300.4678068554149490 ) ) ;
#57257=AXIS2_PLACEMENT_3D ( 'NONE', #77510, #35712, #83890 ) ;
#57258=ORIENTED_EDGE ( 'NONE', *, *, #63680, .T. ) ;
#57259=CIRCLE ( 'NONE', #35535, 2.517500000000005844 ) ;
#57260=AXIS2_PLACEMENT_3D ( 'NONE', #40638, #87902, #61517 ) ;
#57261=VECTOR ( 'NONE', #11520, 1000.000000000000000 ) ;
#57263=CARTESIAN_POINT ( 'NONE',  ( 116.6595528204498464, -34.65899032542080960, 179.9956252759109532 ) ) ;
#57265=CARTESIAN_POINT ( 'NONE',  ( 71.24076473329810710, 5.642044068322332961, 394.9756252759101471 ) ) ;
#57266=EDGE_LOOP ( 'NONE', ( #8380, #35806, #52094, #89151 ) ) ;
#57268=AXIS2_PLACEMENT_3D ( 'NONE', #44085, #38179, #16408 ) ;
#57269=CARTESIAN_POINT ( 'NONE',  ( 115.8929840288991642, -32.51563116083749350, 15.18133956162492915 ) ) ;
#57270=CARTESIAN_POINT ( 'NONE',  ( 172.5664832912740110, -9.303447159940999356, 136.8086252759119645 ) ) ;
#57271=LINE ( 'NONE', #52112, #31601 ) ;
#57274=DIRECTION ( 'NONE',  ( 0.000000000000000000, 0.000000000000000000, -1.000000000000000000 ) ) ;
#57275=DIRECTION ( 'NONE',  ( 5.512527431108029424E-15, -1.000000000000000000, 0.000000000000000000 ) ) ;
#57276=EDGE_CURVE ( 'NONE', #22553, #50424, #65639, .T. ) ;
#57277=CARTESIAN_POINT ( 'NONE',  ( 100.0046238269856929, -29.91446987444270178, 250.7156252759109520 ) ) ;
#57279=ORIENTED_EDGE ( 'NONE', *, *, #36483, .T. ) ;
#57280=CARTESIAN_POINT ( 'NONE',  ( 98.85146132857330770, -40.05235142642286661, 203.0644404487539703 ) ) ;
#57281=DIRECTION ( 'NONE',  ( -0.9834602067153815907, -0.1811243269341220596, 0.000000000000000000 ) ) ;
#57282=CARTESIAN_POINT ( 'NONE',  ( 111.1996377132626748, -28.89074107182586815, 56.12158330589694799 ) ) ;
#57284=CARTESIAN_POINT ( 'NONE',  ( 99.04399467038047078, -42.84115622384206290, 266.8440302632771477 ) ) ;
#57285=EDGE_CURVE ( 'NONE', #58867, #30864, #89678, .T. ) ;
#57288=DIRECTION ( 'NONE',  ( 1.000000000000000000, 3.999999999999999995E-14, 1.000000000000000078E-15 ) ) ;
#57289=CARTESIAN_POINT ( 'NONE',  ( 123.6837132603321692, -53.34645651782491882, 249.5838068554164693 ) ) ;
#57290=EDGE_CURVE ( 'NONE', #64042, #17117, #25275, .T. ) ;
#57291=CARTESIAN_POINT ( 'NONE',  ( 96.54020141486694229, -31.34005042439572009, 245.9499109901969689 ) ) ;
#57292=CARTESIAN_POINT ( 'NONE',  ( 91.06648329127389729, -36.72944715993924802, 13.92562527591095467 ) ) ;
#57293=VERTEX_POINT ( 'NONE', #74690 ) ;
#57294=VERTEX_POINT ( 'NONE', #39709 ) ;
#57295=CARTESIAN_POINT ( 'NONE',  ( 115.0372575007767466, -42.90846257426783694, 88.30229194183291952 ) ) ;
#57297=CARTESIAN_POINT ( 'NONE',  ( 98.38028489613425620, -41.69503615009242736, 122.7390885072009468 ) ) ;
#57298=CARTESIAN_POINT ( 'NONE',  ( 177.8371591254545478, -47.82818131005477369, 129.9678068554150059 ) ) ;
#57299=CARTESIAN_POINT ( 'NONE',  ( 111.1466539572837320, -45.61852150024213870, 23.91848241876692782 ) ) ;
#57302=CARTESIAN_POINT ( 'NONE',  ( 115.0558824863888390, -43.54908903376227158, 59.26419670448196086 ) ) ;
#57306=CARTESIAN_POINT ( 'NONE',  ( 110.2909773106953111, -46.66674596437654543, 12.82705384733995402 ) ) ;
#57307=ORIENTED_EDGE ( 'NONE', *, *, #44117, .F. ) ;
#57308=DIRECTION ( 'NONE',  ( 0.7071067811989762975, -0.7071067811741188480, 7.071067811989771216E-16 ) ) ;
#57309=CARTESIAN_POINT ( 'NONE',  ( 194.5667039024479834, -48.82844715994099971, 310.9178068554150514 ) ) ;
#57310=LINE ( 'NONE', #72306, #87207 ) ;
#57311=CARTESIAN_POINT ( 'NONE',  ( 98.42009728606723229, -37.10485906011713553, 114.1671379886389559 ) ) ;
#57312=CARTESIAN_POINT ( 'NONE',  ( 113.6994007951720107, -45.60016365472323230, 184.0994347997199725 ) ) ;
#57313=FACE_OUTER_BOUND ( 'NONE', #49769, .T. ) ;
#57315=CARTESIAN_POINT ( 'NONE',  ( 48.45959712127301344, -26.00627455219131789, -5.074374724088000832 ) ) ;
#57316=ORIENTED_EDGE ( 'NONE', *, *, #88370, .T. ) ;
#57322=ORIENTED_EDGE ( 'NONE', *, *, #37105, .F. ) ;
#57323=ORIENTED_EDGE ( 'NONE', *, *, #45006, .T. ) ;
#57324=DIRECTION ( 'NONE',  ( 0.000000000000000000, -1.000000000000000000, 0.000000000000000000 ) ) ;
#57325=CIRCLE ( 'NONE', #70452, 4.750000000000004441 ) ;
#57327=CARTESIAN_POINT ( 'NONE',  ( 103.4331722345071682, -27.41248267999953114, 41.37236127975815236 ) ) ;
#57328=CARTESIAN_POINT ( 'NONE',  ( 102.9824767429641525, -29.22764064321736299, 144.8952769709339634 ) ) ;
#57329=AXIS2_PLACEMENT_3D ( 'NONE', #89343, #33908, #34804 ) ;
#57330=CARTESIAN_POINT ( 'NONE',  ( 105.7736212422599777, -26.36243834887274673, 270.1756252759109884 ) ) ;
#57331=CARTESIAN_POINT ( 'NONE',  ( 172.5667039024478129, -36.32844715993500273, 300.4678068554149490 ) ) ;
#57334=ORIENTED_EDGE ( 'NONE', *, *, #48176, .T. ) ;
#57335=CARTESIAN_POINT ( 'NONE',  ( 45.76696975232824371, -48.62818131006036992, 300.4678068554150059 ) ) ;
#57338=VECTOR ( 'NONE', #30030, 1000.000000000000000 ) ;
#57339=B_SPLINE_CURVE_WITH_KNOTS ( 'NONE', 3,
 ( #8141, #29035, #67908, #32930, #60179, #66559, #82009, #54695, #19764, #33386, #47443, #32478, #46550, #5696, #54243, #74284, #12056, #47890 ),
 .UNSPECIFIED., .F., .F.,
 ( 4, 2, 2, 2, 2, 2, 2, 2, 4 ),
 ( 0.000000000000000000, 0.06249933430492867620, 0.1249986686098573524, 0.1874980029147860217, 0.2499973372197147048, 0.3124966715246433879, 0.3749960058295720433, 0.4374953401345007542, 0.4999946744394294096 ),
 .UNSPECIFIED. ) ;
#57340=CARTESIAN_POINT ( 'NONE',  ( 98.29927950267186532, -42.45157995928803984, 101.7870538473399620 ) ) ;
#57341=CARTESIAN_POINT ( 'NONE',  ( 101.0612956599395602, -45.30524461813642745, 282.0899109901967563 ) ) ;
#57342=ORIENTED_EDGE ( 'NONE', *, *, #74397, .T. ) ;
#57344=EDGE_CURVE ( 'NONE', #47547, #43903, #798, .T. ) ;
#57345=CARTESIAN_POINT ( 'NONE',  ( 96.91416677013903325, -34.20826173260762459, 276.1327681330537871 ) ) ;
#57346=CARTESIAN_POINT ( 'NONE',  ( 83.06670390244796920, -58.72944715994098175, 228.3338068554150198 ) ) ;
#57349=CARTESIAN_POINT ( 'NONE',  ( 97.81943421394399252, -40.53634900077776848, 27.63767384540028971 ) ) ;
#57350=CIRCLE ( 'NONE', #83494, 1.219499999999975159 ) ;
#57351=LINE ( 'NONE', #16930, #37553 ) ;
#57352=DIRECTION ( 'NONE',  ( 0.000000000000000000, 1.000000000000000000, 0.000000000000000000 ) ) ;
#57353=FACE_BOUND ( 'NONE', #48465, .T. ) ;
#57358=EDGE_CURVE ( 'NONE', #85897, #59253, #68332, .T. ) ;
#57361=EDGE_LOOP ( 'NONE', ( #15909, #41228, #13845, #27493 ) ) ;
#57363=DIRECTION ( 'NONE',  ( 1.000000000000000078E-15, 1.000000000000000083E-30, -1.000000000000000000 ) ) ;
#57364=CARTESIAN_POINT ( 'NONE',  ( 112.1386966202503430, -26.85596833298010111, 19.71086337114896736 ) ) ;
#57365=CARTESIAN_POINT ( 'NONE',  ( 102.8440116971490852, -46.26114276377411016, 173.2441967044829596 ) ) ;
#57366=CARTESIAN_POINT ( 'NONE',  ( 112.2081591769286177, -26.91769754996824560, 10.68038718067299087 ) ) ;
#57367=DIRECTION ( 'NONE',  ( -6.524622321627019585E-16, -3.741823817616790462E-31, -1.000000000000000000 ) ) ;
#57368=CARTESIAN_POINT ( 'NONE',  ( 81.60736025277958561, -34.45223222829589815, 7.843813999040315288 ) ) ;
#57369=FACE_OUTER_BOUND ( 'NONE', #31159, .T. ) ;
#57370=CIRCLE ( 'NONE', #18206, 2.117000000000000881 ) ;
#57371=CIRCLE ( 'NONE', #68995, 2.517499999999998739 ) ;
#57372=ADVANCED_FACE ( 'NONE', ( #26994 ), #60599, .F. ) ;
#57373=VERTEX_POINT ( 'NONE', #89230 ) ;
#57375=ORIENTED_EDGE ( 'NONE', *, *, #71259, .F. ) ;
#57376=CARTESIAN_POINT ( 'NONE',  ( 104.9021620152489476, -46.26774620671717031, 68.39848241876694601 ) ) ;
#57377=CYLINDRICAL_SURFACE ( 'NONE', #39898, 4.750000000000004441 ) ;
#57378=EDGE_LOOP ( 'NONE', ( #7969, #62247 ) ) ;
#57379=CARTESIAN_POINT ( 'NONE',  ( 113.1777857331995847, -44.75224829125603776, 49.09390862630768737 ) ) ;
#57380=CARTESIAN_POINT ( 'NONE',  ( 113.6717327907683597, -45.56316108038139845, 184.0994347997199725 ) ) ;
#57381=FACE_OUTER_BOUND ( 'NONE', #36539, .T. ) ;
#57383=CARTESIAN_POINT ( 'NONE',  ( 118.5256205435843526, -36.72944715994100306, 293.2242906452868851 ) ) ;
#57384=EDGE_CURVE ( 'NONE', #6767, #83511, #20629, .T. ) ;
#57385=CARTESIAN_POINT ( 'NONE',  ( 111.9582691220362847, -27.98680779792547213, 85.67040919175906311 ) ) ;
#57387=CARTESIAN_POINT ( 'NONE',  ( 97.81846061703993200, -40.53393429449062069, 96.63704516963355218 ) ) ;
#57388=CARTESIAN_POINT ( 'NONE',  ( 100.1408543393098682, -45.42701269980184975, 122.0413395616259606 ) ) ;
#57390=EDGE_LOOP ( 'NONE', ( #40294, #25853, #77886, #20461, #19650, #51373, #32218, #57438, #47583, #19292, #13446, #15606, #28613, #29680, #50341, #80839, #33360, #423, #75368, #6011, #78973, #64695, #57590, #53173, #8729, #70175, #45861, #71004, #48915, #55873, #86059, #35983, #63523, #78521, #84621, #46634, #40099, #131, #55681, #76024, #31448, #72531, #82212, #22600, #50765, #81805, #33657, #25028 ) ) ;
#57392=CARTESIAN_POINT ( 'NONE',  ( 110.2353755222631833, -45.00509823041481638, 59.29872616303999422 ) ) ;
#57394=CARTESIAN_POINT ( 'NONE',  ( 126.8164832912740110, -36.72944715994101017, -4.824374724089010691 ) ) ;
#57395=AXIS2_PLACEMENT_3D ( 'NONE', #3338, #51896, #59173 ) ;
#57396=CARTESIAN_POINT ( 'NONE',  ( 96.02263050233435138, -38.01213896886783061, 232.4184824187679794 ) ) ;
#57397=CARTESIAN_POINT ( 'NONE',  ( 181.9790560690337031, -31.62489322947608628, 313.9678068554149490 ) ) ;
#57399=DIRECTION ( 'NONE',  ( 0.000000000000000000, 0.000000000000000000, 1.000000000000000000 ) ) ;
#57400=CARTESIAN_POINT ( 'NONE',  ( 107.0664832912739257, -50.72944715994095333, 311.6343304127839815 ) ) ;
#57402=DIRECTION ( 'NONE',  ( -0.7071067811874389708, 0.7071067811856560636, 0.000000000000000000 ) ) ;
#57404=EDGE_CURVE ( 'NONE', #80932, #88430, #82426, .T. ) ;
#57405=CARTESIAN_POINT ( 'NONE',  ( 98.29923130492881000, -31.06375673945261440, 145.8699109901969848 ) ) ;
#57406=EDGE_LOOP ( 'NONE', ( #74975, #5365 ) ) ;
#57407=ORIENTED_EDGE ( 'NONE', *, *, #52348, .T. ) ;
#57408=ORIENTED_EDGE ( 'NONE', *, *, #65264, .T. ) ;
#57410=VECTOR ( 'NONE', #87340, 1000.000000000000000 ) ;
#57411=FACE_OUTER_BOUND ( 'NONE', #33529, .T. ) ;
#57413=EDGE_CURVE ( 'NONE', #26158, #75304, #31069, .T. ) ;
#57414=CARTESIAN_POINT ( 'NONE',  ( 113.2439442825823761, -28.75748049084303659, 129.5524476564171437 ) ) ;
#57415=CARTESIAN_POINT ( 'NONE',  ( 116.7950883839698690, -39.38797980936810461, 104.6147798141180942 ) ) ;
#57417=CARTESIAN_POINT ( 'NONE',  ( 107.2095755159442376, -27.45176125347251173, 227.8823760838769488 ) ) ;
#57420=CARTESIAN_POINT ( 'NONE',  ( 117.3102356154742836, -34.79226824040635790, 158.9756252759109714 ) ) ;
#57421=CARTESIAN_POINT ( 'NONE',  ( 152.5667039024474718, -23.42844715993585325, 117.4678068554150485 ) ) ;
#57426=ORIENTED_EDGE ( 'NONE', *, *, #45753, .F. ) ;
#57427=ORIENTED_EDGE ( 'NONE', *, *, #60861, .F. ) ;
#57429=CARTESIAN_POINT ( 'NONE',  ( 131.3164832912740110, -36.72944715994100306, 6.749768910606454675 ) ) ;
#57430=CARTESIAN_POINT ( 'NONE',  ( 114.0183221777719638, -41.00747610084435024, 16.20523322673395228 ) ) ;
#57431=DIRECTION ( 'NONE',  ( 0.000000000000000000, 0.000000000000000000, -1.000000000000000000 ) ) ;
#57432=VERTEX_POINT ( 'NONE', #69225 ) ;
#57433=CARTESIAN_POINT ( 'NONE',  ( 112.2391605817208529, -43.63979212946189534, 9.635625275910943088 ) ) ;
#57434=DIRECTION ( 'NONE',  ( 1.000000000000000000, 4.299999999999999979E-14, 1.000000000000000078E-15 ) ) ;
#57435=ORIENTED_EDGE ( 'NONE', *, *, #83826, .T. ) ;
#57436=ORIENTED_EDGE ( 'NONE', *, *, #26180, .F. ) ;
#57437=CARTESIAN_POINT ( 'NONE',  ( 110.9492230250103830, -45.94497800772926155, 112.8937869644549750 ) ) ;
#57438=ORIENTED_EDGE ( 'NONE', *, *, #51509, .F. ) ;
#57441=CARTESIAN_POINT ( 'NONE',  ( 100.5619151801845419, -43.03049977154007166, 41.37337220902998070 ) ) ;
#57442=CARTESIAN_POINT ( 'NONE',  ( 96.72113125116129595, -35.27340624960861959, 181.2156252759109805 ) ) ;
#57443=CARTESIAN_POINT ( 'NONE',  ( 98.47430666977638225, -42.65725675464092603, 126.8070538473389490 ) ) ;
#57444=CARTESIAN_POINT ( 'NONE',  ( 107.0664832912739968, -36.72944715994100306, -2.114374724089040924 ) ) ;
#57445=CARTESIAN_POINT ( 'NONE',  ( 98.83931482081872844, -29.34787013040062931, 231.7565776568629587 ) ) ;
#57448=EDGE_LOOP ( 'NONE', ( #13970, #507, #12270, #45684 ) ) ;
#57451=ORIENTED_EDGE ( 'NONE', *, *, #18355, .T. ) ;
#57452=CONICAL_SURFACE ( 'NONE', #24141, 1.625000000000001332, 1.029744258676650093 ) ;
#57453=B_SPLINE_CURVE_WITH_KNOTS ( 'NONE', 3,
 ( #79432, #24010, #80321, #73480, #53455, #82119, #68917, #73936, #75732, #46656, #80763, #74388, #61193, #41192, #6684, #61632, #26231, #12613 ),
 .UNSPECIFIED., .F., .F.,
 ( 4, 2, 2, 2, 2, 2, 2, 2, 4 ),
 ( 0.000000000000000000, 0.06249676073301599355, 0.1249935214660319871, 0.1874902821990479806, 0.2499870429320639742, 0.3124838036650799955, 0.3749805643980959613, 0.4374773251311119271, 0.4999740858641279484 ),
 .UNSPECIFIED. ) ;
#57455=CIRCLE ( 'NONE', #79209, 13.50000000000000533 ) ;
#57456=CARTESIAN_POINT ( 'NONE',  ( 104.4426401758756100, -26.59425533393106633, 200.2784824187679362 ) ) ;
#57458=VECTOR ( 'NONE', #23254, 1000.000000000000000 ) ;
#57459=ADVANCED_FACE ( 'NONE', ( #87879 ), #53318, .F. ) ;
#57460=CARTESIAN_POINT ( 'NONE',  ( 98.16810232779933187, -31.29751870953477422, 170.8899109901960003 ) ) ;
#57461=DIRECTION ( 'NONE',  ( 1.000000000000000000, 4.163336342344333240E-14, 0.000000000000000000 ) ) ;
#57465=EDGE_CURVE ( 'NONE', #67672, #74946, #74253, .T. ) ;
#57467=CARTESIAN_POINT ( 'NONE',  ( 101.5871053484441120, -45.11049957908544172, 57.11545923762081856 ) ) ;
#57468=CARTESIAN_POINT ( 'NONE',  ( 96.29057984255084079, -34.37493501460200207, 252.1432443235302969 ) ) ;
#57472=ADVANCED_FACE ( 'NONE', ( #5206 ), #12409, .T. ) ;
#57474=FACE_OUTER_BOUND ( 'NONE', #58061, .T. ) ;
#57475=EDGE_CURVE ( 'NONE', #241, #8294, #177, .T. ) ;
#57476=DIRECTION ( 'NONE',  ( 4.299999999999999979E-14, -1.000000000000000000, 4.400000000000000367E-29 ) ) ;
#57477=CARTESIAN_POINT ( 'NONE',  ( 99.76431239122888428, -40.48807882857454388, 195.5838068554172935 ) ) ;
#57479=EDGE_CURVE ( 'NONE', #75220, #74301, #47001, .T. ) ;
#57481=CARTESIAN_POINT ( 'NONE',  ( 107.6542440074338458, -47.14984605634950299, 152.6213395616249500 ) ) ;
#57482=CARTESIAN_POINT ( 'NONE',  ( 113.3423928682155406, -27.63071431045342763, 85.60800622829195561 ) ) ;
#57483=CARTESIAN_POINT ( 'NONE',  ( 101.4018018619443922, -46.27454447023805528, 203.1622919425779514 ) ) ;
#57484=DIRECTION ( 'NONE',  ( 9.351236661543306751E-17, -3.725950533538267725E-29, -1.000000000000000000 ) ) ;
#57485=DIRECTION ( 'NONE',  ( 1.000000000000000078E-15, -1.000000000000000083E-30, -1.000000000000000000 ) ) ;
#57486=AXIS2_PLACEMENT_3D ( 'NONE', #75284, #69368, #42087 ) ;
#57489=CARTESIAN_POINT ( 'NONE',  ( 83.56670390244798341, -34.21194715994108293, 239.5838068554169809 ) ) ;
#57491=ORIENTED_EDGE ( 'NONE', *, *, #74827, .T. ) ;
#57492=EDGE_CURVE ( 'NONE', #15894, #79308, #83306, .T. ) ;
#57495=EDGE_CURVE ( 'NONE', #74639, #41728, #62398, .T. ) ;
#57497=ORIENTED_EDGE ( 'NONE', *, *, #40901, .T. ) ;
#57498=DIRECTION ( 'NONE',  ( 1.000000000000000000, 0.000000000000000000, 0.000000000000000000 ) ) ;
#57500=CARTESIAN_POINT ( 'NONE',  ( 98.85726102317303798, -28.21728661942041683, 111.6870538473389587 ) ) ;
#57502=EDGE_CURVE ( 'NONE', #86684, #58845, #3343, .T. ) ;
#57503=FACE_OUTER_BOUND ( 'NONE', #69648, .T. ) ;
#57505=CARTESIAN_POINT ( 'NONE',  ( 113.6564618781686704, -45.68400828401192371, 33.08133956162595268 ) ) ;
#57506=EDGE_LOOP ( 'NONE', ( #10987, #67424 ) ) ;
#57507=ORIENTED_EDGE ( 'NONE', *, *, #58631, .F. ) ;
#57508=ORIENTED_EDGE ( 'NONE', *, *, #44797, .F. ) ;
#57509=LINE ( 'NONE', #85252, #39879 ) ;
#57510=CARTESIAN_POINT ( 'NONE',  ( 150.5667039024473866, -25.42844715993594562, 249.9678068554149490 ) ) ;
#57511=CYLINDRICAL_SURFACE ( 'NONE', #40464, 9.999999999999998224 ) ;
#57512=FACE_OUTER_BOUND ( 'NONE', #78799, .T. ) ;
#57515=CARTESIAN_POINT ( 'NONE',  ( 151.0371591254573502, -24.42818131005592974, 237.4678068554150059 ) ) ;
#57517=CARTESIAN_POINT ( 'NONE',  ( 105.4244226815142156, -47.00233879195506148, 37.44991099019695469 ) ) ;
#57520=CARTESIAN_POINT ( 'NONE',  ( 97.33784162416169750, -34.07106341398686311, 271.1147918510543491 ) ) ;
#57523=DIRECTION ( 'NONE',  ( -1.000000000000000000, 0.000000000000000000, 0.000000000000000000 ) ) ;
#57524=CARTESIAN_POINT ( 'NONE',  ( 104.0192455041231767, -29.15686055524244935, 128.1995189410199600 ) ) ;
#57525=CONICAL_SURFACE ( 'NONE', #85111, 1.258750000000002922, 1.029744258676650093 ) ;
#57526=CIRCLE ( 'NONE', #64728, 2.029999999999997140 ) ;
#57528=CONICAL_SURFACE ( 'NONE', #5267, 1.624999999999987566, 1.029744258676650093 ) ;
#57529=CARTESIAN_POINT ( 'NONE',  ( 97.80997330134053414, -40.51323221472250680, 96.63526432594667881 ) ) ;
#57530=CARTESIAN_POINT ( 'NONE',  ( 107.0664832912748068, -36.72944715993923381, -4.074374724089028454 ) ) ;
#57532=EDGE_LOOP ( 'NONE', ( #86174, #15107, #8887, #61330 ) ) ;
#57533=CARTESIAN_POINT ( 'NONE',  ( 98.38056611065501045, -41.69552606520213800, 136.7397481390533756 ) ) ;
#57534=ORIENTED_EDGE ( 'NONE', *, *, #64096, .T. ) ;
#57536=CARTESIAN_POINT ( 'NONE',  ( 115.8726827828676704, -31.83848043880258061, 175.6615833058969827 ) ) ;
#57538=VECTOR ( 'NONE', #10089, 1000.000000000000000 ) ;
#57539=CARTESIAN_POINT ( 'NONE',  ( 113.8705839548662908, -44.65670854160515546, 104.1413395616249744 ) ) ;
#57540=CARTESIAN_POINT ( 'NONE',  ( 115.9563521928378691, -41.38085296308364036, 18.44300400888693758 ) ) ;
#57541=ORIENTED_EDGE ( 'NONE', *, *, #30428, .T. ) ;
#57542=ORIENTED_EDGE ( 'NONE', *, *, #21081, .T. ) ;
#57543=EDGE_LOOP ( 'NONE', ( #28127, #52550, #88897, #44367, #53720, #87550, #66097, #26615 ) ) ;
#57544=CARTESIAN_POINT ( 'NONE',  ( 112.2491357751623582, -43.66061143999345262, 185.9176141791149917 ) ) ;
#57545=CARTESIAN_POINT ( 'NONE',  ( 106.6594718829666704, -26.29006472227095870, 85.10705384733896040 ) ) ;
#57546=ORIENTED_EDGE ( 'NONE', *, *, #23387, .T. ) ;
#57547=CARTESIAN_POINT ( 'NONE',  ( 99.14404768239418786, -44.40400490628097430, 41.95086337114900488 ) ) ;
#57548=CARTESIAN_POINT ( 'NONE',  ( 108.6783733978936226, -26.40767070732865562, 185.9527681330539792 ) ) ;
#57549=DIRECTION ( 'NONE',  ( 1.000000000000000000, 0.000000000000000000, 0.000000000000000000 ) ) ;
#57550=DIRECTION ( 'NONE',  ( 0.000000000000000000, 0.000000000000000000, -1.000000000000000000 ) ) ;
#57551=CARTESIAN_POINT ( 'NONE',  ( 97.57126093554219892, -31.07129084365559279, 126.9108633711489915 ) ) ;
#57552=CARTESIAN_POINT ( 'NONE',  ( 99.04406188299498126, -42.84125767153000908, 261.8439586123985237 ) ) ;
#57553=ORIENTED_EDGE ( 'NONE', *, *, #71436, .T. ) ;
#57555=ORIENTED_EDGE ( 'NONE', *, *, #78720, .F. ) ;
#57556=CARTESIAN_POINT ( 'NONE',  ( 46.03715912545432332, -48.62818131006086020, 237.4678068554150059 ) ) ;
#57558=EDGE_CURVE ( 'NONE', #87995, #76720, #75895, .T. ) ;
#57563=CARTESIAN_POINT ( 'NONE',  ( 117.4476241407275978, -37.68806341539836069, 78.75276813305399060 ) ) ;
#57565=ADVANCED_FACE ( 'NONE', ( #58699 ), #59585, .F. ) ;
#57568=EDGE_CURVE ( 'NONE', #74209, #60920, #25084, .T. ) ;
#57569=CARTESIAN_POINT ( 'NONE',  ( 99.56037394151441333, -43.88466257697688633, 36.92038718067297509 ) ) ;
#57571=CARTESIAN_POINT ( 'NONE',  ( 117.6568287320715882, -39.81301747186223139, 134.5889586092439743 ) ) ;
#57572=CARTESIAN_POINT ( 'NONE',  ( 71.06648329127399677, -18.82844715994099971, -5.074374724088000832 ) ) ;
#57575=DIRECTION ( 'NONE',  ( -1.000000000000000000, -4.299999999999999979E-14, 1.230419385187874527E-43 ) ) ;
#57578=ORIENTED_EDGE ( 'NONE', *, *, #13625, .T. ) ;
#57579=EDGE_CURVE ( 'NONE', #16547, #78479, #37385, .T. ) ;
#57580=CARTESIAN_POINT ( 'NONE',  ( 164.9212702847350158, -29.73316016639540749, 342.9256252759119548 ) ) ;
#57581=CARTESIAN_POINT ( 'NONE',  ( 117.4565820116822010, -35.18101482210430930, 218.9441967044829482 ) ) ;
#57584=CYLINDRICAL_SURFACE ( 'NONE', #10315, 2.750000000000002665 ) ;
#57585=CARTESIAN_POINT ( 'NONE',  ( 104.8366293861751330, -26.48703790372925937, 256.2470538473397710 ) ) ;
#57586=CARTESIAN_POINT ( 'NONE',  ( 113.8847749867171046, -44.67324210339663182, 104.1413395616249744 ) ) ;
#57589=DIRECTION ( 'NONE',  ( 1.000000000000000000, 0.000000000000000000, 0.000000000000000000 ) ) ;
#57590=ORIENTED_EDGE ( 'NONE', *, *, #23176, .F. ) ;
#57591=ADVANCED_FACE ( 'NONE', ( #3754 ), #3314, .T. ) ;
#57592=AXIS2_PLACEMENT_3D ( 'NONE', #56913, #84649, #84204 ) ;
#57594=VECTOR ( 'NONE', #31260, 1000.000000000000000 ) ;
#57595=ORIENTED_EDGE ( 'NONE', *, *, #7364, .T. ) ;
#57598=ORIENTED_EDGE ( 'NONE', *, *, #57568, .F. ) ;
#57600=CARTESIAN_POINT ( 'NONE',  ( 116.1393041698827346, -43.00708073170991952, 9.356577656862985037 ) ) ;
#57601=DIRECTION ( 'NONE',  ( 1.000000000000000078E-15, -1.000000000000000000, 0.000000000000000000 ) ) ;
#57602=LINE ( 'NONE', #16727, #39689 ) ;
#57603=EDGE_CURVE ( 'NONE', #67926, #27744, #65883, .T. ) ;
#57604=CIRCLE ( 'NONE', #66286, 4.874999999999990230 ) ;
#57605=DIRECTION ( 'NONE',  ( 1.000000000000000000, 6.831565154159360295E-14, 0.000000000000000000 ) ) ;
#57607=CARTESIAN_POINT ( 'NONE',  ( 141.8164832912740110, -9.833000550534297446, -5.074374724088994704 ) ) ;
#57608=CIRCLE ( 'NONE', #12620, 2.749999999999974687 ) ;
#57609=CARTESIAN_POINT ( 'NONE',  ( 104.4852212567679004, -46.88943973524933995, 47.37848241876796607 ) ) ;
#57610=VERTEX_POINT ( 'NONE', #72358 ) ;
#57611=EDGE_LOOP ( 'NONE', ( #32519, #60924, #73609, #75205 ) ) ;
#57612=EDGE_LOOP ( 'NONE', ( #74399, #3569, #83477, #38328 ) ) ;
#57613=VECTOR ( 'NONE', #81459, 1000.000000000000000 ) ;
#57616=CARTESIAN_POINT ( 'NONE',  ( 115.7455327456632403, -41.23958449135837867, 284.4441967044819535 ) ) ;
#57617=LINE ( 'NONE', #29030, #82090 ) ;
#57618=CARTESIAN_POINT ( 'NONE',  ( 113.6473777113567820, -44.00994186338851932, 129.1613395616249704 ) ) ;
#57619=CARTESIAN_POINT ( 'NONE',  ( 115.0365192675815820, -42.90939908788407564, 28.30219775253060632 ) ) ;
#57621=CARTESIAN_POINT ( 'NONE',  ( 168.0371591254543944, -48.62818131005519717, 249.9678068554149775 ) ) ;
#57622=CARTESIAN_POINT ( 'NONE',  ( 77.85922577376808817, -35.08568546290069179, 2.471387922371498735 ) ) ;
#57623=VERTEX_POINT ( 'NONE', #24640 ) ;
#57624=EDGE_CURVE ( 'NONE', #10976, #16372, #61537, .T. ) ;
#57626=CARTESIAN_POINT ( 'NONE',  ( 101.8980524138101345, -43.06915566006364315, 9.850947512448971821 ) ) ;
#57627=CONICAL_SURFACE ( 'NONE', #18456, 1.258750000000002922, 1.029744258676650093 ) ;
#57628=CARTESIAN_POINT ( 'NONE',  ( 168.5667039024483529, -48.82844715993517326, 300.4678068554149490 ) ) ;
#57630=DIRECTION ( 'NONE',  ( 0.000000000000000000, 0.000000000000000000, -1.000000000000000000 ) ) ;
#57631=ORIENTED_EDGE ( 'NONE', *, *, #86324, .T. ) ;
#57632=CARTESIAN_POINT ( 'NONE',  ( 45.56670390244626390, -48.82844715994099971, 180.4678068554150911 ) ) ;
#57633=PLANE ( 'NONE',  #22337 ) ;
#57635=CARTESIAN_POINT ( 'NONE',  ( 117.9889986865933196, -38.42583888725547325, 68.69181575210198787 ) ) ;
#57637=CARTESIAN_POINT ( 'NONE',  ( 111.7785660440950011, -28.99582275371927764, 49.05146744712496343 ) ) ;
#57638=CARTESIAN_POINT ( 'NONE',  ( 113.1984054845878092, -44.65944206278228279, 89.09955263830856609 ) ) ;
#57639=CARTESIAN_POINT ( 'NONE',  ( 103.2204921605863888, -27.09891563476508836, 175.3908633711489813 ) ) ;
#57640=EDGE_CURVE ( 'NONE', #45127, #28392, #66412, .T. ) ;
#57641=DIRECTION ( 'NONE',  ( 1.000000000000000000, 0.000000000000000000, -0.000000000000000000 ) ) ;
#57642=DIRECTION ( 'NONE',  ( 0.7071067811864661934, 0.7071067811866289521, 7.071067811864654918E-16 ) ) ;
#57643=AXIS2_PLACEMENT_3D ( 'NONE', #81607, #60669, #87950 ) ;
#57645=CARTESIAN_POINT ( 'NONE',  ( 100.1098231460999841, -44.55235322945014076, 262.9984824187678782 ) ) ;
#57647=VERTEX_POINT ( 'NONE', #44178 ) ;
#57648=EDGE_CURVE ( 'NONE', #76973, #82153, #26785, .T. ) ;
#57650=VERTEX_POINT ( 'NONE', #23335 ) ;
#57651=CARTESIAN_POINT ( 'NONE',  ( 114.2698949211017663, -45.17901133753223064, 149.1508633711489722 ) ) ;
#57655=ORIENTED_EDGE ( 'NONE', *, *, #41669, .F. ) ;
#57656=ORIENTED_EDGE ( 'NONE', *, *, #84779, .T. ) ;
#57658=B_SPLINE_CURVE_WITH_KNOTS ( 'NONE', 3,
 ( #76979, #19882, #43780, #57414, #16102, #75296, #14762, #78339, #29720, #658, #85150, #56513, #64243, #15651, #8388, #43331, #36544, #15196, #71517, #71072, #70155, #2017, #7927, #22918, #26682, #9276, #61204, #88927, #8845 ),
 .UNSPECIFIED., .F., .F.,
 ( 4, 2, 2, 2, 2, 2, 2, 2, 2, 2, 1, 1, 1, 1, 1, 2, 4 ),
 ( 0.000000000000000000, 0.06250188046431207067, 0.1250037609286241413, 0.1875056413929362398, 0.2500075218572482827, 0.3125094023215603256, 0.3750112827858724796, 0.4375131632501845225, 0.4687641034823402664, 0.4843895735984181661, 0.4922023086564571992, 0.4961086761854766602, 0.4980618599499865295, 0.4990384518322412699, 0.4995267477733687511, 0.4997708957439324085, 0.5000150437144960103 ),
 .UNSPECIFIED. ) ;
#57659=CARTESIAN_POINT ( 'NONE',  ( 142.8821648370248170, -72.54478064608022692, 540.9756252759101471 ) ) ;
#57660=FACE_OUTER_BOUND ( 'NONE', #26471, .T. ) ;
#57661=CARTESIAN_POINT ( 'NONE',  ( 110.2867295656602664, -27.49400189596543242, 209.8099109901969541 ) ) ;
#57662=DIRECTION ( 'NONE',  ( 0.000000000000000000, 0.000000000000000000, -1.000000000000000000 ) ) ;
#57663=CARTESIAN_POINT ( 'NONE',  ( 80.06648329127399677, -8.350947159940998787, 2.408125275911999097 ) ) ;
#57664=DIRECTION ( 'NONE',  ( 1.000000000000000000, 1.261617073437676668E-15, 9.462128050782575008E-16 ) ) ;
#57665=CARTESIAN_POINT ( 'NONE',  ( 101.3842069476886394, -27.98906827703155642, 21.53562527591096298 ) ) ;
#57666=CARTESIAN_POINT ( 'NONE',  ( 34.33598329127384829, -36.32844715994141893, 193.9678068554150911 ) ) ;
#57670=CIRCLE ( 'NONE', #59145, 2.030000000002079918 ) ;
#57673=EDGE_LOOP ( 'NONE', ( #13187, #63200 ) ) ;
#57674=VECTOR ( 'NONE', #19416, 1000.000000000000000 ) ;
#57675=CARTESIAN_POINT ( 'NONE',  ( 130.3998166246059895, 12.92155284005730387, 355.9756252759109998 ) ) ;
#57677=CARTESIAN_POINT ( 'NONE',  ( 103.6457867198658107, -26.24313906103844474, 210.3394347997209763 ) ) ;
#57678=DIRECTION ( 'NONE',  ( -1.000000000000000000, 1.011922027653136551E-15, 0.000000000000000000 ) ) ;
#57679=EDGE_CURVE ( 'NONE', #47547, #79573, #16498, .T. ) ;
#57680=DIRECTION ( 'NONE',  ( 0.000000000000000000, 1.000000000000000000, 0.000000000000000000 ) ) ;
#57681=DIRECTION ( 'NONE',  ( 0.000000000000000000, 1.000000000000000000, 0.000000000000000000 ) ) ;
#57682=EDGE_CURVE ( 'NONE', #73752, #29169, #58677, .T. ) ;
#57683=CARTESIAN_POINT ( 'NONE',  ( 112.0098809771561577, -44.31729861111978153, 222.4705150661719983 ) ) ;
#57685=CARTESIAN_POINT ( 'NONE',  ( 110.4495079430909357, -47.22796928374258130, 53.83657765686300678 ) ) ;
#57687=CARTESIAN_POINT ( 'NONE',  ( 101.6881215347969345, -27.70586588967184483, 85.50419670448295051 ) ) ;
#57689=CARTESIAN_POINT ( 'NONE',  ( 131.4905132191145753, -19.69637952316714546, 6.988870342668328739 ) ) ;
#57691=EDGE_CURVE ( 'NONE', #54341, #64435, #77570, .T. ) ;
#57693=CARTESIAN_POINT ( 'NONE',  ( 97.07170145856559884, -35.38119765756442092, 277.2191086048737247 ) ) ;
#57694=VERTEX_POINT ( 'NONE', #67767 ) ;
#57695=DIRECTION ( 'NONE',  ( -1.000000000000000000, 0.000000000000000000, 0.000000000000000000 ) ) ;
#57696=EDGE_CURVE ( 'NONE', #53395, #38195, #67307, .T. ) ;
#57698=CARTESIAN_POINT ( 'NONE',  ( 46.03715912545349909, -48.62818131006090283, 117.4678068554150485 ) ) ;
#57700=AXIS2_PLACEMENT_3D ( 'NONE', #83464, #68936, #14436 ) ;
#57701=CARTESIAN_POINT ( 'NONE',  ( 184.5664832912740110, 15.62155284005900491, 328.6381252759109088 ) ) ;
#57702=ORIENTED_EDGE ( 'NONE', *, *, #51808, .T. ) ;
#57703=CARTESIAN_POINT ( 'NONE',  ( 113.4288541212755348, -27.66216098611360152, 84.57753003781698453 ) ) ;
#57705=LINE ( 'NONE', #79513, #47765 ) ;
#57706=DIRECTION ( 'NONE',  ( -0.7071067811865614505, -0.7071067811865336949, 0.000000000000000000 ) ) ;
#57707=DIRECTION ( 'NONE',  ( 1.907762142705490052E-15, 7.167082501179359715E-16, -1.000000000000000000 ) ) ;
#57708=ORIENTED_EDGE ( 'NONE', *, *, #26106, .F. ) ;
#57709=EDGE_CURVE ( 'NONE', #87604, #86462, #41234, .T. ) ;
#57710=CARTESIAN_POINT ( 'NONE',  ( 107.8226678445051192, -26.73166616839828791, 121.0146427918937206 ) ) ;
#57711=CARTESIAN_POINT ( 'NONE',  ( 163.0664832912739826, 22.62155284005901024, 333.4006252759110112 ) ) ;
#57713=AXIS2_PLACEMENT_3D ( 'NONE', #22737, #15016, #84968 ) ;
#57714=PLANE ( 'NONE',  #61003 ) ;
#57715=LINE ( 'NONE', #23233, #8008 ) ;
#57716=DIRECTION ( 'NONE',  ( 0.000000000000000000, 1.000000000000000000, 0.000000000000000000 ) ) ;
#57719=CIRCLE ( 'NONE', #14216, 3.299999999999997158 ) ;
#57720=CARTESIAN_POINT ( 'NONE',  ( 152.5667039024471592, -23.42844715993585325, 180.4678068554149775 ) ) ;
#57721=CARTESIAN_POINT ( 'NONE',  ( 108.2029444874845723, -47.03713394308625340, 153.6518157521009584 ) ) ;
#57722=DIRECTION ( 'NONE',  ( 0.000000000000000000, 1.000000000000000000, 0.000000000000000000 ) ) ;
#57723=ORIENTED_EDGE ( 'NONE', *, *, #41069, .F. ) ;
#57724=VECTOR ( 'NONE', #20335, 1000.000000000000000 ) ;
#57725=CARTESIAN_POINT ( 'NONE',  ( 97.00695478131298444, -39.24785563725447446, 12.53372051400597442 ) ) ;
#57726=CARTESIAN_POINT ( 'NONE',  ( 49.35211078756498893, -35.65087443492551245, -5.074374724088000832 ) ) ;
#57727=CARTESIAN_POINT ( 'NONE',  ( 97.81847533801933992, -40.53397008005389779, 51.63704823906684993 ) ) ;
#57728=CARTESIAN_POINT ( 'NONE',  ( 113.1760415728007558, -44.75355146995899247, 13.09421906058726748 ) ) ;
#57730=CARTESIAN_POINT ( 'NONE',  ( 73.06670390244801183, -58.72944715994110254, 250.9178068554160461 ) ) ;
#57733=CARTESIAN_POINT ( 'NONE',  ( 114.9410966442422648, -29.98191058901448969, 229.4022919425779605 ) ) ;
#57734=ORIENTED_EDGE ( 'NONE', *, *, #64673, .F. ) ;
#57735=ORIENTED_EDGE ( 'NONE', *, *, #8156, .T. ) ;
#57737=CARTESIAN_POINT ( 'NONE',  ( 99.58187507909633496, -41.47380365182278439, 183.2072975916109385 ) ) ;
#57738=CIRCLE ( 'NONE', #18568, 2.517500000000000071 ) ;
#57740=CARTESIAN_POINT ( 'NONE',  ( 98.80858115845356338, -33.43260291865056644, 37.45586902018299469 ) ) ;
#57742=EDGE_CURVE ( 'NONE', #23552, #51283, #20965, .T. ) ;
#57743=LINE ( 'NONE', #31369, #77987 ) ;
#57744=AXIS2_PLACEMENT_3D ( 'NONE', #17344, #87718, #52707 ) ;
#57748=LINE ( 'NONE', #50930, #80750 ) ;
#57749=CARTESIAN_POINT ( 'NONE',  ( 118.0799254396265923, -36.12288750354066735, 273.8822919425776945 ) ) ;
#57750=CARTESIAN_POINT ( 'NONE',  ( 176.7669697523288335, -48.62818131005461453, 180.4678068554150059 ) ) ;
#57751=VERTEX_POINT ( 'NONE', #5557 ) ;
#57752=ORIENTED_EDGE ( 'NONE', *, *, #11007, .T. ) ;
#57756=FACE_BOUND ( 'NONE', #82433, .T. ) ;
#57757=AXIS2_PLACEMENT_3D ( 'NONE', #70962, #8735, #79563 ) ;
#57758=VECTOR ( 'NONE', #43414, 1000.000000000000000 ) ;
#57759=CARTESIAN_POINT ( 'NONE',  ( 116.1300133678978170, -31.69047823903422412, 25.24229194257693365 ) ) ;
#57761=ORIENTED_EDGE ( 'NONE', *, *, #28481, .F. ) ;
#57762=ADVANCED_FACE ( 'NONE', ( #12822 ), #60033, .F. ) ;
#57763=CARTESIAN_POINT ( 'NONE',  ( 99.95113126132085313, -44.40829767532816419, 42.98133956162492098 ) ) ;
#57765=CARTESIAN_POINT ( 'NONE',  ( 101.0865414634836696, -45.26919196907830667, 282.0899109901967563 ) ) ;
#57766=ORIENTED_EDGE ( 'NONE', *, *, #46305, .F. ) ;
#57767=CARTESIAN_POINT ( 'NONE',  ( 82.60038231476900705, -17.66080131299329281, 2.811527311783403427 ) ) ;
#57768=LINE ( 'NONE', #30517, #51483 ) ;
#57770=CARTESIAN_POINT ( 'NONE',  ( 98.47016933319702048, -37.73160053143655546, 84.24904275054394986 ) ) ;
#57771=CARTESIAN_POINT ( 'NONE',  ( 97.07541381888600540, -41.51105113164680915, 212.6937205140059461 ) ) ;
#57773=ORIENTED_EDGE ( 'NONE', *, *, #53371, .F. ) ;
#57778=TOROIDAL_SURFACE ( 'NONE', #18620, 15.69999999999999929, 0.2999999999999999889 ) ;
#57779=FACE_BOUND ( 'NONE', #63823, .T. ) ;
#57780=EDGE_LOOP ( 'NONE', ( #75432, #16824, #81645, #28387 ) ) ;
#57782=CARTESIAN_POINT ( 'NONE',  ( 130.3998166246059895, 12.92155284005730387, 355.9756252759109998 ) ) ;
#57783=CARTESIAN_POINT ( 'NONE',  ( 97.53181966783076007, -39.74887802330798792, 42.57051035864261479 ) ) ;
#57785=CARTESIAN_POINT ( 'NONE',  ( 108.7098619460078481, -45.63517435782368636, 127.1562293518869780 ) ) ;
#57786=CARTESIAN_POINT ( 'NONE',  ( 114.4306803301698778, -27.41265490572180141, 274.5441967044824878 ) ) ;
#57787=VECTOR ( 'NONE', #2358, 1000.000000000000114 ) ;
#57788=EDGE_CURVE ( 'NONE', #58668, #64292, #81861, .T. ) ;
#57790=EDGE_CURVE ( 'NONE', #67149, #70138, #32793, .T. ) ;
#57792=AXIS2_PLACEMENT_3D ( 'NONE', #55135, #6139, #68803 ) ;
#57793=EDGE_CURVE ( 'NONE', #73698, #15487, #34131, .T. ) ;
#57796=VECTOR ( 'NONE', #57695, 1000.000000000000000 ) ;
#57797=CARTESIAN_POINT ( 'NONE',  ( 113.1770345814885701, -44.75280961174332361, 33.09405132221606749 ) ) ;
#57798=CARTESIAN_POINT ( 'NONE',  ( 97.83900096657649215, -40.58357506337067377, 131.6413213018817601 ) ) ;
#57799=CARTESIAN_POINT ( 'NONE',  ( 179.7974245136200011, -36.32844715994040996, -5.074374724088000832 ) ) ;
#57800=ORIENTED_EDGE ( 'NONE', *, *, #28258, .T. ) ;
#57801=CARTESIAN_POINT ( 'NONE',  ( 97.22365000156210613, -40.27127430222545001, 266.6013395616254797 ) ) ;
#57802=CARTESIAN_POINT ( 'NONE',  ( 117.5558648759066926, -37.28717672647940873, 14.78419670448294454 ) ) ;
#57804=CARTESIAN_POINT ( 'NONE',  ( 117.0718954854907139, -35.46248235721044750, 119.9272919425023787 ) ) ;
#57806=DIRECTION ( 'NONE',  ( 0.000000000000000000, 0.000000000000000000, 1.000000000000000000 ) ) ;
#57807=CYLINDRICAL_SURFACE ( 'NONE', #58308, 5.599999999999994316 ) ;
#57808=LINE ( 'NONE', #85544, #78811 ) ;
#57809=LINE ( 'NONE', #44165, #73063 ) ;
#57813=DIRECTION ( 'NONE',  ( -1.000000000000000078E-15, 1.000000000000000083E-30, 1.000000000000000000 ) ) ;
#57815=LINE ( 'NONE', #65525, #76226 ) ;
#57816=DIRECTION ( 'NONE',  ( -0.8571673007021084478, -0.5150380749100604838, -8.571673007021083688E-16 ) ) ;
#57817=CARTESIAN_POINT ( 'NONE',  ( 100.4373464023292826, -44.86011580501824625, 12.03276813305398463 ) ) ;
#57818=CARTESIAN_POINT ( 'NONE',  ( 99.28859025714638165, -29.78777103691475858, 186.7470538473389752 ) ) ;
#57819=CARTESIAN_POINT ( 'NONE',  ( 117.4061096064183971, -38.22256018827695101, 24.71276813305395237 ) ) ;
#57820=AXIS2_PLACEMENT_3D ( 'NONE', #19099, #67244, #5483 ) ;
#57823=DIRECTION ( 'NONE',  ( 1.000000000000000078E-15, 1.000000000000000083E-30, -1.000000000000000000 ) ) ;
#57825=ORIENTED_EDGE ( 'NONE', *, *, #46582, .T. ) ;
#57826=PLANE ( 'NONE',  #34563 ) ;
#57828=CARTESIAN_POINT ( 'NONE',  ( 117.2535196871929770, -41.18324016912737306, 54.49848241876692612 ) ) ;
#57830=VERTEX_POINT ( 'NONE', #88234 ) ;
#57831=CARTESIAN_POINT ( 'NONE',  ( 33.78129701732998313, -35.65087443492610930, 237.4678068554150059 ) ) ;
#57832=CARTESIAN_POINT ( 'NONE',  ( 115.0229693000240303, -29.09019634776603169, 185.4232443235299570 ) ) ;
#57834=CYLINDRICAL_SURFACE ( 'NONE', #83507, 18.00000000000000000 ) ;
#57835=CARTESIAN_POINT ( 'NONE',  ( 97.81219835445369881, -40.51719899421586746, 151.6362400511890769 ) ) ;
#57836=CARTESIAN_POINT ( 'NONE',  ( 97.31584372111100834, -39.30597601896262461, 47.53145861081645762 ) ) ;
#57837=VECTOR ( 'NONE', #51091, 1000.000000000000000 ) ;
#57838=PLANE ( 'NONE',  #1299 ) ;
#57839=CARTESIAN_POINT ( 'NONE',  ( 110.8526248007088952, -45.98499320073891994, 97.88546641285240923 ) ) ;
#57840=CARTESIAN_POINT ( 'NONE',  ( 102.8912152862169762, -46.22186109533351583, 132.2346728949589760 ) ) ;
#57842=ORIENTED_EDGE ( 'NONE', *, *, #1624, .T. ) ;
#57845=CARTESIAN_POINT ( 'NONE',  ( 104.6418561626188364, -26.95233673609813962, 86.70158330589694629 ) ) ;
#57846=VECTOR ( 'NONE', #58206, 1000.000000000000000 ) ;
#57847=DIRECTION ( 'NONE',  ( 0.000000000000000000, 0.000000000000000000, -1.000000000000000000 ) ) ;
#57848=CARTESIAN_POINT ( 'NONE',  ( 96.80143343076643703, -35.25719154489702589, 222.2251490854339693 ) ) ;
#57850=DIRECTION ( 'NONE',  ( 0.000000000000000000, 0.000000000000000000, -1.000000000000000000 ) ) ;
#57852=EDGE_CURVE ( 'NONE', #82260, #73068, #68669, .T. ) ;
#57853=DIRECTION ( 'NONE',  ( -1.000000000000000078E-15, 1.000000000000000083E-30, 1.000000000000000000 ) ) ;
#57855=DIRECTION ( 'NONE',  ( 1.000000000000000078E-15, -1.000000000000000083E-30, -1.000000000000000000 ) ) ;
#57857=CARTESIAN_POINT ( 'NONE',  ( 102.9221092647373865, -27.14930527916904168, 155.4013395616249795 ) ) ;
#57858=ORIENTED_EDGE ( 'NONE', *, *, #80368, .T. ) ;
#57859=ORIENTED_EDGE ( 'NONE', *, *, #19630, .F. ) ;
#57861=AXIS2_PLACEMENT_3D ( 'NONE', #10375, #4457, #45754 ) ;
#57863=CARTESIAN_POINT ( 'NONE',  ( 51.42025729304100423, -33.70561438051981185, -5.074374724088000832 ) ) ;
#57864=AXIS2_PLACEMENT_3D ( 'NONE', #31211, #3080, #79842 ) ;
#57865=LINE ( 'NONE', #64686, #2987 ) ;
#57867=CARTESIAN_POINT ( 'NONE',  ( 100.8178804068425904, -31.43438811971037339, 213.5852332267339762 ) ) ;
#57868=ADVANCED_FACE ( 'NONE', ( #20078 ), #47752, .F. ) ;
#57870=CARTESIAN_POINT ( 'NONE',  ( 106.4836019150615840, -24.89303152268002606, 195.1156252759109861 ) ) ;
#57872=ORIENTED_EDGE ( 'NONE', *, *, #15452, .T. ) ;
#57874=VERTEX_POINT ( 'NONE', #27326 ) ;
#57877=ORIENTED_EDGE ( 'NONE', *, *, #74021, .T. ) ;
#57878=ORIENTED_EDGE ( 'NONE', *, *, #2329, .F. ) ;
#57879=CARTESIAN_POINT ( 'NONE',  ( 120.0664832912739399, -36.72944715994095333, 294.6356252759106837 ) ) ;
#57880=CARTESIAN_POINT ( 'NONE',  ( 133.1862368104903567, -34.12360705087674262, 8.106403045240790917 ) ) ;
#57881=CARTESIAN_POINT ( 'NONE',  ( 100.5471494818408189, -29.96373860736636274, 262.1063452106591853 ) ) ;
#57882=ADVANCED_FACE ( 'NONE', ( #87767 ), #9369, .T. ) ;
#57883=CARTESIAN_POINT ( 'NONE',  ( 41.56648329127398966, -27.82844715994070484, 138.9256252759119832 ) ) ;
#57884=ORIENTED_EDGE ( 'NONE', *, *, #7154, .T. ) ;
#57885=CARTESIAN_POINT ( 'NONE',  ( 116.0151837961063563, -39.81228804796826637, 9.635625275910943088 ) ) ;
#57888=ORIENTED_EDGE ( 'NONE', *, *, #49317, .T. ) ;
#57889=ORIENTED_EDGE ( 'NONE', *, *, #51644, .F. ) ;
#57890=CARTESIAN_POINT ( 'NONE',  ( 110.8556403160020238, -45.98375910300359948, 112.8857257452675071 ) ) ;
#57891=VERTEX_POINT ( 'NONE', #18721 ) ;
#57893=CARTESIAN_POINT ( 'NONE',  ( 99.10695020771697727, -33.55172231072156563, 40.44670554236296312 ) ) ;
#57894=CARTESIAN_POINT ( 'NONE',  ( 97.65468660891812647, -41.26425114427870255, 171.6841967044819626 ) ) ;
#57895=CARTESIAN_POINT ( 'NONE',  ( 113.3182355088851381, -45.04474967211709924, 143.0899109901969553 ) ) ;
#57896=CARTESIAN_POINT ( 'NONE',  ( 82.81648329127399677, -36.72944715994106701, 3.101481641215461327 ) ) ;
#57897=CARTESIAN_POINT ( 'NONE',  ( 101.6506511131177461, -45.63737897744897509, 243.1413395616249886 ) ) ;
#57899=EDGE_CURVE ( 'NONE', #22872, #20321, #34568, .T. ) ;
#57901=CARTESIAN_POINT ( 'NONE',  ( 188.5667039024479834, -67.87844715994100397, 168.3428068554150059 ) ) ;
#57902=ORIENTED_EDGE ( 'NONE', *, *, #32952, .F. ) ;
#57903=AXIS2_PLACEMENT_3D ( 'NONE', #76599, #85225, #71585 ) ;
#57904=EDGE_LOOP ( 'NONE', ( #46539, #700, #60942, #20362 ) ) ;
#57905=VECTOR ( 'NONE', #52248, 1000.000000000000000 ) ;
#57906=CARTESIAN_POINT ( 'NONE',  ( 106.4811411369643679, -24.84306116243460139, 195.1156252759109861 ) ) ;
#57908=CARTESIAN_POINT ( 'NONE',  ( 117.3102356154742836, -34.79226824040635790, 158.9756252759109714 ) ) ;
#57909=CARTESIAN_POINT ( 'NONE',  ( 51.06670390244676128, -33.35206098992668444, 193.9678068554150911 ) ) ;
#57911=DIRECTION ( 'NONE',  ( -1.058811598242755461E-16, 0.5150380749100580413, -0.8571673007021100021 ) ) ;
#57912=DIRECTION ( 'NONE',  ( 1.000000000000000000, 3.999999999999999995E-14, 1.000000000000000078E-15 ) ) ;
#57913=DIRECTION ( 'NONE',  ( 0.000000000000000000, 0.000000000000000000, -1.000000000000000000 ) ) ;
#57914=CARTESIAN_POINT ( 'NONE',  ( 104.8459308146384785, -26.52976224399709082, 256.2470538473397141 ) ) ;
#57915=CARTESIAN_POINT ( 'NONE',  ( 107.0664832912739541, -22.72944715994095688, 311.6343304127839815 ) ) ;
#57916=CARTESIAN_POINT ( 'NONE',  ( 73.06648329127399677, -8.729447159941065237, -4.824374724089063982 ) ) ;
#57917=CARTESIAN_POINT ( 'NONE',  ( 115.0859250807855574, -30.61377459443286142, 270.3439221990611827 ) ) ;
#57918=EDGE_CURVE ( 'NONE', #83511, #43446, #84797, .T. ) ;
#57919=CIRCLE ( 'NONE', #56410, 3.249999999999975131 ) ;
#57921=ADVANCED_FACE ( 'NONE', ( #69564 ), #29129, .T. ) ;
#57923=DIRECTION ( 'NONE',  ( 1.000000000000000078E-15, -1.000000000000000083E-30, -1.000000000000000000 ) ) ;
#57924=CARTESIAN_POINT ( 'NONE',  ( 113.2699234598519524, -29.59411848847293669, 195.5838068554167535 ) ) ;
#57926=CARTESIAN_POINT ( 'NONE',  ( 32.15435173586076445, -31.62489322948364290, 117.4678068554150485 ) ) ;
#57927=CARTESIAN_POINT ( 'NONE',  ( 101.1881973814857076, -45.36612005690837890, 197.1013395616249966 ) ) ;
#57928=CARTESIAN_POINT ( 'NONE',  ( 113.4153195569882087, -27.68144967124534261, 80.57753003781597556 ) ) ;
#57929=CARTESIAN_POINT ( 'NONE',  ( 106.9746138897780696, -47.19771061482636298, 183.5699109901969734 ) ) ;
#57930=DIRECTION ( 'NONE',  ( -6.524622321627019585E-16, -4.013151879589939944E-16, -1.000000000000000000 ) ) ;
#57931=AXIS2_PLACEMENT_3D ( 'NONE', #63290, #35122, #69661 ) ;
#57932=LINE ( 'NONE', #77491, #50357 ) ;
#57933=FACE_OUTER_BOUND ( 'NONE', #64464, .T. ) ;
#57934=CARTESIAN_POINT ( 'NONE',  ( 180.2143765759489895, -35.91149509761070391, 193.9678068554150059 ) ) ;
#57935=CARTESIAN_POINT ( 'NONE',  ( 156.5667039024483245, -42.82844715993568485, 173.2178068554149775 ) ) ;
#57936=CARTESIAN_POINT ( 'NONE',  ( 179.7974245136200011, -36.32844715994040996, -5.074374724088000832 ) ) ;
#57937=ORIENTED_EDGE ( 'NONE', *, *, #6672, .T. ) ;
#57938=FACE_OUTER_BOUND ( 'NONE', #35292, .T. ) ;
#57940=ORIENTED_EDGE ( 'NONE', *, *, #85801, .T. ) ;
#57941=VECTOR ( 'NONE', #81172, 1000.000000000000000 ) ;
#57942=CARTESIAN_POINT ( 'NONE',  ( 107.8593070027901746, -27.70813345913228076, 109.4171817328389551 ) ) ;
#57944=VERTEX_POINT ( 'NONE', #1427 ) ;
#57945=CARTESIAN_POINT ( 'NONE',  ( 109.7644292386349889, -47.42453529627113085, 88.78514908543493789 ) ) ;
#57946=DIRECTION ( 'NONE',  ( 0.000000000000000000, 0.000000000000000000, -1.000000000000000000 ) ) ;
#57947=DIRECTION ( 'NONE',  ( -0.9254794337955620787, -0.3787978585227822492, 0.000000000000000000 ) ) ;
#57948=CARTESIAN_POINT ( 'NONE',  ( 139.7494832912729805, -1.929447159941395817, 361.9756252759109998 ) ) ;
#57949=CARTESIAN_POINT ( 'NONE',  ( 98.38136461969642710, -29.78821554292430207, 45.78991099019597044 ) ) ;
#57952=ORIENTED_EDGE ( 'NONE', *, *, #76241, .T. ) ;
#57953=EDGE_LOOP ( 'NONE', ( #84322, #69107, #50106, #17939 ) ) ;
#57957=DIRECTION ( 'NONE',  ( 0.000000000000000000, 0.000000000000000000, -1.000000000000000000 ) ) ;
#57959=CARTESIAN_POINT ( 'NONE',  ( 104.4905195348742240, -26.97865216368831653, 51.28294879281423846 ) ) ;
#57961=AXIS2_PLACEMENT_3D ( 'NONE', #28234, #14179, #61858 ) ;
#57963=CARTESIAN_POINT ( 'NONE',  ( 96.21590750668994474, -38.71157422997263353, 51.48229194257797303 ) ) ;
#57964=ORIENTED_EDGE ( 'NONE', *, *, #69173, .T. ) ;
#57965=CIRCLE ( 'NONE', #62303, 2.117000000000007987 ) ;
#57968=CARTESIAN_POINT ( 'NONE',  ( 102.7086973628091187, -29.82731503872160417, 108.3423760838769851 ) ) ;
#57969=VECTOR ( 'NONE', #55980, 1000.000000000000000 ) ;
#57972=EDGE_CURVE ( 'NONE', #70165, #74183, #67368, .T. ) ;
#57973=FACE_OUTER_BOUND ( 'NONE', #56092, .T. ) ;
#57974=DIRECTION ( 'NONE',  ( 1.000000000000000000, 8.843517682682131024E-16, 1.000000000000000078E-15 ) ) ;
#57975=ORIENTED_EDGE ( 'NONE', *, *, #61345, .T. ) ;
#57976=ORIENTED_EDGE ( 'NONE', *, *, #7027, .F. ) ;
#57977=AXIS2_PLACEMENT_3D ( 'NONE', #36640, #64341, #8026 ) ;
#57978=ADVANCED_FACE ( 'NONE', ( #28670 ), #14153, .F. ) ;
#57979=CARTESIAN_POINT ( 'NONE',  ( 97.92336871694494960, -40.78101110081310310, 136.6586925773791563 ) ) ;
#57980=ORIENTED_EDGE ( 'NONE', *, *, #80244, .F. ) ;
#57981=ORIENTED_EDGE ( 'NONE', *, *, #64456, .T. ) ;
#57983=EDGE_CURVE ( 'NONE', #76720, #58643, #22772, .T. ) ;
#57984=CARTESIAN_POINT ( 'NONE',  ( 107.7905181614329564, -45.59160847044328335, 174.0730118773249728 ) ) ;
#57985=EDGE_CURVE ( 'NONE', #75709, #33402, #56362, .T. ) ;
#57987=CIRCLE ( 'NONE', #84142, 1.000000000000000888 ) ;
#57988=CARTESIAN_POINT ( 'NONE',  ( 118.9284187910711665, -36.16665333732972698, 114.8641967044819694 ) ) ;
#57989=DIRECTION ( 'NONE',  ( 0.8571673007021115565, -0.5150380749100554878, 7.521945815882500121E-16 ) ) ;
#57991=CARTESIAN_POINT ( 'NONE',  ( 116.9889466309420527, -35.34522876095464738, 18.93671031070073951 ) ) ;
#57995=ORIENTED_EDGE ( 'NONE', *, *, #58202, .F. ) ;
#57996=EDGE_CURVE ( 'NONE', #30195, #43969, #35469, .T. ) ;
#57997=CARTESIAN_POINT ( 'NONE',  ( 113.2609745038455742, -30.68550774403005121, 192.2718998934009562 ) ) ;
#57998=CARTESIAN_POINT ( 'NONE',  ( 101.0534108623914591, -27.42684531413746285, 70.54514908543497143 ) ) ;
#58000=CARTESIAN_POINT ( 'NONE',  ( 109.6376038899290677, -46.81002275840761939, 47.77562527591094721 ) ) ;
#58001=CARTESIAN_POINT ( 'NONE',  ( 117.5090302172161500, -40.42247023647522752, 174.5680062282919778 ) ) ;
#58002=EDGE_CURVE ( 'NONE', #10270, #34697, #63191, .T. ) ;
#58003=CARTESIAN_POINT ( 'NONE',  ( 188.5667039024479834, -62.87844715994099687, 173.2178068554149775 ) ) ;
#58005=CARTESIAN_POINT ( 'NONE',  ( 108.3194443806174405, -47.07896772641721839, 113.6727681330539639 ) ) ;
#58006=ADVANCED_FACE ( 'NONE', ( #42282 ), #85005, .T. ) ;
#58007=DIRECTION ( 'NONE',  ( -0.9254794337955620787, -0.3787978585227822492, 0.000000000000000000 ) ) ;
#58008=ORIENTED_EDGE ( 'NONE', *, *, #26106, .T. ) ;
#58016=CARTESIAN_POINT ( 'NONE',  ( 99.00936352106049299, -30.68773460668057851, 131.8138018080218217 ) ) ;
#58017=CARTESIAN_POINT ( 'NONE',  ( 99.29363446503140267, -43.73007054641615809, 56.90991099019593236 ) ) ;
#58018=DIRECTION ( 'NONE',  ( 0.000000000000000000, 0.000000000000000000, 1.000000000000000000 ) ) ;
#58020=CARTESIAN_POINT ( 'NONE',  ( 142.0664832912740110, -9.729447159940995959, -4.824374724088994704 ) ) ;
#58021=CARTESIAN_POINT ( 'NONE',  ( 105.5226833586260682, -46.38761039419750176, 37.44991099019695469 ) ) ;
#58022=CARTESIAN_POINT ( 'NONE',  ( 72.17003668186733023, -45.68655394112764156, -5.074374724089090627 ) ) ;
#58023=CARTESIAN_POINT ( 'NONE',  ( 102.4028819069269645, -26.73371583578780886, 131.4118157521009778 ) ) ;
#58025=FACE_OUTER_BOUND ( 'NONE', #87835, .T. ) ;
#58027=DIRECTION ( 'NONE',  ( 1.000000000000000078E-15, -1.000000000000000083E-30, -1.000000000000000000 ) ) ;
#58028=AXIS2_PLACEMENT_3D ( 'NONE', #8260, #42306, #70039 ) ;
#58029=ADVANCED_FACE ( 'NONE', ( #77276, #15051 ), #13697, .F. ) ;
#58031=EDGE_CURVE ( 'NONE', #53830, #29616, #70465, .T. ) ;
#58033=EDGE_CURVE ( 'NONE', #44371, #23155, #18044, .T. ) ;
#58035=DIRECTION ( 'NONE',  ( -0.7071067812158990940, -0.7071067811571960515, 0.000000000000000000 ) ) ;
#58036=CARTESIAN_POINT ( 'NONE',  ( 103.6240789207236475, -26.17659276989511596, 210.3394347997209763 ) ) ;
#58037=ORIENTED_EDGE ( 'NONE', *, *, #4665, .T. ) ;
#58038=FACE_OUTER_BOUND ( 'NONE', #82056, .T. ) ;
#58039=CARTESIAN_POINT ( 'NONE',  ( 101.2819412958853320, -26.35826957050098329, 251.4813395616249920 ) ) ;
#58040=CARTESIAN_POINT ( 'NONE',  ( 98.05938055883913762, -31.39417958322244218, 81.90133956162493689 ) ) ;
#58044=FACE_OUTER_BOUND ( 'NONE', #15876, .T. ) ;
#58046=ORIENTED_EDGE ( 'NONE', *, *, #47826, .T. ) ;
#58047=VECTOR ( 'NONE', #85307, 1000.000000000000000 ) ;
#58048=B_SPLINE_CURVE_WITH_KNOTS ( 'NONE', 3,
 ( #89629, #34193, #13319, #20137, #88736, #54165, #41006, #68726, #47810, #81925, #6492, #26491, #19681, #33755, #75549, #47361, #75090, #12880, #26945, #40567, #6067, #61444, #89175, #54613, #82372, #73136 ),
 .UNSPECIFIED., .F., .F.,
 ( 4, 2, 1, 1, 2, 2, 2, 2, 2, 2, 2, 2, 2, 4 ),
 ( 0.5000914289992475226, 0.5020441968547191269, 0.5039969647101907313, 0.5079025004211340510, 0.5157135718430211346, 0.5313357146867948577, 0.5625800003743418598, 0.6250685717494358640, 0.6875571431245298681, 0.7500457144996239833, 0.8125342858747179875, 0.8750228572498119917, 0.9375114286249059958, 1.000000000000000000 ),
 .UNSPECIFIED. ) ;
#58049=EDGE_LOOP ( 'NONE', ( #4485, #73393, #39308, #33108 ) ) ;
#58050=ORIENTED_EDGE ( 'NONE', *, *, #62778, .F. ) ;
#58052=DIRECTION ( 'NONE',  ( 0.000000000000000000, 1.000000000000000000, 0.000000000000000000 ) ) ;
#58053=CARTESIAN_POINT ( 'NONE',  ( 105.8935855965125938, -47.12395608077676457, 278.4870538473395527 ) ) ;
#58055=CARTESIAN_POINT ( 'NONE',  ( 131.8086190314097337, -35.15582774929892196, 2.518078172612455479 ) ) ;
#58057=DIRECTION ( 'NONE',  ( 4.299999999999999979E-14, -1.000000000000000000, 4.400000000000000367E-29 ) ) ;
#58059=DIRECTION ( 'NONE',  ( 4.299999999999999979E-14, -1.000000000000000000, 4.400000000000000367E-29 ) ) ;
#58060=CARTESIAN_POINT ( 'NONE',  ( 114.6728154972408475, -42.76387655025251888, 197.7152769709339566 ) ) ;
#58061=EDGE_LOOP ( 'NONE', ( #82464, #45736, #51712, #8481 ) ) ;
#58062=VERTEX_POINT ( 'NONE', #3647 ) ;
#58063=ORIENTED_EDGE ( 'NONE', *, *, #60849, .F. ) ;
#58064=PLANE ( 'NONE',  #18045 ) ;
#58066=CARTESIAN_POINT ( 'NONE',  ( 114.5610390845466071, -30.44493693613353358, 265.3813395616247135 ) ) ;
#58068=DIRECTION ( 'NONE',  ( 0.000000000000000000, 0.000000000000000000, -1.000000000000000000 ) ) ;
#58072=ORIENTED_EDGE ( 'NONE', *, *, #54892, .F. ) ;
#58073=CIRCLE ( 'NONE', #4458, 7.499999999999992895 ) ;
#58075=CARTESIAN_POINT ( 'NONE',  ( 102.7933444172945769, -44.96577155458380304, 15.01380465530593966 ) ) ;
#58076=CARTESIAN_POINT ( 'NONE',  ( 136.8118108219001101, -18.54506369576942149, 6.756870619998893268 ) ) ;
#58077=EDGE_CURVE ( 'NONE', #9110, #61450, #45405, .T. ) ;
#58079=LINE ( 'NONE', #3561, #56285 ) ;
#58082=VECTOR ( 'NONE', #16538, 1000.000000000000000 ) ;
#58085=CARTESIAN_POINT ( 'NONE',  ( 172.5667039024478413, -36.32844715993500273, 249.9678068554149775 ) ) ;
#58086=EDGE_LOOP ( 'NONE', ( #76548, #12682, #11524, #26432 ) ) ;
#58087=CARTESIAN_POINT ( 'NONE',  ( 100.2985985360463843, -46.45756217656626319, 87.09276813305393716 ) ) ;
#58088=ORIENTED_EDGE ( 'NONE', *, *, #13077, .F. ) ;
#58089=CARTESIAN_POINT ( 'NONE',  ( 101.6694414210978294, -29.45726664942652917, 35.01908649474394508 ) ) ;
#58090=EDGE_CURVE ( 'NONE', #17303, #68744, #71804, .T. ) ;
#58091=CARTESIAN_POINT ( 'NONE',  ( 106.9373099352470007, -46.76238444484523171, 88.56563845889516529 ) ) ;
#58092=CARTESIAN_POINT ( 'NONE',  ( 111.6972492074939396, -29.17403283370891032, 91.07015473446894305 ) ) ;
#58093=CARTESIAN_POINT ( 'NONE',  ( 117.0721298179341829, -35.46442564195397296, 14.92713738205877583 ) ) ;
#58097=CARTESIAN_POINT ( 'NONE',  ( 96.84642183402544902, -30.63342722027062592, 276.8984824187680829 ) ) ;
#58098=AXIS2_PLACEMENT_3D ( 'NONE', #38681, #58669, #73655 ) ;
#58099=CARTESIAN_POINT ( 'NONE',  ( 188.5667039024479834, -65.37844715994100397, 178.0928068554149775 ) ) ;
#58102=CARTESIAN_POINT ( 'NONE',  ( 162.7131505118539962, -33.70561438052090608, -5.074374724088000832 ) ) ;
#58104=CARTESIAN_POINT ( 'NONE',  ( 116.9452694852055998, -40.19391870447465465, 129.5584824187679658 ) ) ;
#58108=EDGE_CURVE ( 'NONE', #29962, #31120, #73208, .T. ) ;
#58109=VECTOR ( 'NONE', #28, 1000.000000000000000 ) ;
#58110=DIRECTION ( 'NONE',  ( -1.000000000000000000, 0.000000000000000000, 0.000000000000000000 ) ) ;
#58111=FACE_OUTER_BOUND ( 'NONE', #2784, .T. ) ;
#58112=CARTESIAN_POINT ( 'NONE',  ( 97.67678136301120162, -41.13084272647608941, 211.6632443235309893 ) ) ;
#58113=DIRECTION ( 'NONE',  ( -4.237773401492740281E-14, 1.000000000000000000, 0.000000000000000000 ) ) ;
#58116=CARTESIAN_POINT ( 'NONE',  ( 101.6089948421187898, -47.24856100052405594, 13.19562527591094891 ) ) ;
#58118=CARTESIAN_POINT ( 'NONE',  ( 72.06648329127396835, -9.729447159941065237, 14.67562527591093513 ) ) ;
#58119=ORIENTED_EDGE ( 'NONE', *, *, #26929, .F. ) ;
#58120=DIRECTION ( 'NONE',  ( 1.000000000000000078E-15, -1.000000000000000083E-30, -1.000000000000000000 ) ) ;
#58121=DIRECTION ( 'NONE',  ( 1.000000000000000000, 8.326672684688666480E-14, 0.000000000000000000 ) ) ;
#58124=DIRECTION ( 'NONE',  ( -0.7071067811865171526, -0.7071067811865779928, -7.071067811865164719E-16 ) ) ;
#58126=CARTESIAN_POINT ( 'NONE',  ( 103.0988156209413233, -47.86972635628425365, 252.3041967044823366 ) ) ;
#58128=CARTESIAN_POINT ( 'NONE',  ( 172.5664832912729878, -27.82844715994070484, 78.92562527591199739 ) ) ;
#58129=CYLINDRICAL_SURFACE ( 'NONE', #5533, 4.749999999999976907 ) ;
#58130=AXIS2_PLACEMENT_3D ( 'NONE', #21967, #77816, #7868 ) ;
#58131=CARTESIAN_POINT ( 'NONE',  ( 115.5432862745613676, -35.46615253551063063, 218.3667055423629790 ) ) ;
#58132=CARTESIAN_POINT ( 'NONE',  ( 151.0371591254582597, -46.82818131005583240, 300.4678068554149490 ) ) ;
#58133=CARTESIAN_POINT ( 'NONE',  ( 116.3681181406586518, -31.99193570193499525, 40.20133956162496958 ) ) ;
#58134=CARTESIAN_POINT ( 'NONE',  ( 73.06670390244801183, -50.82844715994100682, 310.9178068554150514 ) ) ;
#58135=CARTESIAN_POINT ( 'NONE',  ( 108.5962597759698127, -47.12230983477568458, 142.6927681330539883 ) ) ;
#58136=EDGE_LOOP ( 'NONE', ( #31857, #28004, #7056, #24885 ) ) ;
#58137=CARTESIAN_POINT ( 'NONE',  ( 131.9720459101981760, -20.52018918696424166, 7.480061334662067019 ) ) ;
#58140=DIRECTION ( 'NONE',  ( -1.000000000000000000, -4.299999999999999979E-14, -1.000000000000000078E-15 ) ) ;
#58141=CARTESIAN_POINT ( 'NONE',  ( 97.31637614840812489, -39.30795178117394073, 277.5316211441031555 ) ) ;
#58144=DIRECTION ( 'NONE',  ( 1.000000000000000000, 0.000000000000000000, 0.000000000000000000 ) ) ;
#58145=ORIENTED_EDGE ( 'NONE', *, *, #76874, .T. ) ;
#58150=CARTESIAN_POINT ( 'NONE',  ( 49.16670390244701139, -28.27351298637340093, 342.9256252759119548 ) ) ;
#58151=ORIENTED_EDGE ( 'NONE', *, *, #9659, .T. ) ;
#58153=CARTESIAN_POINT ( 'NONE',  ( 115.2845782536562353, -44.15631435451261666, 83.25372051400698581 ) ) ;
#58154=SHAPE_REPRESENTATION_RELATIONSHIP ( 'NONE' , 'NONE' ,  #64293, #56477 ) ;
#58156=CYLINDRICAL_SURFACE ( 'NONE', #66942, 1.000000000000003775 ) ;
#58159=LINE ( 'NONE', #79067, #14155 ) ;
#58160=DIRECTION ( 'NONE',  ( 0.000000000000000000, 0.000000000000000000, 1.000000000000000000 ) ) ;
#58161=CARTESIAN_POINT ( 'NONE',  ( 20.56670390244643443, -48.82844715994099971, 180.4678068554150911 ) ) ;
#58162=VECTOR ( 'NONE', #13502, 1000.000000000000000 ) ;
#58163=ADVANCED_FACE ( 'NONE', ( #24546, #52209 ), #3214, .F. ) ;
#58164=DIRECTION ( 'NONE',  ( -1.000000000000000078E-15, 1.000000000000000083E-30, 1.000000000000000000 ) ) ;
#58166=CARTESIAN_POINT ( 'NONE',  ( 31.78666935232898894, -29.62846900982320264, -5.074374724088000832 ) ) ;
#58168=ADVANCED_FACE ( 'NONE', ( #58594 ), #16689, .T. ) ;
#58171=CARTESIAN_POINT ( 'NONE',  ( 116.0678243078410787, -40.55558035091540603, 164.5070538473389661 ) ) ;
#58173=CARTESIAN_POINT ( 'NONE',  ( 80.06648329127399677, -36.72944715994107412, 14.92562527591094224 ) ) ;
#58175=CARTESIAN_POINT ( 'NONE',  ( 97.30224646444959546, -33.23681714887386818, 22.06514908543394426 ) ) ;
#58178=CARTESIAN_POINT ( 'NONE',  ( 105.7138873538276727, -46.72361729074350478, 12.46910743858308379 ) ) ;
#58179=AXIS2_PLACEMENT_3D ( 'NONE', #47162, #12222, #26730 ) ;
#58180=VERTEX_POINT ( 'NONE', #51773 ) ;
#58181=CARTESIAN_POINT ( 'NONE',  ( 115.0899025498120807, -30.61893087844507733, 29.34406161155381199 ) ) ;
#58182=CARTESIAN_POINT ( 'NONE',  ( 106.9482321581270270, -47.09886382165569785, 232.5794347997209854 ) ) ;
#58183=EDGE_LOOP ( 'NONE', ( #38444, #60692, #66696, #85971 ) ) ;
#58186=CARTESIAN_POINT ( 'NONE',  ( 113.7913652599847438, -30.16800768036728542, 190.8853928297069444 ) ) ;
#58188=CARTESIAN_POINT ( 'NONE',  ( 101.0434111811767224, -43.22951492638978266, 43.41301187732599232 ) ) ;
#58190=ADVANCED_FACE ( 'NONE', ( #64540 ), #2322, .T. ) ;
#58191=EDGE_CURVE ( 'NONE', #78957, #50094, #57715, .T. ) ;
#58192=CARTESIAN_POINT ( 'NONE',  ( 115.8254323921426874, -31.73001882930526207, 79.23979194253121250 ) ) ;
#58193=DIRECTION ( 'NONE',  ( 4.194175870806139918E-14, -1.000000000000000000, 0.000000000000000000 ) ) ;
#58196=EDGE_CURVE ( 'NONE', #68666, #65898, #78643, .T. ) ;
#58198=ORIENTED_EDGE ( 'NONE', *, *, #28144, .T. ) ;
#58199=CARTESIAN_POINT ( 'NONE',  ( 109.9831304889623027, -26.74336511273919115, 259.8499109901965767 ) ) ;
#58200=FACE_OUTER_BOUND ( 'NONE', #35995, .T. ) ;
#58201=ORIENTED_EDGE ( 'NONE', *, *, #30911, .F. ) ;
#58202=EDGE_CURVE ( 'NONE', #87802, #64292, #44217, .T. ) ;
#58203=DIRECTION ( 'NONE',  ( 0.000000000000000000, 0.000000000000000000, 1.000000000000000000 ) ) ;
#58205=DIRECTION ( 'NONE',  ( -0.7071067811864671926, -0.7071067811866279529, -7.071067811864664779E-16 ) ) ;
#58206=DIRECTION ( 'NONE',  ( -1.058811598242755461E-16, 0.5150380749100580413, -0.8571673007021100021 ) ) ;
#58207=AXIS2_PLACEMENT_3D ( 'NONE', #83695, #21010, #15551 ) ;
#58208=CARTESIAN_POINT ( 'NONE',  ( 107.5734549334945314, -47.83597508069280480, 38.61276813305297395 ) ) ;
#58212=AXIS2_PLACEMENT_3D ( 'NONE', #82606, #68510, #68954 ) ;
#58213=CARTESIAN_POINT ( 'NONE',  ( 115.7091107927249283, -43.69381994074442588, 39.27467289495895386 ) ) ;
#58215=CARTESIAN_POINT ( 'NONE',  ( 105.1090048964814940, -25.85068961359000284, 275.2061014663871674 ) ) ;
#58216=ORIENTED_EDGE ( 'NONE', *, *, #34693, .T. ) ;
#58218=DIRECTION ( 'NONE',  ( 0.000000000000000000, 0.000000000000000000, -1.000000000000000000 ) ) ;
#58219=CARTESIAN_POINT ( 'NONE',  ( 180.2121375201600131, -29.73316016639650172, -5.074374724088000832 ) ) ;
#58220=CARTESIAN_POINT ( 'NONE',  ( 57.56670390244804736, -42.82844715994040286, 293.2178068554150627 ) ) ;
#58221=CARTESIAN_POINT ( 'NONE',  ( 100.0846959373945566, -41.84369885408329992, 104.6357094172109470 ) ) ;
#58222=CARTESIAN_POINT ( 'NONE',  ( 110.5060411634814557, -26.86503128786541694, 205.8099109901969541 ) ) ;
#58223=DIRECTION ( 'NONE',  ( 1.000000000000000078E-15, -1.000000000000000083E-30, -1.000000000000000000 ) ) ;
#58227=DIRECTION ( 'NONE',  ( 1.907762142705490052E-15, 7.167082501179359715E-16, -1.000000000000000000 ) ) ;
#58228=EDGE_LOOP ( 'NONE', ( #74404, #63841, #2448, #33480 ) ) ;
#58229=VECTOR ( 'NONE', #84323, 1000.000000000000000 ) ;
#58233=ORIENTED_EDGE ( 'NONE', *, *, #22019, .T. ) ;
#58234=CARTESIAN_POINT ( 'NONE',  ( 116.7958028337206855, -39.38540548342588465, 169.6153133619191067 ) ) ;
#58235=CARTESIAN_POINT ( 'NONE',  ( 103.2785305379161969, -27.47464224906687491, 41.38562391700290988 ) ) ;
#58236=CARTESIAN_POINT ( 'NONE',  ( 104.1185212827848545, -44.74603268130591971, 141.7181341137909669 ) ) ;
#58237=VECTOR ( 'NONE', #77916, 1000.000000000000000 ) ;
#58238=CARTESIAN_POINT ( 'NONE',  ( 100.2336795655629089, -28.82633655636628589, 260.6441967044821695 ) ) ;
#58240=VECTOR ( 'NONE', #42481, 1000.000000000000000 ) ;
#58241=ORIENTED_EDGE ( 'NONE', *, *, #75886, .T. ) ;
#58242=CARTESIAN_POINT ( 'NONE',  ( 99.09542022332205136, -30.55081675378443862, 136.8022615499500603 ) ) ;
#58243=ORIENTED_EDGE ( 'NONE', *, *, #89197, .F. ) ;
#58245=DIRECTION ( 'NONE',  ( 1.000000000000000000, 8.141040168700802252E-12, 0.000000000000000000 ) ) ;
#58246=ADVANCED_FACE ( 'NONE', ( #80862 ), #88568, .T. ) ;
#58247=DIRECTION ( 'NONE',  ( 1.000000000000000000, 4.163336342344333240E-14, 0.000000000000000000 ) ) ;
#58248=CARTESIAN_POINT ( 'NONE',  ( 113.7843247631140571, -29.05179538500707892, 289.5032443235299979 ) ) ;
#58250=CARTESIAN_POINT ( 'NONE',  ( 118.6541713771196527, -39.21258442193070692, 258.6584824187679033 ) ) ;
#58251=CARTESIAN_POINT ( 'NONE',  ( 96.29945253806019423, -39.42498279898523350, 12.53372051400597442 ) ) ;
#58252=CYLINDRICAL_SURFACE ( 'NONE', #3941, 2.750000000000002665 ) ;
#58254=CARTESIAN_POINT ( 'NONE',  ( 79.56670390244796920, -50.82844715994100682, 280.9178068554149945 ) ) ;
#58256=DIRECTION ( 'NONE',  ( 0.7071067811989784069, -0.7071067811741166276, 6.612322855976402389E-17 ) ) ;
#58257=CARTESIAN_POINT ( 'NONE',  ( 131.5922609085481838, -37.93375462386097752, 7.110117206094888509 ) ) ;
#58258=AXIS2_PLACEMENT_3D ( 'NONE', #71796, #30013, #15940 ) ;
#58259=DIRECTION ( 'NONE',  ( 0.000000000000000000, 0.000000000000000000, 1.000000000000000000 ) ) ;
#58260=CARTESIAN_POINT ( 'NONE',  ( 116.8169175499061936, -34.15212344989235760, 164.0313744165063667 ) ) ;
#58261=CARTESIAN_POINT ( 'NONE',  ( 107.0664832912739968, -36.72944715994100306, 287.6356252759109680 ) ) ;
#58262=CARTESIAN_POINT ( 'NONE',  ( 123.6837132603320413, -23.41243780205710578, 239.5838068554165545 ) ) ;
#58263=CARTESIAN_POINT ( 'NONE',  ( 116.6022279875747216, -42.36549642380604297, 283.4137205140060018 ) ) ;
#58264=CARTESIAN_POINT ( 'NONE',  ( 95.56951908670150431, -39.60249947413915805, 162.5213395616259788 ) ) ;
#58265=CARTESIAN_POINT ( 'NONE',  ( 117.0746561606024869, -31.98374578269911339, 60.19086337114898555 ) ) ;
#58266=AXIS2_PLACEMENT_3D ( 'NONE', #43163, #56795, #36820 ) ;
#58267=CARTESIAN_POINT ( 'NONE',  ( 116.3274949261486881, -32.94048995676258329, 25.13562527591095375 ) ) ;
#58269=CARTESIAN_POINT ( 'NONE',  ( 82.81648329127399677, -36.72944715994106701, 3.101481641215461327 ) ) ;
#58270=AXIS2_PLACEMENT_3D ( 'NONE', #3048, #67049, #37569 ) ;
#58271=EDGE_CURVE ( 'NONE', #25851, #2950, #61718, .T. ) ;
#58272=EDGE_LOOP ( 'NONE', ( #83361, #48362, #10643, #50380 ) ) ;
#58273=CARTESIAN_POINT ( 'NONE',  ( 41.56648329127398966, -27.82844715994070484, 318.9256252759120116 ) ) ;
#58274=ORIENTED_EDGE ( 'NONE', *, *, #71382, .F. ) ;
#58275=CARTESIAN_POINT ( 'NONE',  ( 113.9027609268605659, -43.72435554967452731, 69.19276813305297935 ) ) ;
#58276=DIRECTION ( 'NONE',  ( -4.237773401492740281E-14, 1.000000000000000000, 0.000000000000000000 ) ) ;
#58277=EDGE_LOOP ( 'NONE', ( #34633, #3638, #81254, #21612 ) ) ;
#58278=DIRECTION ( 'NONE',  ( 1.000000000000000078E-15, -1.000000000000000083E-30, -1.000000000000000000 ) ) ;
#58279=CARTESIAN_POINT ( 'NONE',  ( 103.5497706991577189, -26.90106182813410740, 186.3499109901969746 ) ) ;
#58280=CARTESIAN_POINT ( 'NONE',  ( 163.0664832912739826, 19.62155284005901024, 333.4006252759110112 ) ) ;
#58281=DIRECTION ( 'NONE',  ( 0.7071067811865046071, 0.7071067811865904273, 7.071067811865351088E-16 ) ) ;
#58284=CIRCLE ( 'NONE', #80027, 0.5000000000000104361 ) ;
#58285=DIRECTION ( 'NONE',  ( 1.000000000000000000, 0.000000000000000000, 0.000000000000000000 ) ) ;
#58286=CARTESIAN_POINT ( 'NONE',  ( 98.04149280439727931, -41.04180111718832791, 96.68119745713256918 ) ) ;
#58287=CARTESIAN_POINT ( 'NONE',  ( 113.4245949246308243, -29.25360672088980962, 139.5156252759109634 ) ) ;
#58288=EDGE_LOOP ( 'NONE', ( #41894, #86752, #1753, #19010 ) ) ;
#58289=ORIENTED_EDGE ( 'NONE', *, *, #73126, .T. ) ;
#58290=AXIS2_PLACEMENT_3D ( 'NONE', #12703, #27662, #55340 ) ;
#58291=CARTESIAN_POINT ( 'NONE',  ( 102.5140397859015877, -29.09155558458053292, 81.93586902018296314 ) ) ;
#58292=AXIS2_PLACEMENT_3D ( 'NONE', #44905, #59426, #51711 ) ;
#58293=CARTESIAN_POINT ( 'NONE',  ( 90.44969454456415292, -55.86395651782494554, 239.5838068554169809 ) ) ;
#58294=CARTESIAN_POINT ( 'NONE',  ( 101.0525363619397581, -44.44280425155404401, 228.0499109901959400 ) ) ;
#58295=FACE_OUTER_BOUND ( 'NONE', #52677, .T. ) ;
#58296=DIRECTION ( 'NONE',  ( 0.000000000000000000, 1.000000000000000000, 0.000000000000000000 ) ) ;
#58297=DIRECTION ( 'NONE',  ( -0.000000000000000000, 1.000000000000000000, 0.000000000000000000 ) ) ;
#58298=ADVANCED_FACE ( 'NONE', ( #32234 ), #50055, .F. ) ;
#58299=AXIS2_PLACEMENT_3D ( 'NONE', #77584, #56211, #63046 ) ;
#58302=LINE ( 'NONE', #86475, #56516 ) ;
#58305=CARTESIAN_POINT ( 'NONE',  ( 99.43809884604145566, -27.69271567064627604, 150.6356252759109680 ) ) ;
#58306=EDGE_CURVE ( 'NONE', #76939, #54739, #5892, .T. ) ;
#58307=ORIENTED_EDGE ( 'NONE', *, *, #18617, .F. ) ;
#58308=AXIS2_PLACEMENT_3D ( 'NONE', #85543, #85985, #23322 ) ;
#58310=EDGE_CURVE ( 'NONE', #7448, #57293, #61283, .T. ) ;
#58311=DIRECTION ( 'NONE',  ( -0.000000000000000000, -0.000000000000000000, 1.000000000000000000 ) ) ;
#58312=DIRECTION ( 'NONE',  ( 1.000000000000000078E-15, 0.000000000000000000, 1.000000000000000000 ) ) ;
#58313=CARTESIAN_POINT ( 'NONE',  ( 98.30753418069124905, -41.72887547393442986, 77.73979194101322321 ) ) ;
#58314=CARTESIAN_POINT ( 'NONE',  ( 97.82501843714776157, -40.54985425570063029, 102.6384157449830923 ) ) ;
#58315=CARTESIAN_POINT ( 'NONE',  ( 113.6834210241909346, -31.15118039646248249, 222.1899951314959480 ) ) ;
#58316=PLANE ( 'NONE',  #53768 ) ;
#58317=CARTESIAN_POINT ( 'NONE',  ( 117.4265927121613089, -30.97543824232759135, 179.2299109901959753 ) ) ;
#58320=ORIENTED_EDGE ( 'NONE', *, *, #77237, .F. ) ;
#58324=DIRECTION ( 'NONE',  ( -2.900000000000000265E-14, 2.000000000000000155E-15, -1.000000000000000000 ) ) ;
#58325=CARTESIAN_POINT ( 'NONE',  ( 131.6729728819624370, -35.37149612623981909, 7.198162082935252393 ) ) ;
#58326=CARTESIAN_POINT ( 'NONE',  ( 98.67113652751868358, -38.83122756767168227, 14.35189989340096517 ) ) ;
#58328=ORIENTED_EDGE ( 'NONE', *, *, #30229, .T. ) ;
#58329=CIRCLE ( 'NONE', #22049, 1.000000000000000888 ) ;
#58330=CARTESIAN_POINT ( 'NONE',  ( 116.7260014990201284, -39.09146540103774470, 9.635625275910941312 ) ) ;
#58332=ORIENTED_EDGE ( 'NONE', *, *, #12279, .F. ) ;
#58333=ORIENTED_EDGE ( 'NONE', *, *, #50924, .T. ) ;
#58335=CARTESIAN_POINT ( 'NONE',  ( 107.0664832912739968, -36.72944715994100306, 287.6356252759109680 ) ) ;
#58336=ORIENTED_EDGE ( 'NONE', *, *, #87246, .T. ) ;
#58337=ORIENTED_EDGE ( 'NONE', *, *, #49776, .T. ) ;
#58338=CARTESIAN_POINT ( 'NONE',  ( 105.6358988306284346, -28.30874812457275524, 14.63241982807694797 ) ) ;
#58339=CARTESIAN_POINT ( 'NONE',  ( 105.7175586466805157, -24.93052779236126781, 160.1670538473389627 ) ) ;
#58340=CARTESIAN_POINT ( 'NONE',  ( 114.1602155298370036, -45.17592836263241196, 148.1203871806719405 ) ) ;
#58342=CARTESIAN_POINT ( 'NONE',  ( 96.26801084314395496, -34.37000373589627600, 252.1432443235302969 ) ) ;
#58343=CARTESIAN_POINT ( 'NONE',  ( 177.4809174648215162, -48.32844715993478246, 180.4678068554150059 ) ) ;
#58344=CARTESIAN_POINT ( 'NONE',  ( 29.77381068363482441, -48.62134037875501491, 249.9678068554150059 ) ) ;
#58347=AXIS2_PLACEMENT_3D ( 'NONE', #20773, #325, #28022 ) ;
#58350=AXIS2_PLACEMENT_3D ( 'NONE', #68065, #39895, #39457 ) ;
#58351=CARTESIAN_POINT ( 'NONE',  ( 98.39836552415940218, -29.79571670633027836, 195.7775300378159784 ) ) ;
#58352=VERTEX_POINT ( 'NONE', #32687 ) ;
#58353=CARTESIAN_POINT ( 'NONE',  ( 112.7802237386950992, -45.44955040250216172, 178.0384824187679556 ) ) ;
#58356=CYLINDRICAL_SURFACE ( 'NONE', #66753, 0.5000000000000007772 ) ;
#58357=DIRECTION ( 'NONE',  ( 1.000000000000000078E-15, 1.000000000000000083E-30, -1.000000000000000000 ) ) ;
#58358=CARTESIAN_POINT ( 'NONE',  ( 129.8079539024480198, -42.97311385574000298, 231.5838068554170093 ) ) ;
#58359=DIRECTION ( 'NONE',  ( 1.000000000000000078E-15, 0.000000000000000000, -1.000000000000000000 ) ) ;
#58360=CARTESIAN_POINT ( 'NONE',  ( 101.0991643652557599, -45.25116564454916102, 278.0899109901965858 ) ) ;
#58362=CYLINDRICAL_SURFACE ( 'NONE', #52559, 14.00000000000000888 ) ;
#58363=VECTOR ( 'NONE', #8443, 1000.000000000000000 ) ;
#58364=CARTESIAN_POINT ( 'NONE',  ( 115.8228748906924750, -31.72559827118475440, 270.2397737374858480 ) ) ;
#58367=LINE ( 'NONE', #11104, #59339 ) ;
#58368=CARTESIAN_POINT ( 'NONE',  ( 112.9239127876531938, -29.01757442955986477, 195.5838068554168387 ) ) ;
#58369=EDGE_LOOP ( 'NONE', ( #13378, #14400, #61386, #7399, #69714 ) ) ;
#58370=DIRECTION ( 'NONE',  ( 0.000000000000000000, -1.000000000000000000, 0.000000000000000000 ) ) ;
#58371=CARTESIAN_POINT ( 'NONE',  ( 98.64801509901850807, -30.48302769619336416, 180.8184824187679567 ) ) ;
#58372=CARTESIAN_POINT ( 'NONE',  ( 115.0226255289246922, -43.52070134976005988, 59.26419670448196086 ) ) ;
#58373=CARTESIAN_POINT ( 'NONE',  ( 101.6280127420326522, -45.67461444920139257, 243.1413395616249886 ) ) ;
#58374=DIRECTION ( 'NONE',  ( -0.7071067811567173234, 0.7071067812163779331, 0.000000000000000000 ) ) ;
#58375=LINE ( 'NONE', #4758, #28650 ) ;
#58376=DIRECTION ( 'NONE',  ( 0.000000000000000000, 0.000000000000000000, -1.000000000000000000 ) ) ;
#58377=CARTESIAN_POINT ( 'NONE',  ( 97.83668494123075732, -40.57802212005890397, 37.64055050525384161 ) ) ;
#58379=CARTESIAN_POINT ( 'NONE',  ( 25.56670390244797275, -58.35344715994099829, 137.2178068554150059 ) ) ;
#58380=ORIENTED_EDGE ( 'NONE', *, *, #16815, .T. ) ;
#58382=EDGE_CURVE ( 'NONE', #83503, #56235, #64545, .T. ) ;
#58383=VERTEX_POINT ( 'NONE', #55347 ) ;
#58384=VERTEX_POINT ( 'NONE', #48979 ) ;
#58385=CARTESIAN_POINT ( 'NONE',  ( 111.5299334411454311, -29.44702005892069607, 94.06099125664896121 ) ) ;
#58386=CARTESIAN_POINT ( 'NONE',  ( 30.48091746481741637, -48.32844715994156815, 180.4678068554150911 ) ) ;
#58388=VECTOR ( 'NONE', #87555, 1000.000000000000000 ) ;
#58389=CARTESIAN_POINT ( 'NONE',  ( 106.6611865629619160, -26.33404432545466634, 81.10705384733896040 ) ) ;
#58390=DIRECTION ( 'NONE',  ( 1.000000000000000000, 3.999999999999999995E-14, 1.000000000000000078E-15 ) ) ;
#58391=CARTESIAN_POINT ( 'NONE',  ( 162.7131505118549342, -33.70561438051439040, 117.4678068554150485 ) ) ;
#58392=CARTESIAN_POINT ( 'NONE',  ( 113.2454987028225730, -28.75867294873037494, 175.5522919420834853 ) ) ;
#58393=CARTESIAN_POINT ( 'NONE',  ( 100.2135729635196242, -43.75450166755856429, 21.96133956162593748 ) ) ;
#58395=VERTEX_POINT ( 'NONE', #27669 ) ;
#58398=CARTESIAN_POINT ( 'NONE',  ( 172.5667039024478129, -36.32844715993500273, 313.9678068554149490 ) ) ;
#58399=LINE ( 'NONE', #66553, #15737 ) ;
#58400=DIRECTION ( 'NONE',  ( 0.000000000000000000, 0.000000000000000000, 1.000000000000000000 ) ) ;
#58401=CARTESIAN_POINT ( 'NONE',  ( 135.0664832912729878, -36.72944715994189835, 361.9756252759079871 ) ) ;
#58402=CARTESIAN_POINT ( 'NONE',  ( 32.09598329127609873, -23.42844715994129956, 193.9678068554150911 ) ) ;
#58403=CARTESIAN_POINT ( 'NONE',  ( 97.12551982384144367, -37.99658701952105133, 52.42742285273963887 ) ) ;
#58406=CARTESIAN_POINT ( 'NONE',  ( 116.3681181406587370, -31.99193570193495262, 44.20133956162491984 ) ) ;
#58408=AXIS2_PLACEMENT_3D ( 'NONE', #66911, #68269, #39201 ) ;
#58413=CARTESIAN_POINT ( 'NONE',  ( 111.7725766154891431, -30.05993356141850015, 127.4052332267339693 ) ) ;
#58414=VECTOR ( 'NONE', #699, 1000.000000000000000 ) ;
#58415=CARTESIAN_POINT ( 'NONE',  ( 97.39148490005503334, -39.27924475881587085, 96.53152011028632273 ) ) ;
#58421=LINE ( 'NONE', #80230, #19180 ) ;
#58422=VERTEX_POINT ( 'NONE', #89918 ) ;
#58423=ORIENTED_EDGE ( 'NONE', *, *, #85310, .F. ) ;
#58424=EDGE_CURVE ( 'NONE', #56522, #65097, #55783, .T. ) ;
#58425=CARTESIAN_POINT ( 'NONE',  ( 115.8619398590553260, -35.64860379657582712, 190.3558690201829506 ) ) ;
#58427=CARTESIAN_POINT ( 'NONE',  ( 114.5277216628477248, -29.41153075798395733, 145.4441967044819819 ) ) ;
#58429=CARTESIAN_POINT ( 'NONE',  ( 110.8617057341842695, -45.98127435360438398, 17.88624725593324882 ) ) ;
#58431=ORIENTED_EDGE ( 'NONE', *, *, #66709, .T. ) ;
#58433=CARTESIAN_POINT ( 'NONE',  ( 100.2649065926023297, -31.37786052998579223, 198.6261856076869776 ) ) ;
#58434=CIRCLE ( 'NONE', #57018, 2.030000000001807248 ) ;
#58435=CARTESIAN_POINT ( 'NONE',  ( 103.4695482323410118, -25.41149354249025549, 55.32133956162594046 ) ) ;
#58437=CARTESIAN_POINT ( 'NONE',  ( 96.21590750668994474, -38.71157422997263353, 51.48229194257797303 ) ) ;
#58438=LINE ( 'NONE', #87500, #84898 ) ;
#58439=DIRECTION ( 'NONE',  ( 1.000000000000000000, -6.745093096447288888E-17, 0.000000000000000000 ) ) ;
#58440=DIRECTION ( 'NONE',  ( -4.299999999999999979E-14, 1.000000000000000000, 0.000000000000000000 ) ) ;
#58441=CARTESIAN_POINT ( 'NONE',  ( 108.6487146914112287, -25.79677769486274386, 145.9737205140069420 ) ) ;
#58443=ORIENTED_EDGE ( 'NONE', *, *, #1142, .T. ) ;
#58444=DIRECTION ( 'NONE',  ( 1.000000000000000078E-15, -1.000000000000000000, 0.000000000000000000 ) ) ;
#58445=VERTEX_POINT ( 'NONE', #54894 ) ;
#58446=CARTESIAN_POINT ( 'NONE',  ( 97.81085527707094229, -40.51777768585955641, 251.6359959587111064 ) ) ;
#58448=ORIENTED_EDGE ( 'NONE', *, *, #5898, .F. ) ;
#58449=AXIS2_PLACEMENT_3D ( 'NONE', #54381, #48029, #75763 ) ;
#58451=DIRECTION ( 'NONE',  ( 0.000000000000000000, 1.000000000000000000, 0.000000000000000000 ) ) ;
#58452=CARTESIAN_POINT ( 'NONE',  ( 103.5987056385471448, -46.56110768157568458, 57.30705384733997221 ) ) ;
#58453=DIRECTION ( 'NONE',  ( 1.000000000000000078E-15, 9.367723249499513438E-31, -1.000000000000000000 ) ) ;
#58454=EDGE_CURVE ( 'NONE', #59703, #71348, #28552, .T. ) ;
#58455=DIRECTION ( 'NONE',  ( 1.000000000000000078E-15, -1.000000000000000083E-30, -1.000000000000000000 ) ) ;
#58456=CARTESIAN_POINT ( 'NONE',  ( 73.06670390244801183, -48.82844715994099971, 10.91780685541510110 ) ) ;
#58457=CARTESIAN_POINT ( 'NONE',  ( 115.0479362680066515, -42.38275094372912122, 53.33562527591095659 ) ) ;
#58458=DIRECTION ( 'NONE',  ( 0.000000000000000000, 0.000000000000000000, -1.000000000000000000 ) ) ;
#58459=CARTESIAN_POINT ( 'NONE',  ( 104.4591861284130232, -26.65816784528765382, 196.2784824187679362 ) ) ;
#58460=CARTESIAN_POINT ( 'NONE',  ( 106.5207973735215319, -24.24134984979954410, 321.1698005525342978 ) ) ;
#58462=EDGE_LOOP ( 'NONE', ( #36330, #56723, #57752, #42898, #63016, #51877 ) ) ;
#58463=DIRECTION ( 'NONE',  ( -1.000000000000000000, -3.999999999999999995E-14, -1.000000000000000078E-15 ) ) ;
#58465=CYLINDRICAL_SURFACE ( 'NONE', #71997, 3.000000000000002665 ) ;
#58466=CARTESIAN_POINT ( 'NONE',  ( 29.56670390244797630, -48.82844715994099971, 10.91780685541479734 ) ) ;
#58467=CARTESIAN_POINT ( 'NONE',  ( 98.34291691341793751, -29.86560907334282788, 200.8080062282919869 ) ) ;
#58469=LINE ( 'NONE', #45715, #13173 ) ;
#58470=CARTESIAN_POINT ( 'NONE',  ( 118.1305967499472160, -36.20925573564677791, 264.8518157521014587 ) ) ;
#58471=CARTESIAN_POINT ( 'NONE',  ( 98.16534761909046836, -43.36023007783336425, 107.8480062282919647 ) ) ;
#58472=CARTESIAN_POINT ( 'NONE',  ( 97.07216957362197718, -35.37749098132034931, 252.2221255759655207 ) ) ;
#58473=CARTESIAN_POINT ( 'NONE',  ( 100.9534681770906275, -28.70796848357117881, 191.5938865662113244 ) ) ;
#58476=ORIENTED_EDGE ( 'NONE', *, *, #63334, .T. ) ;
#58477=CIRCLE ( 'NONE', #75867, 2.116999999999993776 ) ;
#58478=EDGE_CURVE ( 'NONE', #69697, #80300, #42617, .T. ) ;
#58479=VECTOR ( 'NONE', #34089, 1000.000000000000000 ) ;
#58482=AXIS2_PLACEMENT_3D ( 'NONE', #12189, #5832, #60314 ) ;
#58483=ADVANCED_FACE ( 'NONE', ( #28100 ), #20854, .T. ) ;
#58486=CARTESIAN_POINT ( 'NONE',  ( 111.7390528236686436, -27.41013440965690862, 275.7070538473395800 ) ) ;
#58487=CARTESIAN_POINT ( 'NONE',  ( 118.7735074478422348, -37.73348171986721411, 298.1356252759109680 ) ) ;
#58489=EDGE_CURVE ( 'NONE', #48583, #76359, #42785, .T. ) ;
#58491=CARTESIAN_POINT ( 'NONE',  ( 141.0664832912740394, -46.72944715994099596, 14.67562527591100441 ) ) ;
#58494=CARTESIAN_POINT ( 'NONE',  ( 113.8843833678302389, -31.58431642611541434, 218.7638483995049796 ) ) ;
#58495=VERTEX_POINT ( 'NONE', #70804 ) ;
#58498=VERTEX_POINT ( 'NONE', #83993 ) ;
#58499=FACE_BOUND ( 'NONE', #4502, .T. ) ;
#58500=AXIS2_PLACEMENT_3D ( 'NONE', #45606, #11111, #46058 ) ;
#58501=CARTESIAN_POINT ( 'NONE',  ( 98.54782206469626260, -41.97725611773798704, 181.7658570118601915 ) ) ;
#58502=EDGE_CURVE ( 'NONE', #39116, #5214, #70349, .T. ) ;
#58503=CARTESIAN_POINT ( 'NONE',  ( 117.4251315444614789, -36.24242395571268816, 264.8518157521010608 ) ) ;
#58506=FACE_OUTER_BOUND ( 'NONE', #8949, .T. ) ;
#58509=ORIENTED_EDGE ( 'NONE', *, *, #77805, .F. ) ;
#58510=CARTESIAN_POINT ( 'NONE',  ( 105.0948228932018083, -26.91303006142818077, 56.23424190894431973 ) ) ;
#58511=ORIENTED_EDGE ( 'NONE', *, *, #4579, .F. ) ;
#58513=CARTESIAN_POINT ( 'NONE',  ( 99.24357903948710202, -34.39880452655780374, 28.91380465530596311 ) ) ;
#58514=DIRECTION ( 'NONE',  ( 0.000000000000000000, 0.000000000000000000, -1.000000000000000000 ) ) ;
#58515=CARTESIAN_POINT ( 'NONE',  ( 162.9033555647770015, -33.89581943344391135, -5.074374724088000832 ) ) ;
#58516=CYLINDRICAL_SURFACE ( 'NONE', #60428, 0.5000000000000104361 ) ;
#58517=ORIENTED_EDGE ( 'NONE', *, *, #65788, .T. ) ;
#58520=LINE ( 'NONE', #86247, #6371 ) ;
#58521=ORIENTED_EDGE ( 'NONE', *, *, #12811, .T. ) ;
#58522=CARTESIAN_POINT ( 'NONE',  ( 115.2672674329477900, -44.14067019768319966, 83.25372051400698581 ) ) ;
#58525=CARTESIAN_POINT ( 'NONE',  ( 106.6171843113225606, -27.68451483556421522, 44.55051506617196821 ) ) ;
#58526=ADVANCED_FACE ( 'NONE', ( #85787 ), #16729, .T. ) ;
#58527=CARTESIAN_POINT ( 'NONE',  ( 130.5667039024480118, -37.98819715994094537, 218.8274735512161158 ) ) ;
#58528=CARTESIAN_POINT ( 'NONE',  ( 115.2337707449818680, -33.21411712777100433, 75.58158330589692753 ) ) ;
#58530=CARTESIAN_POINT ( 'NONE',  ( 41.56648329127381203, -27.82844715994070484, 21.92562527591199739 ) ) ;
#58532=CARTESIAN_POINT ( 'NONE',  ( 99.96594057013267332, -44.39231554709003547, 42.98133956162492098 ) ) ;
#58533=LINE ( 'NONE', #9511, #74257 ) ;
#58534=VERTEX_POINT ( 'NONE', #79869 ) ;
#58537=ORIENTED_EDGE ( 'NONE', *, *, #35830, .T. ) ;
#58538=CARTESIAN_POINT ( 'NONE',  ( 102.6793653923444651, -46.92506852294805952, 133.2651490854349561 ) ) ;
#58539=DIRECTION ( 'NONE',  ( 0.000000000000000000, 0.000000000000000000, -1.000000000000000000 ) ) ;
#58540=CIRCLE ( 'NONE', #4870, 2.517500000000005844 ) ;
#58541=VERTEX_POINT ( 'NONE', #29465 ) ;
#58542=EDGE_LOOP ( 'NONE', ( #71097, #35529, #23566, #57598 ) ) ;
#58544=DIRECTION ( 'NONE',  ( 1.000000000000000000, 3.999999999999999995E-14, 1.000000000000000078E-15 ) ) ;
#58545=CARTESIAN_POINT ( 'NONE',  ( 116.8310051202518309, -36.16593252570070405, 228.8727681330539667 ) ) ;
#58547=CYLINDRICAL_SURFACE ( 'NONE', #37468, 1.000000000000000888 ) ;
#58548=CARTESIAN_POINT ( 'NONE',  ( 117.9887704088505274, -38.42580343310776669, 64.69181575210097890 ) ) ;
#58550=VERTEX_POINT ( 'NONE', #57147 ) ;
#58551=CARTESIAN_POINT ( 'NONE',  ( 112.7461304981565036, -28.44177779729672295, 170.5981271715937169 ) ) ;
#58553=EDGE_LOOP ( 'NONE', ( #13415, #76912, #54278, #17951 ) ) ;
#58555=PLANE ( 'NONE',  #2510 ) ;
#58556=VECTOR ( 'NONE', #47981, 1000.000000000000000 ) ;
#58558=CARTESIAN_POINT ( 'NONE',  ( 96.70388795518319114, -35.81005419191407668, 231.2556252759109725 ) ) ;
#58560=CYLINDRICAL_SURFACE ( 'NONE', #2612, 9.999999999999998224 ) ;
#58561=CARTESIAN_POINT ( 'NONE',  ( 115.4795240695424923, -35.25402295475319647, 243.3867055423619661 ) ) ;
#58563=CARTESIAN_POINT ( 'NONE',  ( 101.1541078795468707, -28.12664281037979208, 46.55562527591094835 ) ) ;
#58565=CARTESIAN_POINT ( 'NONE',  ( 102.2925893952339749, -26.70832846991215703, 140.4422919425769578 ) ) ;
#58567=FACE_OUTER_BOUND ( 'NONE', #26498, .T. ) ;
#58568=VERTEX_POINT ( 'NONE', #22662 ) ;
#58569=CARTESIAN_POINT ( 'NONE',  ( 63.56670390244714497, -40.82844715994014706, 129.9678068554150911 ) ) ;
#58570=CIRCLE ( 'NONE', #48365, 2.500000000000002220 ) ;
#58571=CARTESIAN_POINT ( 'NONE',  ( 160.7738106836350482, -48.62134037874900372, 180.4678068554150059 ) ) ;
#58572=FACE_OUTER_BOUND ( 'NONE', #2826, .T. ) ;
#58575=VERTEX_POINT ( 'NONE', #50336 ) ;
#58576=CARTESIAN_POINT ( 'NONE',  ( 164.9212702847350158, -29.73316016639540749, -5.074374724088000832 ) ) ;
#58579=ORIENTED_EDGE ( 'NONE', *, *, #56966, .T. ) ;
#58580=CARTESIAN_POINT ( 'NONE',  ( 97.52207955639441650, -32.48083311392049666, 100.9927681330539713 ) ) ;
#58582=DIRECTION ( 'NONE',  ( 0.000000000000000000, 0.000000000000000000, -1.000000000000000000 ) ) ;
#58584=EDGE_CURVE ( 'NONE', #18085, #37957, #9463, .T. ) ;
#58586=ORIENTED_EDGE ( 'NONE', *, *, #44504, .F. ) ;
#58589=DIRECTION ( 'NONE',  ( 0.9963424814100680926, -0.08544974978095730422, 0.000000000000000000 ) ) ;
#58590=CARTESIAN_POINT ( 'NONE',  ( 97.81170668756638520, -40.51744870325870806, 152.6352702516163902 ) ) ;
#58591=EDGE_CURVE ( 'NONE', #52987, #46735, #57259, .T. ) ;
#58593=CARTESIAN_POINT ( 'NONE',  ( 107.0664832912739399, -36.72944715994095333, 294.6356252759106837 ) ) ;
#58594=FACE_OUTER_BOUND ( 'NONE', #88068, .T. ) ;
#58595=DIRECTION ( 'NONE',  ( 0.000000000000000000, 0.000000000000000000, 1.000000000000000000 ) ) ;
#58597=ORIENTED_EDGE ( 'NONE', *, *, #44822, .T. ) ;
#58599=AXIS2_PLACEMENT_3D ( 'NONE', #27842, #48264, #53396 ) ;
#58600=CARTESIAN_POINT ( 'NONE',  ( 97.81168736999980240, -40.51740164104307240, 32.63591986563997693 ) ) ;
#58602=CARTESIAN_POINT ( 'NONE',  ( 98.71823956546970180, -31.63334453281608916, 166.8899109901959719 ) ) ;
#58603=DIRECTION ( 'NONE',  ( 1.000000000000000078E-15, 1.000000000000000083E-30, -1.000000000000000000 ) ) ;
#58604=ORIENTED_EDGE ( 'NONE', *, *, #76253, .T. ) ;
#58605=CARTESIAN_POINT ( 'NONE',  ( 100.8224265971273326, -29.20115443902030705, 36.62705384733894221 ) ) ;
#58606=CARTESIAN_POINT ( 'NONE',  ( 192.5667039024474434, -23.42844715993433624, 180.4678068554150343 ) ) ;
#58608=DIRECTION ( 'NONE',  ( 0.000000000000000000, 0.000000000000000000, -1.000000000000000000 ) ) ;
#58610=EDGE_LOOP ( 'NONE', ( #3698, #29796 ) ) ;
#58612=ORIENTED_EDGE ( 'NONE', *, *, #63237, .T. ) ;
#58614=CARTESIAN_POINT ( 'NONE',  ( 98.87114546532168902, -41.32433164768560374, 178.1768214011349585 ) ) ;
#58616=LINE ( 'NONE', #24124, #57458 ) ;
#58617=CARTESIAN_POINT ( 'NONE',  ( 114.5680773229086782, -32.01199386431652272, 30.70444044875397793 ) ) ;
#58620=CIRCLE ( 'NONE', #61474, 4.750000000000004441 ) ;
#58621=CARTESIAN_POINT ( 'NONE',  ( 102.0670549667728579, -27.97049805557078983, 80.48979194197387699 ) ) ;
#58622=DIRECTION ( 'NONE',  ( 0.7071067811866258435, -0.7071067811864693020, 7.071067811866266166E-16 ) ) ;
#58624=ORIENTED_EDGE ( 'NONE', *, *, #53863, .T. ) ;
#58625=LINE ( 'NONE', #43209, #33308 ) ;
#58626=FACE_OUTER_BOUND ( 'NONE', #1100, .T. ) ;
#58627=VERTEX_POINT ( 'NONE', #88004 ) ;
#58628=CARTESIAN_POINT ( 'NONE',  ( 116.1995025514324169, -41.78438384397603045, 263.4241967044824833 ) ) ;
#58630=VERTEX_POINT ( 'NONE', #81209 ) ;
#58631=EDGE_CURVE ( 'NONE', #48907, #9592, #6496, .T. ) ;
#58633=CARTESIAN_POINT ( 'NONE',  ( 29.56648329127298069, -71.37844715994266664, 342.9256252759109884 ) ) ;
#58634=DIRECTION ( 'NONE',  ( 0.000000000000000000, 0.000000000000000000, -1.000000000000000000 ) ) ;
#58635=PLANE ( 'NONE',  #25950 ) ;
#58637=CARTESIAN_POINT ( 'NONE',  ( 96.07947519314286922, -35.15364532898842498, 222.2251490854349640 ) ) ;
#58639=ORIENTED_EDGE ( 'NONE', *, *, #45855, .F. ) ;
#58640=CARTESIAN_POINT ( 'NONE',  ( 106.5158076061070460, -25.64367904723916780, 41.12800622829193742 ) ) ;
#58641=CARTESIAN_POINT ( 'NONE',  ( 97.81170669197712186, -40.51744871389600178, 156.6352702525290681 ) ) ;
#58642=CARTESIAN_POINT ( 'NONE',  ( 95.23113311243525914, -37.33357626913954164, 271.3670538473393776 ) ) ;
#58643=VERTEX_POINT ( 'NONE', #73922 ) ;
#58644=CARTESIAN_POINT ( 'NONE',  ( 78.88274585166558950, -39.21170328186890686, 8.006085407565089795 ) ) ;
#58645=CARTESIAN_POINT ( 'NONE',  ( 97.84282136733131097, -40.59266849988905079, 17.64178760023652970 ) ) ;
#58647=CARTESIAN_POINT ( 'NONE',  ( 108.7800423072870046, -44.73859216708707720, 105.5623760838769698 ) ) ;
#58648=CARTESIAN_POINT ( 'NONE',  ( 116.8778831976698882, -40.31743973661899361, 214.5470538473389581 ) ) ;
#58649=CYLINDRICAL_SURFACE ( 'NONE', #5801, 0.5000000000000129896 ) ;
#58650=EDGE_LOOP ( 'NONE', ( #67473, #58072 ) ) ;
#58651=AXIS2_PLACEMENT_3D ( 'NONE', #73754, #39672, #17891 ) ;
#58653=VERTEX_POINT ( 'NONE', #62412 ) ;
#58655=AXIS2_PLACEMENT_3D ( 'NONE', #1418, #37726, #57248 ) ;
#58657=VERTEX_POINT ( 'NONE', #47086 ) ;
#58659=FACE_OUTER_BOUND ( 'NONE', #22434, .T. ) ;
#58661=CARTESIAN_POINT ( 'NONE',  ( 46.83715912545424231, -47.82818131006082751, 300.4678068554150059 ) ) ;
#58662=CARTESIAN_POINT ( 'NONE',  ( 103.8954607204944693, -27.23986633091804777, 41.33311113083999544 ) ) ;
#58663=CARTESIAN_POINT ( 'NONE',  ( 103.9030524752275397, -44.69467205304180624, 116.6981341137909567 ) ) ;
#58664=CARTESIAN_POINT ( 'NONE',  ( 112.2192032947272509, -26.89661630634724432, 14.68038718067299442 ) ) ;
#58667=CARTESIAN_POINT ( 'NONE',  ( 103.2783699128477934, -27.47470799093264660, 136.3856377475192687 ) ) ;
#58668=VERTEX_POINT ( 'NONE', #67552 ) ;
#58669=DIRECTION ( 'NONE',  ( -2.999999999999999839E-15, 1.000000000000000000, -2.999999999999999900E-30 ) ) ;
#58670=CARTESIAN_POINT ( 'NONE',  ( 117.0721904964497355, -35.46492929623623525, 33.92731048517197934 ) ) ;
#58671=CARTESIAN_POINT ( 'NONE',  ( 188.5667039024485518, -48.82844715993430640, 170.7178068554150059 ) ) ;
#58672=EDGE_CURVE ( 'NONE', #72716, #38840, #12146, .T. ) ;
#58673=CARTESIAN_POINT ( 'NONE',  ( 107.0664832912739399, -36.72944715994095333, 294.6356252759106837 ) ) ;
#58675=VERTEX_POINT ( 'NONE', #68003 ) ;
#58676=CARTESIAN_POINT ( 'NONE',  ( 105.8935610739654010, -47.12417332243212087, 282.4870538473394390 ) ) ;
#58677=CIRCLE ( 'NONE', #23899, 2.117000000000000881 ) ;
#58678=CARTESIAN_POINT ( 'NONE',  ( 118.6189051447874903, -33.88680481589229743, 10.01848241876795953 ) ) ;
#58679=AXIS2_PLACEMENT_3D ( 'NONE', #73025, #51230, #3993 ) ;
#58682=EDGE_CURVE ( 'NONE', #36659, #27646, #7008, .T. ) ;
#58686=EDGE_CURVE ( 'NONE', #49816, #14401, #68166, .T. ) ;
#58688=PLANE ( 'NONE',  #44075 ) ;
#58691=CYLINDRICAL_SURFACE ( 'NONE', #17011, 2.500000000000002220 ) ;
#58693=DIRECTION ( 'NONE',  ( 0.000000000000000000, 0.000000000000000000, -1.000000000000000000 ) ) ;
#58695=CARTESIAN_POINT ( 'NONE',  ( 97.44607596320715004, -32.59944340835617282, 16.00419670448194154 ) ) ;
#58696=CARTESIAN_POINT ( 'NONE',  ( 115.0396333253530230, -29.07419673827904916, 185.4232443235299570 ) ) ;
#58697=CARTESIAN_POINT ( 'NONE',  ( 117.4762281475856724, -37.96087228405902181, 49.73276813305393773 ) ) ;
#58698=CARTESIAN_POINT ( 'NONE',  ( 78.13314995793999174, 12.92155284005730387, 361.9756252759109998 ) ) ;
#58699=FACE_OUTER_BOUND ( 'NONE', #31085, .T. ) ;
#58700=CARTESIAN_POINT ( 'NONE',  ( 80.71968614772352169, -34.05633243510678909, 1.689562801603114339 ) ) ;
#58703=CARTESIAN_POINT ( 'NONE',  ( 115.8254323940393107, -31.73001883393573053, 185.2397919421337633 ) ) ;
#58704=VERTEX_POINT ( 'NONE', #7457 ) ;
#58705=EDGE_CURVE ( 'NONE', #36809, #57891, #68944, .T. ) ;
#58706=CARTESIAN_POINT ( 'NONE',  ( 99.16769444712207360, -43.44866735504064081, 72.89943479971999807 ) ) ;
#58708=ORIENTED_EDGE ( 'NONE', *, *, #11323, .F. ) ;
#58709=CARTESIAN_POINT ( 'NONE',  ( 193.0374249753375011, -23.42844715993432558, 249.9678068554149775 ) ) ;
#58710=CARTESIAN_POINT ( 'NONE',  ( 110.1310368924891208, -26.13358316477614451, 210.8403871806729626 ) ) ;
#58711=PLANE ( 'NONE',  #87497 ) ;
#58712=LINE ( 'NONE', #44190, #833 ) ;
#58714=CARTESIAN_POINT ( 'NONE',  ( 33.78309357196401663, -29.99615139349950965, -5.074374724088000832 ) ) ;
#58716=FACE_OUTER_BOUND ( 'NONE', #37309, .T. ) ;
#58717=CARTESIAN_POINT ( 'NONE',  ( 116.8035579096021337, -34.12169190864647561, 99.03416637764169650 ) ) ;
#58718=CARTESIAN_POINT ( 'NONE',  ( 117.0460787713799817, -39.54838250520750620, 143.6194347997209775 ) ) ;
#58719=ORIENTED_EDGE ( 'NONE', *, *, #21911, .F. ) ;
#58720=EDGE_LOOP ( 'NONE', ( #75573, #57322 ) ) ;
#58722=CARTESIAN_POINT ( 'NONE',  ( 100.6361971157895283, -42.82696290926312344, 78.36158330589692866 ) ) ;
#58723=DIRECTION ( 'NONE',  ( 0.000000000000000000, 0.000000000000000000, -1.000000000000000000 ) ) ;
#58724=CARTESIAN_POINT ( 'NONE',  ( 116.7002268312855051, -35.03994406823841246, 239.9641967044819637 ) ) ;
#58726=VECTOR ( 'NONE', #66626, 1000.000000000000000 ) ;
#58727=LINE ( 'NONE', #10154, #71082 ) ;
#58730=CYLINDRICAL_SURFACE ( 'NONE', #12478, 9.999999999999998224 ) ;
#58733=CARTESIAN_POINT ( 'NONE',  ( 114.3286968523004248, -29.23113535793732254, 174.4641967044819637 ) ) ;
#58734=VERTEX_POINT ( 'NONE', #35147 ) ;
#58735=ORIENTED_EDGE ( 'NONE', *, *, #79577, .T. ) ;
#58737=CARTESIAN_POINT ( 'NONE',  ( 100.9546728785971794, -28.70702567698208085, 151.5939586026250083 ) ) ;
#58740=EDGE_CURVE ( 'NONE', #20535, #43140, #43754, .T. ) ;
#58741=VECTOR ( 'NONE', #59166, 1000.000000000000000 ) ;
#58742=CARTESIAN_POINT ( 'NONE',  ( 127.0664832912740394, -46.72944715994101017, -5.074374724089008915 ) ) ;
#58745=CARTESIAN_POINT ( 'NONE',  ( 114.9651742339629976, -29.92520496456729262, 184.3927681330539770 ) ) ;
#58746=CARTESIAN_POINT ( 'NONE',  ( 107.0664832912739968, -36.72944715994100306, 287.6356252759109680 ) ) ;
#58747=ORIENTED_EDGE ( 'NONE', *, *, #6340, .F. ) ;
#58748=ORIENTED_EDGE ( 'NONE', *, *, #81004, .T. ) ;
#58750=AXIS2_PLACEMENT_3D ( 'NONE', #46174, #66181, #65737 ) ;
#58751=CARTESIAN_POINT ( 'NONE',  ( 97.81475986870147210, -40.52492237179531287, 62.63673496744226554 ) ) ;
#58753=CARTESIAN_POINT ( 'NONE',  ( 131.0667039024480118, -61.87844715994100397, 204.3338068554149913 ) ) ;
#58754=CARTESIAN_POINT ( 'NONE',  ( 115.1548909598205057, -41.51005587062507374, 279.8453928297065545 ) ) ;
#58756=CARTESIAN_POINT ( 'NONE',  ( 41.56648329127399677, -18.82844715994099971, 138.9256252759119832 ) ) ;
#58757=ORIENTED_EDGE ( 'NONE', *, *, #46185, .T. ) ;
#58758=ADVANCED_FACE ( 'NONE', ( #84230 ), #41954, .T. ) ;
#58760=CARTESIAN_POINT ( 'NONE',  ( 115.0845091798801008, -41.07331283931524268, 9.635625275910939536 ) ) ;
#58764=ADVANCED_FACE ( 'NONE', ( #1550, #49669 ), #70586, .T. ) ;
#58766=VERTEX_POINT ( 'NONE', #51018 ) ;
#58768=CARTESIAN_POINT ( 'NONE',  ( 113.2433956935301467, -28.75706466399318373, 155.5522588166994069 ) ) ;
#58769=CIRCLE ( 'NONE', #25452, 3.600000000000000089 ) ;
#58770=CARTESIAN_POINT ( 'NONE',  ( 98.58513254605244924, -37.74079342042374918, 40.84384839950494239 ) ) ;
#58771=CARTESIAN_POINT ( 'NONE',  ( 106.9748012750099946, -47.17635858745483546, 187.5699109901969734 ) ) ;
#58772=CARTESIAN_POINT ( 'NONE',  ( 98.87380182923577365, -30.31772012733808808, 155.7984824187679465 ) ) ;
#58773=DIRECTION ( 'NONE',  ( -0.5180656453708486486, -0.02186357193551463976, -0.8550613845266940016 ) ) ;
#58774=CARTESIAN_POINT ( 'NONE',  ( 96.80890382254112581, -40.84721887859184619, 247.6422919425769749 ) ) ;
#58775=CARTESIAN_POINT ( 'NONE',  ( 104.4081952550981214, -46.45811700621415241, 98.36623602494283602 ) ) ;
#58780=CARTESIAN_POINT ( 'NONE',  ( 114.1546619933443480, -29.02461823700197741, 199.4841967044819739 ) ) ;
#58782=CARTESIAN_POINT ( 'NONE',  ( 102.8439234467419965, -46.26134197790700853, 177.2441967044819648 ) ) ;
#58784=CARTESIAN_POINT ( 'NONE',  ( 73.10937651008745775, -46.62589376934776908, 14.92562527591095645 ) ) ;
#58788=DIRECTION ( 'NONE',  ( 0.000000000000000000, 0.000000000000000000, 1.000000000000000000 ) ) ;
#58790=CARTESIAN_POINT ( 'NONE',  ( 100.0388059118473052, -29.01104360887439526, 281.6641967044822650 ) ) ;
#58792=EDGE_CURVE ( 'NONE', #27930, #37713, #71045, .T. ) ;
#58793=DIRECTION ( 'NONE',  ( 1.000000000000000078E-15, 0.000000000000000000, 1.000000000000000000 ) ) ;
#58798=DIRECTION ( 'NONE',  ( 0.000000000000000000, 0.000000000000000000, -1.000000000000000000 ) ) ;
#58799=CARTESIAN_POINT ( 'NONE',  ( 107.6136016015418448, -44.72672411580607132, 195.5838068554169524 ) ) ;
#58801=ADVANCED_FACE ( 'NONE', ( #78311 ), #87813, .F. ) ;
#58802=CARTESIAN_POINT ( 'NONE',  ( 135.2096432771652701, -21.23067567606553752, 8.021372095561345006 ) ) ;
#58803=CARTESIAN_POINT ( 'NONE',  ( 113.0348518357461955, -45.34727401701223926, 203.0584824187679374 ) ) ;
#58804=CARTESIAN_POINT ( 'NONE',  ( 108.9852221676114539, -46.97644323546262513, 78.72419670448194040 ) ) ;
#58805=CARTESIAN_POINT ( 'NONE',  ( 118.1276453766531915, -32.34061975111649190, 245.1270538473389706 ) ) ;
#58806=CARTESIAN_POINT ( 'NONE',  ( 168.5667039024483529, -48.82844715993496720, 180.4678068554150059 ) ) ;
#58807=DIRECTION ( 'NONE',  ( 1.000000000000000078E-15, -1.000000000000000000, 0.000000000000000000 ) ) ;
#58810=DIRECTION ( 'NONE',  ( 0.7071067811869283792, -0.7071067811861665442, 7.071067811869291448E-16 ) ) ;
#58811=CYLINDRICAL_SURFACE ( 'NONE', #43602, 0.5000000000000031086 ) ;
#58816=CIRCLE ( 'NONE', #24019, 0.5000000000000004441 ) ;
#58818=VERTEX_POINT ( 'NONE', #77851 ) ;
#58821=AXIS2_PLACEMENT_3D ( 'NONE', #32902, #1977, #29674 ) ;
#58822=CARTESIAN_POINT ( 'NONE',  ( 115.1410662219050067, -33.85660664540706222, 113.5209912566479744 ) ) ;
#58823=CARTESIAN_POINT ( 'NONE',  ( 97.81168895331838087, -40.51742574516882200, 287.6356252759109680 ) ) ;
#58824=ORIENTED_EDGE ( 'NONE', *, *, #13399, .T. ) ;
#58825=CARTESIAN_POINT ( 'NONE',  ( 112.5028774994481466, -27.85959465031284310, 90.63848241876793566 ) ) ;
#58827=AXIS2_PLACEMENT_3D ( 'NONE', #61959, #19300, #39723 ) ;
#58830=AXIS2_PLACEMENT_3D ( 'NONE', #6783, #75827, #34932 ) ;
#58831=CARTESIAN_POINT ( 'NONE',  ( 116.7468388360755966, -38.12735696270561903, 28.71276813305495423 ) ) ;
#58832=ORIENTED_EDGE ( 'NONE', *, *, #53234, .T. ) ;
#58833=ORIENTED_EDGE ( 'NONE', *, *, #5227, .T. ) ;
#58834=ORIENTED_EDGE ( 'NONE', *, *, #62872, .T. ) ;
#58835=LINE ( 'NONE', #72044, #3654 ) ;
#58836=CARTESIAN_POINT ( 'NONE',  ( 73.06648329127396835, -46.72944715994108122, -4.970821333495798022 ) ) ;
#58837=CARTESIAN_POINT ( 'NONE',  ( 115.8254323921038491, -31.73001882920818773, 115.2397919425400232 ) ) ;
#58839=CIRCLE ( 'NONE', #19688, 2.124999999999994227 ) ;
#58840=DIRECTION ( 'NONE',  ( -0.02150753337723538411, -0.0009076677972193728959, -0.9997682742251812194 ) ) ;
#58842=DIRECTION ( 'NONE',  ( 1.000000000000000078E-15, 1.000000000000000083E-30, -1.000000000000000000 ) ) ;
#58844=CARTESIAN_POINT ( 'NONE',  ( 117.0705705820184477, -32.08379757587633208, 59.16038718067295576 ) ) ;
#58845=VERTEX_POINT ( 'NONE', #83774 ) ;
#58847=DIRECTION ( 'NONE',  ( 4.299999999999999979E-14, -1.000000000000000000, 4.400000000000000367E-29 ) ) ;
#58848=DIRECTION ( 'NONE',  ( 0.000000000000000000, 0.000000000000000000, 1.000000000000000000 ) ) ;
#58851=CARTESIAN_POINT ( 'NONE',  ( 112.1548083954980939, -43.14751820055241893, 165.9280903695909615 ) ) ;
#58856=EDGE_LOOP ( 'NONE', ( #54798, #77417, #56060, #14516 ) ) ;
#58857=ORIENTED_EDGE ( 'NONE', *, *, #10737, .F. ) ;
#58858=CARTESIAN_POINT ( 'NONE',  ( 131.3164832912739826, -18.72944715994100662, 6.749768910606465333 ) ) ;
#58860=ORIENTED_EDGE ( 'NONE', *, *, #24163, .F. ) ;
#58862=CARTESIAN_POINT ( 'NONE',  ( 101.0667092185316989, -28.63788266170726260, 182.0158690201829756 ) ) ;
#58864=CARTESIAN_POINT ( 'NONE',  ( 100.9546728989441533, -28.70702566177422455, 120.5939586006224431 ) ) ;
#58865=CARTESIAN_POINT ( 'NONE',  ( 110.8538822462197970, -45.98447871898064676, 17.88557456161885639 ) ) ;
#58867=VERTEX_POINT ( 'NONE', #39176 ) ;
#58868=ADVANCED_FACE ( 'NONE', ( #24221, #18280 ), #59163, .F. ) ;
#58869=AXIS2_PLACEMENT_3D ( 'NONE', #29589, #36852, #3234 ) ;
#58872=ORIENTED_EDGE ( 'NONE', *, *, #18026, .F. ) ;
#58873=CARTESIAN_POINT ( 'NONE',  ( 104.3825147926133354, -28.50161402210781603, 208.1576141791150008 ) ) ;
#58874=CARTESIAN_POINT ( 'NONE',  ( 117.1128946550982732, -32.06414332788899912, 59.16038718067295576 ) ) ;
#58875=CARTESIAN_POINT ( 'NONE',  ( 99.16013801855501697, -43.49098322490566204, 31.88991099019594699 ) ) ;
#58878=DIRECTION ( 'NONE',  ( 0.000000000000000000, 2.135044278125299371E-15, -1.000000000000000000 ) ) ;
#58879=CARTESIAN_POINT ( 'NONE',  ( 117.2380278806138278, -39.01742120631563893, 144.6499109901969859 ) ) ;
#58880=DIRECTION ( 'NONE',  ( 0.000000000000000000, 0.000000000000000000, -1.000000000000000000 ) ) ;
#58883=ORIENTED_EDGE ( 'NONE', *, *, #78299, .T. ) ;
#58885=DIRECTION ( 'NONE',  ( -1.000000000000000078E-15, 1.000000000000000083E-30, 1.000000000000000000 ) ) ;
#58887=ORIENTED_EDGE ( 'NONE', *, *, #3979, .T. ) ;
#58888=CARTESIAN_POINT ( 'NONE',  ( 19.56670390244824631, -47.82844715994191631, 300.4678068554150059 ) ) ;
#58889=CARTESIAN_POINT ( 'NONE',  ( 97.81541071992751313, -32.74985850689276390, 132.0034678584867436 ) ) ;
#58890=CARTESIAN_POINT ( 'NONE',  ( 97.77227622453175115, -32.00665715170008951, 50.95276813305294183 ) ) ;
#58894=DIRECTION ( 'NONE',  ( 1.000000000000000000, -5.337610695313248426E-16, 0.000000000000000000 ) ) ;
#58895=CARTESIAN_POINT ( 'NONE',  ( 116.3624975636024317, -33.68846805112525544, 89.07848241876791917 ) ) ;
#58896=DIRECTION ( 'NONE',  ( 0.000000000000000000, 1.000000000000000000, 0.000000000000000000 ) ) ;
#58897=CARTESIAN_POINT ( 'NONE',  ( 97.44537786355549258, -42.12371753947135744, 177.7451490854349743 ) ) ;
#58898=CARTESIAN_POINT ( 'NONE',  ( 97.07197965290352215, -35.37934377285892396, 61.21903046452214880 ) ) ;
#58900=FACE_OUTER_BOUND ( 'NONE', #63975, .T. ) ;
#58902=CARTESIAN_POINT ( 'NONE',  ( 97.80893753052176010, -40.51861053356429920, 37.63533870039827178 ) ) ;
#58903=LINE ( 'NONE', #52520, #60147 ) ;
#58904=EDGE_CURVE ( 'NONE', #49439, #8126, #48620, .T. ) ;
#58905=CARTESIAN_POINT ( 'NONE',  ( 100.9551865876383090, -28.70660340941259037, 135.5938645509268383 ) ) ;
#58906=CARTESIAN_POINT ( 'NONE',  ( 188.5667039024483529, -48.82844715993431350, 295.7178068554150059 ) ) ;
#58907=CARTESIAN_POINT ( 'NONE',  ( 97.72299786849482928, -41.53060059208619492, 196.7041967044819728 ) ) ;
#58909=EDGE_CURVE ( 'NONE', #63964, #63276, #45084, .T. ) ;
#58910=CARTESIAN_POINT ( 'NONE',  ( 97.60798650947359079, -39.98270781540073671, 146.5900883612529810 ) ) ;
#58911=CARTESIAN_POINT ( 'NONE',  ( 110.8246185410185944, -26.31015614812341141, 245.7889586092439629 ) ) ;
#58912=CARTESIAN_POINT ( 'NONE',  ( 97.79748285543813324, -31.86337989110288405, 131.9413395616259947 ) ) ;
#58914=CARTESIAN_POINT ( 'NONE',  ( 82.59390026530674334, -37.81452881268462107, 7.047625865511941257 ) ) ;
#58915=PLANE ( 'NONE',  #73282 ) ;
#58917=ORIENTED_EDGE ( 'NONE', *, *, #68136, .T. ) ;
#58918=ORIENTED_EDGE ( 'NONE', *, *, #54174, .T. ) ;
#58919=ORIENTED_EDGE ( 'NONE', *, *, #11842, .T. ) ;
#58920=EDGE_CURVE ( 'NONE', #54314, #63468, #25542, .T. ) ;
#58921=ORIENTED_EDGE ( 'NONE', *, *, #47390, .T. ) ;
#58922=CARTESIAN_POINT ( 'NONE',  ( 108.3334480812130352, -46.73485935584395889, 72.67729194148455463 ) ) ;
#58923=CARTESIAN_POINT ( 'NONE',  ( 102.3792474187797694, -47.61030217832540501, 283.2527681330539053 ) ) ;
#58924=CARTESIAN_POINT ( 'NONE',  ( 172.5664832912740110, -32.07844715994070839, 198.9256252759119832 ) ) ;
#58925=ADVANCED_FACE ( 'NONE', ( #79201 ), #65978, .F. ) ;
#58926=CARTESIAN_POINT ( 'NONE',  ( 132.2189018279138679, -34.68450975841484052, 2.186797062530981162 ) ) ;
#58927=DIRECTION ( 'NONE',  ( 1.000000000000000078E-15, -1.000000000000000083E-30, -1.000000000000000000 ) ) ;
#58929=VECTOR ( 'NONE', #31279, 1000.000000000000000 ) ;
#58930=CARTESIAN_POINT ( 'NONE',  ( 100.0786887504289666, -31.81753722825460429, 205.2609912566479693 ) ) ;
#58931=ORIENTED_EDGE ( 'NONE', *, *, #72390, .T. ) ;
#58932=EDGE_LOOP ( 'NONE', ( #17396, #2150, #40176, #13759, #22137, #59014 ) ) ;
#58934=ORIENTED_EDGE ( 'NONE', *, *, #8509, .T. ) ;
#58935=CIRCLE ( 'NONE', #82196, 4.750000000000004441 ) ;
#58936=VECTOR ( 'NONE', #43329, 1000.000000000000000 ) ;
#58937=FACE_BOUND ( 'NONE', #36551, .T. ) ;
#58938=AXIS2_PLACEMENT_3D ( 'NONE', #38194, #71835, #9599 ) ;
#58939=B_SPLINE_CURVE_WITH_KNOTS ( 'NONE', 3,
 ( #28063, #48937, #56665, #84409, #30762, #72103, #58889, #58016, #52504, #43925, #80270, #23523, #80710, #32089, #72981, #59785, #71662, #9425, #73426, #4401, #85752, #31645, #64838, #10748, #51186, #59345 ),
 .UNSPECIFIED., .F., .F.,
 ( 4, 2, 2, 2, 2, 2, 2, 2, 2, 2, 2, 2, 4 ),
 ( 0.4999451768748383040, 0.5624520297654835854, 0.6249588826561287558, 0.6874657355467740372, 0.7499725884374193186, 0.7812260148827419037, 0.8124794413280644889, 0.8437328677733870741, 0.8749862942187095483, 0.9062397206640322445, 0.9374931471093547186, 0.9687465735546774148, 1.000000000000000000 ),
 .UNSPECIFIED. ) ;
#58940=DIRECTION ( 'NONE',  ( 1.000000000000000000, 4.237773401492740281E-14, 0.000000000000000000 ) ) ;
#58941=CYLINDRICAL_SURFACE ( 'NONE', #53291, 4.875000000000017764 ) ;
#58942=CARTESIAN_POINT ( 'NONE',  ( 102.4274648318396146, -45.67098835673295554, 13.62729759161196341 ) ) ;
#58944=CARTESIAN_POINT ( 'NONE',  ( 62.56670390244743629, -48.82844715994018969, 180.4678068554151196 ) ) ;
#58945=FACE_BOUND ( 'NONE', #47892, .T. ) ;
#58946=ORIENTED_EDGE ( 'NONE', *, *, #6012, .F. ) ;
#58947=CARTESIAN_POINT ( 'NONE',  ( 97.06385931607105988, -37.34243354152794581, 57.37519869820856400 ) ) ;
#58948=ORIENTED_EDGE ( 'NONE', *, *, #45551, .T. ) ;
#58949=VECTOR ( 'NONE', #35088, 1000.000000000000000 ) ;
#58951=CARTESIAN_POINT ( 'NONE',  ( 100.2991084500796575, -40.90897653417852098, 9.586185607686982024 ) ) ;
#58953=CARTESIAN_POINT ( 'NONE',  ( 176.7669697523286061, -48.62818131005482059, 300.4678068554149490 ) ) ;
#58954=EDGE_CURVE ( 'NONE', #89309, #26329, #66879, .T. ) ;
#58955=CARTESIAN_POINT ( 'NONE',  ( 152.0371591254585724, -47.82818131005588214, 117.4678068554150485 ) ) ;
#58956=LINE ( 'NONE', #64903, #19864 ) ;
#58957=ORIENTED_EDGE ( 'NONE', *, *, #85804, .T. ) ;
#58961=CARTESIAN_POINT ( 'NONE',  ( 102.3603858057123972, -46.03211757857948783, 127.2041967044829960 ) ) ;
#58963=CARTESIAN_POINT ( 'NONE',  ( 102.2122376447956213, -29.66627497393060509, 49.97813411379098625 ) ) ;
#58965=CARTESIAN_POINT ( 'NONE',  ( 101.8615262650677522, -29.55750872133152640, 72.00729759161094989 ) ) ;
#58966=LINE ( 'NONE', #23599, #78185 ) ;
#58969=AXIS2_PLACEMENT_3D ( 'NONE', #65791, #79905, #43560 ) ;
#58970=CARTESIAN_POINT ( 'NONE',  ( 106.2504415414193488, -26.27893178022805998, 21.13848241876792144 ) ) ;
#58971=CARTESIAN_POINT ( 'NONE',  ( 184.5667039024550888, -48.82844715994099971, 180.4678068554150343 ) ) ;
#58972=ORIENTED_EDGE ( 'NONE', *, *, #7476, .T. ) ;
#58974=ORIENTED_EDGE ( 'NONE', *, *, #82972, .F. ) ;
#58976=CARTESIAN_POINT ( 'NONE',  ( 62.03715912545634836, -23.42818131006021787, 180.4678068554151196 ) ) ;
#58977=ORIENTED_EDGE ( 'NONE', *, *, #51912, .T. ) ;
#58980=CARTESIAN_POINT ( 'NONE',  ( 97.48942487598446860, -34.74365074496812156, 216.1641967044829755 ) ) ;
#58981=CARTESIAN_POINT ( 'NONE',  ( 99.89301282343141963, -29.72232929382336053, 125.7099027331620960 ) ) ;
#58983=CARTESIAN_POINT ( 'NONE',  ( 97.77247047105220190, -32.00675585678803969, 46.95276813305393659 ) ) ;
#58985=EDGE_LOOP ( 'NONE', ( #35743, #21114 ) ) ;
#58986=CARTESIAN_POINT ( 'NONE',  ( 110.1977257015883822, -27.19759275805366627, 170.8237533411364382 ) ) ;
#58988=VECTOR ( 'NONE', #70741, 1000.000000000000000 ) ;
#58991=VECTOR ( 'NONE', #35120, 1000.000000000000000 ) ;
#58995=CARTESIAN_POINT ( 'NONE',  ( 96.54020141486694229, -31.34005042439572009, 245.9499109901969689 ) ) ;
#58996=CARTESIAN_POINT ( 'NONE',  ( 163.5667039024460223, -22.48495420874110806, 342.9256252759119548 ) ) ;
#58997=AXIS2_PLACEMENT_3D ( 'NONE', #61643, #42542, #28945 ) ;
#58998=EDGE_CURVE ( 'NONE', #18060, #38962, #31909, .T. ) ;
#58999=CARTESIAN_POINT ( 'NONE',  ( 83.06670390244796920, -64.87844715994098976, 225.9838068554150254 ) ) ;
#59000=DIRECTION ( 'NONE',  ( 4.299999999999999979E-14, -1.000000000000000000, 0.000000000000000000 ) ) ;
#59001=CARTESIAN_POINT ( 'NONE',  ( 115.5572469886287479, -35.80043457063792545, 278.3352769709341032 ) ) ;
#59003=CARTESIAN_POINT ( 'NONE',  ( 117.0854383170105564, -39.53109055650221393, 94.60991099019693706 ) ) ;
#59005=CARTESIAN_POINT ( 'NONE',  ( 98.80516515778722919, -28.16326830255935221, 115.6870538473389587 ) ) ;
#59006=VERTEX_POINT ( 'NONE', #37849 ) ;
#59008=EDGE_LOOP ( 'NONE', ( #76860, #43409, #36940, #9453, #75002 ) ) ;
#59010=CYLINDRICAL_SURFACE ( 'NONE', #68243, 9.999999999999998224 ) ;
#59011=B_SPLINE_CURVE_WITH_KNOTS ( 'NONE', 3,
 ( #59107, #31859, #87285, #59551, #11879, #45469 ),
 .UNSPECIFIED., .F., .F.,
 ( 4, 2, 4 ),
 ( 0.000000000000000000, 0.5000000000000000000, 1.000000000000000000 ),
 .UNSPECIFIED. ) ;
#59014=ORIENTED_EDGE ( 'NONE', *, *, #29123, .T. ) ;
#59016=CARTESIAN_POINT ( 'NONE',  ( 110.1710482807090585, -46.72786414817543488, 97.81562527591097478 ) ) ;
#59017=ORIENTED_EDGE ( 'NONE', *, *, #85815, .F. ) ;
#59019=DIRECTION ( 'NONE',  ( -0.000000000000000000, -0.000000000000000000, 1.000000000000000000 ) ) ;
#59020=AXIS2_PLACEMENT_3D ( 'NONE', #84063, #43588, #9098 ) ;
#59022=ORIENTED_EDGE ( 'NONE', *, *, #32811, .T. ) ;
#59023=CARTESIAN_POINT ( 'NONE',  ( 118.9289135900544494, -36.16662986141290048, 118.8641967044819836 ) ) ;
#59024=SURFACE_SIDE_STYLE ('',( #10891 ) ) ;
#59025=DIRECTION ( 'NONE',  ( -4.299999999999999979E-14, 1.000000000000000000, 0.000000000000000000 ) ) ;
#59029=EDGE_CURVE ( 'NONE', #49695, #62712, #86390, .T. ) ;
#59030=ORIENTED_EDGE ( 'NONE', *, *, #71995, .T. ) ;
#59031=CYLINDRICAL_SURFACE ( 'NONE', #79465, 2.999999999999999112 ) ;
#59032=EDGE_CURVE ( 'NONE', #84350, #26697, #31458, .T. ) ;
#59033=CARTESIAN_POINT ( 'NONE',  ( 188.5667039024479834, -67.87844715994100397, 257.2178068554150059 ) ) ;
#59034=EDGE_CURVE ( 'NONE', #82293, #68666, #44191, .T. ) ;
#59035=FACE_OUTER_BOUND ( 'NONE', #76568, .T. ) ;
#59042=CARTESIAN_POINT ( 'NONE',  ( 165.2748236753140247, -30.08671355700301575, -5.074374724088000832 ) ) ;
#59043=CARTESIAN_POINT ( 'NONE',  ( 113.2095242374419541, -45.08419629851108823, 179.0689586092439640 ) ) ;
#59044=CYLINDRICAL_SURFACE ( 'NONE', #73362, 3.250000000000002665 ) ;
#59046=CARTESIAN_POINT ( 'NONE',  ( 115.1412022171004281, -43.23618977845870148, 39.27467289495795200 ) ) ;
#59047=DIRECTION ( 'NONE',  ( 0.000000000000000000, 0.000000000000000000, -1.000000000000000000 ) ) ;
#59049=ORIENTED_EDGE ( 'NONE', *, *, #85322, .F. ) ;
#59051=AXIS2_PLACEMENT_3D ( 'NONE', #64751, #57930, #50665 ) ;
#59052=VECTOR ( 'NONE', #88134, 1000.000000000000000 ) ;
#59054=ORIENTED_EDGE ( 'NONE', *, *, #34124, .F. ) ;
#59055=CARTESIAN_POINT ( 'NONE',  ( 99.81674604704261355, -31.63341061165540680, 202.2701547344679796 ) ) ;
#59057=CARTESIAN_POINT ( 'NONE',  ( 116.1804594027163375, -40.96476762480074996, 25.56312527591098060 ) ) ;
#59059=VECTOR ( 'NONE', #8852, 1000.000000000000000 ) ;
#59062=CARTESIAN_POINT ( 'NONE',  ( 51.56670390244799762, -33.35206098992650681, -5.074374724088000832 ) ) ;
#59063=CARTESIAN_POINT ( 'NONE',  ( 41.56648329127398966, -18.82844715994071194, 198.9256252759119832 ) ) ;
#59066=CARTESIAN_POINT ( 'NONE',  ( 115.8196560889659139, -31.72004084542335534, 35.23981128565909415 ) ) ;
#59067=ORIENTED_EDGE ( 'NONE', *, *, #15977, .T. ) ;
#59068=CARTESIAN_POINT ( 'NONE',  ( 115.8883252675857847, -30.10835006627621269, 264.3508633711492735 ) ) ;
#59070=VERTEX_POINT ( 'NONE', #82328 ) ;
#59071=AXIS2_PLACEMENT_3D ( 'NONE', #4403, #58453, #86183 ) ;
#59072=DIRECTION ( 'NONE',  ( 1.000000000000000000, 4.299999999999999979E-14, 1.000000000000000078E-15 ) ) ;
#59073=DIRECTION ( 'NONE',  ( 0.000000000000000000, 0.000000000000000000, -1.000000000000000000 ) ) ;
#59075=CIRCLE ( 'NONE', #67783, 3.299999999999997158 ) ;
#59077=AXIS2_PLACEMENT_3D ( 'NONE', #77569, #62589, #29426 ) ;
#59078=CARTESIAN_POINT ( 'NONE',  ( 116.4163124136858443, -41.43834035574819552, 199.4556252759109611 ) ) ;
#59080=AXIS2_PLACEMENT_3D ( 'NONE', #76111, #77023, #13890 ) ;
#59081=ORIENTED_EDGE ( 'NONE', *, *, #80079, .F. ) ;
#59082=CARTESIAN_POINT ( 'NONE',  ( 100.3832715781272356, -28.67167693828054453, 36.62705384733894221 ) ) ;
#59083=EDGE_CURVE ( 'NONE', #29939, #49937, #54448, .T. ) ;
#59085=CARTESIAN_POINT ( 'NONE',  ( 97.21658504226680009, -33.31410993950169086, 286.0613395616252888 ) ) ;
#59087=ORIENTED_EDGE ( 'NONE', *, *, #29402, .T. ) ;
#59089=CARTESIAN_POINT ( 'NONE',  ( 81.70522810116327150, -16.51875982968476109, 2.060081176871058517 ) ) ;
#59090=CARTESIAN_POINT ( 'NONE',  ( 97.92325040394680968, -40.78074430601089517, 17.65808851064360141 ) ) ;
#59091=CARTESIAN_POINT ( 'NONE',  ( 115.0352805544412718, -42.91097007997968404, 153.3027619676027484 ) ) ;
#59092=CARTESIAN_POINT ( 'NONE',  ( 99.95702547362903090, -40.74009991652987139, 134.5538046553059530 ) ) ;
#59093=CARTESIAN_POINT ( 'NONE',  ( 101.6393319275751992, -45.65599671332518028, 243.1413395616249886 ) ) ;
#59094=ADVANCED_FACE ( 'NONE', ( #40517 ), #60500, .F. ) ;
#59096=ORIENTED_EDGE ( 'NONE', *, *, #47725, .F. ) ;
#59097=ADVANCED_FACE ( 'NONE', ( #41399 ), #53672, .T. ) ;
#59098=CARTESIAN_POINT ( 'NONE',  ( 136.1637134158967513, -38.51083119283578071, 2.376725019071385336 ) ) ;
#59101=ORIENTED_EDGE ( 'NONE', *, *, #69384, .F. ) ;
#59103=EDGE_CURVE ( 'NONE', #2140, #42491, #34143, .T. ) ;
#59107=CARTESIAN_POINT ( 'NONE',  ( 116.3212776292296127, -32.94146857471318413, 10.13562527591094309 ) ) ;
#59108=LINE ( 'NONE', #59552, #15316 ) ;
#59109=ADVANCED_FACE ( 'NONE', ( #6021 ), #12833, .F. ) ;
#59110=CARTESIAN_POINT ( 'NONE',  ( 49.21213752015856358, -29.73316016639572368, 193.9678068554150911 ) ) ;
#59111=CARTESIAN_POINT ( 'NONE',  ( 108.8156685800011303, -28.36903548837926792, 139.3352769709339896 ) ) ;
#59112=CARTESIAN_POINT ( 'NONE',  ( 96.64195684025510502, -42.47035700268206426, 26.72705384733997747 ) ) ;
#59113=ORIENTED_EDGE ( 'NONE', *, *, #73381, .T. ) ;
#59116=EDGE_CURVE ( 'NONE', #28057, #36904, #5138, .T. ) ;
#59117=ORIENTED_EDGE ( 'NONE', *, *, #56137, .F. ) ;
#59118=DIRECTION ( 'NONE',  ( 0.000000000000000000, 1.000000000000000000, 0.000000000000000000 ) ) ;
#59119=EDGE_LOOP ( 'NONE', ( #41100, #51557, #41231, #5495 ) ) ;
#59120=CARTESIAN_POINT ( 'NONE',  ( 97.81493411881378108, -40.51644251795452334, 167.6359250042934264 ) ) ;
#59121=DIRECTION ( 'NONE',  ( 2.900000000000000265E-14, -2.000000000000000155E-15, 1.000000000000000000 ) ) ;
#59122=CARTESIAN_POINT ( 'NONE',  ( 80.06648329127401098, -41.22944715994105280, 4.925625275910944012 ) ) ;
#59125=ORIENTED_EDGE ( 'NONE', *, *, #18270, .F. ) ;
#59126=CARTESIAN_POINT ( 'NONE',  ( 102.3791524630845799, -47.61053145109372764, 287.2527681330536780 ) ) ;
#59127=CARTESIAN_POINT ( 'NONE',  ( 106.2487395568334421, -26.25713557174866253, 21.13848241876792144 ) ) ;
#59130=FACE_OUTER_BOUND ( 'NONE', #77435, .T. ) ;
#59132=CARTESIAN_POINT ( 'NONE',  ( 193.0374249753375011, -23.42844715993432558, 249.9678068554149775 ) ) ;
#59133=DIRECTION ( 'NONE',  ( 0.000000000000000000, 1.000000000000000000, 0.000000000000000000 ) ) ;
#59137=ADVANCED_FACE ( 'NONE', ( #20091 ), #89577, .T. ) ;
#59140=VECTOR ( 'NONE', #67839, 1000.000000000000000 ) ;
#59142=CARTESIAN_POINT ( 'NONE',  ( 98.38709084977145380, -42.09077886617859576, 11.76800622829193799 ) ) ;
#59143=CARTESIAN_POINT ( 'NONE',  ( 96.85852386828889848, -34.61283385893091236, 212.1641967044819808 ) ) ;
#59144=CARTESIAN_POINT ( 'NONE',  ( 115.0392540076567656, -43.53489519176116573, 59.26419670448196086 ) ) ;
#59145=AXIS2_PLACEMENT_3D ( 'NONE', #2795, #38630, #37306 ) ;
#59147=EDGE_CURVE ( 'NONE', #37193, #79159, #74845, .T. ) ;
#59149=DIRECTION ( 'NONE',  ( 1.000000000000000000, 4.299999999999999979E-14, 1.000000000000000078E-15 ) ) ;
#59150=CARTESIAN_POINT ( 'NONE',  ( 116.3212776292270973, -32.94146857470704504, 49.13562527591097506 ) ) ;
#59151=CARTESIAN_POINT ( 'NONE',  ( 33.91903122894498779, -35.91149509761220315, -5.074374724088000832 ) ) ;
#59152=AXIS2_PLACEMENT_3D ( 'NONE', #50457, #22327, #72603 ) ;
#59153=ORIENTED_EDGE ( 'NONE', *, *, #46582, .F. ) ;
#59154=DIRECTION ( 'NONE',  ( 0.000000000000000000, 0.000000000000000000, -1.000000000000000000 ) ) ;
#59156=CARTESIAN_POINT ( 'NONE',  ( 115.5638989210037124, -29.55965564860111527, 70.38419670448092802 ) ) ;
#59157=DIRECTION ( 'NONE',  ( 1.000000000000000000, 4.299999999999999979E-14, 1.000000000000000078E-15 ) ) ;
#59158=ORIENTED_EDGE ( 'NONE', *, *, #42702, .F. ) ;
#59159=PLANE ( 'NONE',  #85306 ) ;
#59160=CARTESIAN_POINT ( 'NONE',  ( 115.4423046205436094, -29.55243945206544609, 225.4022919425769658 ) ) ;
#59161=CARTESIAN_POINT ( 'NONE',  ( 98.54715120129765182, -41.97616799658815268, 252.7661222402538499 ) ) ;
#59162=CARTESIAN_POINT ( 'NONE',  ( 107.0667039024479834, -36.72944715994100306, 239.5838068554170093 ) ) ;
#59163=PLANE ( 'NONE',  #16752 ) ;
#59164=CARTESIAN_POINT ( 'NONE',  ( 80.06648329127398256, -15.97944715994105813, 8.225625275910942946 ) ) ;
#59165=DIRECTION ( 'NONE',  ( -1.000000000000000078E-15, 1.000000000000000083E-30, 1.000000000000000000 ) ) ;
#59166=DIRECTION ( 'NONE',  ( -1.000000000000000000, -3.999999999999999995E-14, -1.000000000000000078E-15 ) ) ;
#59167=CARTESIAN_POINT ( 'NONE',  ( 96.71010325458811963, -37.26253042779857338, 121.3794347997209684 ) ) ;
#59168=AXIS2_PLACEMENT_3D ( 'NONE', #65467, #38642, #58205 ) ;
#59169=ORIENTED_EDGE ( 'NONE', *, *, #69116, .T. ) ;
#59170=VERTEX_POINT ( 'NONE', #32804 ) ;
#59171=AXIS2_PLACEMENT_3D ( 'NONE', #468, #49040, #21366 ) ;
#59172=CARTESIAN_POINT ( 'NONE',  ( 107.8890265924388814, -27.36996276949999185, 106.4263452106589654 ) ) ;
#59173=DIRECTION ( 'NONE',  ( -3.360405532702990443E-14, 1.000000000000000000, 0.000000000000000000 ) ) ;
#59174=CARTESIAN_POINT ( 'NONE',  ( 116.2522929705882859, -40.08866370952546987, 214.5470538473389581 ) ) ;
#59175=DIRECTION ( 'NONE',  ( 1.000000000000000000, 3.999999999999999995E-14, 1.000000000000000078E-15 ) ) ;
#59179=FACE_OUTER_BOUND ( 'NONE', #44291, .T. ) ;
#59181=CARTESIAN_POINT ( 'NONE',  ( 61.68306511546570903, -72.55869591834559174, 542.9756252759101471 ) ) ;
#59182=CARTESIAN_POINT ( 'NONE',  ( 114.4965984691701664, -29.44205611023136626, 149.4441967044819819 ) ) ;
#59183=EDGE_LOOP ( 'NONE', ( #54385, #66752, #69344, #8417 ) ) ;
#59186=CARTESIAN_POINT ( 'NONE',  ( 115.0889047306568074, -30.61763669006579747, 150.3439586082987205 ) ) ;
#59191=VECTOR ( 'NONE', #69886, 1000.000000000000000 ) ;
#59192=CYLINDRICAL_SURFACE ( 'NONE', #34985, 0.2500000000000039968 ) ;
#59194=CARTESIAN_POINT ( 'NONE',  ( 98.16810232779933187, -31.29751870953477422, 170.8899109901960003 ) ) ;
#59197=ORIENTED_EDGE ( 'NONE', *, *, #16874, .F. ) ;
#59198=EDGE_LOOP ( 'NONE', ( #6624, #59158, #332, #39056 ) ) ;
#59199=ORIENTED_EDGE ( 'NONE', *, *, #76976, .T. ) ;
#59200=AXIS2_PLACEMENT_3D ( 'NONE', #10061, #37768, #65021 ) ;
#59202=CARTESIAN_POINT ( 'NONE',  ( 117.0649963017320090, -35.84647789964886755, 64.89715894876896130 ) ) ;
#59203=DIRECTION ( 'NONE',  ( 0.000000000000000000, 0.000000000000000000, 1.000000000000000000 ) ) ;
#59205=CARTESIAN_POINT ( 'NONE',  ( 101.2699428795238106, -44.12381293138377458, 273.4911071154209594 ) ) ;
#59206=CIRCLE ( 'NONE', #62134, 4.874999999999990230 ) ;
#59208=CARTESIAN_POINT ( 'NONE',  ( 118.5256205435842958, -36.72944715994100306, 300.2406250056037038 ) ) ;
#59209=ORIENTED_EDGE ( 'NONE', *, *, #21925, .F. ) ;
#59213=CARTESIAN_POINT ( 'NONE',  ( 81.63820548406826560, -16.47341874818874174, 7.827313014937786306 ) ) ;
#59216=EDGE_CURVE ( 'NONE', #23298, #71348, #49106, .T. ) ;
#59219=VERTEX_POINT ( 'NONE', #76835 ) ;
#59220=CARTESIAN_POINT ( 'NONE',  ( 115.8239080365019902, -31.72738345397822002, 155.2397836611081061 ) ) ;
#59221=CIRCLE ( 'NONE', #27331, 2.517500000000000071 ) ;
#59222=CARTESIAN_POINT ( 'NONE',  ( 105.5073833390055853, -45.15143093073633196, 11.85241982807799843 ) ) ;
#59223=CARTESIAN_POINT ( 'NONE',  ( 108.6784406349466110, -26.40724015326817664, 189.9527681330539792 ) ) ;
#59224=CARTESIAN_POINT ( 'NONE',  ( 101.9951592035502017, -45.85337710724439830, 187.1727681330539781 ) ) ;
#59225=DIRECTION ( 'NONE',  ( 1.000000000000000000, 3.999999999999999995E-14, 1.000000000000000078E-15 ) ) ;
#59226=CARTESIAN_POINT ( 'NONE',  ( 109.2119659639152047, -48.38412513495681111, 273.7213395616252569 ) ) ;
#59227=CARTESIAN_POINT ( 'NONE',  ( 100.8875087413080678, -44.70025551109045381, 98.05342680442112169 ) ) ;
#59229=ORIENTED_EDGE ( 'NONE', *, *, #49249, .F. ) ;
#59231=ORIENTED_EDGE ( 'NONE', *, *, #63667, .F. ) ;
#59234=ADVANCED_FACE ( 'NONE', ( #78204 ), #49555, .F. ) ;
#59236=CARTESIAN_POINT ( 'NONE',  ( 112.4772085026190354, -45.73365988577116070, 238.0070538473389377 ) ) ;
#59238=CARTESIAN_POINT ( 'NONE',  ( 97.42502596350711030, -42.13512825026991493, 181.7451490854349743 ) ) ;
#59239=DIRECTION ( 'NONE',  ( 0.000000000000000000, 0.000000000000000000, -1.000000000000000000 ) ) ;
#59242=DIRECTION ( 'NONE',  ( -0.9963424814100679816, 0.08544974978095724871, 0.000000000000000000 ) ) ;
#59245=CARTESIAN_POINT ( 'NONE',  ( 112.3272512417296554, -28.22507648531182056, 285.6356252759109680 ) ) ;
#59246=CYLINDRICAL_SURFACE ( 'NONE', #29273, 4.875000000000017764 ) ;
#59252=CARTESIAN_POINT ( 'NONE',  ( 99.02250180400051249, -33.12202411512905798, 195.5838068554173788 ) ) ;
#59253=VERTEX_POINT ( 'NONE', #35944 ) ;
#59254=AXIS2_PLACEMENT_3D ( 'NONE', #81174, #33886, #12562 ) ;
#59255=DIRECTION ( 'NONE',  ( -1.000000000000000078E-15, 0.000000000000000000, -1.000000000000000000 ) ) ;
#59256=CARTESIAN_POINT ( 'NONE',  ( 96.65194983638532733, -35.53535514585328059, 206.2356252759109623 ) ) ;
#59257=CARTESIAN_POINT ( 'NONE',  ( 103.2054172826541816, -46.45125265344608323, 113.2756252759109827 ) ) ;
#59258=CARTESIAN_POINT ( 'NONE',  ( 109.3463552500793554, -26.51205201248422583, 220.9013395616249795 ) ) ;
#59259=FACE_OUTER_BOUND ( 'NONE', #43045, .T. ) ;
#59260=EDGE_CURVE ( 'NONE', #29962, #32906, #29141, .T. ) ;
#59262=CARTESIAN_POINT ( 'NONE',  ( 172.5664832912729878, -27.82844715994070484, 198.9256252759119832 ) ) ;
#59263=CARTESIAN_POINT ( 'NONE',  ( 51.42025729304100423, -33.70561438051981185, 237.4678068554150059 ) ) ;
#59264=FACE_OUTER_BOUND ( 'NONE', #10794, .T. ) ;
#59265=CARTESIAN_POINT ( 'NONE',  ( 126.0667039024479266, -14.72944715994094977, 239.5838068554170377 ) ) ;
#59266=CARTESIAN_POINT ( 'NONE',  ( 97.78115606164335816, -40.44200917047258770, 66.62962555244023122 ) ) ;
#59270=CARTESIAN_POINT ( 'NONE',  ( 103.3727720482000620, -29.02797788616916108, 94.85527697093499455 ) ) ;
#59271=VECTOR ( 'NONE', #63118, 1000.000000000000000 ) ;
#59273=ORIENTED_EDGE ( 'NONE', *, *, #88043, .F. ) ;
#59274=CARTESIAN_POINT ( 'NONE',  ( 109.2504006710444173, -46.93703897017532967, 103.7441967044829880 ) ) ;
#59275=CARTESIAN_POINT ( 'NONE',  ( 51.34673845256598668, -29.62846900982231446, 342.9256252759119548 ) ) ;
#59276=CARTESIAN_POINT ( 'NONE',  ( 32.24491389929978169, -32.11662333284649407, 117.4678068554150485 ) ) ;
#59277=EDGE_CURVE ( 'NONE', #41907, #74757, #55464, .T. ) ;
#59278=CARTESIAN_POINT ( 'NONE',  ( 112.1393456483219921, -28.01282278529340530, 175.6564586086265933 ) ) ;
#59279=VECTOR ( 'NONE', #78943, 1000.000000000000000 ) ;
#59280=CARTESIAN_POINT ( 'NONE',  ( 100.9974734301594310, -29.01720366022859565, 15.60705384733995871 ) ) ;
#59281=EDGE_LOOP ( 'NONE', ( #65046, #73044, #62126, #31618, #81570, #57702, #32736, #3440, #84379, #70033, #17454, #19634 ) ) ;
#59282=ORIENTED_EDGE ( 'NONE', *, *, #51439, .T. ) ;
#59283=ORIENTED_EDGE ( 'NONE', *, *, #79689, .T. ) ;
#59284=ADVANCED_FACE ( 'NONE', ( #22328 ), #43192, .F. ) ;
#59286=CARTESIAN_POINT ( 'NONE',  ( 102.8912152862170188, -46.22186109533342346, 128.2346728949579528 ) ) ;
#59287=DIRECTION ( 'NONE',  ( 1.000000000000000078E-15, -1.000000000000000083E-30, -1.000000000000000000 ) ) ;
#59289=DIRECTION ( 'NONE',  ( 0.000000000000000000, 0.000000000000000000, -1.000000000000000000 ) ) ;
#59290=AXIS2_PLACEMENT_3D ( 'NONE', #2163, #42567, #70761 ) ;
#59291=CARTESIAN_POINT ( 'NONE',  ( 107.0664832912739968, 22.62155284005901024, 327.8006252759110453 ) ) ;
#59294=CARTESIAN_POINT ( 'NONE',  ( 117.9019101119220068, -41.46671778014666643, 58.49848241876792798 ) ) ;
#59296=ORIENTED_EDGE ( 'NONE', *, *, #69189, .F. ) ;
#59300=CARTESIAN_POINT ( 'NONE',  ( 102.9190449779222405, -43.75998617602524376, 159.9709475124489586 ) ) ;
#59301=CIRCLE ( 'NONE', #53445, 0.5000000000000004441 ) ;
#59303=EDGE_CURVE ( 'NONE', #30460, #9382, #60297, .T. ) ;
#59305=ORIENTED_EDGE ( 'NONE', *, *, #14117, .T. ) ;
#59306=VERTEX_POINT ( 'NONE', #70027 ) ;
#59307=CARTESIAN_POINT ( 'NONE',  ( 141.0664832912739826, -8.729447159940995959, 14.92562527591100618 ) ) ;
#59309=EDGE_LOOP ( 'NONE', ( #3925, #13185, #78583, #7394 ) ) ;
#59310=ORIENTED_EDGE ( 'NONE', *, *, #81525, .F. ) ;
#59311=LINE ( 'NONE', #31609, #75295 ) ;
#59312=CARTESIAN_POINT ( 'NONE',  ( 109.0885512386393259, -27.55405797182273631, 176.3234880678019465 ) ) ;
#59314=EDGE_CURVE ( 'NONE', #89556, #43538, #85468, .T. ) ;
#59315=CARTESIAN_POINT ( 'NONE',  ( 194.5667039024482108, -40.82844715993405060, 180.4678068554150343 ) ) ;
#59316=DIRECTION ( 'NONE',  ( 1.000000000000000000, 0.000000000000000000, 0.000000000000000000 ) ) ;
#59317=LINE ( 'NONE', #25702, #14020 ) ;
#59318=VECTOR ( 'NONE', #2219, 1000.000000000000000 ) ;
#59319=ORIENTED_EDGE ( 'NONE', *, *, #43210, .F. ) ;
#59322=EDGE_CURVE ( 'NONE', #24293, #48080, #85907, .T. ) ;
#59323=ORIENTED_EDGE ( 'NONE', *, *, #86029, .T. ) ;
#59324=ORIENTED_EDGE ( 'NONE', *, *, #40651, .F. ) ;
#59326=CARTESIAN_POINT ( 'NONE',  ( 99.25992742994408502, -40.46556956555936324, 214.5118998934009653 ) ) ;
#59327=VECTOR ( 'NONE', #465, 1000.000000000000000 ) ;
#59328=CARTESIAN_POINT ( 'NONE',  ( 107.9474950258210413, -25.68774170017952940, 115.0251490854349612 ) ) ;
#59329=CARTESIAN_POINT ( 'NONE',  ( 104.2468583329775669, -46.74335657891444384, 22.35848241876792031 ) ) ;
#59330=DIRECTION ( 'NONE',  ( 6.745093096447288888E-17, 1.000000000000000000, -3.328006943901140051E-31 ) ) ;
#59331=CARTESIAN_POINT ( 'NONE',  ( 106.6155744189988326, -25.27918481551454732, 323.5352776872487652 ) ) ;
#59333=CARTESIAN_POINT ( 'NONE',  ( 113.6144894440835031, -28.61735105040022376, 160.5356252759109736 ) ) ;
#59335=ORIENTED_EDGE ( 'NONE', *, *, #44551, .T. ) ;
#59336=LINE ( 'NONE', #26614, #56857 ) ;
#59339=VECTOR ( 'NONE', #57923, 1000.000000000000000 ) ;
#59340=DIRECTION ( 'NONE',  ( 0.000000000000000000, 0.000000000000000000, -1.000000000000000000 ) ) ;
#59341=VERTEX_POINT ( 'NONE', #44980 ) ;
#59343=CARTESIAN_POINT ( 'NONE',  ( 19.56648329127400032, -18.82844715994099971, -5.074374724088000832 ) ) ;
#59345=CARTESIAN_POINT ( 'NONE',  ( 116.3192736897089645, -32.94707975126958388, 130.1356252759109680 ) ) ;
#59346=CARTESIAN_POINT ( 'NONE',  ( 100.9430784815160251, -28.29197455274081463, 75.57562527591093726 ) ) ;
#59348=CARTESIAN_POINT ( 'NONE',  ( 87.31648329127403940, -46.47944715994105280, -5.074374724089048883 ) ) ;
#59350=CARTESIAN_POINT ( 'NONE',  ( 104.0406618471960201, -46.06530165129709076, 82.32705384733995402 ) ) ;
#59351=DIRECTION ( 'NONE',  ( -1.110223024625155531E-13, -1.000000000000000000, 0.000000000000000000 ) ) ;
#59352=CARTESIAN_POINT ( 'NONE',  ( 98.56907362037671305, -44.95393718666134930, 187.9384824187679612 ) ) ;
#59353=CARTESIAN_POINT ( 'NONE',  ( 102.0648915419311606, -27.97176698159946184, 60.48998952755263758 ) ) ;
#59355=ORIENTED_EDGE ( 'NONE', *, *, #48109, .T. ) ;
#59357=CARTESIAN_POINT ( 'NONE',  ( 48.45959712127301344, -26.00627455219131789, -5.074374724088000832 ) ) ;
#59358=LINE ( 'NONE', #80283, #28255 ) ;
#59359=DIRECTION ( 'NONE',  ( 0.000000000000000000, 0.000000000000000000, 1.000000000000000000 ) ) ;
#59360=DIRECTION ( 'NONE',  ( 0.000000000000000000, 0.000000000000000000, -1.000000000000000000 ) ) ;
#59361=CARTESIAN_POINT ( 'NONE',  ( 109.3464976042218524, -26.51141404309336735, 224.9013395616249511 ) ) ;
#59364=CARTESIAN_POINT ( 'NONE',  ( 106.2251562910655309, -47.77378392694726017, 263.5280062282920994 ) ) ;
#59365=CARTESIAN_POINT ( 'NONE',  ( 102.3735796352302714, -26.67091080359734434, 131.4118157521009778 ) ) ;
#59366=FACE_OUTER_BOUND ( 'NONE', #56641, .T. ) ;
#59367=EDGE_CURVE ( 'NONE', #70652, #66586, #38178, .T. ) ;
#59371=ORIENTED_EDGE ( 'NONE', *, *, #61563, .F. ) ;
#59372=ORIENTED_EDGE ( 'NONE', *, *, #20290, .T. ) ;
#59373=VERTEX_POINT ( 'NONE', #86786 ) ;
#59374=ORIENTED_EDGE ( 'NONE', *, *, #50801, .F. ) ;
#59375=CARTESIAN_POINT ( 'NONE',  ( 116.7951252702546441, -39.38782979486860825, 73.61479194218726718 ) ) ;
#59376=CARTESIAN_POINT ( 'NONE',  ( 99.39693184722126773, -28.77005263954443492, 261.6746728949588032 ) ) ;
#59378=CARTESIAN_POINT ( 'NONE',  ( 131.6688901780889864, -35.37024878623139301, 2.654395752964708866 ) ) ;
#59382=CARTESIAN_POINT ( 'NONE',  ( 112.0552156641497703, -28.39979068407086515, 204.0695626852199496 ) ) ;
#59385=AXIS2_PLACEMENT_3D ( 'NONE', #36473, #2398, #55524 ) ;
#59386=AXIS2_PLACEMENT_3D ( 'NONE', #72847, #58324, #3369 ) ;
#59387=ORIENTED_EDGE ( 'NONE', *, *, #82675, .T. ) ;
#59388=EDGE_CURVE ( 'NONE', #89037, #60619, #44084, .T. ) ;
#59390=CARTESIAN_POINT ( 'NONE',  ( 110.8543111526358018, -45.98430318780785342, 182.8856114468024145 ) ) ;
#59392=CARTESIAN_POINT ( 'NONE',  ( 99.72008180067200556, -41.26785689822659009, 8.199678543991950619 ) ) ;
#59395=DIRECTION ( 'NONE',  ( -1.000000000000000000, -4.299999999999999979E-14, -1.000000000000000078E-15 ) ) ;
#59396=CARTESIAN_POINT ( 'NONE',  ( 142.8838050580813501, -82.11588141944041297, 542.9756252759101471 ) ) ;
#59398=CARTESIAN_POINT ( 'NONE',  ( 103.2800637878028454, -27.47401470249857880, 56.38549218839290234 ) ) ;
#59401=CARTESIAN_POINT ( 'NONE',  ( 107.0664832912750057, -36.72944715993903486, 9.125625275910969947 ) ) ;
#59402=CARTESIAN_POINT ( 'NONE',  ( 115.6923476351215641, -37.43328618085965331, 36.59189989340094940 ) ) ;
#59406=ADVANCED_FACE ( 'NONE', ( #45415 ), #72711, .F. ) ;
#59407=AXIS2_PLACEMENT_3D ( 'NONE', #57110, #58455, #29430 ) ;
#59409=ORIENTED_EDGE ( 'NONE', *, *, #16411, .T. ) ;
#59410=DIRECTION ( 'NONE',  ( -4.299999999999999979E-14, 1.000000000000000000, -4.128053709984630540E-29 ) ) ;
#59412=ADVANCED_FACE ( 'NONE', ( #25000 ), #44528, .F. ) ;
#59414=CARTESIAN_POINT ( 'NONE',  ( 116.5985118214053813, -29.68807528100325044, 109.3327681330539605 ) ) ;
#59416=EDGE_CURVE ( 'NONE', #87084, #27718, #20382, .T. ) ;
#59417=CARTESIAN_POINT ( 'NONE',  ( 99.32879058785749748, -33.04431300321336806, 75.39527697093394920 ) ) ;
#59418=PLANE ( 'NONE',  #31508 ) ;
#59419=CARTESIAN_POINT ( 'NONE',  ( 109.8610415383596148, -27.05157811987473337, 61.28444044875497099 ) ) ;
#59420=CARTESIAN_POINT ( 'NONE',  ( 61.67079006425787924, -0.9306969701470987344, 394.9756252759102040 ) ) ;
#59421=EDGE_CURVE ( 'NONE', #15206, #66455, #47207, .T. ) ;
#59425=CARTESIAN_POINT ( 'NONE',  ( 96.69309474412473548, -37.96640669985919914, 37.42133956162496844 ) ) ;
#59426=DIRECTION ( 'NONE',  ( 0.000000000000000000, 0.000000000000000000, 1.000000000000000000 ) ) ;
#59428=DIRECTION ( 'NONE',  ( 0.000000000000000000, 0.000000000000000000, 1.000000000000000000 ) ) ;
#59432=VERTEX_POINT ( 'NONE', #88580 ) ;
#59434=AXIS2_PLACEMENT_3D ( 'NONE', #66441, #4228, #71504 ) ;
#59436=CARTESIAN_POINT ( 'NONE',  ( 103.8504807240352790, -26.87063827031080621, 210.3394347997209763 ) ) ;
#59437=CARTESIAN_POINT ( 'NONE',  ( 97.48373141833911859, -33.75867255000157741, 126.0865479483587990 ) ) ;
#59439=CARTESIAN_POINT ( 'NONE',  ( 97.80922128671791427, -29.33095300656633597, 41.78991099019596334 ) ) ;
#59440=CARTESIAN_POINT ( 'NONE',  ( 105.7150778794604662, -46.72380765957736060, 43.46892697967506081 ) ) ;
#59442=CARTESIAN_POINT ( 'NONE',  ( 103.2783743724242811, -27.47470615678986761, 171.3856373841866514 ) ) ;
#59443=CARTESIAN_POINT ( 'NONE',  ( 138.8167039024479834, -50.82844715994100682, 37.63480685541480852 ) ) ;
#59448=CARTESIAN_POINT ( 'NONE',  ( 116.9047011640240754, -41.71676023082953577, 248.4651490854349731 ) ) ;
#59449=DIRECTION ( 'NONE',  ( 1.000000000000000078E-15, -1.000000000000000083E-30, -1.000000000000000000 ) ) ;
#59450=CARTESIAN_POINT ( 'NONE',  ( 152.0371591254582881, -47.82818131005588214, 313.9678068554149490 ) ) ;
#59451=LINE ( 'NONE', #87184, #9868 ) ;
#59452=CARTESIAN_POINT ( 'NONE',  ( 98.43953089107090193, -39.48415132980177589, 280.9828960185531059 ) ) ;
#59454=CARTESIAN_POINT ( 'NONE',  ( 111.0741232671659020, -25.60348521778456288, 95.80133956162495679 ) ) ;
#59456=CARTESIAN_POINT ( 'NONE',  ( 96.56283406263658264, -36.88802528585984675, 136.3384824187679385 ) ) ;
#59457=ORIENTED_EDGE ( 'NONE', *, *, #72937, .T. ) ;
#59458=LINE ( 'NONE', #24956, #32099 ) ;
#59460=AXIS2_PLACEMENT_3D ( 'NONE', #16008, #84161, #21935 ) ;
#59462=CARTESIAN_POINT ( 'NONE',  ( 63.03715912545737865, -24.42818131006027826, 236.4678068554150343 ) ) ;
#59463=CARTESIAN_POINT ( 'NONE',  ( 134.8111839727902748, -34.08035908359602217, 1.709393751551410823 ) ) ;
#59464=ORIENTED_EDGE ( 'NONE', *, *, #485, .F. ) ;
#59465=CARTESIAN_POINT ( 'NONE',  ( 251.6756888531239156, -13.32818131005263140, 117.4678068554150627 ) ) ;
#59466=CARTESIAN_POINT ( 'NONE',  ( 107.6054179116733707, -26.23843464447702090, 95.03562527591097364 ) ) ;
#59467=EDGE_LOOP ( 'NONE', ( #41130, #30450, #23062, #82099 ) ) ;
#59468=CARTESIAN_POINT ( 'NONE',  ( 95.60734603896362671, -36.72944715994100306, 294.6356252759106837 ) ) ;
#59470=CARTESIAN_POINT ( 'NONE',  ( 62.03715912545744260, -47.82818131006020934, 129.9678068554150911 ) ) ;
#59471=EDGE_CURVE ( 'NONE', #12734, #23174, #61789, .T. ) ;
#59472=DIRECTION ( 'NONE',  ( 0.000000000000000000, -1.000000000000000000, 0.000000000000000000 ) ) ;
#59474=CARTESIAN_POINT ( 'NONE',  ( 96.67713595657845360, -37.82845849995531040, 126.4099109901969626 ) ) ;
#59476=ADVANCED_FACE ( 'NONE', ( #46757 ), #5000, .T. ) ;
#59477=DIRECTION ( 'NONE',  ( -1.000000000000000000, -4.299999999999999979E-14, -1.000000000000000078E-15 ) ) ;
#59478=FACE_OUTER_BOUND ( 'NONE', #20665, .T. ) ;
#59480=VECTOR ( 'NONE', #6524, 1000.000000000000000 ) ;
#59483=DIRECTION ( 'NONE',  ( -4.237773401492740281E-14, 1.000000000000000000, 0.000000000000000000 ) ) ;
#59485=CARTESIAN_POINT ( 'NONE',  ( 134.0664832912740110, -8.729447159940999512, 291.1181252759119502 ) ) ;
#59487=FACE_OUTER_BOUND ( 'NONE', #65353, .T. ) ;
#59488=VERTEX_POINT ( 'NONE', #32700 ) ;
#59489=EDGE_CURVE ( 'NONE', #35904, #41861, #57455, .T. ) ;
#59491=DIRECTION ( 'NONE',  ( -4.237773401492740281E-14, 1.000000000000000000, 0.000000000000000000 ) ) ;
#59492=CARTESIAN_POINT ( 'NONE',  ( 107.2322476904470108, -46.54200526979089858, 208.5899109901959605 ) ) ;
#59493=CARTESIAN_POINT ( 'NONE',  ( 106.0715115987692201, -25.31091405536793459, 321.4693626932605071 ) ) ;
#59494=ORIENTED_EDGE ( 'NONE', *, *, #1826, .F. ) ;
#59496=CARTESIAN_POINT ( 'NONE',  ( 96.85055626654755656, -38.51091292166574220, 42.45181575209999636 ) ) ;
#59497=CARTESIAN_POINT ( 'NONE',  ( 109.6427594141682675, -46.48015053188884593, 52.78146225493246391 ) ) ;
#59505=ORIENTED_EDGE ( 'NONE', *, *, #82217, .F. ) ;
#59506=CARTESIAN_POINT ( 'NONE',  ( 112.1317502087781293, -44.64270164792750961, 214.4492023535159717 ) ) ;
#59507=AXIS2_PLACEMENT_3D ( 'NONE', #45480, #65939, #31419 ) ;
#59508=CARTESIAN_POINT ( 'NONE',  ( 98.15076410364456194, -41.26119453264894332, 52.70027500851303159 ) ) ;
#59509=CARTESIAN_POINT ( 'NONE',  ( 107.0664832912739968, -36.72944715994100306, 293.2242906452868851 ) ) ;
#59512=CARTESIAN_POINT ( 'NONE',  ( 81.77804793993006172, -38.88970947304841275, 2.099345637340709114 ) ) ;
#59513=ORIENTED_EDGE ( 'NONE', *, *, #71650, .F. ) ;
#59514=DIRECTION ( 'NONE',  ( -4.237773401492740281E-14, 1.000000000000000000, 0.000000000000000000 ) ) ;
#59515=CARTESIAN_POINT ( 'NONE',  ( 108.4095123903694713, -26.73402528341915030, 35.96903173305258150 ) ) ;
#59516=ORIENTED_EDGE ( 'NONE', *, *, #82620, .T. ) ;
#59517=CARTESIAN_POINT ( 'NONE',  ( 112.1173730388400287, -26.89747643418222722, 19.71086337114896736 ) ) ;
#59523=CARTESIAN_POINT ( 'NONE',  ( 177.4809174648213173, -48.32844715993478957, 300.4678068554149490 ) ) ;
#59524=DIRECTION ( 'NONE',  ( 0.9825752044328148749, 0.1858654557302456822, 0.000000000000000000 ) ) ;
#59525=CARTESIAN_POINT ( 'NONE',  ( 100.6107886340239901, -26.73269172650989489, 216.5327681330539633 ) ) ;
#59528=CARTESIAN_POINT ( 'NONE',  ( 98.61215933031529346, -43.92124142298762735, 72.89943479972099283 ) ) ;
#59529=LINE ( 'NONE', #74971, #32313 ) ;
#59530=VERTEX_POINT ( 'NONE', #80873 ) ;
#59534=EDGE_CURVE ( 'NONE', #41030, #55155, #71935, .T. ) ;
#59535=CIRCLE ( 'NONE', #40680, 2.500000000000002220 ) ;
#59536=CARTESIAN_POINT ( 'NONE',  ( 80.44276116895755990, -15.99866847873249931, 1.641799428525830828 ) ) ;
#59537=FACE_OUTER_BOUND ( 'NONE', #25583, .T. ) ;
#59540=CARTESIAN_POINT ( 'NONE',  ( 115.3951208896509399, -39.08203659613434411, 141.4376141791150019 ) ) ;
#59541=CARTESIAN_POINT ( 'NONE',  ( 106.8511646352646380, -47.80368950967726249, 223.5489586092439538 ) ) ;
#59543=ORIENTED_EDGE ( 'NONE', *, *, #29187, .F. ) ;
#59547=EDGE_LOOP ( 'NONE', ( #10961, #67233, #65610, #9307 ) ) ;
#59548=CARTESIAN_POINT ( 'NONE',  ( 37.03715912545343514, -48.62818131006128652, 180.4678068554150911 ) ) ;
#59549=EDGE_LOOP ( 'NONE', ( #24829, #39996 ) ) ;
#59551=CARTESIAN_POINT ( 'NONE',  ( 117.1166401382700002, -37.03105959670597258, 9.802291942577573636 ) ) ;
#59552=CARTESIAN_POINT ( 'NONE',  ( 49.21437657594998427, -35.91149509761070391, -5.074374724088000832 ) ) ;
#59553=CARTESIAN_POINT ( 'NONE',  ( 97.33767582200576385, -34.07173766446835117, 26.11484643626505786 ) ) ;
#59554=CARTESIAN_POINT ( 'NONE',  ( 108.0589421777836492, -45.73103505524393597, 157.0743245899819556 ) ) ;
#59555=CARTESIAN_POINT ( 'NONE',  ( 116.1589316287842735, -31.54115767207924748, 289.2384824187681716 ) ) ;
#59556=ORIENTED_EDGE ( 'NONE', *, *, #46752, .T. ) ;
#59559=VERTEX_POINT ( 'NONE', #5904 ) ;
#59563=ORIENTED_EDGE ( 'NONE', *, *, #12507, .F. ) ;
#59564=LINE ( 'NONE', #10541, #2998 ) ;
#59565=CARTESIAN_POINT ( 'NONE',  ( 176.7669697523285208, -48.62818131005431610, 180.4678068554150059 ) ) ;
#59566=LINE ( 'NONE', #36910, #69342 ) ;
#59569=ORIENTED_EDGE ( 'NONE', *, *, #72161, .F. ) ;
#59570=CARTESIAN_POINT ( 'NONE',  ( 104.5881283732255156, -26.60288457357396652, 285.2670538473396391 ) ) ;
#59571=CARTESIAN_POINT ( 'NONE',  ( 107.1959371850970086, -26.26158102413311468, 31.06705384733893283 ) ) ;
#59574=EDGE_CURVE ( 'NONE', #16891, #67680, #83542, .T. ) ;
#59575=CARTESIAN_POINT ( 'NONE',  ( 115.8254407911606734, -31.73003342290389028, 145.2401058703679837 ) ) ;
#59578=VECTOR ( 'NONE', #31181, 1000.000000000000000 ) ;
#59579=CYLINDRICAL_SURFACE ( 'NONE', #24271, 0.2499999999999941991 ) ;
#59581=CARTESIAN_POINT ( 'NONE',  ( 117.4985906579250354, -37.96351766657803495, 53.73276813305394484 ) ) ;
#59582=CARTESIAN_POINT ( 'NONE',  ( 117.2274905824790778, -41.08006910540670731, 209.5165776568640013 ) ) ;
#59583=CARTESIAN_POINT ( 'NONE',  ( 110.4636787236150184, -47.27194539037950705, 53.83657765686300678 ) ) ;
#59585=PLANE ( 'NONE',  #86402 ) ;
#59588=EDGE_LOOP ( 'NONE', ( #74540, #37470 ) ) ;
#59589=CYLINDRICAL_SURFACE ( 'NONE', #56266, 4.749999999999976907 ) ;
#59590=VERTEX_POINT ( 'NONE', #54906 ) ;
#59591=AXIS2_PLACEMENT_3D ( 'NONE', #11979, #26489, #5156 ) ;
#59592=CARTESIAN_POINT ( 'NONE',  ( 116.7176835877704093, -38.50936494796416554, 84.68133956162493803 ) ) ;
#59593=ADVANCED_FACE ( 'NONE', ( #63088 ), #77185, .T. ) ;
#59596=VECTOR ( 'NONE', #44969, 1000.000000000000000 ) ;
#59597=DIRECTION ( 'NONE',  ( -1.000000000000000078E-15, 1.000000000000000083E-30, 1.000000000000000000 ) ) ;
#59598=CARTESIAN_POINT ( 'NONE',  ( 103.0988156209413518, -47.86972635628415418, 248.3041967044829619 ) ) ;
#59599=LINE ( 'NONE', #25098, #32364 ) ;
#59602=DIRECTION ( 'NONE',  ( -0.1811243269279065315, 0.9834602067165264527, 0.000000000000000000 ) ) ;
#59603=EDGE_CURVE ( 'NONE', #14767, #17736, #51607, .T. ) ;
#59605=CARTESIAN_POINT ( 'NONE',  ( 133.6902059199477435, -39.46022584114956544, 1.641799370504869238 ) ) ;
#59607=CARTESIAN_POINT ( 'NONE',  ( 116.4500618263486444, -39.48841239489308919, 183.5984824187689526 ) ) ;
#59611=CARTESIAN_POINT ( 'NONE',  ( 98.20536012454746810, -36.63577306554869750, 107.7501547344689783 ) ) ;
#59613=CARTESIAN_POINT ( 'NONE',  ( 152.0368932755772562, -23.42844715993587812, 180.4678068554149775 ) ) ;
#59614=CARTESIAN_POINT ( 'NONE',  ( 107.9555263298577188, -25.64695713395855137, 261.0127681330532710 ) ) ;
#59615=CARTESIAN_POINT ( 'NONE',  ( 152.0371591254582881, -47.82818131005588214, 300.4678068554149490 ) ) ;
#59616=DIRECTION ( 'NONE',  ( 0.000000000000000000, 0.000000000000000000, -1.000000000000000000 ) ) ;
#59618=LINE ( 'NONE', #80542, #55344 ) ;
#59620=CARTESIAN_POINT ( 'NONE',  ( 33.96670390244752014, -28.27351298637434240, 237.4678068554150059 ) ) ;
#59621=FACE_OUTER_BOUND ( 'NONE', #74945, .T. ) ;
#59622=DIRECTION ( 'NONE',  ( -1.346944695195362088E-15, 1.000000000000000000, -3.469446951953620425E-31 ) ) ;
#59623=CARTESIAN_POINT ( 'NONE',  ( 101.4371718687637838, -46.21494532752030437, 207.1622919425779514 ) ) ;
#59626=ORIENTED_EDGE ( 'NONE', *, *, #10510, .F. ) ;
#59628=DIRECTION ( 'NONE',  ( 4.299999999999999979E-14, -1.000000000000000000, 4.400000000000000367E-29 ) ) ;
#59631=FACE_OUTER_BOUND ( 'NONE', #74614, .T. ) ;
#59632=AXIS2_PLACEMENT_3D ( 'NONE', #36149, #34797, #43843 ) ;
#59633=ORIENTED_EDGE ( 'NONE', *, *, #58954, .F. ) ;
#59634=CARTESIAN_POINT ( 'NONE',  ( 97.81170051792484799, -40.51743816602341752, 61.63542871443850402 ) ) ;
#59635=CARTESIAN_POINT ( 'NONE',  ( 113.6857051329922683, -45.58184738042410800, 188.0994347997199725 ) ) ;
#59639=ORIENTED_EDGE ( 'NONE', *, *, #33998, .T. ) ;
#59640=VECTOR ( 'NONE', #79497, 1000.000000000000000 ) ;
#59643=DIRECTION ( 'NONE',  ( 0.000000000000000000, 1.000000000000000000, 0.000000000000000000 ) ) ;
#59644=EDGE_CURVE ( 'NONE', #17950, #31900, #84004, .T. ) ;
#59645=CARTESIAN_POINT ( 'NONE',  ( 167.6524903400753601, -49.32844715993521589, 300.4678068554149490 ) ) ;
#59646=AXIS2_PLACEMENT_3D ( 'NONE', #62041, #87973, #19376 ) ;
#59648=CARTESIAN_POINT ( 'NONE',  ( 99.78939748087903183, -33.03164401141575723, 48.77094751244892734 ) ) ;
#59650=ORIENTED_EDGE ( 'NONE', *, *, #71092, .T. ) ;
#59653=CARTESIAN_POINT ( 'NONE',  ( 82.80005790026137902, -18.42904715602866972, 6.774297104451808771 ) ) ;
#59654=ORIENTED_EDGE ( 'NONE', *, *, #20164, .F. ) ;
#59657=VERTEX_POINT ( 'NONE', #83111 ) ;
#59658=EDGE_LOOP ( 'NONE', ( #14286, #25381, #46065, #88088 ) ) ;
#59660=CARTESIAN_POINT ( 'NONE',  ( 114.1634876701351402, -42.35485373834646339, 47.72765792331495760 ) ) ;
#59661=CARTESIAN_POINT ( 'NONE',  ( 103.7160641590222809, -26.17150546779393494, 205.3089586092439731 ) ) ;
#59662=AXIS2_PLACEMENT_3D ( 'NONE', #81643, #75707, #12584 ) ;
#59663=CARTESIAN_POINT ( 'NONE',  ( 109.3536845750984412, -25.93905639472648872, 184.9222919425779708 ) ) ;
#59664=FACE_BOUND ( 'NONE', #41132, .T. ) ;
#59665=CARTESIAN_POINT ( 'NONE',  ( 99.53941477645811631, -29.46552450412116997, 246.7156252759109520 ) ) ;
#59667=CARTESIAN_POINT ( 'NONE',  ( 183.6524903400783160, -48.32844715993452667, 300.4678068554149490 ) ) ;
#59669=VERTEX_POINT ( 'NONE', #49447 ) ;
#59670=VECTOR ( 'NONE', #57240, 1000.000000000000000 ) ;
#59671=CIRCLE ( 'NONE', #56773, 3.249999999999975131 ) ;
#59673=CARTESIAN_POINT ( 'NONE',  ( 98.80440911621268185, -29.31655204712020080, 235.7565776568629872 ) ) ;
#59674=ORIENTED_EDGE ( 'NONE', *, *, #33588, .F. ) ;
#59675=CARTESIAN_POINT ( 'NONE',  ( 107.5657785589506688, -47.77162953885341778, 192.6003871806729535 ) ) ;
#59676=CARTESIAN_POINT ( 'NONE',  ( 108.4162223138522307, -26.73487509134323048, 264.9689798130800682 ) ) ;
#59678=DIRECTION ( 'NONE',  ( 1.000000000000000078E-15, -1.000000000000000083E-30, -1.000000000000000000 ) ) ;
#59682=CARTESIAN_POINT ( 'NONE',  ( 111.7637953458031745, -46.71243375810358600, 283.9146728949585849 ) ) ;
#59683=DIRECTION ( 'NONE',  ( 0.000000000000000000, 0.000000000000000000, 1.000000000000000000 ) ) ;
#59684=FACE_OUTER_BOUND ( 'NONE', #71694, .T. ) ;
#59685=LINE ( 'NONE', #86978, #4925 ) ;
#59687=DIRECTION ( 'NONE',  ( 1.000000000000000078E-15, -1.000000000000000083E-30, -1.000000000000000000 ) ) ;
#59688=CYLINDRICAL_SURFACE ( 'NONE', #34713, 5.599999999999994316 ) ;
#59690=CARTESIAN_POINT ( 'NONE',  ( 100.1309283041910874, -30.67620045321505273, 195.5838068554170661 ) ) ;
#59691=VERTEX_POINT ( 'NONE', #20868 ) ;
#59692=CARTESIAN_POINT ( 'NONE',  ( 127.0664832912740110, -54.72944906728950798, 14.67562527591099197 ) ) ;
#59693=CARTESIAN_POINT ( 'NONE',  ( 117.4347420270075730, -35.18426962645584410, 218.9441967044829482 ) ) ;
#59694=CARTESIAN_POINT ( 'NONE',  ( 112.5142634568524329, -27.84101767465772070, 90.63848241876793566 ) ) ;
#59695=CARTESIAN_POINT ( 'NONE',  ( 97.88103918441719031, -41.75145834149261503, 217.7241967044829494 ) ) ;
#59701=AXIS2_PLACEMENT_3D ( 'NONE', #1972, #70109, #7883 ) ;
#59703=VERTEX_POINT ( 'NONE', #76278 ) ;
#59704=EDGE_CURVE ( 'NONE', #58550, #9949, #5249, .T. ) ;
#59705=ORIENTED_EDGE ( 'NONE', *, *, #22634, .F. ) ;
#59706=VECTOR ( 'NONE', #8094, 1000.000000000000000 ) ;
#59707=CARTESIAN_POINT ( 'NONE',  ( 109.2815815313881558, -45.51044995646627456, 92.20765792331498290 ) ) ;
#59708=ADVANCED_FACE ( 'NONE', ( #4180 ), #72334, .T. ) ;
#59709=DIRECTION ( 'NONE',  ( -1.000000000000000000, -4.510281037539694659E-14, 0.000000000000000000 ) ) ;
#59712=CARTESIAN_POINT ( 'NONE',  ( 102.3122812202564802, -27.43633205498518635, 116.4527681330539650 ) ) ;
#59714=AXIS2_PLACEMENT_3D ( 'NONE', #1964, #86867, #24628 ) ;
#59715=LINE ( 'NONE', #24769, #44216 ) ;
#59716=EDGE_CURVE ( 'NONE', #62685, #35953, #54512, .T. ) ;
#59719=CARTESIAN_POINT ( 'NONE',  ( 104.4081006675575054, -46.45808914180122429, 108.3647919430991351 ) ) ;
#59720=CARTESIAN_POINT ( 'NONE',  ( 101.5072281473882043, -27.97539281467247108, 65.51467289495899138 ) ) ;
#59721=ORIENTED_EDGE ( 'NONE', *, *, #55558, .F. ) ;
#59723=ORIENTED_EDGE ( 'NONE', *, *, #71330, .F. ) ;
#59724=EDGE_CURVE ( 'NONE', #78458, #51305, #16471, .T. ) ;
#59725=DIRECTION ( 'NONE',  ( 0.000000000000000000, 0.000000000000000000, 1.000000000000000000 ) ) ;
#59726=CARTESIAN_POINT ( 'NONE',  ( 102.6513375509277779, -45.45698538002849176, 123.2041967044819870 ) ) ;
#59728=DIRECTION ( 'NONE',  ( 0.000000000000000000, 1.000000000000000000, 0.000000000000000000 ) ) ;
#59729=EDGE_CURVE ( 'NONE', #12518, #49937, #65066, .T. ) ;
#59730=CARTESIAN_POINT ( 'NONE',  ( 94.86917197795301604, -31.06128196069622760, 3.024967495036138931 ) ) ;
#59731=CARTESIAN_POINT ( 'NONE',  ( 154.4532657509292051, -72.54478064608022692, 396.9756252759102040 ) ) ;
#59734=CARTESIAN_POINT ( 'NONE',  ( 101.0787430638808928, -27.46603582566399027, 70.54514908543497143 ) ) ;
#59735=VERTEX_POINT ( 'NONE', #45926 ) ;
#59737=ORIENTED_EDGE ( 'NONE', *, *, #78860, .T. ) ;
#59739=CARTESIAN_POINT ( 'NONE',  ( 107.0664832912739968, -36.72944715994100306, 287.6356252759109680 ) ) ;
#59740=AXIS2_PLACEMENT_3D ( 'NONE', #35350, #50321, #14486 ) ;
#59741=DIRECTION ( 'NONE',  ( 0.9825752044328147639, 0.1858654557302462929, 0.000000000000000000 ) ) ;
#59742=CARTESIAN_POINT ( 'NONE',  ( 99.80647774793122551, -41.44074323372286273, 144.6147570362579415 ) ) ;
#59743=EDGE_CURVE ( 'NONE', #770, #29891, #37810, .T. ) ;
#59746=VERTEX_POINT ( 'NONE', #72776 ) ;
#59754=ADVANCED_FACE ( 'NONE', ( #44148 ), #37356, .T. ) ;
#59755=CARTESIAN_POINT ( 'NONE',  ( 103.8678987209337947, -28.46522696937008945, 211.8015833058969690 ) ) ;
#59756=DIRECTION ( 'NONE',  ( -1.054009200593500181E-15, -1.000000000000000000, 0.000000000000000000 ) ) ;
#59757=EDGE_CURVE ( 'NONE', #63968, #78226, #79161, .T. ) ;
#59758=DIRECTION ( 'NONE',  ( 1.000000000000000078E-15, -1.000000000000000083E-30, -1.000000000000000000 ) ) ;
#59759=AXIS2_PLACEMENT_3D ( 'NONE', #8571, #35809, #15391 ) ;
#59760=CARTESIAN_POINT ( 'NONE',  ( 116.3212776292271258, -32.94146857470711609, 44.13562527591097506 ) ) ;
#59762=ORIENTED_EDGE ( 'NONE', *, *, #56980, .F. ) ;
#59764=ORIENTED_EDGE ( 'NONE', *, *, #78299, .F. ) ;
#59765=ORIENTED_EDGE ( 'NONE', *, *, #10421, .F. ) ;
#59766=CARTESIAN_POINT ( 'NONE',  ( 99.78156907347540994, -40.47280301881529851, 194.5223760838769920 ) ) ;
#59767=CARTESIAN_POINT ( 'NONE',  ( 118.9289135900544494, -36.16662986141290048, 118.8641967044819836 ) ) ;
#59768=CARTESIAN_POINT ( 'NONE',  ( 106.6611865629619018, -26.33404432545455265, 85.10705384733896040 ) ) ;
#59769=LINE ( 'NONE', #11183, #48597 ) ;
#59771=CARTESIAN_POINT ( 'NONE',  ( 51.56670390244699576, -22.48495420874030515, -5.074374724088000832 ) ) ;
#59772=CARTESIAN_POINT ( 'NONE',  ( 108.9451852418780362, -26.43907245703257303, 160.9327681330539690 ) ) ;
#59773=CIRCLE ( 'NONE', #16302, 13.16666666666669627 ) ;
#59779=DIRECTION ( 'NONE',  ( 0.000000000000000000, 1.000000000000000000, 0.000000000000000000 ) ) ;
#59783=CARTESIAN_POINT ( 'NONE',  ( 184.5667039024480118, -48.82844715994099971, 20.91780685541479912 ) ) ;
#59784=EDGE_LOOP ( 'NONE', ( #50948, #26318 ) ) ;
#59785=CARTESIAN_POINT ( 'NONE',  ( 107.3887696601165374, -26.70707029421490120, 131.0506897302312836 ) ) ;
#59786=CARTESIAN_POINT ( 'NONE',  ( 106.6603292229642790, -26.31205452386275212, 85.10705384733896040 ) ) ;
#59790=CARTESIAN_POINT ( 'NONE',  ( 106.6854394624702707, -26.95610377642487165, 85.10705384733996937 ) ) ;
#59791=CARTESIAN_POINT ( 'NONE',  ( 72.06648329127401098, -45.72944715994111675, -4.970821333495738514 ) ) ;
#59792=CARTESIAN_POINT ( 'NONE',  ( 101.3611157396114635, -46.16939438856402944, 198.1318157521009482 ) ) ;
#59794=PLANE ( 'NONE',  #29266 ) ;
#59796=DIRECTION ( 'NONE',  ( -4.554376769437570034E-14, 1.000000000000000000, 0.000000000000000000 ) ) ;
#59798=CARTESIAN_POINT ( 'NONE',  ( 49.16670390244701139, -28.27351298637340093, -5.074374724088000832 ) ) ;
#59800=CARTESIAN_POINT ( 'NONE',  ( 118.0975507117283883, -35.49314816969329200, 233.9032443235299752 ) ) ;
#59802=CARTESIAN_POINT ( 'NONE',  ( 108.4173341213413835, -26.73501241750527413, 144.9689709186055779 ) ) ;
#59803=CARTESIAN_POINT ( 'NONE',  ( 102.7553090513238487, -25.69095112480093945, 16.37276813305293999 ) ) ;
#59804=CARTESIAN_POINT ( 'NONE',  ( 114.0153296496652615, -28.07433117884028206, 115.5261014663869474 ) ) ;
#59805=FACE_OUTER_BOUND ( 'NONE', #27779, .T. ) ;
#59806=CARTESIAN_POINT ( 'NONE',  ( 81.55977255144560445, -39.04085022828763840, 7.869587501222556014 ) ) ;
#59808=DIRECTION ( 'NONE',  ( -1.000000000000000078E-15, 1.000000000000000083E-30, 1.000000000000000000 ) ) ;
#59810=VERTEX_POINT ( 'NONE', #10982 ) ;
#59813=ORIENTED_EDGE ( 'NONE', *, *, #83914, .F. ) ;
#59814=EDGE_CURVE ( 'NONE', #31265, #43132, #58935, .T. ) ;
#59815=ORIENTED_EDGE ( 'NONE', *, *, #20372, .F. ) ;
#59817=VERTEX_POINT ( 'NONE', #46380 ) ;
#59818=CARTESIAN_POINT ( 'NONE',  ( 105.7154773147163098, -46.72385839023237253, 72.46895860799507716 ) ) ;
#59819=CARTESIAN_POINT ( 'NONE',  ( 106.2538455105912050, -26.32252419718687619, 21.13848241876792144 ) ) ;
#59820=CARTESIAN_POINT ( 'NONE',  ( 149.4409906032288404, -0.9156555935619370423, 361.9756252759100335 ) ) ;
#59822=VECTOR ( 'NONE', #15197, 1000.000000000000000 ) ;
#59824=CARTESIAN_POINT ( 'NONE',  ( 151.0371591254585155, -46.82818131005592477, 117.4678068554150485 ) ) ;
#59826=CARTESIAN_POINT ( 'NONE',  ( 109.4373255760682611, -46.14484595950412427, 242.1952769709339464 ) ) ;
#59827=EDGE_LOOP ( 'NONE', ( #49422, #55261 ) ) ;
#59828=ORIENTED_EDGE ( 'NONE', *, *, #27687, .T. ) ;
#59830=ADVANCED_FACE ( 'NONE', ( #40486 ), #25511, .T. ) ;
#59831=VECTOR ( 'NONE', #57001, 1000.000000000000000 ) ;
#59832=CARTESIAN_POINT ( 'NONE',  ( 150.5667039024475571, -25.42844715993593852, 180.4678068554149775 ) ) ;
#59833=CARTESIAN_POINT ( 'NONE',  ( 98.04153869695548451, -41.04189868359566873, 181.6812057122477597 ) ) ;
#59834=CARTESIAN_POINT ( 'NONE',  ( 41.56648329127398966, -27.82844715994070484, 318.9256252759120116 ) ) ;
#59835=CARTESIAN_POINT ( 'NONE',  ( 115.9247622085524085, -36.97270265434710979, 40.23586902018294609 ) ) ;
#59840=CARTESIAN_POINT ( 'NONE',  ( 115.4995704134666994, -41.68388727776413560, 238.4041967044829562 ) ) ;
#59841=CARTESIAN_POINT ( 'NONE',  ( 107.0664832912730020, -27.87844715994269862, 342.9256252759109884 ) ) ;
#59843=ORIENTED_EDGE ( 'NONE', *, *, #34732, .T. ) ;
#59844=FACE_OUTER_BOUND ( 'NONE', #29967, .T. ) ;
#59846=CARTESIAN_POINT ( 'NONE',  ( 114.8864029495430685, -33.02137736771143750, 62.00904275054391945 ) ) ;
#59847=DIRECTION ( 'NONE',  ( -1.000000000000000000, -2.756263715554006823E-15, 0.000000000000000000 ) ) ;
#59848=CARTESIAN_POINT ( 'NONE',  ( 152.0371591254583450, -47.82818131005588214, 249.9678068554149490 ) ) ;
#59850=VERTEX_POINT ( 'NONE', #17154 ) ;
#59851=CARTESIAN_POINT ( 'NONE',  ( 141.0664832912740110, -8.729447159940995959, -4.824374724088994704 ) ) ;
#59854=ORIENTED_EDGE ( 'NONE', *, *, #24771, .F. ) ;
#59855=CARTESIAN_POINT ( 'NONE',  ( 96.64175856332744274, -36.61924367559645788, 111.3184824187679567 ) ) ;
#59856=ORIENTED_EDGE ( 'NONE', *, *, #33276, .F. ) ;
#59857=CARTESIAN_POINT ( 'NONE',  ( 109.7600704110825802, -27.40125247274746556, 64.27527697093398729 ) ) ;
#59858=CARTESIAN_POINT ( 'NONE',  ( 165.2748236753140247, -30.08671355700301575, 342.9256252759119548 ) ) ;
#59859=CARTESIAN_POINT ( 'NONE',  ( 113.2603198993755882, -43.06700715444978300, 69.62444044875392990 ) ) ;
#59861=ADVANCED_FACE ( 'NONE', ( #42264 ), #37599, .F. ) ;
#59862=DIRECTION ( 'NONE',  ( 0.000000000000000000, 0.000000000000000000, 1.000000000000000000 ) ) ;
#59863=CARTESIAN_POINT ( 'NONE',  ( 106.6058858729755201, -25.66269263286424263, 36.09753003781596448 ) ) ;
#59864=CARTESIAN_POINT ( 'NONE',  ( 142.8821648370248170, -72.54478064608022692, 540.9756252759101471 ) ) ;
#59867=CARTESIAN_POINT ( 'NONE',  ( 30.48091746481745901, -49.32844715994156815, 180.4678068554150911 ) ) ;
#59869=CARTESIAN_POINT ( 'NONE',  ( 180.2121375201600131, -29.73316016639649462, 342.9256252759109884 ) ) ;
#59871=ORIENTED_EDGE ( 'NONE', *, *, #84045, .T. ) ;
#59874=CARTESIAN_POINT ( 'NONE',  ( 97.41213207386795148, -40.51524797426110069, 246.6118157521019896 ) ) ;
#59875=CARTESIAN_POINT ( 'NONE',  ( 108.7144426859271391, -26.79521004361802028, 124.9450481620639408 ) ) ;
#59876=DIRECTION ( 'NONE',  ( -6.524622321627019585E-16, -3.741823817616790462E-31, -1.000000000000000000 ) ) ;
#59877=CARTESIAN_POINT ( 'NONE',  ( 98.59006141831567049, -43.82340604873675716, 67.86895860924497015 ) ) ;
#59878=CARTESIAN_POINT ( 'NONE',  ( 113.1780956839291150, -44.75202357551225418, 44.09393879976367003 ) ) ;
#59879=ORIENTED_EDGE ( 'NONE', *, *, #51644, .T. ) ;
#59881=EDGE_CURVE ( 'NONE', #8532, #51252, #28647, .T. ) ;
#59882=DIRECTION ( 'NONE',  ( 0.000000000000000000, 1.000000000000000000, 0.000000000000000000 ) ) ;
#59884=VECTOR ( 'NONE', #55757, 1000.000000000000000 ) ;
#59885=EDGE_CURVE ( 'NONE', #54474, #63459, #27753, .T. ) ;
#59886=CARTESIAN_POINT ( 'NONE',  ( 194.5667039024482676, -40.82844715993405060, 129.9678068554150343 ) ) ;
#59887=CARTESIAN_POINT ( 'NONE',  ( 107.0664832912739683, -25.27030990763060103, 309.2406250056037038 ) ) ;
#59888=CARTESIAN_POINT ( 'NONE',  ( 115.2346088729120339, -30.22974330756297690, 244.3613395616249875 ) ) ;
#59889=DIRECTION ( 'NONE',  ( 0.7071067811861589947, -0.7071067811869361508, 0.000000000000000000 ) ) ;
#59890=B_SPLINE_CURVE_WITH_KNOTS ( 'NONE', 3,
 ( #62051, #20729, #40713, #74352, #33004, #53873, #19832, #5765, #26640, #61596, #53420, #89334, #6650, #26199, #47516, #75253, #47061, #27539 ),
 .UNSPECIFIED., .F., .F.,
 ( 4, 2, 2, 2, 2, 2, 2, 2, 4 ),
 ( 0.000000000000000000, 0.03620097733914664356, 0.07240195467829316223, 0.1086029320174396740, 0.1448039093565861857, 0.1810048866957326974, 0.2172058640348792369, 0.2534068413740257486, 0.2896078187131722603 ),
 .UNSPECIFIED. ) ;
#59891=CIRCLE ( 'NONE', #46850, 2.750000000000002665 ) ;
#59892=LINE ( 'NONE', #32646, #34654 ) ;
#59894=CARTESIAN_POINT ( 'NONE',  ( 104.5043403851385904, -28.58134581971437882, 249.7409912566480727 ) ) ;
#59896=DIRECTION ( 'NONE',  ( 1.000000000000000000, 4.272717921125132861E-14, 0.000000000000000000 ) ) ;
#59897=CARTESIAN_POINT ( 'NONE',  ( 106.6611865629619160, -26.33404432545466634, 81.10705384733896040 ) ) ;
#59899=CARTESIAN_POINT ( 'NONE',  ( 99.02022134730059122, -43.42753157066677261, 116.8784824187679732 ) ) ;
#59901=CARTESIAN_POINT ( 'NONE',  ( 132.1654742078716538, -20.71744337670341451, 7.623533105439178392 ) ) ;
#59904=DIRECTION ( 'NONE',  ( -4.299999999999999979E-14, 1.000000000000000000, -4.400000000000000367E-29 ) ) ;
#59905=CARTESIAN_POINT ( 'NONE',  ( 97.80969226196111777, -40.51824922604903634, 262.6357212258262166 ) ) ;
#59906=DIRECTION ( 'NONE',  ( 0.000000000000000000, 0.000000000000000000, -1.000000000000000000 ) ) ;
#59907=ORIENTED_EDGE ( 'NONE', *, *, #78657, .F. ) ;
#59909=CARTESIAN_POINT ( 'NONE',  ( 116.6387536407295329, -29.65834838561569242, 109.3327681330539605 ) ) ;
#59910=ORIENTED_EDGE ( 'NONE', *, *, #16751, .F. ) ;
#59914=VERTEX_POINT ( 'NONE', #14131 ) ;
#59915=CARTESIAN_POINT ( 'NONE',  ( 116.9251198095579554, -40.18685225151752860, 133.5584824187679658 ) ) ;
#59918=LINE ( 'NONE', #24536, #48601 ) ;
#59919=CARTESIAN_POINT ( 'NONE',  ( 162.5667039024488361, -33.35206098992174617, 117.4678068554150485 ) ) ;
#59920=ORIENTED_EDGE ( 'NONE', *, *, #16568, .F. ) ;
#59921=ADVANCED_FACE ( 'NONE', ( #9441 ), #30338, .T. ) ;
#59923=ADVANCED_FACE ( 'NONE', ( #76354 ), #58465, .F. ) ;
#59924=ORIENTED_EDGE ( 'NONE', *, *, #19918, .T. ) ;
#59925=CARTESIAN_POINT ( 'NONE',  ( 21.56670390244696733, -23.42844715994183957, 300.4678068554150059 ) ) ;
#59927=DIRECTION ( 'NONE',  ( 1.000000000000000078E-15, 0.000000000000000000, -1.000000000000000000 ) ) ;
#59930=LINE ( 'NONE', #67663, #63939 ) ;
#59932=CARTESIAN_POINT ( 'NONE',  ( 97.75841769537090897, -40.38496945966961960, 181.6242637945837259 ) ) ;
#59933=ORIENTED_EDGE ( 'NONE', *, *, #49774, .T. ) ;
#59934=EDGE_CURVE ( 'NONE', #20871, #53911, #48614, .T. ) ;
#59935=CARTESIAN_POINT ( 'NONE',  ( 117.0718954810517261, -35.46248233408972084, 34.92729194434081563 ) ) ;
#59936=CARTESIAN_POINT ( 'NONE',  ( 97.67678136301130110, -41.13084272647604678, 207.6632443235299661 ) ) ;
#59940=CARTESIAN_POINT ( 'NONE',  ( 101.4370486012140589, -28.02035706366318379, 66.54514908543396245 ) ) ;
#59941=CARTESIAN_POINT ( 'NONE',  ( 107.0664832912739399, -36.72944715994095333, 289.6356252759107406 ) ) ;
#59943=PLANE ( 'NONE',  #35859 ) ;
#59945=DIRECTION ( 'NONE',  ( 0.000000000000000000, 2.135044278125299371E-15, -1.000000000000000000 ) ) ;
#59947=EDGE_LOOP ( 'NONE', ( #87677, #44081, #13745, #60911 ) ) ;
#59948=CARTESIAN_POINT ( 'NONE',  ( 109.6042693146342515, -27.68311267370638618, 216.3025356868499500 ) ) ;
#59949=CIRCLE ( 'NONE', #10625, 5.499999999999999112 ) ;
#59952=CIRCLE ( 'NONE', #26651, 13.00000000000000355 ) ;
#59953=CARTESIAN_POINT ( 'NONE',  ( 36.65249034007445772, -49.32844715994130524, 180.4678068554150911 ) ) ;
#59954=CARTESIAN_POINT ( 'NONE',  ( 82.54112294217885903, -37.94037323192714695, 2.740176903238848993 ) ) ;
#59955=ORIENTED_EDGE ( 'NONE', *, *, #38378, .F. ) ;
#59959=CARTESIAN_POINT ( 'NONE',  ( 105.8960369669305805, -47.10223136823075407, 282.4870538473394390 ) ) ;
#59961=VERTEX_POINT ( 'NONE', #55435 ) ;
#59962=CARTESIAN_POINT ( 'NONE',  ( 110.8229109585819003, -44.00762958608321895, 270.7738046553057529 ) ) ;
#59963=FACE_BOUND ( 'NONE', #85397, .T. ) ;
#59965=DIRECTION ( 'NONE',  ( 0.7071067811865460184, 0.000000000000000000, 0.7071067811865487940 ) ) ;
#59968=CARTESIAN_POINT ( 'NONE',  ( 107.6569575903311318, -47.81316668278100224, 193.6308633711489620 ) ) ;
#59971=AXIS2_PLACEMENT_3D ( 'NONE', #75750, #69383, #48906 ) ;
#59972=CARTESIAN_POINT ( 'NONE',  ( 97.24759266268939939, -33.09869426670887549, 62.04419670448196911 ) ) ;
#59974=CIRCLE ( 'NONE', #32418, 0.5000000000000073275 ) ;
#59978=VERTEX_POINT ( 'NONE', #49071 ) ;
#59980=CARTESIAN_POINT ( 'NONE',  ( 104.4882991616608905, -26.97926274729260854, 160.2813675197272403 ) ) ;
#59981=FACE_OUTER_BOUND ( 'NONE', #19780, .T. ) ;
#59982=CARTESIAN_POINT ( 'NONE',  ( 116.7941005169256385, -39.39147994404237352, 153.6152460865006617 ) ) ;
#59983=CARTESIAN_POINT ( 'NONE',  ( 112.5586783213544066, -42.80550525696455821, 130.9795189410199612 ) ) ;
#59984=CARTESIAN_POINT ( 'NONE',  ( 96.66048121734328902, -35.80620304765527351, 227.2556252759109725 ) ) ;
#59988=CARTESIAN_POINT ( 'NONE',  ( 31.89136050872128791, -31.76306994223899238, 117.4678068554150485 ) ) ;
#59989=ORIENTED_EDGE ( 'NONE', *, *, #32967, .F. ) ;
#59992=ADVANCED_FACE ( 'NONE', ( #76805, #37150 ), #9891, .F. ) ;
#59993=DIRECTION ( 'NONE',  ( 0.000000000000000000, 0.000000000000000000, 1.000000000000000000 ) ) ;
#59994=VERTEX_POINT ( 'NONE', #78942 ) ;
#59995=VERTEX_POINT ( 'NONE', #6862 ) ;
#59996=DIRECTION ( 'NONE',  ( 0.000000000000000000, 0.000000000000000000, 1.000000000000000000 ) ) ;
#59999=CARTESIAN_POINT ( 'NONE',  ( 98.01111206384085506, -36.61009632703314765, 155.7505150661719995 ) ) ;
#60000=CARTESIAN_POINT ( 'NONE',  ( 110.5699785786504918, -46.63284631861461804, 37.84705384733994293 ) ) ;
#60001=CARTESIAN_POINT ( 'NONE',  ( 162.5667039024470171, -33.35206098992711077, 342.9256252759119548 ) ) ;
#60003=CARTESIAN_POINT ( 'NONE',  ( 172.5664832912740110, -27.82844715994070484, 323.6756252759119548 ) ) ;
#60004=VERTEX_POINT ( 'NONE', #20942 ) ;
#60005=DIRECTION ( 'NONE',  ( 0.000000000000000000, 0.000000000000000000, -1.000000000000000000 ) ) ;
#60006=ORIENTED_EDGE ( 'NONE', *, *, #23035, .T. ) ;
#60007=CARTESIAN_POINT ( 'NONE',  ( 97.80672817134072261, -40.50528890471652943, 167.6348551699710185 ) ) ;
#60008=CARTESIAN_POINT ( 'NONE',  ( 88.24325903289650341, -55.55267141831875222, 14.67562527591095112 ) ) ;
#60009=CARTESIAN_POINT ( 'NONE',  ( 117.0486299590089203, -35.90762754657916389, 133.8918835446932007 ) ) ;
#60013=CARTESIAN_POINT ( 'NONE',  ( 110.2909773106953111, -46.66674596437654543, 12.82705384733995402 ) ) ;
#60014=CARTESIAN_POINT ( 'NONE',  ( 99.95113126132085313, -44.40829767532816419, 42.98133956162492098 ) ) ;
#60015=( BOUNDED_CURVE ( )  B_SPLINE_CURVE ( 3, ( #63961, #24296, #58784, #84867 ),
 .UNSPECIFIED., .F., .T. ) 
 B_SPLINE_CURVE_WITH_KNOTS ( ( 4, 4 ),
 ( 2.824060085324058217E-12, 1.570796326798421738 ),
 .UNSPECIFIED. ) 
 CURVE ( )  GEOMETRIC_REPRESENTATION_ITEM ( )  RATIONAL_B_SPLINE_CURVE ( ( 1.000000000000000000, 0.8047378541241997363, 0.8047378541241997363, 1.000000000000000000 ) ) 
 REPRESENTATION_ITEM ( '' )  );
#60017=AXIS2_PLACEMENT_3D ( 'NONE', #7758, #12788, #89540 ) ;
#60018=CARTESIAN_POINT ( 'NONE',  ( 141.8545562996767444, -1.932463243632623229, 361.9756252759100335 ) ) ;
#60020=DIRECTION ( 'NONE',  ( 0.000000000000000000, 0.000000000000000000, -1.000000000000000000 ) ) ;
#60022=DIRECTION ( 'NONE',  ( -0.000000000000000000, -0.000000000000000000, 1.000000000000000000 ) ) ;
#60023=EDGE_CURVE ( 'NONE', #61816, #56160, #47325, .T. ) ;
#60024=LINE ( 'NONE', #87760, #22852 ) ;
#60028=CARTESIAN_POINT ( 'NONE',  ( 99.10996421577944204, -43.53389204880360097, 31.88991099019594699 ) ) ;
#60029=CARTESIAN_POINT ( 'NONE',  ( 96.12521010412353917, -35.16020481777900386, 222.2251490854349640 ) ) ;
#60030=CARTESIAN_POINT ( 'NONE',  ( 109.6483737747080198, -46.85224817473300618, 43.77562527591094721 ) ) ;
#60032=LINE ( 'NONE', #32792, #69715 ) ;
#60033=CYLINDRICAL_SURFACE ( 'NONE', #13701, 2.517500000000005844 ) ;
#60034=DIRECTION ( 'NONE',  ( 0.000000000000000000, 1.000000000000000000, 0.000000000000000000 ) ) ;
#60036=AXIS2_PLACEMENT_3D ( 'NONE', #6875, #62283, #7336 ) ;
#60040=EDGE_LOOP ( 'NONE', ( #63892, #54980, #47756, #37793, #66582 ) ) ;
#60041=CARTESIAN_POINT ( 'NONE',  ( 98.13101841594846064, -32.75189731695859763, 96.99276813305296230 ) ) ;
#60042=EDGE_CURVE ( 'NONE', #70341, #810, #32543, .T. ) ;
#60045=AXIS2_PLACEMENT_3D ( 'NONE', #87413, #3847, #10216 ) ;
#60046=CARTESIAN_POINT ( 'NONE',  ( 104.1918496689535090, -26.69446299336411599, 221.2984824187679465 ) ) ;
#60048=LINE ( 'NONE', #25541, #47797 ) ;
#60051=CARTESIAN_POINT ( 'NONE',  ( 115.8254323915925568, -31.73001882795865214, 45.23979194264600778 ) ) ;
#60052=CARTESIAN_POINT ( 'NONE',  ( 131.5441285970347280, -37.82508440162272478, 2.797770139040990589 ) ) ;
#60054=CARTESIAN_POINT ( 'NONE',  ( 108.5509251780138271, -26.47246927008487205, 149.9737205140069420 ) ) ;
#60055=ORIENTED_EDGE ( 'NONE', *, *, #34710, .F. ) ;
#60057=CARTESIAN_POINT ( 'NONE',  ( 97.47186360698646013, -39.79766782782348855, 128.0044404487539396 ) ) ;
#60058=CARTESIAN_POINT ( 'NONE',  ( 168.0371591254543091, -48.62818131005519717, 313.9678068554149490 ) ) ;
#60059=CARTESIAN_POINT ( 'NONE',  ( 117.4251315444614789, -36.24242395571268816, 264.8518157521010608 ) ) ;
#60060=DIRECTION ( 'NONE',  ( -1.000000000000000078E-15, 1.000000000000000083E-30, 1.000000000000000000 ) ) ;
#60061=CARTESIAN_POINT ( 'NONE',  ( 105.8694971003958614, -26.37070548771162493, 321.6188579224977389 ) ) ;
#60062=DIRECTION ( 'NONE',  ( 0.000000000000000000, 0.000000000000000000, -1.000000000000000000 ) ) ;
#60066=CARTESIAN_POINT ( 'NONE',  ( 107.0664832912739683, -23.56278049327427482, 308.7195067599733420 ) ) ;
#60068=CARTESIAN_POINT ( 'NONE',  ( 117.2701380961606645, -34.52720868313122082, 183.9956252759109532 ) ) ;
#60069=CARTESIAN_POINT ( 'NONE',  ( 102.0673672214506098, -27.97029977251938959, 170.4888039060526808 ) ) ;
#60071=ORIENTED_EDGE ( 'NONE', *, *, #63331, .F. ) ;
#60073=CARTESIAN_POINT ( 'NONE',  ( 81.24992100027586162, -21.21189388394623165, 8.006199623923167863 ) ) ;
#60074=CARTESIAN_POINT ( 'NONE',  ( 115.0895278777549606, -30.61844485430380303, 184.3443006593670930 ) ) ;
#60075=LINE ( 'NONE', #18763, #85445 ) ;
#60077=CARTESIAN_POINT ( 'NONE',  ( 97.07191748774732787, -35.37976532927168449, 96.21906654814019078 ) ) ;
#60079=CARTESIAN_POINT ( 'NONE',  ( 98.30747362804066825, -41.72872748435885626, 61.73977921712166506 ) ) ;
#60081=ADVANCED_FACE ( 'NONE', ( #53866 ), #46616, .F. ) ;
#60082=CARTESIAN_POINT ( 'NONE',  ( 98.53748378420890219, -30.73418253943381728, 205.8384824187679669 ) ) ;
#60083=DIRECTION ( 'NONE',  ( 0.000000000000000000, 0.000000000000000000, 1.000000000000000000 ) ) ;
#60084=ORIENTED_EDGE ( 'NONE', *, *, #23526, .T. ) ;
#60086=CARTESIAN_POINT ( 'NONE',  ( 114.6261096459129760, -43.30823112647709650, 64.25718145844111007 ) ) ;
#60087=DIRECTION ( 'NONE',  ( -0.000000000000000000, 1.000000000000000000, 0.000000000000000000 ) ) ;
#60088=CARTESIAN_POINT ( 'NONE',  ( 98.38054347145074985, -41.69548487457510078, 166.7398071395968486 ) ) ;
#60089=CARTESIAN_POINT ( 'NONE',  ( 111.0211786934911231, -29.03130846684521060, 17.52904275054395455 ) ) ;
#60090=CARTESIAN_POINT ( 'NONE',  ( 117.1846329980857178, -34.12938843674525202, 120.0270538473389479 ) ) ;
#60093=PLANE ( 'NONE',  #2963 ) ;
#60094=CARTESIAN_POINT ( 'NONE',  ( 82.59705637153267332, -17.65296049054653338, 7.043700149389792387 ) ) ;
#60096=ORIENTED_EDGE ( 'NONE', *, *, #78745, .T. ) ;
#60097=VECTOR ( 'NONE', #49810, 1000.000000000000000 ) ;
#60099=CARTESIAN_POINT ( 'NONE',  ( 30.48091746481830100, -49.32844715994148288, 300.4678068554150059 ) ) ;
#60100=AXIS2_PLACEMENT_3D ( 'NONE', #51679, #25324, #66202 ) ;
#60102=VERTEX_POINT ( 'NONE', #45277 ) ;
#60103=DIRECTION ( 'NONE',  ( 1.000000000000000000, 4.163336342344333240E-14, 0.000000000000000000 ) ) ;
#60104=VECTOR ( 'NONE', #57911, 1000.000000000000000 ) ;
#60105=CARTESIAN_POINT ( 'NONE',  ( 98.14502816950557929, -38.28518133910327492, 45.87432458998197404 ) ) ;
#60106=CIRCLE ( 'NONE', #20975, 2.116999999999980009 ) ;
#60107=CARTESIAN_POINT ( 'NONE',  ( 97.07499705966343129, -41.51125058752681696, 216.6937205140059461 ) ) ;
#60109=CARTESIAN_POINT ( 'NONE',  ( 117.7567108552515265, -34.01230579303179979, 169.0365776568629599 ) ) ;
#60110=CARTESIAN_POINT ( 'NONE',  ( 180.3503142329310265, -29.99615139349890569, -5.074374724088000832 ) ) ;
#60111=CARTESIAN_POINT ( 'NONE',  ( 112.3382693683599314, -28.20726497302192826, 285.6356252759109680 ) ) ;
#60112=CARTESIAN_POINT ( 'NONE',  ( 31.85959712127300847, -23.19206098994050436, -5.074374724088000832 ) ) ;
#60114=EDGE_CURVE ( 'NONE', #8213, #66245, #69076, .T. ) ;
#60115=ORIENTED_EDGE ( 'NONE', *, *, #14221, .F. ) ;
#60116=EDGE_CURVE ( 'NONE', #43969, #75973, #66171, .T. ) ;
#60117=VERTEX_POINT ( 'NONE', #80284 ) ;
#60119=CARTESIAN_POINT ( 'NONE',  ( 116.8989603263487567, -40.32514756444775372, 218.5470538473399529 ) ) ;
#60121=CARTESIAN_POINT ( 'NONE',  ( 98.37959078170875671, -29.89446464491232192, 200.8080062282919869 ) ) ;
#60122=CARTESIAN_POINT ( 'NONE',  ( 90.44969454456416713, -55.86395651782494554, 229.5838068554169809 ) ) ;
#60123=EDGE_CURVE ( 'NONE', #4783, #49381, #38038, .T. ) ;
#60124=CARTESIAN_POINT ( 'NONE',  ( 134.0664832912740110, -36.72944715994100306, -5.074374724089001809 ) ) ;
#60126=CARTESIAN_POINT ( 'NONE',  ( 114.9425050820284184, -34.80279201792794908, 277.6356252759108543 ) ) ;
#60128=FACE_OUTER_BOUND ( 'NONE', #29980, .T. ) ;
#60129=DIRECTION ( 'NONE',  ( 0.000000000000000000, 0.000000000000000000, -1.000000000000000000 ) ) ;
#60130=DIRECTION ( 'NONE',  ( 1.000000000000000078E-15, 0.000000000000000000, 1.000000000000000000 ) ) ;
#60132=CYLINDRICAL_SURFACE ( 'NONE', #41624, 0.9999999999999731326 ) ;
#60133=EDGE_CURVE ( 'NONE', #8036, #32982, #23613, .T. ) ;
#60134=CARTESIAN_POINT ( 'NONE',  ( 80.06648329127399677, -8.350947159940998787, 293.6356252759119911 ) ) ;
#60136=ORIENTED_EDGE ( 'NONE', *, *, #30644, .T. ) ;
#60137=DIRECTION ( 'NONE',  ( 1.000000000000000078E-15, -1.000000000000000083E-30, -1.000000000000000000 ) ) ;
#60138=CARTESIAN_POINT ( 'NONE',  ( 110.2626856154920603, -26.74582790018529366, 234.8299109901969643 ) ) ;
#60139=CARTESIAN_POINT ( 'NONE',  ( 95.48802730109245829, -34.20477442036718685, 102.1556252759109640 ) ) ;
#60140=CARTESIAN_POINT ( 'NONE',  ( 97.43303641489029587, -40.91689460032421266, 227.6527681330539679 ) ) ;
#60141=DIRECTION ( 'NONE',  ( -0.9068632946707805287, 0.4214249218767882610, -9.068632946707800501E-16 ) ) ;
#60142=DIRECTION ( 'NONE',  ( -1.000000000000000000, -5.512527431108013646E-15, 0.000000000000000000 ) ) ;
#60143=CARTESIAN_POINT ( 'NONE',  ( 19.56670390244734747, -25.42844715994192129, 300.4678068554150059 ) ) ;
#60145=FACE_OUTER_BOUND ( 'NONE', #29457, .T. ) ;
#60146=LINE ( 'NONE', #33358, #74692 ) ;
#60147=VECTOR ( 'NONE', #79839, 1000.000000000000000 ) ;
#60148=ORIENTED_EDGE ( 'NONE', *, *, #87704, .T. ) ;
#60150=CARTESIAN_POINT ( 'NONE',  ( 99.43039265704440766, -41.59799905411310306, 141.1886103042669731 ) ) ;
#60151=ADVANCED_FACE ( 'NONE', ( #72996 ), #73471, .T. ) ;
#60155=CARTESIAN_POINT ( 'NONE',  ( 114.7552509866191599, -44.63809267644810319, 114.2022919425779719 ) ) ;
#60156=DIRECTION ( 'NONE',  ( -0.9254794337955620787, -0.3787978585227822492, 0.000000000000000000 ) ) ;
#60162=EDGE_CURVE ( 'NONE', #27495, #47011, #44416, .T. ) ;
#60163=CARTESIAN_POINT ( 'NONE',  ( 99.77418633167435758, -43.29726106931981633, 56.90991099019693422 ) ) ;
#60164=ORIENTED_EDGE ( 'NONE', *, *, #24204, .F. ) ;
#60167=VECTOR ( 'NONE', #65028, 1000.000000000000000 ) ;
#60168=VECTOR ( 'NONE', #29021, 1000.000000000000114 ) ;
#60169=CARTESIAN_POINT ( 'NONE',  ( 46.32460016641727663, -48.34074026909785005, 249.9678068554150343 ) ) ;
#60171=CARTESIAN_POINT ( 'NONE',  ( 112.1511370651176662, -26.84216853020821958, 165.6984824187679521 ) ) ;
#60173=DIRECTION ( 'NONE',  ( 0.000000000000000000, 0.000000000000000000, 1.000000000000000000 ) ) ;
#60174=PLANE ( 'NONE',  #88714 ) ;
#60178=CARTESIAN_POINT ( 'NONE',  ( 165.9667039024459996, -26.71338133339301635, 193.9678068554150059 ) ) ;
#60179=CARTESIAN_POINT ( 'NONE',  ( 116.7949810323142117, -39.38834386435669188, 179.6147497770267876 ) ) ;
#60180=CARTESIAN_POINT ( 'NONE',  ( 107.3204973292724276, -25.70223992296332582, 75.04610146638695767 ) ) ;
#60183=DIRECTION ( 'NONE',  ( 1.000000000000000000, 4.443626637970137948E-14, 0.000000000000000000 ) ) ;
#60186=CARTESIAN_POINT ( 'NONE',  ( 100.6382899380647871, -31.69863749346629689, 153.6166617981629656 ) ) ;
#60187=AXIS2_PLACEMENT_3D ( 'NONE', #77357, #22857, #56448 ) ;
#60188=EDGE_CURVE ( 'NONE', #81179, #6628, #2366, .T. ) ;
#60193=EDGE_LOOP ( 'NONE', ( #24858, #23001, #10174, #45464 ) ) ;
#60196=CARTESIAN_POINT ( 'NONE',  ( 102.2713888833019240, -44.80927359098731699, 203.5939642582779641 ) ) ;
#60197=FACE_OUTER_BOUND ( 'NONE', #25034, .T. ) ;
#60200=DIRECTION ( 'NONE',  ( 0.7071067811864687469, 0.7071067811866262875, 7.071067811864681542E-16 ) ) ;
#60201=ORIENTED_EDGE ( 'NONE', *, *, #34177, .F. ) ;
#60202=ORIENTED_EDGE ( 'NONE', *, *, #40782, .F. ) ;
#60203=ADVANCED_FACE ( 'NONE', ( #41591 ), #69324, .F. ) ;
#60204=CIRCLE ( 'NONE', #51525, 27.99999999999999645 ) ;
#60205=VERTEX_POINT ( 'NONE', #27091 ) ;
#60206=ORIENTED_EDGE ( 'NONE', *, *, #52171, .F. ) ;
#60208=CARTESIAN_POINT ( 'NONE',  ( 99.19750579858670392, -34.55944272753168889, 248.9309475124489950 ) ) ;
#60209=EDGE_CURVE ( 'NONE', #10240, #27695, #56110, .T. ) ;
#60210=CARTESIAN_POINT ( 'NONE',  ( 100.2843123851674960, -46.47809700006297362, 87.09276813305393716 ) ) ;
#60211=CARTESIAN_POINT ( 'NONE',  ( 101.1533894386775074, -27.41820966596953468, 65.51467289495799662 ) ) ;
#60212=CARTESIAN_POINT ( 'NONE',  ( 112.6007387669400686, -28.69124247953021367, 249.5838068554169240 ) ) ;
#60213=DIRECTION ( 'NONE',  ( -0.0001713722456127401463, 0.9999999853157766072, 1.713722456137401502E-19 ) ) ;
#60214=DIRECTION ( 'NONE',  ( -4.012088370409549976E-14, 1.000000000000000000, 0.000000000000000000 ) ) ;
#60215=CARTESIAN_POINT ( 'NONE',  ( 95.56951908670150431, -39.60249947413915805, 162.5213395616259788 ) ) ;
#60218=CARTESIAN_POINT ( 'NONE',  ( 63.06670390244732971, -24.92844715994017690, 300.4678068554150627 ) ) ;
#60219=ADVANCED_FACE ( 'NONE', ( #7099, #47510 ), #89329, .T. ) ;
#60221=EDGE_CURVE ( 'NONE', #27344, #59219, #54760, .T. ) ;
#60222=VERTEX_POINT ( 'NONE', #62499 ) ;
#60223=CARTESIAN_POINT ( 'NONE',  ( 97.81541838259728650, -40.52652817096748805, 132.6367908339016424 ) ) ;
#60224=LINE ( 'NONE', #53397, #66292 ) ;
#60225=VERTEX_POINT ( 'NONE', #47056 ) ;
#60227=VECTOR ( 'NONE', #77964, 1000.000000000000000 ) ;
#60228=CARTESIAN_POINT ( 'NONE',  ( 87.06648329127425257, -46.72944715994106701, -4.970821333495708316 ) ) ;
#60230=VECTOR ( 'NONE', #86454, 1000.000000000000114 ) ;
#60231=VECTOR ( 'NONE', #33271, 1000.000000000000000 ) ;
#60232=CARTESIAN_POINT ( 'NONE',  ( 104.4081006355542058, -46.45808913331583767, 177.3647919407246434 ) ) ;
#60233=CARTESIAN_POINT ( 'NONE',  ( 104.2140152791992875, -25.22710339543701963, 90.26991099019693365 ) ) ;
#60236=EDGE_CURVE ( 'NONE', #43365, #59070, #57526, .T. ) ;
#60237=DIRECTION ( 'NONE',  ( 0.000000000000000000, -1.000000000000000000, 0.000000000000000000 ) ) ;
#60238=DIRECTION ( 'NONE',  ( 1.000000000000000000, 4.163336342344333240E-14, 0.000000000000000000 ) ) ;
#60239=CARTESIAN_POINT ( 'NONE',  ( 104.4081006511264320, -46.45808913744465229, 143.3647919417593357 ) ) ;
#60240=CARTESIAN_POINT ( 'NONE',  ( 97.81225633602475966, -40.51881169864816457, 56.63532730191191433 ) ) ;
#60241=CARTESIAN_POINT ( 'NONE',  ( 98.45302666770176359, -29.83944080489372652, 191.7775300378159784 ) ) ;
#60242=CYLINDRICAL_SURFACE ( 'NONE', #59646, 0.4999999999999933387 ) ;
#60244=ORIENTED_EDGE ( 'NONE', *, *, #49877, .F. ) ;
#60245=DIRECTION ( 'NONE',  ( 0.000000000000000000, 0.000000000000000000, -1.000000000000000000 ) ) ;
#60247=DIRECTION ( 'NONE',  ( 0.000000000000000000, 1.000000000000000000, 0.000000000000000000 ) ) ;
#60248=CARTESIAN_POINT ( 'NONE',  ( 112.1414192606818574, -28.01400143680720944, 134.6564062991808441 ) ) ;
#60249=ADVANCED_FACE ( 'NONE', ( #48850 ), #26636, .T. ) ;
#60251=DIRECTION ( 'NONE',  ( -1.000000000000000000, 0.000000000000000000, 0.000000000000000000 ) ) ;
#60252=CARTESIAN_POINT ( 'NONE',  ( 110.2694181837619141, -26.72479813065621812, 234.8299109901969643 ) ) ;
#60253=ORIENTED_EDGE ( 'NONE', *, *, #8953, .F. ) ;
#60254=CARTESIAN_POINT ( 'NONE',  ( 63.56670390244800473, -40.82844715994016127, 249.9678068554150343 ) ) ;
#60255=CARTESIAN_POINT ( 'NONE',  ( 115.9451031845006099, -42.19318012571019949, 14.38705384733995984 ) ) ;
#60256=CARTESIAN_POINT ( 'NONE',  ( 98.24414503606394078, -31.02815815664761345, 141.8699109901969564 ) ) ;
#60257=CARTESIAN_POINT ( 'NONE',  ( 19.56670390244740076, -47.82844715994204421, 180.4678068554150911 ) ) ;
#60262=FACE_OUTER_BOUND ( 'NONE', #20305, .T. ) ;
#60263=VERTEX_POINT ( 'NONE', #88883 ) ;
#60264=CIRCLE ( 'NONE', #44318, 2.517500000000005844 ) ;
#60265=VERTEX_POINT ( 'NONE', #48394 ) ;
#60267=VERTEX_POINT ( 'NONE', #82079 ) ;
#60268=DIRECTION ( 'NONE',  ( 0.000000000000000000, -1.000000000000000000, 0.000000000000000000 ) ) ;
#60269=CARTESIAN_POINT ( 'NONE',  ( 111.3142535964730371, -27.23286288913599051, 20.74133956162494030 ) ) ;
#60270=DIRECTION ( 'NONE',  ( 0.000000000000000000, 1.000000000000000000, 0.000000000000000000 ) ) ;
#60273=EDGE_CURVE ( 'NONE', #20049, #14493, #76332, .T. ) ;
#60274=CARTESIAN_POINT ( 'NONE',  ( 188.5667039024479834, -62.87844715994099687, 295.9678068554150059 ) ) ;
#60276=EDGE_CURVE ( 'NONE', #69613, #30635, #22472, .T. ) ;
#60277=CARTESIAN_POINT ( 'NONE',  ( 115.1107970995275736, -40.88897666221423322, 242.8571817328389670 ) ) ;
#60280=CIRCLE ( 'NONE', #48665, 11.45913725231036118 ) ;
#60284=DIRECTION ( 'NONE',  ( 0.000000000000000000, 1.000000000000000000, 0.000000000000000000 ) ) ;
#60286=CARTESIAN_POINT ( 'NONE',  ( 83.06670390244796920, -64.87844715994098976, 207.5838068554149913 ) ) ;
#60287=CARTESIAN_POINT ( 'NONE',  ( 104.6647032408819200, -45.25937870008434771, 18.79015473446898810 ) ) ;
#60289=CARTESIAN_POINT ( 'NONE',  ( 36.65249034007445772, -49.32844715994130524, 180.4678068554150911 ) ) ;
#60290=CARTESIAN_POINT ( 'NONE',  ( 95.96284676697203508, -37.29622633765243478, 271.3670538473399461 ) ) ;
#60291=LINE ( 'NONE', #12615, #68946 ) ;
#60292=ORIENTED_EDGE ( 'NONE', *, *, #19678, .T. ) ;
#60293=CARTESIAN_POINT ( 'NONE',  ( 61.67079006425787924, -0.9306969701470987344, 394.9756252759102040 ) ) ;
#60294=CARTESIAN_POINT ( 'NONE',  ( 107.2792697713003776, -24.20934055526686279, 321.5865679059475610 ) ) ;
#60295=CARTESIAN_POINT ( 'NONE',  ( 104.3513172347134770, -44.42734293102004273, 55.12523322673396109 ) ) ;
#60297=CIRCLE ( 'NONE', #55948, 10.04999999999999361 ) ;
#60299=DIRECTION ( 'NONE',  ( 0.000000000000000000, -1.000000000000000000, 0.000000000000000000 ) ) ;
#60300=CARTESIAN_POINT ( 'NONE',  ( 99.04404928436410671, -42.84123934602111206, 192.8438477477418758 ) ) ;
#60304=ORIENTED_EDGE ( 'NONE', *, *, #16812, .F. ) ;
#60305=CARTESIAN_POINT ( 'NONE',  ( 102.3022244709477775, -27.41667396567568815, 120.4527681330539792 ) ) ;
#60307=CARTESIAN_POINT ( 'NONE',  ( 100.1216203692562630, -42.54163687813885275, 71.29146744712500094 ) ) ;
#60308=CARTESIAN_POINT ( 'NONE',  ( 99.87975691711011450, -43.74731000462409725, 87.94166648727369306 ) ) ;
#60309=CARTESIAN_POINT ( 'NONE',  ( 108.7714652236932835, -45.96901220096565055, 124.1653928297069882 ) ) ;
#60310=CARTESIAN_POINT ( 'NONE',  ( 156.5667039024485518, -48.82844715993568485, 175.7178068554150059 ) ) ;
#60312=CIRCLE ( 'NONE', #15420, 11.45913725231036118 ) ;
#60313=CARTESIAN_POINT ( 'NONE',  ( 117.4691034930615103, -37.69004686371126667, 74.75276813305397638 ) ) ;
#60314=DIRECTION ( 'NONE',  ( 0.0001713722456120069274, -0.9999999853157766072, 0.000000000000000000 ) ) ;
#60317=ORIENTED_EDGE ( 'NONE', *, *, #74207, .F. ) ;
#60319=ORIENTED_EDGE ( 'NONE', *, *, #33229, .F. ) ;
#60320=CIRCLE ( 'NONE', #53033, 2.999999999999929834 ) ;
#60322=EDGE_CURVE ( 'NONE', #43121, #7616, #16598, .T. ) ;
#60325=DIRECTION ( 'NONE',  ( 4.299999999999999979E-14, -1.000000000000000000, 4.400000000000000367E-29 ) ) ;
#60327=CARTESIAN_POINT ( 'NONE',  ( 110.5064767540468296, -26.94654216138279068, 254.8194347997213640 ) ) ;
#60328=CARTESIAN_POINT ( 'NONE',  ( 142.8821648370248170, -72.54478064608022692, 542.9756252759101471 ) ) ;
#60329=CARTESIAN_POINT ( 'NONE',  ( 116.7951252646970772, -39.38782981747054635, 189.6147919403582591 ) ) ;
#60330=CARTESIAN_POINT ( 'NONE',  ( 101.0662023700742935, -27.44663458233410935, 66.54514908543495721 ) ) ;
#60332=EDGE_LOOP ( 'NONE', ( #56069, #35716 ) ) ;
#60333=CARTESIAN_POINT ( 'NONE',  ( 102.0667429138110691, -27.97066660765753099, 115.4919662677435213 ) ) ;
#60335=DIRECTION ( 'NONE',  ( 0.000000000000000000, 0.000000000000000000, -1.000000000000000000 ) ) ;
#60336=VERTEX_POINT ( 'NONE', #2528 ) ;
#60337=ADVANCED_FACE ( 'NONE', ( #57474 ), #70671, .T. ) ;
#60340=CARTESIAN_POINT ( 'NONE',  ( 105.8960369669305805, -47.10223136823075407, 282.4870538473394390 ) ) ;
#60341=LINE ( 'NONE', #74439, #68991 ) ;
#60342=DIRECTION ( 'NONE',  ( 1.000000000000000000, 4.163336342344333240E-14, 0.000000000000000000 ) ) ;
#60343=CARTESIAN_POINT ( 'NONE',  ( 78.35735255112980724, -38.88611802718641286, 2.101554303227473941 ) ) ;
#60344=EDGE_CURVE ( 'NONE', #45788, #69613, #41896, .T. ) ;
#60345=CARTESIAN_POINT ( 'NONE',  ( 100.7700969181924506, -30.95782257301981488, 275.1581341137911068 ) ) ;
#60347=CARTESIAN_POINT ( 'NONE',  ( 116.6546583390152279, -32.60254457569000408, 75.14991099019697174 ) ) ;
#60349=CARTESIAN_POINT ( 'NONE',  ( 113.5926674049485854, -44.96113684323219672, 168.1099109901969939 ) ) ;
#60350=ORIENTED_EDGE ( 'NONE', *, *, #45551, .F. ) ;
#60351=CARTESIAN_POINT ( 'NONE',  ( 84.06648329127399677, -18.82844715994099971, 199.5838068554169524 ) ) ;
#60352=ORIENTED_EDGE ( 'NONE', *, *, #12507, .T. ) ;
#60353=DIRECTION ( 'NONE',  ( 1.000000000000000078E-15, -1.000000000000000083E-30, -1.000000000000000000 ) ) ;
#60354=DIRECTION ( 'NONE',  ( 0.000000000000000000, 0.000000000000000000, -1.000000000000000000 ) ) ;
#60355=CARTESIAN_POINT ( 'NONE',  ( 21.03715912545829170, -47.82818131006186491, 249.9678068554150059 ) ) ;
#60356=VERTEX_POINT ( 'NONE', #83861 ) ;
#60357=EDGE_CURVE ( 'NONE', #26148, #58495, #28535, .T. ) ;
#60359=CARTESIAN_POINT ( 'NONE',  ( 95.62691733261443972, -33.44842233792613229, 141.1041967044829732 ) ) ;
#60360=ORIENTED_EDGE ( 'NONE', *, *, #49494, .T. ) ;
#60361=DIRECTION ( 'NONE',  ( -0.9254794337955620787, -0.3787978585227822492, 0.000000000000000000 ) ) ;
#60362=VECTOR ( 'NONE', #75311, 1000.000000000000000 ) ;
#60364=CARTESIAN_POINT ( 'NONE',  ( 98.30753418512887265, -41.72887548160911564, 117.7397919417121983 ) ) ;
#60366=VECTOR ( 'NONE', #7029, 999.9999999999998863 ) ;
#60367=ORIENTED_EDGE ( 'NONE', *, *, #15866, .F. ) ;
#60368=CARTESIAN_POINT ( 'NONE',  ( 101.4890226443523744, -27.89551843606815495, 110.5241967044819944 ) ) ;
#60369=VECTOR ( 'NONE', #69096, 1000.000000000000000 ) ;
#60370=AXIS2_PLACEMENT_3D ( 'NONE', #18412, #39310, #44780 ) ;
#60373=DIRECTION ( 'NONE',  ( 0.7071067811865192621, 0.7071067811865758834, 7.071067811865186413E-16 ) ) ;
#60374=DIRECTION ( 'NONE',  ( 0.000000000000000000, 0.000000000000000000, 1.000000000000000000 ) ) ;
#60376=ORIENTED_EDGE ( 'NONE', *, *, #51125, .T. ) ;
#60377=CARTESIAN_POINT ( 'NONE',  ( 162.9033555647784226, -33.89581943343761594, 237.4678068554150059 ) ) ;
#60381=CARTESIAN_POINT ( 'NONE',  ( 188.5667039024479834, -58.35344715994099829, 254.4678068554150343 ) ) ;
#60383=CARTESIAN_POINT ( 'NONE',  ( 123.6837132603318707, -20.11243780205705534, 218.8274735512161158 ) ) ;
#60384=EDGE_CURVE ( 'NONE', #32906, #16372, #56576, .T. ) ;
#60385=CARTESIAN_POINT ( 'NONE',  ( 115.0888856295657803, -30.61760799569063707, 179.3439612979183266 ) ) ;
#60386=CONICAL_SURFACE ( 'NONE', #27138, 1.258749999999999369, 1.029744258676650093 ) ;
#60389=CARTESIAN_POINT ( 'NONE',  ( 41.56648329127399677, -9.303447159940999356, 136.8086252759119645 ) ) ;
#60390=CARTESIAN_POINT ( 'NONE',  ( 116.5994914424365021, -40.81117973626238893, 209.5165776568629497 ) ) ;
#60391=CARTESIAN_POINT ( 'NONE',  ( 188.5667039024479834, -65.37844715994100397, 252.3428068554150059 ) ) ;
#60392=ORIENTED_EDGE ( 'NONE', *, *, #67864, .F. ) ;
#60393=CARTESIAN_POINT ( 'NONE',  ( 104.1495640007033501, -46.68084741754449851, 58.33753003781600199 ) ) ;
#60394=DIRECTION ( 'NONE',  ( 1.639958061481212836E-42, -4.100000000000000342E-29, -1.000000000000000000 ) ) ;
#60397=ORIENTED_EDGE ( 'NONE', *, *, #79660, .T. ) ;
#60400=ORIENTED_EDGE ( 'NONE', *, *, #81571, .F. ) ;
#60401=VERTEX_POINT ( 'NONE', #46504 ) ;
#60402=CARTESIAN_POINT ( 'NONE',  ( 105.4042388664825722, -28.02512512522124410, 231.6587261630399439 ) ) ;
#60407=CARTESIAN_POINT ( 'NONE',  ( 82.72805595269750256, -37.42731094489875687, 2.974216770161541845 ) ) ;
#60408=ORIENTED_EDGE ( 'NONE', *, *, #67518, .F. ) ;
#60410=CARTESIAN_POINT ( 'NONE',  ( 113.2375207001889947, -28.75257540792464539, 35.55234988136929530 ) ) ;
#60412=CARTESIAN_POINT ( 'NONE',  ( 106.2521265061568130, -26.30051002661620885, 25.13848241876792855 ) ) ;
#60413=ORIENTED_EDGE ( 'NONE', *, *, #62090, .F. ) ;
#60414=ORIENTED_EDGE ( 'NONE', *, *, #60273, .T. ) ;
#60415=CARTESIAN_POINT ( 'NONE',  ( 100.7056284991137289, -31.61385801203766377, 238.6052332267339580 ) ) ;
#60416=CARTESIAN_POINT ( 'NONE',  ( 95.60734603896362671, -36.72944715994100306, 293.2242906452868851 ) ) ;
#60417=CARTESIAN_POINT ( 'NONE',  ( 114.0056865186722490, -29.02320718445394476, 159.5051490854349652 ) ) ;
#60420=CARTESIAN_POINT ( 'NONE',  ( 162.7866693523289996, -36.02818131005891189, -5.074374724088000832 ) ) ;
#60421=CARTESIAN_POINT ( 'NONE',  ( 101.1761829863686160, -45.38377220964024161, 193.1013395616249682 ) ) ;
#60423=ORIENTED_EDGE ( 'NONE', *, *, #83670, .T. ) ;
#60424=VECTOR ( 'NONE', #17045, 1000.000000000000000 ) ;
#60425=CARTESIAN_POINT ( 'NONE',  ( 100.9176109441957436, -28.25688269532019348, 71.57562527591099411 ) ) ;
#60427=CARTESIAN_POINT ( 'NONE',  ( 107.0664832912739399, -36.72944715994095333, 305.7141315223800007 ) ) ;
#60428=AXIS2_PLACEMENT_3D ( 'NONE', #65347, #16757, #57176 ) ;
#60434=EDGE_CURVE ( 'NONE', #84376, #13709, #11571, .T. ) ;
#60435=LINE ( 'NONE', #18667, #65118 ) ;
#60436=CARTESIAN_POINT ( 'NONE',  ( 33.92127028473601769, -29.73316016639540749, -5.074374724088000832 ) ) ;
#60437=DIRECTION ( 'NONE',  ( 1.000000000000000000, 3.999999999999999995E-14, 1.000000000000000078E-15 ) ) ;
#60438=CARTESIAN_POINT ( 'NONE',  ( 113.0638415271824897, -42.26672268200739069, 121.0509475124479906 ) ) ;
#60439=CARTESIAN_POINT ( 'NONE',  ( 115.5350430195811668, -29.59021037493291573, 220.3718157521019521 ) ) ;
#60440=CARTESIAN_POINT ( 'NONE',  ( 188.5667039024479834, -58.35344715994099829, 173.2178068554149775 ) ) ;
#60441=ORIENTED_EDGE ( 'NONE', *, *, #14985, .F. ) ;
#60442=EDGE_CURVE ( 'NONE', #47492, #84886, #32431, .T. ) ;
#60443=VECTOR ( 'NONE', #76333, 1000.000000000000000 ) ;
#60444=CARTESIAN_POINT ( 'NONE',  ( 141.8164832912740394, -45.62589376934770513, -5.074374724088994704 ) ) ;
#60445=ORIENTED_EDGE ( 'NONE', *, *, #63881, .F. ) ;
#60446=ORIENTED_EDGE ( 'NONE', *, *, #27423, .T. ) ;
#60447=EDGE_CURVE ( 'NONE', #23436, #59530, #17486, .T. ) ;
#60448=CLOSED_SHELL ( 'NONE', ( #4143, #54990, #67222, #66172 ) ) ;
#60451=ORIENTED_EDGE ( 'NONE', *, *, #14781, .T. ) ;
#60452=CARTESIAN_POINT ( 'NONE',  ( 104.4091854452810253, -46.45840093360554590, 168.3656309447823674 ) ) ;
#60453=LINE ( 'NONE', #10969, #76182 ) ;
#60455=EDGE_CURVE ( 'NONE', #56594, #31182, #24742, .T. ) ;
#60456=CARTESIAN_POINT ( 'NONE',  ( 99.13191293290623207, -41.09468066504173578, 176.1371817328389966 ) ) ;
#60457=CARTESIAN_POINT ( 'NONE',  ( 100.5702229155400858, -28.47427015469623868, 15.60705384733995871 ) ) ;
#60458=CARTESIAN_POINT ( 'NONE',  ( 116.3265940946004378, -32.93621273019581253, 125.1356252759109680 ) ) ;
#60463=ORIENTED_EDGE ( 'NONE', *, *, #73918, .F. ) ;
#60464=CARTESIAN_POINT ( 'NONE',  ( 97.77633413480816671, -40.43004283583653091, 167.6283907404767888 ) ) ;
#60466=CARTESIAN_POINT ( 'NONE',  ( 110.8543515439697558, -45.98428674439771413, 132.8856148800098538 ) ) ;
#60468=FACE_OUTER_BOUND ( 'NONE', #10098, .T. ) ;
#60470=CARTESIAN_POINT ( 'NONE',  ( 110.5626142325126153, -46.61202937628593190, 37.84705384733994293 ) ) ;
#60471=CARTESIAN_POINT ( 'NONE',  ( 96.67154112854022685, -38.24047072676557946, 62.44133956162495025 ) ) ;
#60472=DIRECTION ( 'NONE',  ( 0.000000000000000000, 1.000000000000000000, 0.000000000000000000 ) ) ;
#60475=CARTESIAN_POINT ( 'NONE',  ( 172.5664832912740110, -32.07844715994070839, 318.9256252759120116 ) ) ;
#60476=CARTESIAN_POINT ( 'NONE',  ( 97.21111501186732085, -38.70825661063340561, 122.4834732151292087 ) ) ;
#60479=CARTESIAN_POINT ( 'NONE',  ( 110.4709766755849643, -47.29459308529762041, 57.83657765686300678 ) ) ;
#60480=CARTESIAN_POINT ( 'NONE',  ( 98.53766203808953605, -30.73430783891158669, 201.8384824187679385 ) ) ;
#60481=CARTESIAN_POINT ( 'NONE',  ( 117.8789659794968543, -39.13265831612300616, 99.64038718067195077 ) ) ;
#60484=CARTESIAN_POINT ( 'NONE',  ( 108.3347997046528093, -46.73470615375604353, 172.6734346717588835 ) ) ;
#60485=CARTESIAN_POINT ( 'NONE',  ( 188.5667039024484097, -48.82844715993431350, 257.2178068554150059 ) ) ;
#60486=ADVANCED_FACE ( 'NONE', ( #24306 ), #45166, .T. ) ;
#60487=FACE_OUTER_BOUND ( 'NONE', #60987, .T. ) ;
#60488=VECTOR ( 'NONE', #73676, 1000.000000000000000 ) ;
#60489=CIRCLE ( 'NONE', #53272, 0.5000000000000104361 ) ;
#60490=CIRCLE ( 'NONE', #21357, 3.250000000000002665 ) ;
#60491=CARTESIAN_POINT ( 'NONE',  ( 99.09570913176251850, -30.55043168255618014, 186.8022919354755800 ) ) ;
#60493=CARTESIAN_POINT ( 'NONE',  ( 116.7343647603065619, -32.97833357388816466, 90.10895860924395606 ) ) ;
#60496=CARTESIAN_POINT ( 'NONE',  ( 104.4161250475293485, -26.02246701806305751, 236.2575300378159682 ) ) ;
#60499=CARTESIAN_POINT ( 'NONE',  ( 62.03715912545834499, -47.82818131006021645, 300.4678068554150627 ) ) ;
#60500=CYLINDRICAL_SURFACE ( 'NONE', #45694, 2.750000000000002665 ) ;
#60501=PLANE ( 'NONE',  #67378 ) ;
#60504=VECTOR ( 'NONE', #60629, 1000.000000000000000 ) ;
#60505=AXIS2_PLACEMENT_3D ( 'NONE', #64837, #87513, #72549 ) ;
#60506=CARTESIAN_POINT ( 'NONE',  ( 96.59955023297820276, -32.98040794253977737, 176.0527681330549683 ) ) ;
#60507=ORIENTED_EDGE ( 'NONE', *, *, #34202, .T. ) ;
#60508=VERTEX_POINT ( 'NONE', #38362 ) ;
#60509=CARTESIAN_POINT ( 'NONE',  ( 112.8270896756726671, -29.95615083465972006, 135.9472975916109476 ) ) ;
#60510=AXIS2_PLACEMENT_3D ( 'NONE', #86807, #87255, #24574 ) ;
#60511=ADVANCED_FACE ( 'NONE', ( #65628 ), #60132, .F. ) ;
#60513=CARTESIAN_POINT ( 'NONE',  ( 97.60228370342871074, -39.19771807616534431, 272.5299109901961856 ) ) ;
#60518=DIRECTION ( 'NONE',  ( 0.000000000000000000, 0.000000000000000000, 1.000000000000000000 ) ) ;
#60519=DIRECTION ( 'NONE',  ( 5.512527431108029424E-15, -1.000000000000000000, 0.000000000000000000 ) ) ;
#60520=CARTESIAN_POINT ( 'NONE',  ( 98.39792771585416631, -29.90889243069706538, 200.8080062282919869 ) ) ;
#60521=ORIENTED_EDGE ( 'NONE', *, *, #45371, .F. ) ;
#60522=EDGE_LOOP ( 'NONE', ( #81369, #44118, #16852, #86347 ) ) ;
#60524=DIRECTION ( 'NONE',  ( 1.639958061481212836E-42, -4.100000000000000342E-29, -1.000000000000000000 ) ) ;
#60525=CARTESIAN_POINT ( 'NONE',  ( 194.5664832912739826, -18.82844715994099971, -5.074374724088000832 ) ) ;
#60528=VECTOR ( 'NONE', #2143, 1000.000000000000000 ) ;
#60529=AXIS2_PLACEMENT_3D ( 'NONE', #31110, #31557, #45607 ) ;
#60530=DIRECTION ( 'NONE',  ( 0.000000000000000000, 0.000000000000000000, -1.000000000000000000 ) ) ;
#60531=ORIENTED_EDGE ( 'NONE', *, *, #46475, .T. ) ;
#60532=CARTESIAN_POINT ( 'NONE',  ( 49.35031423293676056, -29.99615139352232873, 117.4678068554150485 ) ) ;
#60533=CARTESIAN_POINT ( 'NONE',  ( 96.12498142956854963, -35.16017202033504674, 226.2251490854349640 ) ) ;
#60534=DIRECTION ( 'NONE',  ( 3.999999999999999995E-14, -1.000000000000000000, 4.100000000000000342E-29 ) ) ;
#60536=VERTEX_POINT ( 'NONE', #74239 ) ;
#60541=CARTESIAN_POINT ( 'NONE',  ( 97.81944346430564963, -40.53631996860134734, 166.6372505363765413 ) ) ;
#60542=CARTESIAN_POINT ( 'NONE',  ( 106.7065939435451440, -28.08240114970028856, 37.91570941720995336 ) ) ;
#60543=CARTESIAN_POINT ( 'NONE',  ( 116.8158478801051530, -32.97616202413719577, 135.1184824187679396 ) ) ;
#60544=DIRECTION ( 'NONE',  ( 1.000000000000000000, -5.689893001203922423E-12, 0.000000000000000000 ) ) ;
#60545=ORIENTED_EDGE ( 'NONE', *, *, #39126, .F. ) ;
#60546=EDGE_CURVE ( 'NONE', #40888, #10162, #72064, .T. ) ;
#60547=CIRCLE ( 'NONE', #21418, 3.000000000000002665 ) ;
#60548=DIRECTION ( 'NONE',  ( 1.000000000000000078E-15, -1.000000000000000083E-30, -1.000000000000000000 ) ) ;
#60549=CARTESIAN_POINT ( 'NONE',  ( 82.73027604518254918, -18.02416100035393853, 6.874390491353741695 ) ) ;
#60550=ORIENTED_EDGE ( 'NONE', *, *, #25827, .T. ) ;
#60552=AXIS2_PLACEMENT_3D ( 'NONE', #72335, #51853, #50978 ) ;
#60554=ORIENTED_EDGE ( 'NONE', *, *, #89388, .F. ) ;
#60558=CARTESIAN_POINT ( 'NONE',  ( 98.27686124684872482, -40.85414981714398408, 61.09813411379100501 ) ) ;
#60559=CARTESIAN_POINT ( 'NONE',  ( 113.6996774752161201, -45.60053368046675359, 188.0994347997199725 ) ) ;
#60560=CIRCLE ( 'NONE', #22931, 4.874999999999990230 ) ;
#60561=CARTESIAN_POINT ( 'NONE',  ( 104.5678333644583944, -48.28820816006152938, 182.4070538473399665 ) ) ;
#60563=CARTESIAN_POINT ( 'NONE',  ( 98.60180739276366069, -42.06509604122263113, 21.77386757017102425 ) ) ;
#60564=CARTESIAN_POINT ( 'NONE',  ( 111.4803918977840169, -26.59589994751270936, 280.7375300378156453 ) ) ;
#60565=LINE ( 'NONE', #12893, #11758 ) ;
#60567=EDGE_LOOP ( 'NONE', ( #9935, #6761, #28154, #42700 ) ) ;
#60568=AXIS2_PLACEMENT_3D ( 'NONE', #82170, #27180, #63038 ) ;
#60569=ORIENTED_EDGE ( 'NONE', *, *, #86926, .F. ) ;
#60570=AXIS2_PLACEMENT_3D ( 'NONE', #52675, #17312, #86358 ) ;
#60572=CIRCLE ( 'NONE', #59152, 2.750000000000002665 ) ;
#60573=CARTESIAN_POINT ( 'NONE',  ( 128.8897065959775148, -58.55267046464430791, 14.67562527591099375 ) ) ;
#60574=CARTESIAN_POINT ( 'NONE',  ( 109.3464976042218524, -26.51141404309336735, 224.9013395616249511 ) ) ;
#60575=ORIENTED_EDGE ( 'NONE', *, *, #30399, .T. ) ;
#60576=CARTESIAN_POINT ( 'NONE',  ( 117.7765707488592710, -31.65652763686493998, 214.1784824187679419 ) ) ;
#60577=CARTESIAN_POINT ( 'NONE',  ( 97.07207204382144994, -35.37844130610024251, 36.21895861776621928 ) ) ;
#60581=CARTESIAN_POINT ( 'NONE',  ( 105.2412389168119233, -28.82906800083503995, 277.6356252759112522 ) ) ;
#60582=CARTESIAN_POINT ( 'NONE',  ( 95.60734603896358408, -36.72944715994100306, 296.0306255462182321 ) ) ;
#60583=CYLINDRICAL_SURFACE ( 'NONE', #53930, 0.4999999999999976685 ) ;
#60584=CARTESIAN_POINT ( 'NONE',  ( 194.5667039024479834, -48.82844715994099971, 10.91780685541479734 ) ) ;
#60586=DIRECTION ( 'NONE',  ( -1.000000000000000000, -4.299999999999999979E-14, -1.000000000000000078E-15 ) ) ;
#60587=DIRECTION ( 'NONE',  ( 0.000000000000000000, 1.000000000000000000, 0.000000000000000000 ) ) ;
#60588=CARTESIAN_POINT ( 'NONE',  ( 102.0670549698788250, -27.97049805383846888, 76.48979194169342577 ) ) ;
#60591=FACE_OUTER_BOUND ( 'NONE', #19362, .T. ) ;
#60592=CARTESIAN_POINT ( 'NONE',  ( 115.4777400244682042, -29.52207584268309759, 229.4022919425779605 ) ) ;
#60593=CARTESIAN_POINT ( 'NONE',  ( 96.63924282488838458, -37.56250720137591514, 97.38991099019594344 ) ) ;
#60594=CARTESIAN_POINT ( 'NONE',  ( 96.87194279380025819, -34.19777600025749109, 272.1327681330539576 ) ) ;
#60595=DIRECTION ( 'NONE',  ( -1.000000000000000000, -4.299999999999999979E-14, -9.351236661543306751E-17 ) ) ;
#60596=DIRECTION ( 'NONE',  ( -1.000000000000000000, -6.493183223601999383E-14, -1.000000000000000078E-15 ) ) ;
#60597=VECTOR ( 'NONE', #26474, 1000.000000000000000 ) ;
#60599=CYLINDRICAL_SURFACE ( 'NONE', #63183, 3.250000000000002665 ) ;
#60601=DIRECTION ( 'NONE',  ( 0.000000000000000000, 0.000000000000000000, -1.000000000000000000 ) ) ;
#60602=AXIS2_PLACEMENT_3D ( 'NONE', #49496, #36786, #84953 ) ;
#60603=CARTESIAN_POINT ( 'NONE',  ( 133.6902059199370854, -21.46022584114957255, 1.641799370506089595 ) ) ;
#60605=ORIENTED_EDGE ( 'NONE', *, *, #31355, .T. ) ;
#60606=ORIENTED_EDGE ( 'NONE', *, *, #40290, .F. ) ;
#60607=CARTESIAN_POINT ( 'NONE',  ( 102.0031328989874027, -44.23578847709845263, 151.5143245899819817 ) ) ;
#60609=EDGE_LOOP ( 'NONE', ( #6951, #30828, #63876, #30981 ) ) ;
#60611=CARTESIAN_POINT ( 'NONE',  ( 96.62907006607247240, -36.88702529232762828, 132.3384824187679669 ) ) ;
#60613=CYLINDRICAL_SURFACE ( 'NONE', #50139, 4.874999999999990230 ) ;
#60616=AXIS2_PLACEMENT_3D ( 'NONE', #88970, #62146, #41686 ) ;
#60617=CARTESIAN_POINT ( 'NONE',  ( 99.11394507416765975, -43.38496525699394368, 71.86895860924497015 ) ) ;
#60618=EDGE_LOOP ( 'NONE', ( #2561, #86639 ) ) ;
#60619=VERTEX_POINT ( 'NONE', #27867 ) ;
#60620=ORIENTED_EDGE ( 'NONE', *, *, #60857, .F. ) ;
#60622=VECTOR ( 'NONE', #23981, 1000.000000000000000 ) ;
#60623=EDGE_CURVE ( 'NONE', #84501, #82293, #88772, .T. ) ;
#60624=DIRECTION ( 'NONE',  ( 0.7071067811865516806, -0.7071067811865434649, 7.071067811865511818E-16 ) ) ;
#60625=CARTESIAN_POINT ( 'NONE',  ( 99.89458030379221043, -28.23347241844150091, 146.6356252759109395 ) ) ;
#60626=CYLINDRICAL_SURFACE ( 'NONE', #57792, 2.116999999999993776 ) ;
#60629=DIRECTION ( 'NONE',  ( 1.000000000000000078E-15, -1.000000000000000000, 0.000000000000000000 ) ) ;
#60630=AXIS2_PLACEMENT_3D ( 'NONE', #12745, #68603, #25922 ) ;
#60631=DIRECTION ( 'NONE',  ( 1.000000000000000000, 3.999999999999999995E-14, 1.000000000000000078E-15 ) ) ;
#60633=CARTESIAN_POINT ( 'NONE',  ( 107.2318599658364207, -25.70055450771768690, 80.07657765686299456 ) ) ;
#60636=EDGE_CURVE ( 'NONE', #32451, #62736, #89503, .T. ) ;
#60637=LINE ( 'NONE', #61983, #31388 ) ;
#60639=AXIS2_PLACEMENT_3D ( 'NONE', #63385, #16468, #1167 ) ;
#60641=CARTESIAN_POINT ( 'NONE',  ( 108.0840670587429599, -45.32394831497818899, 160.5004713219719861 ) ) ;
#60643=ORIENTED_EDGE ( 'NONE', *, *, #16595, .F. ) ;
#60646=DIRECTION ( 'NONE',  ( 0.000000000000000000, 1.000000000000000000, 0.000000000000000000 ) ) ;
#60647=ORIENTED_EDGE ( 'NONE', *, *, #17491, .F. ) ;
#60649=CARTESIAN_POINT ( 'NONE',  ( 77.46225723383568607, -19.61690131754105693, 6.952852217897422804 ) ) ;
#60650=ADVANCED_FACE ( 'NONE', ( #83296 ), #69660, .F. ) ;
#60651=CARTESIAN_POINT ( 'NONE',  ( 112.1289716242999361, -44.03925847519028025, 199.4901547344690016 ) ) ;
#60652=CARTESIAN_POINT ( 'NONE',  ( 41.56670390244801894, -27.57844715994070484, 342.9256252759119548 ) ) ;
#60653=VECTOR ( 'NONE', #74064, 1000.000000000000000 ) ;
#60654=LINE ( 'NONE', #88392, #34219 ) ;
#60655=AXIS2_PLACEMENT_3D ( 'NONE', #45197, #3881, #29815 ) ;
#60657=ORIENTED_EDGE ( 'NONE', *, *, #25677, .T. ) ;
#60658=ORIENTED_EDGE ( 'NONE', *, *, #45303, .T. ) ;
#60662=EDGE_CURVE ( 'NONE', #8963, #55318, #53757, .T. ) ;
#60663=CARTESIAN_POINT ( 'NONE',  ( 102.1208986914200665, -43.83170863157916131, 234.8985665600679624 ) ) ;
#60664=CARTESIAN_POINT ( 'NONE',  ( 116.9960073371140652, -33.48122977351050622, 89.07848241876791917 ) ) ;
#60665=CARTESIAN_POINT ( 'NONE',  ( 118.8180844208009717, -35.40729807334668067, 83.91562527591095488 ) ) ;
#60666=CARTESIAN_POINT ( 'NONE',  ( 106.6920129052768544, -28.07392614262452213, 249.5838068554171514 ) ) ;
#60667=EDGE_CURVE ( 'NONE', #85439, #81096, #37239, .T. ) ;
#60668=CARTESIAN_POINT ( 'NONE',  ( 133.8780722764265079, -15.97944715994100306, 8.225625275910996237 ) ) ;
#60669=DIRECTION ( 'NONE',  ( 1.000000000000000078E-15, -1.000000000000000000, 0.000000000000000000 ) ) ;
#60670=CARTESIAN_POINT ( 'NONE',  ( 117.1921950572609603, -41.16159581679399793, 204.4861014663869696 ) ) ;
#60672=ORIENTED_EDGE ( 'NONE', *, *, #18118, .T. ) ;
#60674=VERTEX_POINT ( 'NONE', #81522 ) ;
#60676=ORIENTED_EDGE ( 'NONE', *, *, #30964, .T. ) ;
#60677=CARTESIAN_POINT ( 'NONE',  ( 63.06670390244641311, -24.92844715994017335, 180.4678068554151196 ) ) ;
#60678=VERTEX_POINT ( 'NONE', #41044 ) ;
#60679=AXIS2_PLACEMENT_3D ( 'NONE', #66309, #53101, #4551 ) ;
#60680=CARTESIAN_POINT ( 'NONE',  ( 97.80849178533165400, -40.50961443681259055, 137.6349539298032596 ) ) ;
#60681=AXIS2_PLACEMENT_3D ( 'NONE', #87876, #32441, #53315 ) ;
#60682=CARTESIAN_POINT ( 'NONE',  ( 53.56670390244872237, -48.82844715994099971, 300.4678068554149490 ) ) ;
#60683=CARTESIAN_POINT ( 'NONE',  ( 103.8412645720801493, -46.68052101597508852, 82.32705384733995402 ) ) ;
#60685=LINE ( 'NONE', #4405, #85588 ) ;
#60686=CARTESIAN_POINT ( 'NONE',  ( 168.5667039024544636, -48.82844715994099971, 129.9678068554150059 ) ) ;
#60688=DIRECTION ( 'NONE',  ( -0.7071067811865165975, -0.7071067811865784369, -7.071067811865470403E-16 ) ) ;
#60689=CARTESIAN_POINT ( 'NONE',  ( 116.3579325164319016, -41.40893824611048757, 199.4556252759109611 ) ) ;
#60690=CARTESIAN_POINT ( 'NONE',  ( 116.3185006702053244, -32.93849971620830530, 275.1356252759109680 ) ) ;
#60692=ORIENTED_EDGE ( 'NONE', *, *, #55856, .F. ) ;
#60693=LINE ( 'NONE', #46160, #38186 ) ;
#60696=DIRECTION ( 'NONE',  ( 0.000000000000000000, 0.000000000000000000, 1.000000000000000000 ) ) ;
#60698=DIRECTION ( 'NONE',  ( -4.299999999999999979E-14, 1.000000000000000000, -4.128053709984630540E-29 ) ) ;
#60699=CARTESIAN_POINT ( 'NONE',  ( 96.22219577434788107, -34.35999324012363587, 256.1432443235299843 ) ) ;
#60702=CARTESIAN_POINT ( 'NONE',  ( 98.42378885047078541, -42.06819960529416136, 7.768006228291934434 ) ) ;
#60703=CARTESIAN_POINT ( 'NONE',  ( 102.3408129182306823, -46.07080783562200565, 123.2041967044829818 ) ) ;
#60705=VECTOR ( 'NONE', #8103, 999.9999999999998863 ) ;
#60707=DIRECTION ( 'NONE',  ( 1.705911707540438309E-29, 0.7071067811865391350, -0.7071067811865560104 ) ) ;
#60708=CARTESIAN_POINT ( 'NONE',  ( 184.5664832912729878, -71.37844715994266664, 342.9256252759109884 ) ) ;
#60709=DIRECTION ( 'NONE',  ( -4.299999999999999979E-14, 1.000000000000000000, -4.400000000000000367E-29 ) ) ;
#60710=CARTESIAN_POINT ( 'NONE',  ( 94.86917197795301604, -31.06128196069622760, 0.4256252759109587225 ) ) ;
#60711=VERTEX_POINT ( 'NONE', #40143 ) ;
#60712=EDGE_CURVE ( 'NONE', #63781, #26765, #21331, .T. ) ;
#60714=EDGE_LOOP ( 'NONE', ( #89459, #63324, #45073, #27055 ) ) ;
#60716=ORIENTED_EDGE ( 'NONE', *, *, #59534, .T. ) ;
#60718=CARTESIAN_POINT ( 'NONE',  ( 104.6539710028519039, -47.49251396406760506, 23.38895860924494841 ) ) ;
#60719=CARTESIAN_POINT ( 'NONE',  ( 162.5667039024478413, -32.29483332967974718, 193.9678068554149775 ) ) ;
#60720=CARTESIAN_POINT ( 'NONE',  ( 116.7618137187695595, -39.33727037636729307, 118.6187472951199453 ) ) ;
#60723=CARTESIAN_POINT ( 'NONE',  ( 110.7878219579318255, -44.41760495294317934, 247.3581341137909533 ) ) ;
#60725=AXIS2_PLACEMENT_3D ( 'NONE', #16516, #44193, #59165 ) ;
#60726=ORIENTED_EDGE ( 'NONE', *, *, #61854, .F. ) ;
#60728=EDGE_CURVE ( 'NONE', #50014, #19244, #47379, .T. ) ;
#60729=CARTESIAN_POINT ( 'NONE',  ( 151.0371591254576060, -24.95799193692592155, 129.9678068554149775 ) ) ;
#60730=DIRECTION ( 'NONE',  ( -0.7071067811864671926, -0.7071067811866279529, -7.071067811864664779E-16 ) ) ;
#60731=LINE ( 'NONE', #68467, #35357 ) ;
#60732=LINE ( 'NONE', #12610, #57674 ) ;
#60733=ADVANCED_FACE ( 'NONE', ( #12458 ), #48287, .F. ) ;
#60734=CARTESIAN_POINT ( 'NONE',  ( 116.5375268006221319, -40.16019621794498562, 19.98158330589694387 ) ) ;
#60736=EDGE_CURVE ( 'NONE', #21752, #33552, #41481, .T. ) ;
#60738=CARTESIAN_POINT ( 'NONE',  ( 115.9938418408662244, -42.00591315737207054, 283.4137205140066271 ) ) ;
#60739=DIRECTION ( 'NONE',  ( 0.000000000000000000, 0.000000000000000000, -1.000000000000000000 ) ) ;
#60741=ORIENTED_EDGE ( 'NONE', *, *, #31629, .F. ) ;
#60742=VECTOR ( 'NONE', #30993, 1000.000000000000000 ) ;
#60743=EDGE_CURVE ( 'NONE', #29576, #82508, #63289, .T. ) ;
#60744=CARTESIAN_POINT ( 'NONE',  ( 188.5667039024479834, -62.87844715994099687, 142.0928068554150059 ) ) ;
#60745=DIRECTION ( 'NONE',  ( 4.299999999999999979E-14, -1.000000000000000000, 4.400000000000000367E-29 ) ) ;
#60746=CARTESIAN_POINT ( 'NONE',  ( 99.81817287040931319, -30.93652672145504567, 43.60809036959195595 ) ) ;
#60747=EDGE_CURVE ( 'NONE', #15026, #61208, #608, .T. ) ;
#60748=VECTOR ( 'NONE', #34480, 1000.000000000000000 ) ;
#60749=EDGE_CURVE ( 'NONE', #67882, #11886, #50992, .T. ) ;
#60750=CARTESIAN_POINT ( 'NONE',  ( 83.06670390244802604, -43.72944715994108122, 231.5838068554169524 ) ) ;
#60754=ORIENTED_EDGE ( 'NONE', *, *, #49600, .T. ) ;
#60755=LINE ( 'NONE', #87584, #33434 ) ;
#60756=AXIS2_PLACEMENT_3D ( 'NONE', #47801, #61885, #77780 ) ;
#60758=ORIENTED_EDGE ( 'NONE', *, *, #41404, .F. ) ;
#60759=CARTESIAN_POINT ( 'NONE',  ( 108.0341695913198521, -25.71842219955733810, 109.9946728949589811 ) ) ;
#60760=ORIENTED_EDGE ( 'NONE', *, *, #80203, .T. ) ;
#60761=CARTESIAN_POINT ( 'NONE',  ( 112.3425469992411649, -30.01235824646559891, 78.96956268521998368 ) ) ;
#60762=EDGE_CURVE ( 'NONE', #65338, #84820, #27122, .T. ) ;
#60763=AXIS2_PLACEMENT_3D ( 'NONE', #31920, #11035, #79658 ) ;
#60764=DIRECTION ( 'NONE',  ( 0.000000000000000000, 0.000000000000000000, -1.000000000000000000 ) ) ;
#60765=CARTESIAN_POINT ( 'NONE',  ( 104.5515342781392008, -45.22670024980423165, 103.7787261630399911 ) ) ;
#60766=LINE ( 'NONE', #80341, #12636 ) ;
#60767=AXIS2_PLACEMENT_3D ( 'NONE', #46618, #47512, #61593 ) ;
#60768=CARTESIAN_POINT ( 'NONE',  ( 37.36643805256573359, -48.62818131006127231, 129.9678068554150911 ) ) ;
#60769=CARTESIAN_POINT ( 'NONE',  ( 96.05470400087912708, -37.92356717231275098, 77.40038718067299328 ) ) ;
#60773=CARTESIAN_POINT ( 'NONE',  ( 77.85525873417948617, -20.37463194332874750, 2.472581811070362789 ) ) ;
#60774=ORIENTED_EDGE ( 'NONE', *, *, #83540, .T. ) ;
#60775=EDGE_LOOP ( 'NONE', ( #44821, #42077, #11811, #76765 ) ) ;
#60777=EDGE_CURVE ( 'NONE', #39460, #28724, #85098, .T. ) ;
#60778=CARTESIAN_POINT ( 'NONE',  ( 57.56670390244744340, -48.82844715994040286, 170.7178068554150911 ) ) ;
#60779=ORIENTED_EDGE ( 'NONE', *, *, #36293, .F. ) ;
#60780=CARTESIAN_POINT ( 'NONE',  ( 100.0046238269856929, -29.91446987444270178, 250.7156252759109520 ) ) ;
#60781=CARTESIAN_POINT ( 'NONE',  ( 98.26250712568560175, -31.04002435091596368, 141.8699109901969564 ) ) ;
#60782=ADVANCED_FACE ( 'NONE', ( #22415, #71016 ), #78286, .F. ) ;
#60783=FACE_OUTER_BOUND ( 'NONE', #57953, .T. ) ;
#60784=CARTESIAN_POINT ( 'NONE',  ( 105.7140088855255868, -46.72363573100787448, 128.4688416786118523 ) ) ;
#60785=CARTESIAN_POINT ( 'NONE',  ( 95.48802730109245829, -34.20477442036718685, 102.1556252759109640 ) ) ;
#60786=DIRECTION ( 'NONE',  ( -0.9068632946707805287, 0.4214249218767882610, -9.068632946707800501E-16 ) ) ;
#60787=EDGE_CURVE ( 'NONE', #24712, #84043, #2413, .T. ) ;
#60788=EDGE_LOOP ( 'NONE', ( #55756, #83200, #60716, #58872 ) ) ;
#60790=EDGE_CURVE ( 'NONE', #89625, #41277, #16489, .T. ) ;
#60793=VERTEX_POINT ( 'NONE', #63745 ) ;
#60794=LINE ( 'NONE', #61681, #63449 ) ;
#60796=CARTESIAN_POINT ( 'NONE',  ( 100.1532602078032568, -44.50350736857021161, 266.9984824187679919 ) ) ;
#60797=DIRECTION ( 'NONE',  ( 0.000000000000000000, 0.000000000000000000, 1.000000000000000000 ) ) ;
#60798=CARTESIAN_POINT ( 'NONE',  ( 63.03715912545736444, -24.42818131006017879, 237.4678068554150059 ) ) ;
#60799=CARTESIAN_POINT ( 'NONE',  ( 77.96454488115740844, -38.51222316632514975, 2.376608873920554643 ) ) ;
#60800=CARTESIAN_POINT ( 'NONE',  ( 114.5649785483395249, -40.87970871860825639, 262.8467055423626562 ) ) ;
#60802=CARTESIAN_POINT ( 'NONE',  ( 108.9812119692459049, -46.95502683147942236, 78.72419670448194040 ) ) ;
#60804=CARTESIAN_POINT ( 'NONE',  ( 116.8478532179160680, -43.50835558345241338, 163.3441967044829823 ) ) ;
#60805=ORIENTED_EDGE ( 'NONE', *, *, #76391, .T. ) ;
#60808=DIRECTION ( 'NONE',  ( 0.000000000000000000, -1.000000000000000000, 0.000000000000000000 ) ) ;
#60810=CARTESIAN_POINT ( 'NONE',  ( 152.0368932755772562, -23.42844715993587812, 193.9678068554149775 ) ) ;
#60811=ORIENTED_EDGE ( 'NONE', *, *, #63750, .T. ) ;
#60812=CIRCLE ( 'NONE', #30360, 0.9999999999999940048 ) ;
#60813=CARTESIAN_POINT ( 'NONE',  ( 97.81413224952068219, -40.51639846094042952, 101.6360726122380100 ) ) ;
#60814=CARTESIAN_POINT ( 'NONE',  ( 105.3088311808849937, -48.49934056980919905, 147.4584824187679715 ) ) ;
#60815=ORIENTED_EDGE ( 'NONE', *, *, #83129, .F. ) ;
#60816=DIRECTION ( 'NONE',  ( -1.000000000000000000, 0.000000000000000000, 0.000000000000000000 ) ) ;
#60817=CARTESIAN_POINT ( 'NONE',  ( 128.0667039024480118, -48.82844715994099971, 10.91780685541499807 ) ) ;
#60820=CARTESIAN_POINT ( 'NONE',  ( 104.4081006714045401, -46.45808914282129365, 77.36479194341235655 ) ) ;
#60821=ORIENTED_EDGE ( 'NONE', *, *, #9135, .T. ) ;
#60824=VERTEX_POINT ( 'NONE', #8793 ) ;
#60826=VECTOR ( 'NONE', #31498, 1000.000000000000000 ) ;
#60828=DIRECTION ( 'NONE',  ( -4.237773401492740281E-14, 1.000000000000000000, 0.000000000000000000 ) ) ;
#60832=VECTOR ( 'NONE', #28778, 1000.000000000000000 ) ;
#60833=CARTESIAN_POINT ( 'NONE',  ( 97.81169585860149596, -40.51742224678086046, 106.6356332503197137 ) ) ;
#60834=DIRECTION ( 'NONE',  ( -0.7071067811865794361, 0.7071067811865157093, -7.071067811865803697E-16 ) ) ;
#60835=DIRECTION ( 'NONE',  ( 1.000000000000000078E-15, -1.000000000000000083E-30, -1.000000000000000000 ) ) ;
#60838=FACE_OUTER_BOUND ( 'NONE', #66601, .T. ) ;
#60839=EDGE_CURVE ( 'NONE', #14129, #39083, #7430, .T. ) ;
#60840=CARTESIAN_POINT ( 'NONE',  ( 117.1144258088630039, -31.97015794161414703, 210.1784824187679703 ) ) ;
#60841=AXIS2_PLACEMENT_3D ( 'NONE', #66161, #79381, #45268 ) ;
#60842=CARTESIAN_POINT ( 'NONE',  ( 107.0664832912750057, -36.72944715993903486, 9.425625275910970657 ) ) ;
#60843=VERTEX_POINT ( 'NONE', #64194 ) ;
#60845=CARTESIAN_POINT ( 'NONE',  ( 116.8435662018513028, -36.99793375417353758, 39.80419670448193159 ) ) ;
#60847=CARTESIAN_POINT ( 'NONE',  ( 116.8182762850237992, -34.15738849411049216, 14.03188649359343110 ) ) ;
#60848=LINE ( 'NONE', #4106, #80816 ) ;
#60849=EDGE_CURVE ( 'NONE', #21043, #62123, #56058, .T. ) ;
#60851=DIRECTION ( 'NONE',  ( -1.000000000000000078E-15, 0.000000000000000000, 1.000000000000000000 ) ) ;
#60852=EDGE_CURVE ( 'NONE', #60267, #48081, #37827, .T. ) ;
#60853=ORIENTED_EDGE ( 'NONE', *, *, #39126, .T. ) ;
#60854=VERTEX_POINT ( 'NONE', #17819 ) ;
#60856=CARTESIAN_POINT ( 'NONE',  ( 110.5184084024339626, -28.56779955429167472, 241.1901547344679670 ) ) ;
#60857=EDGE_CURVE ( 'NONE', #58867, #22696, #6818, .T. ) ;
#60858=CARTESIAN_POINT ( 'NONE',  ( 109.6449249915308997, -46.47961346067916111, 53.78125628650596468 ) ) ;
#60859=B_SPLINE_CURVE_WITH_KNOTS ( 'NONE', 3,
 ( #44280, #9784, #17926, #37492, #58802, #51103, #86097, #45602, #51977, #23870, #79289, #17049, #44730, #72461, #37933, #73334, #3416, #66521, #31998, #79734, #25186, #52848, #80620, #17492, #45172, #46054, #37042, #33348, #19280, #40148, #75133, #66972, #47404, #39267, #88334 ),
 .UNSPECIFIED., .F., .F.,
 ( 4, 2, 2, 1, 1, 2, 2, 2, 2, 2, 2, 1, 1, 2, 2, 2, 1, 1, 1, 2, 4 ),
 ( 0.3333434881890884882, 0.4166701562233637857, 0.4218780729755075565, 0.4270859897276513273, 0.4375018232319339284, 0.4583334902404989086, 0.4999968242576238175, 0.5208284912661862442, 0.5416601582747487820, 0.5624918252833113197, 0.5650957836593817341, 0.5676997420354521484, 0.5729076587875948645, 0.5833234922918794085, 0.6249868263090219145, 0.6275907846850933280, 0.6301947430611646306, 0.6354026598133065695, 0.6458184933175894482, 0.6562343268218724379, 0.6666501603261554276 ),
 .UNSPECIFIED. ) ;
#60861=EDGE_CURVE ( 'NONE', #19807, #6482, #66859, .T. ) ;
#60862=CARTESIAN_POINT ( 'NONE',  ( 117.0608945211236716, -38.08045314457236685, 154.7189586073530165 ) ) ;
#60863=DIRECTION ( 'NONE',  ( 3.340531404218880531E-13, -1.000000000000000000, 2.910531404218880430E-28 ) ) ;
#60865=CIRCLE ( 'NONE', #23179, 2.117000000000000881 ) ;
#60866=CARTESIAN_POINT ( 'NONE',  ( 53.56670390244833158, -48.82844715994055917, 249.9678068554150343 ) ) ;
#60867=DIRECTION ( 'NONE',  ( 0.000000000000000000, 0.000000000000000000, 1.000000000000000000 ) ) ;
#60868=VERTEX_POINT ( 'NONE', #9663 ) ;
#60869=CARTESIAN_POINT ( 'NONE',  ( 116.4746376734894255, -32.23794665461475972, 19.18133956162493092 ) ) ;
#60871=ORIENTED_EDGE ( 'NONE', *, *, #57691, .F. ) ;
#60872=CARTESIAN_POINT ( 'NONE',  ( 101.1728908740289512, -31.04189437634028437, 248.5338046553059428 ) ) ;
#60873=EDGE_CURVE ( 'NONE', #63079, #23299, #79175, .T. ) ;
#60875=CARTESIAN_POINT ( 'NONE',  ( 107.0667039024479834, -48.82844715994099971, 160.9178068554150229 ) ) ;
#60876=CARTESIAN_POINT ( 'NONE',  ( 114.0519814166327563, -29.87813257090970609, 149.4441967044829767 ) ) ;
#60878=CARTESIAN_POINT ( 'NONE',  ( 162.5667039024470171, -32.29483332968611364, -5.074374724088000832 ) ) ;
#60879=CARTESIAN_POINT ( 'NONE',  ( 147.9173673660669124, -72.54478064608022692, 542.9756252759101471 ) ) ;
#60882=CARTESIAN_POINT ( 'NONE',  ( 96.72972436280956288, -34.86144565006776475, 237.1841967044819626 ) ) ;
#60884=CARTESIAN_POINT ( 'NONE',  ( 162.5667039024470171, -32.29483332968611364, 342.9256252759109884 ) ) ;
#60885=AXIS2_PLACEMENT_3D ( 'NONE', #33410, #89285, #75651 ) ;
#60886=ORIENTED_EDGE ( 'NONE', *, *, #25827, .F. ) ;
#60887=CARTESIAN_POINT ( 'NONE',  ( 117.3964687521579293, -38.63454956243933225, 84.68133956162593279 ) ) ;
#60888=LINE ( 'NONE', #19553, #13478 ) ;
#60890=VERTEX_POINT ( 'NONE', #39153 ) ;
#60891=ORIENTED_EDGE ( 'NONE', *, *, #80876, .F. ) ;
#60892=VECTOR ( 'NONE', #21019, 1000.000000000000000 ) ;
#60893=LINE ( 'NONE', #68617, #26021 ) ;
#60894=DIRECTION ( 'NONE',  ( 0.000000000000000000, 0.000000000000000000, -1.000000000000000000 ) ) ;
#60895=VECTOR ( 'NONE', #79665, 1000.000000000000000 ) ;
#60896=CARTESIAN_POINT ( 'NONE',  ( 99.04383488216355147, -42.84091735427421810, 151.8445027460794279 ) ) ;
#60897=DIRECTION ( 'NONE',  ( -0.000000000000000000, 1.000000000000000000, 0.000000000000000000 ) ) ;
#60898=CARTESIAN_POINT ( 'NONE',  ( 112.3727512366848487, -30.49036002617200936, 137.3338046553059826 ) ) ;
#60899=CARTESIAN_POINT ( 'NONE',  ( 96.99552470177088992, -33.95220897389439330, 247.1127681330539758 ) ) ;
#60905=ADVANCED_FACE ( 'NONE', ( #3306 ), #3746, .T. ) ;
#60906=CARTESIAN_POINT ( 'NONE',  ( 142.8841478025725849, -84.11588139007200482, 396.9756252759102040 ) ) ;
#60909=CARTESIAN_POINT ( 'NONE',  ( 179.1667039024460166, -26.71338133339251542, -5.074374724088000832 ) ) ;
#60910=ORIENTED_EDGE ( 'NONE', *, *, #47667, .T. ) ;
#60911=ORIENTED_EDGE ( 'NONE', *, *, #35583, .T. ) ;
#60917=CARTESIAN_POINT ( 'NONE',  ( 99.86829443779211601, -32.07773762820211516, 145.2924198280769872 ) ) ;
#60918=CARTESIAN_POINT ( 'NONE',  ( 109.6539202653692087, -46.87399426414072678, 47.77562527591094721 ) ) ;
#60920=VERTEX_POINT ( 'NONE', #73218 ) ;
#60921=DIRECTION ( 'NONE',  ( -1.000000000000000078E-15, 1.000000000000000083E-30, 1.000000000000000000 ) ) ;
#60922=ORIENTED_EDGE ( 'NONE', *, *, #24287, .T. ) ;
#60924=ORIENTED_EDGE ( 'NONE', *, *, #3689, .T. ) ;
#60927=CARTESIAN_POINT ( 'NONE',  ( 98.54776827858368904, -41.97716740062048757, 131.7658491656293620 ) ) ;
#60929=ADVANCED_FACE ( 'NONE', ( #37373 ), #58691, .F. ) ;
#60930=CARTESIAN_POINT ( 'NONE',  ( 62.03742497533746558, -23.42844715994041849, 300.4678068554150627 ) ) ;
#60932=CARTESIAN_POINT ( 'NONE',  ( 101.3720933679328482, -27.97043537882594322, 25.53562527591096654 ) ) ;
#60933=CARTESIAN_POINT ( 'NONE',  ( 115.6092852924205943, -42.78035731602705027, 49.33562527591095659 ) ) ;
#60934=CYLINDRICAL_SURFACE ( 'NONE', #11481, 3.000000000000002665 ) ;
#60936=CARTESIAN_POINT ( 'NONE',  ( 100.9546813260442519, -28.70701916483188398, 146.5944087211518365 ) ) ;
#60937=CARTESIAN_POINT ( 'NONE',  ( 97.81168895331838087, -40.51742574516882200, 287.6356252759109680 ) ) ;
#60940=VECTOR ( 'NONE', #27772, 1000.000000000000000 ) ;
#60941=CARTESIAN_POINT ( 'NONE',  ( 176.7669697523288335, -48.62818131005481348, 180.4678068554150059 ) ) ;
#60942=ORIENTED_EDGE ( 'NONE', *, *, #46072, .T. ) ;
#60943=CARTESIAN_POINT ( 'NONE',  ( 96.79018504364255193, -38.90877927100929412, 31.49276813305495892 ) ) ;
#60944=CARTESIAN_POINT ( 'NONE',  ( 115.1837411929738977, -43.30572140991047547, 84.28419670448195689 ) ) ;
#60948=DIRECTION ( 'NONE',  ( 0.000000000000000000, 0.000000000000000000, 1.000000000000000000 ) ) ;
#60949=EDGE_CURVE ( 'NONE', #53618, #89279, #69343, .T. ) ;
#60950=CIRCLE ( 'NONE', #21811, 4.875000000000017764 ) ;
#60954=ADVANCED_FACE ( 'NONE', ( #17376 ), #59579, .T. ) ;
#60955=CARTESIAN_POINT ( 'NONE',  ( 96.20363159075265003, -34.36081134307599427, 102.1556252759109640 ) ) ;
#60958=ORIENTED_EDGE ( 'NONE', *, *, #63727, .F. ) ;
#60959=EDGE_CURVE ( 'NONE', #50481, #71480, #24632, .T. ) ;
#60960=CARTESIAN_POINT ( 'NONE',  ( 96.16101635903912381, -35.07578045570940617, 217.1946728949589840 ) ) ;
#60962=DIRECTION ( 'NONE',  ( 1.000000000000000000, 0.000000000000000000, 0.000000000000000000 ) ) ;
#60964=CARTESIAN_POINT ( 'NONE',  ( 97.07207206298383539, -35.37844117089505858, 82.21895860700102787 ) ) ;
#60965=CARTESIAN_POINT ( 'NONE',  ( 131.6729728819749710, -38.08739819366338253, 2.653088468873541661 ) ) ;
#60966=EDGE_CURVE ( 'NONE', #25485, #18963, #45494, .T. ) ;
#60967=DIRECTION ( 'NONE',  ( 0.000000000000000000, -1.000000000000000000, 0.000000000000000000 ) ) ;
#60968=AXIS2_PLACEMENT_3D ( 'NONE', #75350, #27192, #14472 ) ;
#60969=CARTESIAN_POINT ( 'NONE',  ( 103.1049807579881161, -45.67203811392948865, 177.2441967044829596 ) ) ;
#60970=ORIENTED_EDGE ( 'NONE', *, *, #14885, .F. ) ;
#60971=EDGE_LOOP ( 'NONE', ( #73009, #18588, #70986 ) ) ;
#60972=CARTESIAN_POINT ( 'NONE',  ( 103.0168143257329092, -28.81349422576414554, 116.8844404487539634 ) ) ;
#60973=EDGE_CURVE ( 'NONE', #26689, #44076, #18261, .T. ) ;
#60974=FACE_BOUND ( 'NONE', #24548, .T. ) ;
#60975=CARTESIAN_POINT ( 'NONE',  ( 99.81116105471878086, -29.32005551970522461, 266.7051490854344706 ) ) ;
#60976=PLANE ( 'NONE',  #44815 ) ;
#60977=DIRECTION ( 'NONE',  ( 0.000000000000000000, 0.000000000000000000, -1.000000000000000000 ) ) ;
#60978=EDGE_CURVE ( 'NONE', #37421, #60824, #60024, .T. ) ;
#60979=AXIS2_PLACEMENT_3D ( 'NONE', #7949, #27490, #13867 ) ;
#60983=DIRECTION ( 'NONE',  ( -1.000000000000000078E-15, 1.000000000000000083E-30, 1.000000000000000000 ) ) ;
#60984=CARTESIAN_POINT ( 'NONE',  ( 106.4848323041101850, -24.91801670280273129, 195.1156252759109861 ) ) ;
#60985=FACE_OUTER_BOUND ( 'NONE', #24589, .T. ) ;
#60986=ORIENTED_EDGE ( 'NONE', *, *, #1554, .T. ) ;
#60987=EDGE_LOOP ( 'NONE', ( #1031, #81857, #18451, #85715 ) ) ;
#60988=DIRECTION ( 'NONE',  ( 0.000000000000000000, 0.000000000000000000, 1.000000000000000000 ) ) ;
#60989=CARTESIAN_POINT ( 'NONE',  ( 78.64819577387126515, -16.37139167074854385, 1.944749297849994951 ) ) ;
#60995=CARTESIAN_POINT ( 'NONE',  ( 113.0222799004901333, -45.32912119007338703, 203.0584824187679374 ) ) ;
#60996=ORIENTED_EDGE ( 'NONE', *, *, #49692, .F. ) ;
#60998=CARTESIAN_POINT ( 'NONE',  ( 19.56648329127400032, 15.62155284005900491, 328.6381252759109088 ) ) ;
#60999=CARTESIAN_POINT ( 'NONE',  ( 72.06648329127396835, -9.729447159941065237, 14.67562527591093513 ) ) ;
#61000=VECTOR ( 'NONE', #12049, 1000.000000000000000 ) ;
#61001=CARTESIAN_POINT ( 'NONE',  ( 105.2414988608755522, -45.18937368885499950, 30.23761417911497063 ) ) ;
#61002=CARTESIAN_POINT ( 'NONE',  ( 108.5929805111718593, -47.10003145027929605, 138.6927681330539883 ) ) ;
#61003=AXIS2_PLACEMENT_3D ( 'NONE', #44967, #30904, #10027 ) ;
#61005=ORIENTED_EDGE ( 'NONE', *, *, #65763, .T. ) ;
#61008=DIRECTION ( 'NONE',  ( 3.999999999999999995E-14, -1.000000000000000000, 4.100000000000000342E-29 ) ) ;
#61010=CIRCLE ( 'NONE', #62445, 2.029999999999997140 ) ;
#61013=ORIENTED_EDGE ( 'NONE', *, *, #39589, .F. ) ;
#61014=ORIENTED_EDGE ( 'NONE', *, *, #6225, .F. ) ;
#61016=CARTESIAN_POINT ( 'NONE',  ( 98.58519923211989067, -37.96229866499883343, 65.86384839950598291 ) ) ;
#61017=VECTOR ( 'NONE', #10856, 1000.000000000000000 ) ;
#61018=CARTESIAN_POINT ( 'NONE',  ( 107.5109734667377239, -47.16730098390026882, 237.6099109901969655 ) ) ;
#61019=CARTESIAN_POINT ( 'NONE',  ( 106.9751875180390641, -47.13234726572967759, 187.5699109901969734 ) ) ;
#61020=LINE ( 'NONE', #26957, #28688 ) ;
#61021=CARTESIAN_POINT ( 'NONE',  ( 118.1852327621006538, -40.75705396371408540, 19.54991099019698453 ) ) ;
#61022=FACE_OUTER_BOUND ( 'NONE', #77318, .T. ) ;
#61023=LINE ( 'NONE', #39240, #61271 ) ;
#61026=CARTESIAN_POINT ( 'NONE',  ( 97.81848045301514105, -40.53398251383325146, 111.6370493081401918 ) ) ;
#61027=CARTESIAN_POINT ( 'NONE',  ( 97.43243490695729747, -40.91715606259069204, 231.6527681330539679 ) ) ;
#61028=ORIENTED_EDGE ( 'NONE', *, *, #75235, .T. ) ;
#61029=CARTESIAN_POINT ( 'NONE',  ( 113.1555140577670215, -26.56262906569767068, 204.6470538473399756 ) ) ;
#61030=DIRECTION ( 'NONE',  ( 0.000000000000000000, 0.000000000000000000, -1.000000000000000000 ) ) ;
#61031=LINE ( 'NONE', #27407, #59480 ) ;
#61032=PLANE ( 'NONE',  #74652 ) ;
#61033=CARTESIAN_POINT ( 'NONE',  ( 113.9483801512686370, -32.56050311478266934, 277.6356252759111953 ) ) ;
#61034=DIRECTION ( 'NONE',  ( 0.000000000000000000, 0.000000000000000000, -1.000000000000000000 ) ) ;
#61035=CARTESIAN_POINT ( 'NONE',  ( 116.7951064495445905, -39.38790633866764779, 174.6147857624885660 ) ) ;
#61036=CARTESIAN_POINT ( 'NONE',  ( 32.09598329127729954, -23.42844715994138838, 237.4678068554150059 ) ) ;
#61039=AXIS2_PLACEMENT_3D ( 'NONE', #47414, #13368, #20631 ) ;
#61040=CARTESIAN_POINT ( 'NONE',  ( 50.88849390559499142, -32.11662333284530746, -5.074374724088000832 ) ) ;
#61041=DIRECTION ( 'NONE',  ( 0.000000000000000000, 0.000000000000000000, -1.000000000000000000 ) ) ;
#61044=DIRECTION ( 'NONE',  ( 0.000000000000000000, 0.000000000000000000, -1.000000000000000000 ) ) ;
#61046=ORIENTED_EDGE ( 'NONE', *, *, #59716, .F. ) ;
#61047=CARTESIAN_POINT ( 'NONE',  ( 181.8884939055948848, -32.11662333283959470, 117.4678068554150627 ) ) ;
#61048=CARTESIAN_POINT ( 'NONE',  ( 116.8782924623045290, -40.31758940317881468, 218.5470538473399529 ) ) ;
#61049=CARTESIAN_POINT ( 'NONE',  ( 101.6782318212999314, -27.07850282373152950, 101.4937205140059575 ) ) ;
#61050=CARTESIAN_POINT ( 'NONE',  ( 116.6456181429820447, -40.95237922671789477, 249.4956252759109532 ) ) ;
#61051=CARTESIAN_POINT ( 'NONE',  ( 193.0371591254585724, -47.82818131005411999, 117.4678068554150627 ) ) ;
#61055=DIRECTION ( 'NONE',  ( 1.000000000000000078E-15, -1.000000000000000000, 0.000000000000000000 ) ) ;
#61057=CARTESIAN_POINT ( 'NONE',  ( 132.2214349158059861, -20.77077206072004500, 2.188418444514679262 ) ) ;
#61059=ORIENTED_EDGE ( 'NONE', *, *, #86822, .T. ) ;
#61060=ORIENTED_EDGE ( 'NONE', *, *, #30084, .F. ) ;
#61062=CARTESIAN_POINT ( 'NONE',  ( 97.81853004928629503, -39.68680891125094234, 130.9952769709339577 ) ) ;
#61063=CARTESIAN_POINT ( 'NONE',  ( 25.56670390244797275, -62.87844715994099687, 137.2178068554150059 ) ) ;
#61065=CARTESIAN_POINT ( 'NONE',  ( 105.7994081972685194, -26.72404989547063181, 90.17573085178008796 ) ) ;
#61067=CARTESIAN_POINT ( 'NONE',  ( 95.69905522618357452, -33.46911247776740339, 137.1041967044819501 ) ) ;
#61068=CARTESIAN_POINT ( 'NONE',  ( 97.81168895331838087, -40.51742574516882200, 287.6356252759109680 ) ) ;
#61069=EDGE_CURVE ( 'NONE', #54835, #48081, #53271, .T. ) ;
#61073=EDGE_CURVE ( 'NONE', #79263, #11190, #28605, .T. ) ;
#61074=LINE ( 'NONE', #39292, #26562 ) ;
#61075=CARTESIAN_POINT ( 'NONE',  ( 98.34688518126456813, -32.29864090244028318, 50.95276813305393659 ) ) ;
#61077=VERTEX_POINT ( 'NONE', #39593 ) ;
#61081=CARTESIAN_POINT ( 'NONE',  ( 113.8941270090216733, -29.67983328691853018, 170.4641967044819637 ) ) ;
#61082=CARTESIAN_POINT ( 'NONE',  ( 184.5667039024480118, -67.87844715994100397, 20.91780685541479912 ) ) ;
#61083=LINE ( 'NONE', #54690, #85739 ) ;
#61090=CARTESIAN_POINT ( 'NONE',  ( 101.7670726180548115, -27.05576796868577460, 100.4632443235299633 ) ) ;
#61091=ORIENTED_EDGE ( 'NONE', *, *, #78150, .T. ) ;
#61092=VERTEX_POINT ( 'NONE', #13251 ) ;
#61093=VECTOR ( 'NONE', #20388, 1000.000000000000000 ) ;
#61094=ORIENTED_EDGE ( 'NONE', *, *, #33403, .T. ) ;
#61095=CARTESIAN_POINT ( 'NONE',  ( 107.0664832912739968, -36.72944715994100306, 287.6356252759109680 ) ) ;
#61097=CARTESIAN_POINT ( 'NONE',  ( 76.06670390244796920, -26.72944715994109899, 239.5838068554169809 ) ) ;
#61098=CARTESIAN_POINT ( 'NONE',  ( 107.7334136049453406, -44.89265071023657327, 175.4595189410199509 ) ) ;
#61104=DIRECTION ( 'NONE',  ( 1.000000000000000000, 0.000000000000000000, 0.000000000000000000 ) ) ;
#61107=VERTEX_POINT ( 'NONE', #19167 ) ;
#61109=LINE ( 'NONE', #34295, #21753 ) ;
#61110=CARTESIAN_POINT ( 'NONE',  ( 104.3066903214637620, -46.41728735870637479, 213.7872975916119458 ) ) ;
#61112=EDGE_CURVE ( 'NONE', #52724, #38949, #19919, .T. ) ;
#61115=ORIENTED_EDGE ( 'NONE', *, *, #47448, .T. ) ;
#61116=ORIENTED_EDGE ( 'NONE', *, *, #33629, .F. ) ;
#61117=VECTOR ( 'NONE', #60213, 1000.000000000000000 ) ;
#61121=EDGE_CURVE ( 'NONE', #72918, #51700, #67759, .T. ) ;
#61122=CARTESIAN_POINT ( 'NONE',  ( 115.2156275924750020, -36.25915663771239394, 226.6909475124489575 ) ) ;
#61123=CARTESIAN_POINT ( 'NONE',  ( 106.0743573402139930, -48.56370683269541644, 112.5099109901969712 ) ) ;
#61124=CARTESIAN_POINT ( 'NONE',  ( 113.4926247784321021, -28.54816540729036589, 79.54705384733995288 ) ) ;
#61125=CARTESIAN_POINT ( 'NONE',  ( 99.10784393885515442, -37.74513723391706321, 249.5838068554171514 ) ) ;
#61129=CARTESIAN_POINT ( 'NONE',  ( 109.4453082753925770, -25.93522777273083335, 175.8918157521009391 ) ) ;
#61135=EDGE_LOOP ( 'NONE', ( #36220, #60115, #67213, #14093 ) ) ;
#61138=AXIS2_PLACEMENT_3D ( 'NONE', #56580, #16164, #29786 ) ;
#61140=EDGE_CURVE ( 'NONE', #52939, #20535, #8318, .T. ) ;
#61141=CARTESIAN_POINT ( 'NONE',  ( 97.31591551022792430, -39.30615138698252053, 92.53147369008412682 ) ) ;
#61142=CARTESIAN_POINT ( 'NONE',  ( 101.6781192058861762, -27.07830111727894362, 105.4937205140069665 ) ) ;
#61143=CARTESIAN_POINT ( 'NONE',  ( 108.4212764309556150, -26.73551762798052778, 254.9689079379394059 ) ) ;
#61144=CARTESIAN_POINT ( 'NONE',  ( 172.5664832912729878, -27.57844715994070484, 261.9256252759120116 ) ) ;
#61145=LINE ( 'NONE', #26626, #54329 ) ;
#61146=CARTESIAN_POINT ( 'NONE',  ( 172.5664832912729878, -27.82844715994070484, 78.92562527591199739 ) ) ;
#61148=CARTESIAN_POINT ( 'NONE',  ( 96.16101635903912381, -35.07578045570940617, 217.1946728949589840 ) ) ;
#61149=DIRECTION ( 'NONE',  ( 1.000000000000000000, 0.000000000000000000, 0.000000000000000000 ) ) ;
#61150=DIRECTION ( 'NONE',  ( 0.000000000000000000, 0.000000000000000000, -1.000000000000000000 ) ) ;
#61151=ORIENTED_EDGE ( 'NONE', *, *, #61664, .F. ) ;
#61153=LINE ( 'NONE', #68871, #80297 ) ;
#61155=DIRECTION ( 'NONE',  ( 0.000000000000000000, 0.000000000000000000, 1.000000000000000000 ) ) ;
#61157=DIRECTION ( 'NONE',  ( -1.000000000000000000, -3.999999999999999995E-14, -1.000000000000000078E-15 ) ) ;
#61158=CARTESIAN_POINT ( 'NONE',  ( 96.63812674735558517, -35.80421970836195555, 231.2556252759109725 ) ) ;
#61159=ORIENTED_EDGE ( 'NONE', *, *, #49083, .F. ) ;
#61160=CYLINDRICAL_SURFACE ( 'NONE', #13241, 9.999999999999998224 ) ;
#61161=CARTESIAN_POINT ( 'NONE',  ( 117.5407444095047111, -36.54548251031545192, 284.8413395616252615 ) ) ;
#61162=CARTESIAN_POINT ( 'NONE',  ( 112.5087493249093455, -26.14677957921270846, 165.6984824187679521 ) ) ;
#61163=DIRECTION ( 'NONE',  ( 0.9963424814100680926, -0.08544974978095698503, 0.000000000000000000 ) ) ;
#61164=DIRECTION ( 'NONE',  ( -0.0001484127182050486030, 0.8660253910675250744, 0.5000000000000052180 ) ) ;
#61167=CARTESIAN_POINT ( 'NONE',  ( 97.31584368502818450, -39.30597587925219472, 191.5314585994741492 ) ) ;
#61168=DIRECTION ( 'NONE',  ( 1.000000000000000000, 4.163336342344333240E-14, 0.000000000000000000 ) ) ;
#61169=ORIENTED_EDGE ( 'NONE', *, *, #72063, .F. ) ;
#61174=VERTEX_POINT ( 'NONE', #5087 ) ;
#61175=DIRECTION ( 'NONE',  ( -1.000000000000000078E-15, 1.000000000000000083E-30, 1.000000000000000000 ) ) ;
#61176=CARTESIAN_POINT ( 'NONE',  ( 100.4929927897290582, -27.87207479535962662, 31.59657765686396758 ) ) ;
#61178=EDGE_CURVE ( 'NONE', #45388, #23016, #25684, .T. ) ;
#61180=LINE ( 'NONE', #59824, #56952 ) ;
#61181=CARTESIAN_POINT ( 'NONE',  ( 116.0578256703656308, -35.64850657512946697, 238.3562293518859576 ) ) ;
#61182=ORIENTED_EDGE ( 'NONE', *, *, #72938, .F. ) ;
#61184=ORIENTED_EDGE ( 'NONE', *, *, #17987, .T. ) ;
#61186=DIRECTION ( 'NONE',  ( 0.000000000000000000, 1.000000000000000000, 0.000000000000000000 ) ) ;
#61187=CARTESIAN_POINT ( 'NONE',  ( 98.38058909753313230, -41.69556604885146101, 101.7401552394820214 ) ) ;
#61189=CARTESIAN_POINT ( 'NONE',  ( 167.7413838386819691, -48.33240602328260849, 129.9678068554150059 ) ) ;
#61190=CARTESIAN_POINT ( 'NONE',  ( 100.4594818976507753, -42.68004899263244312, 53.34158330589694685 ) ) ;
#61191=CARTESIAN_POINT ( 'NONE',  ( 49.21437657594919557, -35.91149509761192604, 117.4678068554150485 ) ) ;
#61192=EDGE_CURVE ( 'NONE', #71209, #26208, #11228, .T. ) ;
#61193=CARTESIAN_POINT ( 'NONE',  ( 98.34939355853579457, -31.65741951873318172, 175.9065341848446451 ) ) ;
#61194=EDGE_CURVE ( 'NONE', #22726, #28809, #62337, .T. ) ;
#61195=CARTESIAN_POINT ( 'NONE',  ( 117.9377692877172450, -39.05906590213767515, 258.6584824187686422 ) ) ;
#61196=CARTESIAN_POINT ( 'NONE',  ( 156.5667039024483813, -48.82844715993569196, 257.2178068554149490 ) ) ;
#61197=AXIS2_PLACEMENT_3D ( 'NONE', #24459, #72164, #9939 ) ;
#61198=VERTEX_POINT ( 'NONE', #55893 ) ;
#61199=CARTESIAN_POINT ( 'NONE',  ( 33.91903122894529332, -35.91149509761239500, 313.9678068554150059 ) ) ;
#61201=CARTESIAN_POINT ( 'NONE',  ( 112.0721450080970669, -44.54221119967598241, 65.84809036959194373 ) ) ;
#61202=AXIS2_PLACEMENT_3D ( 'NONE', #42169, #6768, #34468 ) ;
#61203=AXIS2_PLACEMENT_3D ( 'NONE', #78026, #71210, #36685 ) ;
#61204=CARTESIAN_POINT ( 'NONE',  ( 97.80798641811291816, -40.50837052410136607, 131.6348463817457457 ) ) ;
#61205=DIRECTION ( 'NONE',  ( 0.000000000000000000, 0.000000000000000000, 1.000000000000000000 ) ) ;
#61207=DIRECTION ( 'NONE',  ( -1.000000000000000000, 1.011922027653136551E-15, 0.000000000000000000 ) ) ;
#61208=VERTEX_POINT ( 'NONE', #21413 ) ;
#61209=CARTESIAN_POINT ( 'NONE',  ( 107.0664832912750057, -36.72944715993903486, 6.826283056785790393 ) ) ;
#61210=ORIENTED_EDGE ( 'NONE', *, *, #12054, .F. ) ;
#61211=CARTESIAN_POINT ( 'NONE',  ( 114.0810491752689160, -44.48971597834975000, 133.1613395616249989 ) ) ;
#61213=CARTESIAN_POINT ( 'NONE',  ( 114.9386757252747771, -33.34113070369811993, 78.57241982807700253 ) ) ;
#61214=AXIS2_PLACEMENT_3D ( 'NONE', #67859, #52838, #13352 ) ;
#61215=CARTESIAN_POINT ( 'NONE',  ( 182.5667039024477276, -33.35206098992156853, 237.4678068554150059 ) ) ;
#61216=CARTESIAN_POINT ( 'NONE',  ( 97.68334685095105385, -37.21243378447991290, 117.8111071154209526 ) ) ;
#61217=AXIS2_PLACEMENT_3D ( 'NONE', #36664, #50723, #71191 ) ;
#61220=CARTESIAN_POINT ( 'NONE',  ( 96.90588099414922851, -39.15831928773680914, 52.51276813305394597 ) ) ;
#61222=CARTESIAN_POINT ( 'NONE',  ( 123.6837132603318707, -22.62993780205705718, 229.5838068554170093 ) ) ;
#61223=ORIENTED_EDGE ( 'NONE', *, *, #20381, .T. ) ;
#61224=DIRECTION ( 'NONE',  ( 0.000000000000000000, 0.000000000000000000, -1.000000000000000000 ) ) ;
#61225=ORIENTED_EDGE ( 'NONE', *, *, #80285, .T. ) ;
#61227=EDGE_CURVE ( 'NONE', #24376, #39785, #76369, .T. ) ;
#61230=CARTESIAN_POINT ( 'NONE',  ( 99.87094702832891358, -29.26198151734318742, 265.6746728949591443 ) ) ;
#61231=CARTESIAN_POINT ( 'NONE',  ( 111.8040564975826356, -25.84011059577494152, 130.7499109901969518 ) ) ;
#61232=DIRECTION ( 'NONE',  ( 0.000000000000000000, 0.000000000000000000, -1.000000000000000000 ) ) ;
#61234=CARTESIAN_POINT ( 'NONE',  ( 96.08760325403525826, -38.00935872415581684, 82.43086337114895912 ) ) ;
#61235=LINE ( 'NONE', #82161, #24786 ) ;
#61236=ORIENTED_EDGE ( 'NONE', *, *, #12427, .T. ) ;
#61238=DIRECTION ( 'NONE',  ( 0.000000000000000000, 0.000000000000000000, 1.000000000000000000 ) ) ;
#61244=CARTESIAN_POINT ( 'NONE',  ( 41.56648329127499153, -32.07844715994070839, 258.9256252759120116 ) ) ;
#61245=CARTESIAN_POINT ( 'NONE',  ( 101.0991643652557173, -45.25116564454923207, 282.0899109901967563 ) ) ;
#61246=CARTESIAN_POINT ( 'NONE',  ( 179.1667039024460166, -28.27351298637280408, -5.074374724088000832 ) ) ;
#61248=DIRECTION ( 'NONE',  ( 4.299999999999999979E-14, -1.000000000000000000, 4.400000000000000367E-29 ) ) ;
#61249=CARTESIAN_POINT ( 'NONE',  ( 97.30224646447496184, -33.23681714893609751, 26.06514908543594444 ) ) ;
#61251=CARTESIAN_POINT ( 'NONE',  ( 113.9025887763447997, -28.07314977735667938, 120.5565776568639507 ) ) ;
#61253=CARTESIAN_POINT ( 'NONE',  ( 108.9531560784502915, -26.39541311287850434, 164.9327681330529742 ) ) ;
#61255=DIRECTION ( 'NONE',  ( 1.000000000000000078E-15, -1.000000000000000083E-30, -1.000000000000000000 ) ) ;
#61259=VERTEX_POINT ( 'NONE', #1866 ) ;
#61261=AXIS2_PLACEMENT_3D ( 'NONE', #54356, #6251, #74393 ) ;
#61262=EDGE_CURVE ( 'NONE', #89527, #63276, #40197, .T. ) ;
#61263=CARTESIAN_POINT ( 'NONE',  ( 99.09656185782638715, -30.54930221101325927, 61.80248345295675705 ) ) ;
#61264=CARTESIAN_POINT ( 'NONE',  ( 111.8142338872566626, -25.81671781287135303, 134.7499109901969518 ) ) ;
#61266=LINE ( 'NONE', #88549, #40775 ) ;
#61267=CARTESIAN_POINT ( 'NONE',  ( 107.0664832912750057, -36.72944715993903486, 0.4256252759109709349 ) ) ;
#61268=DIRECTION ( 'NONE',  ( 5.512527431108029424E-15, -1.000000000000000000, 0.000000000000000000 ) ) ;
#61271=VECTOR ( 'NONE', #46028, 1000.000000000000000 ) ;
#61272=EDGE_CURVE ( 'NONE', #77176, #38542, #43621, .T. ) ;
#61273=ORIENTED_EDGE ( 'NONE', *, *, #53565, .F. ) ;
#61275=AXIS2_PLACEMENT_3D ( 'NONE', #72010, #85651, #25177 ) ;
#61278=CARTESIAN_POINT ( 'NONE',  ( 112.8677825012601375, -28.59025478454122648, 249.5838084826162913 ) ) ;
#61279=CARTESIAN_POINT ( 'NONE',  ( 179.4595971212720258, -26.00627455219131789, -5.074374724088000832 ) ) ;
#61280=EDGE_CURVE ( 'NONE', #37453, #8408, #76817, .T. ) ;
#61283=LINE ( 'NONE', #6328, #80494 ) ;
#61284=CARTESIAN_POINT ( 'NONE',  ( 99.09554038107577867, -30.55064579012594450, 180.8023132925306129 ) ) ;
#61286=CYLINDRICAL_SURFACE ( 'NONE', #65949, 2.500000000000002220 ) ;
#61288=CARTESIAN_POINT ( 'NONE',  ( 109.9476544338203041, -26.76763818355061986, 210.8403871806729626 ) ) ;
#61290=EDGE_LOOP ( 'NONE', ( #33823, #68610, #49488, #37454 ) ) ;
#61291=EDGE_CURVE ( 'NONE', #33391, #81541, #30018, .T. ) ;
#61293=CARTESIAN_POINT ( 'NONE',  ( 96.20363159075265003, -34.36081134307599427, 102.1556252759109640 ) ) ;
#61294=DIRECTION ( 'NONE',  ( 0.000000000000000000, -1.000000000000000000, 0.000000000000000000 ) ) ;
#61297=EDGE_CURVE ( 'NONE', #27267, #56032, #14143, .T. ) ;
#61298=DIRECTION ( 'NONE',  ( 1.367269734760046851E-14, -1.000000000000000000, 0.000000000000000000 ) ) ;
#61299=VERTEX_POINT ( 'NONE', #961 ) ;
#61302=ORIENTED_EDGE ( 'NONE', *, *, #19498, .F. ) ;
#61303=ORIENTED_EDGE ( 'NONE', *, *, #76905, .F. ) ;
#61304=CARTESIAN_POINT ( 'NONE',  ( 115.3890540380527767, -39.77298043176836018, 214.9787261630399655 ) ) ;
#61306=CARTESIAN_POINT ( 'NONE',  ( 99.08970433676087453, -42.79570825176563176, 52.84354550488869506 ) ) ;
#61309=CARTESIAN_POINT ( 'NONE',  ( 165.6738106836047280, -28.98061976758432223, 117.4678068554150485 ) ) ;
#61310=ORIENTED_EDGE ( 'NONE', *, *, #69193, .T. ) ;
#61312=DIRECTION ( 'NONE',  ( 0.000000000000000000, 0.000000000000000000, -1.000000000000000000 ) ) ;
#61314=CARTESIAN_POINT ( 'NONE',  ( 116.5166575185069462, -42.41785904284980546, 278.3832443235298797 ) ) ;
#61316=CARTESIAN_POINT ( 'NONE',  ( 106.3397725667592368, -45.35341472531973750, 260.3157094172105417 ) ) ;
#61318=CARTESIAN_POINT ( 'NONE',  ( 103.6907823165633005, -45.90921117331532741, 142.2956252759109645 ) ) ;
#61321=DIRECTION ( 'NONE',  ( 1.000000000000000078E-15, 1.000000000000000083E-30, -1.000000000000000000 ) ) ;
#61323=CARTESIAN_POINT ( 'NONE',  ( 115.2859307195537326, -30.18890446381676540, 240.3613395616249875 ) ) ;
#61324=CARTESIAN_POINT ( 'NONE',  ( 19.56648329127303043, -81.37844715994266664, 361.9756252759109998 ) ) ;
#61325=ORIENTED_EDGE ( 'NONE', *, *, #1705, .T. ) ;
#61326=CARTESIAN_POINT ( 'NONE',  ( 113.4862441490110427, -46.74931658189198913, 64.02991099019695298 ) ) ;
#61327=DIRECTION ( 'NONE',  ( -3.999999999999999995E-14, 1.000000000000000000, -4.100000000000000342E-29 ) ) ;
#61328=ORIENTED_EDGE ( 'NONE', *, *, #48131, .F. ) ;
#61329=ORIENTED_EDGE ( 'NONE', *, *, #39436, .T. ) ;
#61330=ORIENTED_EDGE ( 'NONE', *, *, #57384, .F. ) ;
#61332=CARTESIAN_POINT ( 'NONE',  ( 97.07201853420016846, -35.37896439202069843, 161.2187929919405178 ) ) ;
#61333=CARTESIAN_POINT ( 'NONE',  ( 34.96670390244699433, -28.27351298637401200, 237.4678068554150059 ) ) ;
#61334=LINE ( 'NONE', #467, #88636 ) ;
#61335=CARTESIAN_POINT ( 'NONE',  ( 19.56670390244796920, -67.87844715994100397, 310.9178068554150514 ) ) ;
#61336=CARTESIAN_POINT ( 'NONE',  ( 99.71285092336476907, -40.27258376677666263, 169.5023760838769817 ) ) ;
#61337=CARTESIAN_POINT ( 'NONE',  ( 115.0714481855697926, -30.01693675811307571, 265.3813395616251682 ) ) ;
#61338=CARTESIAN_POINT ( 'NONE',  ( 101.9928070043063002, -45.44557658641289777, 58.15638151446928106 ) ) ;
#61339=VERTEX_POINT ( 'NONE', #1421 ) ;
#61341=CARTESIAN_POINT ( 'NONE',  ( 134.0664832912740110, -39.47944715994100306, 1.625625275910997480 ) ) ;
#61342=EDGE_LOOP ( 'NONE', ( #35641, #18757 ) ) ;
#61344=CARTESIAN_POINT ( 'NONE',  ( 179.8585841295800094, -30.08671355700241179, 342.9256252759119548 ) ) ;
#61345=EDGE_CURVE ( 'NONE', #13942, #46554, #78186, .T. ) ;
#61346=VERTEX_POINT ( 'NONE', #84553 ) ;
#61347=ORIENTED_EDGE ( 'NONE', *, *, #7965, .F. ) ;
#61348=DIRECTION ( 'NONE',  ( 0.000000000000000000, 0.000000000000000000, -1.000000000000000000 ) ) ;
#61349=CARTESIAN_POINT ( 'NONE',  ( 97.06382796133792112, -37.34203019285121883, 16.37521711361123167 ) ) ;
#61351=CARTESIAN_POINT ( 'NONE',  ( 97.81169409577289287, -40.51741657705139232, 81.63570706759205109 ) ) ;
#61352=CARTESIAN_POINT ( 'NONE',  ( 194.0371591254572934, -24.89890238294407965, 300.4678068554149490 ) ) ;
#61353=CARTESIAN_POINT ( 'NONE',  ( 107.5470202762386549, -45.24887850357546171, 152.0438483995049523 ) ) ;
#61354=CARTESIAN_POINT ( 'NONE',  ( 96.13137017992535505, -38.63632546489608188, 46.45181575210094138 ) ) ;
#61357=VERTEX_POINT ( 'NONE', #49986 ) ;
#61358=EDGE_CURVE ( 'NONE', #38912, #25851, #42276, .T. ) ;
#61360=LINE ( 'NONE', #26844, #73128 ) ;
#61363=EDGE_CURVE ( 'NONE', #28268, #26420, #66327, .T. ) ;
#61365=VERTEX_POINT ( 'NONE', #18156 ) ;
#61368=CARTESIAN_POINT ( 'NONE',  ( 116.9857065628338688, -35.32450652603309038, 133.9383772284687382 ) ) ;
#61369=ADVANCED_FACE ( 'NONE', ( #80404 ), #9573, .F. ) ;
#61370=ADVANCED_FACE ( 'NONE', ( #44962 ), #17283, .T. ) ;
#61372=DIRECTION ( 'NONE',  ( 0.7071067811868035902, 0.7071067811862914443, 7.071067811868029270E-16 ) ) ;
#61373=ORIENTED_EDGE ( 'NONE', *, *, #2652, .T. ) ;
#61374=CARTESIAN_POINT ( 'NONE',  ( 99.96564438395634511, -44.39263518965486099, 46.98133956162592284 ) ) ;
#61375=CARTESIAN_POINT ( 'NONE',  ( 116.1615364674122333, -29.05539214145830229, 70.38419670448192278 ) ) ;
#61376=EDGE_CURVE ( 'NONE', #70860, #63937, #88074, .T. ) ;
#61377=LINE ( 'NONE', #89101, #78227 ) ;
#61378=CARTESIAN_POINT ( 'NONE',  ( 76.06670390244805446, -58.72944715994109544, 239.5838068554169809 ) ) ;
#61379=CARTESIAN_POINT ( 'NONE',  ( 63.03715912545735023, -24.42818131006027826, 249.9678068554150343 ) ) ;
#61380=LINE ( 'NONE', #20953, #78986 ) ;
#61382=DIRECTION ( 'NONE',  ( 0.000000000000000000, 0.000000000000000000, -1.000000000000000000 ) ) ;
#61384=CARTESIAN_POINT ( 'NONE',  ( 41.56648329127399677, 0.2215528400590013880, 138.9256252759119832 ) ) ;
#61385=CARTESIAN_POINT ( 'NONE',  ( 31.56670390244800828, -32.29483332968611364, -5.074374724088000832 ) ) ;
#61386=ORIENTED_EDGE ( 'NONE', *, *, #35212, .F. ) ;
#61387=CARTESIAN_POINT ( 'NONE',  ( 104.7547631156620014, -46.91734236372032996, 68.39848241876794077 ) ) ;
#61390=CARTESIAN_POINT ( 'NONE',  ( 83.06670390244796920, -58.35344715994099829, 210.8338068554149913 ) ) ;
#61391=TOROIDAL_SURFACE ( 'NONE', #15053, 11.75000000000000000, 2.125000000000000000 ) ;
#61392=CIRCLE ( 'NONE', #36721, 4.750000000000004441 ) ;
#61393=FACE_OUTER_BOUND ( 'NONE', #16719, .T. ) ;
#61394=VERTEX_POINT ( 'NONE', #4541 ) ;
#61395=CARTESIAN_POINT ( 'NONE',  ( 98.70071965984716655, -42.85747980491196074, 102.8175300378149899 ) ) ;
#61398=CARTESIAN_POINT ( 'NONE',  ( 96.99990081654259200, -39.35482002063352525, 272.5299109901966972 ) ) ;
#61399=DIRECTION ( 'NONE',  ( -0.000000000000000000, -0.000000000000000000, -1.000000000000000000 ) ) ;
#61402=CARTESIAN_POINT ( 'NONE',  ( 112.1393456477353539, -28.01282278493161471, 80.65645860868352202 ) ) ;
#61403=EDGE_CURVE ( 'NONE', #34565, #55396, #58159, .T. ) ;
#61407=CARTESIAN_POINT ( 'NONE',  ( 116.5994914424366016, -40.81117973626242446, 213.5165776568640013 ) ) ;
#61409=EDGE_LOOP ( 'NONE', ( #10923, #17465, #81830, #53980 ) ) ;
#61410=CARTESIAN_POINT ( 'NONE',  ( 98.99527800849182313, -31.91985561591122078, 127.3425356868499705 ) ) ;
#61411=CARTESIAN_POINT ( 'NONE',  ( 177.4809174648215162, -48.32844715993478246, 180.4678068554150059 ) ) ;
#61412=CARTESIAN_POINT ( 'NONE',  ( 101.6507727546967743, -27.01955209951630010, 251.4813395616246510 ) ) ;
#61413=CARTESIAN_POINT ( 'NONE',  ( 107.0667039024468039, -18.72944715994100306, 199.5838068554169809 ) ) ;
#61416=DIRECTION ( 'NONE',  ( -1.000000000000000000, -4.299999999999999979E-14, -1.000000000000000078E-15 ) ) ;
#61418=VECTOR ( 'NONE', #5107, 1000.000000000000000 ) ;
#61419=CYLINDRICAL_SURFACE ( 'NONE', #14456, 4.750000000000000888 ) ;
#61421=CARTESIAN_POINT ( 'NONE',  ( 96.66614461754329568, -36.48121138304695421, 196.3070538473399438 ) ) ;
#61422=CARTESIAN_POINT ( 'NONE',  ( 172.5664832912740110, -9.303447159940999356, 16.80862527591200006 ) ) ;
#61423=EDGE_LOOP ( 'NONE', ( #7075, #71185, #81697, #88776 ) ) ;
#61424=ORIENTED_EDGE ( 'NONE', *, *, #21002, .F. ) ;
#61426=CARTESIAN_POINT ( 'NONE',  ( 81.20964327717335607, -21.23067567606010542, 8.021372095558360726 ) ) ;
#61427=CARTESIAN_POINT ( 'NONE',  ( 116.3265940946004378, -32.93621273019581253, 125.1356252759109680 ) ) ;
#61428=DIRECTION ( 'NONE',  ( -4.237773401492740281E-14, 1.000000000000000000, 0.000000000000000000 ) ) ;
#61430=CARTESIAN_POINT ( 'NONE',  ( 80.06648329127399677, -8.729447159940999512, 293.6356252759119911 ) ) ;
#61432=CARTESIAN_POINT ( 'NONE',  ( 115.7817079743517610, -41.80467255062060161, 63.40624212070690646 ) ) ;
#61433=CARTESIAN_POINT ( 'NONE',  ( 113.1001805014122255, -45.99085015462044623, 223.0480062282919675 ) ) ;
#61434=VERTEX_POINT ( 'NONE', #11348 ) ;
#61438=CARTESIAN_POINT ( 'NONE',  ( 115.7905465638341553, -39.88961339014866070, 21.36809036959191843 ) ) ;
#61439=CARTESIAN_POINT ( 'NONE',  ( 114.2549023322775383, -45.16142510923258868, 149.1508633711489722 ) ) ;
#61440=CARTESIAN_POINT ( 'NONE',  ( 182.2300522401172032, -33.89581943343727488, 193.9678068554150059 ) ) ;
#61443=ADVANCED_FACE ( 'NONE', ( #31341 ), #59031, .F. ) ;
#61444=CARTESIAN_POINT ( 'NONE',  ( 116.7350617727581721, -39.61171646336399732, 68.59767641480858913 ) ) ;
#61445=EDGE_LOOP ( 'NONE', ( #47230, #5218, #36889, #68839 ) ) ;
#61449=ORIENTED_EDGE ( 'NONE', *, *, #74317, .T. ) ;
#61450=VERTEX_POINT ( 'NONE', #24541 ) ;
#61451=PLANE ( 'NONE',  #52611 ) ;
#61452=VECTOR ( 'NONE', #12663, 1000.000000000000114 ) ;
#61455=CARTESIAN_POINT ( 'NONE',  ( 115.4237413257435918, -38.49363815508749553, 63.08384839950497991 ) ) ;
#61456=CARTESIAN_POINT ( 'NONE',  ( 110.7409072761653306, -26.27985149715145496, 254.8194347997204545 ) ) ;
#61458=CARTESIAN_POINT ( 'NONE',  ( 101.4165038149807003, -45.50681337102575696, 222.1213395616249784 ) ) ;
#61459=CARTESIAN_POINT ( 'NONE',  ( 116.3162492855249894, -32.94856389518969308, 154.1356252759109680 ) ) ;
#61460=CARTESIAN_POINT ( 'NONE',  ( 104.6539710028519039, -47.49251396406760506, 23.38895860924494841 ) ) ;
#61461=CARTESIAN_POINT ( 'NONE',  ( 34.33598329127389803, -36.32844715994140472, 180.4678068554150911 ) ) ;
#61463=ADVANCED_FACE ( 'NONE', ( #73571 ), #10020, .F. ) ;
#61464=ORIENTED_EDGE ( 'NONE', *, *, #70312, .T. ) ;
#61466=CARTESIAN_POINT ( 'NONE',  ( 98.87588542518393808, -42.07524381596793006, 101.7870538473399620 ) ) ;
#61467=CARTESIAN_POINT ( 'NONE',  ( 109.9230826530363743, -46.83843495353658426, 72.79562527591099297 ) ) ;
#61468=CARTESIAN_POINT ( 'NONE',  ( 112.6874404347162084, -45.56185944854193792, 263.0270538473394026 ) ) ;
#61470=VERTEX_POINT ( 'NONE', #6770 ) ;
#61471=CARTESIAN_POINT ( 'NONE',  ( 116.7954078171858896, -40.57313474401875197, 193.5270538473389479 ) ) ;
#61472=DIRECTION ( 'NONE',  ( -0.9254794337955620787, -0.3787978585227822492, 0.000000000000000000 ) ) ;
#61473=VECTOR ( 'NONE', #2991, 1000.000000000000000 ) ;
#61474=AXIS2_PLACEMENT_3D ( 'NONE', #11669, #44828, #65289 ) ;
#61476=CARTESIAN_POINT ( 'NONE',  ( 108.8575270723005133, -46.65742102077504683, 28.72049499546754703 ) ) ;
#61477=CARTESIAN_POINT ( 'NONE',  ( 114.8786280730279401, -39.65240915455324000, 277.6356252759111953 ) ) ;
#61478=DIRECTION ( 'NONE',  ( 0.000000000000000000, 0.000000000000000000, -1.000000000000000000 ) ) ;
#61484=CARTESIAN_POINT ( 'NONE',  ( 80.06648329127402519, -36.72944715994107412, -5.074374724089057764 ) ) ;
#61485=CARTESIAN_POINT ( 'NONE',  ( 57.56670390244722313, -42.82844715994040996, 137.2178068554150911 ) ) ;
#61488=CARTESIAN_POINT ( 'NONE',  ( 100.7306467531667096, -29.72269365876263336, 195.5838068554173788 ) ) ;
#61489=EDGE_LOOP ( 'NONE', ( #40313, #38556, #55449, #11839 ) ) ;
#61490=CARTESIAN_POINT ( 'NONE',  ( 142.8698897858160421, -0.9167816978817300289, 361.9756252759100335 ) ) ;
#61491=CARTESIAN_POINT ( 'NONE',  ( 114.8305014334234642, -29.68612513766509053, 209.4127681330539872 ) ) ;
#61492=CARTESIAN_POINT ( 'NONE',  ( 116.7955140328789412, -32.98399009599280873, 135.1184824187679396 ) ) ;
#61493=CARTESIAN_POINT ( 'NONE',  ( 96.20418022731425367, -34.44737123974878301, 257.1737205140064475 ) ) ;
#61494=CARTESIAN_POINT ( 'NONE',  ( 41.56648329127499153, -32.07844715994070839, 254.1756252759120400 ) ) ;
#61495=CARTESIAN_POINT ( 'NONE',  ( 172.5664832912740110, -18.82844715994099971, 21.04262527591200183 ) ) ;
#61498=LINE ( 'NONE', #39710, #71187 ) ;
#61499=CARTESIAN_POINT ( 'NONE',  ( 131.9645448811607480, -20.51222316633629106, 2.376608873918129028 ) ) ;
#61500=ORIENTED_EDGE ( 'NONE', *, *, #21086, .T. ) ;
#61502=CARTESIAN_POINT ( 'NONE',  ( 112.1993679394656453, -43.55657132036190404, 142.5124198280769576 ) ) ;
#61506=CARTESIAN_POINT ( 'NONE',  ( 96.05093434719803724, -37.29646042206077539, 117.3794347997199594 ) ) ;
#61509=DIRECTION ( 'NONE',  ( 1.000000000000000000, 4.163336342344333240E-14, 0.000000000000000000 ) ) ;
#61510=CARTESIAN_POINT ( 'NONE',  ( 105.7154773365650158, -46.72385839300680743, 108.4689586097351395 ) ) ;
#61512=CARTESIAN_POINT ( 'NONE',  ( 101.5079035968563943, -28.64143341885324290, 50.55562527591095545 ) ) ;
#61513=ORIENTED_EDGE ( 'NONE', *, *, #42997, .T. ) ;
#61516=CIRCLE ( 'NONE', #58655, 27.99999999999999645 ) ;
#61517=DIRECTION ( 'NONE',  ( 0.9068632946707805287, -0.4214249218767882055, 8.896017825522093530E-16 ) ) ;
#61518=CARTESIAN_POINT ( 'NONE',  ( 107.9488082096507213, -26.98745991040269487, 151.0041967044819557 ) ) ;
#61521=FACE_OUTER_BOUND ( 'NONE', #80635, .T. ) ;
#61522=CARTESIAN_POINT ( 'NONE',  ( 25.56670390244797275, -65.37844715994100397, 173.2178068554149775 ) ) ;
#61525=DIRECTION ( 'NONE',  ( 5.512527431108029424E-15, -1.000000000000000000, 0.000000000000000000 ) ) ;
#61526=CARTESIAN_POINT ( 'NONE',  ( 101.6894933626719819, -27.09867346898205298, 105.4937205140069665 ) ) ;
#61530=EDGE_CURVE ( 'NONE', #10583, #22550, #39648, .T. ) ;
#61531=LINE ( 'NONE', #41531, #933 ) ;
#61533=FACE_OUTER_BOUND ( 'NONE', #59119, .T. ) ;
#61534=CARTESIAN_POINT ( 'NONE',  ( 114.3355458017429811, -42.49630604348746488, 196.1109475124489450 ) ) ;
#61535=EDGE_CURVE ( 'NONE', #63584, #52727, #48934, .T. ) ;
#61536=VECTOR ( 'NONE', #33292, 1000.000000000000000 ) ;
#61537=CIRCLE ( 'NONE', #9491, 27.99999999999999645 ) ;
#61539=AXIS2_PLACEMENT_3D ( 'NONE', #20166, #13787, #26975 ) ;
#61540=CARTESIAN_POINT ( 'NONE',  ( 98.35006428047149996, -31.65621667114429982, 26.90604011017519781 ) ) ;
#61541=EDGE_LOOP ( 'NONE', ( #58857, #14853, #76490, #59117 ) ) ;
#61543=ORIENTED_EDGE ( 'NONE', *, *, #1049, .F. ) ;
#61544=DIRECTION ( 'NONE',  ( 0.7071067811865171526, 0.7071067811865779928, 7.071067811865164719E-16 ) ) ;
#61545=AXIS2_PLACEMENT_3D ( 'NONE', #81624, #19374, #32990 ) ;
#61547=FACE_OUTER_BOUND ( 'NONE', #27040, .T. ) ;
#61548=VERTEX_POINT ( 'NONE', #28097 ) ;
#61551=CARTESIAN_POINT ( 'NONE',  ( 114.9810172151485546, -40.71547668563403022, 199.8872975916109453 ) ) ;
#61552=CARTESIAN_POINT ( 'NONE',  ( 49.35031423293201414, -29.99615139349890569, -5.074374724088000832 ) ) ;
#61555=EDGE_LOOP ( 'NONE', ( #27306, #8467, #42065, #32829 ) ) ;
#61556=DIRECTION ( 'NONE',  ( 0.000000000000000000, 1.000000000000000000, 0.000000000000000000 ) ) ;
#61557=VERTEX_POINT ( 'NONE', #27664 ) ;
#61558=ORIENTED_EDGE ( 'NONE', *, *, #44066, .F. ) ;
#61560=EDGE_CURVE ( 'NONE', #462, #70290, #84444, .T. ) ;
#61561=CARTESIAN_POINT ( 'NONE',  ( 113.6834210241909346, -31.15118039646248249, 222.1899951314959480 ) ) ;
#61562=CARTESIAN_POINT ( 'NONE',  ( 102.6883137591737665, -46.90427260131782106, 137.2651490854349561 ) ) ;
#61563=EDGE_CURVE ( 'NONE', #88639, #26855, #83530, .T. ) ;
#61564=CARTESIAN_POINT ( 'NONE',  ( 107.8666756518570935, -26.35696637107986717, 70.01562527591099183 ) ) ;
#61565=CARTESIAN_POINT ( 'NONE',  ( 114.4593534627794895, -41.96027977772990170, 249.5838068554169809 ) ) ;
#61566=FACE_OUTER_BOUND ( 'NONE', #27789, .T. ) ;
#61567=CARTESIAN_POINT ( 'NONE',  ( 95.40797249125856183, -38.85400393358575855, 197.4699109901969791 ) ) ;
#61568=DIRECTION ( 'NONE',  ( 1.000000000000000000, 4.163336342344333240E-14, 0.000000000000000000 ) ) ;
#61569=EDGE_LOOP ( 'NONE', ( #27819, #8927 ) ) ;
#61571=ORIENTED_EDGE ( 'NONE', *, *, #55245, .F. ) ;
#61578=CARTESIAN_POINT ( 'NONE',  ( 98.85774631673514534, -43.21346936515602266, 91.85848241876892928 ) ) ;
#61580=AXIS2_PLACEMENT_3D ( 'NONE', #32208, #81293, #59906 ) ;
#61581=CARTESIAN_POINT ( 'NONE',  ( 136.5762189171787782, -35.60488046388145023, 7.068409955839482173 ) ) ;
#61582=CARTESIAN_POINT ( 'NONE',  ( 51.56670390244899238, -32.29483332968450782, -5.074374724088000832 ) ) ;
#61583=CARTESIAN_POINT ( 'NONE',  ( 109.6430121229215615, -46.48008673730067386, 143.7814586086184931 ) ) ;
#61585=CARTESIAN_POINT ( 'NONE',  ( 96.14807755961388125, -35.16348456217431107, 222.2251490854349640 ) ) ;
#61587=CARTESIAN_POINT ( 'NONE',  ( 134.0664832912740110, 0.2215528400590013880, 291.1181252759119502 ) ) ;
#61590=DIRECTION ( 'NONE',  ( 0.000000000000000000, 0.000000000000000000, -1.000000000000000000 ) ) ;
#61591=CARTESIAN_POINT ( 'NONE',  ( 182.0667039024469886, -33.35206098992630075, -5.074374724088000832 ) ) ;
#61593=DIRECTION ( 'NONE',  ( 0.000000000000000000, 0.000000000000000000, -1.000000000000000000 ) ) ;
#61594=CARTESIAN_POINT ( 'NONE',  ( 101.6276731664663089, -45.67517298127779668, 247.1413395616249602 ) ) ;
#61596=CARTESIAN_POINT ( 'NONE',  ( 109.0243740707360018, -26.89372415866576205, 194.9199838810998529 ) ) ;
#61597=CARTESIAN_POINT ( 'NONE',  ( 111.7834783340718872, -46.75425468364281301, 283.9146728949586418 ) ) ;
#61598=CARTESIAN_POINT ( 'NONE',  ( 96.57517526037739231, -36.20937929227457630, 167.2870538473399620 ) ) ;
#61600=CYLINDRICAL_SURFACE ( 'NONE', #54746, 2.750000000000002665 ) ;
#61602=LINE ( 'NONE', #75259, #71815 ) ;
#61603=CARTESIAN_POINT ( 'NONE',  ( 97.33784133871502320, -34.07106443143205610, 191.1147919345066555 ) ) ;
#61609=CIRCLE ( 'NONE', #61539, 2.029999999999997140 ) ;
#61610=ORIENTED_EDGE ( 'NONE', *, *, #3400, .T. ) ;
#61611=ORIENTED_EDGE ( 'NONE', *, *, #12982, .F. ) ;
#61612=CIRCLE ( 'NONE', #5015, 1.000000000000000888 ) ;
#61616=CARTESIAN_POINT ( 'NONE',  ( 97.50674219252222485, -32.62548708300533207, 12.00419670448293985 ) ) ;
#61621=CARTESIAN_POINT ( 'NONE',  ( 115.5937312905896022, -36.23733611532740184, 228.2952769709339691 ) ) ;
#61622=ORIENTED_EDGE ( 'NONE', *, *, #37132, .T. ) ;
#61623=VERTEX_POINT ( 'NONE', #852 ) ;
#61625=CYLINDRICAL_SURFACE ( 'NONE', #81998, 2.517500000000005844 ) ;
#61626=CARTESIAN_POINT ( 'NONE',  ( 112.0533716870284593, -45.40352459978532806, 182.9916912538479039 ) ) ;
#61629=CIRCLE ( 'NONE', #12303, 2.517499999999998739 ) ;
#61631=CYLINDRICAL_SURFACE ( 'NONE', #64753, 2.517500000000000071 ) ;
#61632=CARTESIAN_POINT ( 'NONE',  ( 97.06112323502817674, -37.99668350201224598, 176.4273135337378449 ) ) ;
#61633=CARTESIAN_POINT ( 'NONE',  ( 100.5669465097397506, -44.03830869352251653, 266.9984824187685604 ) ) ;
#61636=DIRECTION ( 'NONE',  ( 1.000000000000000078E-15, -1.000000000000000083E-30, -1.000000000000000000 ) ) ;
#61637=DIRECTION ( 'NONE',  ( 1.000000000000000000, 4.299999999999999979E-14, 1.000000000000000078E-15 ) ) ;
#61638=CARTESIAN_POINT ( 'NONE',  ( 102.9084262957273097, -29.13922403623678292, 98.28142370292496821 ) ) ;
#61639=VECTOR ( 'NONE', #9796, 1000.000000000000000 ) ;
#61643=CARTESIAN_POINT ( 'NONE',  ( 182.2300522401149863, -33.89581943344511217, -5.074374724088000832 ) ) ;
#61644=ORIENTED_EDGE ( 'NONE', *, *, #75271, .T. ) ;
#61645=CARTESIAN_POINT ( 'NONE',  ( 77.33253953643573197, -36.38432368373235448, 6.774690158158751530 ) ) ;
#61647=CARTESIAN_POINT ( 'NONE',  ( 103.8073253818723316, -26.82667379764869153, 165.3299109901969643 ) ) ;
#61648=ORIENTED_EDGE ( 'NONE', *, *, #39043, .F. ) ;
#61651=CARTESIAN_POINT ( 'NONE',  ( 116.2543158056996333, -38.69420140005939857, 105.1025356868499614 ) ) ;
#61654=CARTESIAN_POINT ( 'NONE',  ( 107.2325526940309288, -25.65435679020650639, 76.07657765686298035 ) ) ;
#61655=CARTESIAN_POINT ( 'NONE',  ( 48.85858412958099706, -30.08671355700241179, 342.9256252759119548 ) ) ;
#61656=AXIS2_PLACEMENT_3D ( 'NONE', #69131, #6897, #84118 ) ;
#61657=EDGE_LOOP ( 'NONE', ( #60657, #60821 ) ) ;
#61658=CARTESIAN_POINT ( 'NONE',  ( 34.96670390244699433, -28.27351298637401200, 313.9678068554150059 ) ) ;
#61662=EDGE_LOOP ( 'NONE', ( #10187, #4836 ) ) ;
#61663=EDGE_LOOP ( 'NONE', ( #13670, #59081, #26312, #17757 ) ) ;
#61664=EDGE_CURVE ( 'NONE', #75364, #88639, #15393, .T. ) ;
#61665=CIRCLE ( 'NONE', #48554, 1.000000000000000888 ) ;
#61666=CARTESIAN_POINT ( 'NONE',  ( 123.6837132603318707, -20.11243780205705534, 218.0711402470151370 ) ) ;
#61667=VERTEX_POINT ( 'NONE', #43062 ) ;
#61668=EDGE_CURVE ( 'NONE', #74810, #24368, #4028, .T. ) ;
#61669=CARTESIAN_POINT ( 'NONE',  ( 97.63766479707255996, -34.12929003103648284, 251.1127681330543737 ) ) ;
#61670=CARTESIAN_POINT ( 'NONE',  ( 101.7584646134851596, -45.72734648786122591, 158.1527681330539963 ) ) ;
#61671=CARTESIAN_POINT ( 'NONE',  ( 194.5667039024485234, -47.82844715993405060, 180.4678068554150343 ) ) ;
#61672=CARTESIAN_POINT ( 'NONE',  ( 109.7248659254751715, -27.00080518097527360, 140.8647919422406858 ) ) ;
#61673=EDGE_CURVE ( 'NONE', #11339, #16654, #1308, .T. ) ;
#61674=CARTESIAN_POINT ( 'NONE',  ( 113.3146854497373965, -28.34009065521201265, 100.5670538473389684 ) ) ;
#61675=CARTESIAN_POINT ( 'NONE',  ( 144.4532657509292051, -72.54478064608022692, 540.9756252759101471 ) ) ;
#61676=VERTEX_POINT ( 'NONE', #29462 ) ;
#61680=ORIENTED_EDGE ( 'NONE', *, *, #73503, .T. ) ;
#61681=CARTESIAN_POINT ( 'NONE',  ( 20.56670390244828184, -48.82844715994187368, 300.4678068554150059 ) ) ;
#61682=FACE_OUTER_BOUND ( 'NONE', #51392, .T. ) ;
#61683=CARTESIAN_POINT ( 'NONE',  ( 99.41296134609922319, -28.78668791560518514, 265.6746728949588032 ) ) ;
#61685=VECTOR ( 'NONE', #69662, 1000.000000000000000 ) ;
#61688=CARTESIAN_POINT ( 'NONE',  ( 106.3024736416914493, -26.94527301106431949, 25.13848241876892686 ) ) ;
#61689=FACE_OUTER_BOUND ( 'NONE', #37911, .T. ) ;
#61690=CARTESIAN_POINT ( 'NONE',  ( 104.1140010245780729, -46.70499295924809502, 103.3470538473389411 ) ) ;
#61691=DIRECTION ( 'NONE',  ( 0.000000000000000000, 0.000000000000000000, -1.000000000000000000 ) ) ;
#61692=CARTESIAN_POINT ( 'NONE',  ( 97.63486134215516188, -41.27380337981261960, 171.6841967044819626 ) ) ;
#61694=EDGE_CURVE ( 'NONE', #45647, #32225, #27237, .T. ) ;
#61697=FACE_BOUND ( 'NONE', #88297, .T. ) ;
#61698=EDGE_CURVE ( 'NONE', #88639, #52430, #22658, .T. ) ;
#61700=ORIENTED_EDGE ( 'NONE', *, *, #7044, .F. ) ;
#61701=CARTESIAN_POINT ( 'NONE',  ( 97.33808530593822184, -34.07010290169503719, 62.11506100739555336 ) ) ;
#61702=CARTESIAN_POINT ( 'NONE',  ( 117.6255004633147507, -33.30599276614662330, 134.0880062282919880 ) ) ;
#61704=CARTESIAN_POINT ( 'NONE',  ( 41.56648329127499153, -32.07844715994070839, 78.92562527591199739 ) ) ;
#61706=CYLINDRICAL_SURFACE ( 'NONE', #24247, 2.116999999999980009 ) ;
#61707=DIRECTION ( 'NONE',  ( 0.000000000000000000, 0.000000000000000000, 1.000000000000000000 ) ) ;
#61710=VECTOR ( 'NONE', #12912, 1000.000000000000000 ) ;
#61711=ORIENTED_EDGE ( 'NONE', *, *, #49837, .F. ) ;
#61713=ORIENTED_EDGE ( 'NONE', *, *, #45674, .T. ) ;
#61714=DIRECTION ( 'NONE',  ( 0.000000000000000000, 0.000000000000000000, 1.000000000000000000 ) ) ;
#61715=CARTESIAN_POINT ( 'NONE',  ( 102.6489936009959365, -27.69395558276979941, 250.4388294734751241 ) ) ;
#61716=CARTESIAN_POINT ( 'NONE',  ( 104.4081005665769624, -46.45808911502702188, 157.3647919348640869 ) ) ;
#61717=DIRECTION ( 'NONE',  ( -0.7071067811865475727, 0.000000000000000000, -0.7071067811865475727 ) ) ;
#61718=LINE ( 'NONE', #75378, #76144 ) ;
#61721=ORIENTED_EDGE ( 'NONE', *, *, #57276, .F. ) ;
#61722=AXIS2_PLACEMENT_3D ( 'NONE', #81771, #69023, #55801 ) ;
#61724=AXIS2_PLACEMENT_3D ( 'NONE', #17849, #58723, #86466 ) ;
#61725=DIRECTION ( 'NONE',  ( 1.000000000000000000, 0.000000000000000000, 0.000000000000000000 ) ) ;
#61726=AXIS2_PLACEMENT_3D ( 'NONE', #55402, #466, #62236 ) ;
#61727=CARTESIAN_POINT ( 'NONE',  ( 154.4532657509292051, -72.54478064608022692, 396.9756252759102040 ) ) ;
#61729=CARTESIAN_POINT ( 'NONE',  ( 109.1965444620390286, -27.18343884754229833, 220.9013395616249795 ) ) ;
#61732=CARTESIAN_POINT ( 'NONE',  ( 98.13101841594846064, -32.75189731695859763, 96.99276813305296230 ) ) ;
#61733=CARTESIAN_POINT ( 'NONE',  ( 110.8561346566681891, -45.98355671804449685, 52.88576822912357756 ) ) ;
#61734=VECTOR ( 'NONE', #38342, 999.9999999999998863 ) ;
#61735=CARTESIAN_POINT ( 'NONE',  ( 107.8594798993478747, -26.73948001534716923, 21.01336167101059260 ) ) ;
#61737=DIRECTION ( 'NONE',  ( 0.7071067811865449082, 0.7071067811865501263, 7.071067811865448709E-16 ) ) ;
#61738=ORIENTED_EDGE ( 'NONE', *, *, #40853, .T. ) ;
#61739=VERTEX_POINT ( 'NONE', #79414 ) ;
#61742=CARTESIAN_POINT ( 'NONE',  ( 114.4012193684849734, -41.70236635182605056, 269.7844404487540260 ) ) ;
#61743=DIRECTION ( 'NONE',  ( 0.7071067811566161820, 0.7071067812164789634, 0.000000000000000000 ) ) ;
#61745=DIRECTION ( 'NONE',  ( 1.000000000000000078E-15, -1.000000000000000083E-30, -1.000000000000000000 ) ) ;
#61747=CARTESIAN_POINT ( 'NONE',  ( 100.8874677892395084, -44.70022130223561874, 153.0522919331214098 ) ) ;
#61748=CARTESIAN_POINT ( 'NONE',  ( 80.44338158420812590, -39.47944715994105991, 1.625625275910945300 ) ) ;
#61753=CARTESIAN_POINT ( 'NONE',  ( 96.92094985624760284, -32.34227964863599425, 61.01372051400599616 ) ) ;
#61754=ORIENTED_EDGE ( 'NONE', *, *, #40414, .T. ) ;
#61755=CARTESIAN_POINT ( 'NONE',  ( 99.62303294566419254, -42.26939103296757594, 259.6538046553056915 ) ) ;
#61756=EDGE_CURVE ( 'NONE', #20396, #72641, #51220, .T. ) ;
#61757=DIRECTION ( 'NONE',  ( 1.000000000000000078E-15, -1.000000000000000083E-30, -1.000000000000000000 ) ) ;
#61758=CARTESIAN_POINT ( 'NONE',  ( 107.6167445103326230, -46.48501816386551866, 152.6213395616259731 ) ) ;
#61761=DIRECTION ( 'NONE',  ( 0.000000000000000000, 0.000000000000000000, -1.000000000000000000 ) ) ;
#61763=CARTESIAN_POINT ( 'NONE',  ( 107.2499990610067329, -24.83081552997016317, 226.0641967044829812 ) ) ;
#61765=ORIENTED_EDGE ( 'NONE', *, *, #74070, .T. ) ;
#61766=ORIENTED_EDGE ( 'NONE', *, *, #53258, .T. ) ;
#61767=CARTESIAN_POINT ( 'NONE',  ( 99.02072372077822138, -43.42711337151016693, 112.8784824187679732 ) ) ;
#61769=AXIS2_PLACEMENT_3D ( 'NONE', #46121, #59758, #32959 ) ;
#61770=EDGE_CURVE ( 'NONE', #80206, #51938, #65748, .T. ) ;
#61771=ORIENTED_EDGE ( 'NONE', *, *, #43181, .T. ) ;
#61775=DIRECTION ( 'NONE',  ( 0.000000000000000000, 0.000000000000000000, 1.000000000000000000 ) ) ;
#61777=CARTESIAN_POINT ( 'NONE',  ( 19.56670390244824631, -47.82844715994191631, 300.4678068554150059 ) ) ;
#61778=EDGE_CURVE ( 'NONE', #41960, #3590, #67829, .T. ) ;
#61779=CARTESIAN_POINT ( 'NONE',  ( 98.06451646660192978, -38.97900810122609982, 164.3395189410199464 ) ) ;
#61780=CARTESIAN_POINT ( 'NONE',  ( 95.20664489286731680, -37.33482625718801273, 267.3670538473395482 ) ) ;
#61781=CARTESIAN_POINT ( 'NONE',  ( 98.15086846876572224, -41.26139812777571336, 57.70070366797900618 ) ) ;
#61785=DIRECTION ( 'NONE',  ( 0.000000000000000000, 1.000000000000000000, 0.000000000000000000 ) ) ;
#61787=EDGE_LOOP ( 'NONE', ( #38183, #59563, #13521, #79265 ) ) ;
#61788=AXIS2_PLACEMENT_3D ( 'NONE', #39743, #27027, #32038 ) ;
#61789=CIRCLE ( 'NONE', #21163, 0.5000000000000004441 ) ;
#61790=CARTESIAN_POINT ( 'NONE',  ( 34.33598329127499227, -36.32844715994100682, -5.074374724088000832 ) ) ;
#61791=AXIS2_PLACEMENT_3D ( 'NONE', #42747, #28699, #14177 ) ;
#61792=ORIENTED_EDGE ( 'NONE', *, *, #30825, .F. ) ;
#61796=VECTOR ( 'NONE', #55031, 1000.000000000000000 ) ;
#61797=FACE_OUTER_BOUND ( 'NONE', #1655, .T. ) ;
#61798=CARTESIAN_POINT ( 'NONE',  ( 138.8167039024479834, -50.82844715994100682, 84.20080685541500998 ) ) ;
#61799=CARTESIAN_POINT ( 'NONE',  ( 115.3915529780678781, -40.29397869100746021, 212.9390864947429804 ) ) ;
#61800=CARTESIAN_POINT ( 'NONE',  ( 96.29295924727914269, -41.78513476824832651, 61.67562527591097421 ) ) ;
#61801=DIRECTION ( 'NONE',  ( -0.7071067811861110330, -0.7071067811869841124, 0.000000000000000000 ) ) ;
#61803=ORIENTED_EDGE ( 'NONE', *, *, #22841, .F. ) ;
#61804=EDGE_CURVE ( 'NONE', #15299, #5970, #78965, .T. ) ;
#61805=CARTESIAN_POINT ( 'NONE',  ( 184.5664832912729878, 15.62155284005731204, 361.9756252759109998 ) ) ;
#61806=ORIENTED_EDGE ( 'NONE', *, *, #15688, .T. ) ;
#61809=EDGE_LOOP ( 'NONE', ( #32279, #43215, #39522, #51768 ) ) ;
#61810=CARTESIAN_POINT ( 'NONE',  ( 51.34673845256467928, -29.62846900982267329, 117.4678068554150485 ) ) ;
#61813=CARTESIAN_POINT ( 'NONE',  ( 110.8659606129244253, -45.97952899714481845, 132.8866131168813354 ) ) ;
#61814=CIRCLE ( 'NONE', #53096, 2.999999999999929834 ) ;
#61816=VERTEX_POINT ( 'NONE', #52543 ) ;
#61817=CARTESIAN_POINT ( 'NONE',  ( 100.9280588457464489, -46.89575235069233372, 52.14419670448194921 ) ) ;
#61819=DIRECTION ( 'NONE',  ( 1.000000000000000000, 4.163336342344333240E-14, 0.000000000000000000 ) ) ;
#61821=CARTESIAN_POINT ( 'NONE',  ( 62.03715912545639810, -23.42818131006021076, 117.4678068554150485 ) ) ;
#61822=CARTESIAN_POINT ( 'NONE',  ( 131.9692527705846032, -16.94806367531073832, 2.376725340804930031 ) ) ;
#61824=CARTESIAN_POINT ( 'NONE',  ( 97.81262911421374895, -40.51702269960655656, 122.6351715870756323 ) ) ;
#61827=VERTEX_POINT ( 'NONE', #44404 ) ;
#61828=CARTESIAN_POINT ( 'NONE',  ( 107.6042626387647090, -26.26092342527675072, 91.03562527591097364 ) ) ;
#61829=CARTESIAN_POINT ( 'NONE',  ( 98.04156652576716624, -41.04195827621020243, 171.6811716726206498 ) ) ;
#61830=CARTESIAN_POINT ( 'NONE',  ( 143.0664832912740110, -8.729447159940999512, 17.92562527591199739 ) ) ;
#61831=DIRECTION ( 'NONE',  ( -4.237773401492740281E-14, 1.000000000000000000, 0.000000000000000000 ) ) ;
#61832=CARTESIAN_POINT ( 'NONE',  ( 124.0664832912757021, -36.72944715993921960, 14.92562527591098842 ) ) ;
#61833=VERTEX_POINT ( 'NONE', #31229 ) ;
#61834=ADVANCED_FACE ( 'NONE', ( #65319 ), #50788, .F. ) ;
#61835=CARTESIAN_POINT ( 'NONE',  ( 116.9564367646782728, -33.61053620760072391, 125.0575300378159795 ) ) ;
#61837=EDGE_LOOP ( 'NONE', ( #64477, #22429, #48272, #74418, #80619, #85159 ) ) ;
#61838=CARTESIAN_POINT ( 'NONE',  ( 116.5620552962770802, -42.34175257684895399, 279.4137205140061724 ) ) ;
#61839=FACE_OUTER_BOUND ( 'NONE', #76268, .T. ) ;
#61846=CARTESIAN_POINT ( 'NONE',  ( 97.31640351007376921, -35.61153895465465524, 206.2356252759109623 ) ) ;
#61848=ORIENTED_EDGE ( 'NONE', *, *, #82740, .F. ) ;
#61849=VECTOR ( 'NONE', #30053, 1000.000000000000000 ) ;
#61850=CARTESIAN_POINT ( 'NONE',  ( 111.3621671965809270, -45.84085784651199447, 134.3587261630399894 ) ) ;
#61851=VECTOR ( 'NONE', #87088, 1000.000000000000000 ) ;
#61852=DIRECTION ( 'NONE',  ( 0.7071067811864683028, 0.7071067811866268427, 7.071067811864676611E-16 ) ) ;
#61854=EDGE_CURVE ( 'NONE', #82640, #9211, #22921, .T. ) ;
#61855=CARTESIAN_POINT ( 'NONE',  ( 98.36824592180721538, -38.57411413555575308, 27.92444044875497156 ) ) ;
#61856=CARTESIAN_POINT ( 'NONE',  ( 77.31648329127401098, -36.72944715994107412, 3.101481641215480867 ) ) ;
#61857=AXIS2_PLACEMENT_3D ( 'NONE', #81781, #89031, #74052 ) ;
#61858=DIRECTION ( 'NONE',  ( 1.000000000000000000, 1.261617073437676668E-15, 1.261617073437676668E-15 ) ) ;
#61860=LINE ( 'NONE', #53687, #72207 ) ;
#61861=EDGE_CURVE ( 'NONE', #60508, #51043, #18547, .T. ) ;
#61862=CARTESIAN_POINT ( 'NONE',  ( 97.81168895331838087, -40.51742574516882200, 287.6356252759109680 ) ) ;
#61864=LINE ( 'NONE', #56392, #27054 ) ;
#61865=CARTESIAN_POINT ( 'NONE',  ( 113.0874441278155871, -45.97130050132146550, 223.0480062282919675 ) ) ;
#61866=DIRECTION ( 'NONE',  ( 0.000000000000000000, 1.000000000000000000, 0.000000000000000000 ) ) ;
#61869=EDGE_CURVE ( 'NONE', #28057, #16260, #66189, .T. ) ;
#61871=DIRECTION ( 'NONE',  ( 0.000000000000000000, 0.000000000000000000, -1.000000000000000000 ) ) ;
#61872=CARTESIAN_POINT ( 'NONE',  ( 82.45326694837569903, -20.09809895854153794, 7.205238605742597890 ) ) ;
#61873=CARTESIAN_POINT ( 'NONE',  ( 109.7256292845548842, -27.00100760353820206, 184.8651728498700777 ) ) ;
#61876=ADVANCED_FACE ( 'NONE', ( #36728 ), #27884, .T. ) ;
#61877=DIRECTION ( 'NONE',  ( -0.7071067811745735954, -0.7071067811985214391, 0.000000000000000000 ) ) ;
#61880=ORIENTED_EDGE ( 'NONE', *, *, #58090, .F. ) ;
#61881=CARTESIAN_POINT ( 'NONE',  ( 172.5664832912729878, -27.82844715994070484, 318.9256252759120116 ) ) ;
#61883=CARTESIAN_POINT ( 'NONE',  ( 110.6963687344609184, -48.01060035924083280, 207.8241967044819489 ) ) ;
#61884=ORIENTED_EDGE ( 'NONE', *, *, #12387, .T. ) ;
#61885=DIRECTION ( 'NONE',  ( 0.000000000000000000, 0.000000000000000000, 1.000000000000000000 ) ) ;
#61886=EDGE_CURVE ( 'NONE', #63431, #79504, #30245, .T. ) ;
#61887=FACE_OUTER_BOUND ( 'NONE', #88724, .T. ) ;
#61888=CARTESIAN_POINT ( 'NONE',  ( 115.0947728502038672, -42.74698383566514082, 168.3144758113602393 ) ) ;
#61889=EDGE_CURVE ( 'NONE', #28391, #54796, #8463, .T. ) ;
#61890=CARTESIAN_POINT ( 'NONE',  ( 102.8730905416367278, -29.69395531543277400, 83.32237608387698913 ) ) ;
#61891=CARTESIAN_POINT ( 'NONE',  ( 98.07189402449054683, -42.11243585264244160, 157.7556252759109725 ) ) ;
#61892=DIRECTION ( 'NONE',  ( 0.7071067811864907293, 0.7071067811866043051, 7.071067811864901437E-16 ) ) ;
#61894=B_SPLINE_CURVE_WITH_KNOTS ( 'NONE', 3,
 ( #14061, #55809, #69930, #13614, #41298, #35386, #14969, #35840, #49457, #28120, #48547, #7697, #83562, #884, #20439, #21329, #77197, #63555 ),
 .UNSPECIFIED., .F., .F.,
 ( 4, 2, 2, 2, 2, 2, 2, 2, 4 ),
 ( 0.4999999979610092460, 0.5624999982158831457, 0.6249999984707569345, 0.6874999987256307232, 0.7499999989805046230, 0.8124999992353785228, 0.8749999994902523115, 0.9374999997451261002, 1.000000000000000000 ),
 .UNSPECIFIED. ) ;
#61896=CARTESIAN_POINT ( 'NONE',  ( 52.65249034007747042, -48.32844715994062312, 129.9678068554150911 ) ) ;
#61899=VERTEX_POINT ( 'NONE', #11699 ) ;
#61902=ORIENTED_EDGE ( 'NONE', *, *, #77395, .T. ) ;
#61904=CARTESIAN_POINT ( 'NONE',  ( 108.2720842404240926, -28.27352272357859420, 104.3867055423629608 ) ) ;
#61905=CARTESIAN_POINT ( 'NONE',  ( 101.6391055438642894, -45.65636906804281381, 247.1413395616249602 ) ) ;
#61906=EDGE_CURVE ( 'NONE', #2091, #60004, #76489, .T. ) ;
#61907=CARTESIAN_POINT ( 'NONE',  ( 117.9257662994440494, -34.79559216868040039, 198.9546728949589749 ) ) ;
#61909=CARTESIAN_POINT ( 'NONE',  ( 106.2538455105912050, -26.32252419718687619, 21.13848241876792144 ) ) ;
#61912=CARTESIAN_POINT ( 'NONE',  ( 172.5664832912729878, -18.82844715994071194, 195.9256252759120684 ) ) ;
#61914=ORIENTED_EDGE ( 'NONE', *, *, #1637, .T. ) ;
#61917=CARTESIAN_POINT ( 'NONE',  ( 109.6029845306728419, -46.78454271877410520, 92.78514908543594686 ) ) ;
#61918=CARTESIAN_POINT ( 'NONE',  ( 117.3971137516355014, -38.63466851614541753, 88.68133956162493803 ) ) ;
#61919=CARTESIAN_POINT ( 'NONE',  ( 115.7319096639420906, -42.60456859047142331, 273.3527681330537575 ) ) ;
#61920=EDGE_LOOP ( 'NONE', ( #3492, #50259, #49026, #35300 ) ) ;
#61922=CARTESIAN_POINT ( 'NONE',  ( 100.6562259211013384, -44.95110337444964443, 232.0499109901969632 ) ) ;
#61923=DIRECTION ( 'NONE',  ( 0.000000000000000000, 0.000000000000000000, -1.000000000000000000 ) ) ;
#61925=VECTOR ( 'NONE', #331, 1000.000000000000000 ) ;
#61926=CARTESIAN_POINT ( 'NONE',  ( 117.0720608545349819, -35.46383447611707851, 24.92718395960681477 ) ) ;
#61927=FACE_OUTER_BOUND ( 'NONE', #323, .T. ) ;
#61928=CARTESIAN_POINT ( 'NONE',  ( 115.2527165410365484, -37.46115175898625438, 277.6356252759110248 ) ) ;
#61929=CARTESIAN_POINT ( 'NONE',  ( 49.21213752016101495, -29.73316016639650172, -5.074374724088000832 ) ) ;
#61930=CARTESIAN_POINT ( 'NONE',  ( 105.7152282706593098, -46.72382676192142981, 173.4689389589050563 ) ) ;
#61934=CARTESIAN_POINT ( 'NONE',  ( 108.4095557610607159, -26.73403182108062737, 39.96876094489950759 ) ) ;
#61936=CARTESIAN_POINT ( 'NONE',  ( 109.7248659092072103, -27.00080517620619602, 259.8647919435812241 ) ) ;
#61938=LINE ( 'NONE', #89671, #13369 ) ;
#61939=CARTESIAN_POINT ( 'NONE',  ( 118.1050840190196567, -32.34957160481850025, 249.1270538473389706 ) ) ;
#61940=CARTESIAN_POINT ( 'NONE',  ( 97.61704402414061121, -30.99515748980318719, 121.8803871806729546 ) ) ;
#61941=CARTESIAN_POINT ( 'NONE',  ( 104.8319786719434603, -26.46567573359534364, 256.2470538473397710 ) ) ;
#61942=AXIS2_PLACEMENT_3D ( 'NONE', #67451, #61974, #74726 ) ;
#61948=CARTESIAN_POINT ( 'NONE',  ( 51.34673845256598668, -29.62846900982231446, -5.074374724088000832 ) ) ;
#61949=VECTOR ( 'NONE', #49123, 1000.000000000000000 ) ;
#61951=CARTESIAN_POINT ( 'NONE',  ( 75.31670390244798341, -50.82844715994100682, 60.91780685541480267 ) ) ;
#61952=ORIENTED_EDGE ( 'NONE', *, *, #76090, .T. ) ;
#61953=CARTESIAN_POINT ( 'NONE',  ( 116.7432888474544370, -37.52321155953265475, 188.1838483995059619 ) ) ;
#61955=ORIENTED_EDGE ( 'NONE', *, *, #11132, .T. ) ;
#61956=DIRECTION ( 'NONE',  ( -1.000000000000000078E-15, 0.000000000000000000, -1.000000000000000000 ) ) ;
#61957=CARTESIAN_POINT ( 'NONE',  ( 117.2701380961605651, -34.52720868313124924, 179.9956252759109532 ) ) ;
#61958=CARTESIAN_POINT ( 'NONE',  ( 48.16670390244701139, -28.27351298637280408, -5.074374724088000832 ) ) ;
#61959=CARTESIAN_POINT ( 'NONE',  ( 142.8821648370248170, -72.54478064608022692, 396.9756252759102040 ) ) ;
#61961=DIRECTION ( 'NONE',  ( -4.012088370409549976E-14, 1.000000000000000000, 0.000000000000000000 ) ) ;
#61962=CARTESIAN_POINT ( 'NONE',  ( 104.3903674582245742, -25.93822912171379969, 90.26991099019693365 ) ) ;
#61963=ORIENTED_EDGE ( 'NONE', *, *, #28511, .T. ) ;
#61965=VECTOR ( 'NONE', #25191, 1000.000000000000000 ) ;
#61968=CARTESIAN_POINT ( 'NONE',  ( 116.1939227058877719, -40.33550099034467706, 189.5270538473389479 ) ) ;
#61970=FACE_BOUND ( 'NONE', #46177, .T. ) ;
#61971=EDGE_CURVE ( 'NONE', #86897, #73831, #28737, .T. ) ;
#61973=EDGE_CURVE ( 'NONE', #56977, #78258, #5536, .T. ) ;
#61974=DIRECTION ( 'NONE',  ( -0.000000000000000000, -0.000000000000000000, 1.000000000000000000 ) ) ;
#61976=DIRECTION ( 'NONE',  ( -1.000000000000000000, -4.554376769437570034E-14, 0.000000000000000000 ) ) ;
#61978=CARTESIAN_POINT ( 'NONE',  ( 117.4257108620838181, -37.68603989742254612, 78.75276813305399060 ) ) ;
#61979=ORIENTED_EDGE ( 'NONE', *, *, #71881, .T. ) ;
#61981=ORIENTED_EDGE ( 'NONE', *, *, #59934, .F. ) ;
#61982=EDGE_CURVE ( 'NONE', #71592, #82044, #62847, .T. ) ;
#61983=CARTESIAN_POINT ( 'NONE',  ( 63.06670390244799052, -40.32844715994017548, 249.9678068554150343 ) ) ;
#61985=AXIS2_PLACEMENT_3D ( 'NONE', #52051, #67050, #65703 ) ;
#61986=PLANE ( 'NONE',  #19255 ) ;
#61987=CARTESIAN_POINT ( 'NONE',  ( 103.8567473457716375, -28.69212669812176841, 173.2090427505439720 ) ) ;
#61989=VECTOR ( 'NONE', #35020, 1000.000000000000000 ) ;
#61995=ORIENTED_EDGE ( 'NONE', *, *, #51724, .T. ) ;
#61996=VERTEX_POINT ( 'NONE', #83765 ) ;
#61998=CARTESIAN_POINT ( 'NONE',  ( 136.3243469132239909, -20.30306751043745450, 2.518077574358949189 ) ) ;
#62000=ORIENTED_EDGE ( 'NONE', *, *, #67452, .T. ) ;
#62003=CARTESIAN_POINT ( 'NONE',  ( 101.7809741706781921, -43.87965855000975068, 253.5015833058971850 ) ) ;
#62004=VERTEX_POINT ( 'NONE', #66647 ) ;
#62005=CIRCLE ( 'NONE', #75110, 2.750000000000002665 ) ;
#62007=CARTESIAN_POINT ( 'NONE',  ( 97.81168843500762478, -40.51741166756562507, 12.63579318495451176 ) ) ;
#62008=EDGE_CURVE ( 'NONE', #79518, #52915, #4436, .T. ) ;
#62010=ORIENTED_EDGE ( 'NONE', *, *, #26769, .T. ) ;
#62011=VERTEX_POINT ( 'NONE', #80742 ) ;
#62012=AXIS2_PLACEMENT_3D ( 'NONE', #24891, #77742, #84569 ) ;
#62015=VERTEX_POINT ( 'NONE', #13815 ) ;
#62016=CARTESIAN_POINT ( 'NONE',  ( 98.80728567624888115, -32.50078473314371763, 243.7680903695909649 ) ) ;
#62017=CARTESIAN_POINT ( 'NONE',  ( 102.3831517106511484, -26.69142711411281255, 135.4118157521009493 ) ) ;
#62018=CARTESIAN_POINT ( 'NONE',  ( 113.3292761056179359, -27.64973082387871628, 89.60800622829195561 ) ) ;
#62019=CARTESIAN_POINT ( 'NONE',  ( 110.6845584771929794, -28.26525459981584376, 249.5838068554170093 ) ) ;
#62020=CARTESIAN_POINT ( 'NONE',  ( 172.5667039024478129, -36.32844715993500273, 300.4678068554149490 ) ) ;
#62021=CARTESIAN_POINT ( 'NONE',  ( 117.0682170987564774, -39.67016276869777869, 179.5984824187679294 ) ) ;
#62022=CARTESIAN_POINT ( 'NONE',  ( 62.03742497533751532, -23.42844715994046467, 237.4678068554150059 ) ) ;
#62023=CARTESIAN_POINT ( 'NONE',  ( 97.81168569434709070, -40.51740311210409828, 127.6359003399277441 ) ) ;
#62030=ADVANCED_FACE ( 'NONE', ( #73917 ), #22430, .T. ) ;
#62031=VERTEX_POINT ( 'NONE', #76940 ) ;
#62034=CARTESIAN_POINT ( 'NONE',  ( 117.1637410210353210, -34.13475704353096063, 124.0270538473399426 ) ) ;
#62036=DIRECTION ( 'NONE',  ( -2.981567257902526681E-15, 0.8571673007021100021, 0.5150380749100580413 ) ) ;
#62037=DIRECTION ( 'NONE',  ( 4.299999999999999979E-14, -1.000000000000000000, 0.000000000000000000 ) ) ;
#62038=CARTESIAN_POINT ( 'NONE',  ( 99.04406185041210620, -42.84125762927686765, 142.8439586081852894 ) ) ;
#62040=CARTESIAN_POINT ( 'NONE',  ( 100.7633749303631561, -45.78122309449478422, 233.0803871806729717 ) ) ;
#62041=CARTESIAN_POINT ( 'NONE',  ( 163.2569089553700223, -33.54226604285010893, -5.074374724088000832 ) ) ;
#62042=CARTESIAN_POINT ( 'NONE',  ( 31.56670390244774893, -33.35206098992784263, 117.4678068554150485 ) ) ;
#62046=CARTESIAN_POINT ( 'NONE',  ( 31.78666935232887880, -36.02818131005931690, 193.9678068554150911 ) ) ;
#62047=CARTESIAN_POINT ( 'NONE',  ( 45.76696975232907505, -48.62818131006087441, 249.9678068554150343 ) ) ;
#62049=CARTESIAN_POINT ( 'NONE',  ( 116.2574608483823226, -41.81646255891691766, 263.4241967044824833 ) ) ;
#62051=CARTESIAN_POINT ( 'NONE',  ( 116.3232968930447839, -32.93863405887816498, 194.1356252759109680 ) ) ;
#62052=CARTESIAN_POINT ( 'NONE',  ( 114.7236970816665860, -44.73335358772728654, 113.1718157521009687 ) ) ;
#62053=CARTESIAN_POINT ( 'NONE',  ( 116.7448692891101985, -32.85500114480387168, 50.12991099019698282 ) ) ;
#62054=CARTESIAN_POINT ( 'NONE',  ( 102.9499971297430250, -26.42158413985995580, 171.3908633711489813 ) ) ;
#62055=AXIS2_PLACEMENT_3D ( 'NONE', #63156, #7308, #27739 ) ;
#62056=CARTESIAN_POINT ( 'NONE',  ( 107.0664832912739968, -36.72944715994100306, 287.6356252759109680 ) ) ;
#62057=CARTESIAN_POINT ( 'NONE',  ( 163.2569089553706760, -33.54226604284440327, 313.9678068554149490 ) ) ;
#62058=DIRECTION ( 'NONE',  ( 0.000000000000000000, 0.000000000000000000, 1.000000000000000000 ) ) ;
#62059=DIRECTION ( 'NONE',  ( 0.000000000000000000, -1.000000000000000000, 0.000000000000000000 ) ) ;
#62060=CARTESIAN_POINT ( 'NONE',  ( 50.87649884952473656, -33.54226604284966839, 237.4678068554150059 ) ) ;
#62061=DIRECTION ( 'NONE',  ( 0.000000000000000000, 0.000000000000000000, 1.000000000000000000 ) ) ;
#62062=ORIENTED_EDGE ( 'NONE', *, *, #29298, .F. ) ;
#62063=EDGE_CURVE ( 'NONE', #64817, #47280, #22884, .T. ) ;
#62066=VERTEX_POINT ( 'NONE', #77385 ) ;
#62067=ORIENTED_EDGE ( 'NONE', *, *, #20194, .T. ) ;
#62071=CARTESIAN_POINT ( 'NONE',  ( 115.1902516771092451, -44.19056033372781656, 74.22324432352993995 ) ) ;
#62074=CARTESIAN_POINT ( 'NONE',  ( 164.7830935719630361, -29.99615139349950965, 117.4678068554150485 ) ) ;
#62075=CARTESIAN_POINT ( 'NONE',  ( 108.8562982717690062, -47.04397778784520057, 163.7127681330539701 ) ) ;
#62076=AXIS2_PLACEMENT_3D ( 'NONE', #30826, #85816, #43543 ) ;
#62079=CARTESIAN_POINT ( 'NONE',  ( 106.0094748626272434, -28.25366608065910157, 269.5981341137911613 ) ) ;
#62081=ORIENTED_EDGE ( 'NONE', *, *, #65032, .T. ) ;
#62083=AXIS2_PLACEMENT_3D ( 'NONE', #2117, #50696, #21215 ) ;
#62084=DIRECTION ( 'NONE',  ( 0.000000000000000000, 1.000000000000000000, 0.000000000000000000 ) ) ;
#62085=CARTESIAN_POINT ( 'NONE',  ( 113.6646628792758094, -44.27214913190846346, 183.1483198295319426 ) ) ;
#62086=CARTESIAN_POINT ( 'NONE',  ( 97.31584371959736757, -39.30597601310159916, 76.53145861037360476 ) ) ;
#62087=CARTESIAN_POINT ( 'NONE',  ( 109.7212149768214147, -26.99983785526572788, 274.8646644956127147 ) ) ;
#62088=EDGE_CURVE ( 'NONE', #31310, #79375, #21480, .T. ) ;
#62090=EDGE_CURVE ( 'NONE', #44014, #5447, #36939, .T. ) ;
#62093=DIRECTION ( 'NONE',  ( 1.000000000000000078E-15, 0.000000000000000000, -1.000000000000000000 ) ) ;
#62094=CARTESIAN_POINT ( 'NONE',  ( 116.8464009251322153, -35.91275531464980020, 253.8927681330545454 ) ) ;
#62099=AXIS2_PLACEMENT_3D ( 'NONE', #55943, #50029, #1009 ) ;
#62100=CARTESIAN_POINT ( 'NONE',  ( 25.56670390244828894, -48.82844715994168183, 293.2178068554150059 ) ) ;
#62101=CARTESIAN_POINT ( 'NONE',  ( 114.4788834064733862, -33.31096057238692509, 101.9880903695909780 ) ) ;
#62102=VECTOR ( 'NONE', #73813, 1000.000000000000000 ) ;
#62104=CARTESIAN_POINT ( 'NONE',  ( 193.0374249753375011, -23.42844715993432558, 249.9678068554149775 ) ) ;
#62106=DIRECTION ( 'NONE',  ( 4.299999999999999979E-14, -1.000000000000000000, 0.000000000000000000 ) ) ;
#62107=ORIENTED_EDGE ( 'NONE', *, *, #35583, .F. ) ;
#62108=DIRECTION ( 'NONE',  ( 0.9068632946707807507, -0.4214249218767881500, 9.028300618466658994E-16 ) ) ;
#62110=CARTESIAN_POINT ( 'NONE',  ( 108.5898285964631640, -47.07861824576353627, 142.6927681330539883 ) ) ;
#62113=CARTESIAN_POINT ( 'NONE',  ( 115.1135551441502258, -33.01825958633261848, 100.6015833058969378 ) ) ;
#62116=CARTESIAN_POINT ( 'NONE',  ( 104.7547631156620014, -46.91734236372032996, 68.39848241876794077 ) ) ;
#62119=ORIENTED_EDGE ( 'NONE', *, *, #55239, .F. ) ;
#62123=VERTEX_POINT ( 'NONE', #42394 ) ;
#62126=ORIENTED_EDGE ( 'NONE', *, *, #12968, .T. ) ;
#62127=CARTESIAN_POINT ( 'NONE',  ( 105.8561066403587176, -27.02385992090109568, 270.1756252759109884 ) ) ;
#62128=CARTESIAN_POINT ( 'NONE',  ( 116.8268856436350518, -43.49382415615948361, 159.3441967044829539 ) ) ;
#62131=CARTESIAN_POINT ( 'NONE',  ( 104.2140748950419464, -25.22734379144252870, 86.26991099019699050 ) ) ;
#62134=AXIS2_PLACEMENT_3D ( 'NONE', #38846, #4343, #32029 ) ;
#62135=CARTESIAN_POINT ( 'NONE',  ( 135.0664832912729878, -36.72944715994189835, 342.9256252759109884 ) ) ;
#62136=CIRCLE ( 'NONE', #15740, 2.117000000000007987 ) ;
#62139=EDGE_CURVE ( 'NONE', #40280, #6819, #43241, .T. ) ;
#62140=VERTEX_POINT ( 'NONE', #1980 ) ;
#62141=LINE ( 'NONE', #81717, #48963 ) ;
#62142=CYLINDRICAL_SURFACE ( 'NONE', #47831, 2.116999999999993776 ) ;
#62143=CARTESIAN_POINT ( 'NONE',  ( 96.93559702949573875, -34.21358363697170546, 276.1327681330537871 ) ) ;
#62144=CARTESIAN_POINT ( 'NONE',  ( 162.5667039024470171, -33.35206098992711077, -5.074374724088000832 ) ) ;
#62146=DIRECTION ( 'NONE',  ( 0.000000000000000000, 0.000000000000000000, -1.000000000000000000 ) ) ;
#62147=CARTESIAN_POINT ( 'NONE',  ( 116.3037889147421424, -33.73884459347697629, 283.4981341137910249 ) ) ;
#62148=DIRECTION ( 'NONE',  ( -1.000000000000000078E-15, 1.000000000000000000, 0.000000000000000000 ) ) ;
#62149=CARTESIAN_POINT ( 'NONE',  ( 99.70004787478436015, -45.98060041612298221, 118.0413395616259606 ) ) ;
#62150=LINE ( 'NONE', #40364, #62527 ) ;
#62151=CARTESIAN_POINT ( 'NONE',  ( 97.75494523667518365, -42.77206137223026161, 146.7965776568629508 ) ) ;
#62153=ORIENTED_EDGE ( 'NONE', *, *, #78631, .F. ) ;
#62154=AXIS2_PLACEMENT_3D ( 'NONE', #23519, #3057, #10743 ) ;
#62156=FACE_BOUND ( 'NONE', #54170, .T. ) ;
#62159=CARTESIAN_POINT ( 'NONE',  ( 114.1106629025095458, -44.52247787522302502, 133.1613395616249989 ) ) ;
#62160=ORIENTED_EDGE ( 'NONE', *, *, #52011, .F. ) ;
#62162=CARTESIAN_POINT ( 'NONE',  ( 117.4343095520634108, -35.18433407802718449, 214.9441967044829767 ) ) ;
#62164=VECTOR ( 'NONE', #446, 1000.000000000000000 ) ;
#62165=LINE ( 'NONE', #14931, #28577 ) ;
#62166=AXIS2_PLACEMENT_3D ( 'NONE', #29143, #59395, #52561 ) ;
#62168=ORIENTED_EDGE ( 'NONE', *, *, #31943, .F. ) ;
#62169=ADVANCED_FACE ( 'NONE', ( #1540 ), #29679, .T. ) ;
#62170=EDGE_LOOP ( 'NONE', ( #75643, #70297, #87163 ) ) ;
#62171=ORIENTED_EDGE ( 'NONE', *, *, #43130, .T. ) ;
#62172=VERTEX_POINT ( 'NONE', #42839 ) ;
#62173=DIRECTION ( 'NONE',  ( 0.000000000000000000, 1.000000000000000000, 0.000000000000000000 ) ) ;
#62174=CARTESIAN_POINT ( 'NONE',  ( 109.3368649739139187, -26.55458330520283994, 220.9013395616249795 ) ) ;
#62175=CARTESIAN_POINT ( 'NONE',  ( 49.21213752015854936, -29.73316016639470050, 237.4678068554150059 ) ) ;
#62181=ORIENTED_EDGE ( 'NONE', *, *, #54280, .F. ) ;
#62183=AXIS2_PLACEMENT_3D ( 'NONE', #6050, #33738, #53248 ) ;
#62185=DIRECTION ( 'NONE',  ( 0.7071067811865273667, -0.7071067811865676678, 7.071067811865281076E-16 ) ) ;
#62186=DIRECTION ( 'NONE',  ( 0.000000000000000000, 0.000000000000000000, 1.000000000000000000 ) ) ;
#62187=CARTESIAN_POINT ( 'NONE',  ( 96.02263050233435138, -38.01213896886783061, 232.4184824187679794 ) ) ;
#62188=EDGE_CURVE ( 'NONE', #7620, #8519, #2682, .T. ) ;
#62189=CARTESIAN_POINT ( 'NONE',  ( 94.58945128933383728, -41.88441296220994303, 293.1356252759106837 ) ) ;
#62190=VECTOR ( 'NONE', #74631, 1000.000000000000000 ) ;
#62191=CARTESIAN_POINT ( 'NONE',  ( 97.83387747045378546, -32.00739517038279303, 91.96229194257693962 ) ) ;
#62192=EDGE_CURVE ( 'NONE', #24090, #67994, #22998, .T. ) ;
#62196=CARTESIAN_POINT ( 'NONE',  ( 104.9990148946446737, -26.93299307437888146, 21.24201732517684960 ) ) ;
#62197=EDGE_LOOP ( 'NONE', ( #26175, #69890, #55964, #17560, #26068, #21829 ) ) ;
#62198=FACE_OUTER_BOUND ( 'NONE', #27656, .T. ) ;
#62199=ADVANCED_FACE ( 'NONE', ( #56927, #30129 ), #57826, .F. ) ;
#62200=VECTOR ( 'NONE', #61157, 1000.000000000000000 ) ;
#62202=ORIENTED_EDGE ( 'NONE', *, *, #43405, .F. ) ;
#62203=DIRECTION ( 'NONE',  ( 1.000000000000000000, 6.831565154159360295E-14, 0.000000000000000000 ) ) ;
#62204=CARTESIAN_POINT ( 'NONE',  ( 98.49168440212470443, -38.96576165349271292, 272.9615833058970225 ) ) ;
#62208=EDGE_CURVE ( 'NONE', #2919, #89295, #85369, .T. ) ;
#62209=VECTOR ( 'NONE', #37687, 1000.000000000000000 ) ;
#62211=ORIENTED_EDGE ( 'NONE', *, *, #24471, .F. ) ;
#62212=DIRECTION ( 'NONE',  ( 0.000000000000000000, 0.000000000000000000, -1.000000000000000000 ) ) ;
#62213=DIRECTION ( 'NONE',  ( 1.000000000000000078E-15, -1.000000000000000083E-30, -1.000000000000000000 ) ) ;
#62215=CARTESIAN_POINT ( 'NONE',  ( 117.0917326185583676, -32.07397045188266560, 59.16038718067295576 ) ) ;
#62217=CARTESIAN_POINT ( 'NONE',  ( 108.7463670854851756, -45.85490172528324138, 275.5395189410199919 ) ) ;
#62219=CARTESIAN_POINT ( 'NONE',  ( 116.1942131220466621, -33.21547736372279758, 139.1184824187689628 ) ) ;
#62221=CARTESIAN_POINT ( 'NONE',  ( 194.0667039024473297, -24.92844715993408045, 300.4678068554149490 ) ) ;
#62222=DIRECTION ( 'NONE',  ( 1.000000000000000000, 4.299999999999999979E-14, 1.000000000000000078E-15 ) ) ;
#62225=CARTESIAN_POINT ( 'NONE',  ( 104.3129624051631907, -25.97697669550431243, 241.2880062282919482 ) ) ;
#62227=ORIENTED_EDGE ( 'NONE', *, *, #12588, .F. ) ;
#62228=LINE ( 'NONE', #63127, #2361 ) ;
#62229=ORIENTED_EDGE ( 'NONE', *, *, #44757, .F. ) ;
#62230=CARTESIAN_POINT ( 'NONE',  ( 117.2645927648968183, -42.86211997589052203, 124.3956252759109731 ) ) ;
#62232=VERTEX_POINT ( 'NONE', #38272 ) ;
#62235=DIRECTION ( 'NONE',  ( 0.000000000000000000, 1.000000000000000000, 0.000000000000000000 ) ) ;
#62236=DIRECTION ( 'NONE',  ( 1.000000000000000000, -1.526556658859588981E-13, 0.000000000000000000 ) ) ;
#62239=CARTESIAN_POINT ( 'NONE',  ( 112.1932604131138760, -43.70204218538222563, 180.8871379886389832 ) ) ;
#62240=CARTESIAN_POINT ( 'NONE',  ( 96.24544184373708333, -34.36507245719054282, 252.1432443235302969 ) ) ;
#62241=CARTESIAN_POINT ( 'NONE',  ( 97.81547641113768066, -40.52666954525783183, 57.63642061862653065 ) ) ;
#62245=CARTESIAN_POINT ( 'NONE',  ( 121.3042370176062548, -43.34581843340460239, 0.4256252759109851458 ) ) ;
#62246=ADVANCED_FACE ( 'NONE', ( #45955 ), #45072, .F. ) ;
#62247=ORIENTED_EDGE ( 'NONE', *, *, #16394, .T. ) ;
#62248=ORIENTED_EDGE ( 'NONE', *, *, #10316, .F. ) ;
#62250=AXIS2_PLACEMENT_3D ( 'NONE', #42654, #84493, #10719 ) ;
#62251=CARTESIAN_POINT ( 'NONE',  ( 150.8164832912740110, -8.729447159940999512, -5.074374724088000832 ) ) ;
#62253=DIRECTION ( 'NONE',  ( 0.000000000000000000, 0.000000000000000000, 1.000000000000000000 ) ) ;
#62254=ADVANCED_FACE ( 'NONE', ( #3319 ), #59589, .F. ) ;
#62255=DIRECTION ( 'NONE',  ( 1.000000000000000000, -3.418174336900117128E-15, 0.000000000000000000 ) ) ;
#62256=CARTESIAN_POINT ( 'NONE',  ( 112.4311324297980406, -44.02555639339375659, 182.4914674471249612 ) ) ;
#62257=CARTESIAN_POINT ( 'NONE',  ( 110.8102856614596021, -46.50649220725635757, 62.86705384733992474 ) ) ;
#62258=DIRECTION ( 'NONE',  ( 0.000000000000000000, 1.000000000000000000, 0.000000000000000000 ) ) ;
#62259=EDGE_LOOP ( 'NONE', ( #8050, #87709, #48947, #45290, #62781 ) ) ;
#62261=AXIS2_PLACEMENT_3D ( 'NONE', #49858, #1740, #80161 ) ;
#62264=CARTESIAN_POINT ( 'NONE',  ( 142.8679068202682458, 10.65431904611001634, 540.9756252759101471 ) ) ;
#62266=DIRECTION ( 'NONE',  ( -1.000000000000000078E-15, -1.000000000000000083E-30, 1.000000000000000000 ) ) ;
#62269=LINE ( 'NONE', #34561, #22922 ) ;
#62271=VERTEX_POINT ( 'NONE', #80518 ) ;
#62273=CARTESIAN_POINT ( 'NONE',  ( 116.4074703635738075, -31.97189281592868682, 44.20133956162491984 ) ) ;
#62274=CARTESIAN_POINT ( 'NONE',  ( 165.2725846195389749, -35.55794170701241086, 193.9678068554149775 ) ) ;
#62275=DIRECTION ( 'NONE',  ( 0.000000000000000000, 0.000000000000000000, -1.000000000000000000 ) ) ;
#62276=DIRECTION ( 'NONE',  ( 0.000000000000000000, 1.000000000000000000, 0.000000000000000000 ) ) ;
#62277=AXIS2_PLACEMENT_3D ( 'NONE', #61461, #66491, #40581 ) ;
#62278=FACE_OUTER_BOUND ( 'NONE', #62963, .T. ) ;
#62283=DIRECTION ( 'NONE',  ( -1.000000000000000078E-15, 1.000000000000000083E-30, 1.000000000000000000 ) ) ;
#62285=VERTEX_POINT ( 'NONE', #52311 ) ;
#62286=CARTESIAN_POINT ( 'NONE',  ( 113.5195425369480233, -28.51389573442233427, 75.54705384733995288 ) ) ;
#62287=DIRECTION ( 'NONE',  ( 0.000000000000000000, 0.000000000000000000, 1.000000000000000000 ) ) ;
#62290=VECTOR ( 'NONE', #36077, 1000.000000000000000 ) ;
#62293=CARTESIAN_POINT ( 'NONE',  ( 105.0928733274061813, -25.78792777683075599, 121.2184824187669818 ) ) ;
#62294=CARTESIAN_POINT ( 'NONE',  ( 182.4202572930400095, -33.70561438051981185, 342.9256252759119548 ) ) ;
#62295=EDGE_LOOP ( 'NONE', ( #80582, #81804, #24162, #69135 ) ) ;
#62297=CARTESIAN_POINT ( 'NONE',  ( 115.9412561796927577, -30.17946786548973748, 255.3203871806729524 ) ) ;
#62298=LINE ( 'NONE', #20979, #17919 ) ;
#62303=AXIS2_PLACEMENT_3D ( 'NONE', #38156, #16829, #50435 ) ;
#62306=CARTESIAN_POINT ( 'NONE',  ( 96.73459541816642115, -35.84013382243347223, 186.2461014663879837 ) ) ;
#62307=EDGE_LOOP ( 'NONE', ( #33143, #7331, #21771, #22260, #61611, #8310 ) ) ;
#62309=AXIS2_PLACEMENT_3D ( 'NONE', #9432, #23087, #28985 ) ;
#62310=CARTESIAN_POINT ( 'NONE',  ( 107.7905181614329564, -45.59160847044328335, 174.0730118773249728 ) ) ;
#62311=AXIS2_PLACEMENT_3D ( 'NONE', #26043, #59643, #67357 ) ;
#62313=CARTESIAN_POINT ( 'NONE',  ( 111.4826097991074079, -46.11499196468592743, 283.9146728949579597 ) ) ;
#62314=CARTESIAN_POINT ( 'NONE',  ( 97.81027290652480133, -40.51396607169345288, 57.63532815071263116 ) ) ;
#62316=DIRECTION ( 'NONE',  ( 0.000000000000000000, 0.000000000000000000, -1.000000000000000000 ) ) ;
#62318=AXIS2_PLACEMENT_3D ( 'NONE', #35645, #44237, #57431 ) ;
#62320=FACE_OUTER_BOUND ( 'NONE', #60567, .T. ) ;
#62322=EDGE_CURVE ( 'NONE', #6493, #66368, #24398, .T. ) ;
#62324=CARTESIAN_POINT ( 'NONE',  ( 109.9541224118590890, -48.19721710984623542, 242.7727681330539724 ) ) ;
#62325=CARTESIAN_POINT ( 'NONE',  ( 97.75867135665099283, -40.38561536396691309, 171.6245721619694109 ) ) ;
#62326=ORIENTED_EDGE ( 'NONE', *, *, #10511, .T. ) ;
#62327=ORIENTED_EDGE ( 'NONE', *, *, #11756, .F. ) ;
#62328=CARTESIAN_POINT ( 'NONE',  ( 116.3191775144681515, -32.94222376661483764, 89.13562527591095375 ) ) ;
#62330=AXIS2_PLACEMENT_3D ( 'NONE', #14333, #41114, #82491 ) ;
#62331=CARTESIAN_POINT ( 'NONE',  ( 97.81916166726549022, -40.53564570812252299, 122.6367379950636405 ) ) ;
#62332=DIRECTION ( 'NONE',  ( -1.000000000000000000, -5.512527431108013646E-15, 0.000000000000000000 ) ) ;
#62333=DIRECTION ( 'NONE',  ( -7.723290606088049820E-15, 0.000000000000000000, -1.000000000000000000 ) ) ;
#62335=CARTESIAN_POINT ( 'NONE',  ( 118.6189051447874903, -33.88680481589229743, 10.01848241876795953 ) ) ;
#62337=B_SPLINE_CURVE_WITH_KNOTS ( 'NONE', 3,
 ( #61824, #41379, #60476, #82308, #75480, #82760, #89557, #88223, #6873, #25980, #53649, #14601, #28201, #57710, #36387, #15044, #70007, #15501, #84095, #22767, #20955, #42717, #2318, #48632 ),
 .UNSPECIFIED., .F., .F.,
 ( 4, 2, 2, 2, 2, 2, 2, 2, 2, 2, 2, 4 ),
 ( 0.5000920265313297808, 0.5625805232149136970, 0.6250690198984975021, 0.6875575165820814183, 0.7500460132656651124, 0.8125345099492488066, 0.8437787582910407647, 0.8750230066328326117, 0.9062672549746244588, 0.9375115033164163059, 0.9687557516582081529, 1.000000000000000000 ),
 .UNSPECIFIED. ) ;
#62338=CARTESIAN_POINT ( 'NONE',  ( 98.83914287153486100, -29.34771585412822859, 235.7565776568629872 ) ) ;
#62339=EDGE_LOOP ( 'NONE', ( #35480, #60360, #77793, #66325 ) ) ;
#62340=VECTOR ( 'NONE', #62036, 1000.000000000000000 ) ;
#62341=B_SPLINE_CURVE_WITH_KNOTS ( 'NONE', 3,
 ( #27359, #48229, #26469, #20560, #19210, #75964, #54139, #13734, #41419, #60069, #87801, #25567, #41860, #70497, #21455, #48675, #36430, #77309, #35058, #8269, #22805, #42757, #62325, #6916, #15538, #56394, #83238, #29158 ),
 .UNSPECIFIED., .F., .F.,
 ( 4, 2, 2, 2, 2, 2, 2, 2, 2, 2, 1, 1, 1, 1, 2, 4 ),
 ( 0.000000000000000000, 0.06250757335814957627, 0.1250151467162991525, 0.1875227200744487288, 0.2500302934325983051, 0.3125378667907478536, 0.3750454401488974576, 0.4375530135070470061, 0.4688068001861218081, 0.4844336935256593479, 0.4922471401954281456, 0.4961538635303126554, 0.4981072251977549104, 0.4990839060314760101, 0.4995722464483365877, 0.5000605868651970543 ),
 .UNSPECIFIED. ) ;
#62343=DIRECTION ( 'NONE',  ( -1.639958061481212836E-42, 4.100000000000000342E-29, 1.000000000000000000 ) ) ;
#62344=CARTESIAN_POINT ( 'NONE',  ( 110.9050858514773807, -45.96338816205167177, 167.8899810469827685 ) ) ;
#62345=CARTESIAN_POINT ( 'NONE',  ( 109.7208934110032743, -44.96686374295461519, 55.65475703625794068 ) ) ;
#62346=CARTESIAN_POINT ( 'NONE',  ( 105.7176149122623485, -24.93101994221251516, 156.1670538473399574 ) ) ;
#62347=DIRECTION ( 'NONE',  ( -1.000000000000000078E-15, 1.000000000000000083E-30, 1.000000000000000000 ) ) ;
#62352=ORIENTED_EDGE ( 'NONE', *, *, #66765, .T. ) ;
#62355=ORIENTED_EDGE ( 'NONE', *, *, #61971, .F. ) ;
#62356=FACE_OUTER_BOUND ( 'NONE', #82446, .T. ) ;
#62357=CARTESIAN_POINT ( 'NONE',  ( 98.52552435659306695, -36.63915763587115038, 110.7409912566489680 ) ) ;
#62358=CARTESIAN_POINT ( 'NONE',  ( 115.2691655829841579, -30.20224515277380917, 244.3613395616249875 ) ) ;
#62360=CARTESIAN_POINT ( 'NONE',  ( 103.8265608274144256, -48.10271009292828381, 217.3556252759109668 ) ) ;
#62361=CARTESIAN_POINT ( 'NONE',  ( 118.0600790064083299, -37.62648441163795354, 34.77372051400695341 ) ) ;
#62362=CARTESIAN_POINT ( 'NONE',  ( 165.9667039024459996, -26.71338133339301635, -5.074374724088000832 ) ) ;
#62363=CARTESIAN_POINT ( 'NONE',  ( 99.04382173825221969, -42.84089691445041126, 92.84392477103513386 ) ) ;
#62364=CIRCLE ( 'NONE', #10120, 2.030000000000003801 ) ;
#62367=VECTOR ( 'NONE', #50976, 1000.000000000000000 ) ;
#62368=CARTESIAN_POINT ( 'NONE',  ( 103.4152017835535844, -27.65577212482025971, 130.3813395616259925 ) ) ;
#62369=CARTESIAN_POINT ( 'NONE',  ( 116.1621043582934902, -29.05491297703968101, 74.38419670448293175 ) ) ;
#62370=CARTESIAN_POINT ( 'NONE',  ( 99.50747941120199869, -29.43470559729854230, 250.7156252759109520 ) ) ;
#62373=CARTESIAN_POINT ( 'NONE',  ( 111.1275225509982505, -27.12762490620188771, 244.7584824187679544 ) ) ;
#62374=DIRECTION ( 'NONE',  ( 0.0001713722456127401463, -0.9999999853157766072, -1.713722456137401502E-19 ) ) ;
#62375=CARTESIAN_POINT ( 'NONE',  ( 98.04137945595525139, -41.04156525728014770, 22.68116640241568405 ) ) ;
#62377=CARTESIAN_POINT ( 'NONE',  ( 107.9149127458704243, -46.51730135063228744, 277.6356252759110248 ) ) ;
#62378=PLANE ( 'NONE',  #70322 ) ;
#62383=EDGE_CURVE ( 'NONE', #16304, #64817, #72801, .T. ) ;
#62384=DIRECTION ( 'NONE',  ( 1.000000000000000000, 0.000000000000000000, 9.462128050782575008E-16 ) ) ;
#62386=EDGE_CURVE ( 'NONE', #37616, #39094, #64441, .T. ) ;
#62387=FACE_OUTER_BOUND ( 'NONE', #71752, .T. ) ;
#62388=CARTESIAN_POINT ( 'NONE',  ( 107.0664832912739968, -18.82844715994099971, 333.4006252759120343 ) ) ;
#62389=ORIENTED_EDGE ( 'NONE', *, *, #29172, .F. ) ;
#62390=ADVANCED_FACE ( 'NONE', ( #24212 ), #43308, .F. ) ;
#62392=CARTESIAN_POINT ( 'NONE',  ( 96.78703652860848194, -40.85599721901744630, 251.6422919425777138 ) ) ;
#62393=CARTESIAN_POINT ( 'NONE',  ( 108.2766895582742848, -26.33922418024667422, 125.9841967044819597 ) ) ;
#62394=CARTESIAN_POINT ( 'NONE',  ( 115.9437545354735306, -30.06674848629992880, 260.3508633711495008 ) ) ;
#62395=CIRCLE ( 'NONE', #4374, 2.749999999999974687 ) ;
#62397=DIRECTION ( 'NONE',  ( 0.000000000000000000, 0.000000000000000000, 1.000000000000000000 ) ) ;
#62398=LINE ( 'NONE', #22426, #67517 ) ;
#62401=CARTESIAN_POINT ( 'NONE',  ( 31.46648329127298993, 12.92155284005730387, 355.9756252759109998 ) ) ;
#62402=EDGE_CURVE ( 'NONE', #30574, #1430, #85442, .T. ) ;
#62403=VERTEX_POINT ( 'NONE', #47755 ) ;
#62406=CARTESIAN_POINT ( 'NONE',  ( 108.3843752505750331, -28.29029480288096465, 189.3752769709339816 ) ) ;
#62407=CARTESIAN_POINT ( 'NONE',  ( 105.7129185420862427, -46.72347023951986955, 187.4693006236904580 ) ) ;
#62408=ORIENTED_EDGE ( 'NONE', *, *, #60636, .T. ) ;
#62409=CARTESIAN_POINT ( 'NONE',  ( 75.31670390244798341, -50.82844715994100682, 35.51780685541480409 ) ) ;
#62410=CARTESIAN_POINT ( 'NONE',  ( 98.87380182923587313, -30.31772012733814492, 151.7984824187679465 ) ) ;
#62411=CARTESIAN_POINT ( 'NONE',  ( 180.2121375201600131, -29.73316016639650172, -5.074374724088000832 ) ) ;
#62412=CARTESIAN_POINT ( 'NONE',  ( 97.81168731305311326, -40.51740136754563082, 36.63591984386916067 ) ) ;
#62413=ADVANCED_FACE ( 'NONE', ( #61393 ), #55002, .F. ) ;
#62414=DIRECTION ( 'NONE',  ( -1.000000000000000078E-15, 1.000000000000000083E-30, 1.000000000000000000 ) ) ;
#62415=CARTESIAN_POINT ( 'NONE',  ( 123.6837132603318992, -53.34645651782490461, 239.5838068554164693 ) ) ;
#62417=CARTESIAN_POINT ( 'NONE',  ( 107.5699729851651938, -26.92841289699908458, 95.03562527591097364 ) ) ;
#62418=ORIENTED_EDGE ( 'NONE', *, *, #10795, .T. ) ;
#62420=ORIENTED_EDGE ( 'NONE', *, *, #16336, .F. ) ;
#62424=CARTESIAN_POINT ( 'NONE',  ( 107.6181574201208520, -47.08485352040289484, 193.6308633711479672 ) ) ;
#62426=CARTESIAN_POINT ( 'NONE',  ( 130.5667039024479834, -39.24694715994093741, 239.5838068554170377 ) ) ;
#62427=CYLINDRICAL_SURFACE ( 'NONE', #77105, 4.874999999999990230 ) ;
#62431=CYLINDRICAL_SURFACE ( 'NONE', #55001, 2.030000000002086580 ) ;
#62433=EDGE_CURVE ( 'NONE', #4309, #41740, #30293, .T. ) ;
#62434=CARTESIAN_POINT ( 'NONE',  ( 99.07096106853131801, -43.38529345585687480, 116.8784824187679732 ) ) ;
#62436=ORIENTED_EDGE ( 'NONE', *, *, #12054, .T. ) ;
#62438=EDGE_CURVE ( 'NONE', #6607, #13307, #47306, .T. ) ;
#62440=CARTESIAN_POINT ( 'NONE',  ( 31.71315051185499811, -33.70561438052111214, 342.9256252759109884 ) ) ;
#62443=DIRECTION ( 'NONE',  ( 9.912705577010326536E-16, 1.000000000000000000, 0.000000000000000000 ) ) ;
#62444=CARTESIAN_POINT ( 'NONE',  ( 112.3000890867684234, -42.99355894011079471, 190.9480903695919665 ) ) ;
#62445=AXIS2_PLACEMENT_3D ( 'NONE', #61810, #82745, #12794 ) ;
#62446=DIRECTION ( 'NONE',  ( -1.000000000000000078E-15, -1.000000000000000083E-30, 1.000000000000000000 ) ) ;
#62448=ORIENTED_EDGE ( 'NONE', *, *, #29678, .T. ) ;
#62452=CARTESIAN_POINT ( 'NONE',  ( 136.6880318146010325, -19.56139158947305390, 2.921136715971410336 ) ) ;
#62453=ORIENTED_EDGE ( 'NONE', *, *, #85813, .F. ) ;
#62455=CARTESIAN_POINT ( 'NONE',  ( 78.88274585166998065, -21.21170328186978082, 8.006085407566775558 ) ) ;
#62456=CARTESIAN_POINT ( 'NONE',  ( 114.8460652499425123, -41.03528437643323201, 259.8558690201828654 ) ) ;
#62457=ORIENTED_EDGE ( 'NONE', *, *, #61668, .T. ) ;
#62461=EDGE_LOOP ( 'NONE', ( #60970, #10256, #5531, #86412 ) ) ;
#62462=ORIENTED_EDGE ( 'NONE', *, *, #2519, .T. ) ;
#62463=DIRECTION ( 'NONE',  ( 9.351236661543306751E-17, -3.725950533538267725E-29, -1.000000000000000000 ) ) ;
#62464=ORIENTED_EDGE ( 'NONE', *, *, #29617, .F. ) ;
#62465=EDGE_LOOP ( 'NONE', ( #42116, #23626, #55741, #7893 ) ) ;
#62466=VECTOR ( 'NONE', #9070, 1000.000000000000000 ) ;
#62467=CARTESIAN_POINT ( 'NONE',  ( 112.3037015629680866, -30.74301476610424544, 287.3214237029247897 ) ) ;
#62468=CARTESIAN_POINT ( 'NONE',  ( 117.0544076763083297, -30.30483159375883062, 144.2813395616249750 ) ) ;
#62469=AXIS2_PLACEMENT_3D ( 'NONE', #1078, #84218, #70573 ) ;
#62470=CARTESIAN_POINT ( 'NONE',  ( 97.56228874418788166, -32.49873190831181802, 100.9927681330539713 ) ) ;
#62471=CARTESIAN_POINT ( 'NONE',  ( 46.48091746482135278, -49.32844715994084339, 249.9678068554150343 ) ) ;
#62472=CARTESIAN_POINT ( 'NONE',  ( 131.7155263566451140, -17.29868341350382366, 7.242354772873104807 ) ) ;
#62473=CARTESIAN_POINT ( 'NONE',  ( 101.4253818664906959, -46.23481170842615740, 203.1622919425779514 ) ) ;
#62474=CARTESIAN_POINT ( 'NONE',  ( 107.0664832912730020, -36.72944715994189835, 361.9756252759079871 ) ) ;
#62478=ORIENTED_EDGE ( 'NONE', *, *, #83162, .T. ) ;
#62480=DIRECTION ( 'NONE',  ( 0.000000000000000000, 0.000000000000000000, -1.000000000000000000 ) ) ;
#62481=VECTOR ( 'NONE', #83350, 1000.000000000000000 ) ;
#62483=VECTOR ( 'NONE', #74979, 1000.000000000000000 ) ;
#62484=EDGE_CURVE ( 'NONE', #40888, #65495, #41831, .T. ) ;
#62485=CARTESIAN_POINT ( 'NONE',  ( 103.4683284843053883, -46.51414440030927011, 142.2956252759109645 ) ) ;
#62487=DIRECTION ( 'NONE',  ( 1.000000000000000000, 1.734723475976805580E-13, 0.000000000000000000 ) ) ;
#62489=ADVANCED_FACE ( 'NONE', ( #35031, #88237 ), #46851, .T. ) ;
#62490=DIRECTION ( 'NONE',  ( 0.9999999853157766072, 0.0001713722456143214551, -0.000000000000000000 ) ) ;
#62491=CARTESIAN_POINT ( 'NONE',  ( 31.56670390244800828, -33.35206098992711077, -5.074374724088000832 ) ) ;
#62492=CARTESIAN_POINT ( 'NONE',  ( 109.3321198358311932, -26.57584895156214699, 220.9013395616249795 ) ) ;
#62494=FACE_OUTER_BOUND ( 'NONE', #8298, .T. ) ;
#62499=CARTESIAN_POINT ( 'NONE',  ( 51.06648329127400388, -18.82844715994099971, 335.9181252759120184 ) ) ;
#62500=ADVANCED_FACE ( 'NONE', ( #16400 ), #82509, .T. ) ;
#62503=CARTESIAN_POINT ( 'NONE',  ( 108.0181136390867636, -24.86676629934084559, 265.0127681330534415 ) ) ;
#62504=EDGE_LOOP ( 'NONE', ( #31401, #42108 ) ) ;
#62507=CARTESIAN_POINT ( 'NONE',  ( 105.7175586466805157, -24.93052779236126781, 160.1670538473389627 ) ) ;
#62508=CARTESIAN_POINT ( 'NONE',  ( 103.5987781142019202, -46.56090220241721767, 53.30705384733997221 ) ) ;
#62509=CARTESIAN_POINT ( 'NONE',  ( 117.0647351476834643, -39.95015185843580952, 154.5784824187679476 ) ) ;
#62510=CARTESIAN_POINT ( 'NONE',  ( 109.7248658465021549, -27.00080515782364543, 30.86479194874874921 ) ) ;
#62512=CARTESIAN_POINT ( 'NONE',  ( 152.5667039024472444, -23.42844715993586036, 300.4678068554149490 ) ) ;
#62513=DIRECTION ( 'NONE',  ( 0.000000000000000000, 0.000000000000000000, -1.000000000000000000 ) ) ;
#62516=ORIENTED_EDGE ( 'NONE', *, *, #87021, .F. ) ;
#62517=VECTOR ( 'NONE', #51652, 1000.000000000000000 ) ;
#62518=EDGE_CURVE ( 'NONE', #40389, #68948, #15954, .T. ) ;
#62521=ORIENTED_EDGE ( 'NONE', *, *, #37878, .F. ) ;
#62524=ORIENTED_EDGE ( 'NONE', *, *, #62620, .F. ) ;
#62525=CARTESIAN_POINT ( 'NONE',  ( 107.2318599658364207, -25.70055450771780059, 76.07657765686298035 ) ) ;
#62526=DIRECTION ( 'NONE',  ( 0.000000000000000000, 1.000000000000000000, 0.000000000000000000 ) ) ;
#62527=VECTOR ( 'NONE', #68078, 1000.000000000000000 ) ;
#62530=CARTESIAN_POINT ( 'NONE',  ( 117.0586869608412286, -33.60713302236428746, 170.0670538473399631 ) ) ;
#62531=CARTESIAN_POINT ( 'NONE',  ( 101.4222765643661006, -43.81150905960179642, 271.4514674471243438 ) ) ;
#62532=EDGE_LOOP ( 'NONE', ( #76815, #58639, #52391, #51714, #43472, #25839 ) ) ;
#62535=ORIENTED_EDGE ( 'NONE', *, *, #13091, .F. ) ;
#62536=DIRECTION ( 'NONE',  ( 1.000000000000000078E-15, 0.000000000000000000, 1.000000000000000000 ) ) ;
#62539=CARTESIAN_POINT ( 'NONE',  ( 116.3188053082936051, -32.94429434937755019, 19.13562527591095019 ) ) ;
#62541=DIRECTION ( 'NONE',  ( -1.000000000000000000, -2.756263715554006823E-15, 0.000000000000000000 ) ) ;
#62542=DIRECTION ( 'NONE',  ( 0.000000000000000000, 0.000000000000000000, -1.000000000000000000 ) ) ;
#62543=DIRECTION ( 'NONE',  ( 1.000000000000000000, 1.346944695195362088E-15, 1.000000000000000078E-15 ) ) ;
#62544=CARTESIAN_POINT ( 'NONE',  ( 96.36668125800717633, -39.40815171121898430, 16.53372051400597798 ) ) ;
#62547=EDGE_CURVE ( 'NONE', #31182, #68744, #21877, .T. ) ;
#62552=CARTESIAN_POINT ( 'NONE',  ( 109.1833626410332130, -45.12109460632434121, 90.60332846482899072 ) ) ;
#62555=DIRECTION ( 'NONE',  ( 0.7071067811865493491, -0.7071067811865456854, 7.071067811865500971E-16 ) ) ;
#62556=VERTEX_POINT ( 'NONE', #63649 ) ;
#62557=VERTEX_POINT ( 'NONE', #63197 ) ;
#62558=CARTESIAN_POINT ( 'NONE',  ( 77.53258422225754032, -35.66080143920403600, 7.039723185228990765 ) ) ;
#62559=VERTEX_POINT ( 'NONE', #55905 ) ;
#62560=ORIENTED_EDGE ( 'NONE', *, *, #50320, .F. ) ;
#62563=CARTESIAN_POINT ( 'NONE',  ( 97.67166470235704878, -36.60562237181873257, 152.7596785439919813 ) ) ;
#62565=CARTESIAN_POINT ( 'NONE',  ( 110.1643932622899200, -46.70643130671602705, 93.81562527591097478 ) ) ;
#62566=VECTOR ( 'NONE', #38366, 999.9999999999998863 ) ;
#62568=LINE ( 'NONE', #48459, #35796 ) ;
#62571=ORIENTED_EDGE ( 'NONE', *, *, #17487, .F. ) ;
#62572=ORIENTED_EDGE ( 'NONE', *, *, #8109, .T. ) ;
#62574=CARTESIAN_POINT ( 'NONE',  ( 116.3212776292296127, -32.94146857471318413, 287.6356252759109680 ) ) ;
#62575=ORIENTED_EDGE ( 'NONE', *, *, #20008, .F. ) ;
#62576=CARTESIAN_POINT ( 'NONE',  ( 100.4791399132688809, -44.80881982087489490, 12.03276813305398463 ) ) ;
#62577=CARTESIAN_POINT ( 'NONE',  ( 117.0539910656555094, -30.30509957368958496, 140.2813395616249750 ) ) ;
#62578=B_SPLINE_CURVE_WITH_KNOTS ( 'NONE', 3,
 ( #23642, #58141, #43604, #57693, #63617, #42699, #15486, #2299, #64519, #65408, #78166, #23211, #64074, #70896, #30002, #1401, #51304, #15025, #16816, #56788, #24081, #30446, #9114, #36813, #50878, #29103, #70439, #44497, #72229, #2746, #84535, #71784, #22293, #85435, #3188, #78615 ),
 .UNSPECIFIED., .F., .F.,
 ( 4, 2, 2, 2, 2, 2, 1, 1, 1, 1, 1, 1, 2, 2, 2, 2, 2, 2, 2, 2, 4 ),
 ( 0.4999721494150220491, 0.5624756307362179797, 0.6249791120574139658, 0.6874825933786099519, 0.7499860746998059380, 0.7501081518117613811, 0.7502302289237168242, 0.7504743831476426985, 0.7509626915954943360, 0.7519393084912020520, 0.7538925422826163736, 0.7577990098654362461, 0.7656119450310676644, 0.7812378153623301680, 0.8124895560248543980, 0.8437412966873787390, 0.8749930373499029690, 0.9062447780124271990, 0.9374965186749515400, 0.9687482593374758810, 1.000000000000000000 ),
 .UNSPECIFIED. ) ;
#62579=DIRECTION ( 'NONE',  ( 0.9242245927363026414, 0.3818493186865932754, 0.000000000000000000 ) ) ;
#62581=CARTESIAN_POINT ( 'NONE',  ( 107.2322063299336605, -25.67745564896214816, 76.07657765686298035 ) ) ;
#62583=CARTESIAN_POINT ( 'NONE',  ( 108.3334481201889332, -46.73485935054446827, 262.6772919445848515 ) ) ;
#62585=CARTESIAN_POINT ( 'NONE',  ( 97.60817236302852962, -39.98324860507392486, 116.5905493758438780 ) ) ;
#62587=ADVANCED_FACE ( 'NONE', ( #70471 ), #56813, .T. ) ;
#62588=ORIENTED_EDGE ( 'NONE', *, *, #43939, .T. ) ;
#62589=DIRECTION ( 'NONE',  ( -0.7071067811865436870, 0.7071067811865513475, -7.071067811865430960E-16 ) ) ;
#62591=CARTESIAN_POINT ( 'NONE',  ( 112.9632928630424402, -28.13208318394687524, 44.59848241876795782 ) ) ;
#62595=DIRECTION ( 'NONE',  ( 0.000000000000000000, 1.000000000000000000, 0.000000000000000000 ) ) ;
#62597=CARTESIAN_POINT ( 'NONE',  ( 97.69287098190314111, -33.93680905855605801, 31.09562527591097592 ) ) ;
#62598=CARTESIAN_POINT ( 'NONE',  ( 107.0667039024479834, -36.72944715994100306, 239.5838068554170093 ) ) ;
#62599=CARTESIAN_POINT ( 'NONE',  ( 96.05093434719803724, -37.29646042206077539, 117.3794347997199594 ) ) ;
#62600=CARTESIAN_POINT ( 'NONE',  ( 20.03715912545641231, -24.95799193693202156, 180.4678068554150911 ) ) ;
#62601=DIRECTION ( 'NONE',  ( 0.000000000000000000, 1.000000000000000000, 0.000000000000000000 ) ) ;
#62602=ORIENTED_EDGE ( 'NONE', *, *, #36838, .T. ) ;
#62604=AXIS2_PLACEMENT_3D ( 'NONE', #13925, #731, #29354 ) ;
#62605=ADVANCED_FACE ( 'NONE', ( #64548 ), #30027, .F. ) ;
#62606=FACE_BOUND ( 'NONE', #42958, .T. ) ;
#62607=CARTESIAN_POINT ( 'NONE',  ( 142.0664832912740394, -56.72944715994099596, 14.92562527591100618 ) ) ;
#62608=VERTEX_POINT ( 'NONE', #57720 ) ;
#62609=CARTESIAN_POINT ( 'NONE',  ( 113.2479660781328050, -28.76056331078183348, 60.55236680792867787 ) ) ;
#62610=CARTESIAN_POINT ( 'NONE',  ( 116.8364808817232756, -40.58936182315601116, 193.5270538473389479 ) ) ;
#62611=ORIENTED_EDGE ( 'NONE', *, *, #4195, .F. ) ;
#62613=CARTESIAN_POINT ( 'NONE',  ( 130.5667039024479834, -33.42944715994100591, 239.5838068554162987 ) ) ;
#62614=CARTESIAN_POINT ( 'NONE',  ( 98.88183825371838509, -29.26641886349639066, 226.7261014663869503 ) ) ;
#62616=CIRCLE ( 'NONE', #3103, 2.517500000000005844 ) ;
#62617=LINE ( 'NONE', #47629, #21328 ) ;
#62620=EDGE_CURVE ( 'NONE', #70341, #75711, #85461, .T. ) ;
#62621=VECTOR ( 'NONE', #44469, 1000.000000000000000 ) ;
#62622=ORIENTED_EDGE ( 'NONE', *, *, #5838, .F. ) ;
#62627=CARTESIAN_POINT ( 'NONE',  ( 116.8848192732620390, -41.80628269293674748, 239.4346728949589647 ) ) ;
#62632=CARTESIAN_POINT ( 'NONE',  ( 151.0371591254572934, -24.42818131005592974, 300.4678068554149490 ) ) ;
#62634=CARTESIAN_POINT ( 'NONE',  ( 107.0664832912739399, -36.72944715994095333, 311.3356252759109566 ) ) ;
#62635=CARTESIAN_POINT ( 'NONE',  ( 118.7574168473771152, -34.64232270468420438, 48.96705384733895983 ) ) ;
#62636=VERTEX_POINT ( 'NONE', #518 ) ;
#62637=AXIS2_PLACEMENT_3D ( 'NONE', #74023, #53545, #81314 ) ;
#62638=EDGE_LOOP ( 'NONE', ( #7065, #1737, #13801, #63307 ) ) ;
#62639=AXIS2_PLACEMENT_3D ( 'NONE', #66399, #25074, #5083 ) ;
#62640=CARTESIAN_POINT ( 'NONE',  ( 89.17003477451882532, -56.47944715994104570, 14.92562527591095289 ) ) ;
#62642=CARTESIAN_POINT ( 'NONE',  ( 101.2091419812965256, -45.28691980162477648, 238.1108633711489517 ) ) ;
#62645=CARTESIAN_POINT ( 'NONE',  ( 114.7602587138392209, -43.68247563549507362, 79.25372051400597684 ) ) ;
#62648=CARTESIAN_POINT ( 'NONE',  ( 103.2881778167501921, -27.47069784023410577, 21.38479467184932048 ) ) ;
#62651=ORIENTED_EDGE ( 'NONE', *, *, #64339, .T. ) ;
#62655=CARTESIAN_POINT ( 'NONE',  ( 101.1777422249941338, -43.35145646725580804, 263.4301547344683740 ) ) ;
#62656=CARTESIAN_POINT ( 'NONE',  ( 34.33598329127499227, -36.32844715994100682, -5.074374724088000832 ) ) ;
#62657=DIRECTION ( 'NONE',  ( 6.745093096447288888E-17, 1.000000000000000000, 0.000000000000000000 ) ) ;
#62658=PLANE ( 'NONE',  #53360 ) ;
#62662=LINE ( 'NONE', #40867, #38269 ) ;
#62663=ORIENTED_EDGE ( 'NONE', *, *, #10513, .T. ) ;
#62664=CARTESIAN_POINT ( 'NONE',  ( 112.7417948769132039, -27.24419935825454431, 54.65943479971996055 ) ) ;
#62666=CARTESIAN_POINT ( 'NONE',  ( 113.7913882254195101, -32.05415687329151098, 277.1280903695913480 ) ) ;
#62668=CARTESIAN_POINT ( 'NONE',  ( 107.6181574201208662, -47.08485352040301564, 197.6308633711499567 ) ) ;
#62669=ADVANCED_FACE ( 'NONE', ( #17733 ), #79081, .T. ) ;
#62671=CARTESIAN_POINT ( 'NONE',  ( 107.0667039024467329, -36.72944715994091780, 196.2188068554169718 ) ) ;
#62674=FACE_OUTER_BOUND ( 'NONE', #34526, .T. ) ;
#62675=CARTESIAN_POINT ( 'NONE',  ( 98.90868739403623522, -30.16870437830188934, 236.7870538473399336 ) ) ;
#62676=CARTESIAN_POINT ( 'NONE',  ( 104.6050160698606959, -46.44121287996537717, 117.3807199075759371 ) ) ;
#62677=ORIENTED_EDGE ( 'NONE', *, *, #44049, .F. ) ;
#62679=EDGE_CURVE ( 'NONE', #1672, #40777, #3218, .T. ) ;
#62680=CARTESIAN_POINT ( 'NONE',  ( 136.4105765916224584, -38.17027654744433107, 7.249284792663315713 ) ) ;
#62681=ORIENTED_EDGE ( 'NONE', *, *, #3957, .F. ) ;
#62682=CARTESIAN_POINT ( 'NONE',  ( 98.80568095843470644, -28.16380313737984764, 111.6870538473389587 ) ) ;
#62685=VERTEX_POINT ( 'NONE', #74033 ) ;
#62686=ORIENTED_EDGE ( 'NONE', *, *, #78237, .F. ) ;
#62691=CARTESIAN_POINT ( 'NONE',  ( 85.58420390244808118, -58.72944715994107412, 207.5838068554169809 ) ) ;
#62692=CARTESIAN_POINT ( 'NONE',  ( 106.0125404296577045, -27.51070622278902533, 157.9852332267339534 ) ) ;
#62693=CARTESIAN_POINT ( 'NONE',  ( 111.7834783340718872, -46.75425468364281301, 283.9146728949586418 ) ) ;
#62695=FACE_OUTER_BOUND ( 'NONE', #27060, .T. ) ;
#62697=DIRECTION ( 'NONE',  ( 1.000000000000000000, 0.000000000000000000, 0.000000000000000000 ) ) ;
#62700=AXIS2_PLACEMENT_3D ( 'NONE', #75779, #77125, #22169 ) ;
#62701=DIRECTION ( 'NONE',  ( 3.999999999999999995E-14, -1.000000000000000000, 4.100000000000000342E-29 ) ) ;
#62702=CARTESIAN_POINT ( 'NONE',  ( 161.4809174648183898, -48.32844715993547879, 249.9678068554149490 ) ) ;
#62704=DIRECTION ( 'NONE',  ( 0.0001713722456133601202, -0.9999999853157766072, -1.713722456133601401E-19 ) ) ;
#62705=CARTESIAN_POINT ( 'NONE',  ( 53.56670390244833158, -48.82844715994055917, 249.9678068554150343 ) ) ;
#62706=EDGE_CURVE ( 'NONE', #5742, #27981, #47023, .T. ) ;
#62707=CARTESIAN_POINT ( 'NONE',  ( 107.2112434921279629, -45.29864470754334604, 212.0124198280769861 ) ) ;
#62709=CARTESIAN_POINT ( 'NONE',  ( 96.61245533174189859, -37.29510205964861314, 76.36991099019697060 ) ) ;
#62712=VERTEX_POINT ( 'NONE', #51777 ) ;
#62715=ORIENTED_EDGE ( 'NONE', *, *, #70327, .T. ) ;
#62716=DIRECTION ( 'NONE',  ( 0.0001211784769825750168, -0.7071067708032372501, 0.7071067811865437980 ) ) ;
#62717=ADVANCED_FACE ( 'NONE', ( #3656 ), #31796, .F. ) ;
#62718=ORIENTED_EDGE ( 'NONE', *, *, #37073, .T. ) ;
#62720=DIRECTION ( 'NONE',  ( 0.000000000000000000, 0.000000000000000000, -1.000000000000000000 ) ) ;
#62722=CARTESIAN_POINT ( 'NONE',  ( 188.5667039024479834, -58.35344715994099829, 134.4678068554150059 ) ) ;
#62724=ADVANCED_FACE ( 'NONE', ( #11357 ), #30471, .T. ) ;
#62725=CARTESIAN_POINT ( 'NONE',  ( 96.69274360309970007, -38.23738870492909570, 66.44133956162495735 ) ) ;
#62726=FACE_OUTER_BOUND ( 'NONE', #27314, .T. ) ;
#62727=CARTESIAN_POINT ( 'NONE',  ( 83.73314995793998605, 12.92155284005730387, 358.9756252759109998 ) ) ;
#62729=CYLINDRICAL_SURFACE ( 'NONE', #67347, 5.500000000000000888 ) ;
#62730=ORIENTED_EDGE ( 'NONE', *, *, #14221, .T. ) ;
#62731=ADVANCED_FACE ( 'NONE', ( #52213 ), #73129, .T. ) ;
#62732=AXIS2_PLACEMENT_3D ( 'NONE', #41275, #35364, #61717 ) ;
#62734=DIRECTION ( 'NONE',  ( 0.7071067811868710917, -0.7071067811862240537, 0.000000000000000000 ) ) ;
#62736=VERTEX_POINT ( 'NONE', #46300 ) ;
#62737=CARTESIAN_POINT ( 'NONE',  ( 108.5410322698540853, -26.38715707682645117, 100.9641967044829727 ) ) ;
#62738=FACE_OUTER_BOUND ( 'NONE', #66391, .T. ) ;
#62739=DIRECTION ( 'NONE',  ( -0.7071067812163274180, 0.7071067811567677275, -6.612322856138636565E-17 ) ) ;
#62741=VECTOR ( 'NONE', #40662, 1000.000000000000000 ) ;
#62743=CARTESIAN_POINT ( 'NONE',  ( 103.4152017835536270, -27.65577212482034497, 126.3813395616249835 ) ) ;
#62744=DIRECTION ( 'NONE',  ( -2.999999999999999839E-15, 1.000000000000000000, -2.999999999999999900E-30 ) ) ;
#62746=CARTESIAN_POINT ( 'NONE',  ( 115.8883252675856994, -30.10835006627626953, 260.3508633711493871 ) ) ;
#62750=CARTESIAN_POINT ( 'NONE',  ( 48.85858412957969676, -30.08671355700278127, 117.4678068554150485 ) ) ;
#62754=CARTESIAN_POINT ( 'NONE',  ( 98.96845470676149148, -30.25173782105007803, 195.7775300378159784 ) ) ;
#62755=ORIENTED_EDGE ( 'NONE', *, *, #7247, .F. ) ;
#62757=EDGE_CURVE ( 'NONE', #51366, #35978, #11418, .T. ) ;
#62758=CARTESIAN_POINT ( 'NONE',  ( 115.6173342623064713, -34.29738501013303420, 145.4787261630399371 ) ) ;
#62759=VECTOR ( 'NONE', #66275, 1000.000000000000000 ) ;
#62760=FACE_OUTER_BOUND ( 'NONE', #53370, .T. ) ;
#62761=CARTESIAN_POINT ( 'NONE',  ( 98.24556308671769500, -33.49403671529641713, 17.46634521065892898 ) ) ;
#62762=DIRECTION ( 'NONE',  ( 0.000000000000000000, -1.000000000000000000, 0.000000000000000000 ) ) ;
#62763=ADVANCED_FACE ( 'NONE', ( #85899 ), #38613, .T. ) ;
#62764=CARTESIAN_POINT ( 'NONE',  ( 63.56670390244800473, -40.82844715994016127, 249.9678068554150343 ) ) ;
#62766=CARTESIAN_POINT ( 'NONE',  ( 109.7248659187796136, -27.00080517901244193, 105.8647919427923370 ) ) ;
#62768=CARTESIAN_POINT ( 'NONE',  ( 117.2062538965840304, -41.07097622818930915, 213.5165776568629781 ) ) ;
#62769=CARTESIAN_POINT ( 'NONE',  ( 72.06648329127402519, -45.72944715994106701, -4.824374724089063982 ) ) ;
#62770=VERTEX_POINT ( 'NONE', #72257 ) ;
#62775=DIRECTION ( 'NONE',  ( 2.999999999999999839E-15, -1.000000000000000000, 2.999999999999999900E-30 ) ) ;
#62776=LINE ( 'NONE', #7380, #9368 ) ;
#62777=ORIENTED_EDGE ( 'NONE', *, *, #9830, .T. ) ;
#62778=EDGE_CURVE ( 'NONE', #397, #52666, #72316, .T. ) ;
#62780=CARTESIAN_POINT ( 'NONE',  ( 117.3350766552244977, -34.92860824786317409, 243.9641967044819637 ) ) ;
#62781=ORIENTED_EDGE ( 'NONE', *, *, #47223, .F. ) ;
#62783=CARTESIAN_POINT ( 'NONE',  ( 77.76062680957220152, -38.22815166919947671, 7.286367513304666588 ) ) ;
#62784=DIRECTION ( 'NONE',  ( 3.999999999999999995E-14, -1.000000000000000000, 4.100000000000000342E-29 ) ) ;
#62786=CARTESIAN_POINT ( 'NONE',  ( 114.5896176151078976, -33.49137084947443554, 76.96809036959095351 ) ) ;
#62787=CARTESIAN_POINT ( 'NONE',  ( 108.9491117623569636, -26.41756539094687639, 160.9327681330539690 ) ) ;
#62788=DIRECTION ( 'NONE',  ( 1.000000000000000000, -1.387778780781444413E-14, 0.000000000000000000 ) ) ;
#62789=ORIENTED_EDGE ( 'NONE', *, *, #50391, .F. ) ;
#62790=CARTESIAN_POINT ( 'NONE',  ( 107.0664832912739968, -0.7548456658612000547, 335.0256252759120343 ) ) ;
#62791=VERTEX_POINT ( 'NONE', #40404 ) ;
#62792=VERTEX_POINT ( 'NONE', #32694 ) ;
#62794=DIRECTION ( 'NONE',  ( -0.7071067811861110330, -0.7071067811869841124, 0.000000000000000000 ) ) ;
#62795=ORIENTED_EDGE ( 'NONE', *, *, #89512, .F. ) ;
#62796=ORIENTED_EDGE ( 'NONE', *, *, #47558, .F. ) ;
#62800=CARTESIAN_POINT ( 'NONE',  ( 115.9068402959922111, -38.69432841718559501, 103.0628960185529763 ) ) ;
#62801=CARTESIAN_POINT ( 'NONE',  ( 101.3926005705062749, -45.54394758209068073, 222.1213395616249784 ) ) ;
#62802=CARTESIAN_POINT ( 'NONE',  ( 101.3611157396114066, -46.16939438856412181, 202.1318157521019430 ) ) ;
#62803=CARTESIAN_POINT ( 'NONE',  ( 101.1533894386775501, -27.41820966596962705, 61.51467289495899138 ) ) ;
#62804=FACE_OUTER_BOUND ( 'NONE', #4720, .T. ) ;
#62806=CARTESIAN_POINT ( 'NONE',  ( 116.3244028009478797, -32.94573790848593120, 95.13562527591096796 ) ) ;
#62808=ORIENTED_EDGE ( 'NONE', *, *, #65169, .F. ) ;
#62812=CARTESIAN_POINT ( 'NONE',  ( 116.3126599349421895, -33.43976754494798342, 114.0984824187689668 ) ) ;
#62813=AXIS2_PLACEMENT_3D ( 'NONE', #29438, #63960, #42148 ) ;
#62814=CARTESIAN_POINT ( 'NONE',  ( 106.6586145429690475, -26.26807492067915462, 85.10705384733896040 ) ) ;
#62815=CARTESIAN_POINT ( 'NONE',  ( 115.0886446791137132, -30.00251675211520919, 269.3813395616250546 ) ) ;
#62816=ORIENTED_EDGE ( 'NONE', *, *, #43037, .T. ) ;
#62817=CARTESIAN_POINT ( 'NONE',  ( 96.77592423366979801, -40.76472679528808385, 246.6118157521009664 ) ) ;
#62820=VECTOR ( 'NONE', #78260, 999.9999999999998863 ) ;
#62821=CARTESIAN_POINT ( 'NONE',  ( 31.46648329127298993, 12.92155284005730387, 358.9756252759109998 ) ) ;
#62822=CARTESIAN_POINT ( 'NONE',  ( 31.56670390244768143, -32.29483332968644049, 237.4678068554150059 ) ) ;
#62823=CARTESIAN_POINT ( 'NONE',  ( 108.1902092590197526, -46.32316586329737618, 277.6356252759110816 ) ) ;
#62825=CARTESIAN_POINT ( 'NONE',  ( 106.4519520244838588, -25.28636983920703329, 320.5381088016924309 ) ) ;
#62827=VECTOR ( 'NONE', #24041, 1000.000000000000000 ) ;
#62829=EDGE_CURVE ( 'NONE', #19003, #25445, #41282, .T. ) ;
#62830=CYLINDRICAL_SURFACE ( 'NONE', #6609, 0.9999999999999731326 ) ;
#62831=EDGE_CURVE ( 'NONE', #837, #60890, #67209, .T. ) ;
#62833=DIRECTION ( 'NONE',  ( -1.000000000000000078E-15, 1.000000000000000083E-30, 1.000000000000000000 ) ) ;
#62834=DIRECTION ( 'NONE',  ( 0.000000000000000000, 0.000000000000000000, -1.000000000000000000 ) ) ;
#62837=CARTESIAN_POINT ( 'NONE',  ( 115.7947005615567235, -30.98796762508558444, 254.2899109901966028 ) ) ;
#62838=CARTESIAN_POINT ( 'NONE',  ( 117.0231160686283687, -39.93674523842013713, 154.5784824187679476 ) ) ;
#62839=CARTESIAN_POINT ( 'NONE',  ( 115.9636596525004677, -42.20459941147550609, 14.38705384733995984 ) ) ;
#62840=CARTESIAN_POINT ( 'NONE',  ( 107.0664832912739968, 19.62155284005901024, 333.4006252759110112 ) ) ;
#62841=CARTESIAN_POINT ( 'NONE',  ( 188.5667039024484382, -48.82844715993430640, 175.7178068554150343 ) ) ;
#62842=CARTESIAN_POINT ( 'NONE',  ( 81.23646709782372000, -34.23881677343926100, 8.012604158003382437 ) ) ;
#62843=CARTESIAN_POINT ( 'NONE',  ( 188.5667039024482392, -42.82844715993431350, 295.7178068554150059 ) ) ;
#62845=CIRCLE ( 'NONE', #23714, 3.300000000000000711 ) ;
#62846=VERTEX_POINT ( 'NONE', #67669 ) ;
#62847=LINE ( 'NONE', #25314, #72253 ) ;
#62849=CARTESIAN_POINT ( 'NONE',  ( 98.50657384982324061, -36.30512124771701821, 170.7095626852199359 ) ) ;
#62850=CARTESIAN_POINT ( 'NONE',  ( 80.06648329127402519, -46.72944715994105991, -0.8743747240890559214 ) ) ;
#62852=AXIS2_PLACEMENT_3D ( 'NONE', #50910, #49553, #21884 ) ;
#62854=CARTESIAN_POINT ( 'NONE',  ( 117.4355769707882473, -40.49052663852277334, 169.5375300378159693 ) ) ;
#62855=CARTESIAN_POINT ( 'NONE',  ( 117.0602965032632596, -38.08466649080754252, 149.7193872050756909 ) ) ;
#62856=CARTESIAN_POINT ( 'NONE',  ( 123.6837132603319560, -53.34645651782485487, 218.8274735512161158 ) ) ;
#62857=CARTESIAN_POINT ( 'NONE',  ( 102.6857145224375785, -27.71633897165153471, 86.43730029299915429 ) ) ;
#62860=B_SPLINE_CURVE_WITH_KNOTS ( 'NONE', 3,
 ( #63230, #548, #1007, #22355, #15541, #50483, #84140, #29606, #77312, #15086, #41422, #57295, #34623, #42760, #70500, #8273, #35970, #62328 ),
 .UNSPECIFIED., .F., .F.,
 ( 4, 2, 2, 2, 2, 2, 2, 2, 4 ),
 ( 0.4999999995531766439, 0.5624999996090295218, 0.6249999996648825107, 0.6874999997207353886, 0.7499999997765882664, 0.8124999998324412553, 0.8749999998882941332, 0.9374999999441471221, 1.000000000000000000 ),
 .UNSPECIFIED. ) ;
#62861=CARTESIAN_POINT ( 'NONE',  ( 116.7343647603066614, -32.97833357388812914, 94.10895860924495082 ) ) ;
#62863=ORIENTED_EDGE ( 'NONE', *, *, #53430, .F. ) ;
#62864=ORIENTED_EDGE ( 'NONE', *, *, #83740, .F. ) ;
#62865=TOROIDAL_SURFACE ( 'NONE', #7766, 15.69999999999999929, 0.2999999999999999889 ) ;
#62866=CARTESIAN_POINT ( 'NONE',  ( 101.0434111811767224, -43.22951492638978266, 43.41301187732599232 ) ) ;
#62868=CARTESIAN_POINT ( 'NONE',  ( 113.2764755850017480, -45.03455287549797248, 184.0994347997199725 ) ) ;
#62871=CARTESIAN_POINT ( 'NONE',  ( 179.4595971212889935, -28.98061976758940617, 117.4678068554150627 ) ) ;
#62872=EDGE_CURVE ( 'NONE', #42590, #10255, #4994, .T. ) ;
#62873=DIRECTION ( 'NONE',  ( 0.000000000000000000, 0.000000000000000000, 1.000000000000000000 ) ) ;
#62876=CARTESIAN_POINT ( 'NONE',  ( 113.8292797163802561, -28.77778007523021842, 139.5156252759109634 ) ) ;
#62878=ORIENTED_EDGE ( 'NONE', *, *, #18224, .F. ) ;
#62879=VERTEX_POINT ( 'NONE', #81761 ) ;
#62881=DIRECTION ( 'NONE',  ( 0.000000000000000000, 0.000000000000000000, -1.000000000000000000 ) ) ;
#62882=CARTESIAN_POINT ( 'NONE',  ( 116.8171228668576163, -34.15291832144532691, 80.03145860917631182 ) ) ;
#62883=CARTESIAN_POINT ( 'NONE',  ( 20.56670390244748603, -48.82844715994200158, 129.9678068554150627 ) ) ;
#62884=CARTESIAN_POINT ( 'NONE',  ( 112.7646070568428911, -30.84607450481293256, 172.2823760838769829 ) ) ;
#62886=EDGE_CURVE ( 'NONE', #61996, #70380, #5897, .T. ) ;
#62888=VECTOR ( 'NONE', #81823, 999.9999999999998863 ) ;
#62890=ORIENTED_EDGE ( 'NONE', *, *, #51430, .F. ) ;
#62891=ORIENTED_EDGE ( 'NONE', *, *, #12792, .T. ) ;
#62892=ORIENTED_EDGE ( 'NONE', *, *, #48520, .F. ) ;
#62893=FACE_OUTER_BOUND ( 'NONE', #80662, .T. ) ;
#62894=ORIENTED_EDGE ( 'NONE', *, *, #55173, .F. ) ;
#62897=CARTESIAN_POINT ( 'NONE',  ( 99.03278789346684619, -40.46950289042285220, 253.1044404487540760 ) ) ;
#62898=EDGE_CURVE ( 'NONE', #32750, #52806, #5448, .T. ) ;
#62899=DIRECTION ( 'NONE',  ( -0.000000000000000000, -0.000000000000000000, 1.000000000000000000 ) ) ;
#62900=ORIENTED_EDGE ( 'NONE', *, *, #25677, .F. ) ;
#62901=CARTESIAN_POINT ( 'NONE',  ( 25.56670390244797275, -62.87844715994099687, 293.2178068554150627 ) ) ;
#62904=ORIENTED_EDGE ( 'NONE', *, *, #9115, .F. ) ;
#62907=AXIS2_PLACEMENT_3D ( 'NONE', #46184, #40283, #33474 ) ;
#62908=ORIENTED_EDGE ( 'NONE', *, *, #38614, .T. ) ;
#62910=EDGE_CURVE ( 'NONE', #13427, #52429, #12713, .T. ) ;
#62911=CARTESIAN_POINT ( 'NONE',  ( 105.4654256982276905, -28.22429988993499350, 278.0547570362579677 ) ) ;
#62913=CARTESIAN_POINT ( 'NONE',  ( 116.8162545570497741, -32.97600546270004429, 139.1184824187679396 ) ) ;
#62914=CARTESIAN_POINT ( 'NONE',  ( 96.81317962367440089, -38.48968277746988065, 91.46133956162493917 ) ) ;
#62915=CARTESIAN_POINT ( 'NONE',  ( 116.2163998817092505, -39.91179612511876940, 249.5838068554169524 ) ) ;
#62916=LINE ( 'NONE', #1613, #19106 ) ;
#62917=CARTESIAN_POINT ( 'NONE',  ( 107.5100279102752552, -47.14509671329473406, 233.6099109901969655 ) ) ;
#62918=FACE_OUTER_BOUND ( 'NONE', #25997, .T. ) ;
#62920=FACE_OUTER_BOUND ( 'NONE', #22613, .T. ) ;
#62925=CARTESIAN_POINT ( 'NONE',  ( 172.5664832912740110, -18.82844715994099971, 76.80862527591200717 ) ) ;
#62926=CARTESIAN_POINT ( 'NONE',  ( 104.9606636336513930, -26.94125731171795479, 136.2451343372883912 ) ) ;
#62927=ORIENTED_EDGE ( 'NONE', *, *, #52790, .F. ) ;
#62928=CARTESIAN_POINT ( 'NONE',  ( 102.3126588425671315, -26.75045724741508124, 140.4422919425769578 ) ) ;
#62929=CARTESIAN_POINT ( 'NONE',  ( 102.0693270851732990, -27.96916624019228337, 255.4897280356127567 ) ) ;
#62933=CARTESIAN_POINT ( 'NONE',  ( 97.93479060588762763, -40.80611092822861252, 56.66021516895607846 ) ) ;
#62934=CARTESIAN_POINT ( 'NONE',  ( 97.03753386688410387, -33.96379371595042329, 247.1127681330539758 ) ) ;
#62937=ORIENTED_EDGE ( 'NONE', *, *, #71386, .T. ) ;
#62939=EDGE_CURVE ( 'NONE', #22291, #8503, #34691, .T. ) ;
#62940=CARTESIAN_POINT ( 'NONE',  ( 141.0667039024479834, -58.72944715994110254, 250.9178068554160461 ) ) ;
#62941=EDGE_CURVE ( 'NONE', #62232, #18115, #69015, .T. ) ;
#62945=CARTESIAN_POINT ( 'NONE',  ( 112.3606361654194075, -28.17110760307337713, 289.6356252759109680 ) ) ;
#62946=ORIENTED_EDGE ( 'NONE', *, *, #37600, .F. ) ;
#62947=CARTESIAN_POINT ( 'NONE',  ( 179.4595971212720258, -26.00627455219131789, -5.074374724088000832 ) ) ;
#62948=CARTESIAN_POINT ( 'NONE',  ( 97.98778932149404852, -30.38336575973633913, 160.8289586092449497 ) ) ;
#62949=CARTESIAN_POINT ( 'NONE',  ( 100.4110913530865332, -28.70521849941338033, 36.62705384733894221 ) ) ;
#62950=CARTESIAN_POINT ( 'NONE',  ( 117.1680251128577908, -33.85633223813928794, 145.0470538473399529 ) ) ;
#62951=ADVANCED_FACE ( 'NONE', ( #68570, #60838 ), #82215, .T. ) ;
#62952=CARTESIAN_POINT ( 'NONE',  ( 152.0368932755770288, -23.42844715993589588, 237.4678068554150059 ) ) ;
#62953=CARTESIAN_POINT ( 'NONE',  ( 115.0887396973123202, -30.61742992443682354, 100.3440234672758038 ) ) ;
#62954=CARTESIAN_POINT ( 'NONE',  ( 97.81168895331838087, -40.51742574516882200, 287.6356252759109680 ) ) ;
#62956=CARTESIAN_POINT ( 'NONE',  ( 108.4174892599855866, -26.73503592884603108, 69.96895860861965843 ) ) ;
#62959=AXIS2_PLACEMENT_3D ( 'NONE', #79726, #2525, #2075 ) ;
#62963=EDGE_LOOP ( 'NONE', ( #65136, #64070, #49252, #65743 ) ) ;
#62964=EDGE_LOOP ( 'NONE', ( #23188, #48134, #43323, #88948 ) ) ;
#62965=FACE_OUTER_BOUND ( 'NONE', #68462, .T. ) ;
#62966=ORIENTED_EDGE ( 'NONE', *, *, #74881, .T. ) ;
#62967=CARTESIAN_POINT ( 'NONE',  ( 101.1541078795468707, -28.12664281037979208, 46.55562527591094835 ) ) ;
#62969=FACE_OUTER_BOUND ( 'NONE', #21483, .T. ) ;
#62970=CARTESIAN_POINT ( 'NONE',  ( 113.6415746488294047, -45.67179987042115386, 179.0689586092439640 ) ) ;
#62971=CARTESIAN_POINT ( 'NONE',  ( 114.5649785483395249, -40.87970871860825639, 262.8467055423626562 ) ) ;
#62973=ORIENTED_EDGE ( 'NONE', *, *, #13021, .T. ) ;
#62974=ORIENTED_EDGE ( 'NONE', *, *, #32138, .F. ) ;
#62975=VECTOR ( 'NONE', #50034, 1000.000000000000000 ) ;
#62976=ORIENTED_EDGE ( 'NONE', *, *, #55199, .T. ) ;
#62977=LINE ( 'NONE', #64780, #19599 ) ;
#62978=AXIS2_PLACEMENT_3D ( 'NONE', #40501, #82763, #75922 ) ;
#62980=CARTESIAN_POINT ( 'NONE',  ( 188.5667039024484097, -48.82844715993431350, 257.2178068554150059 ) ) ;
#62981=AXIS2_PLACEMENT_3D ( 'NONE', #46605, #25282, #60238 ) ;
#62982=CARTESIAN_POINT ( 'NONE',  ( 115.0889047232446671, -30.61763667893183083, 74.34395860934252198 ) ) ;
#62987=DIRECTION ( 'NONE',  ( -1.000000000000000000, 0.000000000000000000, 0.000000000000000000 ) ) ;
#62988=CARTESIAN_POINT ( 'NONE',  ( 116.1393041698828057, -43.00708073170995505, 13.35657765686298859 ) ) ;
#62989=PLANE ( 'NONE',  #53007 ) ;
#62991=CARTESIAN_POINT ( 'NONE',  ( 29.56670390244797630, -67.87844715994100397, 20.91780685541479912 ) ) ;
#62993=CARTESIAN_POINT ( 'NONE',  ( 111.9804352529405804, -29.60526291441071578, 87.42618560768700320 ) ) ;
#62994=EDGE_CURVE ( 'NONE', #74036, #7464, #48531, .T. ) ;
#62995=EDGE_CURVE ( 'NONE', #57373, #73910, #1317, .T. ) ;
#62996=CYLINDRICAL_SURFACE ( 'NONE', #25304, 9.999999999999998224 ) ;
#62997=CYLINDRICAL_SURFACE ( 'NONE', #30047, 0.2500000000000002220 ) ;
#62999=ORIENTED_EDGE ( 'NONE', *, *, #16682, .T. ) ;
#63000=EDGE_CURVE ( 'NONE', #16763, #77789, #26011, .T. ) ;
#63001=CARTESIAN_POINT ( 'NONE',  ( 77.31648329127401098, -36.72944715994107412, 6.749768910606400496 ) ) ;
#63003=ORIENTED_EDGE ( 'NONE', *, *, #25665, .T. ) ;
#63004=EDGE_CURVE ( 'NONE', #37766, #64042, #48093, .T. ) ;
#63005=CARTESIAN_POINT ( 'NONE',  ( 112.1755263188685205, -29.48886997617658423, 126.0187261630399718 ) ) ;
#63008=CARTESIAN_POINT ( 'NONE',  ( 114.7233776882958409, -44.73301973330935510, 109.1718157521009687 ) ) ;
#63010=CIRCLE ( 'NONE', #86240, 2.117000000000000881 ) ;
#63011=CARTESIAN_POINT ( 'NONE',  ( 108.3334480752073858, -46.73485935666047908, 83.67729194100738255 ) ) ;
#63012=ORIENTED_EDGE ( 'NONE', *, *, #48728, .F. ) ;
#63016=ORIENTED_EDGE ( 'NONE', *, *, #71993, .F. ) ;
#63018=DIRECTION ( 'NONE',  ( 1.000000000000000000, -3.885780586188044357E-13, 0.000000000000000000 ) ) ;
#63020=CARTESIAN_POINT ( 'NONE',  ( 117.6440887749188846, -33.30491810902906735, 284.0756252759109657 ) ) ;
#63021=CARTESIAN_POINT ( 'NONE',  ( 98.36161695517027681, -29.88032255785606139, 196.8080062282919869 ) ) ;
#63023=CARTESIAN_POINT ( 'NONE',  ( 182.2300522401149863, -33.89581943344511217, 193.9678068554150059 ) ) ;
#63024=DIRECTION ( 'NONE',  ( 1.000000000000000078E-15, 1.000000000000000083E-30, -1.000000000000000000 ) ) ;
#63025=CARTESIAN_POINT ( 'NONE',  ( 109.2014185099688603, -26.52530387367253795, 135.9127681330539872 ) ) ;
#63027=DIRECTION ( 'NONE',  ( 1.000000000000000000, 4.510281037539788691E-14, 0.000000000000000000 ) ) ;
#63028=ORIENTED_EDGE ( 'NONE', *, *, #63540, .T. ) ;
#63029=CARTESIAN_POINT ( 'NONE',  ( 97.80435755565518718, -40.49946745241530266, 116.6343656781801599 ) ) ;
#63030=DIRECTION ( 'NONE',  ( 0.000000000000000000, 0.000000000000000000, -1.000000000000000000 ) ) ;
#63031=ORIENTED_EDGE ( 'NONE', *, *, #84610, .T. ) ;
#63032=AXIS2_PLACEMENT_3D ( 'NONE', #46338, #47688, #25928 ) ;
#63033=CARTESIAN_POINT ( 'NONE',  ( 76.06670390244792657, -14.72944715994109899, 239.5838068554169809 ) ) ;
#63034=VECTOR ( 'NONE', #28208, 1000.000000000000000 ) ;
#63035=AXIS2_PLACEMENT_3D ( 'NONE', #69013, #34023, #89463 ) ;
#63036=DIRECTION ( 'NONE',  ( 1.000000000000000000, 1.387778780781444413E-14, 0.000000000000000000 ) ) ;
#63037=CARTESIAN_POINT ( 'NONE',  ( 99.98060178585627966, -44.37649324013435859, 46.98133956162592284 ) ) ;
#63038=DIRECTION ( 'NONE',  ( -0.7071067811865336949, -0.7071067811865614505, 0.000000000000000000 ) ) ;
#63040=LINE ( 'NONE', #33984, #17295 ) ;
#63042=CARTESIAN_POINT ( 'NONE',  ( 101.9462936730086113, -46.59842863024385196, 17.19562527591095247 ) ) ;
#63043=CARTESIAN_POINT ( 'NONE',  ( 97.39146471609157629, -39.27917510135310408, 111.5315135458968996 ) ) ;
#63044=CARTESIAN_POINT ( 'NONE',  ( 117.2009162446674395, -42.82382785266563019, 124.3956252759109731 ) ) ;
#63045=CARTESIAN_POINT ( 'NONE',  ( 97.31584371926621202, -39.30597601181960243, 72.53145861026970920 ) ) ;
#63046=DIRECTION ( 'NONE',  ( 0.000000000000000000, 0.000000000000000000, -1.000000000000000000 ) ) ;
#63047=ORIENTED_EDGE ( 'NONE', *, *, #25648, .F. ) ;
#63049=VECTOR ( 'NONE', #11563, 1000.000000000000000 ) ;
#63050=CIRCLE ( 'NONE', #3593, 2.999999999999947153 ) ;
#63051=FACE_BOUND ( 'NONE', #28455, .T. ) ;
#63054=EDGE_CURVE ( 'NONE', #37163, #27030, #45895, .T. ) ;
#63055=CARTESIAN_POINT ( 'NONE',  ( 106.5785131942345458, -24.40100501111790621, 323.5352776872487652 ) ) ;
#63056=CARTESIAN_POINT ( 'NONE',  ( 97.34100429996045989, -42.07995573552675950, 176.7146728949589658 ) ) ;
#63057=ORIENTED_EDGE ( 'NONE', *, *, #32033, .F. ) ;
#63059=CARTESIAN_POINT ( 'NONE',  ( 115.5350430195811668, -29.59021037493291573, 220.3718157521019521 ) ) ;
#63060=CARTESIAN_POINT ( 'NONE',  ( 110.3857440325295443, -47.32095349711466525, 48.80610146638797175 ) ) ;
#63061=EDGE_CURVE ( 'NONE', #77895, #81541, #15409, .T. ) ;
#63064=CARTESIAN_POINT ( 'NONE',  ( 116.3212776292269552, -32.94146857470667555, 79.13562527591095375 ) ) ;
#63065=ORIENTED_EDGE ( 'NONE', *, *, #17880, .T. ) ;
#63067=VECTOR ( 'NONE', #77030, 1000.000000000000000 ) ;
#63068=ORIENTED_EDGE ( 'NONE', *, *, #5036, .T. ) ;
#63069=ORIENTED_EDGE ( 'NONE', *, *, #63194, .T. ) ;
#63070=ORIENTED_EDGE ( 'NONE', *, *, #80162, .F. ) ;
#63071=FACE_OUTER_BOUND ( 'NONE', #58542, .T. ) ;
#63072=CARTESIAN_POINT ( 'NONE',  ( 110.8167803534805813, -26.33188723323253910, 245.7889586092439629 ) ) ;
#63077=CARTESIAN_POINT ( 'NONE',  ( 83.56670390244801183, -34.21194715994113267, 219.5838068554169809 ) ) ;
#63078=CARTESIAN_POINT ( 'NONE',  ( 95.23402374720009789, -35.71607800568281021, 36.25848241876794731 ) ) ;
#63079=VERTEX_POINT ( 'NONE', #23128 ) ;
#63080=AXIS2_PLACEMENT_3D ( 'NONE', #28441, #68102, #83418 ) ;
#63082=CYLINDRICAL_SURFACE ( 'NONE', #86266, 11.45913725231036118 ) ;
#63083=CIRCLE ( 'NONE', #81979, 2.517499999999998739 ) ;
#63085=CARTESIAN_POINT ( 'NONE',  ( 97.63766479707265944, -34.12929003103651127, 247.1127681330529811 ) ) ;
#63086=FACE_OUTER_BOUND ( 'NONE', #46442, .T. ) ;
#63087=CARTESIAN_POINT ( 'NONE',  ( 115.9482186066388749, -32.63332544795709111, 100.1699109901959588 ) ) ;
#63088=FACE_OUTER_BOUND ( 'NONE', #84075, .T. ) ;
#63089=CARTESIAN_POINT ( 'NONE',  ( 116.0753558654980822, -32.34106755903779629, 20.18725640462358228 ) ) ;
#63092=ORIENTED_EDGE ( 'NONE', *, *, #86810, .T. ) ;
#63095=CARTESIAN_POINT ( 'NONE',  ( 98.52374054827556904, -34.37364049580116898, 247.5444404487539600 ) ) ;
#63099=VECTOR ( 'NONE', #81559, 1000.000000000000000 ) ;
#63100=CARTESIAN_POINT ( 'NONE',  ( 97.06108120487448332, -37.99646459804690579, 141.4272961276924718 ) ) ;
#63101=VECTOR ( 'NONE', #15000, 1000.000000000000000 ) ;
#63103=ADVANCED_FACE ( 'NONE', ( #29930 ), #85357, .T. ) ;
#63105=DIRECTION ( 'NONE',  ( -1.907762142705490052E-15, -7.167082501179359715E-16, 1.000000000000000000 ) ) ;
#63106=CIRCLE ( 'NONE', #58750, 2.500000000000002220 ) ;
#63107=ORIENTED_EDGE ( 'NONE', *, *, #28568, .F. ) ;
#63108=CARTESIAN_POINT ( 'NONE',  ( 142.0664832912739826, -9.729447159940995959, 14.67562527591100441 ) ) ;
#63110=CARTESIAN_POINT ( 'NONE',  ( 41.56648329127398966, -27.57844715994070484, 258.9256252759120116 ) ) ;
#63111=ORIENTED_EDGE ( 'NONE', *, *, #85672, .T. ) ;
#63112=CARTESIAN_POINT ( 'NONE',  ( 107.1954010100577364, -26.30493706674213428, 35.06705384733893283 ) ) ;
#63114=CARTESIAN_POINT ( 'NONE',  ( 112.3037015629680866, -30.74301476610424544, 287.3214237029247897 ) ) ;
#63117=CARTESIAN_POINT ( 'NONE',  ( 100.4443968677459083, -27.79860430499261881, 185.5841967044829630 ) ) ;
#63118=DIRECTION ( 'NONE',  ( 0.7071067811864683028, 0.7071067811866268427, 7.071067811864676611E-16 ) ) ;
#63119=DIRECTION ( 'NONE',  ( 4.194175870806139918E-14, -1.000000000000000000, 0.000000000000000000 ) ) ;
#63123=CARTESIAN_POINT ( 'NONE',  ( 100.2187443247741783, -45.46477599873944797, 273.0594347997206910 ) ) ;
#63124=CARTESIAN_POINT ( 'NONE',  ( 102.4232139617314061, -45.66021099449668696, 117.1962128419109774 ) ) ;
#63125=EDGE_CURVE ( 'NONE', #20097, #42342, #49205, .T. ) ;
#63126=ORIENTED_EDGE ( 'NONE', *, *, #74133, .T. ) ;
#63127=CARTESIAN_POINT ( 'NONE',  ( 48.45959712129000252, -28.98061976758940617, -5.074374724088000832 ) ) ;
#63128=EDGE_LOOP ( 'NONE', ( #13181, #86840 ) ) ;
#63129=CARTESIAN_POINT ( 'NONE',  ( 108.0381942455320967, -25.67262681319542494, 105.9946728949589811 ) ) ;
#63130=LINE ( 'NONE', #34524, #3294 ) ;
#63131=ORIENTED_EDGE ( 'NONE', *, *, #18924, .F. ) ;
#63132=AXIS2_PLACEMENT_3D ( 'NONE', #54205, #66518, #73786 ) ;
#63136=EDGE_CURVE ( 'NONE', #80351, #914, #86677, .T. ) ;
#63139=CARTESIAN_POINT ( 'NONE',  ( 34.96670390244647564, -26.71338133339322951, 193.9678068554150911 ) ) ;
#63141=DIRECTION ( 'NONE',  ( -4.237773401492740281E-14, 1.000000000000000000, 0.000000000000000000 ) ) ;
#63142=CARTESIAN_POINT ( 'NONE',  ( 105.1635842947561343, -47.00881719185149876, 8.429910990196965770 ) ) ;
#63145=ORIENTED_EDGE ( 'NONE', *, *, #14336, .F. ) ;
#63147=CARTESIAN_POINT ( 'NONE',  ( 182.0667039024480118, -32.29483332968430886, -5.074374724088000832 ) ) ;
#63148=VERTEX_POINT ( 'NONE', #31241 ) ;
#63149=ORIENTED_EDGE ( 'NONE', *, *, #50979, .F. ) ;
#63150=CIRCLE ( 'NONE', #45667, 0.5000000000000004441 ) ;
#63151=CARTESIAN_POINT ( 'NONE',  ( 81.36878785333431097, -21.15209318185135601, 1.893168666203115080 ) ) ;
#63152=CARTESIAN_POINT ( 'NONE',  ( 172.5664832912728457, -18.82844715994071194, 81.92562527591194055 ) ) ;
#63154=CARTESIAN_POINT ( 'NONE',  ( 100.9546144035607540, -28.70706938351655779, 15.59396422068609134 ) ) ;
#63156=CARTESIAN_POINT ( 'NONE',  ( 51.06648329127400388, 25.62155284005901379, 333.4006252759110112 ) ) ;
#63157=CARTESIAN_POINT ( 'NONE',  ( 102.2605585157881194, -43.79055321879850027, 196.5238483995059937 ) ) ;
#63159=CARTESIAN_POINT ( 'NONE',  ( 97.22485937713641135, -31.59570365635885736, 90.93181575210196854 ) ) ;
#63162=ORIENTED_EDGE ( 'NONE', *, *, #12167, .T. ) ;
#63164=ORIENTED_EDGE ( 'NONE', *, *, #62386, .F. ) ;
#63166=ORIENTED_EDGE ( 'NONE', *, *, #52928, .F. ) ;
#63168=DIRECTION ( 'NONE',  ( 1.000000000000000078E-15, 1.000000000000000083E-30, -1.000000000000000000 ) ) ;
#63171=DIRECTION ( 'NONE',  ( 3.999999999999999995E-14, -1.000000000000000000, 4.100000000000000342E-29 ) ) ;
#63172=CIRCLE ( 'NONE', #13891, 2.517500000000005844 ) ;
#63174=CARTESIAN_POINT ( 'NONE',  ( 117.4766623710874853, -37.96092365070988706, 53.73276813305394484 ) ) ;
#63175=VECTOR ( 'NONE', #87338, 1000.000000000000000 ) ;
#63177=B_SPLINE_CURVE_WITH_KNOTS ( 'NONE', 3,
 ( #77796, #23734, #72323, #70989, #2391, #8762, #36463, #64169, #10971, #87728, #3717, #38673, #87289, #59553, #25053, #4615, #81390, #52716 ),
 .UNSPECIFIED., .F., .F.,
 ( 4, 2, 2, 2, 2, 2, 2, 2, 4 ),
 ( 0.000000000000000000, 0.06249849733678987385, 0.1249969946735797477, 0.1874954920103696354, 0.2499939893471594954, 0.3124924866839493554, 0.3749909840207392708, 0.4374894813575291308, 0.4999879786943189908 ),
 .UNSPECIFIED. ) ;
#63178=DIRECTION ( 'NONE',  ( 0.000000000000000000, 1.000000000000000000, 0.000000000000000000 ) ) ;
#63180=CARTESIAN_POINT ( 'NONE',  ( 71.25614885437424562, -84.12815644128085069, 542.9756252759101471 ) ) ;
#63181=DIRECTION ( 'NONE',  ( -0.7071067811734105257, 0.7071067811996846197, 0.000000000000000000 ) ) ;
#63183=AXIS2_PLACEMENT_3D ( 'NONE', #75599, #33803, #6111 ) ;
#63184=DIRECTION ( 'NONE',  ( 4.299999999999999979E-14, -1.000000000000000000, 0.000000000000000000 ) ) ;
#63185=CARTESIAN_POINT ( 'NONE',  ( 108.4174892977290767, -26.73503593456633709, 154.9689586056143469 ) ) ;
#63187=DIRECTION ( 'NONE',  ( 0.000000000000000000, 1.000000000000000000, 0.000000000000000000 ) ) ;
#63188=ADVANCED_FACE ( 'NONE', ( #10797, #37183 ), #52111, .F. ) ;
#63189=CARTESIAN_POINT ( 'NONE',  ( 114.7233776882958409, -44.73301973330935510, 109.1718157521009687 ) ) ;
#63190=DIRECTION ( 'NONE',  ( 0.000000000000000000, -1.000000000000000000, 0.000000000000000000 ) ) ;
#63191=LINE ( 'NONE', #74, #35474 ) ;
#63193=AXIS2_PLACEMENT_3D ( 'NONE', #60842, #80869, #52658 ) ;
#63194=EDGE_CURVE ( 'NONE', #11890, #25046, #54580, .T. ) ;
#63195=ORIENTED_EDGE ( 'NONE', *, *, #56356, .F. ) ;
#63196=VECTOR ( 'NONE', #73573, 1000.000000000000000 ) ;
#63197=CARTESIAN_POINT ( 'NONE',  ( 41.56648329127381203, -18.82844715994071194, 141.9256252759118979 ) ) ;
#63198=CARTESIAN_POINT ( 'NONE',  ( 108.6395843534182291, -26.47938140272626484, 140.9432443235289725 ) ) ;
#63199=CARTESIAN_POINT ( 'NONE',  ( 177.4809174648215730, -48.32844715993478246, 129.9678068554150059 ) ) ;
#63200=ORIENTED_EDGE ( 'NONE', *, *, #16283, .T. ) ;
#63201=CARTESIAN_POINT ( 'NONE',  ( 117.4080659314678314, -35.59792815749688089, 274.9127681330538735 ) ) ;
#63202=DIRECTION ( 'NONE',  ( -0.9068632946707755327, 0.4214249218767993077, 0.000000000000000000 ) ) ;
#63203=DIRECTION ( 'NONE',  ( -0.7071067811864671926, -0.7071067811866279529, -7.071067811864664779E-16 ) ) ;
#63205=AXIS2_PLACEMENT_3D ( 'NONE', #60652, #46118, #26152 ) ;
#63206=FACE_OUTER_BOUND ( 'NONE', #54937, .T. ) ;
#63209=CARTESIAN_POINT ( 'NONE',  ( 114.5468542906243243, -29.54732804739393615, 189.4232443235299570 ) ) ;
#63210=ORIENTED_EDGE ( 'NONE', *, *, #76847, .T. ) ;
#63211=EDGE_LOOP ( 'NONE', ( #73378, #72311, #52696, #33190 ) ) ;
#63213=CARTESIAN_POINT ( 'NONE',  ( 99.32274084468600961, -31.40864097607868999, 162.2911071154209708 ) ) ;
#63215=CARTESIAN_POINT ( 'NONE',  ( 99.72008180067200556, -41.26785689822659009, 8.199678543991950619 ) ) ;
#63218=EDGE_CURVE ( 'NONE', #51167, #34580, #81662, .T. ) ;
#63220=PLANE ( 'NONE',  #27199 ) ;
#63222=CARTESIAN_POINT ( 'NONE',  ( 115.0889047235099270, -30.61763667932959621, 105.3439586093056590 ) ) ;
#63225=CARTESIAN_POINT ( 'NONE',  ( 97.11708974113231818, -41.49110554365062598, 216.6937205140059461 ) ) ;
#63228=ORIENTED_EDGE ( 'NONE', *, *, #25206, .F. ) ;
#63230=CARTESIAN_POINT ( 'NONE',  ( 97.81169818311565223, -40.51742792548894556, 86.63555527419073599 ) ) ;
#63231=CARTESIAN_POINT ( 'NONE',  ( 82.78958961022061658, -19.11755991741142680, 6.789748280180715412 ) ) ;
#63232=FACE_OUTER_BOUND ( 'NONE', #40798, .T. ) ;
#63234=CARTESIAN_POINT ( 'NONE',  ( 98.34688518126465340, -32.29864090244033292, 46.95276813305293473 ) ) ;
#63236=DIRECTION ( 'NONE',  ( -1.000000000000000078E-15, 1.000000000000000083E-30, 1.000000000000000000 ) ) ;
#63237=EDGE_CURVE ( 'NONE', #71729, #22057, #54346, .T. ) ;
#63238=ORIENTED_EDGE ( 'NONE', *, *, #61178, .F. ) ;
#63239=AXIS2_PLACEMENT_3D ( 'NONE', #1440, #43644, #64555 ) ;
#63242=LINE ( 'NONE', #12520, #62741 ) ;
#63244=CARTESIAN_POINT ( 'NONE',  ( 103.0904226585672916, -47.89329182393425555, 252.3041967044823366 ) ) ;
#63246=ADVANCED_FACE ( 'NONE', ( #53902 ), #46650, .T. ) ;
#63247=CARTESIAN_POINT ( 'NONE',  ( 32.09598329127702243, -23.42844715994121785, 313.9678068554150059 ) ) ;
#63248=DIRECTION ( 'NONE',  ( 0.7071067811865475727, -0.7071067811865475727, 0.000000000000000000 ) ) ;
#63249=CARTESIAN_POINT ( 'NONE',  ( 112.4431012073915213, -45.17550776473990481, 168.0275481766957171 ) ) ;
#63250=CARTESIAN_POINT ( 'NONE',  ( 110.8736562448416549, -29.50897902285196039, 57.50809036959092424 ) ) ;
#63251=CARTESIAN_POINT ( 'NONE',  ( 113.6281748933624556, -28.60039662530314430, 160.5356252759109736 ) ) ;
#63252=CARTESIAN_POINT ( 'NONE',  ( 122.7090602494120049, -38.07100823150197755, 293.9356252759109793 ) ) ;
#63255=EDGE_LOOP ( 'NONE', ( #82475, #13569, #83924, #36213 ) ) ;
#63256=ORIENTED_EDGE ( 'NONE', *, *, #8953, .T. ) ;
#63257=DIRECTION ( 'NONE',  ( 4.299999999999999979E-14, -1.000000000000000000, 0.000000000000000000 ) ) ;
#63259=VERTEX_POINT ( 'NONE', #47990 ) ;
#63262=CARTESIAN_POINT ( 'NONE',  ( 108.0295785460986622, -25.31083404586814112, 321.6169501233419510 ) ) ;
#63263=CARTESIAN_POINT ( 'NONE',  ( 111.7654875973913278, -45.22591620450738503, 102.4009912566479557 ) ) ;
#63264=CARTESIAN_POINT ( 'NONE',  ( 115.0717820980658814, -30.01665675799653599, 269.3813395616251682 ) ) ;
#63268=DIRECTION ( 'NONE',  ( -2.999999999999999839E-15, 1.000000000000000000, -2.999999999999999900E-30 ) ) ;
#63269=CARTESIAN_POINT ( 'NONE',  ( 172.5664832912740110, -32.07844715994070839, 18.92562527591200094 ) ) ;
#63270=EDGE_CURVE ( 'NONE', #87561, #16246, #64275, .T. ) ;
#63273=CARTESIAN_POINT ( 'NONE',  ( 100.1408543393098682, -45.42701269980184975, 122.0413395616259606 ) ) ;
#63274=CARTESIAN_POINT ( 'NONE',  ( 109.6949574390794169, -47.51388072328656165, 87.75467289495897205 ) ) ;
#63275=CARTESIAN_POINT ( 'NONE',  ( 108.0181136390867636, -24.86676629934084559, 265.0127681330534415 ) ) ;
#63276=VERTEX_POINT ( 'NONE', #77522 ) ;
#63278=CARTESIAN_POINT ( 'NONE',  ( 101.4045521927434805, -45.52538047655821885, 222.1213395616249784 ) ) ;
#63279=DIRECTION ( 'NONE',  ( 0.02150753337724187197, 0.0009076677972194977960, 0.9997682742251811083 ) ) ;
#63283=CARTESIAN_POINT ( 'NONE',  ( 140.8897065959773727, -8.906223855237593412, 14.92562527591100441 ) ) ;
#63287=DIRECTION ( 'NONE',  ( 0.000000000000000000, -1.000000000000000000, 0.000000000000000000 ) ) ;
#63289=LINE ( 'NONE', #28305, #9675 ) ;
#63290=CARTESIAN_POINT ( 'NONE',  ( 134.0664832912740110, -46.72944715994100306, 4.925625275910997303 ) ) ;
#63291=CARTESIAN_POINT ( 'NONE',  ( 80.54920390244807038, -58.72944715994108833, 207.5838068554169809 ) ) ;
#63292=ORIENTED_EDGE ( 'NONE', *, *, #86417, .T. ) ;
#63293=DIRECTION ( 'NONE',  ( 0.7071067811864886199, 0.7071067811866064146, 7.071067811865191343E-16 ) ) ;
#63294=CARTESIAN_POINT ( 'NONE',  ( 112.6756251843347627, -45.54329372032184153, 263.0270538473394026 ) ) ;
#63295=CARTESIAN_POINT ( 'NONE',  ( 96.60720999893194971, -36.88735532319633847, 132.3384824187679669 ) ) ;
#63296=CARTESIAN_POINT ( 'NONE',  ( 96.66758392153232649, -32.91525239269808623, 17.03467289495896964 ) ) ;
#63297=CIRCLE ( 'NONE', #80680, 3.000000000000002665 ) ;
#63298=DIRECTION ( 'NONE',  ( -0.000000000000000000, 1.000000000000000000, 0.000000000000000000 ) ) ;
#63299=CARTESIAN_POINT ( 'NONE',  ( 156.5667039024483529, -48.82844715993569196, 293.2178068554149490 ) ) ;
#63300=CARTESIAN_POINT ( 'NONE',  ( 81.57739926165420741, -34.43204134599511690, 7.859568798198143469 ) ) ;
#63302=CIRCLE ( 'NONE', #86521, 0.9999999999992039701 ) ;
#63303=ADVANCED_FACE ( 'NONE', ( #55251 ), #84357, .F. ) ;
#63305=AXIS2_PLACEMENT_3D ( 'NONE', #24794, #10271, #79781 ) ;
#63307=ORIENTED_EDGE ( 'NONE', *, *, #66709, .F. ) ;
#63308=DIRECTION ( 'NONE',  ( 0.000000000000000000, 0.000000000000000000, -1.000000000000000000 ) ) ;
#63309=ORIENTED_EDGE ( 'NONE', *, *, #66907, .F. ) ;
#63310=CARTESIAN_POINT ( 'NONE',  ( 105.0150133346707406, -46.21955246553896757, 181.8295626852199689 ) ) ;
#63311=CARTESIAN_POINT ( 'NONE',  ( 131.0667039024480403, -51.22944715994093201, 231.5838068554170093 ) ) ;
#63312=ORIENTED_EDGE ( 'NONE', *, *, #45006, .F. ) ;
#63313=CARTESIAN_POINT ( 'NONE',  ( 107.0664832912739399, -36.72944715994095333, 302.4856252759109907 ) ) ;
#63314=CARTESIAN_POINT ( 'NONE',  ( 95.93334478249057895, -32.74178691125834462, 172.0527681330539735 ) ) ;
#63317=CARTESIAN_POINT ( 'NONE',  ( 97.06063502581739044, -37.99412314152812797, 87.42674140824780693 ) ) ;
#63321=CARTESIAN_POINT ( 'NONE',  ( 103.5913876162975527, -46.49993820617282125, 102.3165776568639700 ) ) ;
#63322=ORIENTED_EDGE ( 'NONE', *, *, #43040, .F. ) ;
#63324=ORIENTED_EDGE ( 'NONE', *, *, #46072, .F. ) ;
#63325=CARTESIAN_POINT ( 'NONE',  ( 99.97388925556708728, -42.04201607304819532, 63.27015473446895300 ) ) ;
#63326=LINE ( 'NONE', #76959, #71872 ) ;
#63327=CARTESIAN_POINT ( 'NONE',  ( 116.6595528204498464, -34.65899032542080960, 179.9956252759109532 ) ) ;
#63328=CARTESIAN_POINT ( 'NONE',  ( 105.7154774160331954, -46.72385840309821248, 37.46895861606181910 ) ) ;
#63329=CARTESIAN_POINT ( 'NONE',  ( 49.16670390244746613, -26.71338133339273924, 237.4678068554150059 ) ) ;
#63330=CARTESIAN_POINT ( 'NONE',  ( 25.56670390244828894, -48.82844715994168183, 293.2178068554150059 ) ) ;
#63331=EDGE_CURVE ( 'NONE', #81923, #61676, #89835, .T. ) ;
#63333=CARTESIAN_POINT ( 'NONE',  ( 32.16397622748866070, -34.03355364506487746, 193.9678068554150911 ) ) ;
#63334=EDGE_CURVE ( 'NONE', #29546, #82906, #15532, .T. ) ;
#63335=CARTESIAN_POINT ( 'NONE',  ( 188.5667039024483245, -42.82844715993430640, 173.2178068554150059 ) ) ;
#63336=CARTESIAN_POINT ( 'NONE',  ( 98.47671751366513604, -30.86049585540210671, 120.8499109901969604 ) ) ;
#63338=EDGE_CURVE ( 'NONE', #2257, #50856, #69527, .T. ) ;
#63339=ORIENTED_EDGE ( 'NONE', *, *, #15906, .F. ) ;
#63340=EDGE_LOOP ( 'NONE', ( #81750, #27553, #14879, #60071 ) ) ;
#63342=PLANE ( 'NONE',  #56274 ) ;
#63343=FACE_BOUND ( 'NONE', #39500, .T. ) ;
#63345=CARTESIAN_POINT ( 'NONE',  ( 114.7326537306653762, -39.53293727251440970, 216.3652332267339773 ) ) ;
#63347=FACE_OUTER_BOUND ( 'NONE', #38676, .T. ) ;
#63348=ORIENTED_EDGE ( 'NONE', *, *, #54046, .T. ) ;
#63349=EDGE_LOOP ( 'NONE', ( #61223, #72977, #50179, #18894 ) ) ;
#63350=ORIENTED_EDGE ( 'NONE', *, *, #7431, .T. ) ;
#63353=ORIENTED_EDGE ( 'NONE', *, *, #39653, .F. ) ;
#63355=CARTESIAN_POINT ( 'NONE',  ( 71.25416588882599456, -72.55705569728901594, 361.9756252759101471 ) ) ;
#63356=CARTESIAN_POINT ( 'NONE',  ( 114.6260888371869555, -31.15012018194425281, 255.7520594963732492 ) ) ;
#63357=DIRECTION ( 'NONE',  ( 1.000000000000000000, 4.237773401492740281E-14, 0.000000000000000000 ) ) ;
#63358=EDGE_LOOP ( 'NONE', ( #79844, #7692, #33589, #57859 ) ) ;
#63360=DIRECTION ( 'NONE',  ( 1.000000000000000078E-15, 1.000000000000000083E-30, -1.000000000000000000 ) ) ;
#63362=VERTEX_POINT ( 'NONE', #76167 ) ;
#63363=EDGE_LOOP ( 'NONE', ( #36300, #64040, #57087, #53365 ) ) ;
#63364=VECTOR ( 'NONE', #47398, 1000.000000000000000 ) ;
#63365=AXIS2_PLACEMENT_3D ( 'NONE', #80445, #40432, #61757 ) ;
#63367=AXIS2_PLACEMENT_3D ( 'NONE', #65678, #36657, #2586 ) ;
#63368=ORIENTED_EDGE ( 'NONE', *, *, #67904, .F. ) ;
#63370=CARTESIAN_POINT ( 'NONE',  ( 116.1392960594047850, -38.67366927644074082, 256.4766617981626382 ) ) ;
#63371=CARTESIAN_POINT ( 'NONE',  ( 114.1902268275144507, -45.21166270573645107, 148.1203871806719405 ) ) ;
#63372=CARTESIAN_POINT ( 'NONE',  ( 98.85726102317293851, -28.21728661942034577, 115.6870538473389587 ) ) ;
#63375=CARTESIAN_POINT ( 'NONE',  ( 99.08600912489498569, -29.96680234772274787, 211.7670538473399517 ) ) ;
#63376=DIRECTION ( 'NONE',  ( 0.000000000000000000, 0.000000000000000000, -1.000000000000000000 ) ) ;
#63378=EDGE_LOOP ( 'NONE', ( #10193, #476, #83567, #1015, #13167, #45214, #52133, #66385 ) ) ;
#63381=ORIENTED_EDGE ( 'NONE', *, *, #4813, .T. ) ;
#63384=EDGE_CURVE ( 'NONE', #61434, #56160, #8486, .T. ) ;
#63385=CARTESIAN_POINT ( 'NONE',  ( 182.3467384525660009, -36.02818131005237490, 193.9678068554150059 ) ) ;
#63388=CARTESIAN_POINT ( 'NONE',  ( 118.9039262414038944, -36.16781539521252142, 118.8641967044819836 ) ) ;
#63389=DIRECTION ( 'NONE',  ( -0.7071067811874389708, 0.7071067811856560636, 0.000000000000000000 ) ) ;
#63390=EDGE_CURVE ( 'NONE', #83770, #20859, #8027, .T. ) ;
#63391=CARTESIAN_POINT ( 'NONE',  ( 107.0664832912739968, -36.72944715994100306, 287.6356252759109680 ) ) ;
#63394=CARTESIAN_POINT ( 'NONE',  ( 163.0664832912739826, -18.82844715994099971, 333.4006252759120343 ) ) ;
#63395=CARTESIAN_POINT ( 'NONE',  ( 110.7254274611715630, -26.32387412717039155, 250.8194347997206819 ) ) ;
#63396=FACE_OUTER_BOUND ( 'NONE', #33082, .T. ) ;
#63398=DIRECTION ( 'NONE',  ( 0.000000000000000000, 0.000000000000000000, 1.000000000000000000 ) ) ;
#63399=CARTESIAN_POINT ( 'NONE',  ( 128.0667039024480118, -48.82844715994099971, 198.9178068554149945 ) ) ;
#63401=PLANE ( 'NONE',  #65128 ) ;
#63402=CARTESIAN_POINT ( 'NONE',  ( 116.3563860081925725, -41.55700552044970664, 288.4441967044822945 ) ) ;
#63403=EDGE_LOOP ( 'NONE', ( #21938, #75713, #6305, #56983 ) ) ;
#63404=CARTESIAN_POINT ( 'NONE',  ( 34.33598329127499227, -36.32844715994100682, 342.9256252759109884 ) ) ;
#63405=CARTESIAN_POINT ( 'NONE',  ( 98.14931896820920088, -31.28605259387051518, 170.8899109901960003 ) ) ;
#63406=CARTESIAN_POINT ( 'NONE',  ( 114.8194029112656551, -43.69900416259703491, 34.24419670448197905 ) ) ;
#63407=CARTESIAN_POINT ( 'NONE',  ( 102.2170635254687454, -46.00716819922848799, 208.1927681330539599 ) ) ;
#63408=CARTESIAN_POINT ( 'NONE',  ( 102.0670548334093581, -27.97049812994907825, 31.48979195403828157 ) ) ;
#63409=CARTESIAN_POINT ( 'NONE',  ( 41.56648329127398966, -27.57844715994070484, 258.9256252759120116 ) ) ;
#63410=FACE_OUTER_BOUND ( 'NONE', #60609, .T. ) ;
#63413=DIRECTION ( 'NONE',  ( 0.0001713722455994027248, -0.9999999853157766072, 0.000000000000000000 ) ) ;
#63414=ORIENTED_EDGE ( 'NONE', *, *, #24380, .T. ) ;
#63415=AXIS2_PLACEMENT_3D ( 'NONE', #86204, #2196, #77600 ) ;
#63418=ORIENTED_EDGE ( 'NONE', *, *, #35434, .T. ) ;
#63420=DIRECTION ( 'NONE',  ( 0.000000000000000000, 0.000000000000000000, -1.000000000000000000 ) ) ;
#63422=CARTESIAN_POINT ( 'NONE',  ( 116.2124334422529870, -31.77159869865918296, 65.22133956162595325 ) ) ;
#63423=CARTESIAN_POINT ( 'NONE',  ( 37.03715912545342093, -48.62818131006128652, 193.9678068554150911 ) ) ;
#63424=CARTESIAN_POINT ( 'NONE',  ( 25.56670390244747892, -48.82844715994178841, 139.7178068554150627 ) ) ;
#63425=CARTESIAN_POINT ( 'NONE',  ( 97.34161151642148013, -42.07962167312376067, 172.7146728949589942 ) ) ;
#63427=AXIS2_PLACEMENT_3D ( 'NONE', #29935, #72159, #78545 ) ;
#63428=CARTESIAN_POINT ( 'NONE',  ( 103.2261711710990824, -45.64430683061108596, 286.6752769709340782 ) ) ;
#63430=EDGE_LOOP ( 'NONE', ( #23932, #12754 ) ) ;
#63431=VERTEX_POINT ( 'NONE', #63898 ) ;
#63432=VECTOR ( 'NONE', #63184, 1000.000000000000000 ) ;
#63433=VECTOR ( 'NONE', #28328, 1000.000000000000000 ) ;
#63435=CARTESIAN_POINT ( 'NONE',  ( 108.3334480986085708, -46.73485935347873976, 107.6772919428708946 ) ) ;
#63436=PLANE ( 'NONE',  #57977 ) ;
#63438=CARTESIAN_POINT ( 'NONE',  ( 115.8254323916879258, -31.73001882819412245, 74.23979194262673786 ) ) ;
#63442=DIRECTION ( 'NONE',  ( 4.299999999999999979E-14, -1.000000000000000000, 4.400000000000000367E-29 ) ) ;
#63443=CARTESIAN_POINT ( 'NONE',  ( 97.81168895331671820, -40.51742574516950413, 11.63562527591094309 ) ) ;
#63444=ADVANCED_FACE ( 'NONE', ( #84800 ), #71167, .F. ) ;
#63446=VERTEX_POINT ( 'NONE', #8942 ) ;
#63448=CARTESIAN_POINT ( 'NONE',  ( 97.81186544543886896, -40.51730612966257183, 271.6361395295153898 ) ) ;
#63449=VECTOR ( 'NONE', #89417, 1000.000000000000000 ) ;
#63450=DIRECTION ( 'NONE',  ( 0.000000000000000000, 1.000000000000000000, 0.000000000000000000 ) ) ;
#63451=CARTESIAN_POINT ( 'NONE',  ( 113.4406056323916090, -42.58363279299825876, 76.04142370292498754 ) ) ;
#63452=VECTOR ( 'NONE', #7081, 1000.000000000000000 ) ;
#63453=CARTESIAN_POINT ( 'NONE',  ( 71.25416588882599456, -72.55705569728901594, 361.9756252759101471 ) ) ;
#63454=CARTESIAN_POINT ( 'NONE',  ( 73.06670390244801183, -50.82844715994100682, 310.9178068554150514 ) ) ;
#63458=CARTESIAN_POINT ( 'NONE',  ( 182.5667039024480118, -32.29483332968450782, -5.074374724088000832 ) ) ;
#63459=VERTEX_POINT ( 'NONE', #55687 ) ;
#63460=ORIENTED_EDGE ( 'NONE', *, *, #35940, .T. ) ;
#63461=ADVANCED_FACE ( 'NONE', ( #28010 ), #57511, .T. ) ;
#63462=CARTESIAN_POINT ( 'NONE',  ( 116.0040243724562146, -33.83170925634997417, 130.5196785439929670 ) ) ;
#63463=CARTESIAN_POINT ( 'NONE',  ( 107.0664832912739541, -36.72944715994095333, 308.7195067599733420 ) ) ;
#63464=CARTESIAN_POINT ( 'NONE',  ( 113.3277443033378376, -28.32255675095946046, 100.5670538473389684 ) ) ;
#63465=CIRCLE ( 'NONE', #22831, 4.749999999999976907 ) ;
#63468=VERTEX_POINT ( 'NONE', #86573 ) ;
#63469=ORIENTED_EDGE ( 'NONE', *, *, #57788, .T. ) ;
#63470=CYLINDRICAL_SURFACE ( 'NONE', #36855, 9.999999999999998224 ) ;
#63471=ORIENTED_EDGE ( 'NONE', *, *, #71546, .T. ) ;
#63472=CARTESIAN_POINT ( 'NONE',  ( 116.1393041698828057, -43.00708073170995505, 13.35657765686298859 ) ) ;
#63473=CARTESIAN_POINT ( 'NONE',  ( 113.6278897941700876, -45.65318799257786964, 179.0689586092439640 ) ) ;
#63476=CARTESIAN_POINT ( 'NONE',  ( 97.93258204476157402, -31.63109636822184711, 106.9213395616259703 ) ) ;
#63477=CARTESIAN_POINT ( 'NONE',  ( 106.5394234437989667, -24.24056378642895737, 322.0356252759110021 ) ) ;
#63479=CARTESIAN_POINT ( 'NONE',  ( 98.34954239462810222, -31.65711219339656424, 115.9083548605937750 ) ) ;
#63481=ORIENTED_EDGE ( 'NONE', *, *, #2228, .F. ) ;
#63482=CARTESIAN_POINT ( 'NONE',  ( 105.7157523590067854, -46.72390646314000406, 133.4701676439947278 ) ) ;
#63484=EDGE_LOOP ( 'NONE', ( #77089, #48871, #75299, #33559, #33838 ) ) ;
#63487=CIRCLE ( 'NONE', #89632, 27.99999999999999645 ) ;
#63489=CARTESIAN_POINT ( 'NONE',  ( 116.4746376734894255, -32.23794665461475972, 19.18133956162493092 ) ) ;
#63492=DIRECTION ( 'NONE',  ( 1.000000000000000000, 0.000000000000000000, 0.000000000000000000 ) ) ;
#63494=CARTESIAN_POINT ( 'NONE',  ( 96.85055626654745708, -38.51091292166576352, 46.45181575210194325 ) ) ;
#63495=CARTESIAN_POINT ( 'NONE',  ( 106.5131950068454216, -24.24167068730766417, 320.8164078654934315 ) ) ;
#63496=CARTESIAN_POINT ( 'NONE',  ( 102.3226935662337524, -26.77152163616663927, 136.4422919425779526 ) ) ;
#63497=CARTESIAN_POINT ( 'NONE',  ( 102.0670549536967400, -27.97049806286341322, 71.48979194315724328 ) ) ;
#63500=DIRECTION ( 'NONE',  ( 0.000000000000000000, 0.000000000000000000, 1.000000000000000000 ) ) ;
#63503=AXIS2_PLACEMENT_3D ( 'NONE', #10431, #3179, #45812 ) ;
#63504=CARTESIAN_POINT ( 'NONE',  ( 37.03715912545433042, -48.62818131006122258, 249.9678068554150343 ) ) ;
#63505=CARTESIAN_POINT ( 'NONE',  ( 107.5678864575881590, -47.81824684668375625, 192.6003871806729535 ) ) ;
#63506=VERTEX_POINT ( 'NONE', #72494 ) ;
#63507=DIRECTION ( 'NONE',  ( 1.000000000000000000, 4.299999999999999979E-14, 1.000000000000000078E-15 ) ) ;
#63508=CARTESIAN_POINT ( 'NONE',  ( 103.2957022058525780, -26.98683617215391806, 211.3699109901969848 ) ) ;
#63509=CARTESIAN_POINT ( 'NONE',  ( 114.5987772146603731, -44.05082428708011832, 94.21276813305395592 ) ) ;
#63510=CIRCLE ( 'NONE', #18500, 1.000000000000000888 ) ;
#63512=VECTOR ( 'NONE', #55196, 1000.000000000000000 ) ;
#63513=CARTESIAN_POINT ( 'NONE',  ( 172.5664832912729878, -27.82844715994070484, 195.9256252759119832 ) ) ;
#63515=ORIENTED_EDGE ( 'NONE', *, *, #49663, .F. ) ;
#63517=EDGE_CURVE ( 'NONE', #73802, #3245, #47772, .T. ) ;
#63519=EDGE_CURVE ( 'NONE', #976, #65985, #36197, .T. ) ;
#63522=EDGE_CURVE ( 'NONE', #12659, #34867, #64782, .T. ) ;
#63523=ORIENTED_EDGE ( 'NONE', *, *, #474, .F. ) ;
#63525=CARTESIAN_POINT ( 'NONE',  ( 118.0816017896457453, -32.35888884030432422, 245.1270538473389706 ) ) ;
#63526=DIRECTION ( 'NONE',  ( 0.000000000000000000, 0.000000000000000000, -1.000000000000000000 ) ) ;
#63527=DIRECTION ( 'NONE',  ( 0.000000000000000000, 0.000000000000000000, -1.000000000000000000 ) ) ;
#63533=CARTESIAN_POINT ( 'NONE',  ( 97.05407301568530443, -33.74649485729950271, 31.09562527591097592 ) ) ;
#63538=CARTESIAN_POINT ( 'NONE',  ( 33.96670390244699433, -28.27351298637401200, 342.9256252759119548 ) ) ;
#63539=CARTESIAN_POINT ( 'NONE',  ( 97.31298885056827430, -38.96024362731790802, 17.50578975050363439 ) ) ;
#63540=EDGE_CURVE ( 'NONE', #25358, #8047, #43657, .T. ) ;
#63541=CARTESIAN_POINT ( 'NONE',  ( 111.2075884809769803, -27.22220029719803591, 280.7375300378151337 ) ) ;
#63542=CARTESIAN_POINT ( 'NONE',  ( 20.03715912545735378, -24.42818131006189830, 249.9678068554150059 ) ) ;
#63543=CARTESIAN_POINT ( 'NONE',  ( 114.2351621074132026, -44.22269940884944361, 109.1718157521009687 ) ) ;
#63545=EDGE_CURVE ( 'NONE', #27744, #62140, #24342, .T. ) ;
#63548=CYLINDRICAL_SURFACE ( 'NONE', #16750, 4.875000000000017764 ) ;
#63549=VECTOR ( 'NONE', #59000, 1000.000000000000000 ) ;
#63550=ORIENTED_EDGE ( 'NONE', *, *, #3499, .F. ) ;
#63551=ORIENTED_EDGE ( 'NONE', *, *, #39242, .F. ) ;
#63553=CARTESIAN_POINT ( 'NONE',  ( 103.6867908865108916, -46.21882986916993730, 248.7358690201829745 ) ) ;
#63555=CARTESIAN_POINT ( 'NONE',  ( 116.3232968930447839, -32.93863405887816498, 194.1356252759109680 ) ) ;
#63556=AXIS2_PLACEMENT_3D ( 'NONE', #61267, #12691, #19946 ) ;
#63558=DIRECTION ( 'NONE',  ( 0.8543009526837940237, 0.03605348183280988883, -0.5185267868599396923 ) ) ;
#63560=EDGE_LOOP ( 'NONE', ( #20191, #10314, #8178, #8300 ) ) ;
#63561=CYLINDRICAL_SURFACE ( 'NONE', #30526, 3.299999999999997158 ) ;
#63562=EDGE_CURVE ( 'NONE', #24002, #49561, #18803, .T. ) ;
#63563=DIRECTION ( 'NONE',  ( 0.000000000000000000, 1.000000000000000000, 0.000000000000000000 ) ) ;
#63564=EDGE_LOOP ( 'NONE', ( #35919, #20694, #75659, #59231 ) ) ;
#63565=CARTESIAN_POINT ( 'NONE',  ( 106.9273489086460387, -26.26968863985776537, 60.08705384733897858 ) ) ;
#63568=CARTESIAN_POINT ( 'NONE',  ( 102.4109068130577356, -29.56832019646944687, 24.95813411379099733 ) ) ;
#63570=VECTOR ( 'NONE', #35158, 1000.000000000000000 ) ;
#63571=CARTESIAN_POINT ( 'NONE',  ( 116.7956373554045939, -39.38598825398587877, 128.6149081173567765 ) ) ;
#63572=CARTESIAN_POINT ( 'NONE',  ( 109.6835627966675162, -27.30531164764922991, 174.8613395616259822 ) ) ;
#63573=CARTESIAN_POINT ( 'NONE',  ( 80.06648329127402519, -46.72944715994105991, 10.72562527591094295 ) ) ;
#63579=CARTESIAN_POINT ( 'NONE',  ( 156.5667039024482108, -48.82844715993569196, 295.7178068554149490 ) ) ;
#63580=CARTESIAN_POINT ( 'NONE',  ( 96.87194279380025819, -34.19777600025749109, 272.1327681330539576 ) ) ;
#63581=CARTESIAN_POINT ( 'NONE',  ( 97.80792351950141494, -40.51905676813210988, 116.6359120812046939 ) ) ;
#63582=VERTEX_POINT ( 'NONE', #35554 ) ;
#63583=CARTESIAN_POINT ( 'NONE',  ( 136.8105871997951226, -36.91414947189760909, 6.758631288823576888 ) ) ;
#63584=VERTEX_POINT ( 'NONE', #70084 ) ;
#63585=CARTESIAN_POINT ( 'NONE',  ( 117.4068710881028323, -38.36326476267787200, 109.7013395616249767 ) ) ;
#63587=ORIENTED_EDGE ( 'NONE', *, *, #9850, .F. ) ;
#63588=ORIENTED_EDGE ( 'NONE', *, *, #15684, .T. ) ;
#63590=AXIS2_PLACEMENT_3D ( 'NONE', #5963, #34542, #75446 ) ;
#63591=DIRECTION ( 'NONE',  ( 0.000000000000000000, 0.000000000000000000, -1.000000000000000000 ) ) ;
#63592=CARTESIAN_POINT ( 'NONE',  ( 100.9546836996216825, -28.70701758901807210, 266.5939575379834423 ) ) ;
#63593=DIRECTION ( 'NONE',  ( 0.000000000000000000, 0.000000000000000000, 1.000000000000000000 ) ) ;
#63595=CYLINDRICAL_SURFACE ( 'NONE', #27283, 12.99999999999999822 ) ;
#63596=CARTESIAN_POINT ( 'NONE',  ( 111.1289525437170056, -47.00905435842401658, 18.88800622829195319 ) ) ;
#63597=CARTESIAN_POINT ( 'NONE',  ( 180.2143765759489895, -35.91149509761070391, -5.074374724088000832 ) ) ;
#63598=VERTEX_POINT ( 'NONE', #43710 ) ;
#63599=DIRECTION ( 'NONE',  ( 0.000000000000000000, 0.000000000000000000, -1.000000000000000000 ) ) ;
#63600=AXIS2_PLACEMENT_3D ( 'NONE', #5937, #75419, #54034 ) ;
#63602=VERTEX_POINT ( 'NONE', #9213 ) ;
#63603=VECTOR ( 'NONE', #76499, 1000.000000000000000 ) ;
#63605=CYLINDRICAL_SURFACE ( 'NONE', #59020, 3.300000000000000711 ) ;
#63606=CARTESIAN_POINT ( 'NONE',  ( 116.3191307872214821, -32.94748812527954840, 115.1356252759109822 ) ) ;
#63608=DIRECTION ( 'NONE',  ( 1.000000000000000000, 0.000000000000000000, 0.000000000000000000 ) ) ;
#63609=DIRECTION ( 'NONE',  ( 0.000000000000000000, 0.000000000000000000, -1.000000000000000000 ) ) ;
#63610=CARTESIAN_POINT ( 'NONE',  ( 108.3843752505750331, -28.29029480288096465, 189.3752769709339816 ) ) ;
#63611=CARTESIAN_POINT ( 'NONE',  ( 62.03715912545838762, -47.82818131006021645, 249.9678068554150343 ) ) ;
#63613=CARTESIAN_POINT ( 'NONE',  ( 103.2628093650484828, -47.15753175352042348, 97.28610146638693834 ) ) ;
#63614=EDGE_LOOP ( 'NONE', ( #79342, #5823, #29765, #20017 ) ) ;
#63615=CARTESIAN_POINT ( 'NONE',  ( 107.0664832912739399, -36.72944715994095333, 311.6356252759109680 ) ) ;
#63616=ORIENTED_EDGE ( 'NONE', *, *, #2457, .T. ) ;
#63617=CARTESIAN_POINT ( 'NONE',  ( 97.33710672311610779, -34.07376039389686184, 277.1149365882106963 ) ) ;
#63620=VERTEX_POINT ( 'NONE', #50528 ) ;
#63621=CARTESIAN_POINT ( 'NONE',  ( 188.5667039024479834, -67.87844715994100397, 262.0928068554150059 ) ) ;
#63623=AXIS2_PLACEMENT_3D ( 'NONE', #74583, #68229, #67771 ) ;
#63626=VECTOR ( 'NONE', #79114, 1000.000000000000000 ) ;
#63627=CARTESIAN_POINT ( 'NONE',  ( 103.8344565422589767, -46.70152647745319996, 82.32705384733995402 ) ) ;
#63629=CARTESIAN_POINT ( 'NONE',  ( 100.9542232131455108, -28.70737172392434644, 165.5940040971896963 ) ) ;
#63632=EDGE_CURVE ( 'NONE', #70197, #39210, #85080, .T. ) ;
#63633=CARTESIAN_POINT ( 'NONE',  ( 116.7951252696762623, -39.38782979722077471, 143.6147919419995844 ) ) ;
#63634=ORIENTED_EDGE ( 'NONE', *, *, #39846, .F. ) ;
#63635=CIRCLE ( 'NONE', #73806, 4.749999999999976907 ) ;
#63636=ADVANCED_FACE ( 'NONE', ( #56439 ), #70543, .F. ) ;
#63638=CARTESIAN_POINT ( 'NONE',  ( 102.0670550253074822, -27.97049802292532306, 155.4897919366790404 ) ) ;
#63639=AXIS2_PLACEMENT_3D ( 'NONE', #12383, #54130, #4677 ) ;
#63641=ADVANCED_FACE ( 'NONE', ( #78269 ), #1046, .F. ) ;
#63642=CARTESIAN_POINT ( 'NONE',  ( 97.91349202876114077, -31.62044072442156306, 106.9213395616259703 ) ) ;
#63647=EDGE_CURVE ( 'NONE', #73852, #9110, #7217, .T. ) ;
#63648=ORIENTED_EDGE ( 'NONE', *, *, #60839, .F. ) ;
#63649=CARTESIAN_POINT ( 'NONE',  ( 86.06670390244796920, -58.72944715994110254, 310.9178068554150514 ) ) ;
#63651=CARTESIAN_POINT ( 'NONE',  ( 108.5509251780138129, -26.47246927008498929, 145.9737205140059473 ) ) ;
#63652=CIRCLE ( 'NONE', #40423, 4.749999999999976907 ) ;
#63655=CARTESIAN_POINT ( 'NONE',  ( 98.07879728544668296, -32.87107120142745487, 12.00419670448193976 ) ) ;
#63656=PLANE ( 'NONE',  #86091 ) ;
#63657=CARTESIAN_POINT ( 'NONE',  ( 62.03742497533654188, -23.42844715994041493, 180.4678068554151196 ) ) ;
#63659=DIRECTION ( 'NONE',  ( 1.000000000000000000, 1.387778780781444413E-14, 0.000000000000000000 ) ) ;
#63661=CARTESIAN_POINT ( 'NONE',  ( 152.0371591254582881, -47.82818131005588214, 313.9678068554149490 ) ) ;
#63662=CYLINDRICAL_SURFACE ( 'NONE', #84985, 9.999999999999998224 ) ;
#63663=CARTESIAN_POINT ( 'NONE',  ( 97.41213207386795148, -40.51524797426110069, 246.6118157521019896 ) ) ;
#63664=EDGE_LOOP ( 'NONE', ( #48462, #17520, #46192, #74807 ) ) ;
#63665=VERTEX_POINT ( 'NONE', #50073 ) ;
#63666=VECTOR ( 'NONE', #48659, 1000.000000000000000 ) ;
#63667=EDGE_CURVE ( 'NONE', #6135, #3336, #43258, .T. ) ;
#63668=CARTESIAN_POINT ( 'NONE',  ( 98.21222678671237816, -37.09057735734792516, 157.7901547344689845 ) ) ;
#63670=CARTESIAN_POINT ( 'NONE',  ( 106.3742716537777113, -27.86474340539431793, 21.57015473446893949 ) ) ;
#63671=DIRECTION ( 'NONE',  ( 0.9999999853157766072, 0.0001713722455994998422, -0.000000000000000000 ) ) ;
#63672=CARTESIAN_POINT ( 'NONE',  ( 33.96670390244699433, -28.27351298637401200, -5.074374724088000832 ) ) ;
#63674=DIRECTION ( 'NONE',  ( 2.900000000000000265E-14, -2.000000000000000155E-15, 1.000000000000000000 ) ) ;
#63676=CARTESIAN_POINT ( 'NONE',  ( 104.1918496689534948, -26.69446299336401296, 225.2984824187679749 ) ) ;
#63678=ORIENTED_EDGE ( 'NONE', *, *, #5222, .T. ) ;
#63679=ORIENTED_EDGE ( 'NONE', *, *, #41167, .T. ) ;
#63680=EDGE_CURVE ( 'NONE', #44764, #36112, #71028, .T. ) ;
#63681=VECTOR ( 'NONE', #74565, 1000.000000000000000 ) ;
#63684=CARTESIAN_POINT ( 'NONE',  ( 172.5664832912740110, -18.82844715994099971, 138.9256252759119832 ) ) ;
#63687=CARTESIAN_POINT ( 'NONE',  ( 111.0600676159102278, -27.80113716328034457, 20.74133956162494030 ) ) ;
#63691=ORIENTED_EDGE ( 'NONE', *, *, #35262, .F. ) ;
#63692=CARTESIAN_POINT ( 'NONE',  ( 105.1556394555663445, -47.05180815895162993, 8.429910990196965770 ) ) ;
#63693=CARTESIAN_POINT ( 'NONE',  ( 51.06648329127400388, -0.2185775633790978945, 333.4006252759120343 ) ) ;
#63694=CARTESIAN_POINT ( 'NONE',  ( 118.6541713771196527, -39.21258442193070692, 258.6584824187679033 ) ) ;
#63695=ORIENTED_EDGE ( 'NONE', *, *, #81332, .F. ) ;
#63697=CARTESIAN_POINT ( 'NONE',  ( 77.31648329127401098, -36.72944715994107412, 6.749768910606400496 ) ) ;
#63698=CARTESIAN_POINT ( 'NONE',  ( 172.5664832912729878, -27.82844715994070484, 258.9256252759120116 ) ) ;
#63699=CARTESIAN_POINT ( 'NONE',  ( 163.5667039024460223, -18.82844715994099971, -5.074374724088000832 ) ) ;
#63700=CARTESIAN_POINT ( 'NONE',  ( 100.2074232480821365, -30.48050913114499849, 78.55666179816195438 ) ) ;
#63702=CARTESIAN_POINT ( 'NONE',  ( 116.3696522983621549, -44.11004992080503229, 194.2927681330539542 ) ) ;
#63707=EDGE_LOOP ( 'NONE', ( #40568, #52872 ) ) ;
#63710=DIRECTION ( 'NONE',  ( 1.000000000000000078E-15, -1.000000000000000083E-30, -1.000000000000000000 ) ) ;
#63712=ORIENTED_EDGE ( 'NONE', *, *, #54670, .F. ) ;
#63714=DIRECTION ( 'NONE',  ( 1.000000000000000000, 4.163336342344333240E-14, 0.000000000000000000 ) ) ;
#63716=CARTESIAN_POINT ( 'NONE',  ( 107.2022627278996652, -27.67438038655213006, 79.49908649474396327 ) ) ;
#63717=CARTESIAN_POINT ( 'NONE',  ( 116.3368571269942464, -41.54685706111320087, 288.4441967044822945 ) ) ;
#63721=ORIENTED_EDGE ( 'NONE', *, *, #8686, .T. ) ;
#63726=VECTOR ( 'NONE', #77086, 1000.000000000000000 ) ;
#63727=EDGE_CURVE ( 'NONE', #84681, #64226, #35102, .T. ) ;
#63728=CARTESIAN_POINT ( 'NONE',  ( 102.5967720069230324, -27.99243076246517603, 120.4527681330539792 ) ) ;
#63729=CARTESIAN_POINT ( 'NONE',  ( 103.1890357985451345, -46.49249970849451330, 117.2756252759109543 ) ) ;
#63730=CARTESIAN_POINT ( 'NONE',  ( 118.3887371170988132, -33.06383674033636311, 284.0756252759109657 ) ) ;
#63731=EDGE_LOOP ( 'NONE', ( #37525, #35184, #28909, #64535 ) ) ;
#63732=CARTESIAN_POINT ( 'NONE',  ( 96.77253738264830929, -34.86918258059447595, 241.1841967044819626 ) ) ;
#63733=FACE_OUTER_BOUND ( 'NONE', #16919, .T. ) ;
#63734=CARTESIAN_POINT ( 'NONE',  ( 172.5664832912740110, 0.2215528400590013880, 198.9256252759119832 ) ) ;
#63735=DIRECTION ( 'NONE',  ( -1.000000000000000078E-15, 1.000000000000000083E-30, 1.000000000000000000 ) ) ;
#63738=DIRECTION ( 'NONE',  ( 0.000000000000000000, 0.000000000000000000, -1.000000000000000000 ) ) ;
#63739=CARTESIAN_POINT ( 'NONE',  ( 105.0911950360329712, -25.44184036110743108, 322.1652889949337464 ) ) ;
#63740=EDGE_CURVE ( 'NONE', #72479, #59669, #81725, .T. ) ;
#63741=CARTESIAN_POINT ( 'NONE',  ( 31.56670390244700641, -19.82844715994111340, -5.074374724088000832 ) ) ;
#63742=CARTESIAN_POINT ( 'NONE',  ( 132.2449836194497550, -38.78962918510080016, 7.677444906558990922 ) ) ;
#63743=EDGE_CURVE ( 'NONE', #26589, #87561, #73909, .T. ) ;
#63745=CARTESIAN_POINT ( 'NONE',  ( 62.03742497533745137, -23.42844715994041849, 313.9678068554150059 ) ) ;
#63747=CARTESIAN_POINT ( 'NONE',  ( 83.56670390244798341, -34.21194715994108293, 229.5838068554169524 ) ) ;
#63748=VERTEX_POINT ( 'NONE', #374 ) ;
#63749=CIRCLE ( 'NONE', #2803, 0.3000000000000062617 ) ;
#63750=EDGE_CURVE ( 'NONE', #1770, #20391, #41688, .T. ) ;
#63752=CARTESIAN_POINT ( 'NONE',  ( 117.5128880048294491, -35.85709896013243281, 253.8927681330537780 ) ) ;
#63753=CARTESIAN_POINT ( 'NONE',  ( 102.0510343613854189, -46.57928231165939081, 168.2137205140059564 ) ) ;
#63754=CARTESIAN_POINT ( 'NONE',  ( 112.1919128969917097, -27.58564230820396190, 30.66991099019694644 ) ) ;
#63755=DIRECTION ( 'NONE',  ( 1.000000000000000078E-15, -1.000000000000000083E-30, -1.000000000000000000 ) ) ;
#63756=CARTESIAN_POINT ( 'NONE',  ( 98.30753419281403183, -41.72887549490040726, 46.73979194292225969 ) ) ;
#63757=CARTESIAN_POINT ( 'NONE',  ( 98.38051519723421734, -41.69543662888409585, 137.7397802884137263 ) ) ;
#63759=VECTOR ( 'NONE', #18775, 1000.000000000000000 ) ;
#63760=ADVANCED_FACE ( 'NONE', ( #89881 ), #43435, .F. ) ;
#63761=ORIENTED_EDGE ( 'NONE', *, *, #37486, .T. ) ;
#63762=CARTESIAN_POINT ( 'NONE',  ( 138.0667039024480971, -58.72944715994091069, 199.5838068554170093 ) ) ;
#63763=ORIENTED_EDGE ( 'NONE', *, *, #48011, .T. ) ;
#63765=CARTESIAN_POINT ( 'NONE',  ( 103.6069473157389922, -44.53891209398362605, 176.6667055423629620 ) ) ;
#63766=AXIS2_PLACEMENT_3D ( 'NONE', #50848, #43576, #58544 ) ;
#63767=DIRECTION ( 'NONE',  ( -1.000000000000000000, -2.756263715554006823E-15, 0.000000000000000000 ) ) ;
#63769=DIRECTION ( 'NONE',  ( 0.000000000000000000, 0.000000000000000000, 1.000000000000000000 ) ) ;
#63770=CARTESIAN_POINT ( 'NONE',  ( 117.7567108552514128, -34.01230579303181401, 165.0365776568629315 ) ) ;
#63773=CARTESIAN_POINT ( 'NONE',  ( 97.06105435396277414, -37.99632269549143615, 151.4278191669818057 ) ) ;
#63774=CARTESIAN_POINT ( 'NONE',  ( 109.7015479400130999, -27.07733610322067008, 85.86488799970449293 ) ) ;
#63777=CIRCLE ( 'NONE', #89916, 4.749999999999976907 ) ;
#63778=CARTESIAN_POINT ( 'NONE',  ( 98.70071965984708129, -42.85747980491203180, 106.8175300378169652 ) ) ;
#63779=ORIENTED_EDGE ( 'NONE', *, *, #26904, .T. ) ;
#63780=ORIENTED_EDGE ( 'NONE', *, *, #77805, .T. ) ;
#63781=VERTEX_POINT ( 'NONE', #5409 ) ;
#63782=CARTESIAN_POINT ( 'NONE',  ( 114.8570798905637673, -32.50631050113013742, 65.65301187732598009 ) ) ;
#63784=CARTESIAN_POINT ( 'NONE',  ( 103.8504807240353500, -26.87063827031099450, 206.3394347997199816 ) ) ;
#63787=DIRECTION ( 'NONE',  ( 0.000000000000000000, 0.000000000000000000, -1.000000000000000000 ) ) ;
#63788=CIRCLE ( 'NONE', #78326, 0.5000000000000004441 ) ;
#63790=LINE ( 'NONE', #70147, #76757 ) ;
#63792=CARTESIAN_POINT ( 'NONE',  ( 117.8527506973083518, -39.03601561205234560, 108.6708633711489824 ) ) ;
#63793=VERTEX_POINT ( 'NONE', #27632 ) ;
#63794=ORIENTED_EDGE ( 'NONE', *, *, #39326, .F. ) ;
#63798=LINE ( 'NONE', #7489, #18928 ) ;
#63800=ADVANCED_FACE ( 'NONE', ( #61689 ), #33548, .F. ) ;
#63801=CARTESIAN_POINT ( 'NONE',  ( 106.4678557813946043, -44.87017016969328864, 220.3366617981629645 ) ) ;
#63803=CYLINDRICAL_SURFACE ( 'NONE', #1557, 1.000000000000000888 ) ;
#63804=CARTESIAN_POINT ( 'NONE',  ( 98.28068559441094010, -31.05177188324158166, 145.8699109901969848 ) ) ;
#63805=DIRECTION ( 'NONE',  ( -0.9254794337955620787, -0.3787978585227822492, 0.000000000000000000 ) ) ;
#63808=ORIENTED_EDGE ( 'NONE', *, *, #87411, .F. ) ;
#63811=EDGE_LOOP ( 'NONE', ( #38529, #29037, #49813, #50961 ) ) ;
#63812=ORIENTED_EDGE ( 'NONE', *, *, #12068, .F. ) ;
#63813=CARTESIAN_POINT ( 'NONE',  ( 78.49243652282237349, -20.98954602991689455, 7.829737527532317998 ) ) ;
#63815=CARTESIAN_POINT ( 'NONE',  ( 114.0241607691103809, -31.19294522270855907, 240.7930118773259665 ) ) ;
#63817=CARTESIAN_POINT ( 'NONE',  ( 142.8698897858160706, -0.9167816978817300289, 542.9756252759101471 ) ) ;
#63818=EDGE_LOOP ( 'NONE', ( #59813, #41609, #14086, #9514 ) ) ;
#63819=CARTESIAN_POINT ( 'NONE',  ( 100.5082931581247152, -41.41740168340257355, 9.635625275910943088 ) ) ;
#63820=CARTESIAN_POINT ( 'NONE',  ( 25.56670390244748248, -48.82844715994178841, 137.2178068554150627 ) ) ;
#63822=AXIS2_PLACEMENT_3D ( 'NONE', #35553, #63268, #1044 ) ;
#63823=EDGE_LOOP ( 'NONE', ( #89371, #2562, #4378 ) ) ;
#63826=ORIENTED_EDGE ( 'NONE', *, *, #78443, .F. ) ;
#63828=CARTESIAN_POINT ( 'NONE',  ( 110.7250417795893611, -29.43255185136001728, 277.5252332267342581 ) ) ;
#63829=VECTOR ( 'NONE', #2825, 1000.000000000000000 ) ;
#63830=CARTESIAN_POINT ( 'NONE',  ( 112.7922847239315161, -45.46795744031502551, 178.0384824187679556 ) ) ;
#63831=CARTESIAN_POINT ( 'NONE',  ( 112.7897778137182030, -47.07797880090547693, 102.9784824187679817 ) ) ;
#63833=DIRECTION ( 'NONE',  ( 1.000000000000000078E-15, 1.000000000000000083E-30, -1.000000000000000000 ) ) ;
#63835=CARTESIAN_POINT ( 'NONE',  ( 106.8516137164961464, -47.78059241960190207, 223.5489586092439538 ) ) ;
#63837=DIRECTION ( 'NONE',  ( -1.000000000000000078E-15, 1.000000000000000083E-30, 1.000000000000000000 ) ) ;
#63839=LINE ( 'NONE', #1619, #59831 ) ;
#63841=ORIENTED_EDGE ( 'NONE', *, *, #3738, .F. ) ;
#63842=AXIS2_PLACEMENT_3D ( 'NONE', #80836, #4963, #73102 ) ;
#63843=CARTESIAN_POINT ( 'NONE',  ( 118.9274366748948069, -37.70237179777471681, 188.7613395616259595 ) ) ;
#63844=EDGE_LOOP ( 'NONE', ( #64601, #84265, #41836, #55144 ) ) ;
#63845=CARTESIAN_POINT ( 'NONE',  ( 117.2096823498778662, -39.28706705594211712, 123.6299109901969615 ) ) ;
#63846=CARTESIAN_POINT ( 'NONE',  ( 97.33812887613856901, -34.06989601086925745, 256.1147306920630058 ) ) ;
#63848=DIRECTION ( 'NONE',  ( 0.000000000000000000, -1.000000000000000000, 0.000000000000000000 ) ) ;
#63850=DIRECTION ( 'NONE',  ( -0.000000000000000000, 0.000000000000000000, -1.000000000000000000 ) ) ;
#63851=CARTESIAN_POINT ( 'NONE',  ( 118.0177608886752836, -35.41288285714062312, 234.9337205140059552 ) ) ;
#63853=ADVANCED_FACE ( 'NONE', ( #20823 ), #69423, .T. ) ;
#63856=DIRECTION ( 'NONE',  ( 0.000000000000000000, 0.000000000000000000, -1.000000000000000000 ) ) ;
#63857=ADVANCED_FACE ( 'NONE', ( #8091 ), #14915, .T. ) ;
#63858=DIRECTION ( 'NONE',  ( -0.9963424814100679816, 0.08544974978095724871, 0.000000000000000000 ) ) ;
#63859=EDGE_CURVE ( 'NONE', #19807, #75042, #16481, .T. ) ;
#63860=CARTESIAN_POINT ( 'NONE',  ( 116.3259296754763028, -32.93870509136930025, 260.1356252759109680 ) ) ;
#63862=DIRECTION ( 'NONE',  ( -0.02150753337724187197, -0.0009076677972194977960, -0.9997682742251811083 ) ) ;
#63864=EDGE_CURVE ( 'NONE', #56032, #51989, #35781, .T. ) ;
#63865=CARTESIAN_POINT ( 'NONE',  ( 123.6837132603320413, -56.64645651782492308, 249.5838068554164693 ) ) ;
#63866=CARTESIAN_POINT ( 'NONE',  ( 117.1474210844629766, -33.86219250605441999, 149.0470538473389581 ) ) ;
#63867=CARTESIAN_POINT ( 'NONE',  ( 97.07537224739735393, -33.75284044148263973, 27.09562527591097236 ) ) ;
#63868=CARTESIAN_POINT ( 'NONE',  ( 107.2439061797007156, -47.23213900083308658, 208.5899109901969837 ) ) ;
#63870=DIRECTION ( 'NONE',  ( 0.000000000000000000, 0.000000000000000000, -1.000000000000000000 ) ) ;
#63872=CARTESIAN_POINT ( 'NONE',  ( 46.48091746482045750, -49.32844715994088602, 180.4678068554150911 ) ) ;
#63873=DIRECTION ( 'NONE',  ( 1.000000000000000078E-15, -1.000000000000000083E-30, -1.000000000000000000 ) ) ;
#63874=CARTESIAN_POINT ( 'NONE',  ( 113.2454987010698773, -28.75867294727909851, 69.55229194226531320 ) ) ;
#63876=ORIENTED_EDGE ( 'NONE', *, *, #25801, .F. ) ;
#63877=DIRECTION ( 'NONE',  ( 4.237773401492740281E-14, -1.000000000000000000, 0.000000000000000000 ) ) ;
#63878=EDGE_CURVE ( 'NONE', #26048, #78226, #29887, .T. ) ;
#63880=ORIENTED_EDGE ( 'NONE', *, *, #58502, .T. ) ;
#63881=EDGE_CURVE ( 'NONE', #43132, #31265, #68097, .T. ) ;
#63883=FACE_OUTER_BOUND ( 'NONE', #71513, .T. ) ;
#63885=CARTESIAN_POINT ( 'NONE',  ( 103.6060256796756960, -46.54035428658114171, 53.30705384733997221 ) ) ;
#63886=CARTESIAN_POINT ( 'NONE',  ( 53.56670390244743629, -48.82844715994058049, 180.4678068554151196 ) ) ;
#63888=CARTESIAN_POINT ( 'NONE',  ( 107.0664832912739968, -36.72944715994100306, 287.6356252759109680 ) ) ;
#63889=CARTESIAN_POINT ( 'NONE',  ( 112.8039874620816789, -45.48581773443041953, 174.0384824187679556 ) ) ;
#63890=CARTESIAN_POINT ( 'NONE',  ( 98.36549455146187881, -40.29075363668734155, 11.63562527591094309 ) ) ;
#63892=ORIENTED_EDGE ( 'NONE', *, *, #39900, .T. ) ;
#63893=VECTOR ( 'NONE', #75907, 1000.000000000000000 ) ;
#63895=ORIENTED_EDGE ( 'NONE', *, *, #53554, .F. ) ;
#63896=CARTESIAN_POINT ( 'NONE',  ( 113.1782937733034089, -44.75186859099120085, 108.0939586094537646 ) ) ;
#63898=CARTESIAN_POINT ( 'NONE',  ( 74.38348329127296665, -1.929447159941392931, 342.9256252759109884 ) ) ;
#63899=CARTESIAN_POINT ( 'NONE',  ( 115.8262517397711946, -31.73143768449714130, 19.23974975539183063 ) ) ;
#63901=DIRECTION ( 'NONE',  ( 1.000000000000000000, 4.163336342344333240E-14, 0.000000000000000000 ) ) ;
#63905=CARTESIAN_POINT ( 'NONE',  ( 98.44183741489689510, -42.05700530801252768, 11.76800622829193799 ) ) ;
#63909=CARTESIAN_POINT ( 'NONE',  ( 162.5667039024476708, -32.29483332968042930, 237.4678068554150059 ) ) ;
#63910=EDGE_CURVE ( 'NONE', #22927, #79637, #8545, .T. ) ;
#63911=CARTESIAN_POINT ( 'NONE',  ( 108.7800423072870046, -44.73859216708707720, 105.5623760838769698 ) ) ;
#63912=ADVANCED_FACE ( 'NONE', ( #36699 ), #15366, .F. ) ;
#63913=CARTESIAN_POINT ( 'NONE',  ( 107.0667039024467613, -18.72944715994092135, 196.8538068554170479 ) ) ;
#63915=ORIENTED_EDGE ( 'NONE', *, *, #1919, .F. ) ;
#63916=ORIENTED_EDGE ( 'NONE', *, *, #49092, .F. ) ;
#63917=CARTESIAN_POINT ( 'NONE',  ( 99.08983322626940549, -42.79586633336889179, 136.8435279569311263 ) ) ;
#63918=VERTEX_POINT ( 'NONE', #36243 ) ;
#63920=CARTESIAN_POINT ( 'NONE',  ( 98.99527800849182313, -31.91985561591122078, 127.3425356868499705 ) ) ;
#63921=CARTESIAN_POINT ( 'NONE',  ( 133.5842039024480812, -51.22944715994092491, 207.5838068554170377 ) ) ;
#63922=VECTOR ( 'NONE', #79894, 1000.000000000000000 ) ;
#63923=CARTESIAN_POINT ( 'NONE',  ( 100.2845952792443569, -46.47769036989463132, 83.09276813305294240 ) ) ;
#63924=CARTESIAN_POINT ( 'NONE',  ( 97.81169817874256012, -40.51742791483425776, 82.63555527327814332 ) ) ;
#63925=ORIENTED_EDGE ( 'NONE', *, *, #78011, .T. ) ;
#63927=ORIENTED_EDGE ( 'NONE', *, *, #58740, .F. ) ;
#63929=CARTESIAN_POINT ( 'NONE',  ( 116.6952228212742995, -32.58508497927773817, 79.14991099019697174 ) ) ;
#63931=CARTESIAN_POINT ( 'NONE',  ( 112.1067112481348858, -26.91823048478329738, 19.71086337114896736 ) ) ;
#63932=CARTESIAN_POINT ( 'NONE',  ( 101.1884425732228436, -45.36575980889334403, 193.1013395616249682 ) ) ;
#63933=FACE_OUTER_BOUND ( 'NONE', #68304, .T. ) ;
#63934=CARTESIAN_POINT ( 'NONE',  ( 41.56648329127499153, -32.07844715994070839, 198.9256252759119832 ) ) ;
#63935=CARTESIAN_POINT ( 'NONE',  ( 113.3313291481109815, -45.06216520097333955, 139.0899109901969553 ) ) ;
#63937=VERTEX_POINT ( 'NONE', #64844 ) ;
#63938=FACE_OUTER_BOUND ( 'NONE', #30298, .T. ) ;
#63939=VECTOR ( 'NONE', #5442, 1000.000000000000000 ) ;
#63940=CIRCLE ( 'NONE', #43819, 3.299999999999999822 ) ;
#63941=ORIENTED_EDGE ( 'NONE', *, *, #13189, .F. ) ;
#63942=CARTESIAN_POINT ( 'NONE',  ( 97.86658439798891607, -40.64924167897070362, 132.6473872692512259 ) ) ;
#63948=CARTESIAN_POINT ( 'NONE',  ( 111.1290374500119498, -47.00926920395730235, 22.88800622829195675 ) ) ;
#63950=DIRECTION ( 'NONE',  ( 0.000000000000000000, 0.000000000000000000, -1.000000000000000000 ) ) ;
#63951=CARTESIAN_POINT ( 'NONE',  ( 115.0372575091651015, -42.90846256308056184, 74.30229194293431760 ) ) ;
#63952=CARTESIAN_POINT ( 'NONE',  ( 115.1412022171004850, -43.23618977845876543, 43.27467289495995573 ) ) ;
#63954=CARTESIAN_POINT ( 'NONE',  ( 97.81366378802363215, -42.73395665195496917, 142.7965776568629508 ) ) ;
#63955=CARTESIAN_POINT ( 'NONE',  ( 97.07207205740387224, -35.37844121026580524, 72.21895861013597084 ) ) ;
#63957=DIRECTION ( 'NONE',  ( 0.000000000000000000, 1.000000000000000000, 0.000000000000000000 ) ) ;
#63958=ORIENTED_EDGE ( 'NONE', *, *, #30070, .F. ) ;
#63959=CIRCLE ( 'NONE', #45060, 5.599999999999994316 ) ;
#63960=DIRECTION ( 'NONE',  ( 1.000000000000000078E-15, 0.000000000000000000, 1.000000000000000000 ) ) ;
#63961=CARTESIAN_POINT ( 'NONE',  ( 73.06648329127401098, -46.72944715994106701, 14.67562527591093513 ) ) ;
#63962=DIRECTION ( 'NONE',  ( 0.7071067811864671926, 0.7071067811866279529, -2.899137802865059124E-29 ) ) ;
#63964=VERTEX_POINT ( 'NONE', #83499 ) ;
#63965=AXIS2_PLACEMENT_3D ( 'NONE', #46716, #48490, #69425 ) ;
#63966=CARTESIAN_POINT ( 'NONE',  ( 182.5667039024469886, -33.35206098992650681, -5.074374724088000832 ) ) ;
#63967=CARTESIAN_POINT ( 'NONE',  ( 109.8678013061348508, -26.64186650728397865, 174.8613395616249591 ) ) ;
#63968=VERTEX_POINT ( 'NONE', #38907 ) ;
#63969=PLANE ( 'NONE',  #78486 ) ;
#63970=CARTESIAN_POINT ( 'NONE',  ( 113.2328747769256410, -45.16229216617723097, 224.0784824187679476 ) ) ;
#63971=CARTESIAN_POINT ( 'NONE',  ( 115.2006710226633004, -43.31943727361606733, 84.28419670448195689 ) ) ;
#63972=DIRECTION ( 'NONE',  ( 0.000000000000000000, 1.000000000000000000, 0.000000000000000000 ) ) ;
#63973=DIRECTION ( 'NONE',  ( -1.000000000000000078E-15, 1.000000000000000083E-30, 1.000000000000000000 ) ) ;
#63974=DIRECTION ( 'NONE',  ( 0.000000000000000000, 0.000000000000000000, -1.000000000000000000 ) ) ;
#63975=EDGE_LOOP ( 'NONE', ( #3478, #6470, #79913 ) ) ;
#63976=ORIENTED_EDGE ( 'NONE', *, *, #38423, .T. ) ;
#63977=VECTOR ( 'NONE', #43692, 1000.000000000000000 ) ;
#63979=EDGE_CURVE ( 'NONE', #60263, #71030, #79384, .T. ) ;
#63983=CARTESIAN_POINT ( 'NONE',  ( 104.4105741502040701, -26.00004237129247642, 236.2575300378159682 ) ) ;
#63986=CARTESIAN_POINT ( 'NONE',  ( 135.7052281012230992, -16.51875982971419532, 2.060081176905330658 ) ) ;
#63991=VECTOR ( 'NONE', #86044, 1000.000000000000000 ) ;
#63992=CARTESIAN_POINT ( 'NONE',  ( 104.6437644399306635, -47.53804903515802494, 27.38895860924395009 ) ) ;
#63993=EDGE_LOOP ( 'NONE', ( #9492, #35025, #55486, #56826, #31808, #81012, #23671, #68246, #70747, #38304, #64612, #24604, #42967, #26347 ) ) ;
#63995=ORIENTED_EDGE ( 'NONE', *, *, #54500, .F. ) ;
#63996=AXIS2_PLACEMENT_3D ( 'NONE', #26936, #49144, #76880 ) ;
#63997=LINE ( 'NONE', #29472, #42727 ) ;
#63998=CARTESIAN_POINT ( 'NONE',  ( 102.0679063313821899, -27.96999881512665098, 16.49307739911019510 ) ) ;
#63999=CARTESIAN_POINT ( 'NONE',  ( 106.1957191385480854, -47.06291487533366080, 258.4975300378154088 ) ) ;
#64000=DIRECTION ( 'NONE',  ( 0.7071067811865789920, -0.7071067811865159314, 0.000000000000000000 ) ) ;
#64001=CARTESIAN_POINT ( 'NONE',  ( 113.5587197313313936, -28.64306037466259625, 115.5261014663869474 ) ) ;
#64005=CARTESIAN_POINT ( 'NONE',  ( 83.06670390244806867, -58.72944715994108122, 231.5838068554169524 ) ) ;
#64006=B_SPLINE_CURVE_WITH_KNOTS ( 'NONE', 3,
 ( #86252, #64467, #79454, #24034, #2250, #16321, #44447, #10392, #38534, #29954, #72178, #43998, #57638, #23158, #71734, #9503, #37210, #64911, #58091, #51704, #66229, #38097, #3573, #86701, #60308, #88044, #88937, #53479, #19438, #47571, #40770, #38981, #11736, #53931, #11276, #46223, #68039 ),
 .UNSPECIFIED., .F., .F.,
 ( 4, 2, 2, 2, 2, 2, 2, 2, 2, 2, 2, 2, 2, 2, 2, 1, 1, 1, 2, 4 ),
 ( 0.000000000000000000, 0.06251153962973163281, 0.1250230792594632656, 0.1875346188891948984, 0.2187903887040607287, 0.2500461585189265867, 0.2813019283337924170, 0.3125576981486583028, 0.3438134679635241886, 0.3750692377783900744, 0.4063250075932559047, 0.4375807774081217905, 0.4688365472229876763, 0.4844644321304208412, 0.4922783745841372016, 0.4961853458109952708, 0.4981388314244243887, 0.4991155742311390586, 0.4996039456344963936, 0.5000923170378537286 ),
 .UNSPECIFIED. ) ;
#64007=CARTESIAN_POINT ( 'NONE',  ( 77.40501520703328708, -36.03131342368239132, 2.974074870387424241 ) ) ;
#64008=ORIENTED_EDGE ( 'NONE', *, *, #70995, .T. ) ;
#64011=CARTESIAN_POINT ( 'NONE',  ( 114.7786440655094680, -32.32849264894101537, 285.6701547344685537 ) ) ;
#64012=VECTOR ( 'NONE', #59255, 1000.000000000000000 ) ;
#64013=DIRECTION ( 'NONE',  ( -1.000000000000000000, -4.299999999999999979E-14, -1.000000000000000078E-15 ) ) ;
#64014=EDGE_CURVE ( 'NONE', #30738, #26931, #1383, .T. ) ;
#64017=LINE ( 'NONE', #17208, #37245 ) ;
#64018=ORIENTED_EDGE ( 'NONE', *, *, #49263, .T. ) ;
#64019=CYLINDRICAL_SURFACE ( 'NONE', #87134, 10.00000000000000888 ) ;
#64020=PLANE ( 'NONE',  #29588 ) ;
#64022=CARTESIAN_POINT ( 'NONE',  ( 102.5580992528948912, -27.32936716964785262, 95.43276813305395478 ) ) ;
#64023=EDGE_LOOP ( 'NONE', ( #14997, #64970, #75162 ) ) ;
#64024=CARTESIAN_POINT ( 'NONE',  ( 106.3992821860680635, -28.18503700880033236, 24.56099125664901095 ) ) ;
#64027=CARTESIAN_POINT ( 'NONE',  ( 107.5349099188610893, -47.08895302312306086, 192.6003871806729535 ) ) ;
#64032=CARTESIAN_POINT ( 'NONE',  ( 99.99465048579469340, -28.96254792738658779, 281.6641967044822650 ) ) ;
#64033=CARTESIAN_POINT ( 'NONE',  ( 105.8119832718298028, -46.66943931204792051, 117.4785273639713239 ) ) ;
#64034=EDGE_LOOP ( 'NONE', ( #26584, #13766, #19588, #60451 ) ) ;
#64035=LINE ( 'NONE', #57193, #67642 ) ;
#64037=CARTESIAN_POINT ( 'NONE',  ( 103.4533635841105479, -46.55483943026052174, 138.2956252759109645 ) ) ;
#64038=ADVANCED_FACE ( 'NONE', ( #3503 ), #72558, .F. ) ;
#64039=CYLINDRICAL_SURFACE ( 'NONE', #29425, 4.749999999999976907 ) ;
#64040=ORIENTED_EDGE ( 'NONE', *, *, #89567, .F. ) ;
#64041=EDGE_LOOP ( 'NONE', ( #42105, #24167 ) ) ;
#64042=VERTEX_POINT ( 'NONE', #4408 ) ;
#64043=AXIS2_PLACEMENT_3D ( 'NONE', #30898, #10014, #64087 ) ;
#64044=CARTESIAN_POINT ( 'NONE',  ( 162.7866693523295680, -29.62846900981742237, 237.4678068554150059 ) ) ;
#64045=CARTESIAN_POINT ( 'NONE',  ( 104.4899648130921008, -26.97880497593449078, 266.2814577675392798 ) ) ;
#64047=FACE_BOUND ( 'NONE', #64238, .T. ) ;
#64048=CARTESIAN_POINT ( 'NONE',  ( 124.7998166246059810, 12.92155284005730387, 355.9756252759109998 ) ) ;
#64049=CARTESIAN_POINT ( 'NONE',  ( 111.0462345608747796, -47.04136251952688497, 13.85753003781498016 ) ) ;
#64051=DIRECTION ( 'NONE',  ( 0.000000000000000000, 0.000000000000000000, 1.000000000000000000 ) ) ;
#64052=ORIENTED_EDGE ( 'NONE', *, *, #23933, .F. ) ;
#64055=CARTESIAN_POINT ( 'NONE',  ( 109.6430060329453937, -46.48008849646763707, 42.78103013062236215 ) ) ;
#64058=VERTEX_POINT ( 'NONE', #44830 ) ;
#64059=VECTOR ( 'NONE', #34420, 1000.000000000000000 ) ;
#64060=CARTESIAN_POINT ( 'NONE',  ( 80.44338158421174967, -21.47944715994105636, 1.625625275910945078 ) ) ;
#64063=EDGE_CURVE ( 'NONE', #84622, #68948, #5790, .T. ) ;
#64064=FACE_BOUND ( 'NONE', #8286, .T. ) ;
#64065=DIRECTION ( 'NONE',  ( -2.999999999999999839E-15, 1.000000000000000000, -2.999999999999999900E-30 ) ) ;
#64066=CARTESIAN_POINT ( 'NONE',  ( 107.2162147037312678, -27.02129552338790575, 229.4867055423629836 ) ) ;
#64067=CYLINDRICAL_SURFACE ( 'NONE', #17092, 4.750000000000004441 ) ;
#64069=CARTESIAN_POINT ( 'NONE',  ( 98.29927950267186532, -42.45157995928803984, 101.7870538473399620 ) ) ;
#64070=ORIENTED_EDGE ( 'NONE', *, *, #85813, .T. ) ;
#64071=CARTESIAN_POINT ( 'NONE',  ( 128.0667039024480118, -48.82844715994099971, 250.9178068554150514 ) ) ;
#64072=ORIENTED_EDGE ( 'NONE', *, *, #38592, .F. ) ;
#64074=CARTESIAN_POINT ( 'NONE',  ( 103.2777252079319652, -27.47497190407113266, 276.3856931979651108 ) ) ;
#64076=ORIENTED_EDGE ( 'NONE', *, *, #6012, .T. ) ;
#64078=LINE ( 'NONE', #8215, #57796 ) ;
#64079=EDGE_LOOP ( 'NONE', ( #78912, #40903, #89734, #74090 ) ) ;
#64081=CARTESIAN_POINT ( 'NONE',  ( 184.5667039024483813, -48.82844715993448403, 249.9678068554149775 ) ) ;
#64082=AXIS2_PLACEMENT_3D ( 'NONE', #26986, #54652, #82418 ) ;
#64084=ORIENTED_EDGE ( 'NONE', *, *, #17708, .T. ) ;
#64085=CARTESIAN_POINT ( 'NONE',  ( 98.62940354253828446, -43.90657238178356181, 76.89943479971999807 ) ) ;
#64087=DIRECTION ( 'NONE',  ( 0.000000000000000000, 0.000000000000000000, -1.000000000000000000 ) ) ;
#64089=ORIENTED_EDGE ( 'NONE', *, *, #18113, .T. ) ;
#64091=EDGE_CURVE ( 'NONE', #74091, #83131, #38029, .T. ) ;
#64092=DIRECTION ( 'NONE',  ( 1.000000000000000078E-15, -1.000000000000000000, 0.000000000000000000 ) ) ;
#64094=DIRECTION ( 'NONE',  ( 1.000000000000000078E-15, 0.000000000000000000, 1.000000000000000000 ) ) ;
#64096=EDGE_CURVE ( 'NONE', #79585, #48818, #81022, .T. ) ;
#64098=CARTESIAN_POINT ( 'NONE',  ( 109.5135917660753506, -46.88567278592853427, 128.7641967044819751 ) ) ;
#64099=EDGE_CURVE ( 'NONE', #50121, #50189, #56332, .T. ) ;
#64100=LINE ( 'NONE', #965, #60940 ) ;
#64104=CARTESIAN_POINT ( 'NONE',  ( 143.0664832912740110, -18.82844715994099971, 323.8756252759120002 ) ) ;
#64105=CARTESIAN_POINT ( 'NONE',  ( 116.8150918559699818, -40.26546416881831192, 169.5375300378149745 ) ) ;
#64106=CARTESIAN_POINT ( 'NONE',  ( 31.71315051185499811, -33.70561438052090608, -5.074374724088000832 ) ) ;
#64108=AXIS2_PLACEMENT_3D ( 'NONE', #56589, #21651, #77053 ) ;
#64109=CARTESIAN_POINT ( 'NONE',  ( 117.8598252335457488, -34.07367295057271406, 10.01848241876795953 ) ) ;
#64110=PLANE ( 'NONE',  #15024 ) ;
#64111=DIRECTION ( 'NONE',  ( 0.000000000000000000, 0.000000000000000000, 1.000000000000000000 ) ) ;
#64112=DIRECTION ( 'NONE',  ( 0.000000000000000000, 0.000000000000000000, 1.000000000000000000 ) ) ;
#64114=CARTESIAN_POINT ( 'NONE',  ( 107.0664832912739968, -8.729447159940999512, 304.4006252759119775 ) ) ;
#64115=CARTESIAN_POINT ( 'NONE',  ( 101.7545977962314225, -44.98157700518534341, 222.1213395616259731 ) ) ;
#64116=ORIENTED_EDGE ( 'NONE', *, *, #75934, .F. ) ;
#64117=VECTOR ( 'NONE', #56690, 1000.000000000000000 ) ;
#64119=CARTESIAN_POINT ( 'NONE',  ( 97.58318307924886881, -33.33272491023742390, 172.4844404487539578 ) ) ;
#64120=MECHANICAL_DESIGN_GEOMETRIC_PRESENTATION_REPRESENTATION('',(#43804),#83002);
#64122=CARTESIAN_POINT ( 'NONE',  ( 104.1188366437555288, -45.08645965563772506, 53.73872616303998484 ) ) ;
#64125=DIRECTION ( 'NONE',  ( 1.000000000000000000, 3.999999999999999995E-14, 1.000000000000000078E-15 ) ) ;
#64127=DIRECTION ( 'NONE',  ( 4.299999999999999979E-14, -1.000000000000000000, 4.400000000000000367E-29 ) ) ;
#64128=CARTESIAN_POINT ( 'NONE',  ( 118.0585799961421429, -32.36802338489820841, 249.1270538473389706 ) ) ;
#64129=PLANE ( 'NONE',  #45977 ) ;
#64130=ORIENTED_EDGE ( 'NONE', *, *, #88997, .F. ) ;
#64131=ORIENTED_EDGE ( 'NONE', *, *, #66546, .F. ) ;
#64132=CIRCLE ( 'NONE', #48147, 2.500000000000002220 ) ;
#64136=LINE ( 'NONE', #57298, #66533 ) ;
#64138=CARTESIAN_POINT ( 'NONE',  ( 104.8797383215544414, -46.86635653470245444, 28.41943479971997988 ) ) ;
#64139=LINE ( 'NONE', #83692, #12210 ) ;
#64140=VERTEX_POINT ( 'NONE', #24846 ) ;
#64141=AXIS2_PLACEMENT_3D ( 'NONE', #27171, #70298, #13545 ) ;
#64142=CARTESIAN_POINT ( 'NONE',  ( 103.5842829832543686, -46.60199803408937669, 53.30705384733997221 ) ) ;
#64143=EDGE_CURVE ( 'NONE', #667, #38195, #65862, .T. ) ;
#64145=CARTESIAN_POINT ( 'NONE',  ( 100.2480723708022197, -28.84298388537911606, 260.6441967044822263 ) ) ;
#64148=VECTOR ( 'NONE', #3407, 1000.000000000000000 ) ;
#64152=DIRECTION ( 'NONE',  ( 0.000000000000000000, 0.000000000000000000, -1.000000000000000000 ) ) ;
#64154=CARTESIAN_POINT ( 'NONE',  ( 115.5148531418241191, -38.60720430987922214, 101.4585665600679647 ) ) ;
#64155=CARTESIAN_POINT ( 'NONE',  ( 117.4353638176713446, -35.45525114565609215, 189.9241967044829664 ) ) ;
#64156=ADVANCED_FACE ( 'NONE', ( #18466 ), #51192, .T. ) ;
#64157=CYLINDRICAL_SURFACE ( 'NONE', #55096, 37.00000000000000711 ) ;
#64159=EDGE_CURVE ( 'NONE', #50262, #46964, #37490, .T. ) ;
#64161=ORIENTED_EDGE ( 'NONE', *, *, #76090, .F. ) ;
#64162=ORIENTED_EDGE ( 'NONE', *, *, #62402, .T. ) ;
#64163=EDGE_CURVE ( 'NONE', #33465, #62792, #38960, .T. ) ;
#64164=FACE_OUTER_BOUND ( 'NONE', #57780, .T. ) ;
#64166=ORIENTED_EDGE ( 'NONE', *, *, #25891, .T. ) ;
#64167=CARTESIAN_POINT ( 'NONE',  ( 141.8664832912729992, -1.929447159941394263, 352.4506252759079530 ) ) ;
#64169=CARTESIAN_POINT ( 'NONE',  ( 105.7976002935269122, -26.72429596296039023, 25.17744450168613213 ) ) ;
#64170=CARTESIAN_POINT ( 'NONE',  ( 99.28690145085043639, -32.09363259137744251, 130.3333722090289655 ) ) ;
#64171=CARTESIAN_POINT ( 'NONE',  ( 109.9954698844069156, -26.70111721404902383, 259.8499109901965767 ) ) ;
#64173=LINE ( 'NONE', #44142, #38312 ) ;
#64176=ORIENTED_EDGE ( 'NONE', *, *, #81492, .F. ) ;
#64178=DIRECTION ( 'NONE',  ( -0.7071067811865634489, 0.7071067811865315855, -7.071067811865330380E-16 ) ) ;
#64180=CARTESIAN_POINT ( 'NONE',  ( 117.4149692539380681, -32.71426074976766074, 94.10895860924395606 ) ) ;
#64182=ORIENTED_EDGE ( 'NONE', *, *, #25382, .T. ) ;
#64184=CARTESIAN_POINT ( 'NONE',  ( 115.6954802162012044, -42.57986958318428350, 273.3527681330537575 ) ) ;
#64185=DIRECTION ( 'NONE',  ( 5.512527431108029424E-15, -1.000000000000000000, 0.000000000000000000 ) ) ;
#64189=FACE_OUTER_BOUND ( 'NONE', #85670, .T. ) ;
#64190=CARTESIAN_POINT ( 'NONE',  ( 41.56670390244801894, -27.57844715994070484, 342.9256252759119548 ) ) ;
#64191=CARTESIAN_POINT ( 'NONE',  ( 48.16670390244654243, -28.27351298637380950, 193.9678068554150911 ) ) ;
#64194=CARTESIAN_POINT ( 'NONE',  ( 128.0667039024480118, -58.72944715994110254, 250.9178068554150514 ) ) ;
#64195=FACE_OUTER_BOUND ( 'NONE', #57532, .T. ) ;
#64197=EDGE_CURVE ( 'NONE', #57650, #77070, #46606, .T. ) ;
#64198=DIRECTION ( 'NONE',  ( 1.000000000000000078E-15, 0.000000000000000000, -1.000000000000000000 ) ) ;
#64199=ORIENTED_EDGE ( 'NONE', *, *, #5379, .T. ) ;
#64200=PLANE ( 'NONE',  #59701 ) ;
#64201=CARTESIAN_POINT ( 'NONE',  ( 111.0013748985821422, -46.40740010236051916, 282.8841967044824628 ) ) ;
#64202=CARTESIAN_POINT ( 'NONE',  ( 108.8488479242245290, -47.00104215551821341, 163.7127681330539701 ) ) ;
#64203=CARTESIAN_POINT ( 'NONE',  ( 111.3320466151124322, -27.19308368994588676, 20.74133956162494030 ) ) ;
#64205=PLANE ( 'NONE',  #74041 ) ;
#64206=CARTESIAN_POINT ( 'NONE',  ( 82.58878920444031735, -35.63370978841373926, 7.053538376720832836 ) ) ;
#64211=EDGE_LOOP ( 'NONE', ( #48345, #30778 ) ) ;
#64213=CARTESIAN_POINT ( 'NONE',  ( 112.4079628628857250, -28.49644221148697198, 65.61848241876694487 ) ) ;
#64214=CARTESIAN_POINT ( 'NONE',  ( 107.0664832912750057, -36.72944715993903486, 0.4256252759109709349 ) ) ;
#64215=VERTEX_POINT ( 'NONE', #32989 ) ;
#64217=CARTESIAN_POINT ( 'NONE',  ( 112.1942863616535817, -45.78120396183486918, 208.9870538473389558 ) ) ;
#64219=CARTESIAN_POINT ( 'NONE',  ( 109.6427860908511036, -46.48014371229046304, 147.7814644202007059 ) ) ;
#64221=CARTESIAN_POINT ( 'NONE',  ( 101.0090012246669886, -28.74596344506981538, 86.59355491815287564 ) ) ;
#64222=CARTESIAN_POINT ( 'NONE',  ( 164.7812970173232543, -35.65087443489315433, 237.4678068554150059 ) ) ;
#64223=CARTESIAN_POINT ( 'NONE',  ( 110.8531357376099891, -45.98478418387610844, 97.88551033190712758 ) ) ;
#64224=CARTESIAN_POINT ( 'NONE',  ( 103.4440497394145808, -45.85039829771051245, 117.2756252759109543 ) ) ;
#64226=VERTEX_POINT ( 'NONE', #88425 ) ;
#64227=CARTESIAN_POINT ( 'NONE',  ( 101.9660762386545514, -28.83879614530413704, 66.97682140113498406 ) ) ;
#64229=CARTESIAN_POINT ( 'NONE',  ( 112.7271506738795779, -45.41826929060054852, 219.0480062282919960 ) ) ;
#64232=CARTESIAN_POINT ( 'NONE',  ( 113.2454969875984290, -28.75867143562818740, 110.5525043974795381 ) ) ;
#64235=LINE ( 'NONE', #9268, #31877 ) ;
#64237=CARTESIAN_POINT ( 'NONE',  ( 116.7861719071672866, -43.46560779248406448, 163.3441967044829823 ) ) ;
#64238=EDGE_LOOP ( 'NONE', ( #15696, #67537 ) ) ;
#64240=EDGE_LOOP ( 'NONE', ( #50155, #75382, #59387, #36371 ) ) ;
#64241=CARTESIAN_POINT ( 'NONE',  ( 21.03715912545744615, -47.82818131006197149, 129.9678068554150627 ) ) ;
#64243=CARTESIAN_POINT ( 'NONE',  ( 98.34937724553353178, -31.65743187412461168, 130.9065372364317454 ) ) ;
#64244=CARTESIAN_POINT ( 'NONE',  ( 99.08943691707119683, -42.79534522775045957, 102.8439055007673915 ) ) ;
#64245=CARTESIAN_POINT ( 'NONE',  ( 101.3402310731127329, -30.91225182618282830, 223.5138046553059894 ) ) ;
#64246=EDGE_CURVE ( 'NONE', #18963, #27831, #44924, .T. ) ;
#64247=CIRCLE ( 'NONE', #48255, 2.749999999999974687 ) ;
#64248=DIRECTION ( 'NONE',  ( 5.512527431108029424E-15, -1.000000000000000000, 0.000000000000000000 ) ) ;
#64250=CARTESIAN_POINT ( 'NONE',  ( 100.8863770005861795, -45.89136241369948976, 152.0918157521009562 ) ) ;
#64251=EDGE_CURVE ( 'NONE', #64543, #66869, #38190, .T. ) ;
#64252=DIRECTION ( 'NONE',  ( 1.000000000000000000, 0.000000000000000000, 0.000000000000000000 ) ) ;
#64254=ORIENTED_EDGE ( 'NONE', *, *, #80019, .T. ) ;
#64255=VERTEX_POINT ( 'NONE', #18920 ) ;
#64256=EDGE_CURVE ( 'NONE', #16018, #20410, #43302, .T. ) ;
#64257=CARTESIAN_POINT ( 'NONE',  ( 29.56670390244784485, -48.82844715994099971, 180.4678068554150911 ) ) ;
#64259=ORIENTED_EDGE ( 'NONE', *, *, #9737, .T. ) ;
#64261=CARTESIAN_POINT ( 'NONE',  ( 52.65249034007825912, -48.32844715994060181, 300.4678068554150059 ) ) ;
#64262=CARTESIAN_POINT ( 'NONE',  ( 102.7933444172945769, -44.96577155458380304, 15.01380465530593966 ) ) ;
#64264=CARTESIAN_POINT ( 'NONE',  ( 117.0608944987687750, -38.08045336284195059, 273.7189585899762960 ) ) ;
#64265=VERTEX_POINT ( 'NONE', #6636 ) ;
#64266=CARTESIAN_POINT ( 'NONE',  ( 115.1001406608323947, -41.05364652694197503, 9.635625275910943088 ) ) ;
#64267=LINE ( 'NONE', #50620, #6757 ) ;
#64271=CARTESIAN_POINT ( 'NONE',  ( 99.50493083782342296, -43.30601922071209486, 111.8960934546087884 ) ) ;
#64273=EDGE_LOOP ( 'NONE', ( #25346, #33654, #51522, #28445 ) ) ;
#64274=CIRCLE ( 'NONE', #71544, 5.599999999999994316 ) ;
#64275=B_SPLINE_CURVE_WITH_KNOTS ( 'NONE', 3,
 ( #68010, #39404, #68465, #88469, #26223, #5795, #61187, #88914, #26668, #82112, #19866, #75281, #13057, #6239, #33930, #73930, #11709, #27124, #75726, #13497, #54802, #41184, #67109, #4891, #7585 ),
 .UNSPECIFIED., .F., .F.,
 ( 4, 2, 1, 2, 2, 2, 2, 2, 2, 2, 2, 2, 4 ),
 ( 0.5000912566136184179, 0.5039967936713244390, 0.5079023307290305711, 0.5157134048444427243, 0.5313355530752669198, 0.5625798495369156438, 0.6250684424602134248, 0.6875570353835112059, 0.7500456283068088759, 0.8125342212301067679, 0.8750228141534044379, 0.9375114070767023300, 1.000000000000000000 ),
 .UNSPECIFIED. ) ;
#64278=CARTESIAN_POINT ( 'NONE',  ( 101.7271154311333135, -43.54062005560803073, 274.8776141791153691 ) ) ;
#64279=CARTESIAN_POINT ( 'NONE',  ( 102.6741928909662391, -27.25030431863982372, 180.4213395616249898 ) ) ;
#64280=CARTESIAN_POINT ( 'NONE',  ( 113.0643619202157879, -28.22920495858469891, 129.5870538473399449 ) ) ;
#64281=PLANE ( 'NONE',  #9469 ) ;
#64282=LINE ( 'NONE', #15234, #26371 ) ;
#64283=CARTESIAN_POINT ( 'NONE',  ( 115.4598468997141509, -29.53740796227222987, 225.4022919425769658 ) ) ;
#64284=CARTESIAN_POINT ( 'NONE',  ( 112.0660770571772105, -45.48830407390881447, 98.99134466148210265 ) ) ;
#64286=ORIENTED_EDGE ( 'NONE', *, *, #26500, .T. ) ;
#64288=ORIENTED_EDGE ( 'NONE', *, *, #72506, .T. ) ;
#64290=ORIENTED_EDGE ( 'NONE', *, *, #87127, .T. ) ;
#64291=CARTESIAN_POINT ( 'NONE',  ( 96.14524839136181811, -32.00129468986670389, 211.0013395616249738 ) ) ;
#64292=VERTEX_POINT ( 'NONE', #42927 ) ;
#64293=SHAPE_REPRESENTATION ( 'Feed Lead', ( #50656 ), #27505 ) ;
#64294=CARTESIAN_POINT ( 'NONE',  ( 95.31140346374353101, -38.27925045402978554, 151.4299109901969871 ) ) ;
#64295=DIRECTION ( 'NONE',  ( -0.7071067811856560636, -0.7071067811874389708, 0.000000000000000000 ) ) ;
#64298=PLANE ( 'NONE',  #32561 ) ;
#64299=FACE_OUTER_BOUND ( 'NONE', #40887, .T. ) ;
#64301=CARTESIAN_POINT ( 'NONE',  ( 109.9541224118590321, -48.19721710984605068, 238.7727681330539724 ) ) ;
#64302=CARTESIAN_POINT ( 'NONE',  ( 194.5667039024485803, -47.82844715993405060, 129.9678068554150343 ) ) ;
#64304=CARTESIAN_POINT ( 'NONE',  ( 98.34910283431625544, -31.65794092288234296, 271.9061491226904081 ) ) ;
#64305=TOROIDAL_SURFACE ( 'NONE', #1985, 13.50000000000000000, 0.5000000000000000000 ) ;
#64306=PLANE ( 'NONE',  #89234 ) ;
#64307=CARTESIAN_POINT ( 'NONE',  ( 113.2454986932114309, -28.75867294076968861, 255.5522919430740387 ) ) ;
#64309=CARTESIAN_POINT ( 'NONE',  ( 113.4887626673159673, -41.81888551505019080, 195.5838068554168103 ) ) ;
#64312=CARTESIAN_POINT ( 'NONE',  ( 117.0383059485392607, -33.61350157978694142, 174.0670538473389399 ) ) ;
#64313=CARTESIAN_POINT ( 'NONE',  ( 113.4595210239597520, -46.70760751678911049, 64.02991099019695298 ) ) ;
#64314=CARTESIAN_POINT ( 'NONE',  ( 116.3890555338844450, -44.12544333927958462, 194.2927681330539542 ) ) ;
#64317=CYLINDRICAL_SURFACE ( 'NONE', #66367, 1.000000000000000888 ) ;
#64318=CARTESIAN_POINT ( 'NONE',  ( 162.7866693523280048, -29.62846900982320264, -5.074374724088000832 ) ) ;
#64319=LINE ( 'NONE', #83874, #26932 ) ;
#64320=DIRECTION ( 'NONE',  ( 1.000000000000000078E-15, 0.000000000000000000, 1.000000000000000000 ) ) ;
#64323=AXIS2_PLACEMENT_3D ( 'NONE', #13533, #33960, #61224 ) ;
#64324=DIRECTION ( 'NONE',  ( 0.000000000000000000, 0.000000000000000000, -1.000000000000000000 ) ) ;
#64325=ORIENTED_EDGE ( 'NONE', *, *, #54056, .F. ) ;
#64326=ORIENTED_EDGE ( 'NONE', *, *, #80577, .F. ) ;
#64328=ORIENTED_EDGE ( 'NONE', *, *, #41619, .T. ) ;
#64329=CARTESIAN_POINT ( 'NONE',  ( 109.6783822832554591, -47.44587409406599221, 83.75467289495897205 ) ) ;
#64333=CARTESIAN_POINT ( 'NONE',  ( 97.07207206336831007, -35.37844116818202878, 177.2189586067734979 ) ) ;
#64334=CARTESIAN_POINT ( 'NONE',  ( 97.32756240343553600, -42.09278592120095652, 26.72705384733997747 ) ) ;
#64337=EDGE_LOOP ( 'NONE', ( #83115, #34148, #74994, #65019 ) ) ;
#64338=VECTOR ( 'NONE', #80282, 1000.000000000000000 ) ;
#64339=EDGE_CURVE ( 'NONE', #810, #64226, #85207, .T. ) ;
#64341=DIRECTION ( 'NONE',  ( 4.299999999999999979E-14, -1.000000000000000000, 0.000000000000000000 ) ) ;
#64342=DIRECTION ( 'NONE',  ( 0.0001211784769825749762, -0.7071067708032375831, -0.7071067811865434649 ) ) ;
#64344=PLANE ( 'NONE',  #13647 ) ;
#64346=CARTESIAN_POINT ( 'NONE',  ( 21.03689327557613709, -23.42844715994197813, 193.9678068554150627 ) ) ;
#64348=DIRECTION ( 'NONE',  ( 0.000000000000000000, 0.000000000000000000, -1.000000000000000000 ) ) ;
#64349=CARTESIAN_POINT ( 'NONE',  ( 111.1204619107249982, -46.98756979655009047, 22.88800622829195675 ) ) ;
#64350=ORIENTED_EDGE ( 'NONE', *, *, #47403, .F. ) ;
#64351=CARTESIAN_POINT ( 'NONE',  ( 105.7995190932148404, -26.72403489713727964, 270.1772918944074604 ) ) ;
#64352=DIRECTION ( 'NONE',  ( -0.000000000000000000, -0.000000000000000000, -1.000000000000000000 ) ) ;
#64353=CARTESIAN_POINT ( 'NONE',  ( 114.7830339860594364, -33.98399025413122843, 111.9166617981629486 ) ) ;
#64356=CARTESIAN_POINT ( 'NONE',  ( 97.31319625472109180, -38.96114016031690852, 96.50548233485649519 ) ) ;
#64357=ADVANCED_FACE ( 'NONE', ( #76579, #64299 ), #21627, .T. ) ;
#64358=CYLINDRICAL_SURFACE ( 'NONE', #63367, 0.9999999999999940048 ) ;
#64359=ORIENTED_EDGE ( 'NONE', *, *, #2526, .F. ) ;
#64361=CARTESIAN_POINT ( 'NONE',  ( 104.4082270698484223, -46.45812771010326259, 137.3629473761069448 ) ) ;
#64362=AXIS2_PLACEMENT_3D ( 'NONE', #12609, #40298, #49795 ) ;
#64363=EDGE_CURVE ( 'NONE', #13968, #64372, #69316, .T. ) ;
#64364=VERTEX_POINT ( 'NONE', #71121 ) ;
#64366=CARTESIAN_POINT ( 'NONE',  ( 99.08321105494920289, -40.57595765811257138, 168.1158690201829700 ) ) ;
#64367=ADVANCED_FACE ( 'NONE', ( #56102 ), #7090, .F. ) ;
#64369=CARTESIAN_POINT ( 'NONE',  ( 96.01268936646508223, -41.06948063400285776, 92.62419670448296927 ) ) ;
#64370=CIRCLE ( 'NONE', #33880, 4.750000000000000888 ) ;
#64371=CARTESIAN_POINT ( 'NONE',  ( 110.8540151137909930, -45.98442434552481473, 17.88558598347468731 ) ) ;
#64372=VERTEX_POINT ( 'NONE', #15704 ) ;
#64376=CARTESIAN_POINT ( 'NONE',  ( 109.2506105747909828, -28.86437792779224409, 172.6795189410199498 ) ) ;
#64377=CARTESIAN_POINT ( 'NONE',  ( 117.9477513149503523, -41.48675964724572651, 58.49848241876792798 ) ) ;
#64379=CARTESIAN_POINT ( 'NONE',  ( 112.9508454419806043, -28.15023113465287352, 44.59848241876795782 ) ) ;
#64380=CARTESIAN_POINT ( 'NONE',  ( 102.0405519839503086, -46.59986864225058412, 168.2137205140059564 ) ) ;
#64381=DIRECTION ( 'NONE',  ( 1.000000000000000000, 0.000000000000000000, 0.000000000000000000 ) ) ;
#64383=CARTESIAN_POINT ( 'NONE',  ( 117.2221417514105610, -42.83659189374058940, 124.3956252759109731 ) ) ;
#64385=ORIENTED_EDGE ( 'NONE', *, *, #44010, .F. ) ;
#64388=LINE ( 'NONE', #14904, #18642 ) ;
#64389=VERTEX_POINT ( 'NONE', #27966 ) ;
#64390=VERTEX_POINT ( 'NONE', #14360 ) ;
#64391=AXIS2_PLACEMENT_3D ( 'NONE', #55095, #14250, #75583 ) ;
#64394=CARTESIAN_POINT ( 'NONE',  ( 96.68578154376476164, -42.44622222083611263, 26.72705384733997747 ) ) ;
#64396=VECTOR ( 'NONE', #42797, 1000.000000000000000 ) ;
#64399=CARTESIAN_POINT ( 'NONE',  ( 110.2470682213182869, -46.59973918892936240, 57.83657765686300678 ) ) ;
#64401=CARTESIAN_POINT ( 'NONE',  ( 116.6407469026008243, -40.79910830432089597, 164.5070538473399608 ) ) ;
#64402=CARTESIAN_POINT ( 'NONE',  ( 97.80969231062213964, -40.51824920587227297, 266.6357212253427633 ) ) ;
#64403=FACE_OUTER_BOUND ( 'NONE', #40407, .T. ) ;
#64404=ORIENTED_EDGE ( 'NONE', *, *, #55853, .F. ) ;
#64409=CARTESIAN_POINT ( 'NONE',  ( 116.7015053437751959, -40.82493444377960401, 168.5070538473399608 ) ) ;
#64410=ORIENTED_EDGE ( 'NONE', *, *, #89515, .F. ) ;
#64412=CARTESIAN_POINT ( 'NONE',  ( 97.59563580048326514, -41.13856347273024738, 252.6727681330536655 ) ) ;
#64413=CARTESIAN_POINT ( 'NONE',  ( 108.5441076757828398, -26.36558658937538269, 100.9641967044829727 ) ) ;
#64414=FACE_OUTER_BOUND ( 'NONE', #6044, .T. ) ;
#64416=CARTESIAN_POINT ( 'NONE',  ( 102.0655984279635504, -27.97135235995153835, 191.4897250454755238 ) ) ;
#64418=VERTEX_POINT ( 'NONE', #69765 ) ;
#64419=CIRCLE ( 'NONE', #81799, 0.9999999999999731326 ) ;
#64423=ORIENTED_EDGE ( 'NONE', *, *, #31953, .F. ) ;
#64425=AXIS2_PLACEMENT_3D ( 'NONE', #11097, #71567, #38803 ) ;
#64428=CARTESIAN_POINT ( 'NONE',  ( 115.2517161551258766, -30.21613035964762517, 240.3613395616249875 ) ) ;
#64429=DIRECTION ( 'NONE',  ( 0.000000000000000000, 0.000000000000000000, -1.000000000000000000 ) ) ;
#64431=LINE ( 'NONE', #86667, #51121 ) ;
#64432=DIRECTION ( 'NONE',  ( 1.000000000000000000, 4.299999999999999979E-14, 1.000000000000000078E-15 ) ) ;
#64433=FACE_OUTER_BOUND ( 'NONE', #35152, .T. ) ;
#64434=CARTESIAN_POINT ( 'NONE',  ( 96.15435578470099642, -38.63231720721949358, 46.45181575210094138 ) ) ;
#64435=VERTEX_POINT ( 'NONE', #36136 ) ;
#64436=ORIENTED_EDGE ( 'NONE', *, *, #30825, .T. ) ;
#64437=ORIENTED_EDGE ( 'NONE', *, *, #74129, .T. ) ;
#64439=DIRECTION ( 'NONE',  ( 0.7071067811865774377, -0.7071067811865175967, 7.071067811865470403E-16 ) ) ;
#64441=B_SPLINE_CURVE_WITH_KNOTS ( 'NONE', 3,
 ( #25534, #38713, #3759, #66417, #10130, #37838, #60491, #23775, #24645, #65537, #32796, #79632, #79192, #87772, #31011, #53209, #58703, #86445 ),
 .UNSPECIFIED., .F., .F.,
 ( 4, 2, 2, 2, 2, 2, 2, 2, 4 ),
 ( 0.5000000021306179043, 0.5625000018642907218, 0.6250000015979634282, 0.6875000013316361347, 0.7500000010653089522, 0.8125000007989817696, 0.8750000005326544761, 0.9375000002663271825, 1.000000000000000000 ),
 .UNSPECIFIED. ) ;
#64442=CARTESIAN_POINT ( 'NONE',  ( 115.5794671477453761, -31.87256924526127477, 285.2384824187676600 ) ) ;
#64443=DIRECTION ( 'NONE',  ( 0.7071067811865453523, 0.7071067811865496822, 7.071067811865460542E-16 ) ) ;
#64444=CARTESIAN_POINT ( 'NONE',  ( 98.20106483660288177, -31.34956418181673854, 121.8803871806729546 ) ) ;
#64445=CARTESIAN_POINT ( 'NONE',  ( 99.04397839509049106, -42.84113223740011733, 26.84394684677412002 ) ) ;
#64448=CARTESIAN_POINT ( 'NONE',  ( 78.57311110803117060, -34.41810224487900172, 1.981704920704651762 ) ) ;
#64451=CARTESIAN_POINT ( 'NONE',  ( 105.6993345102559942, -28.68213381844667609, 13.02809036959096112 ) ) ;
#64453=DIRECTION ( 'NONE',  ( 1.000000000000000078E-15, 1.000000000000000083E-30, -1.000000000000000000 ) ) ;
#64454=AXIS2_PLACEMENT_3D ( 'NONE', #74454, #17705, #3620 ) ;
#64455=PLANE ( 'NONE',  #37446 ) ;
#64456=EDGE_CURVE ( 'NONE', #41571, #53161, #49747, .T. ) ;
#64457=LINE ( 'NONE', #44889, #57594 ) ;
#64458=ORIENTED_EDGE ( 'NONE', *, *, #45674, .F. ) ;
#64460=DIRECTION ( 'NONE',  ( -0.7071067811865274777, 0.7071067811865675568, -7.071067811865283048E-16 ) ) ;
#64461=EDGE_CURVE ( 'NONE', #66495, #48789, #44729, .T. ) ;
#64463=CARTESIAN_POINT ( 'NONE',  ( 97.26623355869948284, -31.61728591124570542, 90.93181575210196854 ) ) ;
#64464=EDGE_LOOP ( 'NONE', ( #89530, #29746, #67185, #62755 ) ) ;
#64465=EDGE_CURVE ( 'NONE', #893, #628, #3403, .T. ) ;
#64466=CARTESIAN_POINT ( 'NONE',  ( 111.7162562550164608, -28.95820004563618610, 54.08194363760093637 ) ) ;
#64467=CARTESIAN_POINT ( 'NONE',  ( 116.5614777235394399, -33.52755762741292500, 90.08470898062006427 ) ) ;
#64468=CARTESIAN_POINT ( 'NONE',  ( 106.9806506443342755, -46.50983917909375265, 187.5699109901969734 ) ) ;
#64472=LINE ( 'NONE', #51259, #53113 ) ;
#64473=DIRECTION ( 'NONE',  ( -0.7071067708032326982, -0.0001211784769776692866, -0.7071067811865484609 ) ) ;
#64474=CARTESIAN_POINT ( 'NONE',  ( 96.72029611048706954, -35.13276604965626859, 262.2041967044821149 ) ) ;
#64477=ORIENTED_EDGE ( 'NONE', *, *, #45725, .F. ) ;
#64478=CARTESIAN_POINT ( 'NONE',  ( 114.5432832596865325, -29.39626808186021378, 145.4441967044819819 ) ) ;
#64479=LINE ( 'NONE', #84503, #75842 ) ;
#64480=AXIS2_PLACEMENT_3D ( 'NONE', #79186, #26437, #74141 ) ;
#64481=CIRCLE ( 'NONE', #9371, 2.029999999999997140 ) ;
#64483=ORIENTED_EDGE ( 'NONE', *, *, #51306, .T. ) ;
#64487=CONICAL_SURFACE ( 'NONE', #64425, 1.624999999999987566, 1.029744258676650093 ) ;
#64490=CARTESIAN_POINT ( 'NONE',  ( 151.0371591254584871, -46.82818131005582529, 180.4678068554149775 ) ) ;
#64491=CARTESIAN_POINT ( 'NONE',  ( 108.1128363339379632, -46.45408497333518483, 202.6613395616259652 ) ) ;
#64492=CARTESIAN_POINT ( 'NONE',  ( 107.0664832912739968, -36.72944715994100306, 287.6356252759109680 ) ) ;
#64493=EDGE_CURVE ( 'NONE', #72226, #84886, #68157, .T. ) ;
#64495=CARTESIAN_POINT ( 'NONE',  ( 134.0664832912740110, -8.350947159940998787, 293.6356252759119911 ) ) ;
#64496=CARTESIAN_POINT ( 'NONE',  ( 100.5976686157419806, -28.50914727160554207, 11.60705384733995515 ) ) ;
#64498=VERTEX_POINT ( 'NONE', #38802 ) ;
#64500=CARTESIAN_POINT ( 'NONE',  ( 116.8171211726486405, -34.15291134256264627, 44.03120960089060532 ) ) ;
#64501=ORIENTED_EDGE ( 'NONE', *, *, #13261, .T. ) ;
#64502=EDGE_LOOP ( 'NONE', ( #31374, #36661 ) ) ;
#64503=DIRECTION ( 'NONE',  ( 0.000000000000000000, 0.000000000000000000, -1.000000000000000000 ) ) ;
#64504=DIRECTION ( 'NONE',  ( -0.000000000000000000, 1.000000000000000000, 0.000000000000000000 ) ) ;
#64505=CARTESIAN_POINT ( 'NONE',  ( 116.3308458273176456, -44.07926308385601999, 198.2927681330539542 ) ) ;
#64506=CARTESIAN_POINT ( 'NONE',  ( 172.5664832912740110, -18.82844715994099971, 138.9256252759119832 ) ) ;
#64508=CARTESIAN_POINT ( 'NONE',  ( 41.56648329127381203, -18.82844715994071194, 261.9256252759119548 ) ) ;
#64509=CARTESIAN_POINT ( 'NONE',  ( 99.57203460073428403, -40.82693060065560076, 221.1467055423629517 ) ) ;
#64511=CARTESIAN_POINT ( 'NONE',  ( 104.4960957391109559, -46.84663716100901354, 43.37848241876896083 ) ) ;
#64512=CARTESIAN_POINT ( 'NONE',  ( 172.5664832912740110, -36.32844715994070839, 18.92562527591200094 ) ) ;
#64513=CARTESIAN_POINT ( 'NONE',  ( 117.9212005353621322, -39.05065313503074975, 108.6708633711489824 ) ) ;
#64515=CARTESIAN_POINT ( 'NONE',  ( 131.3780189692435556, -19.30949827215296821, 6.839365140900929951 ) ) ;
#64517=CARTESIAN_POINT ( 'NONE',  ( 63.56670390244800473, -40.82844715994016127, 249.9678068554150343 ) ) ;
#64519=CARTESIAN_POINT ( 'NONE',  ( 102.0645642710494769, -27.97192201181788462, 276.4899936502032460 ) ) ;
#64520=ORIENTED_EDGE ( 'NONE', *, *, #53357, .F. ) ;
#64524=CARTESIAN_POINT ( 'NONE',  ( 37.03715912545347777, -48.62818131006128652, 129.9678068554150911 ) ) ;
#64529=CARTESIAN_POINT ( 'NONE',  ( 96.61701384456422659, -37.56428313387978335, 101.3899109901969524 ) ) ;
#64531=CARTESIAN_POINT ( 'NONE',  ( 97.81051247419222250, -40.51455135576280497, 166.6353777005785446 ) ) ;
#64534=LINE ( 'NONE', #2316, #74621 ) ;
#64535=ORIENTED_EDGE ( 'NONE', *, *, #89281, .F. ) ;
#64537=CARTESIAN_POINT ( 'NONE',  ( 112.1393456662218568, -28.01282279633491967, 154.6564586069755762 ) ) ;
#64538=CARTESIAN_POINT ( 'NONE',  ( 51.06670390244768498, -32.29483332968566600, 237.4678068554150059 ) ) ;
#64540=FACE_OUTER_BOUND ( 'NONE', #50643, .T. ) ;
#64541=CARTESIAN_POINT ( 'NONE',  ( 107.0664832912739399, -36.72944715994095333, 311.6356252759109680 ) ) ;
#64543=VERTEX_POINT ( 'NONE', #78829 ) ;
#64544=ADVANCED_FACE ( 'NONE', ( #65179 ), #72447, .T. ) ;
#64545=CIRCLE ( 'NONE', #55810, 12.99999999999999822 ) ;
#64546=AXIS2_PLACEMENT_3D ( 'NONE', #36181, #757, #29376 ) ;
#64547=CIRCLE ( 'NONE', #9428, 17.00000000000090239 ) ;
#64548=FACE_OUTER_BOUND ( 'NONE', #63255, .T. ) ;
#64549=CARTESIAN_POINT ( 'NONE',  ( 116.4020974974655047, -33.81230083437814216, 170.0670538473389684 ) ) ;
#64550=CARTESIAN_POINT ( 'NONE',  ( 172.5664832912729878, -27.82844715994070484, 258.9256252759120116 ) ) ;
#64551=ORIENTED_EDGE ( 'NONE', *, *, #56255, .T. ) ;
#64553=CARTESIAN_POINT ( 'NONE',  ( 98.95751068421678553, -41.73716824282166016, 7.768006228290936122 ) ) ;
#64554=DIRECTION ( 'NONE',  ( 1.000000000000000078E-15, -1.000000000000000000, 0.000000000000000000 ) ) ;
#64555=DIRECTION ( 'NONE',  ( -1.000000000000000078E-15, 1.000000000000000083E-30, 1.000000000000000000 ) ) ;
#64559=CARTESIAN_POINT ( 'NONE',  ( 99.40370404213540212, -29.74227323812493751, 230.7261014663879735 ) ) ;
#64561=ORIENTED_EDGE ( 'NONE', *, *, #8218, .F. ) ;
#64562=AXIS2_PLACEMENT_3D ( 'NONE', #71920, #86885, #64648 ) ;
#64563=CARTESIAN_POINT ( 'NONE',  ( 115.6778139412940192, -34.63821234579798158, 205.4472975916109476 ) ) ;
#64564=DIRECTION ( 'NONE',  ( 0.7071067708032339194, 0.0001211784769776690833, -0.7071067811865472397 ) ) ;
#64565=CARTESIAN_POINT ( 'NONE',  ( 102.0302726170450711, -29.40150668315268234, 46.98729759161196284 ) ) ;
#64567=FACE_OUTER_BOUND ( 'NONE', #61409, .T. ) ;
#64568=DIRECTION ( 'NONE',  ( 0.000000000000000000, 1.000000000000000000, 0.000000000000000000 ) ) ;
#64569=ORIENTED_EDGE ( 'NONE', *, *, #35732, .F. ) ;
#64570=CARTESIAN_POINT ( 'NONE',  ( 182.0667039024479550, -33.35206098992058799, 117.4678068554150627 ) ) ;
#64571=CARTESIAN_POINT ( 'NONE',  ( 97.81169266289590780, -40.51741659614882707, 92.63571255866972365 ) ) ;
#64572=CARTESIAN_POINT ( 'NONE',  ( 105.6350724880777392, -47.03380199863529754, 257.4670538473393435 ) ) ;
#64574=EDGE_LOOP ( 'NONE', ( #73868, #21295, #32293, #30671 ) ) ;
#64577=DIRECTION ( 'NONE',  ( 0.1811243268507065352, -0.9834602067307444129, 0.000000000000000000 ) ) ;
#64578=CARTESIAN_POINT ( 'NONE',  ( 32.06670390244800473, -32.29483332968611364, 342.9256252759119548 ) ) ;
#64580=CARTESIAN_POINT ( 'NONE',  ( 72.24325998657057823, -9.906223855237664466, 14.92562527591093691 ) ) ;
#64581=VECTOR ( 'NONE', #12779, 1000.000000000000000 ) ;
#64582=CARTESIAN_POINT ( 'NONE',  ( 111.8051046833288353, -27.50533224649500497, 15.71086337114796549 ) ) ;
#64585=CARTESIAN_POINT ( 'NONE',  ( 104.4799455178094405, -46.91020534057368963, 43.37848241876896083 ) ) ;
#64587=AXIS2_PLACEMENT_3D ( 'NONE', #52842, #87420, #9779 ) ;
#64588=CARTESIAN_POINT ( 'NONE',  ( 101.5973605122076862, -47.27098594307553725, 17.19562527591095247 ) ) ;
#64590=EDGE_CURVE ( 'NONE', #83417, #8508, #52399, .T. ) ;
#64591=CARTESIAN_POINT ( 'NONE',  ( 77.31652006362757845, -36.90534128960240423, 6.749824347015199066 ) ) ;
#64592=CARTESIAN_POINT ( 'NONE',  ( 98.38045758784420514, -41.69533782386550769, 17.73958850095263884 ) ) ;
#64593=ADVANCED_FACE ( 'NONE', ( #87412 ), #10215, .T. ) ;
#64594=LINE ( 'NONE', #2375, #48005 ) ;
#64595=CARTESIAN_POINT ( 'NONE',  ( 106.2913146648166531, -45.97580021205838818, 110.3280903695919903 ) ) ;
#64596=CARTESIAN_POINT ( 'NONE',  ( 98.53347975398118308, -44.98838784992466344, 187.9384824187679612 ) ) ;
#64597=DIRECTION ( 'NONE',  ( 0.000000000000000000, 0.000000000000000000, 1.000000000000000000 ) ) ;
#64598=ORIENTED_EDGE ( 'NONE', *, *, #79148, .F. ) ;
#64599=DIRECTION ( 'NONE',  ( 1.000000000000000000, -5.337610695313248426E-16, 0.000000000000000000 ) ) ;
#64600=ORIENTED_EDGE ( 'NONE', *, *, #16895, .T. ) ;
#64601=ORIENTED_EDGE ( 'NONE', *, *, #43130, .F. ) ;
#64602=VECTOR ( 'NONE', #36056, 1000.000000000000000 ) ;
#64603=DIRECTION ( 'NONE',  ( -0.1858654557293184517, 0.9825752044329902901, 0.000000000000000000 ) ) ;
#64604=ORIENTED_EDGE ( 'NONE', *, *, #71720, .T. ) ;
#64605=ORIENTED_EDGE ( 'NONE', *, *, #22626, .F. ) ;
#64608=CARTESIAN_POINT ( 'NONE',  ( 113.3792027166817320, -43.22269317268541755, 117.6248007804579458 ) ) ;
#64609=CARTESIAN_POINT ( 'NONE',  ( 112.6756251843347627, -45.54329372032184153, 263.0270538473394026 ) ) ;
#64611=ORIENTED_EDGE ( 'NONE', *, *, #18787, .T. ) ;
#64612=ORIENTED_EDGE ( 'NONE', *, *, #66512, .F. ) ;
#64615=CARTESIAN_POINT ( 'NONE',  ( 107.0664832912739257, -49.89611382660765315, 311.6356252759109680 ) ) ;
#64618=ORIENTED_EDGE ( 'NONE', *, *, #26341, .F. ) ;
#64619=CARTESIAN_POINT ( 'NONE',  ( 101.2938852305094173, -26.37968400006201719, 255.4813395616251626 ) ) ;
#64620=CARTESIAN_POINT ( 'NONE',  ( 97.06107111146356203, -37.99641208148336347, 36.42729195195173020 ) ) ;
#64621=PLANE ( 'NONE',  #9725 ) ;
#64622=VECTOR ( 'NONE', #16052, 1000.000000000000000 ) ;
#64625=EDGE_CURVE ( 'NONE', #89932, #19776, #40459, .T. ) ;
#64626=FACE_OUTER_BOUND ( 'NONE', #49522, .T. ) ;
#64628=DIRECTION ( 'NONE',  ( 0.000000000000000000, 1.000000000000000000, 0.000000000000000000 ) ) ;
#64629=CARTESIAN_POINT ( 'NONE',  ( 99.09570904781570277, -30.55043178906333523, 11.80229194609280441 ) ) ;
#64631=CARTESIAN_POINT ( 'NONE',  ( 180.2143765759489895, -35.91149509761070391, -5.074374724088000832 ) ) ;
#64633=CARTESIAN_POINT ( 'NONE',  ( 111.4898014013570560, -26.57429697695857129, 284.7375300378155316 ) ) ;
#64634=CARTESIAN_POINT ( 'NONE',  ( 114.9650091533680722, -29.92534717146685708, 180.3927681330539770 ) ) ;
#64635=CARTESIAN_POINT ( 'NONE',  ( 117.5340331363998985, -37.28601590683526723, 14.78419670448294454 ) ) ;
#64636=DIRECTION ( 'NONE',  ( 4.299999999999999979E-14, -1.000000000000000000, 0.000000000000000000 ) ) ;
#64637=DIRECTION ( 'NONE',  ( 0.000000000000000000, 0.000000000000000000, -1.000000000000000000 ) ) ;
#64638=CARTESIAN_POINT ( 'NONE',  ( 83.06670390244796920, -58.35344715994099829, 231.5838068554150198 ) ) ;
#64641=AXIS2_PLACEMENT_3D ( 'NONE', #68318, #6098, #69210 ) ;
#64645=ORIENTED_EDGE ( 'NONE', *, *, #15049, .F. ) ;
#64646=CARTESIAN_POINT ( 'NONE',  ( 103.8130989789263765, -45.95327097697893493, 53.30705384733897034 ) ) ;
#64647=EDGE_CURVE ( 'NONE', #63602, #58568, #70631, .T. ) ;
#64648=DIRECTION ( 'NONE',  ( -0.7071067811865476838, -0.7071067811865473507, 0.000000000000000000 ) ) ;
#64651=CARTESIAN_POINT ( 'NONE',  ( 95.43233898611183008, -38.84956357215551037, 197.4699109901969791 ) ) ;
#64652=CARTESIAN_POINT ( 'NONE',  ( 161.4809174648185603, -48.32844715993547169, 180.4678068554150059 ) ) ;
#64653=CARTESIAN_POINT ( 'NONE',  ( 110.8600349841776307, -45.98195914306448628, 147.8861036193170264 ) ) ;
#64654=DIRECTION ( 'NONE',  ( 0.000000000000000000, 0.000000000000000000, -1.000000000000000000 ) ) ;
#64655=CARTESIAN_POINT ( 'NONE',  ( 107.0664832912750057, -36.72944715993903486, 0.7256252759109708128 ) ) ;
#64658=DIRECTION ( 'NONE',  ( 0.3818493186865919986, -0.9242245927363031965, 0.000000000000000000 ) ) ;
#64659=CARTESIAN_POINT ( 'NONE',  ( 100.8867824969240559, -44.69965576686789888, 97.05229191759698892 ) ) ;
#64660=CARTESIAN_POINT ( 'NONE',  ( 112.9441315310009628, -44.54716313336201949, 143.0899109901969553 ) ) ;
#64661=EDGE_LOOP ( 'NONE', ( #86593, #45816, #75811, #89076 ) ) ;
#64662=ORIENTED_EDGE ( 'NONE', *, *, #72338, .T. ) ;
#64664=CARTESIAN_POINT ( 'NONE',  ( 102.4863184357179051, -28.52587382674474981, 101.9253928297069791 ) ) ;
#64666=AXIS2_PLACEMENT_3D ( 'NONE', #51784, #30478, #17300 ) ;
#64667=CARTESIAN_POINT ( 'NONE',  ( 184.5667039024485518, -48.82844715993447693, 180.4678068554150343 ) ) ;
#64669=CARTESIAN_POINT ( 'NONE',  ( 101.0349934672011614, -27.38958028709088310, 216.5327681330529686 ) ) ;
#64670=DIRECTION ( 'NONE',  ( 1.000000000000000000, 8.843517682682131024E-16, 1.000000000000000078E-15 ) ) ;
#64673=EDGE_CURVE ( 'NONE', #76993, #17950, #41922, .T. ) ;
#64674=CARTESIAN_POINT ( 'NONE',  ( 99.09569929578050562, -30.55044413325101260, 111.8027284342002048 ) ) ;
#64676=PLANE ( 'NONE',  #52145 ) ;
#64677=DIRECTION ( 'NONE',  ( -1.000000000000000000, -4.299999999999999979E-14, -1.000000000000000078E-15 ) ) ;
#64678=ADVANCED_FACE ( 'NONE', ( #70097 ), #1059, .T. ) ;
#64679=CARTESIAN_POINT ( 'NONE',  ( 105.7232414704440941, -24.98023492732636441, 160.1670538473389627 ) ) ;
#64680=VERTEX_POINT ( 'NONE', #69653 ) ;
#64683=ORIENTED_EDGE ( 'NONE', *, *, #64916, .T. ) ;
#64684=DIRECTION ( 'NONE',  ( 1.175184669632759901E-16, -1.000000000000000000, -2.000000000000003705E-15 ) ) ;
#64685=CARTESIAN_POINT ( 'NONE',  ( 97.81170668756638520, -40.51744870325870806, 152.6352702516163902 ) ) ;
#64686=CARTESIAN_POINT ( 'NONE',  ( 182.4202572930269923, -31.94127993907680718, -5.074374724088000832 ) ) ;
#64687=PLANE ( 'NONE',  #78736 ) ;
#64689=CARTESIAN_POINT ( 'NONE',  ( 111.2851091291901042, -43.74983776777182953, 235.8252332267339852 ) ) ;
#64690=CARTESIAN_POINT ( 'NONE',  ( 117.0608941297925156, -38.08045696544419201, 269.7189583031694156 ) ) ;
#64692=CARTESIAN_POINT ( 'NONE',  ( 118.8775732333442647, -37.69828162312832376, 188.7613395616259595 ) ) ;
#64693=LINE ( 'NONE', #57421, #59059 ) ;
#64695=ORIENTED_EDGE ( 'NONE', *, *, #60546, .T. ) ;
#64696=ORIENTED_EDGE ( 'NONE', *, *, #89848, .T. ) ;
#64697=EDGE_CURVE ( 'NONE', #64904, #8126, #7422, .T. ) ;
#64701=DIRECTION ( 'NONE',  ( -1.000000000000000000, 0.000000000000000000, 0.000000000000000000 ) ) ;
#64704=EDGE_CURVE ( 'NONE', #34216, #14767, #8784, .T. ) ;
#64705=CARTESIAN_POINT ( 'NONE',  ( 110.3188062821955242, -28.45390942821411429, 266.2101547344684604 ) ) ;
#64707=ORIENTED_EDGE ( 'NONE', *, *, #53755, .F. ) ;
#64709=CARTESIAN_POINT ( 'NONE',  ( 105.4444412749903677, -44.73895730596940723, 9.635625275910939536 ) ) ;
#64711=ORIENTED_EDGE ( 'NONE', *, *, #76335, .F. ) ;
#64712=EDGE_LOOP ( 'NONE', ( #77100, #7948 ) ) ;
#64713=FACE_OUTER_BOUND ( 'NONE', #58856, .T. ) ;
#64715=VERTEX_POINT ( 'NONE', #8326 ) ;
#64716=CARTESIAN_POINT ( 'NONE',  ( 115.6047007430436366, -36.96391350797230757, 43.22670554236196239 ) ) ;
#64717=CARTESIAN_POINT ( 'NONE',  ( 117.4794452684060104, -40.50643855513092007, 173.5375300378159693 ) ) ;
#64718=CARTESIAN_POINT ( 'NONE',  ( 95.69905522618344662, -33.46911247776736786, 141.1041967044829732 ) ) ;
#64719=DIRECTION ( 'NONE',  ( 1.000000000000000000, 4.163336342344333240E-14, 0.000000000000000000 ) ) ;
#64720=CARTESIAN_POINT ( 'NONE',  ( 117.4913186190917855, -36.80221964929349809, 259.8213395616249386 ) ) ;
#64721=CARTESIAN_POINT ( 'NONE',  ( 156.5667039024484097, -42.82844715993568485, 175.7178068554150059 ) ) ;
#64724=ORIENTED_EDGE ( 'NONE', *, *, #81334, .T. ) ;
#64728=AXIS2_PLACEMENT_3D ( 'NONE', #62046, #34793, #35234 ) ;
#64729=CARTESIAN_POINT ( 'NONE',  ( 104.5519768891453651, -48.36156025571956718, 182.4070538473399665 ) ) ;
#64730=VERTEX_POINT ( 'NONE', #1962 ) ;
#64731=CARTESIAN_POINT ( 'NONE',  ( 98.09046607155295305, -42.10132104613245474, 161.7556252759109725 ) ) ;
#64732=LINE ( 'NONE', #49297, #63067 ) ;
#64733=CIRCLE ( 'NONE', #79274, 2.517500000000005844 ) ;
#64734=CARTESIAN_POINT ( 'NONE',  ( 127.0664832912740110, -46.72944715994101017, 14.67562527591099197 ) ) ;
#64736=CARTESIAN_POINT ( 'NONE',  ( 98.00804396577686362, -39.67311905263231608, 277.6356252759111385 ) ) ;
#64737=DIRECTION ( 'NONE',  ( 0.000000000000000000, 0.000000000000000000, -1.000000000000000000 ) ) ;
#64738=CARTESIAN_POINT ( 'NONE',  ( 98.95962429139169103, -30.20966935044063462, 236.7870538473399336 ) ) ;
#64743=CARTESIAN_POINT ( 'NONE',  ( 113.1782937836032659, -44.75186858293219672, 259.0939586104858563 ) ) ;
#64744=CARTESIAN_POINT ( 'NONE',  ( 126.8164832912740394, -46.47944715994101017, -5.074374724089010691 ) ) ;
#64745=CARTESIAN_POINT ( 'NONE',  ( 115.3517163442624707, -37.78381771408454171, 195.5838068554166966 ) ) ;
#64747=CARTESIAN_POINT ( 'NONE',  ( 131.0667039024480118, -61.87844715994100397, 207.5838068554149913 ) ) ;
#64748=CARTESIAN_POINT ( 'NONE',  ( 98.53312381531716824, -44.98873235655736380, 191.9384824187679612 ) ) ;
#64749=CARTESIAN_POINT ( 'NONE',  ( 107.3210293350295501, -25.67914459413323058, 71.04610146638795243 ) ) ;
#64750=CARTESIAN_POINT ( 'NONE',  ( 96.60079736239889314, -36.47965167166085365, 192.3070538473399438 ) ) ;
#64751=CARTESIAN_POINT ( 'NONE',  ( 72.26648329127297643, -71.52944715994141234, 352.4506252759078961 ) ) ;
#64752=DIRECTION ( 'NONE',  ( -1.000000000000000078E-15, 1.000000000000000083E-30, 1.000000000000000000 ) ) ;
#64753=AXIS2_PLACEMENT_3D ( 'NONE', #27129, #12612, #41632 ) ;
#64756=DIRECTION ( 'NONE',  ( 0.000000000000000000, 0.000000000000000000, -1.000000000000000000 ) ) ;
#64757=PLANE ( 'NONE',  #19469 ) ;
#64758=EDGE_LOOP ( 'NONE', ( #57534, #22445, #29087, #77847 ) ) ;
#64762=ORIENTED_EDGE ( 'NONE', *, *, #26669, .T. ) ;
#64763=ADVANCED_FACE ( 'NONE', ( #50084 ), #43269, .T. ) ;
#64765=CARTESIAN_POINT ( 'NONE',  ( 115.9068402959922111, -38.69432841718559501, 103.0628960185529763 ) ) ;
#64766=EDGE_CURVE ( 'NONE', #3629, #11834, #13790, .T. ) ;
#64769=CARTESIAN_POINT ( 'NONE',  ( 101.7220374796297335, -27.76276858577408291, 81.50419670448295051 ) ) ;
#64771=DIRECTION ( 'NONE',  ( 0.000000000000000000, 0.000000000000000000, 1.000000000000000000 ) ) ;
#64772=ADVANCED_FACE ( 'NONE', ( #6977 ), #27422, .T. ) ;
#64773=EDGE_CURVE ( 'NONE', #84886, #72226, #34681, .T. ) ;
#64774=CYLINDRICAL_SURFACE ( 'NONE', #82487, 0.5000000000000004441 ) ;
#64775=CARTESIAN_POINT ( 'NONE',  ( 100.9534786964907482, -28.35269599622599301, 30.56610146638794134 ) ) ;
#64776=ORIENTED_EDGE ( 'NONE', *, *, #4192, .T. ) ;
#64777=ORIENTED_EDGE ( 'NONE', *, *, #2556, .F. ) ;
#64778=ORIENTED_EDGE ( 'NONE', *, *, #24705, .T. ) ;
#64780=CARTESIAN_POINT ( 'NONE',  ( 51.42025729302656600, -31.94127993907661889, 313.9678068554150059 ) ) ;
#64781=CYLINDRICAL_SURFACE ( 'NONE', #85382, 16.00000000000090239 ) ;
#64782=LINE ( 'NONE', #30704, #8651 ) ;
#64784=CARTESIAN_POINT ( 'NONE',  ( 180.3503142329366824, -29.99615139351640636, 313.9678068554149490 ) ) ;
#64786=CARTESIAN_POINT ( 'NONE',  ( 102.0674824855994842, -27.97024723768227261, 51.49124353025893441 ) ) ;
#64787=CARTESIAN_POINT ( 'NONE',  ( 182.5667039024469886, -33.35206098992650681, 193.9678068554150059 ) ) ;
#64789=CARTESIAN_POINT ( 'NONE',  ( 104.0490797691969647, -47.33883444496888160, 67.36800622829191809 ) ) ;
#64791=ORIENTED_EDGE ( 'NONE', *, *, #42687, .T. ) ;
#64792=CARTESIAN_POINT ( 'NONE',  ( 100.9546734967587156, -28.70702521494872173, 270.5939585418061029 ) ) ;
#64795=CARTESIAN_POINT ( 'NONE',  ( 115.2991214174112002, -34.06025354975611918, 131.9061856076869788 ) ) ;
#64796=EDGE_CURVE ( 'NONE', #60920, #137, #57351, .T. ) ;
#64797=AXIS2_PLACEMENT_3D ( 'NONE', #30497, #15983, #71838 ) ;
#64801=CARTESIAN_POINT ( 'NONE',  ( 97.81168883536605563, -40.51740680051663190, 96.63562987897269352 ) ) ;
#64802=DIRECTION ( 'NONE',  ( 0.000000000000000000, 1.000000000000000000, 0.000000000000000000 ) ) ;
#64805=CARTESIAN_POINT ( 'NONE',  ( 97.83897911476498166, -40.58352276682783355, 136.6416734916348616 ) ) ;
#64806=ORIENTED_EDGE ( 'NONE', *, *, #10906, .F. ) ;
#64807=ORIENTED_EDGE ( 'NONE', *, *, #13072, .T. ) ;
#64809=CARTESIAN_POINT ( 'NONE',  ( 106.9887167903908392, -45.59072421142732168, 184.0015833058969577 ) ) ;
#64810=FACE_OUTER_BOUND ( 'NONE', #66136, .T. ) ;
#64811=EDGE_CURVE ( 'NONE', #85401, #43446, #65951, .T. ) ;
#64812=CIRCLE ( 'NONE', #21241, 0.9999999999999974465 ) ;
#64813=CARTESIAN_POINT ( 'NONE',  ( 109.2058805625337925, -26.50397703278076733, 135.9127681330539872 ) ) ;
#64814=DIRECTION ( 'NONE',  ( 1.000000000000000000, 3.999999999999999995E-14, 1.000000000000000078E-15 ) ) ;
#64815=CARTESIAN_POINT ( 'NONE',  ( 116.9194122960482929, -38.69773298920891591, 18.66981024198805628 ) ) ;
#64817=VERTEX_POINT ( 'NONE', #24626 ) ;
#64819=CARTESIAN_POINT ( 'NONE',  ( 111.7296936849409406, -43.46273440104761221, 200.8766617981629565 ) ) ;
#64820=CARTESIAN_POINT ( 'NONE',  ( 95.32417067969559810, -34.95402877631575222, 71.20705384733993526 ) ) ;
#64822=CARTESIAN_POINT ( 'NONE',  ( 100.5643946202652330, -27.81952766013690237, 30.56610146638794134 ) ) ;
#64823=CARTESIAN_POINT ( 'NONE',  ( 96.62257978078039855, -36.48017157545621814, 192.3070538473399438 ) ) ;
#64824=LINE ( 'NONE', #15343, #14717 ) ;
#64826=CARTESIAN_POINT ( 'NONE',  ( 109.0722782120600840, -47.59916505968618594, 123.7337205140059666 ) ) ;
#64830=EDGE_CURVE ( 'NONE', #18386, #75279, #30108, .T. ) ;
#64833=ORIENTED_EDGE ( 'NONE', *, *, #26418, .T. ) ;
#64834=ORIENTED_EDGE ( 'NONE', *, *, #79452, .F. ) ;
#64835=VECTOR ( 'NONE', #34459, 1000.000000000000114 ) ;
#64837=CARTESIAN_POINT ( 'NONE',  ( 107.0664832912750057, -36.72944715993903486, 9.425625275910970657 ) ) ;
#64838=CARTESIAN_POINT ( 'NONE',  ( 114.5019750680372113, -29.98747414221284302, 130.4130031197996402 ) ) ;
#64839=CARTESIAN_POINT ( 'NONE',  ( 96.95653860995706452, -32.26087848594701057, 55.98324432352897162 ) ) ;
#64841=DIRECTION ( 'NONE',  ( 1.000000000000000000, 0.000000000000000000, 0.000000000000000000 ) ) ;
#64842=CARTESIAN_POINT ( 'NONE',  ( 151.0371591254584587, -46.82818131005592477, 193.9678068554149775 ) ) ;
#64843=CARTESIAN_POINT ( 'NONE',  ( 104.1495640007033217, -46.68084741754461220, 62.33753003781600199 ) ) ;
#64844=CARTESIAN_POINT ( 'NONE',  ( 25.56670390244797275, -62.87844715994099687, 288.3428068554150059 ) ) ;
#64845=CARTESIAN_POINT ( 'NONE',  ( 101.9826776100855881, -46.51815199768660847, 163.1832443235299763 ) ) ;
#64846=CARTESIAN_POINT ( 'NONE',  ( 115.8228084649852860, -31.72548357239955763, 59.24020506417635801 ) ) ;
#64848=ORIENTED_EDGE ( 'NONE', *, *, #28781, .T. ) ;
#64853=CARTESIAN_POINT ( 'NONE',  ( 110.7116931949060614, -48.05822654157750407, 207.8241967044819489 ) ) ;
#64857=CARTESIAN_POINT ( 'NONE',  ( 96.49610902845032001, -31.31747537214017640, 241.9499109901969689 ) ) ;
#64858=CARTESIAN_POINT ( 'NONE',  ( 96.59840162804212582, -36.61878533396502888, 107.3184824187679567 ) ) ;
#64862=EDGE_CURVE ( 'NONE', #49976, #31872, #9223, .T. ) ;
#64864=ORIENTED_EDGE ( 'NONE', *, *, #52896, .T. ) ;
#64865=AXIS2_PLACEMENT_3D ( 'NONE', #34122, #13690, #54545 ) ;
#64866=VECTOR ( 'NONE', #61871, 1000.000000000000000 ) ;
#64868=EDGE_CURVE ( 'NONE', #84879, #41258, #17813, .T. ) ;
#64869=ORIENTED_EDGE ( 'NONE', *, *, #30209, .T. ) ;
#64871=ORIENTED_EDGE ( 'NONE', *, *, #43210, .T. ) ;
#64873=ORIENTED_EDGE ( 'NONE', *, *, #78640, .F. ) ;
#64874=CYLINDRICAL_SURFACE ( 'NONE', #56852, 1.000000000002049694 ) ;
#64875=CARTESIAN_POINT ( 'NONE',  ( 112.1867106929447573, -26.95862322015898016, 10.68038718067299087 ) ) ;
#64879=CARTESIAN_POINT ( 'NONE',  ( 107.0664832912750057, -36.72944715993903486, 0.7256252759109708128 ) ) ;
#64881=DIRECTION ( 'NONE',  ( 0.000000000000000000, 1.000000000000000000, 0.000000000000000000 ) ) ;
#64882=CIRCLE ( 'NONE', #43068, 13.31747058675099993 ) ;
#64883=CARTESIAN_POINT ( 'NONE',  ( 115.5441482490607257, -35.68765611295631857, 193.3467055423629688 ) ) ;
#64887=VECTOR ( 'NONE', #84302, 1000.000000000000000 ) ;
#64888=EDGE_CURVE ( 'NONE', #57610, #45317, #17370, .T. ) ;
#64889=DIRECTION ( 'NONE',  ( 1.000000000000000000, 0.000000000000000000, 0.000000000000000000 ) ) ;
#64891=CARTESIAN_POINT ( 'NONE',  ( 116.8470136369841725, -36.79772195930840439, 259.8213395616247681 ) ) ;
#64893=DIRECTION ( 'NONE',  ( 1.017460296392624983E-15, 1.000000000000000000, 0.000000000000000000 ) ) ;
#64894=CARTESIAN_POINT ( 'NONE',  ( 112.0650656126721429, -45.48886803529176603, 27.98971541558280052 ) ) ;
#64895=ORIENTED_EDGE ( 'NONE', *, *, #64766, .T. ) ;
#64896=CARTESIAN_POINT ( 'NONE',  ( 77.51853161617805199, -35.69475198630856738, 2.828485944707570532 ) ) ;
#64899=CARTESIAN_POINT ( 'NONE',  ( 114.6641587241874873, -32.58502278776634142, 22.02999513149600475 ) ) ;
#64900=AXIS2_PLACEMENT_3D ( 'NONE', #65200, #22536, #9344 ) ;
#64901=CARTESIAN_POINT ( 'NONE',  ( 136.8164812439618743, -18.63640413216975844, 6.749771997051317918 ) ) ;
#64902=FACE_OUTER_BOUND ( 'NONE', #12647, .T. ) ;
#64903=CARTESIAN_POINT ( 'NONE',  ( 191.6377717143134873, -67.87844715994100397, 13.84673904354931651 ) ) ;
#64904=VERTEX_POINT ( 'NONE', #50537 ) ;
#64905=CARTESIAN_POINT ( 'NONE',  ( 41.56670390244689628, -36.32844715994109208, 180.4678068554150911 ) ) ;
#64906=CARTESIAN_POINT ( 'NONE',  ( 131.0667039024480118, -58.35344715994099829, 210.8338068554149913 ) ) ;
#64908=CARTESIAN_POINT ( 'NONE',  ( 96.08737379349030050, -38.00938547453511518, 86.43086337114897333 ) ) ;
#64910=CARTESIAN_POINT ( 'NONE',  ( 105.7183000297088284, -45.16381338481517815, 36.87241982807598362 ) ) ;
#64911=CARTESIAN_POINT ( 'NONE',  ( 107.7442340506927252, -46.73693967930866933, 88.62940955498838491 ) ) ;
#64912=CARTESIAN_POINT ( 'NONE',  ( 98.73617028912649118, -32.38405755445656808, 87.36348806780198117 ) ) ;
#64913=CARTESIAN_POINT ( 'NONE',  ( 105.7147715443256715, -46.72375139838595004, 13.46890240877466383 ) ) ;
#64915=VECTOR ( 'NONE', #69532, 1000.000000000000000 ) ;
#64916=EDGE_CURVE ( 'NONE', #89511, #88009, #16043, .T. ) ;
#64918=CARTESIAN_POINT ( 'NONE',  ( 99.34942397265413661, -29.65555323683921074, 271.7356252759109907 ) ) ;
#64920=ORIENTED_EDGE ( 'NONE', *, *, #53660, .F. ) ;
#64921=LINE ( 'NONE', #58102, #53075 ) ;
#64922=VERTEX_POINT ( 'NONE', #19162 ) ;
#64923=CARTESIAN_POINT ( 'NONE',  ( 114.4937323636162176, -28.48121435373123589, 155.5051490854349652 ) ) ;
#64924=AXIS2_PLACEMENT_3D ( 'NONE', #12937, #40166, #81546 ) ;
#64925=CARTESIAN_POINT ( 'NONE',  ( 79.87807227642528574, -21.47944715994105991, 1.625625275910942635 ) ) ;
#64926=EDGE_LOOP ( 'NONE', ( #61963, #82379 ) ) ;
#64929=CYLINDRICAL_SURFACE ( 'NONE', #33353, 0.5000000000000073275 ) ;
#64930=CARTESIAN_POINT ( 'NONE',  ( 34.67381068360336371, -28.98061976759059988, 193.9678068554150911 ) ) ;
#64931=CARTESIAN_POINT ( 'NONE',  ( 116.2522929705883712, -40.08866370952549829, 218.5470538473399529 ) ) ;
#64932=CARTESIAN_POINT ( 'NONE',  ( 107.0667039024479834, -18.72944715994100306, 239.5838068554170377 ) ) ;
#64934=CARTESIAN_POINT ( 'NONE',  ( 31.89136050872298966, -31.76306994223740432, -5.074374724088000832 ) ) ;
#64935=CARTESIAN_POINT ( 'NONE',  ( 96.68927247633037325, -32.92320750051204215, 17.03467289495896964 ) ) ;
#64937=ORIENTED_EDGE ( 'NONE', *, *, #29983, .F. ) ;
#64939=CARTESIAN_POINT ( 'NONE',  ( 97.60786201319120892, -39.98234442571827429, 172.5900479121347928 ) ) ;
#64942=CARTESIAN_POINT ( 'NONE',  ( 117.0608951760848555, -38.08044937632849525, 43.71866473332352143 ) ) ;
#64943=ORIENTED_EDGE ( 'NONE', *, *, #68202, .F. ) ;
#64946=CARTESIAN_POINT ( 'NONE',  ( 81.77804793994209831, -20.88970947304156311, 2.099345637348018823 ) ) ;
#64947=CARTESIAN_POINT ( 'NONE',  ( 31.56670390244800828, -32.29483332968611364, -5.074374724088000832 ) ) ;
#64948=CARTESIAN_POINT ( 'NONE',  ( 105.6350724880777392, -47.03380199863529754, 257.4670538473393435 ) ) ;
#64950=DIRECTION ( 'NONE',  ( 0.9068632946707807507, -0.4214249218767881500, 9.028300618466658994E-16 ) ) ;
#64952=CARTESIAN_POINT ( 'NONE',  ( 110.3936857311090023, -28.86269079874493571, 244.1809912566479568 ) ) ;
#64953=FACE_OUTER_BOUND ( 'NONE', #13579, .T. ) ;
#64954=CARTESIAN_POINT ( 'NONE',  ( 116.7246412902988908, -32.86309880586080823, 50.12991099019698282 ) ) ;
#64956=CARTESIAN_POINT ( 'NONE',  ( 117.3823636748946058, -32.63121637840519895, 99.13943479972098771 ) ) ;
#64957=VERTEX_POINT ( 'NONE', #33235 ) ;
#64958=CARTESIAN_POINT ( 'NONE',  ( 131.4241199117880683, -19.49143581485983034, 6.902478035882034568 ) ) ;
#64959=ORIENTED_EDGE ( 'NONE', *, *, #38621, .F. ) ;
#64962=ORIENTED_EDGE ( 'NONE', *, *, #12979, .F. ) ;
#64964=CARTESIAN_POINT ( 'NONE',  ( 116.3212776292296127, -32.94146857471318413, 287.6356252759109680 ) ) ;
#64967=DIRECTION ( 'NONE',  ( 0.9999999853157766072, 0.0001713722456134972175, 0.000000000000000000 ) ) ;
#64968=VECTOR ( 'NONE', #7887, 1000.000000000000114 ) ;
#64969=CARTESIAN_POINT ( 'NONE',  ( 123.6837132603318992, -53.34645651782490461, 239.5838068554164693 ) ) ;
#64970=ORIENTED_EDGE ( 'NONE', *, *, #38035, .T. ) ;
#64971=CARTESIAN_POINT ( 'NONE',  ( 98.28768183251310120, -28.73153112808589427, 80.73848241876795839 ) ) ;
#64972=DIRECTION ( 'NONE',  ( 1.346944695195362088E-15, -1.000000000000000000, 3.469446951953620425E-31 ) ) ;
#64975=ORIENTED_EDGE ( 'NONE', *, *, #26072, .T. ) ;
#64977=EDGE_CURVE ( 'NONE', #52826, #77857, #18705, .T. ) ;
#64978=CARTESIAN_POINT ( 'NONE',  ( 183.6524903400783444, -49.32844715993451956, 300.4678068554149490 ) ) ;
#64979=DIRECTION ( 'NONE',  ( 0.000000000000000000, -1.000000000000000000, 0.000000000000000000 ) ) ;
#64982=ADVANCED_FACE ( 'NONE', ( #4186 ), #60934, .F. ) ;
#64983=B_SPLINE_CURVE_WITH_KNOTS ( 'NONE', 3,
 ( #65857, #72700, #86773, #3213, #10466, #38167 ),
 .UNSPECIFIED., .F., .F.,
 ( 4, 2, 4 ),
 ( 0.000000000000000000, 0.05514354140252886172, 0.1102870828050577234 ),
 .UNSPECIFIED. ) ;
#64984=DIRECTION ( 'NONE',  ( -4.237773401492740281E-14, 1.000000000000000000, 0.000000000000000000 ) ) ;
#64985=DIRECTION ( 'NONE',  ( 0.9242245927363033076, 0.3818493186865918876, 0.000000000000000000 ) ) ;
#64987=VECTOR ( 'NONE', #72140, 1000.000000000000000 ) ;
#64989=AXIS2_PLACEMENT_3D ( 'NONE', #79162, #16923, #37357 ) ;
#64990=DIRECTION ( 'NONE',  ( 0.000000000000000000, 0.000000000000000000, 1.000000000000000000 ) ) ;
#64991=CARTESIAN_POINT ( 'NONE',  ( 97.29384000864243376, -37.12803473146956890, 157.3584824187679487 ) ) ;
#64992=EDGE_CURVE ( 'NONE', #89473, #7800, #25944, .T. ) ;
#64994=ORIENTED_EDGE ( 'NONE', *, *, #20573, .F. ) ;
#64995=AXIS2_PLACEMENT_3D ( 'NONE', #85492, #72731, #79562 ) ;
#64996=CARTESIAN_POINT ( 'NONE',  ( 107.1874307469290244, -26.94942635195924652, 31.06705384733893283 ) ) ;
#64997=CARTESIAN_POINT ( 'NONE',  ( 49.21213752015869858, -29.73316016639558512, 193.9678068554150911 ) ) ;
#64998=CARTESIAN_POINT ( 'NONE',  ( 97.82529242725978236, -40.55051696138422557, 51.63847270892774333 ) ) ;
#64999=CARTESIAN_POINT ( 'NONE',  ( 99.04383725273962114, -42.84092021590794275, 11.84399581657901379 ) ) ;
#65002=AXIS2_PLACEMENT_3D ( 'NONE', #5358, #61205, #32598 ) ;
#65003=CIRCLE ( 'NONE', #69356, 2.500000000000002220 ) ;
#65004=CARTESIAN_POINT ( 'NONE',  ( 101.9853755998761073, -45.08682593082395584, 247.1413395616259550 ) ) ;
#65007=CARTESIAN_POINT ( 'NONE',  ( 101.0667092185316989, -28.63788266170726260, 182.0158690201829756 ) ) ;
#65008=CARTESIAN_POINT ( 'NONE',  ( 116.3212776292269837, -32.94146857470673240, 74.13562527591093954 ) ) ;
#65009=CARTESIAN_POINT ( 'NONE',  ( 116.4244759746951985, -37.56879123375174601, 30.17491663923099665 ) ) ;
#65011=DIRECTION ( 'NONE',  ( 0.000000000000000000, 0.000000000000000000, -1.000000000000000000 ) ) ;
#65012=CIRCLE ( 'NONE', #63590, 2.999999999999999112 ) ;
#65016=LINE ( 'NONE', #65460, #61849 ) ;
#65017=CARTESIAN_POINT ( 'NONE',  ( 106.5683798796750779, -47.15615894637593897, 247.5384824187679556 ) ) ;
#65018=CYLINDRICAL_SURFACE ( 'NONE', #75112, 10.04999999999999361 ) ;
#65019=ORIENTED_EDGE ( 'NONE', *, *, #72773, .F. ) ;
#65020=PLANE ( 'NONE',  #45951 ) ;
#65021=DIRECTION ( 'NONE',  ( 1.000000000000000000, 4.163336342344333240E-14, 0.000000000000000000 ) ) ;
#65022=DIRECTION ( 'NONE',  ( -0.9254794337955620787, -0.3787978585227822492, 0.000000000000000000 ) ) ;
#65023=DIRECTION ( 'NONE',  ( 0.000000000000000000, -1.000000000000000000, 0.000000000000000000 ) ) ;
#65024=AXIS2_PLACEMENT_3D ( 'NONE', #36871, #86369, #15993 ) ;
#65027=CARTESIAN_POINT ( 'NONE',  ( 116.8435662018513028, -36.99793375417353758, 39.80419670448193159 ) ) ;
#65028=DIRECTION ( 'NONE',  ( 0.000000000000000000, 0.000000000000000000, 1.000000000000000000 ) ) ;
#65029=ORIENTED_EDGE ( 'NONE', *, *, #44797, .T. ) ;
#65030=CARTESIAN_POINT ( 'NONE',  ( 116.4265620360770725, -31.96216903954944399, 40.20133956162496958 ) ) ;
#65032=EDGE_CURVE ( 'NONE', #26697, #36849, #88218, .T. ) ;
#65033=CARTESIAN_POINT ( 'NONE',  ( 118.1032226039154267, -36.12160442421116358, 273.8822919425776945 ) ) ;
#65035=CARTESIAN_POINT ( 'NONE',  ( 82.73250004807569269, -18.03188439721439096, 2.979900720421670979 ) ) ;
#65036=CARTESIAN_POINT ( 'NONE',  ( 98.54772661365011288, -41.97710352008375168, 17.76566672626352528 ) ) ;
#65038=CARTESIAN_POINT ( 'NONE',  ( 108.2186271136511095, -28.64846388872622285, 102.7823760838769687 ) ) ;
#65039=CARTESIAN_POINT ( 'NONE',  ( 109.6111442688334563, -26.56067652042401406, 195.8813395616249977 ) ) ;
#65041=PLANE ( 'NONE',  #7287 ) ;
#65043=VECTOR ( 'NONE', #76120, 1000.000000000000000 ) ;
#65044=DIRECTION ( 'NONE',  ( 1.000000000000000000, 0.000000000000000000, 9.868649107779159826E-16 ) ) ;
#65045=ORIENTED_EDGE ( 'NONE', *, *, #54686, .F. ) ;
#65046=ORIENTED_EDGE ( 'NONE', *, *, #34286, .T. ) ;
#65048=VECTOR ( 'NONE', #85331, 1000.000000000000000 ) ;
#65050=DIRECTION ( 'NONE',  ( -2.999999999999999839E-15, 1.000000000000000000, -2.999999999999999900E-30 ) ) ;
#65052=ORIENTED_EDGE ( 'NONE', *, *, #23681, .F. ) ;
#65054=CARTESIAN_POINT ( 'NONE',  ( 110.9595727330559072, -27.46627978870682441, 40.76010958015512387 ) ) ;
#65055=CARTESIAN_POINT ( 'NONE',  ( 103.2375202873391800, -28.52263824056898756, 134.8343245899819465 ) ) ;
#65056=CARTESIAN_POINT ( 'NONE',  ( 95.20615018136085439, -37.33485150947186781, 271.3670538473392639 ) ) ;
#65059=ORIENTED_EDGE ( 'NONE', *, *, #48532, .T. ) ;
#65060=CIRCLE ( 'NONE', #79539, 10.00000000000000711 ) ;
#65061=EDGE_CURVE ( 'NONE', #69092, #49439, #5080, .T. ) ;
#65062=CARTESIAN_POINT ( 'NONE',  ( 114.7429578716709386, -30.29548818356803608, 135.3815280204426017 ) ) ;
#65065=VECTOR ( 'NONE', #44946, 1000.000000000000000 ) ;
#65066=LINE ( 'NONE', #85534, #24146 ) ;
#65067=CARTESIAN_POINT ( 'NONE',  ( 98.04152589100374371, -41.04187113461722447, 131.6812034471568040 ) ) ;
#65069=VERTEX_POINT ( 'NONE', #67754 ) ;
#65070=CARTESIAN_POINT ( 'NONE',  ( 100.2471064434660093, -45.42859581790747825, 277.0594347997204636 ) ) ;
#65071=CARTESIAN_POINT ( 'NONE',  ( 99.09426955137945470, -44.45222557475181446, 37.95086337114900488 ) ) ;
#65072=CARTESIAN_POINT ( 'NONE',  ( 116.8171228667130634, -34.15291832109217296, 120.0314586092066520 ) ) ;
#65075=LINE ( 'NONE', #68212, #81549 ) ;
#65077=CARTESIAN_POINT ( 'NONE',  ( 131.3780189692434703, -37.30949827216404913, 6.839365140900705242 ) ) ;
#65080=EDGE_CURVE ( 'NONE', #39780, #8105, #54093, .T. ) ;
#65081=CARTESIAN_POINT ( 'NONE',  ( 100.8875763982592844, -44.70031131295115756, 162.0521131232090397 ) ) ;
#65082=CARTESIAN_POINT ( 'NONE',  ( 134.0664832912739826, -8.729447159941003065, 4.925625275910997303 ) ) ;
#65083=CARTESIAN_POINT ( 'NONE',  ( 131.0667039024480118, -61.87844715994100397, 228.3338068554150198 ) ) ;
#65084=CARTESIAN_POINT ( 'NONE',  ( 109.2165397428488376, -48.40897078886088423, 277.7213395616254843 ) ) ;
#65085=CARTESIAN_POINT ( 'NONE',  ( 96.04670619665022002, -35.87009084903410638, 187.2765776568629406 ) ) ;
#65086=CARTESIAN_POINT ( 'NONE',  ( 117.9472974416529638, -41.48656121291797660, 54.49848241876792088 ) ) ;
#65087=FACE_OUTER_BOUND ( 'NONE', #83095, .T. ) ;
#65088=CARTESIAN_POINT ( 'NONE',  ( 75.31670390244798341, -67.87844715994100397, 60.91780685541480267 ) ) ;
#65089=CARTESIAN_POINT ( 'NONE',  ( 82.51836309791163160, -35.48272428399237555, 2.716753546975698264 ) ) ;
#65090=AXIS2_PLACEMENT_3D ( 'NONE', #7796, #69130, #33714 ) ;
#65091=ORIENTED_EDGE ( 'NONE', *, *, #46823, .T. ) ;
#65092=CARTESIAN_POINT ( 'NONE',  ( 177.0371591254545933, -48.62818131005479927, 129.9678068554150059 ) ) ;
#65093=ORIENTED_EDGE ( 'NONE', *, *, #36985, .T. ) ;
#65094=CARTESIAN_POINT ( 'NONE',  ( 97.00151786184787284, -41.45262973156711439, 57.67562527591096710 ) ) ;
#65095=EDGE_CURVE ( 'NONE', #87937, #53694, #61377, .T. ) ;
#65097=VERTEX_POINT ( 'NONE', #75015 ) ;
#65098=FACE_OUTER_BOUND ( 'NONE', #88752, .T. ) ;
#65099=CARTESIAN_POINT ( 'NONE',  ( 117.1759530674218865, -34.27439392744689428, 205.0156252759109634 ) ) ;
#65101=CARTESIAN_POINT ( 'NONE',  ( 98.38057750414245106, -41.69554516216643947, 146.7398124929533196 ) ) ;
#65103=DIRECTION ( 'NONE',  ( 0.7071067811865491270, -0.7071067811865459074, 7.071067811865492096E-16 ) ) ;
#65106=CYLINDRICAL_SURFACE ( 'NONE', #51479, 4.750000000000000888 ) ;
#65107=CARTESIAN_POINT ( 'NONE',  ( 97.25364341294451265, -36.87759583893578252, 136.3384824187689333 ) ) ;
#65110=CARTESIAN_POINT ( 'NONE',  ( 100.0889724914296863, -42.24093267880301994, 88.29015473446894191 ) ) ;
#65111=VECTOR ( 'NONE', #61428, 1000.000000000000000 ) ;
#65112=DIRECTION ( 'NONE',  ( 0.000000000000000000, 0.000000000000000000, -1.000000000000000000 ) ) ;
#65113=CARTESIAN_POINT ( 'NONE',  ( 97.40895461294502411, -34.98419235835276453, 237.1841967044819626 ) ) ;
#65115=CARTESIAN_POINT ( 'NONE',  ( 182.3467384525658019, -29.62846900981657683, 117.4678068554150627 ) ) ;
#65116=DIRECTION ( 'NONE',  ( -0.02150753337723538411, -0.0009076677972193728959, -0.9997682742251812194 ) ) ;
#65118=VECTOR ( 'NONE', #46347, 1000.000000000000000 ) ;
#65120=DIRECTION ( 'NONE',  ( 9.000537910253610245E-13, -1.000000000000000000, 9.010537910253610534E-28 ) ) ;
#65122=CARTESIAN_POINT ( 'NONE',  ( 95.59354794629800267, -39.59649474372138656, 166.5213395616259788 ) ) ;
#65123=VERTEX_POINT ( 'NONE', #80499 ) ;
#65125=AXIS2_PLACEMENT_3D ( 'NONE', #19640, #40531, #11941 ) ;
#65127=LINE ( 'NONE', #45540, #78106 ) ;
#65128=AXIS2_PLACEMENT_3D ( 'NONE', #77941, #21639, #15712 ) ;
#65130=FACE_OUTER_BOUND ( 'NONE', #14430, .T. ) ;
#65131=CARTESIAN_POINT ( 'NONE',  ( 98.50976710839005079, -35.43193677023271704, 219.0128522743539747 ) ) ;
#65134=CARTESIAN_POINT ( 'NONE',  ( 104.4536708109005332, -26.63686367483539996, 200.2784824187679362 ) ) ;
#65135=CARTESIAN_POINT ( 'NONE',  ( 25.56670390244797275, -62.87844715994099687, 257.2178068554150059 ) ) ;
#65136=ORIENTED_EDGE ( 'NONE', *, *, #17692, .F. ) ;
#65137=ORIENTED_EDGE ( 'NONE', *, *, #4784, .T. ) ;
#65138=VERTEX_POINT ( 'NONE', #40932 ) ;
#65139=AXIS2_PLACEMENT_3D ( 'NONE', #29991, #57680, #85423 ) ;
#65142=CARTESIAN_POINT ( 'NONE',  ( 131.5441285970327101, -35.63380991826300459, 7.053480412778572628 ) ) ;
#65143=CARTESIAN_POINT ( 'NONE',  ( 109.5858817268311611, -44.49374890974875285, 10.64523322673399619 ) ) ;
#65144=DIRECTION ( 'NONE',  ( -4.237773401492740281E-14, 1.000000000000000000, 0.000000000000000000 ) ) ;
#65146=CARTESIAN_POINT ( 'NONE',  ( 116.7802871385218282, -39.10473973501323286, 9.635625275910941312 ) ) ;
#65147=VECTOR ( 'NONE', #60631, 1000.000000000000000 ) ;
#65149=ORIENTED_EDGE ( 'NONE', *, *, #21146, .F. ) ;
#65152=CARTESIAN_POINT ( 'NONE',  ( 116.9914377788273327, -35.36134890089079619, 113.9354139663191177 ) ) ;
#65153=ORIENTED_EDGE ( 'NONE', *, *, #60546, .F. ) ;
#65154=ORIENTED_EDGE ( 'NONE', *, *, #11365, .F. ) ;
#65155=CARTESIAN_POINT ( 'NONE',  ( 103.5342718762226895, -27.68543744656516026, 19.79527697093397265 ) ) ;
#65157=CARTESIAN_POINT ( 'NONE',  ( 114.4785830672529130, -28.49803820358978612, 159.5051490854349652 ) ) ;
#65158=CARTESIAN_POINT ( 'NONE',  ( 97.63679352021414104, -31.00714225716590278, 125.8803871806719599 ) ) ;
#65159=CARTESIAN_POINT ( 'NONE',  ( 194.0371591254585155, -46.82818131005407736, 129.9678068554150343 ) ) ;
#65160=CARTESIAN_POINT ( 'NONE',  ( 100.2482148738244661, -28.84314871041893014, 256.6441967044821695 ) ) ;
#65164=ADVANCED_FACE ( 'NONE', ( #62726 ), #21407, .T. ) ;
#65165=ORIENTED_EDGE ( 'NONE', *, *, #14117, .F. ) ;
#65168=VERTEX_POINT ( 'NONE', #55440 ) ;
#65169=EDGE_CURVE ( 'NONE', #27939, #65845, #63749, .T. ) ;
#65171=VECTOR ( 'NONE', #39089, 1000.000000000000000 ) ;
#65172=CARTESIAN_POINT ( 'NONE',  ( 99.97821182074206092, -27.16988623491039334, 185.5841967044829630 ) ) ;
#65174=CARTESIAN_POINT ( 'NONE',  ( 98.85647153018690858, -30.30415715074617111, 155.7984824187679465 ) ) ;
#65175=LINE ( 'NONE', #86081, #15227 ) ;
#65177=DIRECTION ( 'NONE',  ( 1.000000000000000000, 3.999999999999999995E-14, 1.000000000000000078E-15 ) ) ;
#65178=DIRECTION ( 'NONE',  ( 1.000000000000000078E-15, 0.000000000000000000, 1.000000000000000000 ) ) ;
#65179=FACE_OUTER_BOUND ( 'NONE', #32665, .T. ) ;
#65181=CARTESIAN_POINT ( 'NONE',  ( 105.8960369669305948, -47.10223136823062617, 278.4870538473395527 ) ) ;
#65183=CARTESIAN_POINT ( 'NONE',  ( 179.1667039024474661, -26.71338133338671739, 237.4678068554150059 ) ) ;
#65185=DIRECTION ( 'NONE',  ( 1.000000000000000000, -9.073094938289460781E-13, 0.000000000000000000 ) ) ;
#65186=AXIS2_PLACEMENT_3D ( 'NONE', #89513, #82262, #26817 ) ;
#65189=CARTESIAN_POINT ( 'NONE',  ( 99.04406187972965370, -42.84125766729550833, 257.8439586119762339 ) ) ;
#65190=EDGE_CURVE ( 'NONE', #8827, #46455, #7209, .T. ) ;
#65192=CARTESIAN_POINT ( 'NONE',  ( 106.2659377814683808, -44.71837661912690010, 195.5838068554170093 ) ) ;
#65194=LINE ( 'NONE', #11107, #62566 ) ;
#65195=CARTESIAN_POINT ( 'NONE',  ( 116.3972416472496434, -41.42873566659991269, 203.4556252759109611 ) ) ;
#65196=CARTESIAN_POINT ( 'NONE',  ( 96.71481148478426348, -38.23418088628295664, 62.44133956162495025 ) ) ;
#65197=CARTESIAN_POINT ( 'NONE',  ( 118.9266961287330560, -37.70231105260669580, 184.7613395616249647 ) ) ;
#65199=VECTOR ( 'NONE', #13799, 1000.000000000000000 ) ;
#65200=CARTESIAN_POINT ( 'NONE',  ( 107.0664832912739968, -36.72944715994100306, 311.6356252759112522 ) ) ;
#65201=CARTESIAN_POINT ( 'NONE',  ( 167.7413838386817133, -48.33240602328261559, 300.4678068554149490 ) ) ;
#65202=CARTESIAN_POINT ( 'NONE',  ( 116.4174193679775300, -33.16718996298826738, 40.11587310748063118 ) ) ;
#65205=ORIENTED_EDGE ( 'NONE', *, *, #89227, .T. ) ;
#65206=DIRECTION ( 'NONE',  ( 1.000000000000000000, 0.000000000000000000, 0.000000000000000000 ) ) ;
#65208=ORIENTED_EDGE ( 'NONE', *, *, #70026, .F. ) ;
#65210=CARTESIAN_POINT ( 'NONE',  ( 112.7653361951733473, -30.36711996764882571, 113.9181341137909556 ) ) ;
#65214=CARTESIAN_POINT ( 'NONE',  ( 97.56228874418796693, -32.49873190831186776, 96.99276813305395706 ) ) ;
#65215=DIRECTION ( 'NONE',  ( 1.000000000000000078E-15, 0.000000000000000000, 1.000000000000000000 ) ) ;
#65216=EDGE_CURVE ( 'NONE', #11190, #79263, #28936, .T. ) ;
#65218=CARTESIAN_POINT ( 'NONE',  ( 77.85525873416526110, -17.08426237657415570, 7.378668740738687504 ) ) ;
#65221=CARTESIAN_POINT ( 'NONE',  ( 115.3461623907574563, -31.52268719801062957, 34.27276813305396530 ) ) ;
#65224=ORIENTED_EDGE ( 'NONE', *, *, #15384, .F. ) ;
#65226=CARTESIAN_POINT ( 'NONE',  ( 179.1667039024460166, -28.27351298637280408, 117.4678068554150627 ) ) ;
#65227=DIRECTION ( 'NONE',  ( 1.000000000000000000, 8.673617379883546378E-16, 9.757819552368989676E-16 ) ) ;
#65228=DIRECTION ( 'NONE',  ( 0.000000000000000000, 0.000000000000000000, -1.000000000000000000 ) ) ;
#65229=CYLINDRICAL_SURFACE ( 'NONE', #33934, 3.250000000000002665 ) ;
#65231=CARTESIAN_POINT ( 'NONE',  ( 113.2462210345366316, -28.75922547209470181, 50.55319279321858517 ) ) ;
#65233=CIRCLE ( 'NONE', #5779, 10.04999999999999361 ) ;
#65235=CARTESIAN_POINT ( 'NONE',  ( 110.3650187231686743, -47.25482062520524096, 52.80610146638697699 ) ) ;
#65236=ORIENTED_EDGE ( 'NONE', *, *, #38605, .F. ) ;
#65241=CARTESIAN_POINT ( 'NONE',  ( 100.3248355287147291, -41.38056247698398238, 124.6252332267339682 ) ) ;
#65244=LINE ( 'NONE', #44786, #74579 ) ;
#65245=LINE ( 'NONE', #77538, #11158 ) ;
#65246=VERTEX_POINT ( 'NONE', #956 ) ;
#65251=ORIENTED_EDGE ( 'NONE', *, *, #68840, .F. ) ;
#65253=CARTESIAN_POINT ( 'NONE',  ( 97.70553735687687436, -35.92370728225471055, 182.6777737820879679 ) ) ;
#65255=CARTESIAN_POINT ( 'NONE',  ( 114.7874576214283167, -44.67122033332078246, 114.2022919425779719 ) ) ;
#65257=CARTESIAN_POINT ( 'NONE',  ( 97.82725377794338328, -40.55524675897819975, 16.63888027222046873 ) ) ;
#65260=ORIENTED_EDGE ( 'NONE', *, *, #3570, .F. ) ;
#65261=ADVANCED_FACE ( 'NONE', ( #69999 ), #35459, .F. ) ;
#65262=AXIS2_PLACEMENT_3D ( 'NONE', #156, #55088, #20165 ) ;
#65263=CARTESIAN_POINT ( 'NONE',  ( 100.3885320853208896, -32.03533449533603772, 203.6566617981629577 ) ) ;
#65264=EDGE_CURVE ( 'NONE', #74158, #88283, #84089, .T. ) ;
#65265=CARTESIAN_POINT ( 'NONE',  ( 96.93519779220999055, -32.25144590123284161, 55.98324432352897162 ) ) ;
#65266=ORIENTED_EDGE ( 'NONE', *, *, #24809, .F. ) ;
#65267=CARTESIAN_POINT ( 'NONE',  ( 100.4250012405661039, -28.72198927997973783, 40.62705384733894221 ) ) ;
#65268=CARTESIAN_POINT ( 'NONE',  ( 41.56648329127399677, -9.303447159940999356, 198.9256252759119832 ) ) ;
#65269=FACE_BOUND ( 'NONE', #88038, .T. ) ;
#65270=FACE_OUTER_BOUND ( 'NONE', #39138, .T. ) ;
#65271=CARTESIAN_POINT ( 'NONE',  ( 101.7695353289030322, -45.70857994070590991, 158.1527681330539963 ) ) ;
#65274=CARTESIAN_POINT ( 'NONE',  ( 177.0371591254543375, -48.62818131005480637, 300.4678068554149490 ) ) ;
#65275=EDGE_CURVE ( 'NONE', #15124, #66455, #5635, .T. ) ;
#65276=EDGE_CURVE ( 'NONE', #52666, #397, #21681, .T. ) ;
#65277=EDGE_LOOP ( 'NONE', ( #47039, #40478, #56991, #57952 ) ) ;
#65278=FACE_OUTER_BOUND ( 'NONE', #24228, .T. ) ;
#65281=ORIENTED_EDGE ( 'NONE', *, *, #56333, .F. ) ;
#65282=EDGE_CURVE ( 'NONE', #80581, #53161, #70909, .T. ) ;
#65283=CARTESIAN_POINT ( 'NONE',  ( 41.56648329127398966, -27.57844715994070484, 318.9256252759120116 ) ) ;
#65285=CARTESIAN_POINT ( 'NONE',  ( 96.71459513300293054, -38.23421233548538112, 66.44133956162495735 ) ) ;
#65286=DIRECTION ( 'NONE',  ( -1.424786214935630051E-15, 0.000000000000000000, 1.000000000000000000 ) ) ;
#65287=EDGE_CURVE ( 'NONE', #4960, #27387, #86960, .T. ) ;
#65288=FACE_OUTER_BOUND ( 'NONE', #36662, .T. ) ;
#65289=DIRECTION ( 'NONE',  ( 0.000000000000000000, 0.000000000000000000, -1.000000000000000000 ) ) ;
#65290=CARTESIAN_POINT ( 'NONE',  ( 110.3395589168170972, -45.98151452052003663, 37.84705384733994293 ) ) ;
#65291=CARTESIAN_POINT ( 'NONE',  ( 142.8698897858160706, -0.9167816978817300289, 394.9756252759102040 ) ) ;
#65292=CARTESIAN_POINT ( 'NONE',  ( 117.1049515565468226, -33.87427183379793405, 145.0470538473399529 ) ) ;
#65294=DIRECTION ( 'NONE',  ( 1.000000000000000078E-15, -1.000000000000000083E-30, -1.000000000000000000 ) ) ;
#65295=ORIENTED_EDGE ( 'NONE', *, *, #25713, .F. ) ;
#65296=DIRECTION ( 'NONE',  ( 1.000000000000000000, 0.000000000000000000, 0.000000000000000000 ) ) ;
#65297=AXIS2_PLACEMENT_3D ( 'NONE', #78099, #15865, #38082 ) ;
#65298=FACE_OUTER_BOUND ( 'NONE', #55232, .T. ) ;
#65299=DIRECTION ( 'NONE',  ( 0.000000000000000000, 0.000000000000000000, -1.000000000000000000 ) ) ;
#65300=EDGE_CURVE ( 'NONE', #837, #69025, #1379, .T. ) ;
#65301=AXIS2_PLACEMENT_3D ( 'NONE', #31894, #16943, #85555 ) ;
#65303=CARTESIAN_POINT ( 'NONE',  ( 114.1546619933443480, -29.02461823700197741, 199.4841967044819739 ) ) ;
#65304=ORIENTED_EDGE ( 'NONE', *, *, #70425, .T. ) ;
#65305=CYLINDRICAL_SURFACE ( 'NONE', #1656, 13.99999999999999822 ) ;
#65306=CARTESIAN_POINT ( 'NONE',  ( 96.74182981399745529, -35.13608925046722220, 262.2041967044821149 ) ) ;
#65307=CARTESIAN_POINT ( 'NONE',  ( 110.1708544452211100, -46.72723989065711692, 93.81562527591097478 ) ) ;
#65308=CARTESIAN_POINT ( 'NONE',  ( 99.09685934341746361, -30.54889812966678164, 251.8073641162624199 ) ) ;
#65313=ORIENTED_EDGE ( 'NONE', *, *, #57164, .F. ) ;
#65314=ORIENTED_EDGE ( 'NONE', *, *, #84610, .F. ) ;
#65316=ORIENTED_EDGE ( 'NONE', *, *, #4550, .T. ) ;
#65318=CARTESIAN_POINT ( 'NONE',  ( 96.56373827543593791, -40.17738982329606046, 282.5908633711490552 ) ) ;
#65319=FACE_OUTER_BOUND ( 'NONE', #4669, .T. ) ;
#65322=EDGE_CURVE ( 'NONE', #8105, #74330, #60812, .T. ) ;
#65325=EDGE_CURVE ( 'NONE', #45090, #85483, #57705, .T. ) ;
#65327=CARTESIAN_POINT ( 'NONE',  ( 98.55184737119530780, -35.75319039346454986, 205.6581341137909646 ) ) ;
#65328=EDGE_LOOP ( 'NONE', ( #78366, #23175, #57508, #15647 ) ) ;
#65331=LINE ( 'NONE', #24448, #7933 ) ;
#65332=CARTESIAN_POINT ( 'NONE',  ( 97.81168844167092402, -40.51740470302234343, 181.6357138554620576 ) ) ;
#65333=CARTESIAN_POINT ( 'NONE',  ( 104.9788083641148972, -27.14010996210895499, 256.2470538473390889 ) ) ;
#65334=CIRCLE ( 'NONE', #58130, 4.874999999999990230 ) ;
#65338=VERTEX_POINT ( 'NONE', #65848 ) ;
#65339=CARTESIAN_POINT ( 'NONE',  ( 103.2765498915109248, -27.47545316653152625, 56.38579426906439807 ) ) ;
#65341=AXIS2_PLACEMENT_3D ( 'NONE', #64905, #30387, #56736 ) ;
#65342=CARTESIAN_POINT ( 'NONE',  ( 59.68306514483415270, -72.55903866283681225, 540.9756252759101471 ) ) ;
#65343=CARTESIAN_POINT ( 'NONE',  ( 110.4041361119612930, -44.93847832680074106, 279.3158690201827881 ) ) ;
#65345=CYLINDRICAL_SURFACE ( 'NONE', #24694, 2.517499999999998739 ) ;
#65346=CARTESIAN_POINT ( 'NONE',  ( 33.81648329127298780, 12.92155284005802862, 355.9756252759109998 ) ) ;
#65347=CARTESIAN_POINT ( 'NONE',  ( 179.8585841295800094, -30.08671355700241179, -5.074374724088000832 ) ) ;
#65348=ORIENTED_EDGE ( 'NONE', *, *, #55118, .T. ) ;
#65350=DIRECTION ( 'NONE',  ( -4.093947403305260305E-16, 1.000000000000000000, -6.162975822039159109E-32 ) ) ;
#65352=CARTESIAN_POINT ( 'NONE',  ( 118.0022803299065686, -38.33799637688264994, 73.72229194257801055 ) ) ;
#65353=EDGE_LOOP ( 'NONE', ( #17715, #11471 ) ) ;
#65354=CARTESIAN_POINT ( 'NONE',  ( 102.0478764085966361, -45.04113848309104640, 51.56670554236298187 ) ) ;
#65356=DIRECTION ( 'NONE',  ( 2.056463827196271584E-15, -0.8571673007021100021, 0.5150380749100580413 ) ) ;
#65357=CARTESIAN_POINT ( 'NONE',  ( 107.7480938161759951, -27.89408153625565845, 66.44729759161194238 ) ) ;
#65358=CARTESIAN_POINT ( 'NONE',  ( 97.81168843500762478, -40.51741166756562507, 12.63579318495451176 ) ) ;
#65361=EDGE_CURVE ( 'NONE', #62172, #64372, #57965, .T. ) ;
#65362=CARTESIAN_POINT ( 'NONE',  ( 115.6911227382933873, -43.67932486773085543, 39.27467289495895386 ) ) ;
#65363=CIRCLE ( 'NONE', #55151, 2.517499999999998739 ) ;
#65366=LINE ( 'NONE', #33522, #48746 ) ;
#65367=EDGE_LOOP ( 'NONE', ( #85181, #76317 ) ) ;
#65368=CARTESIAN_POINT ( 'NONE',  ( 97.94860405783340696, -41.87310908463563663, 132.7356252759109623 ) ) ;
#65369=CARTESIAN_POINT ( 'NONE',  ( 79.18623681047911589, -21.33528726900534522, 1.744847506584294106 ) ) ;
#65371=ORIENTED_EDGE ( 'NONE', *, *, #84347, .F. ) ;
#65373=EDGE_CURVE ( 'NONE', #21680, #68103, #81560, .T. ) ;
#65374=VECTOR ( 'NONE', #80362, 1000.000000000000000 ) ;
#65375=CYLINDRICAL_SURFACE ( 'NONE', #28955, 2.117000000000000881 ) ;
#65378=CARTESIAN_POINT ( 'NONE',  ( 106.3491918589965763, -46.48387837312656501, 222.5184824187689401 ) ) ;
#65380=CARTESIAN_POINT ( 'NONE',  ( 75.31670390244798341, -57.40094715994099772, 86.31780685541500020 ) ) ;
#65382=CARTESIAN_POINT ( 'NONE',  ( 117.2667774650794428, -38.88269731149204489, 59.66133956162595098 ) ) ;
#65384=ORIENTED_EDGE ( 'NONE', *, *, #51235, .T. ) ;
#65385=CARTESIAN_POINT ( 'NONE',  ( 111.0446433595016913, -27.50350014455446868, 170.7527502710815952 ) ) ;
#65386=EDGE_CURVE ( 'NONE', #2920, #11510, #50889, .T. ) ;
#65389=EDGE_CURVE ( 'NONE', #69283, #16139, #86764, .T. ) ;
#65390=LINE ( 'NONE', #59886, #45972 ) ;
#65392=CARTESIAN_POINT ( 'NONE',  ( 116.8642987764957297, -41.79567201640977459, 243.4346728949589647 ) ) ;
#65394=FACE_BOUND ( 'NONE', #21910, .T. ) ;
#65395=CARTESIAN_POINT ( 'NONE',  ( 135.0664832912729878, -36.72944715994189835, 361.9756252759109998 ) ) ;
#65397=AXIS2_PLACEMENT_3D ( 'NONE', #35531, #568, #21023 ) ;
#65398=CARTESIAN_POINT ( 'NONE',  ( 114.2672205647202048, -43.24251175450689288, 232.6638483995059801 ) ) ;
#65399=DIRECTION ( 'NONE',  ( -0.3818493186865920541, 0.9242245927363033076, 0.000000000000000000 ) ) ;
#65400=CARTESIAN_POINT ( 'NONE',  ( 112.7298150101557610, -27.26422151970083263, 50.65943479972101215 ) ) ;
#65402=CARTESIAN_POINT ( 'NONE',  ( 97.57695254711111943, -30.97082841205668657, 125.8803871806719599 ) ) ;
#65403=VERTEX_POINT ( 'NONE', #51319 ) ;
#65404=DIRECTION ( 'NONE',  ( -2.900000000000000265E-14, 2.000000000000000155E-15, -1.000000000000000000 ) ) ;
#65406=FACE_OUTER_BOUND ( 'NONE', #34827, .T. ) ;
#65407=CARTESIAN_POINT ( 'NONE',  ( 105.7995184603037870, -26.72403496900519926, 66.17729194474850374 ) ) ;
#65408=CARTESIAN_POINT ( 'NONE',  ( 103.2782266777140165, -27.47476627046264142, 276.3856500783257957 ) ) ;
#65409=VECTOR ( 'NONE', #89345, 1000.000000000000000 ) ;
#65410=EDGE_LOOP ( 'NONE', ( #63068, #9762, #20449, #39759 ) ) ;
#65411=EDGE_CURVE ( 'NONE', #26375, #37766, #52199, .T. ) ;
#65412=CARTESIAN_POINT ( 'NONE',  ( 97.31310622223200824, -38.96075413463563564, 51.50544982982146536 ) ) ;
#65413=VERTEX_POINT ( 'NONE', #34351 ) ;
#65415=DIRECTION ( 'NONE',  ( 1.000000000000000078E-15, 0.000000000000000000, 1.000000000000000000 ) ) ;
#65416=VECTOR ( 'NONE', #70547, 1000.000000000000000 ) ;
#65417=DIRECTION ( 'NONE',  ( 0.000000000000000000, 1.000000000000000000, 0.000000000000000000 ) ) ;
#65418=VERTEX_POINT ( 'NONE', #81641 ) ;
#65419=CARTESIAN_POINT ( 'NONE',  ( 107.3215719809018083, -25.65558735872630081, 75.04610146638695767 ) ) ;
#65421=CARTESIAN_POINT ( 'NONE',  ( 97.53191591005956695, -39.74918175134386900, 166.5705498172278851 ) ) ;
#65424=EDGE_LOOP ( 'NONE', ( #57595, #7031 ) ) ;
#65426=DIRECTION ( 'NONE',  ( 1.000000000000000000, 4.299999999999999979E-14, 1.000000000000000078E-15 ) ) ;
#65429=FACE_OUTER_BOUND ( 'NONE', #19019, .T. ) ;
#65431=EDGE_CURVE ( 'NONE', #67028, #12546, #23190, .T. ) ;
#65432=CARTESIAN_POINT ( 'NONE',  ( 25.56670390244797275, -65.37844715994100397, 262.0928068554150059 ) ) ;
#65433=VECTOR ( 'NONE', #19944, 1000.000000000000000 ) ;
#65434=ORIENTED_EDGE ( 'NONE', *, *, #12240, .F. ) ;
#65435=B_SPLINE_CURVE_WITH_KNOTS ( 'NONE', 3,
 ( #56429, #19804, #15117, #65497, #86400, #29636, #15575, #37348, #43701, #43247, #57783, #37797, #16460, #1939, #30089, #44139, #50062, #29199, #3281, #79594, #2835, #24174, #16910, #58235, #51840, #56880, #79149, #51397, #30534, #84624, #30974, #17353, #45034, #57327, #85525, #58662, #72761, #9205, #85072, #10531, #22837, #23301, #85963, #65054, #50966, #22384, #78261, #78709, #71877, #44587, #50518 ),
 .UNSPECIFIED., .F., .F.,
 ( 4, 2, 1, 1, 1, 1, 1, 1, 2, 2, 2, 2, 2, 2, 2, 1, 1, 1, 1, 1, 1, 1, 2, 2, 2, 2, 2, 2, 2, 2, 2, 4 ),
 ( 0.5000144963954069599, 0.5001365631688001745, 0.5002586299421935001, 0.5005027634889802624, 0.5009910305825536758, 0.5019675647696999476, 0.5039206331439923803, 0.5078267698925770235, 0.5156390433897460879, 0.5312635903840843277, 0.5625126843727610293, 0.6250108723501143215, 0.6875090603274676138, 0.7500072483048209060, 0.7500682816915176243, 0.7501293150782144536, 0.7502513818516167721, 0.7504955153982477700, 0.7509837824914034066, 0.7519603166777120151, 0.7539133850503294543, 0.7578195217955624452, 0.7656317952860278719, 0.7812563422669582813, 0.8125054362288213206, 0.8437545301906844708, 0.8750036241525475100, 0.9062527181144106603, 0.9375018120762736995, 0.9687509060381367387, 0.9843754530190684804, 1.000000000000000000 ),
 .UNSPECIFIED. ) ;
#65436=DIRECTION ( 'NONE',  ( 0.000000000000000000, 0.000000000000000000, 1.000000000000000000 ) ) ;
#65437=CARTESIAN_POINT ( 'NONE',  ( 109.2982854457139297, -26.60236246699155416, 175.8918157521009391 ) ) ;
#65440=CARTESIAN_POINT ( 'NONE',  ( 104.8797383215544414, -46.86635653470245444, 28.41943479971997988 ) ) ;
#65441=CARTESIAN_POINT ( 'NONE',  ( 63.06670390244711655, -40.32844715994016838, 129.9678068554150911 ) ) ;
#65442=CARTESIAN_POINT ( 'NONE',  ( 138.8167039024479834, -57.40094715994099772, 86.31780685541500020 ) ) ;
#65447=CARTESIAN_POINT ( 'NONE',  ( 97.31581552154544568, -39.30590672086626824, 31.53167568815738164 ) ) ;
#65448=ORIENTED_EDGE ( 'NONE', *, *, #26418, .F. ) ;
#65450=CARTESIAN_POINT ( 'NONE',  ( 114.9810172151485546, -40.71547668563403022, 199.8872975916109453 ) ) ;
#65453=CARTESIAN_POINT ( 'NONE',  ( 98.26720277155988015, -37.77870449121756025, 37.85301187732598294 ) ) ;
#65455=CARTESIAN_POINT ( 'NONE',  ( 109.7248659253242522, -27.00080518093118442, 79.86479194225255185 ) ) ;
#65457=CIRCLE ( 'NONE', #55257, 13.99999999999999822 ) ;
#65458=ORIENTED_EDGE ( 'NONE', *, *, #11122, .F. ) ;
#65459=DIRECTION ( 'NONE',  ( 1.000000000000000000, 4.299999999999999979E-14, 1.000000000000000078E-15 ) ) ;
#65460=CARTESIAN_POINT ( 'NONE',  ( 41.56648329127399677, -9.303447159940999356, 21.04262527591200183 ) ) ;
#65461=ORIENTED_EDGE ( 'NONE', *, *, #11350, .F. ) ;
#65462=CARTESIAN_POINT ( 'NONE',  ( 100.2624651760415304, -28.85963121439194623, 260.6441967044822263 ) ) ;
#65464=VERTEX_POINT ( 'NONE', #13923 ) ;
#65467=CARTESIAN_POINT ( 'NONE',  ( 63.03715912545735023, -46.82818131006016671, 180.4678068554151196 ) ) ;
#65469=CARTESIAN_POINT ( 'NONE',  ( 99.72256515790628839, -29.26889448616327982, 221.6956252759109702 ) ) ;
#65473=CARTESIAN_POINT ( 'NONE',  ( 99.09426955137945470, -44.45222557475181446, 37.95086337114900488 ) ) ;
#65475=CARTESIAN_POINT ( 'NONE',  ( 96.56351739100374232, -40.17746103522156176, 286.5908633711491120 ) ) ;
#65477=EDGE_CURVE ( 'NONE', #77124, #73910, #26204, .T. ) ;
#65478=VERTEX_POINT ( 'NONE', #27989 ) ;
#65480=DIRECTION ( 'NONE',  ( 1.000000000000000000, 4.299999999999999979E-14, 1.000000000000000078E-15 ) ) ;
#65481=CARTESIAN_POINT ( 'NONE',  ( 116.8164944309794606, -34.15047750347410727, 20.03140278090121029 ) ) ;
#65482=LINE ( 'NONE', #22368, #71268 ) ;
#65483=CARTESIAN_POINT ( 'NONE',  ( 103.8598393684536632, -44.23592174987565073, 90.07380465530594904 ) ) ;
#65484=CARTESIAN_POINT ( 'NONE',  ( 108.6783733978936226, -26.40767070732865562, 185.9527681330539792 ) ) ;
#65487=ORIENTED_EDGE ( 'NONE', *, *, #30863, .F. ) ;
#65489=DIRECTION ( 'NONE',  ( 0.7071067811873692488, 0.7071067811857258967, -2.899137802861360256E-29 ) ) ;
#65490=ORIENTED_EDGE ( 'NONE', *, *, #82786, .T. ) ;
#65493=CARTESIAN_POINT ( 'NONE',  ( 130.0664832912740110, -18.72922654876702353, 239.5838068554170377 ) ) ;
#65494=EDGE_LOOP ( 'NONE', ( #24874, #85686, #12086, #35845 ) ) ;
#65495=VERTEX_POINT ( 'NONE', #47066 ) ;
#65497=CARTESIAN_POINT ( 'NONE',  ( 97.80783779089463792, -40.50800376726066077, 42.63481548141047028 ) ) ;
#65498=EDGE_CURVE ( 'NONE', #9337, #25266, #40718, .T. ) ;
#65499=CARTESIAN_POINT ( 'NONE',  ( 115.2323353771322445, -31.47685829367418009, 143.7038483995059721 ) ) ;
#65501=CARTESIAN_POINT ( 'NONE',  ( 99.09377177006922466, -44.45270778143659385, 41.95086337114900488 ) ) ;
#65503=AXIS2_PLACEMENT_3D ( 'NONE', #25735, #54306, #47051 ) ;
#65504=ORIENTED_EDGE ( 'NONE', *, *, #48016, .F. ) ;
#65505=CARTESIAN_POINT ( 'NONE',  ( 97.12554930137042675, -37.99679140698025748, 137.4272600898537462 ) ) ;
#65507=DIRECTION ( 'NONE',  ( 0.000000000000000000, 0.000000000000000000, -1.000000000000000000 ) ) ;
#65509=CARTESIAN_POINT ( 'NONE',  ( 37.06648329127298780, 12.92155284005730387, 355.9756252759109998 ) ) ;
#65512=CARTESIAN_POINT ( 'NONE',  ( 96.97860658150185031, -39.36037357437717787, 276.5299109901967540 ) ) ;
#65513=CARTESIAN_POINT ( 'NONE',  ( 105.1556394555663445, -47.05180815895162993, 8.429910990196965770 ) ) ;
#65515=DIRECTION ( 'NONE',  ( 0.9242245927363033076, 0.3818493186865918876, 0.000000000000000000 ) ) ;
#65517=DIRECTION ( 'NONE',  ( -4.093947403305260305E-16, 1.000000000000000000, -6.162975822039159109E-32 ) ) ;
#65518=CARTESIAN_POINT ( 'NONE',  ( 105.4062783216046313, -25.39030566700975555, 322.9818289795172177 ) ) ;
#65519=DIRECTION ( 'NONE',  ( 0.000000000000000000, 1.000000000000000000, 0.000000000000000000 ) ) ;
#65520=CARTESIAN_POINT ( 'NONE',  ( 130.0664832912740110, -18.82844715994099971, 284.9256252759119548 ) ) ;
#65521=CIRCLE ( 'NONE', #55320, 11.45913725231036118 ) ;
#65522=CARTESIAN_POINT ( 'NONE',  ( 130.0664832912740110, -18.82844715994099971, 17.92562527591199739 ) ) ;
#65523=B_SPLINE_CURVE_WITH_KNOTS ( 'NONE', 3,
 ( #74476, #47187, #53996, #81754, #19504, #61716, #74926, #19961, #66757, #4542, #11805, #12247, #26757, #74026, #67661, #40831, #68109, #13151 ),
 .UNSPECIFIED., .F., .F.,
 ( 4, 2, 2, 2, 2, 2, 2, 2, 4 ),
 ( 0.4999999978220436292, 0.5624999980942881894, 0.6249999983665327496, 0.6874999986387773099, 0.7499999989110217591, 0.8124999991832664303, 0.8749999994555108795, 0.9374999997277554398, 1.000000000000000000 ),
 .UNSPECIFIED. ) ;
#65524=FACE_OUTER_BOUND ( 'NONE', #86645, .T. ) ;
#65525=CARTESIAN_POINT ( 'NONE',  ( 168.3595971214162148, -48.62134037890298544, 300.4678068554149490 ) ) ;
#65526=CARTESIAN_POINT ( 'NONE',  ( 110.2977701465690643, -46.68767980799292872, 12.82705384733995402 ) ) ;
#65527=CARTESIAN_POINT ( 'NONE',  ( 97.67470816545109358, -41.25460433215529577, 167.6841967044829573 ) ) ;
#65528=CARTESIAN_POINT ( 'NONE',  ( 96.15481094519168437, -38.63223783578033022, 42.45181575210199298 ) ) ;
#65530=DIRECTION ( 'NONE',  ( -4.237773401492740281E-14, 1.000000000000000000, 0.000000000000000000 ) ) ;
#65532=ADVANCED_FACE ( 'NONE', ( #27102 ), #89793, .T. ) ;
#65533=CARTESIAN_POINT ( 'NONE',  ( 31.78666935232998725, -36.02818131005891189, -5.074374724088000832 ) ) ;
#65534=AXIS2_PLACEMENT_3D ( 'NONE', #72538, #38008, #65702 ) ;
#65535=EDGE_CURVE ( 'NONE', #38582, #74068, #55225, .T. ) ;
#65537=CARTESIAN_POINT ( 'NONE',  ( 104.4899545120944566, -26.97880756954710080, 186.2814586043616032 ) ) ;
#65539=CARTESIAN_POINT ( 'NONE',  ( 108.8666348730871078, -46.34312957481623840, 78.72419670448194040 ) ) ;
#65542=CARTESIAN_POINT ( 'NONE',  ( 150.5667039024473297, -25.42844715993594562, 300.4678068554149490 ) ) ;
#65543=CARTESIAN_POINT ( 'NONE',  ( 118.8526415125688800, -37.69623653580512013, 184.7613395616249647 ) ) ;
#65544=CARTESIAN_POINT ( 'NONE',  ( 25.56670390244797275, -67.87844715994100397, 168.3428068554150059 ) ) ;
#65545=DIRECTION ( 'NONE',  ( -0.7071067811865462405, 0.000000000000000000, 0.7071067811865486830 ) ) ;
#65547=CARTESIAN_POINT ( 'NONE',  ( 100.9546728013743149, -28.70702573470092389, 46.59395861020129104 ) ) ;
#65550=CARTESIAN_POINT ( 'NONE',  ( 116.4060884429800922, -40.43037349191362040, 98.52600069756960011 ) ) ;
#65551=CARTESIAN_POINT ( 'NONE',  ( 111.5019814087853831, -26.53443175268781218, 134.7499109901969518 ) ) ;
#65552=ORIENTED_EDGE ( 'NONE', *, *, #57066, .T. ) ;
#65555=CARTESIAN_POINT ( 'NONE',  ( 110.4802244392091950, -27.25226000720831721, 96.23301187732596418 ) ) ;
#65556=AXIS2_PLACEMENT_3D ( 'NONE', #23947, #58444, #43918 ) ;
#65559=CARTESIAN_POINT ( 'NONE',  ( 117.3720538532506623, -35.57445771113446398, 229.9032443235289520 ) ) ;
#65560=DIRECTION ( 'NONE',  ( 0.000000000000000000, 1.000000000000000000, 0.000000000000000000 ) ) ;
#65562=CARTESIAN_POINT ( 'NONE',  ( 115.8254330622582415, -31.73001971111901653, 110.2399483882993820 ) ) ;
#65565=CARTESIAN_POINT ( 'NONE',  ( 62.03742497533652767, -23.42844715994041493, 193.9678068554150911 ) ) ;
#65566=FACE_OUTER_BOUND ( 'NONE', #39098, .T. ) ;
#65567=DIRECTION ( 'NONE',  ( 1.000000000000000078E-15, -1.000000000000000083E-30, -1.000000000000000000 ) ) ;
#65568=CARTESIAN_POINT ( 'NONE',  ( 98.02603654163375779, -30.41010087969369735, 160.8289586092449497 ) ) ;
#65569=ORIENTED_EDGE ( 'NONE', *, *, #54447, .F. ) ;
#65571=ORIENTED_EDGE ( 'NONE', *, *, #76173, .F. ) ;
#65572=ORIENTED_CLOSED_SHELL ( 'NONE', *, #34327, .F. );
#65573=AXIS2_PLACEMENT_3D ( 'NONE', #53374, #25245, #52909 ) ;
#65577=CARTESIAN_POINT ( 'NONE',  ( 108.3330205148376706, -46.73491748175980831, 103.6772580696607378 ) ) ;
#65578=DIRECTION ( 'NONE',  ( -1.907762142705490052E-15, -7.167082501179359715E-16, 1.000000000000000000 ) ) ;
#65579=CARTESIAN_POINT ( 'NONE',  ( 117.0173010276973287, -33.62006509304910651, 174.0670538473389399 ) ) ;
#65580=DIRECTION ( 'NONE',  ( 0.000000000000000000, 1.000000000000000000, 0.000000000000000000 ) ) ;
#65583=ORIENTED_EDGE ( 'NONE', *, *, #37926, .T. ) ;
#65585=CARTESIAN_POINT ( 'NONE',  ( 115.7473634667994560, -41.72957221166183928, 64.41119945959614768 ) ) ;
#65587=CARTESIAN_POINT ( 'NONE',  ( 131.4004675426835718, -36.03188136816541487, 6.871351212842790268 ) ) ;
#65588=CARTESIAN_POINT ( 'NONE',  ( 114.3671945862968045, -31.65384462053443571, 275.7415833058969952 ) ) ;
#65589=CARTESIAN_POINT ( 'NONE',  ( 20.03715912545644073, -24.42818131006202265, 129.9678068554150627 ) ) ;
#65592=VECTOR ( 'NONE', #27549, 1000.000000000000000 ) ;
#65593=CARTESIAN_POINT ( 'NONE',  ( 106.1388935886583624, -44.86984817071454046, 9.635625275910941312 ) ) ;
#65594=DIRECTION ( 'NONE',  ( -4.237773401492740281E-14, 1.000000000000000000, 0.000000000000000000 ) ) ;
#65595=VERTEX_POINT ( 'NONE', #5320 ) ;
#65598=CARTESIAN_POINT ( 'NONE',  ( 110.8925242491656320, -45.96859375203237619, 112.8888992892811700 ) ) ;
#65601=EDGE_CURVE ( 'NONE', #20396, #70423, #5771, .T. ) ;
#65602=CARTESIAN_POINT ( 'NONE',  ( 100.5114817196218411, -42.97801697403279775, 36.34289601855395091 ) ) ;
#65603=CARTESIAN_POINT ( 'NONE',  ( 115.0566306311886819, -29.05787713660226856, 189.4232443235299570 ) ) ;
#65604=CARTESIAN_POINT ( 'NONE',  ( 108.7397100058831541, -25.82697924850565840, 144.9432443235299672 ) ) ;
#65605=EDGE_CURVE ( 'NONE', #54909, #3107, #88444, .T. ) ;
#65607=CARTESIAN_POINT ( 'NONE',  ( 111.8640475646460857, -46.02486053542493494, 268.9556252759110180 ) ) ;
#65608=CARTESIAN_POINT ( 'NONE',  ( 99.04407452439549786, -42.84127747802013175, 97.84479291583183169 ) ) ;
#65610=ORIENTED_EDGE ( 'NONE', *, *, #85198, .F. ) ;
#65611=ORIENTED_EDGE ( 'NONE', *, *, #11939, .F. ) ;
#65613=CARTESIAN_POINT ( 'NONE',  ( 95.99995219064309993, -35.86644482699779246, 191.2765776568629690 ) ) ;
#65615=CARTESIAN_POINT ( 'NONE',  ( 108.8488851759622804, -47.00125683367996032, 167.7127681330539701 ) ) ;
#65616=DIRECTION ( 'NONE',  ( 1.639958061481212836E-42, -4.100000000000000342E-29, -1.000000000000000000 ) ) ;
#65617=CARTESIAN_POINT ( 'NONE',  ( 33.96670390244653959, -28.27351298637442056, 193.9678068554150911 ) ) ;
#65618=CARTESIAN_POINT ( 'NONE',  ( 134.0664832912740110, -9.029447159941003775, 1.625625275910997480 ) ) ;
#65620=CARTESIAN_POINT ( 'NONE',  ( 50.87649884952499946, -33.54226604284930602, -5.074374724088000832 ) ) ;
#65622=CARTESIAN_POINT ( 'NONE',  ( 115.8929840288991642, -32.51563116083749350, 15.18133956162492915 ) ) ;
#65623=CARTESIAN_POINT ( 'NONE',  ( 80.06648329127402519, -46.72944715994105991, 10.72562527591094295 ) ) ;
#65624=CARTESIAN_POINT ( 'NONE',  ( 83.06670390244796920, -58.72944715994094622, 210.8338068554149913 ) ) ;
#65625=VECTOR ( 'NONE', #68869, 1000.000000000000000 ) ;
#65626=DIRECTION ( 'NONE',  ( -9.073094938289460781E-13, -1.000000000000000000, 0.000000000000000000 ) ) ;
#65627=DIRECTION ( 'NONE',  ( -0.9254794337955620787, -0.3787978585227822492, 0.000000000000000000 ) ) ;
#65628=FACE_OUTER_BOUND ( 'NONE', #70090, .T. ) ;
#65629=DIRECTION ( 'NONE',  ( 1.000000000000000000, 0.000000000000000000, 0.000000000000000000 ) ) ;
#65630=CARTESIAN_POINT ( 'NONE',  ( 114.5288898844889047, -31.71472813432939830, 195.5838068554168672 ) ) ;
#65631=ORIENTED_EDGE ( 'NONE', *, *, #9397, .T. ) ;
#65633=CARTESIAN_POINT ( 'NONE',  ( 117.9557474314311349, -34.69982462793587530, 203.9851490854349549 ) ) ;
#65634=CARTESIAN_POINT ( 'NONE',  ( 101.7108440984968212, -27.74398881808361850, 81.50419670448295051 ) ) ;
#65635=CARTESIAN_POINT ( 'NONE',  ( 111.6274790011277247, -46.15230754745154940, 243.9356252759109509 ) ) ;
#65636=DIRECTION ( 'NONE',  ( 4.299999999999999979E-14, -1.000000000000000000, 4.400000000000000367E-29 ) ) ;
#65638=FACE_OUTER_BOUND ( 'NONE', #80031, .T. ) ;
#65639=LINE ( 'NONE', #23877, #19666 ) ;
#65642=CARTESIAN_POINT ( 'NONE',  ( 112.1419326622839776, -28.01430185457018496, 64.65734975839959020 ) ) ;
#65644=VERTEX_POINT ( 'NONE', #29352 ) ;
#65645=ORIENTED_EDGE ( 'NONE', *, *, #5716, .F. ) ;
#65646=CARTESIAN_POINT ( 'NONE',  ( 102.6518059180641416, -28.82227990381128180, 104.9162293518859599 ) ) ;
#65649=AXIS2_PLACEMENT_3D ( 'NONE', #74373, #67551, #88460 ) ;
#65650=CARTESIAN_POINT ( 'NONE',  ( 100.3128846869253294, -46.43702735306945328, 83.09276813305294240 ) ) ;
#65652=CARTESIAN_POINT ( 'NONE',  ( 79.00802158143734744, -16.19118199975294203, 8.051357469095744790 ) ) ;
#65653=CARTESIAN_POINT ( 'NONE',  ( 102.0670549777755696, -27.97049804943433315, 176.4897919409716280 ) ) ;
#65654=CARTESIAN_POINT ( 'NONE',  ( 99.56037394151441333, -43.88466257697688633, 36.92038718067297509 ) ) ;
#65656=ORIENTED_EDGE ( 'NONE', *, *, #55348, .T. ) ;
#65657=ORIENTED_EDGE ( 'NONE', *, *, #19126, .F. ) ;
#65658=EDGE_CURVE ( 'NONE', #67267, #23819, #7147, .T. ) ;
#65660=CARTESIAN_POINT ( 'NONE',  ( 116.3212776292296127, -32.94146857471318413, 287.6356252759109680 ) ) ;
#65661=CARTESIAN_POINT ( 'NONE',  ( 113.2454986995014394, -28.75867294597971124, 115.5522919424271038 ) ) ;
#65662=DIRECTION ( 'NONE',  ( 1.000000000000000000, -5.337610695313248426E-16, 0.000000000000000000 ) ) ;
#65664=LINE ( 'NONE', #43878, #11807 ) ;
#65667=CARTESIAN_POINT ( 'NONE',  ( 104.4960957391109417, -46.84663716100912012, 47.37848241876796607 ) ) ;
#65668=VERTEX_POINT ( 'NONE', #9345 ) ;
#65671=FACE_OUTER_BOUND ( 'NONE', #89307, .T. ) ;
#65672=DIRECTION ( 'NONE',  ( -1.000000000000000078E-15, 1.000000000000000083E-30, 1.000000000000000000 ) ) ;
#65674=CARTESIAN_POINT ( 'NONE',  ( 104.7498880507309451, -44.55652276380406818, 105.1652332267339602 ) ) ;
#65676=ADVANCED_FACE ( 'NONE', ( #1651 ), #15721, .F. ) ;
#65677=VECTOR ( 'NONE', #60129, 1000.000000000000000 ) ;
#65678=CARTESIAN_POINT ( 'NONE',  ( 181.5667039024459939, -22.48495420874030515, -5.074374724088000832 ) ) ;
#65679=ORIENTED_EDGE ( 'NONE', *, *, #4468, .F. ) ;
#65682=ORIENTED_EDGE ( 'NONE', *, *, #67191, .F. ) ;
#65683=ORIENTED_EDGE ( 'NONE', *, *, #64977, .T. ) ;
#65684=DIRECTION ( 'NONE',  ( 0.000000000000000000, 0.000000000000000000, 1.000000000000000000 ) ) ;
#65685=ADVANCED_FACE ( 'NONE', ( #15272 ), #8457, .F. ) ;
#65686=CARTESIAN_POINT ( 'NONE',  ( 98.18569924386140713, -36.28921507361370402, 167.7187261630399462 ) ) ;
#65688=CARTESIAN_POINT ( 'NONE',  ( 117.2306693829537210, -39.29235896168534481, 119.6299109901969615 ) ) ;
#65689=CARTESIAN_POINT ( 'NONE',  ( 99.09570915332048457, -30.55043165520475767, 120.8022919327240601 ) ) ;
#65690=CARTESIAN_POINT ( 'NONE',  ( 98.38055655239837449, -41.69550781276469564, 16.73980917770007437 ) ) ;
#65692=ORIENTED_EDGE ( 'NONE', *, *, #977, .T. ) ;
#65695=CARTESIAN_POINT ( 'NONE',  ( 109.0547627366692041, -28.78404389176943212, 197.6995189410199600 ) ) ;
#65697=CARTESIAN_POINT ( 'NONE',  ( 96.63442969565970486, -37.29391305320381633, 76.36991099019697060 ) ) ;
#65699=CARTESIAN_POINT ( 'NONE',  ( 95.28387218206118803, -35.72034718286344201, 36.25848241876794731 ) ) ;
#65700=CARTESIAN_POINT ( 'NONE',  ( 112.0632082999805448, -45.48990328828745078, 252.9899119478660623 ) ) ;
#65701=ADVANCED_FACE ( 'NONE', ( #71140 ), #14831, .F. ) ;
#65702=DIRECTION ( 'NONE',  ( 1.000000000000000000, 4.299999999999999979E-14, 1.000000000000000078E-15 ) ) ;
#65703=DIRECTION ( 'NONE',  ( -1.000000000000000000, -2.756263715554006823E-15, 0.000000000000000000 ) ) ;
#65704=CARTESIAN_POINT ( 'NONE',  ( 101.9720301123653883, -46.53865341315756154, 163.1832443235299763 ) ) ;
#65706=EDGE_CURVE ( 'NONE', #17773, #32982, #2540, .T. ) ;
#65707=ORIENTED_EDGE ( 'NONE', *, *, #58672, .T. ) ;
#65711=CARTESIAN_POINT ( 'NONE',  ( 29.77381068363827055, -48.62134037875150483, 300.4678068554150059 ) ) ;
#65712=ORIENTED_EDGE ( 'NONE', *, *, #7325, .F. ) ;
#65713=EDGE_LOOP ( 'NONE', ( #6191, #75723 ) ) ;
#65714=FACE_OUTER_BOUND ( 'NONE', #15484, .T. ) ;
#65716=CARTESIAN_POINT ( 'NONE',  ( 116.7450715690984140, -32.85492016819326722, 54.12991099019698282 ) ) ;
#65717=PLANE ( 'NONE',  #76540 ) ;
#65719=CARTESIAN_POINT ( 'NONE',  ( 99.04406186618773233, -42.84125764973450856, 72.84395861022517238 ) ) ;
#65720=CARTESIAN_POINT ( 'NONE',  ( 107.3052971647831555, -26.36210646096926524, 75.04610146638796664 ) ) ;
#65722=CARTESIAN_POINT ( 'NONE',  ( 101.9951592035502586, -45.85337710724431304, 183.1727681330539781 ) ) ;
#65723=CARTESIAN_POINT ( 'NONE',  ( 97.31592924394860233, -39.30618500135939541, 61.53147658036623824 ) ) ;
#65724=CARTESIAN_POINT ( 'NONE',  ( 83.56670390244801183, -36.72944715994108122, 218.8274735512160589 ) ) ;
#65727=DIRECTION ( 'NONE',  ( 0.000000000000000000, 1.000000000000000000, 0.000000000000000000 ) ) ;
#65728=CARTESIAN_POINT ( 'NONE',  ( 109.7268104826868722, -27.00131123978085768, 134.8646848310448263 ) ) ;
#65729=DIRECTION ( 'NONE',  ( 4.299999999999999979E-14, -1.000000000000000000, 4.400000000000000367E-29 ) ) ;
#65730=CARTESIAN_POINT ( 'NONE',  ( 98.50147650033493107, -30.70887204493662281, 205.8384824187679669 ) ) ;
#65731=ORIENTED_EDGE ( 'NONE', *, *, #18603, .F. ) ;
#65732=CARTESIAN_POINT ( 'NONE',  ( 107.0664832912739399, -36.72944715994095333, 311.6343304127839815 ) ) ;
#65733=CARTESIAN_POINT ( 'NONE',  ( 117.3563231384421357, -34.92488217824808316, 239.9641967044819637 ) ) ;
#65734=CARTESIAN_POINT ( 'NONE',  ( 108.2817482635038147, -26.29579267872783177, 125.9841967044819597 ) ) ;
#65735=DIRECTION ( 'NONE',  ( 0.000000000000000000, 0.000000000000000000, -1.000000000000000000 ) ) ;
#65737=DIRECTION ( 'NONE',  ( 0.000000000000000000, 0.000000000000000000, -1.000000000000000000 ) ) ;
#65739=EDGE_LOOP ( 'NONE', ( #52372, #39027 ) ) ;
#65741=VECTOR ( 'NONE', #47267, 999.9999999999998863 ) ;
#65743=ORIENTED_EDGE ( 'NONE', *, *, #42687, .F. ) ;
#65745=VERTEX_POINT ( 'NONE', #28903 ) ;
#65746=CARTESIAN_POINT ( 'NONE',  ( 30.48091746481741637, -48.32844715994156815, 180.4678068554150911 ) ) ;
#65747=CARTESIAN_POINT ( 'NONE',  ( 106.1383564330493812, -47.74364531592736682, 258.4975300378158636 ) ) ;
#65748=LINE ( 'NONE', #78524, #31579 ) ;
#65749=CARTESIAN_POINT ( 'NONE',  ( 131.5185316161781088, -35.69475198630853896, 2.828485944707569644 ) ) ;
#65752=CARTESIAN_POINT ( 'NONE',  ( 107.9802517323619355, -45.22186489331556203, 202.0838483995049728 ) ) ;
#65755=ORIENTED_EDGE ( 'NONE', *, *, #29390, .T. ) ;
#65757=FACE_OUTER_BOUND ( 'NONE', #21695, .T. ) ;
#65758=CARTESIAN_POINT ( 'NONE',  ( 97.86672394365611183, -40.64956911969122189, 181.6470188064607214 ) ) ;
#65759=DIRECTION ( 'NONE',  ( 0.000000000000000000, 0.000000000000000000, 1.000000000000000000 ) ) ;
#65761=CARTESIAN_POINT ( 'NONE',  ( 111.4279401658702682, -28.40658880358809668, 11.11205949637394852 ) ) ;
#65763=EDGE_CURVE ( 'NONE', #10951, #41323, #36617, .T. ) ;
#65764=VECTOR ( 'NONE', #85015, 1000.000000000000000 ) ;
#65766=CARTESIAN_POINT ( 'NONE',  ( 168.5667039024542362, -48.82844715994099971, 249.9678068554149775 ) ) ;
#65767=ADVANCED_FACE ( 'NONE', ( #63410 ), #1193, .F. ) ;
#65768=ORIENTED_EDGE ( 'NONE', *, *, #10292, .F. ) ;
#65770=CARTESIAN_POINT ( 'NONE',  ( 104.6834293286043760, -27.01143314437436160, 56.26782653584942295 ) ) ;
#65773=CARTESIAN_POINT ( 'NONE',  ( 114.4327864602578870, -33.21273682179715792, 16.99951894101997496 ) ) ;
#65776=LINE ( 'NONE', #44886, #17439 ) ;
#65777=EDGE_CURVE ( 'NONE', #40724, #80398, #66978, .T. ) ;
#65778=DIRECTION ( 'NONE',  ( 1.000000000000000000, 4.299999999999999979E-14, 1.000000000000000078E-15 ) ) ;
#65781=CARTESIAN_POINT ( 'NONE',  ( 97.81305373959743577, -40.51655628150228949, 62.63606721061723448 ) ) ;
#65785=CARTESIAN_POINT ( 'NONE',  ( 108.9848901524495801, -47.61516268848960465, 122.7032443235299723 ) ) ;
#65786=ORIENTED_EDGE ( 'NONE', *, *, #62941, .F. ) ;
#65787=CARTESIAN_POINT ( 'NONE',  ( 98.15782025887804707, -38.35683565110198145, 50.90480078045794698 ) ) ;
#65788=EDGE_CURVE ( 'NONE', #58630, #29906, #4353, .T. ) ;
#65789=CARTESIAN_POINT ( 'NONE',  ( 102.0296606431220994, -28.79805742369273958, 61.94634521065894717 ) ) ;
#65790=CARTESIAN_POINT ( 'NONE',  ( 116.3181387014812458, -32.94505625723229514, 15.13562527591094664 ) ) ;
#65791=CARTESIAN_POINT ( 'NONE',  ( 51.06670390244678970, -32.29483332968568021, 117.4678068554150485 ) ) ;
#65792=FACE_OUTER_BOUND ( 'NONE', #43373, .T. ) ;
#65793=CARTESIAN_POINT ( 'NONE',  ( 96.15481094519168437, -38.63223783578033022, 42.45181575210199298 ) ) ;
#65794=LINE ( 'NONE', #52147, #85881 ) ;
#65796=AXIS2_PLACEMENT_3D ( 'NONE', #3073, #24852, #23969 ) ;
#65797=CARTESIAN_POINT ( 'NONE',  ( 130.0664832912740110, -18.82844715994099971, 239.5838068554170377 ) ) ;
#65802=ORIENTED_EDGE ( 'NONE', *, *, #42935, .T. ) ;
#65804=EDGE_CURVE ( 'NONE', #37435, #34937, #79780, .T. ) ;
#65805=CARTESIAN_POINT ( 'NONE',  ( 114.8736367985563334, -30.83777597042981711, 219.3413395616259720 ) ) ;
#65806=ADVANCED_FACE ( 'NONE', ( #57933 ), #80625, .F. ) ;
#65807=CARTESIAN_POINT ( 'NONE',  ( 97.80998548426093464, -40.51326460879650426, 126.6348148350811584 ) ) ;
#65808=DIRECTION ( 'NONE',  ( 1.000000000000000000, 0.000000000000000000, 0.000000000000000000 ) ) ;
#65809=CARTESIAN_POINT ( 'NONE',  ( 117.4545169724989648, -37.95830395151629943, 49.73276813305393773 ) ) ;
#65810=CARTESIAN_POINT ( 'NONE',  ( 112.0656721949375481, -45.48853664962202004, 43.98977015968678472 ) ) ;
#65813=CARTESIAN_POINT ( 'NONE',  ( 103.4714990137023278, -27.39756209775824303, 171.3690893672466871 ) ) ;
#65814=ADVANCED_FACE ( 'NONE', ( #65638 ), #40583, .F. ) ;
#65815=DIRECTION ( 'NONE',  ( 4.299999999999999979E-14, -1.000000000000000000, 4.400000000000000367E-29 ) ) ;
#65816=VERTEX_POINT ( 'NONE', #87433 ) ;
#65817=AXIS2_PLACEMENT_3D ( 'NONE', #83458, #76643, #14428 ) ;
#65818=CARTESIAN_POINT ( 'NONE',  ( 59.67079009362632291, -0.9310397146383332379, 396.9756252759102040 ) ) ;
#65819=AXIS2_PLACEMENT_3D ( 'NONE', #1208, #56600, #75716 ) ;
#65820=CARTESIAN_POINT ( 'NONE',  ( 116.7940759412587539, -39.39156663991244756, 114.6154222936379767 ) ) ;
#65821=CARTESIAN_POINT ( 'NONE',  ( 105.1150531980676277, -26.51080800785435443, 235.2270538473399313 ) ) ;
#65822=LINE ( 'NONE', #3606, #67557 ) ;
#65824=DIRECTION ( 'NONE',  ( -2.900000000000000265E-14, 2.000000000000000155E-15, -1.000000000000000000 ) ) ;
#65825=CARTESIAN_POINT ( 'NONE',  ( 104.7063189284543370, -28.49041042582816630, 224.7209912566489720 ) ) ;
#65826=LINE ( 'NONE', #25392, #2638 ) ;
#65827=CARTESIAN_POINT ( 'NONE',  ( 97.28692064948108964, -31.62807703868918807, 86.93181575210095957 ) ) ;
#65828=B_SPLINE_CURVE_WITH_KNOTS ( 'NONE', 3,
 ( #39256, #75124, #6529, #33784, #61035, #47393, #89212, #81068, #75581, #87862, #46944, #61930, #53749, #5191, #46046, #40139, #89662, #12453, #82407, #20169, #33339, #47843, #12908, #11564, #41039, #88325, #68761, #73778 ),
 .UNSPECIFIED., .F., .F.,
 ( 4, 2, 2, 2, 2, 2, 2, 2, 2, 2, 1, 1, 1, 1, 2, 4 ),
 ( 0.000000000000000000, 0.06250376353546895081, 0.1250075270709379016, 0.1875112906064068663, 0.2500150541418758032, 0.3125188176773447402, 0.3750225812128137326, 0.4375263447482826695, 0.4687782265160169715, 0.4844041673998840669, 0.4922171378418173648, 0.4961236230627839028, 0.4980768656732669775, 0.4990534869785083760, 0.4995417976311288810, 0.5000301082837493860 ),
 .UNSPECIFIED. ) ;
#65830=CARTESIAN_POINT ( 'NONE',  ( 103.1890357985451345, -46.49249970849451330, 117.2756252759109543 ) ) ;
#65831=ORIENTED_EDGE ( 'NONE', *, *, #16353, .F. ) ;
#65832=CARTESIAN_POINT ( 'NONE',  ( 132.4924365228261536, -20.98954602992296614, 7.829737527534494923 ) ) ;
#65834=DIRECTION ( 'NONE',  ( 0.000000000000000000, 1.000000000000000000, 0.000000000000000000 ) ) ;
#65835=VECTOR ( 'NONE', #41629, 1000.000000000000000 ) ;
#65836=DIRECTION ( 'NONE',  ( -4.237773401492740281E-14, 1.000000000000000000, 0.000000000000000000 ) ) ;
#65837=DIRECTION ( 'NONE',  ( 0.000000000000000000, 1.000000000000000000, 0.000000000000000000 ) ) ;
#65838=ORIENTED_EDGE ( 'NONE', *, *, #24705, .F. ) ;
#65839=CARTESIAN_POINT ( 'NONE',  ( 97.53193540606868339, -39.74924357547732967, 51.57055488991837677 ) ) ;
#65840=CARTESIAN_POINT ( 'NONE',  ( 97.89382931228060158, -31.60946541130721954, 110.9213395616259703 ) ) ;
#65843=DIRECTION ( 'NONE',  ( 0.000000000000000000, 0.000000000000000000, -1.000000000000000000 ) ) ;
#65845=VERTEX_POINT ( 'NONE', #18376 ) ;
#65846=CARTESIAN_POINT ( 'NONE',  ( 114.7877796877764922, -44.67155160988957618, 118.2022919425779719 ) ) ;
#65848=CARTESIAN_POINT ( 'NONE',  ( 162.9033555647770015, -33.89581943344391135, -5.074374724088000832 ) ) ;
#65850=CARTESIAN_POINT ( 'NONE',  ( 107.0664832912739399, -36.72944715994095333, 299.5571190294419921 ) ) ;
#65852=VERTEX_POINT ( 'NONE', #85666 ) ;
#65853=ORIENTED_EDGE ( 'NONE', *, *, #26281, .F. ) ;
#65856=LINE ( 'NONE', #32232, #79303 ) ;
#65857=CARTESIAN_POINT ( 'NONE',  ( 116.3186249068867539, -32.94868901193379429, 250.1356252759109395 ) ) ;
#65859=LINE ( 'NONE', #36833, #52317 ) ;
#65860=CIRCLE ( 'NONE', #7839, 4.875000000000017764 ) ;
#65861=ORIENTED_EDGE ( 'NONE', *, *, #15384, .T. ) ;
#65862=( BOUNDED_CURVE ( )  B_SPLINE_CURVE ( 3, ( #85758, #59791, #58022, #23530 ),
 .UNSPECIFIED., .F., .T. ) 
 B_SPLINE_CURVE_WITH_KNOTS ( ( 4, 4 ),
 ( 1.040426005086875085E-11, 1.570796326807755605 ),
 .UNSPECIFIED. ) 
 CURVE ( )  GEOMETRIC_REPRESENTATION_ITEM ( )  RATIONAL_B_SPLINE_CURVE ( ( 1.000000000000000000, 0.8047378541237864003, 0.8047378541237864003, 1.000000000000000000 ) ) 
 REPRESENTATION_ITEM ( '' )  );
#65866=ADVANCED_FACE ( 'NONE', ( #51983 ), #78850, .F. ) ;
#65867=CARTESIAN_POINT ( 'NONE',  ( 116.6769215743979800, -34.91203320259896259, 154.9756252759109714 ) ) ;
#65868=CARTESIAN_POINT ( 'NONE',  ( 142.8679068202682458, 10.65431904611001634, 540.9756252759101471 ) ) ;
#65869=VERTEX_POINT ( 'NONE', #79297 ) ;
#65870=EDGE_CURVE ( 'NONE', #49327, #81785, #25192, .T. ) ;
#65871=CARTESIAN_POINT ( 'NONE',  ( 115.8115096128641284, -32.27542772465451293, 40.20133956162496958 ) ) ;
#65872=CARTESIAN_POINT ( 'NONE',  ( 97.86672743208310976, -40.64957730801459235, 51.64701951407019465 ) ) ;
#65873=CARTESIAN_POINT ( 'NONE',  ( 184.5667039024486087, -48.82844715993447693, 129.9678068554150059 ) ) ;
#65874=EDGE_CURVE ( 'NONE', #89527, #8395, #62364, .T. ) ;
#65879=CARTESIAN_POINT ( 'NONE',  ( 104.8455658278054017, -28.15064746346142144, 196.7101547344689720 ) ) ;
#65882=FACE_OUTER_BOUND ( 'NONE', #63844, .T. ) ;
#65883=CIRCLE ( 'NONE', #38329, 9.571100913904478702 ) ;
#65884=AXIS2_PLACEMENT_3D ( 'NONE', #11751, #47138, #73972 ) ;
#65886=CIRCLE ( 'NONE', #19473, 11.57110091390449469 ) ;
#65887=ADVANCED_FACE ( 'NONE', ( #51546 ), #10235, .T. ) ;
#65888=CARTESIAN_POINT ( 'NONE',  ( 116.3251852747984003, -32.94148267319277323, 269.1356252759109680 ) ) ;
#65892=CARTESIAN_POINT ( 'NONE',  ( 25.56670390244816815, -42.82844715994167473, 295.7178068554150059 ) ) ;
#65893=AXIS2_PLACEMENT_3D ( 'NONE', #2443, #38725, #52764 ) ;
#65894=CARTESIAN_POINT ( 'NONE',  ( 97.80400447685593690, -40.49859989475246635, 37.63371632713159443 ) ) ;
#65895=VERTEX_POINT ( 'NONE', #37498 ) ;
#65896=CARTESIAN_POINT ( 'NONE',  ( 104.8459308146384643, -26.52976224399699134, 260.2470538473397710 ) ) ;
#65897=CARTESIAN_POINT ( 'NONE',  ( 80.06648329127399677, -41.22944715994105280, 1.625625275910943746 ) ) ;
#65898=VERTEX_POINT ( 'NONE', #65201 ) ;
#65899=EDGE_CURVE ( 'NONE', #27672, #63459, #44921, .T. ) ;
#65900=PLANE ( 'NONE',  #63365 ) ;
#65901=LINE ( 'NONE', #10500, #89713 ) ;
#65903=CARTESIAN_POINT ( 'NONE',  ( 34.27482367531500529, -30.08671355700301575, -5.074374724088000832 ) ) ;
#65904=EDGE_CURVE ( 'NONE', #57650, #20562, #37939, .T. ) ;
#65905=CARTESIAN_POINT ( 'NONE',  ( 106.2987435450237541, -47.16992394167115776, 218.5184824187679453 ) ) ;
#65907=ORIENTED_EDGE ( 'NONE', *, *, #3957, .T. ) ;
#65908=CARTESIAN_POINT ( 'NONE',  ( 97.73362116697985869, -31.98701483920769206, 46.95276813305393659 ) ) ;
#65909=CARTESIAN_POINT ( 'NONE',  ( 72.17003668186622178, -9.772340378754034163, -5.074374724089137700 ) ) ;
#65910=CARTESIAN_POINT ( 'NONE',  ( 100.4512775726424820, -44.84301714363712676, 12.03276813305398463 ) ) ;
#65911=ORIENTED_EDGE ( 'NONE', *, *, #31518, .T. ) ;
#65912=CARTESIAN_POINT ( 'NONE',  ( 81.01407827912979087, -16.14703303315387117, 1.764000745017404004 ) ) ;
#65914=CARTESIAN_POINT ( 'NONE',  ( 116.3162492855249894, -32.94856389518969308, 154.1356252759109680 ) ) ;
#65915=CARTESIAN_POINT ( 'NONE',  ( 108.6369934722860506, -45.24028864696019525, 125.5518998934009574 ) ) ;
#65916=CARTESIAN_POINT ( 'NONE',  ( 114.6212291911790402, -29.51397259194560263, 230.4327681330539690 ) ) ;
#65918=ORIENTED_EDGE ( 'NONE', *, *, #68840, .T. ) ;
#65919=ADVANCED_FACE ( 'NONE', ( #19287 ), #8711, .T. ) ;
#65920=CARTESIAN_POINT ( 'NONE',  ( 135.7780479399384603, -38.88970947304356685, 2.099345637345863658 ) ) ;
#65921=ORIENTED_EDGE ( 'NONE', *, *, #20497, .F. ) ;
#65923=VECTOR ( 'NONE', #39932, 1000.000000000000000 ) ;
#65924=CARTESIAN_POINT ( 'NONE',  ( 180.2143765759500980, -35.91149509760582248, 237.4678068554150059 ) ) ;
#65925=ORIENTED_EDGE ( 'NONE', *, *, #84066, .T. ) ;
#65927=CARTESIAN_POINT ( 'NONE',  ( 80.06648329127398256, -18.72944715994105991, 14.92562527591094224 ) ) ;
#65928=VECTOR ( 'NONE', #31659, 1000.000000000000000 ) ;
#65929=CARTESIAN_POINT ( 'NONE',  ( 142.0664832912739826, -9.729447159940995959, 14.67562527591100441 ) ) ;
#65931=CARTESIAN_POINT ( 'NONE',  ( 108.6382307137633205, -45.64809506003439310, 122.1257531614099747 ) ) ;
#65932=CARTESIAN_POINT ( 'NONE',  ( 105.3130012014428445, -26.40811315510063295, 15.20991099019697401 ) ) ;
#65933=VERTEX_POINT ( 'NONE', #12925 ) ;
#65939=DIRECTION ( 'NONE',  ( 6.524622321627019585E-16, 3.741823817616790462E-31, 1.000000000000000000 ) ) ;
#65940=DIRECTION ( 'NONE',  ( -0.9254794337955620787, -0.3787978585227822492, 0.000000000000000000 ) ) ;
#65941=CARTESIAN_POINT ( 'NONE',  ( 72.06648329127402519, -56.72944715994105991, 14.92562527591093691 ) ) ;
#65943=CYLINDRICAL_SURFACE ( 'NONE', #77025, 2.517500000000005844 ) ;
#65946=CARTESIAN_POINT ( 'NONE',  ( 118.1077515449285613, -36.21032982800684152, 268.8518157521015723 ) ) ;
#65948=CARTESIAN_POINT ( 'NONE',  ( 116.1963150171851851, -43.04653558477239272, 9.356577656862985037 ) ) ;
#65949=AXIS2_PLACEMENT_3D ( 'NONE', #89010, #26766, #73235 ) ;
#65951=LINE ( 'NONE', #37819, #14349 ) ;
#65953=CARTESIAN_POINT ( 'NONE',  ( 106.4181540149052694, -25.28825685635689879, 323.5297110109900132 ) ) ;
#65955=CARTESIAN_POINT ( 'NONE',  ( 50.56670390244696733, -18.82844715994099971, 342.9256252759109884 ) ) ;
#65957=CYLINDRICAL_SURFACE ( 'NONE', #51504, 2.749999999999974687 ) ;
#65958=CARTESIAN_POINT ( 'NONE',  ( 102.7370178780992234, -25.64411770250132250, 20.37276813305294354 ) ) ;
#65959=CARTESIAN_POINT ( 'NONE',  ( 107.2431676328701684, -47.18842012194354396, 208.5899109901969837 ) ) ;
#65960=CARTESIAN_POINT ( 'NONE',  ( 99.11086226171772751, -44.43615201859483932, 37.95086337114900488 ) ) ;
#65961=LINE ( 'NONE', #3753, #5851 ) ;
#65962=CARTESIAN_POINT ( 'NONE',  ( 109.6430121329437952, -46.48008673454590678, 47.78145860943909895 ) ) ;
#65963=CARTESIAN_POINT ( 'NONE',  ( 82.68053975348409779, -35.85322261660355281, 2.908039740960799868 ) ) ;
#65964=CIRCLE ( 'NONE', #25387, 2.999999999999929834 ) ;
#65966=ADVANCED_FACE ( 'NONE', ( #47412 ), #25642, .T. ) ;
#65968=ORIENTED_EDGE ( 'NONE', *, *, #6516, .T. ) ;
#65970=CARTESIAN_POINT ( 'NONE',  ( 97.58158007118578325, -32.53714515026965870, 51.98324432352896451 ) ) ;
#65972=EDGE_LOOP ( 'NONE', ( #72530, #65645, #2047, #21013 ) ) ;
#65973=CARTESIAN_POINT ( 'NONE',  ( 50.56670390244699576, -18.82844715994031048, -5.074374724088000832 ) ) ;
#65974=EDGE_CURVE ( 'NONE', #28680, #62123, #75140, .T. ) ;
#65975=CARTESIAN_POINT ( 'NONE',  ( 117.1710321396410421, -41.15233254730026147, 204.4861014663869696 ) ) ;
#65976=CARTESIAN_POINT ( 'NONE',  ( 99.50407054466384693, -43.30503144106609881, 252.8967269992471358 ) ) ;
#65977=CARTESIAN_POINT ( 'NONE',  ( 110.8545073367433105, -45.98422289188966516, 147.8856283147305248 ) ) ;
#65978=PLANE ( 'NONE',  #70449 ) ;
#65980=CARTESIAN_POINT ( 'NONE',  ( 132.9844404253383630, -39.25772566032902944, 1.807989669955520684 ) ) ;
#65983=CARTESIAN_POINT ( 'NONE',  ( 98.99072789581755671, -31.21169308021397981, 120.8499109901969604 ) ) ;
#65985=VERTEX_POINT ( 'NONE', #54660 ) ;
#65987=CARTESIAN_POINT ( 'NONE',  ( 109.6943014565619450, -45.19247559555673632, 94.24729759161093057 ) ) ;
#65989=CARTESIAN_POINT ( 'NONE',  ( 80.06648329127399677, -8.729447159940999512, 4.925625275911999168 ) ) ;
#65990=CARTESIAN_POINT ( 'NONE',  ( 107.2322476904470108, -46.54200526979089858, 208.5899109901959605 ) ) ;
#65992=DIRECTION ( 'NONE',  ( 4.299999999999999979E-14, -1.000000000000000000, 0.000000000000000000 ) ) ;
#65994=EDGE_CURVE ( 'NONE', #44882, #26742, #89229, .T. ) ;
#65999=CARTESIAN_POINT ( 'NONE',  ( 108.2752786314947429, -47.69320359391970499, 157.6518157521019532 ) ) ;
#66003=CARTESIAN_POINT ( 'NONE',  ( 71.24189083761805819, -0.9290567490904538817, 361.9756252759101471 ) ) ;
#66006=VECTOR ( 'NONE', #50232, 1000.000000000000000 ) ;
#66008=CARTESIAN_POINT ( 'NONE',  ( 117.0718958548293784, -35.46248428096206595, 269.9272917895399360 ) ) ;
#66010=AXIS2_PLACEMENT_3D ( 'NONE', #69166, #62343, #55955 ) ;
#66011=CARTESIAN_POINT ( 'NONE',  ( 98.66574799139598895, -30.49618532553466110, 180.8184824187679567 ) ) ;
#66013=ORIENTED_EDGE ( 'NONE', *, *, #71441, .F. ) ;
#66016=CIRCLE ( 'NONE', #79085, 2.749999999999974687 ) ;
#66018=PLANE ( 'NONE',  #56473 ) ;
#66019=CARTESIAN_POINT ( 'NONE',  ( 131.5867845949809691, -35.53883969338462379, 7.103318745415927893 ) ) ;
#66020=CARTESIAN_POINT ( 'NONE',  ( 105.4026065362546802, -27.48239143091520020, 271.6377737820876632 ) ) ;
#66022=DIRECTION ( 'NONE',  ( 1.346944695195362088E-15, -1.000000000000000000, 3.469446951953620425E-31 ) ) ;
#66025=VECTOR ( 'NONE', #10473, 1000.000000000000000 ) ;
#66026=LINE ( 'NONE', #46011, #45074 ) ;
#66027=PLANE ( 'NONE',  #76392 ) ;
#66029=ORIENTED_EDGE ( 'NONE', *, *, #77614, .T. ) ;
#66030=CARTESIAN_POINT ( 'NONE',  ( 152.0371591254585724, -47.82818131005588214, 129.9678068554149775 ) ) ;
#66033=CARTESIAN_POINT ( 'NONE',  ( 97.33768314765630691, -34.07170803572551421, 157.1146345946560530 ) ) ;
#66034=VECTOR ( 'NONE', #5198, 1000.000000000000000 ) ;
#66035=CARTESIAN_POINT ( 'NONE',  ( 101.0819131387675611, -42.86434890131523900, 21.38384839950496641 ) ) ;
#66036=CARTESIAN_POINT ( 'NONE',  ( 100.6239562591623695, -26.75308202300568539, 220.5327681330539633 ) ) ;
#66037=CARTESIAN_POINT ( 'NONE',  ( 118.8526415125689937, -37.69623653580512723, 188.7613395616259595 ) ) ;
#66038=DIRECTION ( 'NONE',  ( 0.000000000000000000, 1.000000000000000000, 0.000000000000000000 ) ) ;
#66039=CARTESIAN_POINT ( 'NONE',  ( 96.24939603668094890, -34.45687069020234361, 257.1737205140064475 ) ) ;
#66041=CARTESIAN_POINT ( 'NONE',  ( 75.31670390244798341, -57.40094715994099772, 60.91780685541480267 ) ) ;
#66042=ORIENTED_EDGE ( 'NONE', *, *, #40222, .F. ) ;
#66043=ORIENTED_EDGE ( 'NONE', *, *, #42587, .F. ) ;
#66044=CIRCLE ( 'NONE', #24003, 0.5000000000000004441 ) ;
#66046=CARTESIAN_POINT ( 'NONE',  ( 118.8398422492546018, -38.46634565031615693, 223.7099109901969598 ) ) ;
#66048=CARTESIAN_POINT ( 'NONE',  ( 109.8560245667294311, -26.68427469084152293, 174.8613395616249591 ) ) ;
#66051=DIRECTION ( 'NONE',  ( -0.7071067811734105257, 0.7071067811996846197, 0.000000000000000000 ) ) ;
#66055=DIRECTION ( 'NONE',  ( -4.237773401492740281E-14, 1.000000000000000000, 0.000000000000000000 ) ) ;
#66057=CARTESIAN_POINT ( 'NONE',  ( 110.8002664325828164, -46.40403567634503901, 13.85753003781498016 ) ) ;
#66058=CARTESIAN_POINT ( 'NONE',  ( 107.0664832912739968, -36.72944715994100306, 293.2242906452868851 ) ) ;
#66060=CARTESIAN_POINT ( 'NONE',  ( 164.9212702847350442, -29.73316016639542170, 342.9256252759109884 ) ) ;
#66061=CARTESIAN_POINT ( 'NONE',  ( 107.0664832912739968, -36.72944715994100306, 287.6356252759109680 ) ) ;
#66062=DIRECTION ( 'NONE',  ( 0.000000000000000000, 0.000000000000000000, 1.000000000000000000 ) ) ;
#66063=CARTESIAN_POINT ( 'NONE',  ( 162.5667039024470171, -32.29483332968611364, -5.074374724088000832 ) ) ;
#66064=CARTESIAN_POINT ( 'NONE',  ( 100.1227369335950215, -41.05608255646721005, 195.5838068554172935 ) ) ;
#66066=CARTESIAN_POINT ( 'NONE',  ( 126.9629299006807059, -54.68655584847603279, 14.92562527591094579 ) ) ;
#66067=CARTESIAN_POINT ( 'NONE',  ( 97.40467406345878487, -42.14653896106843689, 181.7451490854349743 ) ) ;
#66068=CARTESIAN_POINT ( 'NONE',  ( 109.6838526317122273, -47.46831852615197533, 83.75467289495897205 ) ) ;
#66069=CARTESIAN_POINT ( 'NONE',  ( 118.0968619800241299, -35.49322535880637020, 229.9032443235299468 ) ) ;
#66070=LINE ( 'NONE', #74687, #35856 ) ;
#66073=CARTESIAN_POINT ( 'NONE',  ( 99.41715255677500807, -43.19881440323307231, 37.88476161017977972 ) ) ;
#66075=FACE_OUTER_BOUND ( 'NONE', #80046, .T. ) ;
#66076=CARTESIAN_POINT ( 'NONE',  ( 97.75843116786518294, -40.38500386429194577, 66.62475028590972670 ) ) ;
#66078=AXIS2_PLACEMENT_3D ( 'NONE', #40062, #88691, #47763 ) ;
#66079=CIRCLE ( 'NONE', #10970, 0.5000000000000031086 ) ;
#66082=ADVANCED_FACE ( 'NONE', ( #53769 ), #13808, .T. ) ;
#66084=CARTESIAN_POINT ( 'NONE',  ( 115.6929481903037100, -41.18531195142565338, 92.86956268521994673 ) ) ;
#66086=EDGE_LOOP ( 'NONE', ( #85928, #35514, #12990, #22562 ) ) ;
#66087=ADVANCED_FACE ( 'NONE', ( #81534 ), #18834, .T. ) ;
#66088=CARTESIAN_POINT ( 'NONE',  ( 95.51222647996985415, -34.21005103128004521, 102.1556252759109640 ) ) ;
#66089=DIRECTION ( 'NONE',  ( 0.000000000000000000, -1.000000000000000000, 0.000000000000000000 ) ) ;
#66090=EDGE_CURVE ( 'NONE', #88057, #68436, #26069, .T. ) ;
#66092=DIRECTION ( 'NONE',  ( 1.000000000000000000, 0.000000000000000000, 0.000000000000000000 ) ) ;
#66093=CARTESIAN_POINT ( 'NONE',  ( 97.06107109313440162, -37.99641192960685032, 177.4272919398598560 ) ) ;
#66094=EDGE_CURVE ( 'NONE', #27069, #67994, #69224, .T. ) ;
#66096=CARTESIAN_POINT ( 'NONE',  ( 101.9462936730086113, -46.59842863024385196, 17.19562527591095247 ) ) ;
#66097=ORIENTED_EDGE ( 'NONE', *, *, #34809, .T. ) ;
#66098=ORIENTED_EDGE ( 'NONE', *, *, #14236, .F. ) ;
#66099=EDGE_LOOP ( 'NONE', ( #67713, #32170, #86945, #57316 ) ) ;
#66101=CARTESIAN_POINT ( 'NONE',  ( 98.54774150848832903, -41.53511815344519675, 132.7356252759109623 ) ) ;
#66102=CARTESIAN_POINT ( 'NONE',  ( 123.6837132603319702, -55.86395651782485317, 219.5838068554170093 ) ) ;
#66105=LINE ( 'NONE', #16638, #69361 ) ;
#66108=DIRECTION ( 'NONE',  ( -7.723290606088049820E-15, 0.000000000000000000, 1.000000000000000000 ) ) ;
#66110=CARTESIAN_POINT ( 'NONE',  ( 63.06670390244707392, -40.32844715994016838, 180.4678068554151196 ) ) ;
#66111=CARTESIAN_POINT ( 'NONE',  ( 105.9906760191434358, -26.38192068051316141, 50.15848241876796720 ) ) ;
#66112=ORIENTED_EDGE ( 'NONE', *, *, #41864, .T. ) ;
#66113=EDGE_LOOP ( 'NONE', ( #3041, #66644 ) ) ;
#66116=FACE_OUTER_BOUND ( 'NONE', #81737, .T. ) ;
#66117=CARTESIAN_POINT ( 'NONE',  ( 114.6841822258597148, -33.79680514827971649, 136.9366617981629588 ) ) ;
#66118=AXIS2_PLACEMENT_3D ( 'NONE', #81491, #52377, #66939 ) ;
#66119=CARTESIAN_POINT ( 'NONE',  ( 59.67078992371373403, -0.9290567490904538817, 540.9756252759101471 ) ) ;
#66121=EDGE_LOOP ( 'NONE', ( #30888, #85117, #224, #63616 ) ) ;
#66123=EDGE_LOOP ( 'NONE', ( #32854, #47080, #9404, #25303 ) ) ;
#66125=DIRECTION ( 'NONE',  ( -8.673617379884035472E-16, -1.000000000000000000, 0.000000000000000000 ) ) ;
#66126=CARTESIAN_POINT ( 'NONE',  ( 112.5904859203986206, -43.69705252635404236, 164.5415833058969781 ) ) ;
#66127=LINE ( 'NONE', #18887, #25461 ) ;
#66128=VECTOR ( 'NONE', #16330, 1000.000000000000000 ) ;
#66131=DIRECTION ( 'NONE',  ( 0.000000000000000000, 0.000000000000000000, 1.000000000000000000 ) ) ;
#66132=AXIS2_PLACEMENT_3D ( 'NONE', #54137, #12390, #19647 ) ;
#66133=ORIENTED_EDGE ( 'NONE', *, *, #88470, .F. ) ;
#66136=EDGE_LOOP ( 'NONE', ( #12932, #53844, #70248, #16337 ) ) ;
#66137=VERTEX_POINT ( 'NONE', #28314 ) ;
#66138=EDGE_CURVE ( 'NONE', #10255, #36562, #76837, .T. ) ;
#66139=CARTESIAN_POINT ( 'NONE',  ( 107.2048247310825388, -44.91868093929326022, 210.4080903695909512 ) ) ;
#66140=CARTESIAN_POINT ( 'NONE',  ( 116.9427733469681385, -33.21558069166144378, 114.0984824187679720 ) ) ;
#66141=CARTESIAN_POINT ( 'NONE',  ( 107.1951288810177090, -26.32694189238797833, 35.06705384733893283 ) ) ;
#66145=CARTESIAN_POINT ( 'NONE',  ( 109.8559662660393172, -26.68448463234438606, 170.8613395616249591 ) ) ;
#66147=ORIENTED_EDGE ( 'NONE', *, *, #9282, .F. ) ;
#66149=ORIENTED_EDGE ( 'NONE', *, *, #66094, .F. ) ;
#66150=EDGE_LOOP ( 'NONE', ( #235, #60006, #52899, #69830, #55373, #42028, #32066, #4810, #19490, #530, #38523, #87786, #13984 ) ) ;
#66151=CARTESIAN_POINT ( 'NONE',  ( 97.81169818311565223, -40.51742792548894556, 86.63555527419073599 ) ) ;
#66153=ORIENTED_EDGE ( 'NONE', *, *, #74293, .F. ) ;
#66156=VERTEX_POINT ( 'NONE', #77835 ) ;
#66158=CARTESIAN_POINT ( 'NONE',  ( 101.9604343285081569, -27.64015156285208974, 60.48419670448296159 ) ) ;
#66159=LINE ( 'NONE', #81171, #82331 ) ;
#66160=CIRCLE ( 'NONE', #44433, 14.00000000000000888 ) ;
#66161=CARTESIAN_POINT ( 'NONE',  ( 138.8167039024479834, -50.82844715994100682, 60.91780685541480267 ) ) ;
#66163=CARTESIAN_POINT ( 'NONE',  ( 99.36524671511898532, -42.81259845621070781, 91.85848241876892928 ) ) ;
#66164=CARTESIAN_POINT ( 'NONE',  ( 72.06648329127393993, -45.72944715994110965, 14.82207188531764253 ) ) ;
#66165=CARTESIAN_POINT ( 'NONE',  ( 101.2129617469313132, -45.32973500739954886, 193.1013395616249682 ) ) ;
#66166=DIRECTION ( 'NONE',  ( 0.000000000000000000, 0.000000000000000000, -1.000000000000000000 ) ) ;
#66167=CARTESIAN_POINT ( 'NONE',  ( 142.8682495647594806, 8.654319075478467127, 394.9756252759102040 ) ) ;
#66168=EDGE_LOOP ( 'NONE', ( #72815, #31172, #78444, #61981, #21995, #88797 ) ) ;
#66170=DIRECTION ( 'NONE',  ( 0.000000000000000000, 0.000000000000000000, -1.000000000000000000 ) ) ;
#66171=LINE ( 'NONE', #80724, #61851 ) ;
#66172=ADVANCED_FACE ( 'NONE', ( #56468 ), #84216, .F. ) ;
#66173=CARTESIAN_POINT ( 'NONE',  ( 25.56670390244832447, -48.82844715994168183, 257.2178068554150059 ) ) ;
#66174=CARTESIAN_POINT ( 'NONE',  ( 97.36106687025375095, -40.65520290104787904, 206.6327681330539860 ) ) ;
#66175=ORIENTED_EDGE ( 'NONE', *, *, #89403, .T. ) ;
#66176=DIRECTION ( 'NONE',  ( -4.237773401492740281E-14, 1.000000000000000000, 0.000000000000000000 ) ) ;
#66177=CARTESIAN_POINT ( 'NONE',  ( 100.7369725318012570, -45.81913908486538389, 233.0803871806729717 ) ) ;
#66178=CARTESIAN_POINT ( 'NONE',  ( 103.1892778894433320, -46.49189014610453086, 113.2756252759109827 ) ) ;
#66180=CARTESIAN_POINT ( 'NONE',  ( 81.24992100026079811, -39.21189388395703190, 8.006199623928925035 ) ) ;
#66181=DIRECTION ( 'NONE',  ( 4.299999999999999979E-14, -1.000000000000000000, 4.400000000000000367E-29 ) ) ;
#66183=ORIENTED_EDGE ( 'NONE', *, *, #77021, .F. ) ;
#66186=ORIENTED_EDGE ( 'NONE', *, *, #80783, .T. ) ;
#66187=CARTESIAN_POINT ( 'NONE',  ( 117.0718954856852321, -35.46248235822151429, 73.92729194242146207 ) ) ;
#66188=CARTESIAN_POINT ( 'NONE',  ( 111.7736368399375522, -46.73334422087322082, 283.9146728949585849 ) ) ;
#66189=LINE ( 'NONE', #38489, #41743 ) ;
#66190=CARTESIAN_POINT ( 'NONE',  ( 41.56648329127398966, -27.82844715994070484, 195.9256252759119832 ) ) ;
#66192=CARTESIAN_POINT ( 'NONE',  ( 150.5667039024473297, -25.42844715993594562, 300.4678068554149490 ) ) ;
#66195=CARTESIAN_POINT ( 'NONE',  ( 115.5432862745613676, -35.46615253551063063, 218.3667055423629790 ) ) ;
#66198=VECTOR ( 'NONE', #20107, 1000.000000000000000 ) ;
#66199=VERTEX_POINT ( 'NONE', #62841 ) ;
#66200=AXIS2_PLACEMENT_3D ( 'NONE', #38244, #73201, #65940 ) ;
#66201=CIRCLE ( 'NONE', #16886, 2.030000000000003801 ) ;
#66202=DIRECTION ( 'NONE',  ( 1.000000000000000000, 0.000000000000000000, 0.000000000000000000 ) ) ;
#66204=CARTESIAN_POINT ( 'NONE',  ( 110.8542088300284263, -45.98434506554588097, 182.8856026504752492 ) ) ;
#66206=CARTESIAN_POINT ( 'NONE',  ( 100.2657625843003899, -43.21224928579215430, 33.35205949637398959 ) ) ;
#66209=DIRECTION ( 'NONE',  ( 3.999999999999999995E-14, -1.000000000000000000, 4.100000000000000342E-29 ) ) ;
#66210=EDGE_CURVE ( 'NONE', #37176, #12768, #76483, .T. ) ;
#66213=DIRECTION ( 'NONE',  ( -0.7071067708032339194, -0.0001211784769831122661, 0.7071067811865472397 ) ) ;
#66214=ORIENTED_EDGE ( 'NONE', *, *, #67706, .T. ) ;
#66217=CARTESIAN_POINT ( 'NONE',  ( 101.5184502652259084, -42.71685524349225460, 44.79951894101996857 ) ) ;
#66218=VECTOR ( 'NONE', #39784, 1000.000000000000114 ) ;
#66219=CARTESIAN_POINT ( 'NONE',  ( 134.0664832912739826, -15.97944715994100306, 8.225625275910998013 ) ) ;
#66225=EDGE_LOOP ( 'NONE', ( #78, #9353, #7667 ) ) ;
#66226=CARTESIAN_POINT ( 'NONE',  ( 117.1637410210353210, -34.13475704353096063, 124.0270538473399426 ) ) ;
#66227=ORIENTED_EDGE ( 'NONE', *, *, #66374, .F. ) ;
#66228=CARTESIAN_POINT ( 'NONE',  ( 98.75910798445569583, -38.71530899645634349, 55.93527697093397677 ) ) ;
#66229=CARTESIAN_POINT ( 'NONE',  ( 104.4690831045889894, -46.42484882949283076, 88.36765422304442552 ) ) ;
#66230=CARTESIAN_POINT ( 'NONE',  ( 107.2073525216087120, -27.33494443775582639, 76.50824997256394511 ) ) ;
#66231=CARTESIAN_POINT ( 'NONE',  ( 136.8165183345649041, -18.90056224776383687, 3.101534470964332879 ) ) ;
#66234=CARTESIAN_POINT ( 'NONE',  ( 105.4175444341163939, -47.04536977979798706, 33.44991099019695469 ) ) ;
#66237=ORIENTED_EDGE ( 'NONE', *, *, #87867, .F. ) ;
#66244=CARTESIAN_POINT ( 'NONE',  ( 138.8167039024479834, -57.40094715994099772, 60.91780685541480267 ) ) ;
#66245=VERTEX_POINT ( 'NONE', #14265 ) ;
#66246=CARTESIAN_POINT ( 'NONE',  ( 112.8396959964676682, -44.62460075896473910, 228.0784824187689708 ) ) ;
#66247=CARTESIAN_POINT ( 'NONE',  ( 114.4495774554661836, -29.91993045966185250, 124.4189032693139865 ) ) ;
#66249=CARTESIAN_POINT ( 'NONE',  ( 110.4565933333529699, -47.24995733706104062, 53.83657765686300678 ) ) ;
#66252=CARTESIAN_POINT ( 'NONE',  ( 100.9537918767618976, -28.70771463842614679, 171.5940036888151781 ) ) ;
#66253=AXIS2_PLACEMENT_3D ( 'NONE', #74752, #88842, #47473 ) ;
#66256=VECTOR ( 'NONE', #36491, 1000.000000000000000 ) ;
#66259=ADVANCED_FACE ( 'NONE', ( #84657 ), #64205, .F. ) ;
#66260=DIRECTION ( 'NONE',  ( 1.000000000000000078E-15, 1.000000000000000083E-30, -1.000000000000000000 ) ) ;
#66261=CARTESIAN_POINT ( 'NONE',  ( 109.9541224118590890, -48.19721710984623542, 242.7727681330539724 ) ) ;
#66263=AXIS2_PLACEMENT_3D ( 'NONE', #22690, #50361, #9057 ) ;
#66266=CARTESIAN_POINT ( 'NONE',  ( 98.72788526414296939, -31.75567473670096774, 280.3209912566482558 ) ) ;
#66267=CARTESIAN_POINT ( 'NONE',  ( 168.0371591254545365, -48.62818131005519007, 193.9678068554149775 ) ) ;
#66268=CARTESIAN_POINT ( 'NONE',  ( 114.3378803067696197, -44.16957155219873243, 69.19276813305397411 ) ) ;
#66270=CARTESIAN_POINT ( 'NONE',  ( 102.2821109723304431, -27.37735778705684098, 120.4527681330539792 ) ) ;
#66273=ORIENTED_EDGE ( 'NONE', *, *, #61770, .F. ) ;
#66274=EDGE_CURVE ( 'NONE', #70541, #4931, #69670, .T. ) ;
#66275=DIRECTION ( 'NONE',  ( 0.000000000000000000, 0.000000000000000000, 1.000000000000000000 ) ) ;
#66278=CARTESIAN_POINT ( 'NONE',  ( 194.5667039024480403, -40.82844715993405771, 249.9678068554149775 ) ) ;
#66279=ORIENTED_EDGE ( 'NONE', *, *, #10737, .T. ) ;
#66281=EDGE_CURVE ( 'NONE', #64435, #54341, #42070, .T. ) ;
#66283=CARTESIAN_POINT ( 'NONE',  ( 98.42220671263785903, -30.82325138971081557, 120.8499109901969604 ) ) ;
#66284=ORIENTED_EDGE ( 'NONE', *, *, #15170, .T. ) ;
#66286=AXIS2_PLACEMENT_3D ( 'NONE', #88371, #40185, #5694 ) ;
#66287=DIRECTION ( 'NONE',  ( 4.194175870806139918E-14, -1.000000000000000000, 0.000000000000000000 ) ) ;
#66289=EDGE_CURVE ( 'NONE', #55083, #462, #36501, .T. ) ;
#66290=LINE ( 'NONE', #45391, #88698 ) ;
#66291=ORIENTED_EDGE ( 'NONE', *, *, #84432, .T. ) ;
#66292=VECTOR ( 'NONE', #74331, 1000.000000000000000 ) ;
#66293=CARTESIAN_POINT ( 'NONE',  ( 117.6304226258691727, -33.39798698885631012, 129.0575300378159795 ) ) ;
#66296=CARTESIAN_POINT ( 'NONE',  ( 167.7413838386817702, -48.33240602328261559, 249.9678068554149775 ) ) ;
#66297=CARTESIAN_POINT ( 'NONE',  ( 107.0664832912739399, -36.72944715994095333, 312.1356252759112522 ) ) ;
#66302=EDGE_CURVE ( 'NONE', #49032, #63259, #22879, .T. ) ;
#66305=CARTESIAN_POINT ( 'NONE',  ( 131.0667039024480118, -61.87844715994100397, 231.5838068554150198 ) ) ;
#66306=FACE_OUTER_BOUND ( 'NONE', #17349, .T. ) ;
#66309=CARTESIAN_POINT ( 'NONE',  ( 107.0620278373210539, -36.73691869758540207, 394.9756252759100903 ) ) ;
#66310=CARTESIAN_POINT ( 'NONE',  ( 114.8736367985562623, -30.83777597042988106, 215.3413395616249773 ) ) ;
#66311=DIRECTION ( 'NONE',  ( -1.000000000000000078E-15, -1.000000000000000083E-30, 1.000000000000000000 ) ) ;
#66312=VERTEX_POINT ( 'NONE', #85996 ) ;
#66313=EDGE_CURVE ( 'NONE', #67833, #74158, #10124, .T. ) ;
#66314=CARTESIAN_POINT ( 'NONE',  ( 116.6363502066642468, -38.74961609181404043, 59.66133956162394725 ) ) ;
#66315=CARTESIAN_POINT ( 'NONE',  ( 105.7152859519171244, -46.72382961504868604, 52.46901143198183348 ) ) ;
#66316=ADVANCED_FACE ( 'NONE', ( #31004, #51873 ), #86438, .F. ) ;
#66317=CARTESIAN_POINT ( 'NONE',  ( 25.56670390244797275, -58.35344715994099829, 175.9678068554150059 ) ) ;
#66318=ADVANCED_FACE ( 'NONE', ( #24206 ), #30567, .T. ) ;
#66319=CARTESIAN_POINT ( 'NONE',  ( 31.56670390244700641, -19.82844715994111340, -5.074374724088000832 ) ) ;
#66320=VERTEX_POINT ( 'NONE', #36935 ) ;
#66322=ADVANCED_FACE ( 'NONE', ( #65087 ), #2870, .T. ) ;
#66324=ORIENTED_EDGE ( 'NONE', *, *, #2662, .F. ) ;
#66325=ORIENTED_EDGE ( 'NONE', *, *, #68222, .F. ) ;
#66326=CARTESIAN_POINT ( 'NONE',  ( 114.1399574501865999, -31.39144735336052605, 215.7730118773249899 ) ) ;
#66327=CIRCLE ( 'NONE', #85249, 2.517500000000005844 ) ;
#66328=CARTESIAN_POINT ( 'NONE',  ( 40.31648329127400388, 12.92155284005802507, 336.5756252759108520 ) ) ;
#66329=VECTOR ( 'NONE', #65356, 1000.000000000000000 ) ;
#66332=DIRECTION ( 'NONE',  ( -9.073094938289460781E-13, -1.000000000000000000, 0.000000000000000000 ) ) ;
#66334=VERTEX_POINT ( 'NONE', #58267 ) ;
#66335=CARTESIAN_POINT ( 'NONE',  ( 107.0664832912739399, -36.72944715994095333, 293.6356252759109680 ) ) ;
#66337=EDGE_LOOP ( 'NONE', ( #69711, #62067, #85642, #36327 ) ) ;
#66338=CARTESIAN_POINT ( 'NONE',  ( 111.4711666614669099, -26.61707918639087822, 284.7375300378156453 ) ) ;
#66339=DIRECTION ( 'NONE',  ( 0.000000000000000000, 0.000000000000000000, -1.000000000000000000 ) ) ;
#66341=VECTOR ( 'NONE', #74336, 1000.000000000000000 ) ;
#66342=CARTESIAN_POINT ( 'NONE',  ( 116.7951252707350562, -39.38782979291476494, 83.61479194234540557 ) ) ;
#66345=AXIS2_PLACEMENT_3D ( 'NONE', #29595, #78217, #41854 ) ;
#66346=DIRECTION ( 'NONE',  ( -0.1858654557293118459, 0.9825752044329915114, 0.000000000000000000 ) ) ;
#66348=CARTESIAN_POINT ( 'NONE',  ( 117.4559332992660075, -35.18111149946130922, 214.9441967044829767 ) ) ;
#66350=VECTOR ( 'NONE', #33433, 1000.000000000000000 ) ;
#66351=ORIENTED_EDGE ( 'NONE', *, *, #302, .F. ) ;
#66352=CARTESIAN_POINT ( 'NONE',  ( 118.0344259573852810, -38.43289426264998099, 64.69181575210097890 ) ) ;
#66353=CARTESIAN_POINT ( 'NONE',  ( 107.0664832912739399, -48.47944715994096043, 307.1356252759109680 ) ) ;
#66354=ORIENTED_EDGE ( 'NONE', *, *, #19837, .F. ) ;
#66355=ORIENTED_EDGE ( 'NONE', *, *, #47730, .F. ) ;
#66357=DIRECTION ( 'NONE',  ( 4.299999999999999979E-14, -1.000000000000000000, 4.400000000000000367E-29 ) ) ;
#66359=FACE_OUTER_BOUND ( 'NONE', #61809, .T. ) ;
#66360=CARTESIAN_POINT ( 'NONE',  ( 103.5819438468105744, -44.65149928713079674, 130.0528522743539668 ) ) ;
#66361=CARTESIAN_POINT ( 'NONE',  ( 115.8735763837842256, -44.69546008661756531, 229.2413395616249545 ) ) ;
#66363=ORIENTED_EDGE ( 'NONE', *, *, #31977, .T. ) ;
#66364=CIRCLE ( 'NONE', #89609, 5.599999999999994316 ) ;
#66365=CARTESIAN_POINT ( 'NONE',  ( 136.6734006051289612, -37.60624470236170680, 2.902100967938293863 ) ) ;
#66366=ORIENTED_EDGE ( 'NONE', *, *, #35761, .F. ) ;
#66367=AXIS2_PLACEMENT_3D ( 'NONE', #30238, #16607, #2976 ) ;
#66368=VERTEX_POINT ( 'NONE', #58698 ) ;
#66369=LINE ( 'NONE', #39564, #37194 ) ;
#66370=ORIENTED_EDGE ( 'NONE', *, *, #51125, .F. ) ;
#66371=ORIENTED_EDGE ( 'NONE', *, *, #53885, .F. ) ;
#66372=CARTESIAN_POINT ( 'NONE',  ( 101.9943922633895710, -45.44653761360012112, 168.1571991305824270 ) ) ;
#66373=CARTESIAN_POINT ( 'NONE',  ( 156.5667039024485518, -48.82844715993568485, 170.7178068554149775 ) ) ;
#66374=EDGE_CURVE ( 'NONE', #18008, #44647, #72357, .T. ) ;
#66376=CARTESIAN_POINT ( 'NONE',  ( 103.6638222329471262, -28.86385020797125733, 154.8238483995059767 ) ) ;
#66377=CARTESIAN_POINT ( 'NONE',  ( 107.1959452681378053, -26.26092741545045328, 35.06705384733893283 ) ) ;
#66383=EDGE_CURVE ( 'NONE', #33468, #56522, #65961, .T. ) ;
#66385=ORIENTED_EDGE ( 'NONE', *, *, #44504, .T. ) ;
#66386=LINE ( 'NONE', #86856, #46469 ) ;
#66388=DIRECTION ( 'NONE',  ( 4.299999999999999979E-14, -1.000000000000000000, 0.000000000000000000 ) ) ;
#66391=EDGE_LOOP ( 'NONE', ( #64161, #17882, #63780, #9349 ) ) ;
#66393=CARTESIAN_POINT ( 'NONE',  ( 114.8359307259106856, -43.71386199060815869, 38.24419670448192221 ) ) ;
#66394=CARTESIAN_POINT ( 'NONE',  ( 116.4265620360770725, -31.96216903954944399, 40.20133956162496958 ) ) ;
#66396=DIRECTION ( 'NONE',  ( 0.000000000000000000, 0.000000000000000000, 1.000000000000000000 ) ) ;
#66399=CARTESIAN_POINT ( 'NONE',  ( 188.5667039024483245, -42.82844715993430640, 173.2178068554150059 ) ) ;
#66400=LINE ( 'NONE', #40040, #67288 ) ;
#66402=DIRECTION ( 'NONE',  ( 0.000000000000000000, 0.000000000000000000, 1.000000000000000000 ) ) ;
#66403=EDGE_CURVE ( 'NONE', #76842, #611, #16026, .T. ) ;
#66405=DIRECTION ( 'NONE',  ( -0.9963424814100678706, 0.08544974978095865037, 0.000000000000000000 ) ) ;
#66406=CARTESIAN_POINT ( 'NONE',  ( 116.7859321266972330, -32.83856289285826335, 54.12991099019698282 ) ) ;
#66407=CARTESIAN_POINT ( 'NONE',  ( 103.6386224297199163, -26.22117658871400181, 206.3394347997209763 ) ) ;
#66408=CARTESIAN_POINT ( 'NONE',  ( 103.9509101786591287, -47.35857741242491414, 58.33753003781600199 ) ) ;
#66411=DIRECTION ( 'NONE',  ( 1.000000000000000000, 0.000000000000000000, 0.000000000000000000 ) ) ;
#66412=LINE ( 'NONE', #4202, #71747 ) ;
#66413=DIRECTION ( 'NONE',  ( -0.9254794337955623007, -0.3787978585227819162, 0.000000000000000000 ) ) ;
#66414=EDGE_CURVE ( 'NONE', #88572, #74091, #17444, .T. ) ;
#66415=CIRCLE ( 'NONE', #44625, 3.000000000000002665 ) ;
#66417=CARTESIAN_POINT ( 'NONE',  ( 97.07207207479322619, -35.37844108757092698, 187.2189586003667330 ) ) ;
#66419=CARTESIAN_POINT ( 'NONE',  ( 98.99072789581764198, -31.21169308021403310, 116.8499109901959514 ) ) ;
#66422=DIRECTION ( 'NONE',  ( -0.7071067811866279529, 0.7071067811864671926, -7.071067811865978232E-16 ) ) ;
#66423=CARTESIAN_POINT ( 'NONE',  ( 111.5990003564989479, -46.09347164638224825, 243.9356252759109509 ) ) ;
#66425=CARTESIAN_POINT ( 'NONE',  ( 117.0520078648838336, -35.94494220078347269, 148.8889094017758907 ) ) ;
#66429=CARTESIAN_POINT ( 'NONE',  ( 134.0664832912740110, -39.47944715994100306, 1.625625275910997480 ) ) ;
#66431=EDGE_CURVE ( 'NONE', #829, #43897, #17825, .T. ) ;
#66432=CARTESIAN_POINT ( 'NONE',  ( 102.0969121991172557, -45.15362633196983211, 162.1527681330539679 ) ) ;
#66433=VECTOR ( 'NONE', #32833, 1000.000000000000000 ) ;
#66437=CARTESIAN_POINT ( 'NONE',  ( 97.73412737207827661, -37.81740788287748956, 82.86253568684892912 ) ) ;
#66438=CARTESIAN_POINT ( 'NONE',  ( 192.5667039024475002, -23.42844715993433624, 129.9678068554150343 ) ) ;
#66439=CARTESIAN_POINT ( 'NONE',  ( 104.9788083641148972, -27.14010996210895499, 256.2470538473390889 ) ) ;
#66441=CARTESIAN_POINT ( 'NONE',  ( 107.0667039024479834, -36.72944715994099596, 239.5838068554170093 ) ) ;
#66442=CARTESIAN_POINT ( 'NONE',  ( 52.65249034007741358, -48.32844715994062312, 180.4678068554151196 ) ) ;
#66445=DIRECTION ( 'NONE',  ( -1.000000000000000000, -4.299999999999999979E-14, 1.230419385187874527E-43 ) ) ;
#66447=CARTESIAN_POINT ( 'NONE',  ( 101.9951592035502017, -45.85337710724439830, 187.1727681330539781 ) ) ;
#66450=DIRECTION ( 'NONE',  ( 1.000000000000000078E-15, -1.000000000000000000, 0.000000000000000000 ) ) ;
#66451=CARTESIAN_POINT ( 'NONE',  ( 97.07207207582297315, -35.37844108030525092, 152.2189585997880386 ) ) ;
#66452=CARTESIAN_POINT ( 'NONE',  ( 162.5667039024460223, -19.82844715994111340, 342.9256252759109884 ) ) ;
#66454=EDGE_CURVE ( 'NONE', #21457, #24776, #23334, .T. ) ;
#66455=VERTEX_POINT ( 'NONE', #16497 ) ;
#66456=CIRCLE ( 'NONE', #44672, 3.000000000000002665 ) ;
#66457=CARTESIAN_POINT ( 'NONE',  ( 100.8874524663688277, -44.70020958072196748, 268.0522904122051955 ) ) ;
#66458=CARTESIAN_POINT ( 'NONE',  ( 108.8488851759622804, -47.00125683367996032, 167.7127681330539701 ) ) ;
#66459=FACE_OUTER_BOUND ( 'NONE', #16451, .T. ) ;
#66464=CARTESIAN_POINT ( 'NONE',  ( 99.13948424873241549, -42.84779535630594438, 62.85003987030304984 ) ) ;
#66465=CYLINDRICAL_SURFACE ( 'NONE', #84855, 10.00000000000000711 ) ;
#66466=CARTESIAN_POINT ( 'NONE',  ( 117.0606841593708225, -38.08193661114533057, 164.7188404860883395 ) ) ;
#66467=CARTESIAN_POINT ( 'NONE',  ( 111.6835086010359532, -29.99796862204811987, 42.41666179816294857 ) ) ;
#66468=AXIS2_PLACEMENT_3D ( 'NONE', #45637, #87460, #85691 ) ;
#66469=CARTESIAN_POINT ( 'NONE',  ( 80.06648329127402519, -46.72944715994105991, 1.625625275910943746 ) ) ;
#66472=VECTOR ( 'NONE', #15818, 1000.000000000000000 ) ;
#66475=LINE ( 'NONE', #4715, #2422 ) ;
#66476=EDGE_LOOP ( 'NONE', ( #74210, #33310 ) ) ;
#66478=CARTESIAN_POINT ( 'NONE',  ( 116.3212776292278363, -32.94146857470881429, 179.1356252759109395 ) ) ;
#66479=VERTEX_POINT ( 'NONE', #27325 ) ;
#66484=VECTOR ( 'NONE', #46805, 1000.000000000000000 ) ;
#66485=CARTESIAN_POINT ( 'NONE',  ( 102.5950791370611768, -45.34791940167762192, 16.61813411379198158 ) ) ;
#66486=CARTESIAN_POINT ( 'NONE',  ( 104.4481554933880716, -26.61555950438322427, 200.2784824187679362 ) ) ;
#66487=EDGE_CURVE ( 'NONE', #5130, #73456, #68, .T. ) ;
#66488=CARTESIAN_POINT ( 'NONE',  ( 114.3286968523004248, -29.23113535793732254, 174.4641967044819637 ) ) ;
#66489=CARTESIAN_POINT ( 'NONE',  ( 97.93091671000914289, -40.79819621030469534, 21.65960399723592289 ) ) ;
#66490=CARTESIAN_POINT ( 'NONE',  ( 112.4893506266177070, -46.36098340020668473, 253.9965776568634510 ) ) ;
#66491=DIRECTION ( 'NONE',  ( -4.299999999999999979E-14, 1.000000000000000000, -4.400000000000000367E-29 ) ) ;
#66492=DIRECTION ( 'NONE',  ( 1.000000000000000078E-15, -1.000000000000000083E-30, -1.000000000000000000 ) ) ;
#66493=ORIENTED_EDGE ( 'NONE', *, *, #47200, .T. ) ;
#66495=VERTEX_POINT ( 'NONE', #33696 ) ;
#66496=AXIS2_PLACEMENT_3D ( 'NONE', #66799, #32271, #59965 ) ;
#66499=CARTESIAN_POINT ( 'NONE',  ( 97.82529773858178146, -40.55052980792035555, 111.6384738132450991 ) ) ;
#66500=CARTESIAN_POINT ( 'NONE',  ( 96.47340144944560336, -31.30584922022854144, 245.9499109901969689 ) ) ;
#66501=ORIENTED_EDGE ( 'NONE', *, *, #38096, .F. ) ;
#66502=CARTESIAN_POINT ( 'NONE',  ( 97.40186843559010299, -40.63869902605510731, 206.6327681330539860 ) ) ;
#66503=CARTESIAN_POINT ( 'NONE',  ( 105.7984081882492120, -26.72418595412763764, 265.1773184473723290 ) ) ;
#66507=CARTESIAN_POINT ( 'NONE',  ( 97.81281252356875200, -40.52015776331121089, 277.6356251289804504 ) ) ;
#66509=CARTESIAN_POINT ( 'NONE',  ( 97.23737678141888807, -33.32131919061086478, 282.0613395616252888 ) ) ;
#66510=CARTESIAN_POINT ( 'NONE',  ( 83.06670390244796920, -61.87844715994100397, 231.5838068554150198 ) ) ;
#66512=EDGE_CURVE ( 'NONE', #38542, #89690, #39162, .T. ) ;
#66513=CARTESIAN_POINT ( 'NONE',  ( 62.03715912545731470, -23.42818131006022142, 249.9678068554150343 ) ) ;
#66516=DIRECTION ( 'NONE',  ( 0.000000000000000000, 1.000000000000000000, 0.000000000000000000 ) ) ;
#66517=ADVANCED_FACE ( 'NONE', ( #4646 ), #40944, .T. ) ;
#66518=DIRECTION ( 'NONE',  ( 0.7071067811862279395, -0.7071067811868672059, 7.071067811862286363E-16 ) ) ;
#66520=VECTOR ( 'NONE', #84754, 1000.000000000000000 ) ;
#66521=CARTESIAN_POINT ( 'NONE',  ( 136.4975570085109382, -20.01506174167543506, 7.157201688892354419 ) ) ;
#66522=CARTESIAN_POINT ( 'NONE',  ( 98.36125384756333290, -29.88003685912757490, 200.8080062282919869 ) ) ;
#66523=CARTESIAN_POINT ( 'NONE',  ( 99.68461964852595258, -45.99997598619422234, 118.0413395616259606 ) ) ;
#66524=CARTESIAN_POINT ( 'NONE',  ( 96.81585423491817721, -34.60398634006848795, 212.1641967044819808 ) ) ;
#66526=DIRECTION ( 'NONE',  ( 0.000000000000000000, 0.000000000000000000, -1.000000000000000000 ) ) ;
#66527=CARTESIAN_POINT ( 'NONE',  ( 131.0667039024480118, -58.35344715994099829, 231.5838068554150198 ) ) ;
#66529=CYLINDRICAL_SURFACE ( 'NONE', #79882, 9.999999999999998224 ) ;
#66531=DIRECTION ( 'NONE',  ( -0.8571673007021110013, 1.917331853055865018E-16, 0.5150380749100563760 ) ) ;
#66533=VECTOR ( 'NONE', #70963, 1000.000000000000000 ) ;
#66536=CARTESIAN_POINT ( 'NONE',  ( 110.3568814055478242, -27.59468345507334064, 99.22384839950498758 ) ) ;
#66538=CARTESIAN_POINT ( 'NONE',  ( 163.5667039024460223, -22.48495420874110806, -5.074374724088000832 ) ) ;
#66540=CARTESIAN_POINT ( 'NONE',  ( 96.69266148864274157, -35.94780844399463149, 142.2670538473399517 ) ) ;
#66541=LINE ( 'NONE', #75153, #46819 ) ;
#66542=CARTESIAN_POINT ( 'NONE',  ( 79.11888855178470692, -16.14703303315388183, 8.087249882925839017 ) ) ;
#66543=CARTESIAN_POINT ( 'NONE',  ( 51.24204729617298426, -31.76306994223730840, -5.074374724088000832 ) ) ;
#66544=DIRECTION ( 'NONE',  ( 1.000000000000000000, 8.163404592831600092E-16, 1.020425574103949962E-15 ) ) ;
#66545=AXIS2_PLACEMENT_3D ( 'NONE', #30776, #86197, #38470 ) ;
#66546=EDGE_CURVE ( 'NONE', #74639, #6566, #60032, .T. ) ;
#66547=CARTESIAN_POINT ( 'NONE',  ( 99.23822674327645643, -42.59304969680529496, 66.83848241876894747 ) ) ;
#66549=ORIENTED_EDGE ( 'NONE', *, *, #57640, .T. ) ;
#66552=CARTESIAN_POINT ( 'NONE',  ( 109.3575602964533289, -46.23809593081413993, 128.7641967044819751 ) ) ;
#66553=CARTESIAN_POINT ( 'NONE',  ( 162.5667039024470171, -33.35206098992711077, -5.074374724088000832 ) ) ;
#66557=FACE_OUTER_BOUND ( 'NONE', #21851, .T. ) ;
#66559=CARTESIAN_POINT ( 'NONE',  ( 115.7828637914807786, -41.80272134509917947, 179.4064208818603561 ) ) ;
#66560=CARTESIAN_POINT ( 'NONE',  ( 98.73996931189270754, -42.96625968561445319, 66.83848241876793850 ) ) ;
#66561=ORIENTED_EDGE ( 'NONE', *, *, #59729, .F. ) ;
#66563=EDGE_CURVE ( 'NONE', #68206, #73498, #29278, .T. ) ;
#66564=CARTESIAN_POINT ( 'NONE',  ( 63.03715912545640521, -24.89890238295017255, 180.4678068554151196 ) ) ;
#66567=CARTESIAN_POINT ( 'NONE',  ( 98.06451646660192978, -38.97900810122609982, 164.3395189410199464 ) ) ;
#66571=ORIENTED_EDGE ( 'NONE', *, *, #76437, .F. ) ;
#66572=ORIENTED_EDGE ( 'NONE', *, *, #59885, .F. ) ;
#66573=DIRECTION ( 'NONE',  ( 0.1811243268507098381, -0.9834602067307437467, 0.000000000000000000 ) ) ;
#66575=ORIENTED_EDGE ( 'NONE', *, *, #72271, .T. ) ;
#66577=CARTESIAN_POINT ( 'NONE',  ( 100.1238157808075186, -30.39889478464921524, 227.1577737820879577 ) ) ;
#66578=VECTOR ( 'NONE', #13245, 1000.000000000000000 ) ;
#66580=CARTESIAN_POINT ( 'NONE',  ( 177.3246001664174969, -48.34074026909178912, 180.4678068554150059 ) ) ;
#66581=DIRECTION ( 'NONE',  ( 0.000000000000000000, 0.000000000000000000, 1.000000000000000000 ) ) ;
#66582=ORIENTED_EDGE ( 'NONE', *, *, #86621, .F. ) ;
#66583=VECTOR ( 'NONE', #53372, 1000.000000000000000 ) ;
#66584=ORIENTED_EDGE ( 'NONE', *, *, #57709, .T. ) ;
#66586=VERTEX_POINT ( 'NONE', #13696 ) ;
#66587=ADVANCED_FACE ( 'NONE', ( #62738 ), #8694, .T. ) ;
#66588=CARTESIAN_POINT ( 'NONE',  ( 109.4041143893713297, -28.39659615353044231, 217.6890427505439902 ) ) ;
#66589=AXIS2_PLACEMENT_3D ( 'NONE', #83596, #62235, #48585 ) ;
#66590=CARTESIAN_POINT ( 'NONE',  ( 102.9623509218069302, -46.33686416246144546, 92.25562527591097250 ) ) ;
#66592=CARTESIAN_POINT ( 'NONE',  ( 103.8480726019013218, -46.65951555449696997, 82.32705384733995402 ) ) ;
#66594=CARTESIAN_POINT ( 'NONE',  ( 154.4439038579832300, -17.91479848270203945, 396.9756252759102040 ) ) ;
#66597=CARTESIAN_POINT ( 'NONE',  ( 95.31164914186729220, -38.27921806354234491, 147.4299109901969871 ) ) ;
#66601=EDGE_LOOP ( 'NONE', ( #82550, #17009 ) ) ;
#66604=AXIS2_PLACEMENT_3D ( 'NONE', #72893, #44726, #73331 ) ;
#66605=DIRECTION ( 'NONE',  ( 1.000000000000000000, 4.299999999999999979E-14, 1.000000000000000078E-15 ) ) ;
#66606=FACE_OUTER_BOUND ( 'NONE', #72380, .T. ) ;
#66609=EDGE_CURVE ( 'NONE', #52361, #65845, #14606, .T. ) ;
#66610=ORIENTED_EDGE ( 'NONE', *, *, #7142, .F. ) ;
#66612=CARTESIAN_POINT ( 'NONE',  ( 103.9573432206533283, -47.33663036165624050, 62.33753003781600199 ) ) ;
#66613=DIRECTION ( 'NONE',  ( -0.000000000000000000, -0.000000000000000000, 1.000000000000000000 ) ) ;
#66614=LINE ( 'NONE', #73881, #76816 ) ;
#66616=CARTESIAN_POINT ( 'NONE',  ( 116.0809032858471852, -32.84949784884745583, 79.14991099019697174 ) ) ;
#66617=CARTESIAN_POINT ( 'NONE',  ( 25.56670390244797275, -62.87844715994099687, 137.2178068554150059 ) ) ;
#66618=CARTESIAN_POINT ( 'NONE',  ( 102.8528367378537922, -46.24122135049434235, 173.2441967044829596 ) ) ;
#66619=CARTESIAN_POINT ( 'NONE',  ( 182.5667039024459939, -22.48495420874030515, -5.074374724088000832 ) ) ;
#66620=VECTOR ( 'NONE', #67382, 1000.000000000000000 ) ;
#66622=EDGE_CURVE ( 'NONE', #16372, #10976, #76822, .T. ) ;
#66624=AXIS2_PLACEMENT_3D ( 'NONE', #75340, #76227, #12667 ) ;
#66626=DIRECTION ( 'NONE',  ( 0.000000000000000000, 0.000000000000000000, 1.000000000000000000 ) ) ;
#66628=CARTESIAN_POINT ( 'NONE',  ( 97.81169607051373305, -40.51742273377266912, 46.63562653399714009 ) ) ;
#66629=CARTESIAN_POINT ( 'NONE',  ( 113.0474237710022578, -45.36542684395109148, 203.0584824187679374 ) ) ;
#66632=CARTESIAN_POINT ( 'NONE',  ( 105.1049547281328671, -25.82818065531082041, 271.2061014663873380 ) ) ;
#66633=CARTESIAN_POINT ( 'NONE',  ( 113.8717716195138792, -28.72781827743602889, 135.5156252759109634 ) ) ;
#66637=DIRECTION ( 'NONE',  ( 1.000000000000000078E-15, -1.000000000000000083E-30, -1.000000000000000000 ) ) ;
#66639=EDGE_LOOP ( 'NONE', ( #58957, #16745, #36760, #77920 ) ) ;
#66641=ORIENTED_EDGE ( 'NONE', *, *, #46853, .F. ) ;
#66642=ORIENTED_EDGE ( 'NONE', *, *, #75547, .F. ) ;
#66643=AXIS2_PLACEMENT_3D ( 'NONE', #87461, #52881, #58840 ) ;
#66644=ORIENTED_EDGE ( 'NONE', *, *, #33409, .F. ) ;
#66645=CARTESIAN_POINT ( 'NONE',  ( 25.56670390244805091, -42.82844715994167473, 293.2178068554150059 ) ) ;
#66646=CARTESIAN_POINT ( 'NONE',  ( 98.44183741489698036, -42.05700530801248505, 7.768006228291934434 ) ) ;
#66647=CARTESIAN_POINT ( 'NONE',  ( 37.35959712133899302, -48.62134037883190985, 300.4678068554150059 ) ) ;
#66649=VECTOR ( 'NONE', #64972, 1000.000000000000000 ) ;
#66653=CARTESIAN_POINT ( 'NONE',  ( 106.5889295881363950, -27.03189230550456656, 194.5381341137909601 ) ) ;
#66655=VERTEX_POINT ( 'NONE', #55898 ) ;
#66657=VECTOR ( 'NONE', #19228, 1000.000000000000000 ) ;
#66658=ORIENTED_EDGE ( 'NONE', *, *, #81841, .F. ) ;
#66659=LINE ( 'NONE', #17630, #54328 ) ;
#66662=CARTESIAN_POINT ( 'NONE',  ( 33.78129701732998313, -35.65087443492610930, -5.074374724088000832 ) ) ;
#66663=CARTESIAN_POINT ( 'NONE',  ( 114.3823783366371316, -42.62471689273790076, 39.70634521065896649 ) ) ;
#66665=AXIS2_PLACEMENT_3D ( 'NONE', #57883, #65144, #63357 ) ;
#66666=CARTESIAN_POINT ( 'NONE',  ( 49.35211078756498893, -35.65087443492551245, -5.074374724088000832 ) ) ;
#66668=CARTESIAN_POINT ( 'NONE',  ( 112.1213531720970309, -45.14146623880455422, 238.0070538473399324 ) ) ;
#66669=LINE ( 'NONE', #46203, #5141 ) ;
#66670=VERTEX_POINT ( 'NONE', #69117 ) ;
#66671=CARTESIAN_POINT ( 'NONE',  ( 103.3201801717304136, -27.45767654545007375, 56.38204572563600436 ) ) ;
#66673=FACE_OUTER_BOUND ( 'NONE', #88058, .T. ) ;
#66674=CARTESIAN_POINT ( 'NONE',  ( 101.8554017947406862, -30.44658510084856218, 38.44523322673398980 ) ) ;
#66675=EDGE_CURVE ( 'NONE', #48555, #38912, #18933, .T. ) ;
#66676=AXIS2_PLACEMENT_3D ( 'NONE', #23349, #8818, #23785 ) ;
#66677=CARTESIAN_POINT ( 'NONE',  ( 136.5887892044422642, -17.63370978841804870, 7.053538376718607950 ) ) ;
#66678=DIRECTION ( 'NONE',  ( 1.000000000000000000, 6.055337108828351666E-16, 0.000000000000000000 ) ) ;
#66681=ORIENTED_EDGE ( 'NONE', *, *, #79153, .F. ) ;
#66684=EDGE_LOOP ( 'NONE', ( #21582, #19211 ) ) ;
#66685=CARTESIAN_POINT ( 'NONE',  ( 95.77883191840808763, -40.33907488607122360, 131.5727681330539554 ) ) ;
#66686=ORIENTED_EDGE ( 'NONE', *, *, #45855, .T. ) ;
#66687=CARTESIAN_POINT ( 'NONE',  ( 115.5717340297064197, -37.51483979961712123, 78.17527697093396455 ) ) ;
#66688=ORIENTED_CLOSED_SHELL ( 'NONE', *, #76417, .F. );
#66689=CARTESIAN_POINT ( 'NONE',  ( 151.0371591254575776, -24.42818131005592264, 129.9678068554149775 ) ) ;
#66690=CARTESIAN_POINT ( 'NONE',  ( 115.8107094469502272, -38.34209669562990541, 85.11301187732594542 ) ) ;
#66693=AXIS2_PLACEMENT_3D ( 'NONE', #11498, #39193, #40980 ) ;
#66694=CARTESIAN_POINT ( 'NONE',  ( 96.81221355789537597, -38.90410760351644370, 27.49276813305395706 ) ) ;
#66696=ORIENTED_EDGE ( 'NONE', *, *, #81519, .T. ) ;
#66697=CARTESIAN_POINT ( 'NONE',  ( 177.8371591254545478, -47.82818131005477369, 129.9678068554150059 ) ) ;
#66698=ORIENTED_EDGE ( 'NONE', *, *, #85850, .T. ) ;
#66700=EDGE_LOOP ( 'NONE', ( #33147, #2751 ) ) ;
#66701=EDGE_LOOP ( 'NONE', ( #31853, #54569, #10958, #15415 ) ) ;
#66702=EDGE_CURVE ( 'NONE', #49269, #28852, #64100, .T. ) ;
#66706=CARTESIAN_POINT ( 'NONE',  ( 96.93540839703290146, -34.51582869190840341, 256.1432443235307232 ) ) ;
#66707=DIRECTION ( 'NONE',  ( 0.000000000000000000, 0.000000000000000000, -1.000000000000000000 ) ) ;
#66708=CARTESIAN_POINT ( 'NONE',  ( 115.7831076508929300, -41.80230954465056215, 189.4064586061371358 ) ) ;
#66709=EDGE_CURVE ( 'NONE', #58383, #26947, #1572, .T. ) ;
#66710=CARTESIAN_POINT ( 'NONE',  ( 104.0427601340384030, -47.36105469373795529, 63.36800622829197494 ) ) ;
#66711=CARTESIAN_POINT ( 'NONE',  ( 117.0719050840518065, -35.46253235289662342, 44.92728796927281110 ) ) ;
#66712=ORIENTED_EDGE ( 'NONE', *, *, #38419, .T. ) ;
#66713=CARTESIAN_POINT ( 'NONE',  ( 113.2456828512594598, -28.75880519094399546, 114.5535222254891750 ) ) ;
#66714=AXIS2_PLACEMENT_3D ( 'NONE', #87878, #32901, #82425 ) ;
#66715=ADVANCED_FACE ( 'NONE', ( #49542 ), #75925, .F. ) ;
#66717=VERTEX_POINT ( 'NONE', #29568 ) ;
#66718=VECTOR ( 'NONE', #8993, 1000.000000000000000 ) ;
#66719=CARTESIAN_POINT ( 'NONE',  ( 46.03715912545343514, -48.62818131006090283, 180.4678068554150911 ) ) ;
#66720=CARTESIAN_POINT ( 'NONE',  ( 100.8868559669706713, -44.69971346806422474, 113.0528871607769332 ) ) ;
#66721=CARTESIAN_POINT ( 'NONE',  ( 97.03753386688401861, -33.96379371595038776, 251.1127681330538337 ) ) ;
#66723=CARTESIAN_POINT ( 'NONE',  ( 72.06648329127396835, -9.729447159941065237, 14.67562527591093513 ) ) ;
#66724=CARTESIAN_POINT ( 'NONE',  ( 78.22143491579828378, -38.77077206071901117, 2.188418444519958150 ) ) ;
#66725=CARTESIAN_POINT ( 'NONE',  ( 102.3370036867683268, -28.24990410829322940, 254.9038483995052502 ) ) ;
#66727=CARTESIAN_POINT ( 'NONE',  ( 98.60777729073579678, -43.80857954853289016, 67.86895860924497015 ) ) ;
#66729=CARTESIAN_POINT ( 'NONE',  ( 113.1024245609201984, -28.17526227570857955, 129.5870538473399449 ) ) ;
#66731=CARTESIAN_POINT ( 'NONE',  ( 132.6453213455548337, -21.08531275930677040, 7.905164235256782135 ) ) ;
#66733=VERTEX_POINT ( 'NONE', #77730 ) ;
#66734=VECTOR ( 'NONE', #75086, 1000.000000000000000 ) ;
#66735=PLANE ( 'NONE',  #6172 ) ;
#66737=EDGE_CURVE ( 'NONE', #19244, #34907, #6879, .T. ) ;
#66740=CARTESIAN_POINT ( 'NONE',  ( 98.34969834581170289, -31.65685598046560045, 50.90648325210623426 ) ) ;
#66741=CARTESIAN_POINT ( 'NONE',  ( 116.9635770353169733, -33.20817898692279613, 114.0984824187679720 ) ) ;
#66742=ORIENTED_EDGE ( 'NONE', *, *, #5734, .F. ) ;
#66743=LINE ( 'NONE', #10447, #55230 ) ;
#66748=CARTESIAN_POINT ( 'NONE',  ( 114.7424063621565722, -43.81651770963347303, 123.2327681330539519 ) ) ;
#66750=DIRECTION ( 'NONE',  ( 0.000000000000000000, 0.000000000000000000, 1.000000000000000000 ) ) ;
#66752=ORIENTED_EDGE ( 'NONE', *, *, #50230, .T. ) ;
#66753=AXIS2_PLACEMENT_3D ( 'NONE', #4740, #53299, #87858 ) ;
#66755=FACE_OUTER_BOUND ( 'NONE', #86137, .T. ) ;
#66756=CARTESIAN_POINT ( 'NONE',  ( 107.0664832912739399, -36.72944715994095333, 357.5272416190308604 ) ) ;
#66757=CARTESIAN_POINT ( 'NONE',  ( 109.6430120585716281, -46.48008675498888209, 157.7814586033456692 ) ) ;
#66759=CARTESIAN_POINT ( 'NONE',  ( 113.2452453786383728, -28.75847917007356003, 104.5523170862238800 ) ) ;
#66761=PLANE ( 'NONE',  #89266 ) ;
#66762=VECTOR ( 'NONE', #25456, 1000.000000000000000 ) ;
#66765=EDGE_CURVE ( 'NONE', #73152, #85115, #16837, .T. ) ;
#66766=CARTESIAN_POINT ( 'NONE',  ( 110.4719531740380063, -47.31314961125941210, 203.8241967044819489 ) ) ;
#66767=DIRECTION ( 'NONE',  ( 0.000000000000000000, 1.000000000000000000, 0.000000000000000000 ) ) ;
#66768=ORIENTED_EDGE ( 'NONE', *, *, #85011, .F. ) ;
#66770=CARTESIAN_POINT ( 'NONE',  ( 101.5079035968564654, -28.64143341885332816, 46.55562527591094835 ) ) ;
#66771=CARTESIAN_POINT ( 'NONE',  ( 116.9902980441214595, -35.35395306989185116, 53.93600868140660509 ) ) ;
#66773=CARTESIAN_POINT ( 'NONE',  ( 162.7866693523297954, -29.62846900981741527, 117.4678068554150485 ) ) ;
#66775=ORIENTED_EDGE ( 'NONE', *, *, #62484, .T. ) ;
#66778=ORIENTED_EDGE ( 'NONE', *, *, #89274, .F. ) ;
#66779=CARTESIAN_POINT ( 'NONE',  ( 116.3948728625927060, -35.60798670905003860, 235.3653928297059679 ) ) ;
#66780=CIRCLE ( 'NONE', #58098, 2.517500000000005844 ) ;
#66782=EDGE_CURVE ( 'NONE', #62285, #9081, #21870, .T. ) ;
#66785=AXIS2_PLACEMENT_3D ( 'NONE', #60440, #88185, #25940 ) ;
#66786=CARTESIAN_POINT ( 'NONE',  ( 82.64938057483485068, -37.67376371870361851, 2.871651383883024433 ) ) ;
#66787=ORIENTED_EDGE ( 'NONE', *, *, #32770, .T. ) ;
#66789=DIRECTION ( 'NONE',  ( 4.299999999999999979E-14, -1.000000000000000000, 0.000000000000000000 ) ) ;
#66791=CARTESIAN_POINT ( 'NONE',  ( 111.7637953458032172, -46.71243375810367837, 287.9146728949587555 ) ) ;
#66792=ORIENTED_EDGE ( 'NONE', *, *, #73679, .T. ) ;
#66794=CARTESIAN_POINT ( 'NONE',  ( 101.6725443455464131, -43.49748584897681525, 269.8471379886391901 ) ) ;
#66795=EDGE_CURVE ( 'NONE', #65852, #24816, #71211, .T. ) ;
#66796=EDGE_CURVE ( 'NONE', #23298, #85840, #16396, .T. ) ;
#66799=CARTESIAN_POINT ( 'NONE',  ( 184.5667039024480118, -48.82844715994099971, 300.9178068554150514 ) ) ;
#66801=CARTESIAN_POINT ( 'NONE',  ( 98.39890672360048995, -29.79614961819730468, 191.7775300378159784 ) ) ;
#66804=CARTESIAN_POINT ( 'NONE',  ( 101.0411209824609813, -27.40783209567417700, 66.54514908543495721 ) ) ;
#66807=VERTEX_POINT ( 'NONE', #78642 ) ;
#66808=ORIENTED_EDGE ( 'NONE', *, *, #42935, .F. ) ;
#66809=VERTEX_POINT ( 'NONE', #17729 ) ;
#66811=AXIS2_PLACEMENT_3D ( 'NONE', #15159, #21535, #42835 ) ;
#66815=ADVANCED_FACE ( 'NONE', ( #45404 ), #57714, .T. ) ;
#66816=CARTESIAN_POINT ( 'NONE',  ( 101.2865843167392654, -43.98814532200950822, 119.8595189410199566 ) ) ;
#66817=CARTESIAN_POINT ( 'NONE',  ( 96.49610902845032001, -31.31747537214017640, 241.9499109901969689 ) ) ;
#66818=DIRECTION ( 'NONE',  ( 0.7071067809773464719, -0.7071067813957485626, 7.071067809773472419E-16 ) ) ;
#66819=EDGE_LOOP ( 'NONE', ( #39172, #1128, #2191, #5159 ) ) ;
#66823=ORIENTED_EDGE ( 'NONE', *, *, #485, .T. ) ;
#66824=ORIENTED_EDGE ( 'NONE', *, *, #29455, .T. ) ;
#66827=ORIENTED_EDGE ( 'NONE', *, *, #18411, .T. ) ;
#66829=LINE ( 'NONE', #65929, #34150 ) ;
#66831=CARTESIAN_POINT ( 'NONE',  ( 115.2191710476659665, -34.18193581181276386, 173.4895626852199371 ) ) ;
#66832=CARTESIAN_POINT ( 'NONE',  ( 117.4283214861109457, -38.22576773620406954, 28.71276813305395592 ) ) ;
#66834=ADVANCED_FACE ( 'NONE', ( #65429 ), #10899, .T. ) ;
#66835=EDGE_LOOP ( 'NONE', ( #5056, #4465, #35968, #48774 ) ) ;
#66836=EDGE_CURVE ( 'NONE', #80800, #43956, #29125, .T. ) ;
#66838=VECTOR ( 'NONE', #12952, 1000.000000000000000 ) ;
#66841=CIRCLE ( 'NONE', #81400, 0.9999999999999940048 ) ;
#66843=ORIENTED_EDGE ( 'NONE', *, *, #53549, .F. ) ;
#66844=CARTESIAN_POINT ( 'NONE',  ( 98.32086286370073935, -31.82106486744336493, 166.9192892379911655 ) ) ;
#66845=ADVANCED_FACE ( 'NONE', ( #71803 ), #9576, .F. ) ;
#66846=CARTESIAN_POINT ( 'NONE',  ( 101.9931413102871005, -45.44577570166600822, 32.15663476389070752 ) ) ;
#66847=DIRECTION ( 'NONE',  ( 0.000000000000000000, 0.000000000000000000, 1.000000000000000000 ) ) ;
#66849=PLANE ( 'NONE',  #71263 ) ;
#66851=CARTESIAN_POINT ( 'NONE',  ( 115.9640307963821186, -42.20482783266999149, 18.38705384733896153 ) ) ;
#66852=CARTESIAN_POINT ( 'NONE',  ( 101.9391980234526187, -27.60234874203171884, 56.48419670448296159 ) ) ;
#66856=CARTESIAN_POINT ( 'NONE',  ( 108.4175026908246622, -26.73503768359202937, 145.9693458669439110 ) ) ;
#66857=FACE_BOUND ( 'NONE', #70400, .T. ) ;
#66858=VECTOR ( 'NONE', #81710, 1000.000000000000000 ) ;
#66859=LINE ( 'NONE', #16935, #41553 ) ;
#66862=ORIENTED_EDGE ( 'NONE', *, *, #27986, .F. ) ;
#66863=CARTESIAN_POINT ( 'NONE',  ( 116.4271464750313498, -31.96187137292554681, 44.20133956162491984 ) ) ;
#66864=CARTESIAN_POINT ( 'NONE',  ( 104.1858290503737408, -26.67344577167302688, 221.2984824187679465 ) ) ;
#66865=CARTESIAN_POINT ( 'NONE',  ( 107.6079817216441796, -48.59237387041279987, 38.61276813305397582 ) ) ;
#66866=DIRECTION ( 'NONE',  ( -0.7071067811865274777, 0.7071067811865675568, -7.071067811864971448E-16 ) ) ;
#66867=DIRECTION ( 'NONE',  ( 0.000000000000000000, 0.000000000000000000, 1.000000000000000000 ) ) ;
#66869=VERTEX_POINT ( 'NONE', #85894 ) ;
#66871=ORIENTED_EDGE ( 'NONE', *, *, #23977, .T. ) ;
#66872=CARTESIAN_POINT ( 'NONE',  ( 114.6661721138974315, -42.88640786233941782, 84.28419670448195689 ) ) ;
#66874=VERTEX_POINT ( 'NONE', #85456 ) ;
#66875=AXIS2_PLACEMENT_3D ( 'NONE', #71372, #79525, #10901 ) ;
#66876=CARTESIAN_POINT ( 'NONE',  ( 101.6619702986603073, -45.61876124157276280, 243.1413395616249886 ) ) ;
#66878=CARTESIAN_POINT ( 'NONE',  ( 29.56648329127298069, -71.37844715994266664, 342.9256252759109884 ) ) ;
#66879=LINE ( 'NONE', #10142, #8061 ) ;
#66880=CARTESIAN_POINT ( 'NONE',  ( 177.0371591254543375, -48.62818131005480637, 300.4678068554149490 ) ) ;
#66881=DIRECTION ( 'NONE',  ( 0.000000000000000000, 0.000000000000000000, -1.000000000000000000 ) ) ;
#66883=CARTESIAN_POINT ( 'NONE',  ( 116.8431970675092515, -40.18699730018606431, 178.5680062282919778 ) ) ;
#66884=ORIENTED_EDGE ( 'NONE', *, *, #85507, .F. ) ;
#66886=ORIENTED_EDGE ( 'NONE', *, *, #809, .F. ) ;
#66887=CARTESIAN_POINT ( 'NONE',  ( 108.0951925567892431, -27.89746624773302841, 126.4158690201829813 ) ) ;
#66888=AXIS2_PLACEMENT_3D ( 'NONE', #8290, #86381, #71860 ) ;
#66889=PLANE ( 'NONE',  #83471 ) ;
#66891=CARTESIAN_POINT ( 'NONE',  ( 115.2378349030890092, -31.35427756934441845, 250.2899109901960344 ) ) ;
#66892=DIRECTION ( 'NONE',  ( 0.000000000000000000, 1.000000000000000000, 0.000000000000000000 ) ) ;
#66893=DIRECTION ( 'NONE',  ( 4.299999999999999979E-14, -1.000000000000000000, 0.000000000000000000 ) ) ;
#66894=DIRECTION ( 'NONE',  ( 2.775557561562888827E-14, -1.000000000000000000, 0.000000000000000000 ) ) ;
#66895=EDGE_CURVE ( 'NONE', #84235, #5137, #64983, .T. ) ;
#66896=CARTESIAN_POINT ( 'NONE',  ( 19.56648329127400032, 12.92155284005902516, 333.4006252759108975 ) ) ;
#66902=CARTESIAN_POINT ( 'NONE',  ( 113.1426608820138426, -26.58408993604425419, 204.6470538473399756 ) ) ;
#66904=ORIENTED_EDGE ( 'NONE', *, *, #38192, .F. ) ;
#66905=EDGE_CURVE ( 'NONE', #79856, #36953, #24545, .T. ) ;
#66907=EDGE_CURVE ( 'NONE', #8413, #74068, #84253, .T. ) ;
#66909=CARTESIAN_POINT ( 'NONE',  ( 80.06648329127399677, -15.97944715994105813, 1.625625275910943746 ) ) ;
#66911=CARTESIAN_POINT ( 'NONE',  ( 138.8167039024479834, -57.40094715994099772, 60.91780685541480267 ) ) ;
#66913=ADVANCED_FACE ( 'NONE', ( #30023 ), #82208, .F. ) ;
#66915=VERTEX_POINT ( 'NONE', #25424 ) ;
#66918=CARTESIAN_POINT ( 'NONE',  ( 117.1973380236488111, -34.26920065746595867, 209.0156252759109634 ) ) ;
#66919=CARTESIAN_POINT ( 'NONE',  ( 172.5664832912740110, -9.303447159940999356, 138.9256252759119832 ) ) ;
#66922=CIRCLE ( 'NONE', #27766, 3.299999999999997158 ) ;
#66923=CARTESIAN_POINT ( 'NONE',  ( 98.09052178646700781, -41.13971508595705728, 62.69037633451134184 ) ) ;
#66924=DIRECTION ( 'NONE',  ( 0.000000000000000000, 0.000000000000000000, 1.000000000000000000 ) ) ;
#66925=B_SPLINE_CURVE_WITH_KNOTS ( 'NONE', 3,
 ( #34745, #66231, #87153, #19779, #48800, #62452, #27043, #74743, #19335, #75195, #76535, #226, #40663, #82480, #61998, #12521, #40205, #55606, #38536, #31723, #24919, #53816, #81583, #67925, #20234, #12975, #5712, #68384, #47906, #6161 ),
 .UNSPECIFIED., .F., .F.,
 ( 4, 2, 2, 2, 1, 2, 2, 2, 2, 2, 2, 2, 1, 2, 2, 4 ),
 ( 0.5000000000000000000, 0.5624999999999806821, 0.5937499999999708011, 0.6093749999999663602, 0.6171874999999658051, 0.6210937499999669154, 0.6249999999999680256, 0.6874999999999692468, 0.7187499999999715783, 0.7499999999999740208, 0.8124999999999727995, 0.8437499999999724665, 0.8593749999999686917, 0.8671874999999705791, 0.8749999999999724665, 1.000000000000000000 ),
 .UNSPECIFIED. ) ;
#66926=CARTESIAN_POINT ( 'NONE',  ( 97.92338036926128098, -40.78103718271854916, 166.6584133301706458 ) ) ;
#66928=EDGE_CURVE ( 'NONE', #65246, #29858, #4987, .T. ) ;
#66929=CARTESIAN_POINT ( 'NONE',  ( 107.1674220045319288, -28.56736792770730560, 32.88523322673398042 ) ) ;
#66931=ORIENTED_EDGE ( 'NONE', *, *, #23337, .T. ) ;
#66933=CARTESIAN_POINT ( 'NONE',  ( 81.91948822002333941, -16.69035895458603846, 7.660272404653420963 ) ) ;
#66937=ORIENTED_EDGE ( 'NONE', *, *, #24154, .T. ) ;
#66939=DIRECTION ( 'NONE',  ( 0.000000000000000000, 0.000000000000000000, -1.000000000000000000 ) ) ;
#66940=CARTESIAN_POINT ( 'NONE',  ( 111.7162562550164608, -28.95820004563618610, 54.08194363760093637 ) ) ;
#66941=CARTESIAN_POINT ( 'NONE',  ( 117.4357963365922615, -35.45519799489562729, 193.9241967044829664 ) ) ;
#66942=AXIS2_PLACEMENT_3D ( 'NONE', #51320, #85885, #17278 ) ;
#66943=CARTESIAN_POINT ( 'NONE',  ( 113.6008039948045933, -28.63430547549723570, 164.5356252759109736 ) ) ;
#66944=CARTESIAN_POINT ( 'NONE',  ( 31.71315051186898870, -31.94127993907790852, 237.4678068554150059 ) ) ;
#66945=CARTESIAN_POINT ( 'NONE',  ( 111.7736368399375522, -46.73334422087322082, 283.9146728949585849 ) ) ;
#66946=DIRECTION ( 'NONE',  ( 0.000000000000000000, 0.000000000000000000, 1.000000000000000000 ) ) ;
#66948=VERTEX_POINT ( 'NONE', #80861 ) ;
#66949=EDGE_CURVE ( 'NONE', #16246, #38148, #8693, .T. ) ;
#66950=ORIENTED_EDGE ( 'NONE', *, *, #37105, .T. ) ;
#66951=EDGE_CURVE ( 'NONE', #75328, #26178, #74028, .T. ) ;
#66953=VECTOR ( 'NONE', #48924, 1000.000000000000000 ) ;
#66954=CARTESIAN_POINT ( 'NONE',  ( 123.6837132603318707, -17.59493780205716362, 219.5838068554170093 ) ) ;
#66955=CARTESIAN_POINT ( 'NONE',  ( 112.2268274879326668, -45.83864656583022423, 212.9870538473389558 ) ) ;
#66956=ORIENTED_EDGE ( 'NONE', *, *, #83207, .F. ) ;
#66957=CARTESIAN_POINT ( 'NONE',  ( 108.6750451637706618, -26.42898313331718541, 189.9527681330539792 ) ) ;
#66961=CARTESIAN_POINT ( 'NONE',  ( 107.0664832912739399, -36.72944715994096754, 299.5704287327187103 ) ) ;
#66962=CARTESIAN_POINT ( 'NONE',  ( 112.8804553289902799, -43.12032145944222350, 277.6356252759110816 ) ) ;
#66970=FACE_OUTER_BOUND ( 'NONE', #32563, .T. ) ;
#66972=CARTESIAN_POINT ( 'NONE',  ( 136.8105871997954921, -18.91414947189459994, 6.758631288822851246 ) ) ;
#66973=CARTESIAN_POINT ( 'NONE',  ( 98.92532678050559980, -30.18208626920050719, 240.7870538473399620 ) ) ;
#66974=CARTESIAN_POINT ( 'NONE',  ( 117.5953528424095254, -42.16796915894857278, 89.44705384733997278 ) ) ;
#66975=CARTESIAN_POINT ( 'NONE',  ( 96.72972436280956288, -34.86144565006776475, 237.1841967044819626 ) ) ;
#66976=FACE_OUTER_BOUND ( 'NONE', #75919, .T. ) ;
#66978=LINE ( 'NONE', #17932, #2 ) ;
#66979=CARTESIAN_POINT ( 'NONE',  ( 115.5712346005784354, -42.04052312869856678, 39.38203999088909057 ) ) ;
#66983=AXIS2_PLACEMENT_3D ( 'NONE', #71463, #36924, #30111 ) ;
#66986=CARTESIAN_POINT ( 'NONE',  ( 115.7614890496577402, -39.26115509793221747, 138.0114674471239766 ) ) ;
#66988=ORIENTED_EDGE ( 'NONE', *, *, #48226, .T. ) ;
#66989=CARTESIAN_POINT ( 'NONE',  ( 51.06648329127400388, 0.2215528400590083269, 330.1506252759110680 ) ) ;
#66990=CARTESIAN_POINT ( 'NONE',  ( 97.81366378802363215, -42.73395665195496917, 142.7965776568629508 ) ) ;
#66992=CIRCLE ( 'NONE', #24984, 4.874999999999990230 ) ;
#66993=CARTESIAN_POINT ( 'NONE',  ( 78.35735255114492759, -16.57277629268521224, 7.749696248603636484 ) ) ;
#66994=FACE_OUTER_BOUND ( 'NONE', #70523, .T. ) ;
#66996=CARTESIAN_POINT ( 'NONE',  ( 117.3137205126584348, -38.32096045344801638, 68.69181575210198787 ) ) ;
#67001=CARTESIAN_POINT ( 'NONE',  ( 142.8679068202682458, 10.65431904611001634, 396.9756252759102040 ) ) ;
#67002=CARTESIAN_POINT ( 'NONE',  ( 98.25516505653069999, -40.97492784622581041, 167.6841967044819626 ) ) ;
#67007=EDGE_CURVE ( 'NONE', #83824, #23447, #59930, .T. ) ;
#67009=EDGE_CURVE ( 'NONE', #49381, #54125, #54441, .T. ) ;
#67010=CARTESIAN_POINT ( 'NONE',  ( 180.3521107875639871, -35.65087443492551245, -5.074374724088000832 ) ) ;
#67012=CARTESIAN_POINT ( 'NONE',  ( 102.9796410358629828, -46.29638950891627047, 92.25562527591097250 ) ) ;
#67014=EDGE_LOOP ( 'NONE', ( #87041, #83153, #80598, #9700 ) ) ;
#67015=EDGE_CURVE ( 'NONE', #53062, #58845, #89005, .T. ) ;
#67017=DIRECTION ( 'NONE',  ( 1.000000000000000078E-15, -1.000000000000000000, 0.000000000000000000 ) ) ;
#67020=CARTESIAN_POINT ( 'NONE',  ( 103.8146984276687022, -29.21261587019397155, 153.2195189410199418 ) ) ;
#67022=CIRCLE ( 'NONE', #53900, 3.299999999999997158 ) ;
#67023=ADVANCED_FACE ( 'NONE', ( #13153 ), #80407, .T. ) ;
#67026=ORIENTED_EDGE ( 'NONE', *, *, #10906, .T. ) ;
#67028=VERTEX_POINT ( 'NONE', #12707 ) ;
#67030=VERTEX_POINT ( 'NONE', #59485 ) ;
#67031=CARTESIAN_POINT ( 'NONE',  ( 77.31652006362755003, -18.90534128960216620, 6.749824347015198178 ) ) ;
#67034=CARTESIAN_POINT ( 'NONE',  ( 108.9963713912396912, -28.08052754339530921, 221.3330118773259585 ) ) ;
#67035=CARTESIAN_POINT ( 'NONE',  ( 41.56648329127399677, -18.82844715994099971, 141.0426252759120018 ) ) ;
#67036=CARTESIAN_POINT ( 'NONE',  ( 31.71315051186898870, -31.94127993907790852, -5.074374724088000832 ) ) ;
#67037=VECTOR ( 'NONE', #29911, 1000.000000000000000 ) ;
#67038=LINE ( 'NONE', #88393, #18345 ) ;
#67039=ORIENTED_EDGE ( 'NONE', *, *, #77706, .T. ) ;
#67040=ORIENTED_EDGE ( 'NONE', *, *, #79747, .F. ) ;
#67044=AXIS2_PLACEMENT_3D ( 'NONE', #22086, #7984, #69769 ) ;
#67045=CARTESIAN_POINT ( 'NONE',  ( 114.7858077920586908, -40.64262416812939449, 246.2833284648299639 ) ) ;
#67046=CARTESIAN_POINT ( 'NONE',  ( 96.01222827763220380, -41.06966167057572648, 96.62419670448197451 ) ) ;
#67047=CARTESIAN_POINT ( 'NONE',  ( 117.0329088946583624, -32.00354160957719074, 64.19086337114899266 ) ) ;
#67048=CARTESIAN_POINT ( 'NONE',  ( 112.6580179424443884, -28.69101886885839647, 249.5838068554166398 ) ) ;
#67049=DIRECTION ( 'NONE',  ( 0.000000000000000000, -1.000000000000000000, 0.000000000000000000 ) ) ;
#67050=DIRECTION ( 'NONE',  ( -2.999999999999999839E-15, 1.000000000000000000, -2.999999999999999900E-30 ) ) ;
#67051=CARTESIAN_POINT ( 'NONE',  ( 105.7204281913532355, -24.95562743476950018, 156.1670538473399574 ) ) ;
#67057=CARTESIAN_POINT ( 'NONE',  ( 134.0664832912740110, -8.729447159940999512, 306.1181252759120071 ) ) ;
#67061=B_SPLINE_CURVE_WITH_KNOTS ( 'NONE', 3,
 ( #10301, #3047, #17997, #52049, #79810, #4386, #73411, #38436, #4828, #65700, #30745, #17564, #32511, #38007, #3929, #16674, #25258, #73862 ),
 .UNSPECIFIED., .F., .F.,
 ( 4, 2, 2, 2, 2, 2, 2, 2, 4 ),
 ( 0.5000523659440618829, 0.5625458202010541475, 0.6250392744580464122, 0.6875327287150386768, 0.7500261829720309414, 0.8125196372290232061, 0.8750130914860154707, 0.9375065457430077354, 1.000000000000000000 ),
 .UNSPECIFIED. ) ;
#67063=ORIENTED_EDGE ( 'NONE', *, *, #57495, .T. ) ;
#67064=CARTESIAN_POINT ( 'NONE',  ( 112.0659116076490136, -45.48839626926737623, 177.9897919413786553 ) ) ;
#67065=CARTESIAN_POINT ( 'NONE',  ( 117.8566403422286299, -39.12769616061267186, 103.6403871806729455 ) ) ;
#67066=CARTESIAN_POINT ( 'NONE',  ( 134.0664832912740110, -46.72944715994100306, 8.225625275910998013 ) ) ;
#67067=CARTESIAN_POINT ( 'NONE',  ( 63.03715912545637678, -24.42818131006026761, 193.9678068554150911 ) ) ;
#67069=CARTESIAN_POINT ( 'NONE',  ( 98.13101841594837538, -32.75189731695855500, 100.9927681330539713 ) ) ;
#67071=CARTESIAN_POINT ( 'NONE',  ( 118.8526415125688800, -37.69623653580512013, 184.7613395616249647 ) ) ;
#67074=EDGE_LOOP ( 'NONE', ( #32145, #57884 ) ) ;
#67076=VECTOR ( 'NONE', #4438, 1000.000000000000000 ) ;
#67080=EDGE_CURVE ( 'NONE', #43693, #21567, #28551, .T. ) ;
#67081=CARTESIAN_POINT ( 'NONE',  ( 107.5119097530387933, -47.18928756557821202, 237.6099109901969655 ) ) ;
#67082=EDGE_LOOP ( 'NONE', ( #30638, #12083, #47807, #9549, #10364, #9729, #77162, #65692, #79825, #32639, #23491, #21197 ) ) ;
#67083=CYLINDRICAL_SURFACE ( 'NONE', #30614, 3.000000000000002665 ) ;
#67084=CARTESIAN_POINT ( 'NONE',  ( 112.1974349349366804, -26.93816038506360755, 10.68038718067299087 ) ) ;
#67085=CARTESIAN_POINT ( 'NONE',  ( 107.9492956907162267, -25.66517399690753720, 111.0251490854349754 ) ) ;
#67086=PLANE ( 'NONE',  #79528 ) ;
#67087=CARTESIAN_POINT ( 'NONE',  ( 80.81782300813070208, -39.40255221908358862, 8.160479982094777540 ) ) ;
#67088=CARTESIAN_POINT ( 'NONE',  ( 19.56648329127303043, -71.37844715994266664, 342.9256252759109884 ) ) ;
#67089=DIRECTION ( 'NONE',  ( 0.000000000000000000, 0.000000000000000000, -1.000000000000000000 ) ) ;
#67090=VERTEX_POINT ( 'NONE', #34921 ) ;
#67091=AXIS2_PLACEMENT_3D ( 'NONE', #1474, #61544, #89280 ) ;
#67092=EDGE_CURVE ( 'NONE', #4783, #70047, #27910, .T. ) ;
#67093=ORIENTED_EDGE ( 'NONE', *, *, #14776, .F. ) ;
#67095=VERTEX_POINT ( 'NONE', #27213 ) ;
#67096=DIRECTION ( 'NONE',  ( 0.000000000000000000, 0.000000000000000000, 1.000000000000000000 ) ) ;
#67097=CARTESIAN_POINT ( 'NONE',  ( 96.20032699425235023, -38.62430069186628856, 42.45181575210199298 ) ) ;
#67098=CARTESIAN_POINT ( 'NONE',  ( 107.0664832912739968, -36.72944715994100306, 287.6356252759109680 ) ) ;
#67100=CIRCLE ( 'NONE', #3308, 2.029999999999997140 ) ;
#67103=CARTESIAN_POINT ( 'NONE',  ( 106.8904373410712481, -45.78382058659838094, 226.9714674471249509 ) ) ;
#67105=ORIENTED_EDGE ( 'NONE', *, *, #28078, .T. ) ;
#67108=PLANE ( 'NONE',  #34039 ) ;
#67109=CARTESIAN_POINT ( 'NONE',  ( 117.0718539717828008, -35.46213750492159278, 103.9271830989822263 ) ) ;
#67110=DIRECTION ( 'NONE',  ( -1.000000000000000078E-15, 1.000000000000000083E-30, 1.000000000000000000 ) ) ;
#67111=CARTESIAN_POINT ( 'NONE',  ( 179.8608231853560255, -35.55794170701751256, -5.074374724088000832 ) ) ;
#67113=CARTESIAN_POINT ( 'NONE',  ( 98.24556308671769500, -33.49403671529641713, 17.46634521065892898 ) ) ;
#67116=EDGE_CURVE ( 'NONE', #63079, #11460, #56241, .T. ) ;
#67118=CARTESIAN_POINT ( 'NONE',  ( 107.9555263298577330, -25.64695713395843413, 265.0127681330543510 ) ) ;
#67121=ADVANCED_FACE ( 'NONE', ( #76715 ), #14499, .T. ) ;
#67122=CARTESIAN_POINT ( 'NONE',  ( 98.34917020181003977, -31.65781948494475628, 56.90649411614629827 ) ) ;
#67124=CARTESIAN_POINT ( 'NONE',  ( 113.8488019003066825, -42.10541956792432217, 46.12332846482897253 ) ) ;
#67126=CARTESIAN_POINT ( 'NONE',  ( 163.0959832912771219, -23.42844715993521021, 237.4678068554150059 ) ) ;
#67127=EDGE_CURVE ( 'NONE', #72016, #56141, #42173, .T. ) ;
#67129=VERTEX_POINT ( 'NONE', #29020 ) ;
#67132=VECTOR ( 'NONE', #46530, 1000.000000000000114 ) ;
#67133=ORIENTED_EDGE ( 'NONE', *, *, #71601, .F. ) ;
#67134=CARTESIAN_POINT ( 'NONE',  ( 118.9039262414038944, -36.16781539521252142, 118.8641967044819836 ) ) ;
#67136=CARTESIAN_POINT ( 'NONE',  ( 116.0261628859374383, -38.04732875056770780, 73.14480078045792766 ) ) ;
#67137=CARTESIAN_POINT ( 'NONE',  ( 160.5667039024485518, -48.82844715993551432, 180.4678068554150059 ) ) ;
#67138=CARTESIAN_POINT ( 'NONE',  ( 103.0168143257329092, -28.81349422576414554, 116.8844404487539634 ) ) ;
#67141=CARTESIAN_POINT ( 'NONE',  ( 107.1956677504039135, -26.28336798021810239, 31.06705384733893283 ) ) ;
#67142=DIRECTION ( 'NONE',  ( 1.000000000000000000, 0.000000000000000000, 0.000000000000000000 ) ) ;
#67143=ORIENTED_EDGE ( 'NONE', *, *, #44114, .F. ) ;
#67144=CIRCLE ( 'NONE', #14906, 2.125000000000001776 ) ;
#67145=FACE_OUTER_BOUND ( 'NONE', #72579, .T. ) ;
#67149=VERTEX_POINT ( 'NONE', #48086 ) ;
#67151=ORIENTED_EDGE ( 'NONE', *, *, #12427, .F. ) ;
#67152=CARTESIAN_POINT ( 'NONE',  ( 100.6696166679599003, -29.33055989933767904, 260.6441967044828516 ) ) ;
#67153=CARTESIAN_POINT ( 'NONE',  ( 97.19489835230788799, -38.38517845848406296, 126.4581417767985698 ) ) ;
#67155=CARTESIAN_POINT ( 'NONE',  ( 100.9411170126626587, -46.87412574091977291, 48.14419670448194211 ) ) ;
#67156=FACE_OUTER_BOUND ( 'NONE', #2708, .T. ) ;
#67157=EDGE_LOOP ( 'NONE', ( #4537, #73735, #75145, #51556 ) ) ;
#67158=LINE ( 'NONE', #33092, #87348 ) ;
#67160=EDGE_CURVE ( 'NONE', #47420, #87937, #39514, .T. ) ;
#67162=AXIS2_PLACEMENT_3D ( 'NONE', #54418, #39915, #60808 ) ;
#67165=CARTESIAN_POINT ( 'NONE',  ( 104.5933598291445463, -26.62426044571792616, 285.2670538473396391 ) ) ;
#67166=CARTESIAN_POINT ( 'NONE',  ( 62.03742497533746558, -23.42844715994041849, 300.4678068554150627 ) ) ;
#67167=AXIS2_PLACEMENT_3D ( 'NONE', #53167, #59996, #39124 ) ;
#67170=CARTESIAN_POINT ( 'NONE',  ( 106.8780034376490278, -45.26880352128168283, 271.9809912566482808 ) ) ;
#67172=CARTESIAN_POINT ( 'NONE',  ( 172.5664832912729878, -18.82844715994071194, 258.9256252759120116 ) ) ;
#67173=CARTESIAN_POINT ( 'NONE',  ( 96.67837842349544530, -37.29153504031420141, 72.36991099019596163 ) ) ;
#67175=CARTESIAN_POINT ( 'NONE',  ( 108.8564100269821608, -47.04462182233018552, 167.7127681330539701 ) ) ;
#67176=ORIENTED_EDGE ( 'NONE', *, *, #53761, .T. ) ;
#67179=FACE_OUTER_BOUND ( 'NONE', #64023, .T. ) ;
#67180=CARTESIAN_POINT ( 'NONE',  ( 115.0889047208644627, -30.61763667535547029, 65.34395860967845238 ) ) ;
#67181=DIRECTION ( 'NONE',  ( 0.000000000000000000, -1.000000000000000000, 0.000000000000000000 ) ) ;
#67183=CARTESIAN_POINT ( 'NONE',  ( 63.06670390244707392, -40.32844715994016838, 180.4678068554151196 ) ) ;
#67184=CARTESIAN_POINT ( 'NONE',  ( 95.96722792477895325, -36.58315769931292749, 156.3280062282919687 ) ) ;
#67185=ORIENTED_EDGE ( 'NONE', *, *, #42607, .T. ) ;
#67186=LINE ( 'NONE', #88102, #43632 ) ;
#67189=CARTESIAN_POINT ( 'NONE',  ( 167.6524903400753033, -48.32844715993521589, 300.4678068554149490 ) ) ;
#67190=ORIENTED_EDGE ( 'NONE', *, *, #86925, .F. ) ;
#67191=EDGE_CURVE ( 'NONE', #74209, #53860, #43065, .T. ) ;
#67192=CARTESIAN_POINT ( 'NONE',  ( 111.8042541167996546, -25.83965636698058432, 134.7499109901969518 ) ) ;
#67195=CYLINDRICAL_SURFACE ( 'NONE', #24006, 5.599999999999994316 ) ;
#67197=VERTEX_POINT ( 'NONE', #41721 ) ;
#67198=CIRCLE ( 'NONE', #45452, 2.500000000000002220 ) ;
#67204=CARTESIAN_POINT ( 'NONE',  ( 116.3183303039212291, -32.94226276200836878, 104.1356252759109680 ) ) ;
#67205=DIRECTION ( 'NONE',  ( 0.000000000000000000, 0.000000000000000000, 1.000000000000000000 ) ) ;
#67206=CARTESIAN_POINT ( 'NONE',  ( 104.4897722840256904, -26.97885345335833662, 180.2814733255143551 ) ) ;
#67207=CIRCLE ( 'NONE', #52654, 0.5000000000000004441 ) ;
#67208=ORIENTED_EDGE ( 'NONE', *, *, #57918, .F. ) ;
#67209=LINE ( 'NONE', #89011, #40399 ) ;
#67210=CARTESIAN_POINT ( 'NONE',  ( 98.91665286848252947, -30.31703347128394910, 196.8080062282909637 ) ) ;
#67211=EDGE_CURVE ( 'NONE', #19079, #89932, #77170, .T. ) ;
#67212=DIRECTION ( 'NONE',  ( 0.7071067811865758834, -0.7071067811865192621, 7.071067811865766226E-16 ) ) ;
#67213=ORIENTED_EDGE ( 'NONE', *, *, #7878, .F. ) ;
#67214=CARTESIAN_POINT ( 'NONE',  ( 99.11394507416773081, -43.38496525699387973, 67.86895860924396118 ) ) ;
#67215=ADVANCED_FACE ( 'NONE', ( #83992 ), #21765, .F. ) ;
#67216=CARTESIAN_POINT ( 'NONE',  ( 117.0886499745419513, -37.65698274825507497, 53.75263814202077839 ) ) ;
#67218=CARTESIAN_POINT ( 'NONE',  ( 46.83715912545429205, -47.82818131006082751, 249.9678068554150343 ) ) ;
#67219=CARTESIAN_POINT ( 'NONE',  ( 97.78478733939310530, -40.45112047135063449, 22.62993014185689944 ) ) ;
#67221=DIRECTION ( 'NONE',  ( 1.000000000000000000, 0.000000000000000000, 0.000000000000000000 ) ) ;
#67222=ADVANCED_FACE ( 'NONE', ( #13589 ), #69005, .T. ) ;
#67223=VERTEX_POINT ( 'NONE', #31232 ) ;
#67224=ORIENTED_EDGE ( 'NONE', *, *, #257, .T. ) ;
#67225=CARTESIAN_POINT ( 'NONE',  ( 100.1238157808075186, -30.39889478464921524, 227.1577737820879577 ) ) ;
#67227=CARTESIAN_POINT ( 'NONE',  ( 108.3351572350362062, -46.73467433967125118, 53.67707132820591909 ) ) ;
#67230=CARTESIAN_POINT ( 'NONE',  ( 97.06107109568941382, -37.99641195077763456, 81.42729194155585049 ) ) ;
#67233=ORIENTED_EDGE ( 'NONE', *, *, #38318, .T. ) ;
#67234=CARTESIAN_POINT ( 'NONE',  ( 123.6837132603318992, -20.11243780205710507, 239.5838068554165545 ) ) ;
#67235=CARTESIAN_POINT ( 'NONE',  ( 100.9506838420298749, -28.71014652038285320, 36.59397677644053459 ) ) ;
#67236=ADVANCED_FACE ( 'NONE', ( #9462 ), #78528, .T. ) ;
#67237=ORIENTED_EDGE ( 'NONE', *, *, #22224, .F. ) ;
#67238=CARTESIAN_POINT ( 'NONE',  ( 111.0463177226254174, -47.04157800189014438, 17.85753003781598380 ) ) ;
#67239=ORIENTED_EDGE ( 'NONE', *, *, #21379, .T. ) ;
#67240=EDGE_LOOP ( 'NONE', ( #199, #21375 ) ) ;
#67241=CARTESIAN_POINT ( 'NONE',  ( 102.1781415585801511, -43.87122846086534622, 239.9290427505439709 ) ) ;
#67242=CARTESIAN_POINT ( 'NONE',  ( 98.36735121233621726, -42.37464764417353535, 146.7965776568640024 ) ) ;
#67244=DIRECTION ( 'NONE',  ( 1.000000000000000078E-15, -1.000000000000000083E-30, -1.000000000000000000 ) ) ;
#67245=CARTESIAN_POINT ( 'NONE',  ( 182.3467384525650061, -36.02818131005800950, -5.074374724088000832 ) ) ;
#67246=CARTESIAN_POINT ( 'NONE',  ( 103.7092163704185026, -26.14992651007402813, 201.3089586092439731 ) ) ;
#67248=ORIENTED_EDGE ( 'NONE', *, *, #46986, .F. ) ;
#67249=AXIS2_PLACEMENT_3D ( 'NONE', #55711, #68032, #28482 ) ;
#67250=CARTESIAN_POINT ( 'NONE',  ( 113.3686263934108780, -27.59268128360266914, 85.60800622829195561 ) ) ;
#67251=DIRECTION ( 'NONE',  ( 1.387778780781444492E-15, 0.000000000000000000, -1.000000000000000000 ) ) ;
#67253=EDGE_LOOP ( 'NONE', ( #42782, #76178 ) ) ;
#67257=CARTESIAN_POINT ( 'NONE',  ( 165.6738106836030227, -28.98061976758901892, -5.074374724088000832 ) ) ;
#67259=CARTESIAN_POINT ( 'NONE',  ( 117.0603328428218077, -38.08441083969534446, 153.7194074594665381 ) ) ;
#67260=CARTESIAN_POINT ( 'NONE',  ( 101.0810522191901981, -29.63898995574150419, 148.4538046553059587 ) ) ;
#67261=CARTESIAN_POINT ( 'NONE',  ( 113.1126646695910409, -46.01001268607183903, 219.0480062282919960 ) ) ;
#67263=ORIENTED_EDGE ( 'NONE', *, *, #40125, .T. ) ;
#67267=VERTEX_POINT ( 'NONE', #37170 ) ;
#67268=VERTEX_POINT ( 'NONE', #79868 ) ;
#67269=CIRCLE ( 'NONE', #32447, 1.000000000000000888 ) ;
#67271=ORIENTED_EDGE ( 'NONE', *, *, #32024, .T. ) ;
#67273=CARTESIAN_POINT ( 'NONE',  ( 107.0664832912739399, -36.72944715994095333, 293.1356252759106837 ) ) ;
#67275=EDGE_CURVE ( 'NONE', #79236, #311, #29362, .T. ) ;
#67276=DIRECTION ( 'NONE',  ( -0.9068632946707806397, 0.4214249218767882055, -9.068632946707802473E-16 ) ) ;
#67277=CARTESIAN_POINT ( 'NONE',  ( 97.92582740012257148, -33.45545302834237589, 175.4752769709339759 ) ) ;
#67278=CARTESIAN_POINT ( 'NONE',  ( 102.7370178780992234, -25.64411770250132250, 20.37276813305294354 ) ) ;
#67280=ORIENTED_EDGE ( 'NONE', *, *, #85322, .T. ) ;
#67284=VERTEX_POINT ( 'NONE', #85347 ) ;
#67287=CARTESIAN_POINT ( 'NONE',  ( 110.8534530311471400, -45.98465435386854949, 132.8855376447518211 ) ) ;
#67288=VECTOR ( 'NONE', #31886, 1000.000000000000000 ) ;
#67291=CARTESIAN_POINT ( 'NONE',  ( 112.1921266949303373, -27.58526089107821733, 34.66991099019695355 ) ) ;
#67292=CARTESIAN_POINT ( 'NONE',  ( 100.9176109441957436, -28.25688269532019348, 71.57562527591099411 ) ) ;
#67293=AXIS2_PLACEMENT_3D ( 'NONE', #57331, #23305, #9208 ) ;
#67296=CARTESIAN_POINT ( 'NONE',  ( 113.2455109352893743, -28.75868235514402116, 145.5526372974719322 ) ) ;
#67298=FACE_BOUND ( 'NONE', #61662, .T. ) ;
#67301=EDGE_CURVE ( 'NONE', #8428, #76842, #26481, .T. ) ;
#67303=CARTESIAN_POINT ( 'NONE',  ( 96.91385697446291658, -32.24201331651869396, 55.98324432352897162 ) ) ;
#67304=CARTESIAN_POINT ( 'NONE',  ( 109.6058369744873886, -26.58188510553521056, 195.8813395616249977 ) ) ;
#67305=CARTESIAN_POINT ( 'NONE',  ( 110.1643932622899200, -46.70643130671602705, 93.81562527591097478 ) ) ;
#67306=CARTESIAN_POINT ( 'NONE',  ( 104.4090054903168578, -46.45835489918496819, 172.3615705418780522 ) ) ;
#67307=LINE ( 'NONE', #74577, #36916 ) ;
#67313=CARTESIAN_POINT ( 'NONE',  ( 116.9446180447426826, -41.83184233209001235, 89.44705384733897802 ) ) ;
#67317=CARTESIAN_POINT ( 'NONE',  ( 116.5068947302721369, -41.18400185692900806, 224.4756252759109714 ) ) ;
#67318=CARTESIAN_POINT ( 'NONE',  ( 116.7949704630636063, -39.38841653000326914, 254.6162222944404334 ) ) ;
#67319=CARTESIAN_POINT ( 'NONE',  ( 114.5888079921489719, -43.35084876185531044, 148.2521628986096971 ) ) ;
#67320=DIRECTION ( 'NONE',  ( 0.000000000000000000, 0.000000000000000000, 1.000000000000000000 ) ) ;
#67321=EDGE_CURVE ( 'NONE', #60536, #11261, #64431, .T. ) ;
#67322=CARTESIAN_POINT ( 'NONE',  ( 113.2454986953204781, -28.75867294251674267, 45.55229194285107752 ) ) ;
#67323=CARTESIAN_POINT ( 'NONE',  ( 51.24204729617298426, -31.76306994223730840, -5.074374724088000832 ) ) ;
#67325=CARTESIAN_POINT ( 'NONE',  ( 114.0056865186722490, -29.02320718445394476, 159.5051490854349652 ) ) ;
#67326=VERTEX_POINT ( 'NONE', #9032 ) ;
#67328=CARTESIAN_POINT ( 'NONE',  ( 104.0080147226004925, -45.04654038386073012, 138.7272975916119435 ) ) ;
#67329=CARTESIAN_POINT ( 'NONE',  ( 165.3359832912740046, -36.32844715994100682, -5.074374724088000832 ) ) ;
#67330=CARTESIAN_POINT ( 'NONE',  ( 104.1325824198641783, -27.39908484284276469, 246.3184824187669619 ) ) ;
#67333=CARTESIAN_POINT ( 'NONE',  ( 182.5667039024469886, -33.35206098992650681, -5.074374724088000832 ) ) ;
#67334=EDGE_CURVE ( 'NONE', #36063, #46977, #44406, .T. ) ;
#67335=FACE_OUTER_BOUND ( 'NONE', #77602, .T. ) ;
#67337=LINE ( 'NONE', #45535, #44413 ) ;
#67338=EDGE_CURVE ( 'NONE', #39978, #12989, #9918, .T. ) ;
#67339=CARTESIAN_POINT ( 'NONE',  ( 117.4047238282099102, -30.98758422922431066, 179.2299109901959753 ) ) ;
#67341=VERTEX_POINT ( 'NONE', #30798 ) ;
#67345=CARTESIAN_POINT ( 'NONE',  ( 188.5667039024479834, -65.37844715994100397, 132.3428068554150343 ) ) ;
#67347=AXIS2_PLACEMENT_3D ( 'NONE', #56350, #54986, #75018 ) ;
#67349=VERTEX_POINT ( 'NONE', #58491 ) ;
#67351=AXIS2_PLACEMENT_3D ( 'NONE', #19486, #83506, #76694 ) ;
#67352=CARTESIAN_POINT ( 'NONE',  ( 103.8197072928965810, -48.12676840017521585, 217.3556252759109668 ) ) ;
#67353=CARTESIAN_POINT ( 'NONE',  ( 134.8178230081300910, -39.40255221908513761, 8.160479982094942741 ) ) ;
#67355=ORIENTED_EDGE ( 'NONE', *, *, #29850, .T. ) ;
#67357=DIRECTION ( 'NONE',  ( 0.7071067811865460184, 0.000000000000000000, 0.7071067811865487940 ) ) ;
#67358=CARTESIAN_POINT ( 'NONE',  ( 97.81168148112675453, -40.51739256386586163, 162.6360428395636859 ) ) ;
#67359=CARTESIAN_POINT ( 'NONE',  ( 99.24357903948710202, -34.39880452655780374, 28.91380465530596311 ) ) ;
#67360=CARTESIAN_POINT ( 'NONE',  ( 117.2592865896494345, -39.02220311275136311, 144.6499109901969859 ) ) ;
#67361=DIRECTION ( 'NONE',  ( 0.000000000000000000, 1.000000000000000000, 0.000000000000000000 ) ) ;
#67364=CARTESIAN_POINT ( 'NONE',  ( 62.03715912545748523, -47.82818131006031592, 193.9678068554150911 ) ) ;
#67365=ORIENTED_EDGE ( 'NONE', *, *, #76037, .T. ) ;
#67366=ORIENTED_EDGE ( 'NONE', *, *, #42294, .T. ) ;
#67368=CIRCLE ( 'NONE', #52808, 2.999999999999919176 ) ;
#67369=LINE ( 'NONE', #39228, #72023 ) ;
#67374=VECTOR ( 'NONE', #20611, 1000.000000000000000 ) ;
#67376=CARTESIAN_POINT ( 'NONE',  ( 115.9627085491522536, -40.61889491704908295, 57.92099125664801562 ) ) ;
#67377=CARTESIAN_POINT ( 'NONE',  ( 115.4056828889858650, -30.43626719779562251, 219.3413395616249773 ) ) ;
#67378=AXIS2_PLACEMENT_3D ( 'NONE', #66880, #18735, #39615 ) ;
#67379=CARTESIAN_POINT ( 'NONE',  ( 117.0023065291009061, -39.93004192841232936, 158.5784824187679476 ) ) ;
#67380=DIRECTION ( 'NONE',  ( -4.012088370409549976E-14, 1.000000000000000000, 0.000000000000000000 ) ) ;
#67381=CARTESIAN_POINT ( 'NONE',  ( 99.77739493559407435, -44.20163642594127396, 17.96133956162493206 ) ) ;
#67382=DIRECTION ( 'NONE',  ( 0.000000000000000000, 0.000000000000000000, -1.000000000000000000 ) ) ;
#67384=ORIENTED_EDGE ( 'NONE', *, *, #12391, .T. ) ;
#67386=DIRECTION ( 'NONE',  ( 0.000000000000000000, 0.000000000000000000, -1.000000000000000000 ) ) ;
#67387=CARTESIAN_POINT ( 'NONE',  ( 97.05395071892901626, -41.52132310946490890, 216.6937205140059461 ) ) ;
#67388=EDGE_LOOP ( 'NONE', ( #50861, #78899, #36913, #17063 ) ) ;
#67390=CARTESIAN_POINT ( 'NONE',  ( 112.2051334037466432, -45.80035149650004200, 212.9870538473389558 ) ) ;
#67391=CARTESIAN_POINT ( 'NONE',  ( 149.4532656544376721, -72.54365454176046057, 361.9756252759100335 ) ) ;
#67393=CARTESIAN_POINT ( 'NONE',  ( 97.81542051716436958, -40.52653337087284058, 22.63640890594763633 ) ) ;
#67395=VECTOR ( 'NONE', #61923, 1000.000000000000000 ) ;
#67396=EDGE_CURVE ( 'NONE', #55229, #56684, #8578, .T. ) ;
#67397=CARTESIAN_POINT ( 'NONE',  ( 109.6536531575482769, -29.13850702246578095, 277.6356252759110816 ) ) ;
#67401=LINE ( 'NONE', #5193, #10688 ) ;
#67402=EDGE_CURVE ( 'NONE', #34477, #51283, #57146, .T. ) ;
#67404=CARTESIAN_POINT ( 'NONE',  ( 51.06670390244764945, -33.35206098992665602, 313.9678068554150059 ) ) ;
#67405=EDGE_CURVE ( 'NONE', #31634, #42012, #84892, .T. ) ;
#67407=CARTESIAN_POINT ( 'NONE',  ( 154.4409905298078058, -0.9147987323338667709, 542.9756252759101471 ) ) ;
#67408=ORIENTED_EDGE ( 'NONE', *, *, #66313, .T. ) ;
#67409=EDGE_CURVE ( 'NONE', #72895, #54496, #75767, .T. ) ;
#67410=DIRECTION ( 'NONE',  ( 1.000000000000000000, 4.299999999999999979E-14, 1.000000000000000078E-15 ) ) ;
#67411=CARTESIAN_POINT ( 'NONE',  ( 103.2955449146038376, -26.98642977692344758, 215.3699109901969848 ) ) ;
#67412=CARTESIAN_POINT ( 'NONE',  ( 108.3194443806174405, -47.07896772641721839, 113.6727681330539639 ) ) ;
#67413=CARTESIAN_POINT ( 'NONE',  ( 96.47406283524195203, -31.30618784601239923, 241.9499109901969689 ) ) ;
#67417=DIRECTION ( 'NONE',  ( 0.000000000000000000, 0.000000000000000000, 1.000000000000000000 ) ) ;
#67419=EDGE_CURVE ( 'NONE', #64922, #60205, #61180, .T. ) ;
#67420=CARTESIAN_POINT ( 'NONE',  ( 134.0664832912739826, -21.47944715994100306, 1.625625275910997480 ) ) ;
#67422=AXIS2_PLACEMENT_3D ( 'NONE', #46615, #60247, #66170 ) ;
#67424=ORIENTED_EDGE ( 'NONE', *, *, #31874, .T. ) ;
#67425=ORIENTED_EDGE ( 'NONE', *, *, #74276, .F. ) ;
#67426=CARTESIAN_POINT ( 'NONE',  ( 111.2069583914694419, -45.51165039160690640, 137.3495626852199507 ) ) ;
#67428=ORIENTED_EDGE ( 'NONE', *, *, #49988, .F. ) ;
#67430=CARTESIAN_POINT ( 'NONE',  ( 97.59110611908495514, -31.08311649095520934, 126.9108633711489915 ) ) ;
#67431=EDGE_CURVE ( 'NONE', #46552, #88862, #17796, .T. ) ;
#67432=DIRECTION ( 'NONE',  ( -0.9834602067153815907, -0.1811243269341220596, 0.000000000000000000 ) ) ;
#67434=DIRECTION ( 'NONE',  ( 1.000000000000000078E-15, 1.000000000000000083E-30, -1.000000000000000000 ) ) ;
#67436=DIRECTION ( 'NONE',  ( 1.639958061481212836E-42, -4.100000000000000342E-29, -1.000000000000000000 ) ) ;
#67437=CARTESIAN_POINT ( 'NONE',  ( 107.2219638487720488, -26.36052190073617041, 80.07657765686398932 ) ) ;
#67439=ORIENTED_EDGE ( 'NONE', *, *, #60712, .F. ) ;
#67441=VECTOR ( 'NONE', #23009, 1000.000000000000000 ) ;
#67444=VECTOR ( 'NONE', #76622, 1000.000000000000000 ) ;
#67445=CARTESIAN_POINT ( 'NONE',  ( 99.36405074150921735, -30.70139697576588134, 151.7984824187679465 ) ) ;
#67447=CIRCLE ( 'NONE', #2174, 3.300000000000000711 ) ;
#67451=CARTESIAN_POINT ( 'NONE',  ( 107.0664832912739968, -36.72944715994100306, 293.2242906452868851 ) ) ;
#67452=EDGE_CURVE ( 'NONE', #27298, #43762, #5333, .T. ) ;
#67453=AXIS2_PLACEMENT_3D ( 'NONE', #14864, #15753, #30273 ) ;
#67454=CARTESIAN_POINT ( 'NONE',  ( 130.3998166246059895, 12.92155284005730387, 355.9756252759109998 ) ) ;
#67457=CARTESIAN_POINT ( 'NONE',  ( 114.5517459224756749, -44.00510994954056088, 98.21276813305395592 ) ) ;
#67458=ORIENTED_EDGE ( 'NONE', *, *, #28026, .T. ) ;
#67459=EDGE_LOOP ( 'NONE', ( #5877, #20250 ) ) ;
#67460=EDGE_CURVE ( 'NONE', #80917, #25435, #45328, .T. ) ;
#67461=CARTESIAN_POINT ( 'NONE',  ( 162.7866693523297101, -29.62846900981741527, 193.9678068554149775 ) ) ;
#67463=EDGE_CURVE ( 'NONE', #7253, #51570, #33028, .T. ) ;
#67464=DIRECTION ( 'NONE',  ( -0.7071067811607679721, 0.7071067812123270624, 0.000000000000000000 ) ) ;
#67466=CARTESIAN_POINT ( 'NONE',  ( 108.2592170473780300, -44.83253820548913637, 140.5109475124479559 ) ) ;
#67467=CIRCLE ( 'NONE', #79101, 2.517500000000005844 ) ;
#67468=DIRECTION ( 'NONE',  ( 0.000000000000000000, 0.000000000000000000, 1.000000000000000000 ) ) ;
#67469=ORIENTED_EDGE ( 'NONE', *, *, #7188, .F. ) ;
#67470=ORIENTED_EDGE ( 'NONE', *, *, #43553, .T. ) ;
#67471=DIRECTION ( 'NONE',  ( 1.000000000000000078E-15, -1.000000000000000083E-30, -1.000000000000000000 ) ) ;
#67472=ORIENTED_EDGE ( 'NONE', *, *, #72717, .T. ) ;
#67473=ORIENTED_EDGE ( 'NONE', *, *, #56043, .F. ) ;
#67475=CARTESIAN_POINT ( 'NONE',  ( 114.1399574501865999, -31.39144735336052605, 215.7730118773249899 ) ) ;
#67476=DIRECTION ( 'NONE',  ( 0.000000000000000000, 0.000000000000000000, -1.000000000000000000 ) ) ;
#67477=DIRECTION ( 'NONE',  ( 0.7071067811571405404, 0.7071067812159546051, 0.000000000000000000 ) ) ;
#67479=CARTESIAN_POINT ( 'NONE',  ( 62.03715912545833078, -47.82818131006032303, 313.9678068554150059 ) ) ;
#67480=VERTEX_POINT ( 'NONE', #74820 ) ;
#67482=VECTOR ( 'NONE', #88328, 1000.000000000000000 ) ;
#67483=ORIENTED_EDGE ( 'NONE', *, *, #54256, .T. ) ;
#67485=CARTESIAN_POINT ( 'NONE',  ( 98.61142602524013512, -34.88203500400037882, 253.9614237029248613 ) ) ;
#67486=CARTESIAN_POINT ( 'NONE',  ( 117.8794170024721240, -39.13275856168890243, 103.6403871806729455 ) ) ;
#67487=CARTESIAN_POINT ( 'NONE',  ( 98.32466564902610173, -28.76522518762216052, 80.73848241876795839 ) ) ;
#67488=CARTESIAN_POINT ( 'NONE',  ( 110.7648612237299801, -44.41958673050639561, 249.5838068554167535 ) ) ;
#67489=CARTESIAN_POINT ( 'NONE',  ( 131.3164832912739826, -18.72944715994100662, 6.749768910606465333 ) ) ;
#67490=DIRECTION ( 'NONE',  ( -0.7071067811865789920, 0.7071067811865159314, 0.000000000000000000 ) ) ;
#67491=CARTESIAN_POINT ( 'NONE',  ( 114.1247157756359769, -29.05716968555177004, 195.4841967044819739 ) ) ;
#67492=CARTESIAN_POINT ( 'NONE',  ( 100.1135588076987943, -43.99268716865574902, 276.9687004125333942 ) ) ;
#67494=CARTESIAN_POINT ( 'NONE',  ( 177.8371591254545478, -47.82818131005478079, 117.4678068554150485 ) ) ;
#67498=ORIENTED_EDGE ( 'NONE', *, *, #51168, .T. ) ;
#67499=AXIS2_PLACEMENT_3D ( 'NONE', #51787, #32703, #39962 ) ;
#67501=VECTOR ( 'NONE', #41517, 1000.000000000000000 ) ;
#67502=CARTESIAN_POINT ( 'NONE',  ( 97.33761227910700597, -34.07199620930350648, 92.11486736599003677 ) ) ;
#67503=CARTESIAN_POINT ( 'NONE',  ( 96.63902489370863691, -37.56252461247890295, 101.3899109901969524 ) ) ;
#67506=ADVANCED_FACE ( 'NONE', ( #54339 ), #18501, .F. ) ;
#67507=CARTESIAN_POINT ( 'NONE',  ( 57.56670390244804736, -42.82844715994040286, 290.7178068554150627 ) ) ;
#67511=CARTESIAN_POINT ( 'NONE',  ( 97.82866780357528569, -40.55868606849465152, 56.63876441442555887 ) ) ;
#67512=CARTESIAN_POINT ( 'NONE',  ( 96.70388795518327640, -35.81005419191409089, 227.2556252759109725 ) ) ;
#67513=DIRECTION ( 'NONE',  ( 1.000000000000000000, -1.000000000000000078E-15, 0.000000000000000000 ) ) ;
#67514=LINE ( 'NONE', #40253, #65625 ) ;
#67515=VERTEX_POINT ( 'NONE', #39833 ) ;
#67516=DIRECTION ( 'NONE',  ( 1.000000000000000000, -1.000000000000000078E-15, 0.000000000000000000 ) ) ;
#67517=VECTOR ( 'NONE', #43739, 1000.000000000000000 ) ;
#67518=EDGE_CURVE ( 'NONE', #3872, #60536, #32126, .T. ) ;
#67520=CARTESIAN_POINT ( 'NONE',  ( 104.4911451993404370, -26.97846757028417031, 135.2813199360520287 ) ) ;
#67521=AXIS2_PLACEMENT_3D ( 'NONE', #62474, #63376, #34771 ) ;
#67522=EDGE_CURVE ( 'NONE', #4391, #13427, #40937, .T. ) ;
#67524=CARTESIAN_POINT ( 'NONE',  ( 116.0932472193867966, -42.03267250216092776, 238.4041967044829562 ) ) ;
#67525=VERTEX_POINT ( 'NONE', #82105 ) ;
#67526=EDGE_CURVE ( 'NONE', #17905, #72562, #1797, .T. ) ;
#67528=CARTESIAN_POINT ( 'NONE',  ( 99.31704471179752147, -28.81544643672065220, 266.7051490854347549 ) ) ;
#67529=CARTESIAN_POINT ( 'NONE',  ( 116.8361817273313790, -32.96833395228159702, 135.1184824187679396 ) ) ;
#67532=CIRCLE ( 'NONE', #35630, 2.750000000000002665 ) ;
#67535=DIRECTION ( 'NONE',  ( -2.900000000000000265E-14, 2.000000000000000155E-15, -1.000000000000000000 ) ) ;
#67536=CARTESIAN_POINT ( 'NONE',  ( 73.10937651008747196, -8.833000550534334749, 14.92562527591099375 ) ) ;
#67537=ORIENTED_EDGE ( 'NONE', *, *, #85470, .F. ) ;
#67539=CIRCLE ( 'NONE', #2326, 3.250000000000002665 ) ;
#67541=VERTEX_POINT ( 'NONE', #60274 ) ;
#67542=ORIENTED_EDGE ( 'NONE', *, *, #65095, .T. ) ;
#67544=DIRECTION ( 'NONE',  ( 0.000000000000000000, 0.000000000000000000, -1.000000000000000000 ) ) ;
#67545=CARTESIAN_POINT ( 'NONE',  ( 109.6066175024219831, -25.17973177368044801, 25.90419670448196143 ) ) ;
#67547=CARTESIAN_POINT ( 'NONE',  ( 134.0664832912740110, -33.97944715994100306, 1.625625275910997480 ) ) ;
#67548=CIRCLE ( 'NONE', #9528, 13.16666666666670160 ) ;
#67549=EDGE_CURVE ( 'NONE', #41311, #59373, #24998, .T. ) ;
#67550=DIRECTION ( 'NONE',  ( 1.000000000000000000, 4.163336342344333240E-14, 0.000000000000000000 ) ) ;
#67551=DIRECTION ( 'NONE',  ( -1.175184669632759901E-16, 1.000000000000000000, 2.000000000000003705E-15 ) ) ;
#67552=CARTESIAN_POINT ( 'NONE',  ( 34.96670390244699433, -26.71338133339301635, -5.074374724088000832 ) ) ;
#67553=CARTESIAN_POINT ( 'NONE',  ( 115.4795240695424923, -35.25402295475319647, 243.3867055423619661 ) ) ;
#67554=ORIENTED_EDGE ( 'NONE', *, *, #35935, .T. ) ;
#67556=ORIENTED_EDGE ( 'NONE', *, *, #88887, .F. ) ;
#67557=VECTOR ( 'NONE', #60797, 1000.000000000000000 ) ;
#67559=CARTESIAN_POINT ( 'NONE',  ( 75.31670390244798341, -50.82844715994100682, 37.63480685541480852 ) ) ;
#67560=AXIS2_PLACEMENT_3D ( 'NONE', #52040, #17555, #85722 ) ;
#67561=CARTESIAN_POINT ( 'NONE',  ( 116.9160198271895723, -38.71580271627102832, 183.6683563841668843 ) ) ;
#67563=DIRECTION ( 'NONE',  ( -3.201858731750027727E-15, 1.000000000000000000, -3.201858731750027724E-30 ) ) ;
#67564=CARTESIAN_POINT ( 'NONE',  ( 114.1881255536272022, -42.05338753103387717, 24.74729759161198217 ) ) ;
#67567=CARTESIAN_POINT ( 'NONE',  ( 117.4251315444616353, -36.24242395571270237, 268.8518157521021408 ) ) ;
#67569=ORIENTED_EDGE ( 'NONE', *, *, #47538, .F. ) ;
#67570=EDGE_CURVE ( 'NONE', #11954, #67267, #41176, .T. ) ;
#67571=CARTESIAN_POINT ( 'NONE',  ( 131.0667039024480118, -61.87844715994100397, 201.9838068554149970 ) ) ;
#67574=CARTESIAN_POINT ( 'NONE',  ( 104.6321197217979488, -45.03455396584281800, 60.15570941721099274 ) ) ;
#67575=VECTOR ( 'NONE', #77190, 999.9999999999998863 ) ;
#67576=AXIS2_PLACEMENT_3D ( 'NONE', #33599, #60394, #61294 ) ;
#67578=CARTESIAN_POINT ( 'NONE',  ( 136.6005499775785665, -17.66120003907372649, 7.039521718172665921 ) ) ;
#67581=CARTESIAN_POINT ( 'NONE',  ( 105.7154054197770137, -46.72384757748508122, 193.4688856702615851 ) ) ;
#67583=CARTESIAN_POINT ( 'NONE',  ( 172.5664832912729878, -27.57844715994070484, 15.92562527591200094 ) ) ;
#67585=ORIENTED_EDGE ( 'NONE', *, *, #70927, .F. ) ;
#67586=CARTESIAN_POINT ( 'NONE',  ( 108.2767148518004490, -26.33900702273897565, 129.9841967044819739 ) ) ;
#67588=CARTESIAN_POINT ( 'NONE',  ( 98.58519923211989067, -37.96229866499883343, 65.86384839950598291 ) ) ;
#67589=CARTESIAN_POINT ( 'NONE',  ( 90.44969454456416713, -55.86395651782489580, 219.5838068554169809 ) ) ;
#67590=CARTESIAN_POINT ( 'NONE',  ( 98.70151408295986073, -32.45115127476004346, 92.39396425827794701 ) ) ;
#67591=DIRECTION ( 'NONE',  ( 0.000000000000000000, 0.000000000000000000, -1.000000000000000000 ) ) ;
#67593=AXIS2_PLACEMENT_3D ( 'NONE', #54350, #27576, #89366 ) ;
#67594=CARTESIAN_POINT ( 'NONE',  ( 98.62975546523678361, -43.90627301359564427, 72.89943479972099283 ) ) ;
#67595=CARTESIAN_POINT ( 'NONE',  ( 97.31583286222694085, -39.30594983826361499, 182.5319644226825062 ) ) ;
#67597=CARTESIAN_POINT ( 'NONE',  ( 163.0664832912739826, -0.2185775633789972805, 335.9181252759120184 ) ) ;
#67599=DIRECTION ( 'NONE',  ( 6.524622321627019585E-16, 3.741823817616790462E-31, 1.000000000000000000 ) ) ;
#67600=ORIENTED_EDGE ( 'NONE', *, *, #33494, .F. ) ;
#67601=TOROIDAL_SURFACE ( 'NONE', #15361, 15.69999999999999929, 0.2999999999999999889 ) ;
#67604=EDGE_LOOP ( 'NONE', ( #15340, #50026, #5778, #15699 ) ) ;
#67605=CARTESIAN_POINT ( 'NONE',  ( 97.78144721833423603, -39.80378292816726571, 241.5813395616259811 ) ) ;
#67606=CARTESIAN_POINT ( 'NONE',  ( 108.7467188015556729, -25.78131109771034701, 140.9432443235299672 ) ) ;
#67607=CYLINDRICAL_SURFACE ( 'NONE', #85794, 11.57110091390439699 ) ;
#67608=CARTESIAN_POINT ( 'NONE',  ( 115.7815011880635723, -41.80502153836215484, 129.4062101450579689 ) ) ;
#67609=CARTESIAN_POINT ( 'NONE',  ( 103.2788791697577295, -47.11347506355160419, 93.28610146638693834 ) ) ;
#67610=DIRECTION ( 'NONE',  ( 0.7071067811865171526, 0.7071067811865779928, 7.071067811865164719E-16 ) ) ;
#67612=PLANE ( 'NONE',  #36590 ) ;
#67613=DIRECTION ( 'NONE',  ( 0.000000000000000000, 0.000000000000000000, 1.000000000000000000 ) ) ;
#67614=EDGE_CURVE ( 'NONE', #82741, #57074, #13490, .T. ) ;
#67618=CARTESIAN_POINT ( 'NONE',  ( 110.2841844748215578, -46.64581212076017636, 12.82705384733995402 ) ) ;
#67619=DIRECTION ( 'NONE',  ( 0.7071067811865503483, -0.7071067811865445751, 7.071067811865509846E-16 ) ) ;
#67624=CARTESIAN_POINT ( 'NONE',  ( 101.9719466847405158, -43.62131184885326007, 256.4924198280769474 ) ) ;
#67625=CARTESIAN_POINT ( 'NONE',  ( 97.37543214736597008, -39.21170434501622992, 101.5265497855716035 ) ) ;
#67626=CARTESIAN_POINT ( 'NONE',  ( 97.64212626138838402, -32.24102647341089778, 71.97276813305397525 ) ) ;
#67628=CARTESIAN_POINT ( 'NONE',  ( 112.8043457091679471, -45.48636447812791062, 178.0384824187679556 ) ) ;
#67631=ORIENTED_EDGE ( 'NONE', *, *, #59574, .T. ) ;
#67632=DIRECTION ( 'NONE',  ( 1.000000000000000000, 4.237773401492740281E-14, 0.000000000000000000 ) ) ;
#67633=EDGE_CURVE ( 'NONE', #32172, #21819, #33091, .T. ) ;
#67634=CARTESIAN_POINT ( 'NONE',  ( 113.2454986895939726, -28.75867293777369227, 65.55229194344597943 ) ) ;
#67635=CARTESIAN_POINT ( 'NONE',  ( 135.0807008692675311, -34.17316201338590531, 1.785258157648855093 ) ) ;
#67639=CARTESIAN_POINT ( 'NONE',  ( 97.53097521295029537, -31.04728477963730171, 130.9108633711489915 ) ) ;
#67640=ORIENTED_EDGE ( 'NONE', *, *, #28772, .T. ) ;
#67641=LINE ( 'NONE', #12235, #11741 ) ;
#67642=VECTOR ( 'NONE', #69953, 1000.000000000000000 ) ;
#67645=CARTESIAN_POINT ( 'NONE',  ( 98.30753419779586011, -41.72887550351619979, 76.73979194370691914 ) ) ;
#67649=AXIS2_PLACEMENT_3D ( 'NONE', #59798, #59359, #4416 ) ;
#67653=LINE ( 'NONE', #4535, #16738 ) ;
#67655=ORIENTED_EDGE ( 'NONE', *, *, #43727, .F. ) ;
#67656=EDGE_CURVE ( 'NONE', #19003, #12758, #89355, .T. ) ;
#67661=CARTESIAN_POINT ( 'NONE',  ( 117.0608945212226786, -38.08045314360793299, 158.7189586074293288 ) ) ;
#67663=CARTESIAN_POINT ( 'NONE',  ( 25.56670390244832092, -48.82844715994168183, 259.7178068554150059 ) ) ;
#67665=CARTESIAN_POINT ( 'NONE',  ( 97.31309884004055277, -38.96072181228549880, 181.5054471926127349 ) ) ;
#67667=ORIENTED_EDGE ( 'NONE', *, *, #62898, .T. ) ;
#67668=AXIS2_PLACEMENT_3D ( 'NONE', #50226, #14842, #57498 ) ;
#67669=CARTESIAN_POINT ( 'NONE',  ( 171.4664832912730219, 12.92155284005730387, 361.9756252759109998 ) ) ;
#67670=CARTESIAN_POINT ( 'NONE',  ( 116.1939227058877719, -40.33550099034467706, 189.5270538473389479 ) ) ;
#67671=CARTESIAN_POINT ( 'NONE',  ( 106.3178592879830973, -25.29212102876796919, 321.3196247216901043 ) ) ;
#67672=VERTEX_POINT ( 'NONE', #61459 ) ;
#67673=CARTESIAN_POINT ( 'NONE',  ( 97.35451824726690973, -37.88753622196094284, 37.42133956162496844 ) ) ;
#67674=CARTESIAN_POINT ( 'NONE',  ( 97.81168895331838087, -40.51742574516882200, 287.6356252759109680 ) ) ;
#67676=CARTESIAN_POINT ( 'NONE',  ( 97.81058606723590287, -40.51473118396398831, 22.63539394696516638 ) ) ;
#67677=EDGE_LOOP ( 'NONE', ( #23925, #53555 ) ) ;
#67680=VERTEX_POINT ( 'NONE', #66944 ) ;
#67681=EDGE_CURVE ( 'NONE', #47987, #38464, #54624, .T. ) ;
#67682=AXIS2_PLACEMENT_3D ( 'NONE', #33066, #54374, #32610 ) ;
#67683=CARTESIAN_POINT ( 'NONE',  ( 98.59150690531237160, -40.78546747480537249, 213.1253928297069535 ) ) ;
#67686=B_SPLINE_CURVE_WITH_KNOTS ( 'NONE', 3,
 ( #59331, #80254, #23943, #51620, #73413, #37570, #86614, #17999, #12998, #67947, #70534, #40229, #6183, #5278, #33871, #63262, #49614, #36001, #82050, #42346, #32973, #33426, #54286, #577, #42792, #28277 ),
 .UNSPECIFIED., .F., .F.,
 ( 4, 2, 2, 2, 2, 2, 2, 2, 2, 2, 2, 2, 4 ),
 ( 0.004694703549784783395, 0.005281399525416200988, 0.005868095501047617714, 0.006161443488863340388, 0.006454791476679063063, 0.006748139464494785737, 0.007041487452310508412, 0.007334835440126231086, 0.007628183427941953761, 0.007921531415757677302, 0.008214879403573398242, 0.008801575379204814101, 0.009388271354836229959 ),
 .UNSPECIFIED. ) ;
#67687=LINE ( 'NONE', #88148, #38790 ) ;
#67688=DIRECTION ( 'NONE',  ( -0.1858654557293118459, 0.9825752044329915114, 0.000000000000000000 ) ) ;
#67689=ORIENTED_EDGE ( 'NONE', *, *, #49774, .F. ) ;
#67691=CARTESIAN_POINT ( 'NONE',  ( 97.07185578696417849, -35.38051917764914123, 37.21882853886443598 ) ) ;
#67693=CARTESIAN_POINT ( 'NONE',  ( 117.4970320020027259, -36.54623693216564106, 288.8413395616252615 ) ) ;
#67694=ORIENTED_EDGE ( 'NONE', *, *, #79312, .F. ) ;
#67695=EDGE_LOOP ( 'NONE', ( #37704, #65755, #14403, #47665 ) ) ;
#67696=CARTESIAN_POINT ( 'NONE',  ( 113.8227294809096435, -41.31015272151215356, 271.1709475124484925 ) ) ;
#67697=PLANE ( 'NONE',  #994 ) ;
#67698=CARTESIAN_POINT ( 'NONE',  ( 98.56701561008806323, -30.78824967682747271, 160.8289586092449497 ) ) ;
#67700=PLANE ( 'NONE',  #9921 ) ;
#67701=FACE_OUTER_BOUND ( 'NONE', #27233, .T. ) ;
#67703=CARTESIAN_POINT ( 'NONE',  ( 118.1276453766531915, -32.34061975111649190, 245.1270538473389706 ) ) ;
#67704=DIRECTION ( 'NONE',  ( 1.000000000000000000, 0.000000000000000000, 0.000000000000000000 ) ) ;
#67706=EDGE_CURVE ( 'NONE', #4391, #89126, #31970, .T. ) ;
#67708=CARTESIAN_POINT ( 'NONE',  ( 117.4143231396408851, -32.71451144048268844, 90.10895860924395606 ) ) ;
#67710=CARTESIAN_POINT ( 'NONE',  ( 87.06648329127423835, -46.72944715994107412, 14.82207188531761055 ) ) ;
#67712=EDGE_LOOP ( 'NONE', ( #72597, #52312 ) ) ;
#67713=ORIENTED_EDGE ( 'NONE', *, *, #78062, .F. ) ;
#67715=FACE_OUTER_BOUND ( 'NONE', #21030, .T. ) ;
#67716=DIRECTION ( 'NONE',  ( 0.000000000000000000, 0.000000000000000000, -1.000000000000000000 ) ) ;
#67717=CARTESIAN_POINT ( 'NONE',  ( 98.92690986002996567, -36.11615286530263091, 144.0852332267349709 ) ) ;
#67718=CARTESIAN_POINT ( 'NONE',  ( 106.9401787849546537, -47.80506239865356122, 228.5794347997199907 ) ) ;
#67719=CARTESIAN_POINT ( 'NONE',  ( 97.83891474888318385, -40.58336863229884273, 57.64130287487746074 ) ) ;
#67722=VECTOR ( 'NONE', #68184, 999.9999999999998863 ) ;
#67723=CARTESIAN_POINT ( 'NONE',  ( 136.7280559526967636, -37.42731094490868315, 2.974216770160591494 ) ) ;
#67724=ORIENTED_EDGE ( 'NONE', *, *, #22923, .F. ) ;
#67725=EDGE_LOOP ( 'NONE', ( #11968, #83641 ) ) ;
#67729=ORIENTED_EDGE ( 'NONE', *, *, #66907, .T. ) ;
#67734=ADVANCED_FACE ( 'NONE', ( #11991 ), #75562, .F. ) ;
#67735=CARTESIAN_POINT ( 'NONE',  ( 115.5545030166667146, -32.01519760825960503, 178.6524198280769724 ) ) ;
#67736=CARTESIAN_POINT ( 'NONE',  ( 111.9494872540039694, -27.46861899264377982, 59.68991099019693536 ) ) ;
#67737=ORIENTED_EDGE ( 'NONE', *, *, #16583, .T. ) ;
#67739=EDGE_LOOP ( 'NONE', ( #72876, #14774, #61373, #72230 ) ) ;
#67742=EDGE_CURVE ( 'NONE', #8195, #86716, #6077, .T. ) ;
#67743=ORIENTED_EDGE ( 'NONE', *, *, #10669, .T. ) ;
#67744=DIRECTION ( 'NONE',  ( -0.9254794337955620787, -0.3787978585227822492, 0.000000000000000000 ) ) ;
#67745=EDGE_CURVE ( 'NONE', #54700, #75621, #53281, .T. ) ;
#67746=ORIENTED_EDGE ( 'NONE', *, *, #42492, .T. ) ;
#67747=CARTESIAN_POINT ( 'NONE',  ( 110.6340492874757473, -27.31029447320501191, 165.7874528756242682 ) ) ;
#67749=CARTESIAN_POINT ( 'NONE',  ( 110.8556210833095435, -45.98376701427152113, 132.8857240236057748 ) ) ;
#67752=CARTESIAN_POINT ( 'NONE',  ( 112.1280348295452001, -26.87672238358117127, 19.71086337114896736 ) ) ;
#67753=CARTESIAN_POINT ( 'NONE',  ( 95.30017103329034001, -34.95040006919153086, 67.20705384733894050 ) ) ;
#67754=CARTESIAN_POINT ( 'NONE',  ( 90.44969454456439450, -16.81243780205712568, 249.5838068554174924 ) ) ;
#67758=EDGE_CURVE ( 'NONE', #52712, #77239, #61020, .T. ) ;
#67759=LINE ( 'NONE', #74570, #14085 ) ;
#67761=ORIENTED_EDGE ( 'NONE', *, *, #76718, .T. ) ;
#67762=CARTESIAN_POINT ( 'NONE',  ( 117.5318583147471401, -37.01683481156648980, 43.80419670448293346 ) ) ;
#67763=CARTESIAN_POINT ( 'NONE',  ( 117.3749687695755171, -38.63058443890392368, 84.68133956162593279 ) ) ;
#67766=DIRECTION ( 'NONE',  ( 0.7071067811578790607, 0.7071067812152160847, 0.000000000000000000 ) ) ;
#67767=CARTESIAN_POINT ( 'NONE',  ( 31.71315051185499811, -33.70561438052090608, 313.9678068554150059 ) ) ;
#67768=CARTESIAN_POINT ( 'NONE',  ( 121.5762960060074960, -43.47224590996763993, 9.125625275910984158 ) ) ;
#67770=AXIS2_PLACEMENT_3D ( 'NONE', #77883, #2026, #15658 ) ;
#67771=DIRECTION ( 'NONE',  ( 0.000000000000000000, 0.000000000000000000, -1.000000000000000000 ) ) ;
#67773=CARTESIAN_POINT ( 'NONE',  ( 96.71749658230667990, -40.79275330125899046, 92.62419670448196030 ) ) ;
#67776=CARTESIAN_POINT ( 'NONE',  ( 104.3301552612371523, -26.04411461992211230, 241.2880062282919482 ) ) ;
#67777=CARTESIAN_POINT ( 'NONE',  ( 109.6421070598780290, -46.48033137427756856, 253.7835689616865125 ) ) ;
#67778=CARTESIAN_POINT ( 'NONE',  ( 107.0664832912739968, -18.82844715994099971, 168.9256252759119832 ) ) ;
#67780=CARTESIAN_POINT ( 'NONE',  ( 179.1667039024460166, -28.27351298637280408, 193.9678068554150059 ) ) ;
#67781=CARTESIAN_POINT ( 'NONE',  ( 91.06648329127500574, -36.72944715993925513, 9.125625275910953960 ) ) ;
#67782=LINE ( 'NONE', #4667, #58741 ) ;
#67783=AXIS2_PLACEMENT_3D ( 'NONE', #22454, #649, #49233 ) ;
#67785=CARTESIAN_POINT ( 'NONE',  ( 116.0678243078411498, -40.55558035091543445, 168.5070538473399608 ) ) ;
#67786=EDGE_LOOP ( 'NONE', ( #22821, #60643, #73871, #38588 ) ) ;
#67788=EDGE_CURVE ( 'NONE', #30574, #16547, #4277, .T. ) ;
#67789=CARTESIAN_POINT ( 'NONE',  ( 100.7916921807572379, -44.60965664144636378, 118.4730118773259733 ) ) ;
#67790=CIRCLE ( 'NONE', #8348, 2.116999999999993776 ) ;
#67791=CARTESIAN_POINT ( 'NONE',  ( 89.06648329127401098, -18.82844715994099971, 17.92562527591199739 ) ) ;
#67792=CARTESIAN_POINT ( 'NONE',  ( 115.9511604134431195, -42.07746527072326614, 274.3832443235294249 ) ) ;
#67793=CARTESIAN_POINT ( 'NONE',  ( 182.4202572930400095, -33.70561438051981185, 193.9678068554150059 ) ) ;
#67794=DIRECTION ( 'NONE',  ( -1.000000000000000078E-15, 0.000000000000000000, -1.000000000000000000 ) ) ;
#67795=ADVANCED_FACE ( 'NONE', ( #59664, #38783 ), #5630, .F. ) ;
#67796=DIRECTION ( 'NONE',  ( -0.9254794337955620787, -0.3787978585227822492, 0.000000000000000000 ) ) ;
#67797=CARTESIAN_POINT ( 'NONE',  ( 177.8371591254545194, -47.82818131005477369, 180.4678068554150343 ) ) ;
#67798=LINE ( 'NONE', #73257, #72488 ) ;
#67799=CARTESIAN_POINT ( 'NONE',  ( 95.60734603896362671, -36.72944715994100306, 293.2242906452868851 ) ) ;
#67800=CARTESIAN_POINT ( 'NONE',  ( 116.7748712849171966, -40.56502120445013304, 193.5270538473389479 ) ) ;
#67801=CARTESIAN_POINT ( 'NONE',  ( 51.06670390244772761, -33.35206098992665602, 237.4678068554150059 ) ) ;
#67803=ORIENTED_EDGE ( 'NONE', *, *, #66563, .F. ) ;
#67804=CARTESIAN_POINT ( 'NONE',  ( 31.89136050872298966, -31.76306994223740432, 313.9678068554150059 ) ) ;
#67805=DIRECTION ( 'NONE',  ( -0.9834602067153815907, -0.1811243269341220596, 0.000000000000000000 ) ) ;
#67808=VECTOR ( 'NONE', #72467, 1000.000000000000000 ) ;
#67809=LINE ( 'NONE', #5597, #61536 ) ;
#67810=EDGE_LOOP ( 'NONE', ( #5745, #49326, #29101, #1570 ) ) ;
#67811=EDGE_CURVE ( 'NONE', #2099, #13645, #52853, .T. ) ;
#67813=CARTESIAN_POINT ( 'NONE',  ( 97.40186843559010299, -40.63869902605510731, 206.6327681330539860 ) ) ;
#67814=CARTESIAN_POINT ( 'NONE',  ( 136.8164806451553659, -36.72944715939129168, 6.749772901088312516 ) ) ;
#67818=CARTESIAN_POINT ( 'NONE',  ( 105.7148838627258556, -46.72376843215531750, 163.4689113525691084 ) ) ;
#67819=CARTESIAN_POINT ( 'NONE',  ( 113.9764273654521674, -32.38405892540742315, 32.09094751244895605 ) ) ;
#67820=CARTESIAN_POINT ( 'NONE',  ( 103.1665349694895895, -27.03781871365087142, 126.3813395616259783 ) ) ;
#67821=ORIENTED_CLOSED_SHELL ( 'NONE', *, #83693, .F. );
#67822=LINE ( 'NONE', #74638, #88541 ) ;
#67826=CARTESIAN_POINT ( 'NONE',  ( 82.41409441626767318, -17.29397280664446868, 7.245803660798958212 ) ) ;
#67827=ORIENTED_EDGE ( 'NONE', *, *, #24979, .T. ) ;
#67829=CIRCLE ( 'NONE', #82375, 2.124999999999994227 ) ;
#67830=AXIS2_PLACEMENT_3D ( 'NONE', #65941, #10543, #86415 ) ;
#67833=VERTEX_POINT ( 'NONE', #12891 ) ;
#67835=CARTESIAN_POINT ( 'NONE',  ( 105.1764056618614944, -45.05913732685939976, 71.82099125664798578 ) ) ;
#67836=CARTESIAN_POINT ( 'NONE',  ( 112.4658351597014843, -45.71473303307890035, 238.0070538473389377 ) ) ;
#67838=CARTESIAN_POINT ( 'NONE',  ( 96.64068249873260186, -36.21262657180042766, 171.2870538473399620 ) ) ;
#67839=DIRECTION ( 'NONE',  ( 1.000000000000000078E-15, 1.000000000000000083E-30, -1.000000000000000000 ) ) ;
#67840=CARTESIAN_POINT ( 'NONE',  ( 111.7390528236686436, -27.41013440965690862, 275.7070538473395800 ) ) ;
#67842=EDGE_CURVE ( 'NONE', #85483, #30005, #83816, .T. ) ;
#67843=CARTESIAN_POINT ( 'NONE',  ( 142.8696205427243626, 0.6543191929522240713, 540.9756252759101471 ) ) ;
#67848=VECTOR ( 'NONE', #12553, 1000.000000000000000 ) ;
#67849=VECTOR ( 'NONE', #48206, 999.9999999999998863 ) ;
#67850=CARTESIAN_POINT ( 'NONE',  ( 97.83900843593762886, -40.58359296468890420, 111.6413228214579050 ) ) ;
#67851=CARTESIAN_POINT ( 'NONE',  ( 107.2500105196458549, -24.83007258495691616, 230.0641967044819580 ) ) ;
#67852=ORIENTED_EDGE ( 'NONE', *, *, #36902, .F. ) ;
#67853=CARTESIAN_POINT ( 'NONE',  ( 116.3775870818408151, -41.41883695635522145, 203.4556252759109611 ) ) ;
#67854=FACE_OUTER_BOUND ( 'NONE', #50275, .T. ) ;
#67856=CARTESIAN_POINT ( 'NONE',  ( 62.56670390244669022, -48.82844715994099971, 129.9678068554150911 ) ) ;
#67857=CARTESIAN_POINT ( 'NONE',  ( 98.05617819296176663, -37.43095703503473004, 277.6356252759115932 ) ) ;
#67858=DIRECTION ( 'NONE',  ( 0.000000000000000000, 1.000000000000000000, 0.000000000000000000 ) ) ;
#67859=CARTESIAN_POINT ( 'NONE',  ( -18.39335205926253280, -13.32818131006344231, 237.4678068554150059 ) ) ;
#67861=CARTESIAN_POINT ( 'NONE',  ( 25.56670390244797275, -67.87844715994100397, 293.2178068554150627 ) ) ;
#67862=ADVANCED_FACE ( 'NONE', ( #85427 ), #23202, .T. ) ;
#67863=CARTESIAN_POINT ( 'NONE',  ( 107.0664832912739968, -36.72944715994100306, 0.4256252759109701023 ) ) ;
#67864=EDGE_CURVE ( 'NONE', #84928, #31634, #1392, .T. ) ;
#67865=CARTESIAN_POINT ( 'NONE',  ( 98.34816318742551289, -31.65962802882244631, 40.90603857251151965 ) ) ;
#67870=CARTESIAN_POINT ( 'NONE',  ( 113.8136090879065563, -26.95650955708257257, 239.5956252759109759 ) ) ;
#67871=CARTESIAN_POINT ( 'NONE',  ( 116.9217636815068033, -33.22305568060546932, 110.0984824187679578 ) ) ;
#67872=CARTESIAN_POINT ( 'NONE',  ( 105.8886828556765494, -47.16740550586902003, 278.4870538473396664 ) ) ;
#67876=CARTESIAN_POINT ( 'NONE',  ( 41.56648329127499153, -32.07844715994070839, 314.1756252759120116 ) ) ;
#67880=CARTESIAN_POINT ( 'NONE',  ( 132.4277392773811073, -20.94013506380670719, 2.060080721657580494 ) ) ;
#67881=VERTEX_POINT ( 'NONE', #77695 ) ;
#67882=VERTEX_POINT ( 'NONE', #42692 ) ;
#67883=CARTESIAN_POINT ( 'NONE',  ( 100.8033404080456705, -29.31000718268690619, 150.0581341137909703 ) ) ;
#67887=CARTESIAN_POINT ( 'NONE',  ( 113.3182355088850386, -45.04474967211692160, 139.0899109901969553 ) ) ;
#67888=DIRECTION ( 'NONE',  ( 1.000000000000000078E-15, 0.000000000000000000, 1.000000000000000000 ) ) ;
#67890=DIRECTION ( 'NONE',  ( 1.000000000000000078E-15, 0.000000000000000000, -1.000000000000000000 ) ) ;
#67892=VECTOR ( 'NONE', #61248, 1000.000000000000000 ) ;
#67893=CARTESIAN_POINT ( 'NONE',  ( 118.0115280580378396, -34.77548253539073642, 48.96705384733996169 ) ) ;
#67894=EDGE_LOOP ( 'NONE', ( #88792, #43454, #22431, #6836 ) ) ;
#67896=ORIENTED_EDGE ( 'NONE', *, *, #18787, .F. ) ;
#67897=VECTOR ( 'NONE', #83311, 1000.000000000000000 ) ;
#67898=CIRCLE ( 'NONE', #89705, 4.749999999999976907 ) ;
#67899=DIRECTION ( 'NONE',  ( 9.351236661543306751E-17, -3.725950533538267725E-29, -1.000000000000000000 ) ) ;
#67900=CARTESIAN_POINT ( 'NONE',  ( 105.4244293397739085, -47.72525222749315787, 143.4584824187679715 ) ) ;
#67902=PLANE ( 'NONE',  #78477 ) ;
#67904=EDGE_CURVE ( 'NONE', #60678, #20709, #38856, .T. ) ;
#67905=CARTESIAN_POINT ( 'NONE',  ( 193.0374249753375011, -23.42844715993436111, 237.4678068554150059 ) ) ;
#67906=AXIS2_PLACEMENT_3D ( 'NONE', #40089, #18760, #67805 ) ;
#67908=CARTESIAN_POINT ( 'NONE',  ( 117.0719695477731790, -35.46309620022125841, 179.9272431197764206 ) ) ;
#67909=CARTESIAN_POINT ( 'NONE',  ( 112.7897778137182030, -47.07797880090547693, 102.9784824187679817 ) ) ;
#67910=ORIENTED_EDGE ( 'NONE', *, *, #75738, .F. ) ;
#67911=ORIENTED_EDGE ( 'NONE', *, *, #55788, .F. ) ;
#67915=CIRCLE ( 'NONE', #85330, 2.500000000000002220 ) ;
#67916=VECTOR ( 'NONE', #23644, 1000.000000000000000 ) ;
#67918=CARTESIAN_POINT ( 'NONE',  ( 111.8340120402796032, -28.76913304608537914, 202.4652332267339716 ) ) ;
#67919=EDGE_CURVE ( 'NONE', #10270, #10148, #21842, .T. ) ;
#67921=VERTEX_POINT ( 'NONE', #58132 ) ;
#67925=CARTESIAN_POINT ( 'NONE',  ( 135.3099588813078924, -21.18301917768702225, 1.868341932368159153 ) ) ;
#67926=VERTEX_POINT ( 'NONE', #84970 ) ;
#67928=CARTESIAN_POINT ( 'NONE',  ( 77.49051321912324397, -19.69637952318584340, 6.988870342679232017 ) ) ;
#67929=ADVANCED_FACE ( 'NONE', ( #70433 ), #64067, .F. ) ;
#67930=CARTESIAN_POINT ( 'NONE',  ( 113.0661788413732580, -30.20779614827405624, 195.9158690201829529 ) ) ;
#67932=CONICAL_SURFACE ( 'NONE', #70878, 17.36499999999999844, 0.7853981633974490562 ) ;
#67933=DIRECTION ( 'NONE',  ( -0.000000000000000000, 1.000000000000000000, 0.000000000000000000 ) ) ;
#67936=ORIENTED_EDGE ( 'NONE', *, *, #22542, .T. ) ;
#67937=ORIENTED_EDGE ( 'NONE', *, *, #80627, .F. ) ;
#67938=CARTESIAN_POINT ( 'NONE',  ( 41.56648329127399677, 0.2215528400590013880, 141.0426252759120018 ) ) ;
#67939=ORIENTED_EDGE ( 'NONE', *, *, #16583, .F. ) ;
#67940=EDGE_LOOP ( 'NONE', ( #53111, #70984, #23419, #44029 ) ) ;
#67942=CARTESIAN_POINT ( 'NONE',  ( 98.49961498605385657, -35.50075171889626091, 224.0433284648299548 ) ) ;
#67943=CARTESIAN_POINT ( 'NONE',  ( 112.5258771334048475, -27.82206915948941273, 94.63848241876793566 ) ) ;
#67944=CARTESIAN_POINT ( 'NONE',  ( 96.67837842349533162, -37.29153504031420141, 76.36991099019697060 ) ) ;
#67945=CARTESIAN_POINT ( 'NONE',  ( 115.0636728013147945, -41.29441372593446857, 249.5838068554169809 ) ) ;
#67947=CARTESIAN_POINT ( 'NONE',  ( 108.0188260930178217, -25.30989513122313994, 322.4896988899195662 ) ) ;
#67948=CARTESIAN_POINT ( 'NONE',  ( 99.28859025714638165, -29.78777103691475858, 186.7470538473389752 ) ) ;
#67949=EDGE_CURVE ( 'NONE', #75765, #21614, #15918, .T. ) ;
#67956=CARTESIAN_POINT ( 'NONE',  ( 152.0368932755770288, -23.42844715993588522, 300.4678068554149490 ) ) ;
#67957=ORIENTED_EDGE ( 'NONE', *, *, #89810, .F. ) ;
#67958=VECTOR ( 'NONE', #33591, 1000.000000000000000 ) ;
#67959=CARTESIAN_POINT ( 'NONE',  ( 97.79627051079565092, -40.47954843556247084, 137.6323705464966167 ) ) ;
#67961=CARTESIAN_POINT ( 'NONE',  ( 109.6430121110707319, -46.48008674055821388, 177.7814586078273464 ) ) ;
#67962=CARTESIAN_POINT ( 'NONE',  ( 110.1579966911880888, -46.68583080861444756, 97.81562527591097478 ) ) ;
#67964=CARTESIAN_POINT ( 'NONE',  ( 136.8000579002614074, -36.42904715602825405, 6.774297104451916240 ) ) ;
#67966=CARTESIAN_POINT ( 'NONE',  ( 113.1782937664330859, -44.75186859636650638, 144.0939586087628754 ) ) ;
#67967=DIRECTION ( 'NONE',  ( 0.000000000000000000, 1.000000000000000000, 0.000000000000000000 ) ) ;
#67968=CARTESIAN_POINT ( 'NONE',  ( 118.0279888096067396, -35.50094427011356402, 229.9032443235299468 ) ) ;
#67970=DIRECTION ( 'NONE',  ( 3.339108161477000479E-13, -1.000000000000000000, 6.848429599184487071E-29 ) ) ;
#67971=ORIENTED_EDGE ( 'NONE', *, *, #36547, .F. ) ;
#67972=DIRECTION ( 'NONE',  ( 1.000000000000000078E-15, -1.000000000000000083E-30, -1.000000000000000000 ) ) ;
#67973=ADVANCED_FACE ( 'NONE', ( #71334 ), #71774, .F. ) ;
#67974=AXIS2_PLACEMENT_3D ( 'NONE', #69277, #27483, #83359 ) ;
#67975=CARTESIAN_POINT ( 'NONE',  ( 142.8838050580815775, -82.11588141944044139, 394.9756252759102040 ) ) ;
#67977=CARTESIAN_POINT ( 'NONE',  ( 50.87649884952377022, -33.54226604284969682, 193.9678068554150911 ) ) ;
#67978=ADVANCED_FACE ( 'NONE', ( #64953 ), #23634, .T. ) ;
#67980=DIRECTION ( 'NONE',  ( 1.000000000000000078E-15, -1.000000000000000083E-30, -1.000000000000000000 ) ) ;
#67981=CARTESIAN_POINT ( 'NONE',  ( 104.3993058286337146, -25.95452033834810024, 240.2575300378159682 ) ) ;
#67984=CARTESIAN_POINT ( 'NONE',  ( 112.1172674779030558, -26.89768192312349271, 15.71086337114896381 ) ) ;
#67985=CARTESIAN_POINT ( 'NONE',  ( 108.3715344132687051, -47.75189438633907457, 158.6822919425779617 ) ) ;
#67987=CARTESIAN_POINT ( 'NONE',  ( 107.0667039024480260, -36.72944715994099596, 199.5838068554169809 ) ) ;
#67988=CARTESIAN_POINT ( 'NONE',  ( 97.60785222787119153, -39.98231739658664452, 102.5900457468837743 ) ) ;
#67990=DIRECTION ( 'NONE',  ( 0.000000000000000000, 0.000000000000000000, 1.000000000000000000 ) ) ;
#67991=PLANE ( 'NONE',  #36489 ) ;
#67992=CYLINDRICAL_SURFACE ( 'NONE', #80132, 13.99999999999999822 ) ;
#67993=ORIENTED_EDGE ( 'NONE', *, *, #67745, .F. ) ;
#67994=VERTEX_POINT ( 'NONE', #84070 ) ;
#67995=ORIENTED_EDGE ( 'NONE', *, *, #4635, .F. ) ;
#67996=CIRCLE ( 'NONE', #31736, 2.999999999999947153 ) ;
#67999=CARTESIAN_POINT ( 'NONE',  ( 96.85498737197835339, -38.89503640450122646, 27.49276813305395706 ) ) ;
#68000=CARTESIAN_POINT ( 'NONE',  ( 29.56670390244797630, -67.87844715994100397, 10.91780685541479734 ) ) ;
#68002=DIRECTION ( 'NONE',  ( 0.000000000000000000, 0.000000000000000000, -1.000000000000000000 ) ) ;
#68003=CARTESIAN_POINT ( 'NONE',  ( 53.35959712126192755, -48.62134037875358672, 180.4678068554151196 ) ) ;
#68004=CARTESIAN_POINT ( 'NONE',  ( 110.0705912124663968, -28.18614534367760172, 254.2419436376007695 ) ) ;
#68006=VECTOR ( 'NONE', #17635, 1000.000000000000000 ) ;
#68007=ORIENTED_EDGE ( 'NONE', *, *, #8575, .F. ) ;
#68008=ORIENTED_EDGE ( 'NONE', *, *, #40752, .T. ) ;
#68009=DIRECTION ( 'NONE',  ( 1.000000000000000000, 0.000000000000000000, 0.000000000000000000 ) ) ;
#68010=CARTESIAN_POINT ( 'NONE',  ( 97.81413224952068219, -40.51639846094042952, 101.6360726122380100 ) ) ;
#68011=CARTESIAN_POINT ( 'NONE',  ( 20.56670390244740076, -48.82844715994099971, 300.4678068554149490 ) ) ;
#68013=CARTESIAN_POINT ( 'NONE',  ( 99.19755098026091389, -30.44051964901187191, 42.22158330589692810 ) ) ;
#68014=CYLINDRICAL_SURFACE ( 'NONE', #89394, 0.9999999999999800160 ) ;
#68015=CYLINDRICAL_SURFACE ( 'NONE', #21594, 2.517499999999998739 ) ;
#68016=CARTESIAN_POINT ( 'NONE',  ( 106.8506556707805260, -46.50783423188027399, 272.5584824187685626 ) ) ;
#68019=VECTOR ( 'NONE', #21969, 1000.000000000000114 ) ;
#68022=CARTESIAN_POINT ( 'NONE',  ( 113.2960346059783774, -42.04690695427109404, 61.08237608387695161 ) ) ;
#68024=CIRCLE ( 'NONE', #43371, 2.517500000000005844 ) ;
#68025=ADVANCED_FACE ( 'NONE', ( #15018 ), #11772, .T. ) ;
#68026=CARTESIAN_POINT ( 'NONE',  ( 136.3178028891481119, -17.14744377622660210, 7.339349742399202903 ) ) ;
#68028=CARTESIAN_POINT ( 'NONE',  ( 101.9935804828795369, -45.44604673876975909, 193.1563667090017020 ) ) ;
#68029=VERTEX_POINT ( 'NONE', #52618 ) ;
#68032=DIRECTION ( 'NONE',  ( -4.237773401492740281E-14, 1.000000000000000000, 0.000000000000000000 ) ) ;
#68034=CARTESIAN_POINT ( 'NONE',  ( 105.7204000585623191, -24.95538135984382677, 160.1670538473389627 ) ) ;
#68036=CARTESIAN_POINT ( 'NONE',  ( 104.5891003629744631, -45.44008686965874944, 66.79051506617194889 ) ) ;
#68039=CARTESIAN_POINT ( 'NONE',  ( 97.81373435033219721, -40.51654435448209313, 87.63515866765291662 ) ) ;
#68040=CARTESIAN_POINT ( 'NONE',  ( 115.4437480007128443, -33.74891607059462473, 110.5301547344689794 ) ) ;
#68041=EDGE_CURVE ( 'NONE', #87716, #50621, #10871, .T. ) ;
#68043=VECTOR ( 'NONE', #19713, 1000.000000000000000 ) ;
#68044=LINE ( 'NONE', #33518, #71636 ) ;
#68045=CARTESIAN_POINT ( 'NONE',  ( 100.9283148882350787, -46.89532829952024429, 48.14419670448194211 ) ) ;
#68047=EDGE_CURVE ( 'NONE', #64058, #35419, #16806, .T. ) ;
#68048=PLANE ( 'NONE',  #12599 ) ;
#68049=ORIENTED_EDGE ( 'NONE', *, *, #28568, .T. ) ;
#68051=ORIENTED_EDGE ( 'NONE', *, *, #23826, .F. ) ;
#68052=ORIENTED_EDGE ( 'NONE', *, *, #45860, .T. ) ;
#68054=AXIS2_PLACEMENT_3D ( 'NONE', #9988, #84525, #64950 ) ;
#68056=VERTEX_POINT ( 'NONE', #39016 ) ;
#68057=CARTESIAN_POINT ( 'NONE',  ( 101.9853755998761073, -45.08682593082395584, 247.1413395616259550 ) ) ;
#68058=CARTESIAN_POINT ( 'NONE',  ( 114.2683966348991760, -44.29710505712337465, 154.1813395616249807 ) ) ;
#68060=DIRECTION ( 'NONE',  ( 0.000000000000000000, -1.000000000000000000, 0.000000000000000000 ) ) ;
#68061=CARTESIAN_POINT ( 'NONE',  ( 113.4153195569882087, -27.68144967124534261, 80.57753003781597556 ) ) ;
#68062=EDGE_CURVE ( 'NONE', #68436, #88057, #80965, .T. ) ;
#68063=CARTESIAN_POINT ( 'NONE',  ( 99.09675058860776176, -30.54904317927480761, 96.80150208561718728 ) ) ;
#68065=CARTESIAN_POINT ( 'NONE',  ( 52.65249034007746332, -49.32844715994061602, 180.4678068554151196 ) ) ;
#68066=CARTESIAN_POINT ( 'NONE',  ( 99.04409650882432459, -42.84130985989413176, 157.8437691819532063 ) ) ;
#68067=VECTOR ( 'NONE', #5240, 1000.000000000000114 ) ;
#68070=PLANE ( 'NONE',  #20322 ) ;
#68071=CARTESIAN_POINT ( 'NONE',  ( 99.39760893136102027, -29.69972230079146769, 275.7356252759109907 ) ) ;
#68073=CYLINDRICAL_SURFACE ( 'NONE', #18773, 2.500000000000002220 ) ;
#68074=CARTESIAN_POINT ( 'NONE',  ( 184.5667039024480118, -67.87844715994100397, 300.9178068554150514 ) ) ;
#68075=CARTESIAN_POINT ( 'NONE',  ( 103.8089036935402021, -45.87596577953674881, 251.7267055423626516 ) ) ;
#68076=CARTESIAN_POINT ( 'NONE',  ( 114.8007373875590531, -30.34631565586484925, 99.37626092783206389 ) ) ;
#68077=CARTESIAN_POINT ( 'NONE',  ( 95.80265872640110558, -40.33145541733360773, 127.5727681330539554 ) ) ;
#68078=DIRECTION ( 'NONE',  ( 0.000000000000000000, 0.000000000000000000, 1.000000000000000000 ) ) ;
#68079=CARTESIAN_POINT ( 'NONE',  ( 98.13053560861905567, -31.27458647820624549, 170.8899109901960003 ) ) ;
#68080=ORIENTED_EDGE ( 'NONE', *, *, #5088, .T. ) ;
#68081=DIRECTION ( 'NONE',  ( 0.000000000000000000, 0.000000000000000000, 1.000000000000000000 ) ) ;
#68082=ORIENTED_EDGE ( 'NONE', *, *, #14668, .F. ) ;
#68084=CARTESIAN_POINT ( 'NONE',  ( 109.7248659029457798, -27.00080517437059768, 65.86479194409724869 ) ) ;
#68086=ORIENTED_EDGE ( 'NONE', *, *, #35303, .T. ) ;
#68087=EDGE_CURVE ( 'NONE', #58498, #61827, #65826, .T. ) ;
#68088=AXIS2_PLACEMENT_3D ( 'NONE', #71795, #59025, #58582 ) ;
#68089=CARTESIAN_POINT ( 'NONE',  ( 105.8017600360789174, -26.72373307582276780, 61.17738641589737369 ) ) ;
#68090=CARTESIAN_POINT ( 'NONE',  ( 108.6554276816787734, -25.75039326353942926, 149.9737205140059473 ) ) ;
#68091=ORIENTED_EDGE ( 'NONE', *, *, #26740, .T. ) ;
#68093=CARTESIAN_POINT ( 'NONE',  ( 80.06648329127402519, -46.42944715994105565, 10.42562527591094401 ) ) ;
#68096=CARTESIAN_POINT ( 'NONE',  ( 172.5664832912740110, -9.303447159940999356, 21.04262527591200183 ) ) ;
#68097=CIRCLE ( 'NONE', #72438, 4.750000000000004441 ) ;
#68098=CARTESIAN_POINT ( 'NONE',  ( 172.5667039024482960, -42.82844715993499563, 180.4678068554150059 ) ) ;
#68099=EDGE_LOOP ( 'NONE', ( #67585, #58198, #28088, #57964, #27369 ) ) ;
#68102=DIRECTION ( 'NONE',  ( -0.000000000000000000, 1.000000000000000000, 0.000000000000000000 ) ) ;
#68103=VERTEX_POINT ( 'NONE', #31757 ) ;
#68104=ORIENTED_EDGE ( 'NONE', *, *, #53700, .T. ) ;
#68105=CIRCLE ( 'NONE', #62318, 3.000000000000002665 ) ;
#68107=CARTESIAN_POINT ( 'NONE',  ( 21.03715912545823130, -47.82818131006186491, 313.9678068554150059 ) ) ;
#68109=CARTESIAN_POINT ( 'NONE',  ( 116.8171228686926639, -34.15291832592715338, 159.0314586087905582 ) ) ;
#68112=CARTESIAN_POINT ( 'NONE',  ( 194.0371591254582313, -46.82818131005407736, 300.4678068554149490 ) ) ;
#68115=ORIENTED_EDGE ( 'NONE', *, *, #14038, .T. ) ;
#68116=DIRECTION ( 'NONE',  ( 0.9242245927363033076, 0.3818493186865917766, 0.000000000000000000 ) ) ;
#68118=CARTESIAN_POINT ( 'NONE',  ( 99.06478422775796844, -31.10483629442216014, 201.8384824187669437 ) ) ;
#68120=CARTESIAN_POINT ( 'NONE',  ( 116.3186249068867539, -32.94868901193379429, 250.1356252759109395 ) ) ;
#68121=ORIENTED_EDGE ( 'NONE', *, *, #87045, .T. ) ;
#68122=CARTESIAN_POINT ( 'NONE',  ( 96.71749658230667990, -40.79275330125899046, 92.62419670448196030 ) ) ;
#68123=CARTESIAN_POINT ( 'NONE',  ( 116.3427928135287885, -40.59072558610812820, 53.51233718776536108 ) ) ;
#68124=DIRECTION ( 'NONE',  ( 0.000000000000000000, 0.000000000000000000, -1.000000000000000000 ) ) ;
#68125=CARTESIAN_POINT ( 'NONE',  ( 182.2300522401149863, -33.89581943344511217, -5.074374724088000832 ) ) ;
#68127=FACE_OUTER_BOUND ( 'NONE', #24831, .T. ) ;
#68132=CARTESIAN_POINT ( 'NONE',  ( 102.4628740603001233, -44.30143901548009211, 243.5730118773259676 ) ) ;
#68136=EDGE_CURVE ( 'NONE', #54444, #35904, #24352, .T. ) ;
#68137=CARTESIAN_POINT ( 'NONE',  ( 108.3334480117198666, -46.73485936529269935, 153.6772919359582943 ) ) ;
#68140=AXIS2_PLACEMENT_3D ( 'NONE', #25113, #89143, #47778 ) ;
#68141=CYLINDRICAL_SURFACE ( 'NONE', #81249, 2.517500000000000071 ) ;
#68142=EDGE_CURVE ( 'NONE', #74286, #11288, #88224, .T. ) ;
#68143=CARTESIAN_POINT ( 'NONE',  ( 71.25529199314597406, -79.12815651470191369, 361.9756252759101471 ) ) ;
#68144=EDGE_LOOP ( 'NONE', ( #84652, #8636, #42886, #31675, #12253, #7853, #63126, #60423, #40388 ) ) ;
#68145=CARTESIAN_POINT ( 'NONE',  ( 118.3173389373707920, -33.08695204176926552, 284.0756252759109657 ) ) ;
#68147=CARTESIAN_POINT ( 'NONE',  ( 110.2461554203946292, -29.21150786992351911, 242.5766617981629452 ) ) ;
#68148=VECTOR ( 'NONE', #33355, 1000.000000000000000 ) ;
#68151=CARTESIAN_POINT ( 'NONE',  ( 109.0694692412632492, -27.15596902575777349, 139.9127681330539872 ) ) ;
#68153=DIRECTION ( 'NONE',  ( -0.7071067811865270336, 0.7071067811865680008, -7.071067811864966518E-16 ) ) ;
#68154=DIRECTION ( 'NONE',  ( 0.000000000000000000, 0.000000000000000000, 1.000000000000000000 ) ) ;
#68156=CARTESIAN_POINT ( 'NONE',  ( 112.4768706805521248, -45.73309770202773450, 234.0070538473389377 ) ) ;
#68157=CIRCLE ( 'NONE', #79786, 2.517499999999998739 ) ;
#68161=VERTEX_POINT ( 'NONE', #73093 ) ;
#68162=CARTESIAN_POINT ( 'NONE',  ( 116.2698991418618419, -31.74044761805202342, 65.22133956162595325 ) ) ;
#68163=CARTESIAN_POINT ( 'NONE',  ( 138.0667039024480403, -58.72944715994091069, 239.5838068554170377 ) ) ;
#68165=ORIENTED_EDGE ( 'NONE', *, *, #63004, .F. ) ;
#68166=B_SPLINE_CURVE_WITH_KNOTS ( 'NONE', 3,
 ( #55569, #48767, #87113, #24881, #38494, #52548, #18056, #16075, #36948, #70131, #1092, #76949, #85573, #56486, #9253, #63773, #29689, #57835 ),
 .UNSPECIFIED., .F., .F.,
 ( 4, 2, 2, 2, 2, 2, 2, 2, 4 ),
 ( 0.000000000000000000, 0.06250571285318999581, 0.1250114257063799916, 0.1875171385595699736, 0.2500228514127599833, 0.3125285642659499930, 0.3750342771191399471, 0.4375399899723299568, 0.5000457028255199665 ),
 .UNSPECIFIED. ) ;
#68168=EDGE_CURVE ( 'NONE', #8740, #54700, #56280, .T. ) ;
#68169=AXIS2_PLACEMENT_3D ( 'NONE', #38323, #66022, #73741 ) ;
#68170=CARTESIAN_POINT ( 'NONE',  ( 100.9536334643938886, -28.70783906175689992, 160.5938426771316188 ) ) ;
#68171=FACE_OUTER_BOUND ( 'NONE', #31764, .T. ) ;
#68172=FACE_OUTER_BOUND ( 'NONE', #81398, .T. ) ;
#68174=CARTESIAN_POINT ( 'NONE',  ( 112.6937225954192172, -42.64246220573352275, 155.9995189410199714 ) ) ;
#68175=CARTESIAN_POINT ( 'NONE',  ( 104.8366293861751330, -26.48703790372925937, 256.2470538473397710 ) ) ;
#68177=LINE ( 'NONE', #88629, #58109 ) ;
#68178=ORIENTED_EDGE ( 'NONE', *, *, #7054, .F. ) ;
#68181=DIRECTION ( 'NONE',  ( 1.000000000000000078E-15, -1.000000000000000083E-30, -1.000000000000000000 ) ) ;
#68183=EDGE_LOOP ( 'NONE', ( #52495, #43922, #60575, #21953 ) ) ;
#68184=DIRECTION ( 'NONE',  ( -0.7071067812162665778, -0.7071067811568285677, -7.071067812162659944E-16 ) ) ;
#68186=ORIENTED_EDGE ( 'NONE', *, *, #6919, .T. ) ;
#68189=FACE_OUTER_BOUND ( 'NONE', #2891, .T. ) ;
#68190=CARTESIAN_POINT ( 'NONE',  ( 124.9629318080292251, -56.47944715994101728, 14.92562527591098842 ) ) ;
#68192=CARTESIAN_POINT ( 'NONE',  ( 115.8434954054525292, -34.49858887834006538, 168.4590864947439854 ) ) ;
#68193=CARTESIAN_POINT ( 'NONE',  ( 113.4866449958868770, -46.74994221786862880, 68.02991099019695298 ) ) ;
#68195=ORIENTED_EDGE ( 'NONE', *, *, #28895, .T. ) ;
#68196=LINE ( 'NONE', #27297, #33961 ) ;
#68197=ORIENTED_EDGE ( 'NONE', *, *, #49334, .F. ) ;
#68200=CARTESIAN_POINT ( 'NONE',  ( 107.0664832912748068, -36.72944715993923381, 13.92562527591097066 ) ) ;
#68201=DIRECTION ( 'NONE',  ( -0.7071067811865516806, 0.7071067811865433539, -7.071067811865510832E-16 ) ) ;
#68202=EDGE_CURVE ( 'NONE', #35758, #53395, #40402, .T. ) ;
#68203=CARTESIAN_POINT ( 'NONE',  ( 114.6570493066734002, -43.27250257336863370, 133.2604112297873371 ) ) ;
#68205=CARTESIAN_POINT ( 'NONE',  ( 162.7866693523294828, -29.62846900981742237, 313.9678068554149490 ) ) ;
#68206=VERTEX_POINT ( 'NONE', #25219 ) ;
#68207=CARTESIAN_POINT ( 'NONE',  ( 113.7561043996362287, -29.08408549058404091, 289.5032443235301116 ) ) ;
#68208=CARTESIAN_POINT ( 'NONE',  ( 96.87875409107806490, -32.32403320637130406, 57.01372051400599616 ) ) ;
#68212=CARTESIAN_POINT ( 'NONE',  ( 136.8164832912740110, -36.72944715994100306, -5.074374724088999145 ) ) ;
#68213=B_SPLINE_CURVE_WITH_KNOTS ( 'NONE', 3,
 ( #18250, #45482, #10983, #4181, #73203, #45927, #57798, #16472, #44149, #65067, #40487, #75009, #60927, #4628, #25969, #88655, #81843, #74557, #27303, #33675, #40030, #60466, #32774, #88211, #67287, #11443, #13240, #67749, #39141, #61813, #26852, #19592, #26417, #18699, #80951, #53634, #82747, #6415, #12337, #54087, #68203, #33230, #54978, #34107, #87743, #5071, #60009, #61368, #5535, #25512, #54532 ),
 .UNSPECIFIED., .F., .F.,
 ( 4, 2, 1, 1, 1, 1, 1, 1, 2, 2, 2, 2, 2, 2, 2, 1, 1, 1, 1, 1, 1, 1, 2, 2, 2, 2, 2, 2, 2, 2, 2, 4 ),
 ( 0.5000150437144960103, 0.5001371103542051610, 0.5002591769939142008, 0.5005033102733320582, 0.5009915768321673291, 0.5019681099498382038, 0.5039211761851796201, 0.5078273086558623417, 0.5156395735972280070, 0.5312641034799590045, 0.5625131632454207775, 0.6250112827763437684, 0.6875094023072667593, 0.7500075218381896391, 0.7500685551580437149, 0.7501295884778977907, 0.7502516551176239279, 0.7504957883970906352, 0.7509840549560078404, 0.7519605880738274850, 0.7539136543094671072, 0.7578197867807463517, 0.7656320517233036194, 0.7812565816084167114, 0.8125056413786428955, 0.8437547011488690796, 0.8750037609190952637, 0.9062528206893214477, 0.9375018804595476318, 0.9687509402297738159, 0.9843754701148869080, 1.000000000000000000 ),
 .UNSPECIFIED. ) ;
#68216=CIRCLE ( 'NONE', #84176, 2.999999999999933387 ) ;
#68217=DIRECTION ( 'NONE',  ( -0.000000000000000000, -0.000000000000000000, 1.000000000000000000 ) ) ;
#68219=VECTOR ( 'NONE', #18267, 1000.000000000000000 ) ;
#68220=DIRECTION ( 'NONE',  ( 0.000000000000000000, 0.000000000000000000, -1.000000000000000000 ) ) ;
#68221=ORIENTED_EDGE ( 'NONE', *, *, #15294, .T. ) ;
#68222=EDGE_CURVE ( 'NONE', #7923, #3091, #10260, .T. ) ;
#68223=CARTESIAN_POINT ( 'NONE',  ( 103.3547197592076969, -47.16534756318074528, 98.31657765686297523 ) ) ;
#68224=CARTESIAN_POINT ( 'NONE',  ( 122.8585116216235065, -38.08382569396911776, 302.4856252759109907 ) ) ;
#68226=LINE ( 'NONE', #89565, #32055 ) ;
#68228=EDGE_CURVE ( 'NONE', #79315, #71373, #37527, .T. ) ;
#68229=DIRECTION ( 'NONE',  ( 4.237773401492740281E-14, -1.000000000000000000, 0.000000000000000000 ) ) ;
#68230=ORIENTED_EDGE ( 'NONE', *, *, #78051, .T. ) ;
#68231=CARTESIAN_POINT ( 'NONE',  ( 116.3126599349420900, -33.43976754494801185, 110.0984824187669631 ) ) ;
#68232=VECTOR ( 'NONE', #77679, 1000.000000000000000 ) ;
#68234=ORIENTED_EDGE ( 'NONE', *, *, #69083, .F. ) ;
#68235=CARTESIAN_POINT ( 'NONE',  ( 116.0363244534468237, -41.99923036749492411, 234.4041967044819899 ) ) ;
#68237=CARTESIAN_POINT ( 'NONE',  ( 112.0504773937687872, -45.40517505809263810, 147.9914262990938312 ) ) ;
#68238=DIRECTION ( 'NONE',  ( 0.000000000000000000, 1.000000000000000000, 0.000000000000000000 ) ) ;
#68239=B_SPLINE_CURVE_WITH_KNOTS ( 'NONE', 3,
 ( #947, #79052, #85438, #28644, #56334, #84080, #21852, #15027, #42701, #35907, #80840, #52188, #66740, #24084, #38146, #46272, #4070, #65412, #51755, #65839, #53070, #18589, #79951, #86753, #3622, #74006, #25404, #81297, #38580 ),
 .UNSPECIFIED., .F., .F.,
 ( 4, 2, 2, 2, 2, 2, 2, 2, 2, 2, 1, 1, 1, 1, 1, 2, 4 ),
 ( 0.000000000000000000, 0.06250187945002849688, 0.1250037589000569938, 0.1875056383500854906, 0.2500075178001139875, 0.3125093972501424844, 0.3750112767001709813, 0.4375131561501994781, 0.4687640958752137266, 0.4843895657377207953, 0.4922023006689741909, 0.4961086681346009719, 0.4980618518674143624, 0.4990384437338208912, 0.4995267396670242110, 0.4997708876336256489, 0.5000150356002270868 ),
 .UNSPECIFIED. ) ;
#68240=CARTESIAN_POINT ( 'NONE',  ( 97.31584370783238569, -39.30597596754859779, 82.53145860666462852 ) ) ;
#68241=DIRECTION ( 'NONE',  ( -1.387778780781444413E-14, -1.000000000000000000, 0.000000000000000000 ) ) ;
#68243=AXIS2_PLACEMENT_3D ( 'NONE', #43603, #2297, #16370 ) ;
#68244=CARTESIAN_POINT ( 'NONE',  ( 113.2097911582632861, -29.11871762112820150, 164.5356252759109736 ) ) ;
#68245=ORIENTED_EDGE ( 'NONE', *, *, #64590, .F. ) ;
#68246=ORIENTED_EDGE ( 'NONE', *, *, #49419, .F. ) ;
#68247=CARTESIAN_POINT ( 'NONE',  ( 107.2938360571228600, -27.87074582556254398, 116.4872975916119771 ) ) ;
#68248=FACE_BOUND ( 'NONE', #14213, .T. ) ;
#68249=CARTESIAN_POINT ( 'NONE',  ( 104.4938967476557821, -26.68352342390111787, 241.2880062282909535 ) ) ;
#68251=CARTESIAN_POINT ( 'NONE',  ( 97.81477617152367543, -40.51601309134415629, 21.63528831556280707 ) ) ;
#68252=EDGE_CURVE ( 'NONE', #46739, #81819, #38396, .T. ) ;
#68253=EDGE_CURVE ( 'NONE', #18676, #32980, #18400, .T. ) ;
#68254=AXIS2_PLACEMENT_3D ( 'NONE', #39664, #74641, #38769 ) ;
#68255=CARTESIAN_POINT ( 'NONE',  ( 144.4532657278588204, -72.54451140298851897, 540.9756252759101471 ) ) ;
#68256=FACE_OUTER_BOUND ( 'NONE', #70640, .T. ) ;
#68257=AXIS2_PLACEMENT_3D ( 'NONE', #20187, #60601, #74691 ) ;
#68259=ADVANCED_FACE ( 'NONE', ( #45204 ), #41822, .F. ) ;
#68261=CARTESIAN_POINT ( 'NONE',  ( 117.9098725419245000, -34.70837513311212064, 203.9851490854349549 ) ) ;
#68262=DIRECTION ( 'NONE',  ( -1.000000000000000000, 0.000000000000000000, -9.974659986866630932E-16 ) ) ;
#68263=ORIENTED_EDGE ( 'NONE', *, *, #54589, .F. ) ;
#68265=ADVANCED_FACE ( 'NONE', ( #37960 ), #64781, .F. ) ;
#68266=CARTESIAN_POINT ( 'NONE',  ( 140.9629299006806775, -8.979447159940995959, -5.074374724088994704 ) ) ;
#68267=CARTESIAN_POINT ( 'NONE',  ( 78.94209639488890673, -16.21971364483396982, 1.822997995688476980 ) ) ;
#68268=DIRECTION ( 'NONE',  ( -3.999999999999999995E-14, 1.000000000000000000, -4.100000000000000342E-29 ) ) ;
#68269=DIRECTION ( 'NONE',  ( 0.000000000000000000, 1.000000000000000000, 0.000000000000000000 ) ) ;
#68270=LINE ( 'NONE', #6052, #592 ) ;
#68271=ORIENTED_EDGE ( 'NONE', *, *, #44176, .T. ) ;
#68273=( BOUNDED_CURVE ( )  B_SPLINE_CURVE ( 3, ( #13008, #60228, #74333, #82510 ),
 .UNSPECIFIED., .F., .F. ) 
 B_SPLINE_CURVE_WITH_KNOTS ( ( 4, 4 ),
 ( 6.752864695426161603E-13, 1.570796326796150222 ),
 .UNSPECIFIED. ) 
 CURVE ( )  GEOMETRIC_REPRESENTATION_ITEM ( )  RATIONAL_B_SPLINE_CURVE ( ( 1.000000000000000000, 0.8047378541242287131, 0.8047378541242287131, 1.000000000000000000 ) ) 
 REPRESENTATION_ITEM ( '' )  );
#68274=CARTESIAN_POINT ( 'NONE',  ( 100.6375269748662760, -26.77409651225141474, 220.5327681330539633 ) ) ;
#68275=VERTEX_POINT ( 'NONE', #66102 ) ;
#68276=EDGE_CURVE ( 'NONE', #80932, #79375, #58399, .T. ) ;
#68278=FACE_OUTER_BOUND ( 'NONE', #68099, .T. ) ;
#68279=CARTESIAN_POINT ( 'NONE',  ( 41.56648329127499153, -36.32844715994070839, 138.9256252759119832 ) ) ;
#68280=CARTESIAN_POINT ( 'NONE',  ( 114.6641587241874873, -32.58502278776634142, 22.02999513149600475 ) ) ;
#68281=CARTESIAN_POINT ( 'NONE',  ( 98.64836624540230048, -30.48328824330908660, 176.8184824187679567 ) ) ;
#68282=AXIS2_PLACEMENT_3D ( 'NONE', #30465, #44072, #51328 ) ;
#68284=VERTEX_POINT ( 'NONE', #31583 ) ;
#68286=CARTESIAN_POINT ( 'NONE',  ( 80.06648329127398256, -15.97944715994105813, 8.225625275910942946 ) ) ;
#68287=ORIENTED_EDGE ( 'NONE', *, *, #24475, .F. ) ;
#68289=ORIENTED_EDGE ( 'NONE', *, *, #20921, .T. ) ;
#68292=ORIENTED_EDGE ( 'NONE', *, *, #6562, .T. ) ;
#68294=CARTESIAN_POINT ( 'NONE',  ( 116.0152812585483275, -38.11929796734737863, 68.11432458998100969 ) ) ;
#68295=CARTESIAN_POINT ( 'NONE',  ( 115.7947005615567235, -30.98796762508558444, 254.2899109901966028 ) ) ;
#68296=CARTESIAN_POINT ( 'NONE',  ( 96.16101635903902434, -35.07578045570937775, 221.1946728949589840 ) ) ;
#68298=CARTESIAN_POINT ( 'NONE',  ( 100.6111884388667335, -28.52632756463412633, 11.60705384733995515 ) ) ;
#68299=CARTESIAN_POINT ( 'NONE',  ( 80.06648329127399677, -21.47944715994105991, 1.625625275910943746 ) ) ;
#68300=CYLINDRICAL_SURFACE ( 'NONE', #3316, 2.116999999999993776 ) ;
#68301=ORIENTED_EDGE ( 'NONE', *, *, #81837, .F. ) ;
#68302=CARTESIAN_POINT ( 'NONE',  ( 117.0169231590003562, -33.47438763928646210, 89.07848241876791917 ) ) ;
#68303=CARTESIAN_POINT ( 'NONE',  ( 96.71965009938165281, -35.13266635363193302, 266.2041967044820581 ) ) ;
#68304=EDGE_LOOP ( 'NONE', ( #20680, #33741, #68412, #75888, #47478 ) ) ;
#68305=CARTESIAN_POINT ( 'NONE',  ( 97.76227787611212250, -41.51041654567812600, 196.7041967044819728 ) ) ;
#68306=FACE_OUTER_BOUND ( 'NONE', #22775, .T. ) ;
#68307=DIRECTION ( 'NONE',  ( 1.000000000000000000, 0.000000000000000000, 0.000000000000000000 ) ) ;
#68309=CARTESIAN_POINT ( 'NONE',  ( 97.81930832768965445, -40.53599170015394293, 22.63722267858115345 ) ) ;
#68310=CARTESIAN_POINT ( 'NONE',  ( 106.1976517883881144, -46.78020009823125491, 28.50853215074594260 ) ) ;
#68311=CARTESIAN_POINT ( 'NONE',  ( 101.6180013298386768, -30.49747046846794518, 277.6356252759111385 ) ) ;
#68312=DIRECTION ( 'NONE',  ( 0.000000000000000000, 0.000000000000000000, 1.000000000000000000 ) ) ;
#68314=LINE ( 'NONE', #33786, #35200 ) ;
#68315=CIRCLE ( 'NONE', #59591, 16.00000000000000000 ) ;
#68316=DIRECTION ( 'NONE',  ( 0.000000000000000000, -1.000000000000000000, 0.000000000000000000 ) ) ;
#68317=CIRCLE ( 'NONE', #7428, 0.3000000000000016542 ) ;
#68318=CARTESIAN_POINT ( 'NONE',  ( 51.06648329127400388, -18.82844715994099971, 333.4006252759120343 ) ) ;
#68319=DIRECTION ( 'NONE',  ( 1.000000000000000000, -5.337610695313248426E-16, 0.000000000000000000 ) ) ;
#68320=VECTOR ( 'NONE', #52423, 1000.000000000000000 ) ;
#68321=FACE_OUTER_BOUND ( 'NONE', #24367, .T. ) ;
#68323=ORIENTED_EDGE ( 'NONE', *, *, #17087, .T. ) ;
#68324=CARTESIAN_POINT ( 'NONE',  ( 138.8167039024479834, -67.87844715994100397, 88.43480685541499042 ) ) ;
#68325=CARTESIAN_POINT ( 'NONE',  ( 105.1067973254952790, -26.46757623491196298, 235.2270538473399313 ) ) ;
#68326=CARTESIAN_POINT ( 'NONE',  ( 108.5897967589408495, -47.07840195076833112, 138.6927681330539883 ) ) ;
#68327=CARTESIAN_POINT ( 'NONE',  ( 103.0738860297313266, -47.93972279484852095, 248.3041967044829619 ) ) ;
#68332=LINE ( 'NONE', #68779, #42866 ) ;
#68335=CIRCLE ( 'NONE', #63996, 2.500000000000002220 ) ;
#68336=EDGE_CURVE ( 'NONE', #54616, #64730, #2695, .T. ) ;
#68337=ORIENTED_EDGE ( 'NONE', *, *, #86023, .T. ) ;
#68338=ORIENTED_EDGE ( 'NONE', *, *, #17380, .F. ) ;
#68339=CARTESIAN_POINT ( 'NONE',  ( 111.9909297607753160, -29.75048171432638355, 129.0095626852189525 ) ) ;
#68341=ORIENTED_EDGE ( 'NONE', *, *, #86919, .T. ) ;
#68342=CARTESIAN_POINT ( 'NONE',  ( 152.0368932755770857, -23.42844715993588522, 249.9678068554149490 ) ) ;
#68343=CARTESIAN_POINT ( 'NONE',  ( 103.2134869792596135, -46.43093390711685231, 113.2756252759109827 ) ) ;
#68344=CARTESIAN_POINT ( 'NONE',  ( 108.3313360409339907, -46.73509903638382923, 148.6777836749537585 ) ) ;
#68345=DIRECTION ( 'NONE',  ( 1.639958061481212836E-42, -4.100000000000000342E-29, -1.000000000000000000 ) ) ;
#68346=PRODUCT_DEFINITION ( 'UNKNOWN', '', #84135, #2404 ) ;
#68347=AXIS2_PLACEMENT_3D ( 'NONE', #39303, #4791, #32032 ) ;
#68348=DIRECTION ( 'NONE',  ( -0.0001713722456120069274, 0.9999999853157766072, 0.000000000000000000 ) ) ;
#68350=CARTESIAN_POINT ( 'NONE',  ( 117.2535196871930481, -41.18324016912744412, 58.49848241876892985 ) ) ;
#68354=ORIENTED_EDGE ( 'NONE', *, *, #12257, .F. ) ;
#68356=CARTESIAN_POINT ( 'NONE',  ( 108.4956486572523602, -46.43878675094416764, 138.6927681330529936 ) ) ;
#68357=LINE ( 'NONE', #46544, #86788 ) ;
#68358=CARTESIAN_POINT ( 'NONE',  ( 88.06670390244791236, -14.72944715994105991, 239.5838068554169809 ) ) ;
#68359=DIRECTION ( 'NONE',  ( 0.000000000000000000, 1.000000000000000000, 0.000000000000000000 ) ) ;
#68360=EDGE_CURVE ( 'NONE', #29833, #74616, #38919, .T. ) ;
#68361=AXIS2_PLACEMENT_3D ( 'NONE', #42696, #36361, #29545 ) ;
#68364=EDGE_CURVE ( 'NONE', #32750, #40462, #9820, .T. ) ;
#68365=FACE_OUTER_BOUND ( 'NONE', #12653, .T. ) ;
#68366=CARTESIAN_POINT ( 'NONE',  ( 96.81317962367440089, -38.48968277746988065, 91.46133956162493917 ) ) ;
#68367=ORIENTED_EDGE ( 'NONE', *, *, #57899, .F. ) ;
#68368=EDGE_CURVE ( 'NONE', #89731, #37957, #9372, .T. ) ;
#68369=VERTEX_POINT ( 'NONE', #17079 ) ;
#68373=DIRECTION ( 'NONE',  ( -1.000000000000000000, -4.299999999999999979E-14, -1.000000000000000078E-15 ) ) ;
#68374=DIRECTION ( 'NONE',  ( 0.000000000000000000, 1.000000000000000000, 0.000000000000000000 ) ) ;
#68376=CARTESIAN_POINT ( 'NONE',  ( 101.5399107887468944, -29.27606352979315574, 183.4023760838769590 ) ) ;
#68379=ORIENTED_EDGE ( 'NONE', *, *, #71881, .F. ) ;
#68380=VERTEX_POINT ( 'NONE', #44315 ) ;
#68381=EDGE_CURVE ( 'NONE', #76536, #37688, #59206, .T. ) ;
#68382=CARTESIAN_POINT ( 'NONE',  ( 150.5667039024482960, -47.82844715993594775, 300.4678068554149490 ) ) ;
#68383=AXIS2_PLACEMENT_3D ( 'NONE', #6219, #69338, #40271 ) ;
#68384=CARTESIAN_POINT ( 'NONE',  ( 134.8178559631273856, -21.40256188477526678, 1.690787648081120143 ) ) ;
#68385=ORIENTED_EDGE ( 'NONE', *, *, #70949, .F. ) ;
#68389=CARTESIAN_POINT ( 'NONE',  ( 99.39098736499681763, -43.25305561222647555, 223.3187261630399689 ) ) ;
#68390=CIRCLE ( 'NONE', #78597, 2.500000000000002220 ) ;
#68394=ORIENTED_EDGE ( 'NONE', *, *, #88171, .F. ) ;
#68395=AXIS2_PLACEMENT_3D ( 'NONE', #20365, #41667, #62579 ) ;
#68396=DIRECTION ( 'NONE',  ( -0.7071067811866258435, 0.7071067811864693020, -7.071067811866266166E-16 ) ) ;
#68397=ORIENTED_EDGE ( 'NONE', *, *, #59147, .T. ) ;
#68398=EDGE_LOOP ( 'NONE', ( #83045, #8397 ) ) ;
#68399=CARTESIAN_POINT ( 'NONE',  ( 103.9533468823514823, -45.47040322110986210, 250.1223760838773273 ) ) ;
#68400=CARTESIAN_POINT ( 'NONE',  ( 99.40582560697848180, -27.65448416857716651, 150.6356252759109680 ) ) ;
#68401=CARTESIAN_POINT ( 'NONE',  ( 116.9541756933415257, -33.49491404195858735, 89.07848241876791917 ) ) ;
#68402=CARTESIAN_POINT ( 'NONE',  ( 99.19001052970209287, -35.07347417754516528, 249.5838068554172935 ) ) ;
#68404=CARTESIAN_POINT ( 'NONE',  ( 107.0664832912739968, -36.72944715994100306, 195.5838068554169809 ) ) ;
#68406=CARTESIAN_POINT ( 'NONE',  ( 98.37977233551227130, -29.89460749427659181, 196.8080062282919869 ) ) ;
#68411=CIRCLE ( 'NONE', #19122, 2.517500000000005844 ) ;
#68412=ORIENTED_EDGE ( 'NONE', *, *, #619, .T. ) ;
#68414=EDGE_LOOP ( 'NONE', ( #56421, #10793, #11639, #57041, #86941 ) ) ;
#68418=CARTESIAN_POINT ( 'NONE',  ( 116.9219696586192754, -33.22298239640010564, 114.0984824187679720 ) ) ;
#68421=LINE ( 'NONE', #47046, #13074 ) ;
#68422=CARTESIAN_POINT ( 'NONE',  ( 130.5667039024480118, -36.72944715994093912, 229.5838068554170093 ) ) ;
#68423=DIRECTION ( 'NONE',  ( -4.237773401492740281E-14, 1.000000000000000000, 0.000000000000000000 ) ) ;
#68425=CARTESIAN_POINT ( 'NONE',  ( 116.5068947302721369, -41.18400185692900806, 224.4756252759109714 ) ) ;
#68427=CARTESIAN_POINT ( 'NONE',  ( 151.0371591254575208, -24.42818131005592264, 180.4678068554149775 ) ) ;
#68430=DIRECTION ( 'NONE',  ( 0.000000000000000000, 1.000000000000000000, 0.000000000000000000 ) ) ;
#68432=DIRECTION ( 'NONE',  ( 1.000000000000000078E-15, 1.000000000000000083E-30, -1.000000000000000000 ) ) ;
#68433=VECTOR ( 'NONE', #12113, 1000.000000000000000 ) ;
#68434=CARTESIAN_POINT ( 'NONE',  ( 194.0667039024473297, -24.92844715993408045, 300.4678068554149490 ) ) ;
#68435=CARTESIAN_POINT ( 'NONE',  ( 104.8318391505165010, -26.46503486849124087, 260.2470538473397710 ) ) ;
#68436=VERTEX_POINT ( 'NONE', #27457 ) ;
#68438=CARTESIAN_POINT ( 'NONE',  ( 111.4896171341011666, -26.57472070863446589, 280.7375300378156453 ) ) ;
#68439=CARTESIAN_POINT ( 'NONE',  ( 102.0300696065151982, -46.62045497284175610, 168.2137205140059564 ) ) ;
#68440=CARTESIAN_POINT ( 'NONE',  ( 97.31584378032250982, -39.30597624822549108, 32.53145862952089118 ) ) ;
#68441=DIRECTION ( 'NONE',  ( -1.000000000000000000, 0.000000000000000000, 0.000000000000000000 ) ) ;
#68444=CARTESIAN_POINT ( 'NONE',  ( 99.09570912936477782, -30.55043168559838307, 190.8022919357809997 ) ) ;
#68445=CARTESIAN_POINT ( 'NONE',  ( 116.3212776292296127, -32.94146857471318413, 287.6356252759109680 ) ) ;
#68446=VERTEX_POINT ( 'NONE', #87905 ) ;
#68447=EDGE_CURVE ( 'NONE', #28440, #64498, #65060, .T. ) ;
#68448=ORIENTED_EDGE ( 'NONE', *, *, #70336, .T. ) ;
#68449=ORIENTED_EDGE ( 'NONE', *, *, #30428, .F. ) ;
#68450=VECTOR ( 'NONE', #74805, 1000.000000000000000 ) ;
#68451=ORIENTED_EDGE ( 'NONE', *, *, #15902, .F. ) ;
#68453=CARTESIAN_POINT ( 'NONE',  ( 118.1852327621006538, -40.75705396371408540, 19.54991099019698453 ) ) ;
#68455=CARTESIAN_POINT ( 'NONE',  ( 51.06670390244671154, -32.29483332968568021, 193.9678068554150911 ) ) ;
#68456=ADVANCED_FACE ( 'NONE', ( #12951 ), #60626, .F. ) ;
#68459=CARTESIAN_POINT ( 'NONE',  ( 98.95796485450003388, -39.41423029504880304, 241.0038483995049603 ) ) ;
#68460=ORIENTED_EDGE ( 'NONE', *, *, #3953, .F. ) ;
#68461=VERTEX_POINT ( 'NONE', #19311 ) ;
#68462=EDGE_LOOP ( 'NONE', ( #86557, #44814, #40736, #57878 ) ) ;
#68463=CONICAL_SURFACE ( 'NONE', #22055, 7.249999999999998224, 0.7853981633974772558 ) ;
#68464=FACE_BOUND ( 'NONE', #37489, .T. ) ;
#68465=CARTESIAN_POINT ( 'NONE',  ( 97.87459229980032660, -40.66846143049065887, 101.6490831034139433 ) ) ;
#68466=EDGE_CURVE ( 'NONE', #54909, #75220, #20069, .T. ) ;
#68467=CARTESIAN_POINT ( 'NONE',  ( 151.0371591254575492, -24.95799193692592155, 180.4678068554149775 ) ) ;
#68471=CARTESIAN_POINT ( 'NONE',  ( 115.1619974903381518, -42.21817061296157192, 273.3527681330542691 ) ) ;
#68473=DIRECTION ( 'NONE',  ( 0.000000000000000000, 0.000000000000000000, 1.000000000000000000 ) ) ;
#68475=ORIENTED_EDGE ( 'NONE', *, *, #23258, .F. ) ;
#68476=CARTESIAN_POINT ( 'NONE',  ( 36.23715912545339535, -47.82818131006131779, 180.4678068554150911 ) ) ;
#68478=CARTESIAN_POINT ( 'NONE',  ( 99.67188489287487130, -33.20771423803368094, 73.79094751244896599 ) ) ;
#68479=AXIS2_PLACEMENT_3D ( 'NONE', #50329, #16279, #83986 ) ;
#68481=CARTESIAN_POINT ( 'NONE',  ( 116.3212776292293995, -32.94146857471265122, 80.13562527591095375 ) ) ;
#68483=VECTOR ( 'NONE', #73437, 1000.000000000000114 ) ;
#68484=CARTESIAN_POINT ( 'NONE',  ( 98.34985891086999743, -31.65658481233683830, 45.90645860949901191 ) ) ;
#68487=CARTESIAN_POINT ( 'NONE',  ( 79.18623681049682261, -34.12360705087682078, 8.106403045242537075 ) ) ;
#68488=EDGE_LOOP ( 'NONE', ( #21468, #66787, #88638, #17610 ) ) ;
#68489=CARTESIAN_POINT ( 'NONE',  ( 102.3930168087890422, -26.71257147495026274, 135.4118157521009493 ) ) ;
#68490=ORIENTED_EDGE ( 'NONE', *, *, #18826, .F. ) ;
#68491=EDGE_CURVE ( 'NONE', #66245, #54835, #68357, .T. ) ;
#68494=CARTESIAN_POINT ( 'NONE',  ( 101.9936209862019467, -45.44607156465968245, 68.15645861336898292 ) ) ;
#68495=CARTESIAN_POINT ( 'NONE',  ( 115.8195149170444296, -38.11245691049232676, 110.1330118773259699 ) ) ;
#68497=EDGE_CURVE ( 'NONE', #30248, #39757, #82000, .T. ) ;
#68498=CARTESIAN_POINT ( 'NONE',  ( 184.5667039024480118, -48.82844715994099971, 10.91780685541479734 ) ) ;
#68499=CARTESIAN_POINT ( 'NONE',  ( 103.8345913547307333, -46.70111052772084292, 78.32705384733995402 ) ) ;
#68500=FACE_OUTER_BOUND ( 'NONE', #70842, .T. ) ;
#68501=VERTEX_POINT ( 'NONE', #53344 ) ;
#68508=CARTESIAN_POINT ( 'NONE',  ( 97.40014589274343848, -35.23768424668791965, 266.2041967044829676 ) ) ;
#68509=CARTESIAN_POINT ( 'NONE',  ( 108.6520215831686329, -25.77392822130451577, 145.9737205140069420 ) ) ;
#68510=DIRECTION ( 'NONE',  ( 0.000000000000000000, 0.000000000000000000, 1.000000000000000000 ) ) ;
#68511=CARTESIAN_POINT ( 'NONE',  ( 97.81169461453751524, -40.51741999607308742, 142.6356648221729131 ) ) ;
#68512=CARTESIAN_POINT ( 'NONE',  ( 118.8426969166518319, -35.40452897077508965, 79.91562527591095488 ) ) ;
#68513=LINE ( 'NONE', #61675, #77061 ) ;
#68515=LINE ( 'NONE', #12206, #20763 ) ;
#68518=ORIENTED_EDGE ( 'NONE', *, *, #28084, .T. ) ;
#68519=VECTOR ( 'NONE', #6160, 1000.000000000000000 ) ;
#68520=DIRECTION ( 'NONE',  ( 9.032638163712999905E-13, -1.000000000000000000, 1.217258424823508649E-28 ) ) ;
#68521=DIRECTION ( 'NONE',  ( 0.000000000000000000, 0.000000000000000000, 1.000000000000000000 ) ) ;
#68522=CARTESIAN_POINT ( 'NONE',  ( 102.3890460933095170, -47.58756240099349100, 287.2527681330536780 ) ) ;
#68524=EDGE_CURVE ( 'NONE', #78468, #22617, #82897, .T. ) ;
#68526=CARTESIAN_POINT ( 'NONE',  ( 51.23005224011683367, -33.89581943344270343, 117.4678068554150485 ) ) ;
#68527=CARTESIAN_POINT ( 'NONE',  ( 110.0852322082900372, -46.03269033891531592, 12.82705384733995402 ) ) ;
#68528=CARTESIAN_POINT ( 'NONE',  ( 107.2382243570020961, -26.63832244206171751, 100.0631150270457255 ) ) ;
#68529=CARTESIAN_POINT ( 'NONE',  ( 109.5033840998383994, -46.84330794493973826, 128.7641967044819751 ) ) ;
#68530=LINE ( 'NONE', #6298, #61093 ) ;
#68531=CARTESIAN_POINT ( 'NONE',  ( 112.5090891374639313, -26.14611880238131647, 169.6984824187679521 ) ) ;
#68533=ORIENTED_EDGE ( 'NONE', *, *, #49469, .T. ) ;
#68534=CYLINDRICAL_SURFACE ( 'NONE', #49724, 9.999999999999998224 ) ;
#68535=DIRECTION ( 'NONE',  ( 1.000000000000000078E-15, 1.000000000000000083E-30, -1.000000000000000000 ) ) ;
#68536=DIRECTION ( 'NONE',  ( -0.7071067811607679721, 0.7071067812123270624, 0.000000000000000000 ) ) ;
#68537=ORIENTED_EDGE ( 'NONE', *, *, #1089, .T. ) ;
#68540=CARTESIAN_POINT ( 'NONE',  ( 117.2652295300992193, -42.86250289712283745, 128.3956252759109873 ) ) ;
#68542=FACE_OUTER_BOUND ( 'NONE', #61489, .T. ) ;
#68545=CARTESIAN_POINT ( 'NONE',  ( 94.12733899296569007, -42.07533762155324553, 293.1356252759106837 ) ) ;
#68547=AXIS2_PLACEMENT_3D ( 'NONE', #32867, #81053, #32408 ) ;
#68551=VERTEX_POINT ( 'NONE', #88812 ) ;
#68554=ADVANCED_FACE ( 'NONE', ( #39736, #32471 ), #34269, .T. ) ;
#68555=ORIENTED_EDGE ( 'NONE', *, *, #46931, .F. ) ;
#68561=EDGE_CURVE ( 'NONE', #25149, #5538, #5549, .T. ) ;
#68562=CARTESIAN_POINT ( 'NONE',  ( 193.0371591254575208, -23.42818131005411786, 129.9678068554150343 ) ) ;
#68564=CARTESIAN_POINT ( 'NONE',  ( 97.53192512710711526, -39.74921111115579464, 181.5705521802071871 ) ) ;
#68566=EDGE_CURVE ( 'NONE', #10240, #81584, #88290, .T. ) ;
#68568=VERTEX_POINT ( 'NONE', #42415 ) ;
#68570=FACE_BOUND ( 'NONE', #67459, .T. ) ;
#68572=CARTESIAN_POINT ( 'NONE',  ( 115.2378349030890092, -31.35427756934441845, 250.2899109901960344 ) ) ;
#68573=LINE ( 'NONE', #21314, #19679 ) ;
#68574=AXIS2_PLACEMENT_3D ( 'NONE', #28099, #21303, #55782 ) ;
#68575=CARTESIAN_POINT ( 'NONE',  ( 113.4367438382843716, -44.15125393826585309, 104.1413395616249744 ) ) ;
#68579=CARTESIAN_POINT ( 'NONE',  ( 105.9764260794164983, -26.77672323648842578, 21.16324968342363277 ) ) ;
#68580=ORIENTED_EDGE ( 'NONE', *, *, #65275, .T. ) ;
#68581=CARTESIAN_POINT ( 'NONE',  ( 156.5667039024483529, -48.82844715993569196, 293.2178068554149490 ) ) ;
#68582=VERTEX_POINT ( 'NONE', #57397 ) ;
#68583=ORIENTED_EDGE ( 'NONE', *, *, #10355, .F. ) ;
#68584=DIRECTION ( 'NONE',  ( 1.639958061481212836E-42, -4.100000000000000342E-29, -1.000000000000000000 ) ) ;
#68585=CARTESIAN_POINT ( 'NONE',  ( 98.43690990026183840, -34.58641363334965035, 272.5644404487542829 ) ) ;
#68586=AXIS2_PLACEMENT_3D ( 'NONE', #4592, #25031, #47243 ) ;
#68587=CARTESIAN_POINT ( 'NONE',  ( 49.21213752016101495, -29.73316016639650172, -5.074374724088000832 ) ) ;
#68589=CARTESIAN_POINT ( 'NONE',  ( 75.31670390244798341, -57.40094715994099772, 86.31780685541500020 ) ) ;
#68591=ORIENTED_EDGE ( 'NONE', *, *, #82936, .T. ) ;
#68595=EDGE_LOOP ( 'NONE', ( #21353, #32057, #72518, #50735, #47266 ) ) ;
#68596=CARTESIAN_POINT ( 'NONE',  ( 115.6733145644062262, -43.66497474544748059, 43.27467289495795200 ) ) ;
#68599=CARTESIAN_POINT ( 'NONE',  ( 99.00928370863422856, -39.88895027456798914, 244.4299951314959571 ) ) ;
#68600=EDGE_CURVE ( 'NONE', #37791, #22595, #8831, .T. ) ;
#68602=CARTESIAN_POINT ( 'NONE',  ( 116.4077482568849859, -39.73851878533137238, 158.5784824187689708 ) ) ;
#68603=DIRECTION ( 'NONE',  ( 1.000000000000000078E-15, -1.000000000000000000, 0.000000000000000000 ) ) ;
#68604=FACE_OUTER_BOUND ( 'NONE', #89112, .T. ) ;
#68605=DIRECTION ( 'NONE',  ( -0.7071067811865758834, 0.7071067811865192621, -7.071067811865766226E-16 ) ) ;
#68606=EDGE_CURVE ( 'NONE', #84043, #32962, #24416, .T. ) ;
#68608=CARTESIAN_POINT ( 'NONE',  ( 110.7484172854196629, -26.25849398357808084, 250.8194347997207387 ) ) ;
#68610=ORIENTED_EDGE ( 'NONE', *, *, #31144, .T. ) ;
#68612=CARTESIAN_POINT ( 'NONE',  ( 112.8257383337702606, -47.14300054286279362, 98.97848241876793907 ) ) ;
#68614=ORIENTED_EDGE ( 'NONE', *, *, #67211, .F. ) ;
#68615=ORIENTED_EDGE ( 'NONE', *, *, #68710, .F. ) ;
#68617=CARTESIAN_POINT ( 'NONE',  ( 141.0667039024479834, -48.82844715994099971, 198.9178068554149945 ) ) ;
#68618=DIRECTION ( 'NONE',  ( 0.000000000000000000, 0.000000000000000000, 1.000000000000000000 ) ) ;
#68619=DIRECTION ( 'NONE',  ( 1.000000000000000000, 4.163336342344333240E-14, 0.000000000000000000 ) ) ;
#68621=CARTESIAN_POINT ( 'NONE',  ( 103.8146984276687022, -29.21261587019397155, 153.2195189410199418 ) ) ;
#68622=CARTESIAN_POINT ( 'NONE',  ( 101.2819412958853320, -26.35826957050098329, 251.4813395616249920 ) ) ;
#68623=CARTESIAN_POINT ( 'NONE',  ( 105.7141124688251352, -46.72365530278647583, 58.46884690485195790 ) ) ;
#68624=ORIENTED_EDGE ( 'NONE', *, *, #26769, .F. ) ;
#68626=FACE_BOUND ( 'NONE', #7015, .T. ) ;
#68628=ORIENTED_EDGE ( 'NONE', *, *, #45802, .F. ) ;
#68632=EDGE_LOOP ( 'NONE', ( #84059, #27757, #39729, #62904 ) ) ;
#68633=CARTESIAN_POINT ( 'NONE',  ( 37.56670390244749314, -48.82844715994126261, 129.9678068554150911 ) ) ;
#68634=CARTESIAN_POINT ( 'NONE',  ( 172.5664832912729878, -27.57844715994070484, 138.9256252759119832 ) ) ;
#68637=CARTESIAN_POINT ( 'NONE',  ( 110.0404421551223209, -45.97207645956791566, 207.2467055423619513 ) ) ;
#68638=CARTESIAN_POINT ( 'NONE',  ( 115.0563813407508889, -43.54951484902237979, 63.26419670448196797 ) ) ;
#68641=VERTEX_POINT ( 'NONE', #70599 ) ;
#68642=AXIS2_PLACEMENT_3D ( 'NONE', #2555, #57043, #37951 ) ;
#68644=ORIENTED_EDGE ( 'NONE', *, *, #58196, .T. ) ;
#68647=CARTESIAN_POINT ( 'NONE',  ( 71.25614885437424562, -84.12815644128085069, 542.9756252759101471 ) ) ;
#68649=DIRECTION ( 'NONE',  ( 0.7071067811865969777, -0.7071067811864980568, 0.000000000000000000 ) ) ;
#68650=CIRCLE ( 'NONE', #23729, 3.250000000000002665 ) ;
#68651=DIRECTION ( 'NONE',  ( 1.000000000000000000, 0.000000000000000000, 0.000000000000000000 ) ) ;
#68652=EDGE_LOOP ( 'NONE', ( #8051, #57407, #72204, #8483 ) ) ;
#68653=CARTESIAN_POINT ( 'NONE',  ( 101.1283730419716562, -27.37881681735623829, 65.51467289495799662 ) ) ;
#68655=CARTESIAN_POINT ( 'NONE',  ( 98.34960815996063843, -31.65702116157642720, 165.9064988554816864 ) ) ;
#68658=EDGE_CURVE ( 'NONE', #58653, #63781, #12690, .T. ) ;
#68659=CYLINDRICAL_SURFACE ( 'NONE', #28190, 2.500000000000002220 ) ;
#68660=ORIENTED_EDGE ( 'NONE', *, *, #40125, .F. ) ;
#68666=VERTEX_POINT ( 'NONE', #17851 ) ;
#68667=CARTESIAN_POINT ( 'NONE',  ( 97.24595611328004452, -31.60670846949429347, 86.93181575210095957 ) ) ;
#68669=LINE ( 'NONE', #61830, #48479 ) ;
#68670=CARTESIAN_POINT ( 'NONE',  ( 172.5664832912729878, -27.82844715994070484, 78.92562527591199739 ) ) ;
#68671=EDGE_CURVE ( 'NONE', #44708, #8522, #88356, .T. ) ;
#68676=CARTESIAN_POINT ( 'NONE',  ( 102.6513375509277779, -45.45698538002849176, 123.2041967044819870 ) ) ;
#68678=ORIENTED_EDGE ( 'NONE', *, *, #862, .T. ) ;
#68679=CARTESIAN_POINT ( 'NONE',  ( 96.27200394136428940, -34.46162041542912391, 257.1737205140064475 ) ) ;
#68680=CARTESIAN_POINT ( 'NONE',  ( 97.82477004090156925, -40.54925333673140386, 252.6383302522648364 ) ) ;
#68681=LINE ( 'NONE', #42737, #14176 ) ;
#68682=DIRECTION ( 'NONE',  ( 1.000000000000000078E-15, 1.000000000000000083E-30, -1.000000000000000000 ) ) ;
#68683=DIRECTION ( 'NONE',  ( 1.000000000000000000, 0.000000000000000000, 0.000000000000000000 ) ) ;
#68686=DIRECTION ( 'NONE',  ( 0.000000000000000000, 1.000000000000000000, 0.000000000000000000 ) ) ;
#68687=CARTESIAN_POINT ( 'NONE',  ( 107.5349099188610893, -47.08895302312306086, 192.6003871806729535 ) ) ;
#68688=ORIENTED_EDGE ( 'NONE', *, *, #2200, .F. ) ;
#68689=VERTEX_POINT ( 'NONE', #78322 ) ;
#68691=CARTESIAN_POINT ( 'NONE',  ( 97.67976800739046439, -37.13700294324897300, 112.7806309249449441 ) ) ;
#68693=CARTESIAN_POINT ( 'NONE',  ( 100.4593337790148837, -29.47290724209160828, 281.6641967044818671 ) ) ;
#68694=DIRECTION ( 'NONE',  ( 0.000000000000000000, 1.000000000000000000, 0.000000000000000000 ) ) ;
#68696=CARTESIAN_POINT ( 'NONE',  ( 107.0664832912739399, -36.72944715994095333, 305.7141315223800007 ) ) ;
#68698=DIRECTION ( 'NONE',  ( -0.7071067811869841124, 0.7071067811861110330, 0.000000000000000000 ) ) ;
#68701=DIRECTION ( 'NONE',  ( 0.000000000000000000, 1.000000000000000000, 0.000000000000000000 ) ) ;
#68702=CARTESIAN_POINT ( 'NONE',  ( 95.31970492887376167, -38.09378048407036488, 236.4184824187679510 ) ) ;
#68703=CARTESIAN_POINT ( 'NONE',  ( 107.0664832912739968, -36.72944715994100306, 0.4256252759109701023 ) ) ;
#68705=EDGE_LOOP ( 'NONE', ( #47976, #84037 ) ) ;
#68707=CARTESIAN_POINT ( 'NONE',  ( 82.41057659162025573, -20.17027654744481779, 7.249284792665543264 ) ) ;
#68708=CARTESIAN_POINT ( 'NONE',  ( 97.31582652829270330, -39.30593436283783149, 186.5319638594795038 ) ) ;
#68710=EDGE_CURVE ( 'NONE', #33465, #85262, #50582, .T. ) ;
#68712=DIRECTION ( 'NONE',  ( -0.9254794337955623007, -0.3787978585227819162, 0.000000000000000000 ) ) ;
#68713=EDGE_LOOP ( 'NONE', ( #36081, #71241, #13136, #32088 ) ) ;
#68715=CARTESIAN_POINT ( 'NONE',  ( 110.0520778049922939, -26.08682939676148038, 219.8708633711489711 ) ) ;
#68716=ORIENTED_EDGE ( 'NONE', *, *, #81308, .F. ) ;
#68717=CARTESIAN_POINT ( 'NONE',  ( 90.44969454456416713, -53.34645651782494724, 218.8274735512160589 ) ) ;
#68718=FACE_OUTER_BOUND ( 'NONE', #20922, .T. ) ;
#68719=CARTESIAN_POINT ( 'NONE',  ( 116.7467640915520093, -34.14836189904143993, 169.0338844110338812 ) ) ;
#68720=CARTESIAN_POINT ( 'NONE',  ( 97.89197038913195570, -35.34227587553755257, 69.02523322673498285 ) ) ;
#68721=CARTESIAN_POINT ( 'NONE',  ( 99.08473320778040261, -45.52208679145996939, 152.9899109901969894 ) ) ;
#68724=EDGE_CURVE ( 'NONE', #2670, #44910, #51032, .T. ) ;
#68726=CARTESIAN_POINT ( 'NONE',  ( 98.35383060353775875, -41.64759613607919420, 66.73610187141720473 ) ) ;
#68727=ORIENTED_EDGE ( 'NONE', *, *, #6455, .F. ) ;
#68729=CIRCLE ( 'NONE', #19445, 0.5000000000000004441 ) ;
#68730=ADVANCED_FACE ( 'NONE', ( #30597 ), #30151, .F. ) ;
#68732=ORIENTED_EDGE ( 'NONE', *, *, #6745, .T. ) ;
#68733=EDGE_LOOP ( 'NONE', ( #27814, #49786, #23400, #83856 ) ) ;
#68734=CARTESIAN_POINT ( 'NONE',  ( 46.83715912545422100, -47.82818131006082751, 313.9678068554150059 ) ) ;
#68735=VECTOR ( 'NONE', #47154, 1000.000000000000000 ) ;
#68736=CARTESIAN_POINT ( 'NONE',  ( 104.4240671743138478, -44.88234475468695450, 81.74956268521998481 ) ) ;
#68737=CARTESIAN_POINT ( 'NONE',  ( 115.8739437555936718, -44.69579237430344421, 233.2413395616259493 ) ) ;
#68738=CARTESIAN_POINT ( 'NONE',  ( 104.1918496689534948, -26.69446299336401296, 225.2984824187679749 ) ) ;
#68740=CARTESIAN_POINT ( 'NONE',  ( 111.1204619107249556, -46.98756979654999810, 18.88800622829195319 ) ) ;
#68744=VERTEX_POINT ( 'NONE', #37410 ) ;
#68746=CARTESIAN_POINT ( 'NONE',  ( 114.7602587138392920, -43.68247563549513046, 83.25372051400698581 ) ) ;
#68747=CARTESIAN_POINT ( 'NONE',  ( 114.3840247170090407, -44.21678670926648635, 73.19276813305397411 ) ) ;
#68748=CARTESIAN_POINT ( 'NONE',  ( 114.4461924768642405, -27.39302975889309266, 274.5441967044824878 ) ) ;
#68751=CARTESIAN_POINT ( 'NONE',  ( 110.2559530472221923, -26.76685766971437630, 234.8299109901969643 ) ) ;
#68752=CARTESIAN_POINT ( 'NONE',  ( 104.4899543942856042, -26.97880759920951732, 35.28145861393137039 ) ) ;
#68753=AXIS2_PLACEMENT_3D ( 'NONE', #78853, #2543, #11117 ) ;
#68756=DIRECTION ( 'NONE',  ( -1.000000000000000000, -2.756263715554006823E-15, 0.000000000000000000 ) ) ;
#68758=ADVANCED_FACE ( 'NONE', ( #45529 ), #44654, .F. ) ;
#68759=CARTESIAN_POINT ( 'NONE',  ( 110.4768011403582904, -29.48025783594732729, 277.6356252759111385 ) ) ;
#68761=CARTESIAN_POINT ( 'NONE',  ( 97.81476338439986762, -40.52493715572875033, 172.6362716151192274 ) ) ;
#68770=DIRECTION ( 'NONE',  ( 0.000000000000000000, 0.000000000000000000, -1.000000000000000000 ) ) ;
#68771=ORIENTED_EDGE ( 'NONE', *, *, #25292, .F. ) ;
#68773=DIRECTION ( 'NONE',  ( 1.000000000000000000, 1.000000000000000078E-15, 1.000000000000000078E-15 ) ) ;
#68774=CARTESIAN_POINT ( 'NONE',  ( 96.11487883884397831, -35.06878432418778146, 221.1946728949589840 ) ) ;
#68775=CARTESIAN_POINT ( 'NONE',  ( 117.6079501356808947, -33.40507394795707796, 125.0575300378149706 ) ) ;
#68776=CARTESIAN_POINT ( 'NONE',  ( 96.93665061341955891, -39.37131572480267749, 272.5299109901966972 ) ) ;
#68777=LINE ( 'NONE', #40153, #89610 ) ;
#68778=DIRECTION ( 'NONE',  ( 0.000000000000000000, 0.000000000000000000, 1.000000000000000000 ) ) ;
#68779=CARTESIAN_POINT ( 'NONE',  ( 123.6837132603318992, -50.04645651782490745, 239.5838068554164693 ) ) ;
#68780=CARTESIAN_POINT ( 'NONE',  ( 107.0664832912739399, -36.72944715994095333, 247.7440089327910755 ) ) ;
#68781=CARTESIAN_POINT ( 'NONE',  ( 172.5667039024480687, -42.82844715993500273, 300.4678068554149490 ) ) ;
#68784=ORIENTED_EDGE ( 'NONE', *, *, #2706, .F. ) ;
#68785=ADVANCED_FACE ( 'NONE', ( #58295 ), #86026, .F. ) ;
#68786=CARTESIAN_POINT ( 'NONE',  ( 105.3429517235655766, -27.17434032488695550, 124.6409912566479647 ) ) ;
#68789=DIRECTION ( 'NONE',  ( -4.299999999999999979E-14, 1.000000000000000000, -4.400000000000000367E-29 ) ) ;
#68790=CARTESIAN_POINT ( 'NONE',  ( 114.2383551682309815, -44.26553795382356071, 154.1813395616249807 ) ) ;
#68791=FACE_OUTER_BOUND ( 'NONE', #49051, .T. ) ;
#68792=CARTESIAN_POINT ( 'NONE',  ( 107.0664832912739968, -18.82844715994099971, 168.9256252759119832 ) ) ;
#68794=CARTESIAN_POINT ( 'NONE',  ( 31.56670390244800828, -32.29483332968611364, 237.4678068554150059 ) ) ;
#68795=CARTESIAN_POINT ( 'NONE',  ( 109.9668656698224822, -46.07028316908886723, 97.81562527591097478 ) ) ;
#68796=ORIENTED_EDGE ( 'NONE', *, *, #15782, .F. ) ;
#68797=VERTEX_POINT ( 'NONE', #80101 ) ;
#68801=( BOUNDED_CURVE ( )  B_SPLINE_CURVE ( 3, ( #76682, #27628, #48485, #55310 ),
 .UNSPECIFIED., .F., .F. ) 
 B_SPLINE_CURVE_WITH_KNOTS ( ( 4, 4 ),
 ( 3.141592653598349827, 4.712388980395617821 ),
 .UNSPECIFIED. ) 
 CURVE ( )  GEOMETRIC_REPRESENTATION_ITEM ( )  RATIONAL_B_SPLINE_CURVE ( ( 1.000000000000000000, 0.8047378541238059402, 0.8047378541238059402, 1.000000000000000000 ) ) 
 REPRESENTATION_ITEM ( '' )  );
#68802=CARTESIAN_POINT ( 'NONE',  ( 96.28008679191522390, -39.42493101749851547, 162.5213395616249841 ) ) ;
#68803=DIRECTION ( 'NONE',  ( 0.000000000000000000, 0.000000000000000000, -1.000000000000000000 ) ) ;
#68807=CYLINDRICAL_SURFACE ( 'NONE', #21372, 0.2500000000000002220 ) ;
#68810=CARTESIAN_POINT ( 'NONE',  ( 98.35456548258453324, -42.41549619454043096, 101.7870538473399620 ) ) ;
#68813=EDGE_LOOP ( 'NONE', ( #16476, #29518, #39536, #3134 ) ) ;
#68816=LINE ( 'NONE', #49243, #59822 ) ;
#68817=EDGE_CURVE ( 'NONE', #67341, #45837, #75249, .T. ) ;
#68818=CARTESIAN_POINT ( 'NONE',  ( 114.8977050226898484, -39.03198754188770891, 181.4166617981629486 ) ) ;
#68819=VECTOR ( 'NONE', #50256, 1000.000000000000000 ) ;
#68823=DIRECTION ( 'NONE',  ( 1.387778780781444492E-15, 0.000000000000000000, -1.000000000000000000 ) ) ;
#68824=ORIENTED_EDGE ( 'NONE', *, *, #74187, .T. ) ;
#68827=LINE ( 'NONE', #41102, #3233 ) ;
#68829=VECTOR ( 'NONE', #14280, 1000.000000000000000 ) ;
#68831=ORIENTED_EDGE ( 'NONE', *, *, #2239, .T. ) ;
#68832=ORIENTED_EDGE ( 'NONE', *, *, #89275, .T. ) ;
#68834=CARTESIAN_POINT ( 'NONE',  ( 102.1597156073931671, -27.93204209654597037, 251.9130118773254026 ) ) ;
#68839=ORIENTED_EDGE ( 'NONE', *, *, #82694, .F. ) ;
#68840=EDGE_CURVE ( 'NONE', #38380, #69742, #22905, .T. ) ;
#68841=DIRECTION ( 'NONE',  ( 0.9068632946707805287, -0.4214249218767882610, 1.035655806553318316E-15 ) ) ;
#68843=ORIENTED_EDGE ( 'NONE', *, *, #30926, .T. ) ;
#68844=CARTESIAN_POINT ( 'NONE',  ( 102.1781415585801511, -43.87122846086534622, 239.9290427505439709 ) ) ;
#68845=CARTESIAN_POINT ( 'NONE',  ( 97.59689953814545049, -30.98293302709309671, 125.8803871806719599 ) ) ;
#68846=CARTESIAN_POINT ( 'NONE',  ( 98.87507392487043489, -43.19978241230797522, 91.85848241876892928 ) ) ;
#68847=CARTESIAN_POINT ( 'NONE',  ( 103.3391524833590438, -29.24345965735583519, 249.5838068554172366 ) ) ;
#68848=CARTESIAN_POINT ( 'NONE',  ( 131.6146038194016796, -17.48272374588585620, 7.134497377256392880 ) ) ;
#68849=CARTESIAN_POINT ( 'NONE',  ( 104.5626002042890974, -48.31241677248981858, 178.4070538473399665 ) ) ;
#68850=LINE ( 'NONE', #26171, #140 ) ;
#68851=ORIENTED_EDGE ( 'NONE', *, *, #306, .F. ) ;
#68853=ORIENTED_EDGE ( 'NONE', *, *, #23258, .T. ) ;
#68854=EDGE_LOOP ( 'NONE', ( #8587, #60414 ) ) ;
#68855=CARTESIAN_POINT ( 'NONE',  ( 162.8595971212720031, -23.19206098994050436, -5.074374724088000832 ) ) ;
#68858=CARTESIAN_POINT ( 'NONE',  ( 162.7131505118680082, -31.94127993907151009, 237.4678068554150059 ) ) ;
#68859=CARTESIAN_POINT ( 'NONE',  ( 102.3930168087890422, -26.71257147495026274, 135.4118157521009493 ) ) ;
#68861=VECTOR ( 'NONE', #42589, 1000.000000000000000 ) ;
#68866=CARTESIAN_POINT ( 'NONE',  ( 98.85650974919605005, -29.36329775763232774, 231.7565776568629587 ) ) ;
#68867=CARTESIAN_POINT ( 'NONE',  ( 179.7974245136200011, -36.32844715994040996, -5.074374724088000832 ) ) ;
#68868=ADVANCED_FACE ( 'NONE', ( #38737 ), #43768, .T. ) ;
#68869=DIRECTION ( 'NONE',  ( 1.000000000000000078E-15, 0.000000000000000000, 1.000000000000000000 ) ) ;
#68871=CARTESIAN_POINT ( 'NONE',  ( 182.5667039024469886, -33.35206098992650681, -5.074374724088000832 ) ) ;
#68875=DIRECTION ( 'NONE',  ( 0.000000000000000000, 0.000000000000000000, -1.000000000000000000 ) ) ;
#68877=CARTESIAN_POINT ( 'NONE',  ( 100.7233752965418034, -45.83866581990632483, 237.0803871806729717 ) ) ;
#68878=VERTEX_POINT ( 'NONE', #47329 ) ;
#68879=ADVANCED_FACE ( 'NONE', ( #54576 ), #53231, .T. ) ;
#68880=DIRECTION ( 'NONE',  ( 1.000000000000000078E-15, 1.000000000000000083E-30, -1.000000000000000000 ) ) ;
#68881=CARTESIAN_POINT ( 'NONE',  ( 109.2059698035850914, -26.50355049596284118, 139.9127681330539872 ) ) ;
#68882=CARTESIAN_POINT ( 'NONE',  ( 106.2521435260052698, -26.30072798870746453, 21.13848241876792144 ) ) ;
#68883=CARTESIAN_POINT ( 'NONE',  ( 114.4937323636162176, -28.48121435373123589, 155.5051490854349652 ) ) ;
#68885=CARTESIAN_POINT ( 'NONE',  ( 116.3185177584062444, -32.94221225046054968, 100.1356252759109680 ) ) ;
#68886=DIRECTION ( 'NONE',  ( 9.351236661543306751E-17, -3.725950533538267725E-29, -1.000000000000000000 ) ) ;
#68888=CARTESIAN_POINT ( 'NONE',  ( 107.0664832912739968, -8.729447159940999512, 6.425625275911999168 ) ) ;
#68889=CARTESIAN_POINT ( 'NONE',  ( 107.0664832912739399, -36.72944715994095333, 311.6343304127839815 ) ) ;
#68890=VERTEX_POINT ( 'NONE', #82341 ) ;
#68893=CIRCLE ( 'NONE', #29727, 4.875000000000017764 ) ;
#68894=ORIENTED_EDGE ( 'NONE', *, *, #61140, .T. ) ;
#68897=AXIS2_PLACEMENT_3D ( 'NONE', #73213, #10993, #52737 ) ;
#68899=ORIENTED_EDGE ( 'NONE', *, *, #47618, .F. ) ;
#68901=CARTESIAN_POINT ( 'NONE',  ( 97.12559377168382468, -39.79659400623918231, 17.56419670448195092 ) ) ;
#68902=CARTESIAN_POINT ( 'NONE',  ( 63.03715912545820999, -46.82818131006018092, 300.4678068554150627 ) ) ;
#68903=CARTESIAN_POINT ( 'NONE',  ( 70.14948329127297200, -1.929447159941395817, 361.9756252759109998 ) ) ;
#68904=CARTESIAN_POINT ( 'NONE',  ( 98.51568282078342520, -45.00561318155631341, 187.9384824187679612 ) ) ;
#68906=CARTESIAN_POINT ( 'NONE',  ( 102.3370036867683268, -28.24990410829322940, 254.9038483995052502 ) ) ;
#68907=ORIENTED_EDGE ( 'NONE', *, *, #87729, .F. ) ;
#68911=CARTESIAN_POINT ( 'NONE',  ( 116.5686102693484685, -33.54593647048663740, 184.0836522168384874 ) ) ;
#68913=AXIS2_PLACEMENT_3D ( 'NONE', #21624, #8893, #29771 ) ;
#68914=CARTESIAN_POINT ( 'NONE',  ( 97.06115611282805844, -37.99685616895267515, 276.4268913949732109 ) ) ;
#68915=CARTESIAN_POINT ( 'NONE',  ( 97.81151460250711693, -40.51751193867107759, 182.6359910548048333 ) ) ;
#68917=CARTESIAN_POINT ( 'NONE',  ( 108.4153195593449510, -26.73476064541128849, 174.9691313568370106 ) ) ;
#68918=CARTESIAN_POINT ( 'NONE',  ( 101.6507727546967175, -27.01955209951621129, 255.4813395616254468 ) ) ;
#68919=CARTESIAN_POINT ( 'NONE',  ( 107.0667039024479834, -36.72944715994099596, 239.5838068554170093 ) ) ;
#68920=VERTEX_POINT ( 'NONE', #87791 ) ;
#68921=CARTESIAN_POINT ( 'NONE',  ( 151.5667039024486087, -48.82844715993590512, 129.9678068554149775 ) ) ;
#68922=DIRECTION ( 'NONE',  ( -1.000000000000000000, 0.000000000000000000, 0.000000000000000000 ) ) ;
#68923=EDGE_CURVE ( 'NONE', #18950, #41648, #75512, .T. ) ;
#68924=CARTESIAN_POINT ( 'NONE',  ( 100.2074232480821365, -30.48050913114499849, 78.55666179816195438 ) ) ;
#68925=VECTOR ( 'NONE', #74545, 1000.000000000000000 ) ;
#68929=ORIENTED_EDGE ( 'NONE', *, *, #84824, .T. ) ;
#68930=CARTESIAN_POINT ( 'NONE',  ( 78.64593636903484253, -34.36767598604495788, 7.908804215170622598 ) ) ;
#68931=ORIENTED_EDGE ( 'NONE', *, *, #45954, .T. ) ;
#68932=CARTESIAN_POINT ( 'NONE',  ( 117.7037197400453437, -39.73414628438690244, 143.6194347997209775 ) ) ;
#68933=ORIENTED_EDGE ( 'NONE', *, *, #27052, .T. ) ;
#68934=CARTESIAN_POINT ( 'NONE',  ( 117.0718954842606507, -35.46248235080364708, 69.92729194301183782 ) ) ;
#68935=CARTESIAN_POINT ( 'NONE',  ( 106.2249424221556922, -46.76750045321607985, 108.9415833058969554 ) ) ;
#68936=DIRECTION ( 'NONE',  ( 1.000000000000000078E-15, -1.000000000000000083E-30, -1.000000000000000000 ) ) ;
#68937=CARTESIAN_POINT ( 'NONE',  ( 89.17003477451885374, -56.47944715994104570, -5.074374724089047106 ) ) ;
#68938=CARTESIAN_POINT ( 'NONE',  ( 117.0746561606024869, -31.98374578269911339, 60.19086337114898555 ) ) ;
#68941=EDGE_LOOP ( 'NONE', ( #10206, #45201, #3456, #62516 ) ) ;
#68942=EDGE_CURVE ( 'NONE', #75252, #66874, #69471, .T. ) ;
#68943=DIRECTION ( 'NONE',  ( -2.900000000000000265E-14, 2.000000000000000155E-15, -1.000000000000000000 ) ) ;
#68944=CIRCLE ( 'NONE', #22596, 37.00000000000000711 ) ;
#68946=VECTOR ( 'NONE', #60739, 1000.000000000000000 ) ;
#68948=VERTEX_POINT ( 'NONE', #88704 ) ;
#68950=DIRECTION ( 'NONE',  ( 1.000000000000000000, 6.145690160522480771E-16, 0.000000000000000000 ) ) ;
#68951=ORIENTED_EDGE ( 'NONE', *, *, #14907, .T. ) ;
#68952=CARTESIAN_POINT ( 'NONE',  ( 102.6689224787387502, -46.93780143634764812, 287.2527681330543601 ) ) ;
#68953=CARTESIAN_POINT ( 'NONE',  ( 97.93745859118190822, -30.45679909449765432, 161.8594347997199918 ) ) ;
#68954=DIRECTION ( 'NONE',  ( -0.1811243269279065315, 0.9834602067165264527, 0.000000000000000000 ) ) ;
#68955=CARTESIAN_POINT ( 'NONE',  ( 105.7995184936499271, -26.72403496521869215, 141.1772919420962751 ) ) ;
#68956=CARTESIAN_POINT ( 'NONE',  ( 106.6603377114791300, -26.31227224467070158, 81.10705384733896040 ) ) ;
#68957=CARTESIAN_POINT ( 'NONE',  ( 98.35059589455165963, -31.65526352089521822, 96.90576211103469007 ) ) ;
#68961=EDGE_CURVE ( 'NONE', #68284, #73560, #38980, .T. ) ;
#68963=AXIS2_PLACEMENT_3D ( 'NONE', #40954, #75936, #35034 ) ;
#68964=ORIENTED_EDGE ( 'NONE', *, *, #55495, .T. ) ;
#68965=DIRECTION ( 'NONE',  ( 1.000000000000000000, 0.000000000000000000, 0.000000000000000000 ) ) ;
#68966=FACE_OUTER_BOUND ( 'NONE', #80348, .T. ) ;
#68967=CARTESIAN_POINT ( 'NONE',  ( 115.6772654923307613, -42.56752007954070649, 273.3527681330537575 ) ) ;
#68969=VECTOR ( 'NONE', #34232, 1000.000000000000000 ) ;
#68970=CARTESIAN_POINT ( 'NONE',  ( 41.56648329127499153, -36.32844715994070839, 134.1756252759119832 ) ) ;
#68972=CARTESIAN_POINT ( 'NONE',  ( 116.1702204290647984, -31.76348745297265808, 24.21181575210196257 ) ) ;
#68973=CARTESIAN_POINT ( 'NONE',  ( 97.80409164390904664, -40.49886389222051264, 101.6344799213053136 ) ) ;
#68974=CARTESIAN_POINT ( 'NONE',  ( 101.5125196766230857, -27.93273449574876111, 106.5241967044819944 ) ) ;
#68976=CARTESIAN_POINT ( 'NONE',  ( 102.8260968645185045, -46.30158323273214904, 177.2441967044819648 ) ) ;
#68977=CARTESIAN_POINT ( 'NONE',  ( 46.48091746482130304, -49.32844715994084339, 300.4678068554150059 ) ) ;
#68982=EDGE_CURVE ( 'NONE', #43693, #2920, #26017, .T. ) ;
#68983=ORIENTED_EDGE ( 'NONE', *, *, #8162, .F. ) ;
#68985=CARTESIAN_POINT ( 'NONE',  ( 96.62682903746573970, -35.94284815129010013, 146.2670538473399517 ) ) ;
#68988=CARTESIAN_POINT ( 'NONE',  ( 114.8301775850900128, -29.68641892472961175, 205.4127681330539872 ) ) ;
#68990=CARTESIAN_POINT ( 'NONE',  ( 172.5664832912740110, -9.303447159940999356, 318.9256252759120116 ) ) ;
#68991=VECTOR ( 'NONE', #39904, 1000.000000000000000 ) ;
#68992=CARTESIAN_POINT ( 'NONE',  ( 51.23005224011598102, -33.89581943344511217, 313.9678068554150059 ) ) ;
#68995=AXIS2_PLACEMENT_3D ( 'NONE', #27865, #78285, #43275 ) ;
#68998=ADVANCED_FACE ( 'NONE', ( #46871 ), #74605, .F. ) ;
#69000=CARTESIAN_POINT ( 'NONE',  ( 107.0664832912749915, -36.72944715993903486, 25.56312527591096995 ) ) ;
#69001=CARTESIAN_POINT ( 'NONE',  ( 115.3879430501622636, -30.44965457351534255, 215.3413395616249773 ) ) ;
#69003=EDGE_CURVE ( 'NONE', #13721, #81923, #6462, .T. ) ;
#69005=PLANE ( 'NONE',  #71442 ) ;
#69013=CARTESIAN_POINT ( 'NONE',  ( 107.0664832912739968, -36.72944715994100306, 287.6356252759109680 ) ) ;
#69015=LINE ( 'NONE', #6780, #78234 ) ;
#69016=CARTESIAN_POINT ( 'NONE',  ( 97.41213207386813622, -40.51524797426102253, 242.6118157521009664 ) ) ;
#69018=CARTESIAN_POINT ( 'NONE',  ( 107.5699729851651938, -26.92841289699918050, 91.03562527591097364 ) ) ;
#69020=VECTOR ( 'NONE', #44255, 1000.000000000000000 ) ;
#69021=CARTESIAN_POINT ( 'NONE',  ( 97.31304403385813373, -38.96047841033755077, 22.50539973119484927 ) ) ;
#69022=ORIENTED_EDGE ( 'NONE', *, *, #48520, .T. ) ;
#69023=DIRECTION ( 'NONE',  ( -4.237773401492740281E-14, 1.000000000000000000, 0.000000000000000000 ) ) ;
#69024=ORIENTED_EDGE ( 'NONE', *, *, #64647, .F. ) ;
#69025=VERTEX_POINT ( 'NONE', #81452 ) ;
#69026=CIRCLE ( 'NONE', #63193, 7.799999999999994493 ) ;
#69028=CARTESIAN_POINT ( 'NONE',  ( 100.4929819111635538, -30.01635508975405031, 267.1368214011352507 ) ) ;
#69029=DIRECTION ( 'NONE',  ( -4.237773401492740281E-14, 1.000000000000000000, 0.000000000000000000 ) ) ;
#69030=CARTESIAN_POINT ( 'NONE',  ( 105.7991499238894875, -26.72408508578766018, 140.1773212550283745 ) ) ;
#69032=EDGE_CURVE ( 'NONE', #19365, #19408, #40076, .T. ) ;
#69035=ORIENTED_EDGE ( 'NONE', *, *, #16033, .T. ) ;
#69037=CARTESIAN_POINT ( 'NONE',  ( 117.0604431937161678, -38.08363390023102824, 184.7192988456124851 ) ) ;
#69039=CARTESIAN_POINT ( 'NONE',  ( 106.5180884070038161, -25.68959433010697779, 45.12800622829193742 ) ) ;
#69040=EDGE_LOOP ( 'NONE', ( #74923, #65371, #67355, #45444 ) ) ;
#69041=CARTESIAN_POINT ( 'NONE',  ( 105.4654256982276905, -28.22429988993499350, 278.0547570362579677 ) ) ;
#69042=DIRECTION ( 'NONE',  ( 0.000000000000000000, 0.000000000000000000, -1.000000000000000000 ) ) ;
#69043=CARTESIAN_POINT ( 'NONE',  ( 108.4956486572523744, -46.43878675094428843, 142.6927681330539883 ) ) ;
#69045=LINE ( 'NONE', #56284, #79188 ) ;
#69046=CARTESIAN_POINT ( 'NONE',  ( 57.56670390244735103, -42.82844715994040996, 139.7178068554150911 ) ) ;
#69048=CARTESIAN_POINT ( 'NONE',  ( 100.2197142693901668, -28.81018370247272742, 256.6441967044821695 ) ) ;
#69050=VERTEX_POINT ( 'NONE', #67793 ) ;
#69052=CARTESIAN_POINT ( 'NONE',  ( 98.42274642353920910, -30.82362014679692308, 116.8499109901969604 ) ) ;
#69053=ADVANCED_FACE ( 'NONE', ( #33273 ), #60976, .T. ) ;
#69054=DIRECTION ( 'NONE',  ( 0.000000000000000000, 1.000000000000000000, 0.000000000000000000 ) ) ;
#69055=VERTEX_POINT ( 'NONE', #61413 ) ;
#69056=ORIENTED_EDGE ( 'NONE', *, *, #65325, .F. ) ;
#69057=EDGE_LOOP ( 'NONE', ( #45512, #74663, #41337, #30651 ) ) ;
#69061=DIRECTION ( 'NONE',  ( 0.000000000000000000, -0.000000000000000000, 1.000000000000000000 ) ) ;
#69063=CARTESIAN_POINT ( 'NONE',  ( 115.2258025850914862, -39.61500320815195408, 176.3861856076869685 ) ) ;
#69064=CARTESIAN_POINT ( 'NONE',  ( 109.2164500608077873, -48.40848361911378817, 273.7213395616253706 ) ) ;
#69066=CARTESIAN_POINT ( 'NONE',  ( 98.54763480789691243, -41.97695032525800940, 57.76580044582079410 ) ) ;
#69067=ORIENTED_EDGE ( 'NONE', *, *, #67080, .F. ) ;
#69071=CARTESIAN_POINT ( 'NONE',  ( 100.8874565155974494, -44.70021274534146727, 42.05175877296590414 ) ) ;
#69072=ORIENTED_EDGE ( 'NONE', *, *, #86857, .T. ) ;
#69073=ORIENTED_EDGE ( 'NONE', *, *, #69395, .T. ) ;
#69074=EDGE_CURVE ( 'NONE', #75636, #43807, #71715, .T. ) ;
#69076=CIRCLE ( 'NONE', #56012, 29.00000000000000000 ) ;
#69080=CARTESIAN_POINT ( 'NONE',  ( 188.5667039024486087, -48.82844715993430640, 137.2178068554150059 ) ) ;
#69082=AXIS2_PLACEMENT_3D ( 'NONE', #49462, #49911, #7260 ) ;
#69083=EDGE_CURVE ( 'NONE', #71344, #37315, #75595, .T. ) ;
#69084=CARTESIAN_POINT ( 'NONE',  ( 29.56648329127298069, 15.62155284005731204, 361.9756252759109998 ) ) ;
#69086=CARTESIAN_POINT ( 'NONE',  ( 115.4440039095595409, -34.92134030032634939, 183.4181341137909556 ) ) ;
#69087=CARTESIAN_POINT ( 'NONE',  ( 118.7820429505835733, -34.63792632846725184, 48.96705384733895983 ) ) ;
#69088=DIRECTION ( 'NONE',  ( 0.7071067811874264253, -0.7071067811856686092, 7.071067811873959532E-16 ) ) ;
#69089=VERTEX_POINT ( 'NONE', #2229 ) ;
#69092=VERTEX_POINT ( 'NONE', #1333 ) ;
#69094=EDGE_LOOP ( 'NONE', ( #42773, #858 ) ) ;
#69095=CARTESIAN_POINT ( 'NONE',  ( 111.6951833200829043, -27.79749774200430323, 165.6959612989590482 ) ) ;
#69096=DIRECTION ( 'NONE',  ( -1.000000000000000000, -4.299999999999999979E-14, -1.000000000000000078E-15 ) ) ;
#69098=AXIS2_PLACEMENT_3D ( 'NONE', #37636, #37186, #64893 ) ;
#69101=CARTESIAN_POINT ( 'NONE',  ( 100.3969032678572262, -28.68811230323557027, 40.62705384733894221 ) ) ;
#69103=CARTESIAN_POINT ( 'NONE',  ( 102.0665444595604328, -27.97079262611111972, 165.4898391514462332 ) ) ;
#69104=CARTESIAN_POINT ( 'NONE',  ( 192.5667039024475002, -23.42844715993433624, 129.9678068554150343 ) ) ;
#69106=CARTESIAN_POINT ( 'NONE',  ( 131.4050152070336424, -18.03131342368210710, 2.974074870386957503 ) ) ;
#69107=ORIENTED_EDGE ( 'NONE', *, *, #59421, .T. ) ;
#69108=ADVANCED_FACE ( 'NONE', ( #23579 ), #44426, .T. ) ;
#69109=DIRECTION ( 'NONE',  ( 1.000000000000000000, 0.000000000000000000, 0.000000000000000000 ) ) ;
#69110=ADVANCED_FACE ( 'NONE', ( #50812 ), #78549, .T. ) ;
#69111=EDGE_CURVE ( 'NONE', #11696, #23732, #34388, .T. ) ;
#69113=FACE_OUTER_BOUND ( 'NONE', #80881, .T. ) ;
#69115=CARTESIAN_POINT ( 'NONE',  ( 118.8673094125028200, -35.40175986820349152, 79.91562527591095488 ) ) ;
#69116=EDGE_CURVE ( 'NONE', #70690, #86125, #45318, .T. ) ;
#69117=CARTESIAN_POINT ( 'NONE',  ( 31.56670390244800828, -32.29483332968611364, 313.9678068554150059 ) ) ;
#69119=LINE ( 'NONE', #77277, #33556 ) ;
#69120=DIRECTION ( 'NONE',  ( 1.000000000000000000, 4.163336342344333240E-14, 0.000000000000000000 ) ) ;
#69122=CARTESIAN_POINT ( 'NONE',  ( 101.2684584845352163, -45.32493232151062301, 148.0918157521009562 ) ) ;
#69124=VERTEX_POINT ( 'NONE', #44883 ) ;
#69125=CARTESIAN_POINT ( 'NONE',  ( 114.3996560367811099, -27.45190519937929707, 270.5441967044823741 ) ) ;
#69126=CARTESIAN_POINT ( 'NONE',  ( 97.92284106446184921, -40.77982016931672149, 252.6583389871856582 ) ) ;
#69127=DIRECTION ( 'NONE',  ( 0.000000000000000000, 0.000000000000000000, -1.000000000000000000 ) ) ;
#69128=DIRECTION ( 'NONE',  ( -0.9825752044165969590, -0.1858654558159821002, 0.000000000000000000 ) ) ;
#69130=DIRECTION ( 'NONE',  ( 1.000000000000000078E-15, -1.000000000000000083E-30, -1.000000000000000000 ) ) ;
#69131=CARTESIAN_POINT ( 'NONE',  ( 107.0664832912739968, -36.72944715994100306, 287.6356252759109680 ) ) ;
#69132=AXIS2_PLACEMENT_3D ( 'NONE', #70633, #49721, #36107 ) ;
#69133=CARTESIAN_POINT ( 'NONE',  ( 104.6152064257953498, -27.26083179018618452, 200.2784824187689310 ) ) ;
#69135=ORIENTED_EDGE ( 'NONE', *, *, #80515, .T. ) ;
#69136=AXIS2_PLACEMENT_3D ( 'NONE', #76856, #13291, #68701 ) ;
#69137=CARTESIAN_POINT ( 'NONE',  ( 116.1725082674369816, -34.41496348756209755, 165.4682499725639957 ) ) ;
#69139=DIRECTION ( 'NONE',  ( 0.000000000000000000, 0.000000000000000000, 1.000000000000000000 ) ) ;
#69140=CARTESIAN_POINT ( 'NONE',  ( 105.9660761217308931, -46.48152529548401901, 278.4870538473389843 ) ) ;
#69141=CARTESIAN_POINT ( 'NONE',  ( 97.78478700746286734, -40.45111962689370699, 57.62993004767697158 ) ) ;
#69142=VECTOR ( 'NONE', #10383, 1000.000000000000000 ) ;
#69143=DIRECTION ( 'NONE',  ( 1.000000000000000078E-15, -1.000000000000000083E-30, -1.000000000000000000 ) ) ;
#69145=CARTESIAN_POINT ( 'NONE',  ( 162.8913605087219878, -31.76306994223740432, 193.9678068554150059 ) ) ;
#69146=CARTESIAN_POINT ( 'NONE',  ( 97.06107109826302803, -37.99641197210306132, 107.4272919432525413 ) ) ;
#69148=CARTESIAN_POINT ( 'NONE',  ( 103.6457867198658107, -26.24313906103844474, 210.3394347997209763 ) ) ;
#69154=CARTESIAN_POINT ( 'NONE',  ( 193.5667039024483529, -48.82844715993410034, 300.4678068554149490 ) ) ;
#69155=CARTESIAN_POINT ( 'NONE',  ( 73.17003668186727339, -8.979447159941065237, 14.92562527591093691 ) ) ;
#69156=VECTOR ( 'NONE', #53273, 1000.000000000000000 ) ;
#69157=CARTESIAN_POINT ( 'NONE',  ( 36.74138383868079671, -48.33240602328870494, 180.4678068554150911 ) ) ;
#69158=EDGE_LOOP ( 'NONE', ( #53985, #60397 ) ) ;
#69159=CARTESIAN_POINT ( 'NONE',  ( 117.4276745381585556, -38.22567431247780689, 24.71276813305395237 ) ) ;
#69160=ADVANCED_FACE ( 'NONE', ( #9937 ), #72610, .T. ) ;
#69161=CARTESIAN_POINT ( 'NONE',  ( 109.9893001866846163, -26.72224116339410571, 259.8499109901965767 ) ) ;
#69164=ADVANCED_FACE ( 'NONE', ( #59844 ), #73035, .T. ) ;
#69165=DIRECTION ( 'NONE',  ( -4.237773401492740281E-14, 1.000000000000000000, 0.000000000000000000 ) ) ;
#69166=CARTESIAN_POINT ( 'NONE',  ( -18.39335205926253280, -13.32818131006344231, 237.4678068554150059 ) ) ;
#69167=CARTESIAN_POINT ( 'NONE',  ( 112.0854389607193724, -45.38515269226328996, 167.9946301825848138 ) ) ;
#69168=CARTESIAN_POINT ( 'NONE',  ( 99.12746238500623974, -38.62725459667914407, 54.33094751244893672 ) ) ;
#69169=CARTESIAN_POINT ( 'NONE',  ( 117.8014899757583578, -34.00092425788908912, 165.0365776568629315 ) ) ;
#69172=ORIENTED_EDGE ( 'NONE', *, *, #79126, .F. ) ;
#69173=EDGE_CURVE ( 'NONE', #51938, #53561, #80769, .T. ) ;
#69174=DIRECTION ( 'NONE',  ( -0.7071067811865192621, -0.7071067811865758834, -7.071067811865186413E-16 ) ) ;
#69177=ADVANCED_FACE ( 'NONE', ( #39415 ), #4903, .T. ) ;
#69178=PLANE ( 'NONE',  #22756 ) ;
#69180=ORIENTED_EDGE ( 'NONE', *, *, #57066, .F. ) ;
#69181=DIRECTION ( 'NONE',  ( -1.000000000000000078E-15, 1.000000000000000083E-30, 1.000000000000000000 ) ) ;
#69182=EDGE_CURVE ( 'NONE', #68582, #1430, #34502, .T. ) ;
#69183=CARTESIAN_POINT ( 'NONE',  ( 104.6424027498074025, -44.91968313032340632, 106.7695626852199808 ) ) ;
#69184=CARTESIAN_POINT ( 'NONE',  ( 98.88149684619317270, -29.26610755689610599, 230.7261014663869503 ) ) ;
#69185=CARTESIAN_POINT ( 'NONE',  ( 98.39792771585416631, -29.90889243069706538, 200.8080062282919869 ) ) ;
#69186=CARTESIAN_POINT ( 'NONE',  ( 100.9539191370902387, -46.85292318231929443, 48.14419670448194211 ) ) ;
#69188=CARTESIAN_POINT ( 'NONE',  ( 116.8183557169515154, -34.15769664919192650, 95.03106952027322052 ) ) ;
#69189=EDGE_CURVE ( 'NONE', #75973, #49111, #21224, .T. ) ;
#69190=CIRCLE ( 'NONE', #51788, 0.5000000000000004441 ) ;
#69191=ORIENTED_EDGE ( 'NONE', *, *, #4382, .T. ) ;
#69192=AXIS2_PLACEMENT_3D ( 'NONE', #74428, #5845, #33533 ) ;
#69193=EDGE_CURVE ( 'NONE', #28735, #15500, #13066, .T. ) ;
#69194=CARTESIAN_POINT ( 'NONE',  ( 108.2018929880948832, -26.98138995270364759, 129.9841967044829687 ) ) ;
#69195=CARTESIAN_POINT ( 'NONE',  ( 112.7839950898761288, -27.91685089337277503, 69.61848241876793963 ) ) ;
#69197=CARTESIAN_POINT ( 'NONE',  ( 103.9260401568723324, -26.74224119611745820, 250.3184824187677577 ) ) ;
#69198=VERTEX_POINT ( 'NONE', #83015 ) ;
#69200=CARTESIAN_POINT ( 'NONE',  ( 100.6375269748662760, -26.77409651225141474, 220.5327681330539633 ) ) ;
#69201=CYLINDRICAL_SURFACE ( 'NONE', #38415, 3.249999999999975131 ) ;
#69203=CARTESIAN_POINT ( 'NONE',  ( 83.06670390244804025, -43.72944715994108122, 207.5838068554169809 ) ) ;
#69204=DIRECTION ( 'NONE',  ( 0.000000000000000000, 0.000000000000000000, -1.000000000000000000 ) ) ;
#69205=DIRECTION ( 'NONE',  ( -1.000000000000000000, 0.000000000000000000, -1.000000000000000078E-15 ) ) ;
#69207=PLANE ( 'NONE',  #11889 ) ;
#69208=CARTESIAN_POINT ( 'NONE',  ( 163.0664832912739826, 25.62155284005901379, 333.4006252759110112 ) ) ;
#69210=DIRECTION ( 'NONE',  ( 0.000000000000000000, 0.000000000000000000, -1.000000000000000000 ) ) ;
#69211=CARTESIAN_POINT ( 'NONE',  ( 142.8841478025725849, -84.11588139007199061, 396.9756252759102040 ) ) ;
#69212=CYLINDRICAL_SURFACE ( 'NONE', #57931, 5.499999999999999112 ) ;
#69213=EDGE_CURVE ( 'NONE', #9112, #12734, #89832, .T. ) ;
#69216=DIRECTION ( 'NONE',  ( -2.900000000000000265E-14, 2.000000000000000155E-15, -1.000000000000000000 ) ) ;
#69217=CARTESIAN_POINT ( 'NONE',  ( 105.1048729065459355, -25.82772592887830854, 275.2061014663870537 ) ) ;
#69218=CARTESIAN_POINT ( 'NONE',  ( 114.5275249938671465, -28.57771476791114296, 150.4746728949579619 ) ) ;
#69219=CARTESIAN_POINT ( 'NONE',  ( 111.8841015539045713, -46.06371569386821818, 268.9556252759110180 ) ) ;
#69220=CIRCLE ( 'NONE', #24289, 15.84999999999999964 ) ;
#69221=EDGE_CURVE ( 'NONE', #87720, #28273, #53912, .T. ) ;
#69222=CARTESIAN_POINT ( 'NONE',  ( 73.17003668186728760, -8.979447159941065237, -5.074374724089063982 ) ) ;
#69224=LINE ( 'NONE', #67876, #20315 ) ;
#69225=CARTESIAN_POINT ( 'NONE',  ( 32.16397622746000451, -34.03355364505800651, -5.074374724088000832 ) ) ;
#69226=CARTESIAN_POINT ( 'NONE',  ( 97.82719644921415636, -40.55510830976606229, 137.6388683552902137 ) ) ;
#69227=DIRECTION ( 'NONE',  ( -1.000000000000000078E-15, 0.000000000000000000, -1.000000000000000000 ) ) ;
#69228=VECTOR ( 'NONE', #83385, 1000.000000000000000 ) ;
#69229=EDGE_LOOP ( 'NONE', ( #50622, #81261 ) ) ;
#69231=ORIENTED_EDGE ( 'NONE', *, *, #45632, .F. ) ;
#69234=CARTESIAN_POINT ( 'NONE',  ( 110.6311418553464279, -45.76071711580824086, 172.2981341137909794 ) ) ;
#69235=DIRECTION ( 'NONE',  ( 0.7071067811869259367, -0.7071067811861692087, 2.899137802863410076E-29 ) ) ;
#69236=ORIENTED_EDGE ( 'NONE', *, *, #71341, .T. ) ;
#69237=CARTESIAN_POINT ( 'NONE',  ( 107.0664832912730020, -36.72944715994189835, 361.9756252759109998 ) ) ;
#69238=CARTESIAN_POINT ( 'NONE',  ( 108.3633857348901159, -47.68307073960293963, 158.6822919425779617 ) ) ;
#69239=DIRECTION ( 'NONE',  ( -0.9068632946707805287, 0.4214249218767882610, -9.068632946707800501E-16 ) ) ;
#69240=CARTESIAN_POINT ( 'NONE',  ( 80.06648329127398256, -18.72944715994105991, 14.92562527591094224 ) ) ;
#69243=CARTESIAN_POINT ( 'NONE',  ( 110.8343066518040416, -26.26926122352943338, 99.80133956162498521 ) ) ;
#69245=VERTEX_POINT ( 'NONE', #67571 ) ;
#69250=CARTESIAN_POINT ( 'NONE',  ( 112.4269750522866076, -44.91043508143932428, 174.0384824187679556 ) ) ;
#69251=CARTESIAN_POINT ( 'NONE',  ( 107.0664832912739968, -36.72944715994100306, 292.6356252759106837 ) ) ;
#69252=CARTESIAN_POINT ( 'NONE',  ( 108.4182423179703392, -26.73513332281806854, 54.96773263005526644 ) ) ;
#69254=CARTESIAN_POINT ( 'NONE',  ( 107.0667039024480260, -36.72944715994100306, 199.5838068554169809 ) ) ;
#69255=FACE_OUTER_BOUND ( 'NONE', #30072, .T. ) ;
#69257=CARTESIAN_POINT ( 'NONE',  ( 106.0785370228624913, -48.51385081415340750, 112.5099109901969712 ) ) ;
#69258=ORIENTED_EDGE ( 'NONE', *, *, #83635, .F. ) ;
#69261=DIRECTION ( 'NONE',  ( 0.000000000000000000, 0.000000000000000000, 1.000000000000000000 ) ) ;
#69263=FACE_OUTER_BOUND ( 'NONE', #26145, .T. ) ;
#69264=CARTESIAN_POINT ( 'NONE',  ( 98.98344471881878803, -35.59181213353920725, 179.0338046553059712 ) ) ;
#69265=EDGE_CURVE ( 'NONE', #7678, #18507, #72196, .T. ) ;
#69268=DIRECTION ( 'NONE',  ( 0.000000000000000000, 0.000000000000000000, -1.000000000000000000 ) ) ;
#69269=AXIS2_PLACEMENT_3D ( 'NONE', #75642, #28370, #68823 ) ;
#69273=EDGE_LOOP ( 'NONE', ( #85030, #57436, #17343, #75948 ) ) ;
#69274=ORIENTED_EDGE ( 'NONE', *, *, #13593, .F. ) ;
#69276=EDGE_CURVE ( 'NONE', #8408, #41728, #48440, .T. ) ;
#69277=CARTESIAN_POINT ( 'NONE',  ( 107.0664832912739399, -36.72944715994096754, 296.0306255462182321 ) ) ;
#69278=ORIENTED_EDGE ( 'NONE', *, *, #20090, .F. ) ;
#69279=ORIENTED_EDGE ( 'NONE', *, *, #46486, .F. ) ;
#69280=CARTESIAN_POINT ( 'NONE',  ( 21.56670390244726576, -23.42844715994183957, 300.4678068554150059 ) ) ;
#69281=CARTESIAN_POINT ( 'NONE',  ( 110.5184084024339626, -28.56779955429167472, 241.1901547344679670 ) ) ;
#69283=VERTEX_POINT ( 'NONE', #76179 ) ;
#69284=AXIS2_PLACEMENT_3D ( 'NONE', #68255, #13287, #54133 ) ;
#69285=CONICAL_SURFACE ( 'NONE', #77988, 17.36499999999999844, 0.7853981633974490562 ) ;
#69288=ORIENTED_EDGE ( 'NONE', *, *, #50555, .F. ) ;
#69290=VECTOR ( 'NONE', #25777, 1000.000000000000000 ) ;
#69291=ADVANCED_FACE ( 'NONE', ( #13510 ), #89372, .F. ) ;
#69292=CARTESIAN_POINT ( 'NONE',  ( 83.06670390244796920, -61.87844715994100397, 207.5838068554149913 ) ) ;
#69294=ORIENTED_EDGE ( 'NONE', *, *, #1410, .F. ) ;
#69295=EDGE_CURVE ( 'NONE', #8752, #65418, #6250, .T. ) ;
#69296=CARTESIAN_POINT ( 'NONE',  ( 106.3397725667592368, -45.35341472531973750, 260.3157094172105417 ) ) ;
#69297=CARTESIAN_POINT ( 'NONE',  ( 117.6033054121008945, -33.31318886634804954, 134.0880062282919880 ) ) ;
#69298=CARTESIAN_POINT ( 'NONE',  ( 107.9437834512411598, -25.73425880284244016, 115.0251490854349612 ) ) ;
#69299=CARTESIAN_POINT ( 'NONE',  ( 101.2293520222977747, -30.88460422255789695, 249.5838068554171798 ) ) ;
#69300=LINE ( 'NONE', #54285, #23483 ) ;
#69301=CARTESIAN_POINT ( 'NONE',  ( 98.43498668633466764, -29.82501040932825020, 191.7775300378159784 ) ) ;
#69302=DIRECTION ( 'NONE',  ( 1.000000000000000078E-15, -1.000000000000000083E-30, -1.000000000000000000 ) ) ;
#69303=CARTESIAN_POINT ( 'NONE',  ( 97.06111640307527466, -37.99664788389067382, 127.4273107009638295 ) ) ;
#69304=ORIENTED_EDGE ( 'NONE', *, *, #72051, .F. ) ;
#69305=DIRECTION ( 'NONE',  ( 0.000000000000000000, 1.000000000000000000, 0.000000000000000000 ) ) ;
#69306=VERTEX_POINT ( 'NONE', #26237 ) ;
#69308=VERTEX_POINT ( 'NONE', #13953 ) ;
#69309=CARTESIAN_POINT ( 'NONE',  ( 156.5667039024483529, -48.82844715993569196, 290.7178068554149490 ) ) ;
#69312=CARTESIAN_POINT ( 'NONE',  ( 113.8435853237685933, -28.76095960330615142, 139.5156252759109634 ) ) ;
#69315=DIRECTION ( 'NONE',  ( 1.000000000000000078E-15, -1.000000000000000083E-30, -1.000000000000000000 ) ) ;
#69316=LINE ( 'NONE', #1632, #66520 ) ;
#69317=CARTESIAN_POINT ( 'NONE',  ( 97.81257721367181546, -40.51959608142212943, 56.63539486199441342 ) ) ;
#69318=CARTESIAN_POINT ( 'NONE',  ( 107.2488531970940073, -24.90511003128411360, 226.0641967044829812 ) ) ;
#69320=CARTESIAN_POINT ( 'NONE',  ( 126.8164832912740110, -54.62589567669621005, 14.92562527591099020 ) ) ;
#69322=LINE ( 'NONE', #82966, #22258 ) ;
#69323=DIRECTION ( 'NONE',  ( 1.000000000000000078E-15, -1.000000000000000083E-30, -1.000000000000000000 ) ) ;
#69324=CYLINDRICAL_SURFACE ( 'NONE', #21229, 5.599999999999994316 ) ;
#69325=LINE ( 'NONE', #81634, #15798 ) ;
#69326=CARTESIAN_POINT ( 'NONE',  ( 100.1483249706684546, -45.40999835672980112, 272.0289586092442278 ) ) ;
#69327=VERTEX_POINT ( 'NONE', #60744 ) ;
#69328=CARTESIAN_POINT ( 'NONE',  ( 107.0664832912739968, -36.72944715994100306, 287.6356252759109680 ) ) ;
#69329=CARTESIAN_POINT ( 'NONE',  ( 108.9491902927665734, -26.41713524962505133, 164.9327681330529742 ) ) ;
#69330=CARTESIAN_POINT ( 'NONE',  ( 112.1812230000633832, -27.60471316448668588, 30.66991099019694644 ) ) ;
#69331=CARTESIAN_POINT ( 'NONE',  ( 95.26251351713513316, -38.28569616102737427, 147.4299109901969871 ) ) ;
#69332=AXIS2_PLACEMENT_3D ( 'NONE', #43592, #57681, #63609 ) ;
#69333=CARTESIAN_POINT ( 'NONE',  ( 115.0889047114336847, -30.61763666118805460, 30.34395861100747283 ) ) ;
#69334=EDGE_CURVE ( 'NONE', #29733, #45890, #74841, .T. ) ;
#69336=DIRECTION ( 'NONE',  ( 0.000000000000000000, 1.000000000000000000, 0.000000000000000000 ) ) ;
#69338=DIRECTION ( 'NONE',  ( 1.000000000000000078E-15, -1.000000000000000000, 0.000000000000000000 ) ) ;
#69339=CARTESIAN_POINT ( 'NONE',  ( 57.56670390244747892, -48.82844715994040286, 139.7178068554150911 ) ) ;
#69340=ORIENTED_EDGE ( 'NONE', *, *, #24465, .F. ) ;
#69341=AXIS2_PLACEMENT_3D ( 'NONE', #404, #83098, #56700 ) ;
#69342=VECTOR ( 'NONE', #3729, 1000.000000000000000 ) ;
#69343=( BOUNDED_CURVE ( )  B_SPLINE_CURVE ( 3, ( #44613, #51865, #25524, #52742 ),
 .UNSPECIFIED., .F., .T. ) 
 B_SPLINE_CURVE_WITH_KNOTS ( ( 4, 4 ),
 ( 4.646092198350402214, 4.710762098922305796 ),
 .UNSPECIFIED. ) 
 CURVE ( )  GEOMETRIC_REPRESENTATION_ITEM ( )  RATIONAL_B_SPLINE_CURVE ( ( 1.000000000000000000, 0.9996515140281859724, 0.9996515140281859724, 1.000000000000000000 ) ) 
 REPRESENTATION_ITEM ( '' )  );
#69344=ORIENTED_EDGE ( 'NONE', *, *, #49692, .T. ) ;
#69346=AXIS2_PLACEMENT_3D ( 'NONE', #8496, #50706, #77533 ) ;
#69347=ORIENTED_EDGE ( 'NONE', *, *, #49577, .F. ) ;
#69348=CARTESIAN_POINT ( 'NONE',  ( 104.0490797691970073, -47.33883444496879633, 63.36800622829197494 ) ) ;
#69349=LINE ( 'NONE', #42960, #26667 ) ;
#69352=EDGE_CURVE ( 'NONE', #79236, #87720, #69373, .T. ) ;
#69353=CARTESIAN_POINT ( 'NONE',  ( 113.7132347973738575, -45.61866494189415988, 184.0994347997199725 ) ) ;
#69354=AXIS2_PLACEMENT_3D ( 'NONE', #43989, #71724, #72617 ) ;
#69356=AXIS2_PLACEMENT_3D ( 'NONE', #39577, #46377, #10979 ) ;
#69357=CARTESIAN_POINT ( 'NONE',  ( 105.2812310726300922, -46.37359664056156561, 12.42991099019696932 ) ) ;
#69360=EDGE_LOOP ( 'NONE', ( #58050, #32011 ) ) ;
#69361=VECTOR ( 'NONE', #24783, 1000.000000000000000 ) ;
#69363=FACE_OUTER_BOUND ( 'NONE', #87106, .T. ) ;
#69365=FACE_OUTER_BOUND ( 'NONE', #43471, .T. ) ;
#69366=CARTESIAN_POINT ( 'NONE',  ( 97.33757460489749747, -34.07214903665462202, 276.1144460151012368 ) ) ;
#69367=DIRECTION ( 'NONE',  ( 0.000000000000000000, 0.000000000000000000, -1.000000000000000000 ) ) ;
#69368=DIRECTION ( 'NONE',  ( -0.7071067811865171526, -0.7071067811865779928, -7.071067811865164719E-16 ) ) ;
#69370=CARTESIAN_POINT ( 'NONE',  ( 105.3240584539683766, -26.47319898023375728, 15.20991099019697401 ) ) ;
#69371=DIRECTION ( 'NONE',  ( 3.999999999999999995E-14, -1.000000000000000000, 4.100000000000000342E-29 ) ) ;
#69372=ORIENTED_EDGE ( 'NONE', *, *, #64339, .F. ) ;
#69373=LINE ( 'NONE', #61199, #46094 ) ;
#69375=PLANE ( 'NONE',  #81587 ) ;
#69376=CARTESIAN_POINT ( 'NONE',  ( 107.1962421797556289, -28.07588791089852265, 77.89475703625792846 ) ) ;
#69377=CIRCLE ( 'NONE', #72296, 2.117000000000007987 ) ;
#69378=CARTESIAN_POINT ( 'NONE',  ( 163.0664832912739826, -0.2185775633789972805, 330.8831252759119934 ) ) ;
#69379=EDGE_CURVE ( 'NONE', #57152, #54835, #16207, .T. ) ;
#69380=CARTESIAN_POINT ( 'NONE',  ( 72.31648329127402519, -36.72944715994106701, -4.824374724089063982 ) ) ;
#69382=ORIENTED_EDGE ( 'NONE', *, *, #34700, .F. ) ;
#69383=DIRECTION ( 'NONE',  ( 0.000000000000000000, 0.000000000000000000, -1.000000000000000000 ) ) ;
#69384=EDGE_CURVE ( 'NONE', #1305, #65168, #32125, .T. ) ;
#69385=ORIENTED_EDGE ( 'NONE', *, *, #53322, .T. ) ;
#69386=CARTESIAN_POINT ( 'NONE',  ( 98.00691293156391737, -30.39673331971502179, 160.8289586092449497 ) ) ;
#69388=CARTESIAN_POINT ( 'NONE',  ( 113.1782937928648352, -44.75186857568589716, 69.09395861141521777 ) ) ;
#69389=CARTESIAN_POINT ( 'NONE',  ( 107.8658914883948512, -27.90296577952642210, 151.4358690201829631 ) ) ;
#69391=CARTESIAN_POINT ( 'NONE',  ( 99.66264782090949836, -39.75983002812326106, 9.635625275910941312 ) ) ;
#69392=CARTESIAN_POINT ( 'NONE',  ( 113.4728825864854116, -46.72846204934055692, 64.02991099019695298 ) ) ;
#69395=EDGE_CURVE ( 'NONE', #34249, #19610, #60560, .T. ) ;
#69396=CIRCLE ( 'NONE', #12802, 2.999999999999919176 ) ;
#69398=EDGE_LOOP ( 'NONE', ( #49368, #61014, #1133, #441 ) ) ;
#69401=AXIS2_PLACEMENT_3D ( 'NONE', #80008, #10939, #59073 ) ;
#69402=DIRECTION ( 'NONE',  ( -6.524622321627019585E-16, -4.013151879589939944E-16, -1.000000000000000000 ) ) ;
#69404=CARTESIAN_POINT ( 'NONE',  ( 110.7503262618283344, -45.78994064700705735, 282.8841967044829744 ) ) ;
#69405=CARTESIAN_POINT ( 'NONE',  ( 117.1470005940874728, -33.86231210335883901, 145.0470538473399529 ) ) ;
#69406=DIRECTION ( 'NONE',  ( 1.000000000000000078E-15, 1.000000000000000083E-30, -1.000000000000000000 ) ) ;
#69407=CARTESIAN_POINT ( 'NONE',  ( 117.0723825543308294, -35.46652509195462954, 129.9269704041947762 ) ) ;
#69408=CARTESIAN_POINT ( 'NONE',  ( 116.5333143132291269, -32.36348817604392991, 100.1699109901969535 ) ) ;
#69409=CARTESIAN_POINT ( 'NONE',  ( 116.3162594664470788, -32.94075446336835000, 20.13562527591095019 ) ) ;
#69410=ORIENTED_EDGE ( 'NONE', *, *, #67758, .T. ) ;
#69412=PLANE ( 'NONE',  #62700 ) ;
#69414=DIRECTION ( 'NONE',  ( -4.237773401492740281E-14, 1.000000000000000000, 0.000000000000000000 ) ) ;
#69415=EDGE_LOOP ( 'NONE', ( #55051, #43348, #79511, #8140, #1853, #65045, #18410, #53432, #21927, #30682, #80323, #72367 ) ) ;
#69416=CARTESIAN_POINT ( 'NONE',  ( 163.0959832912742797, -23.42844715993517113, 193.9678068554149775 ) ) ;
#69418=CARTESIAN_POINT ( 'NONE',  ( 96.68905559037375497, -32.92312794843576995, 21.03467289495897319 ) ) ;
#69420=DIRECTION ( 'NONE',  ( -0.000000000000000000, -0.000000000000000000, -1.000000000000000000 ) ) ;
#69422=CARTESIAN_POINT ( 'NONE',  ( 106.1055101188695602, -45.24582830394255240, 281.9095626852197825 ) ) ;
#69423=CYLINDRICAL_SURFACE ( 'NONE', #33268, 29.00000000000000000 ) ;
#69424=CARTESIAN_POINT ( 'NONE',  ( 114.6914383512287543, -44.69963429152225132, 109.1718157521009687 ) ) ;
#69425=DIRECTION ( 'NONE',  ( 0.000000000000000000, 0.000000000000000000, -1.000000000000000000 ) ) ;
#69426=CARTESIAN_POINT ( 'NONE',  ( 117.2401079361024898, -34.25881411750412298, 209.0156252759109634 ) ) ;
#69427=LINE ( 'NONE', #40367, #42328 ) ;
#69435=CARTESIAN_POINT ( 'NONE',  ( 96.00724586008001893, -35.77752748456175169, 186.2461014663869889 ) ) ;
#69438=CARTESIAN_POINT ( 'NONE',  ( 103.6314581395739793, -26.19921411638948427, 206.3394347997209763 ) ) ;
#69440=EDGE_CURVE ( 'NONE', #77124, #81899, #88152, .T. ) ;
#69443=B_SPLINE_CURVE_WITH_KNOTS ( 'NONE', 3,
 ( #79311, #85682, #11130, #73812, #38836, #52439, #66542, #51564, #65652, #87004, #73359, #3436, #86564, #66993, #37953, #3880, #4775, #65218, #10251, #11597, #52868, #51998, #86120, #17069, #72037, #17516, #45624, #2993, #31571, #45196, #32461 ),
 .UNSPECIFIED., .F., .F.,
 ( 4, 2, 2, 1, 2, 2, 2, 2, 2, 2, 2, 1, 1, 2, 2, 2, 4 ),
 ( 0.000000000000000000, 0.1250000000000044409, 0.1875000000000065226, 0.2187500000000075773, 0.2343750000000083267, 0.2500000000000090483, 0.3750000000000039968, 0.4375000000000053846, 0.5000000000000067724, 0.6250000000000158762, 0.6875000000000174305, 0.7187500000000174305, 0.7343750000000156541, 0.7421875000000148770, 0.7500000000000142109, 0.8750000000000071054, 1.000000000000000000 ),
 .UNSPECIFIED. ) ;
#69446=EDGE_CURVE ( 'NONE', #32225, #54314, #18553, .T. ) ;
#69448=EDGE_LOOP ( 'NONE', ( #54757, #49466, #25268, #22575 ) ) ;
#69449=ORIENTED_EDGE ( 'NONE', *, *, #72969, .T. ) ;
#69451=CARTESIAN_POINT ( 'NONE',  ( 96.68218458626328982, -35.80812861978466799, 227.2556252759109725 ) ) ;
#69455=DIRECTION ( 'NONE',  ( -4.237773401492740281E-14, 1.000000000000000000, 0.000000000000000000 ) ) ;
#69456=DIRECTION ( 'NONE',  ( -4.554376769437570034E-14, 1.000000000000000000, 0.000000000000000000 ) ) ;
#69458=CARTESIAN_POINT ( 'NONE',  ( 99.74655714901966519, -44.23324885335900802, 21.96133956162593748 ) ) ;
#69462=VERTEX_POINT ( 'NONE', #29834 ) ;
#69465=CARTESIAN_POINT ( 'NONE',  ( 105.8007643231009496, -26.72386559662977845, 16.18055911409852854 ) ) ;
#69466=CARTESIAN_POINT ( 'NONE',  ( 116.8310051202517457, -36.16593252570071115, 224.8727681330539667 ) ) ;
#69467=FACE_OUTER_BOUND ( 'NONE', #16777, .T. ) ;
#69468=VECTOR ( 'NONE', #35639, 1000.000000000000000 ) ;
#69469=CARTESIAN_POINT ( 'NONE',  ( 110.8343066518039990, -26.26926122352955062, 95.80133956162396203 ) ) ;
#69470=DIRECTION ( 'NONE',  ( -0.9254794337955620787, -0.3787978585227822492, 0.000000000000000000 ) ) ;
#69471=CIRCLE ( 'NONE', #65125, 1.000000000000000888 ) ;
#69474=FACE_OUTER_BOUND ( 'NONE', #12266, .T. ) ;
#69475=AXIS2_PLACEMENT_3D ( 'NONE', #22983, #14371, #1183 ) ;
#69476=ORIENTED_EDGE ( 'NONE', *, *, #3030, .F. ) ;
#69477=ORIENTED_EDGE ( 'NONE', *, *, #75222, .F. ) ;
#69479=CARTESIAN_POINT ( 'NONE',  ( 114.0851551000824600, -43.95502333027237540, 264.6215833058971043 ) ) ;
#69480=CARTESIAN_POINT ( 'NONE',  ( 163.0664832912739826, 0.2215528400590083269, 336.6506252759110112 ) ) ;
#69481=CARTESIAN_POINT ( 'NONE',  ( 138.8167039024479834, -50.82844715994100682, 86.31780685541500020 ) ) ;
#69486=ORIENTED_EDGE ( 'NONE', *, *, #13956, .T. ) ;
#69488=ORIENTED_EDGE ( 'NONE', *, *, #72506, .F. ) ;
#69489=CARTESIAN_POINT ( 'NONE',  ( 115.7287795988047634, -43.59557489936061359, 48.30514908543492680 ) ) ;
#69490=ORIENTED_EDGE ( 'NONE', *, *, #40637, .F. ) ;
#69492=CARTESIAN_POINT ( 'NONE',  ( 110.5225122084979574, -28.79501634926980458, 282.5557094172103803 ) ) ;
#69494=CARTESIAN_POINT ( 'NONE',  ( 97.28849942844331622, -36.49606577720025768, 196.3070538473399438 ) ) ;
#69496=ADVANCED_FACE ( 'NONE', ( #35281 ), #29386, .T. ) ;
#69497=CARTESIAN_POINT ( 'NONE',  ( 75.25757238336808541, -1.944390235229870978, 361.9756252759101471 ) ) ;
#69498=FACE_OUTER_BOUND ( 'NONE', #15573, .T. ) ;
#69501=CARTESIAN_POINT ( 'NONE',  ( 96.47406283524195203, -31.30618784601239923, 241.9499109901969689 ) ) ;
#69503=ORIENTED_EDGE ( 'NONE', *, *, #68087, .T. ) ;
#69504=CARTESIAN_POINT ( 'NONE',  ( 136.6795104150274653, -37.60592655294975373, 6.943955837751754068 ) ) ;
#69505=ORIENTED_EDGE ( 'NONE', *, *, #51821, .T. ) ;
#69506=CARTESIAN_POINT ( 'NONE',  ( 108.2817482635038147, -26.29579267872783177, 125.9841967044819597 ) ) ;
#69510=ORIENTED_EDGE ( 'NONE', *, *, #38046, .T. ) ;
#69512=CARTESIAN_POINT ( 'NONE',  ( 117.0608945203887572, -38.08045315175083090, 123.7189586067809017 ) ) ;
#69513=CARTESIAN_POINT ( 'NONE',  ( 109.7248724210130462, -27.00080708520160044, 265.8647914069468925 ) ) ;
#69516=CARTESIAN_POINT ( 'NONE',  ( 194.5667039024479834, -40.82844715993405771, 300.4678068554149490 ) ) ;
#69517=DIRECTION ( 'NONE',  ( 0.7071067811868672059, 0.7071067811862279395, -2.899137802863419044E-29 ) ) ;
#69518=CARTESIAN_POINT ( 'NONE',  ( 115.0725392204758890, -35.00151292932243052, 181.8138046553059723 ) ) ;
#69519=CARTESIAN_POINT ( 'NONE',  ( 115.6732227570775819, -30.74586734987101622, 275.3099109901965562 ) ) ;
#69521=ORIENTED_EDGE ( 'NONE', *, *, #39321, .F. ) ;
#69524=DIRECTION ( 'NONE',  ( -1.000000000000000000, -2.756263715554006823E-15, 0.000000000000000000 ) ) ;
#69526=ORIENTED_EDGE ( 'NONE', *, *, #54718, .F. ) ;
#69527=CIRCLE ( 'NONE', #86899, 3.000000000000002665 ) ;
#69528=DIRECTION ( 'NONE',  ( 0.9834602067019598826, 0.1811243270069988198, 0.000000000000000000 ) ) ;
#69529=DIRECTION ( 'NONE',  ( 0.000000000000000000, 0.000000000000000000, -1.000000000000000000 ) ) ;
#69530=CARTESIAN_POINT ( 'NONE',  ( 97.81168921572486852, -40.51740600946125426, 16.63579259794490284 ) ) ;
#69531=PLANE ( 'NONE',  #86934 ) ;
#69532=DIRECTION ( 'NONE',  ( 1.000000000000000000, 4.299999999999999979E-14, -1.230419385187874527E-43 ) ) ;
#69533=CARTESIAN_POINT ( 'NONE',  ( 105.0150133346707406, -46.21955246553896757, 181.8295626852199689 ) ) ;
#69534=CARTESIAN_POINT ( 'NONE',  ( 103.5840655562901134, -46.60261447156455716, 57.30705384733997221 ) ) ;
#69535=VERTEX_POINT ( 'NONE', #79331 ) ;
#69537=ORIENTED_EDGE ( 'NONE', *, *, #68364, .T. ) ;
#69538=VECTOR ( 'NONE', #69165, 1000.000000000000000 ) ;
#69540=ORIENTED_EDGE ( 'NONE', *, *, #32541, .F. ) ;
#69544=AXIS2_PLACEMENT_3D ( 'NONE', #40604, #5197, #54203 ) ;
#69545=DIRECTION ( 'NONE',  ( -0.7071067811865434649, -0.7071067811865516806, -7.071067811865441807E-16 ) ) ;
#69547=CARTESIAN_POINT ( 'NONE',  ( 107.0664832912739968, -18.82844715994099971, 168.9256252759119832 ) ) ;
#69548=ORIENTED_EDGE ( 'NONE', *, *, #52668, .T. ) ;
#69549=CARTESIAN_POINT ( 'NONE',  ( 111.9392231810069944, -27.48808525092397304, 59.68991099019693536 ) ) ;
#69555=FACE_OUTER_BOUND ( 'NONE', #1658, .T. ) ;
#69557=AXIS2_PLACEMENT_3D ( 'NONE', #9880, #23527, #16695 ) ;
#69560=CYLINDRICAL_SURFACE ( 'NONE', #17971, 4.875000000000017764 ) ;
#69562=CARTESIAN_POINT ( 'NONE',  ( 104.1016336957795261, -46.74677842777965253, 103.3470538473389411 ) ) ;
#69563=CARTESIAN_POINT ( 'NONE',  ( 194.5664832912739826, -18.82844715994099971, 342.9256252759119548 ) ) ;
#69564=FACE_OUTER_BOUND ( 'NONE', #20708, .T. ) ;
#69565=CARTESIAN_POINT ( 'NONE',  ( 116.3197976069899795, -32.94561274469138112, 134.1356252759109680 ) ) ;
#69566=VECTOR ( 'NONE', #51469, 1000.000000000000000 ) ;
#69567=EDGE_CURVE ( 'NONE', #83239, #71292, #37973, .T. ) ;
#69569=CARTESIAN_POINT ( 'NONE',  ( 108.2018929880948548, -26.98138995270375062, 125.9841967044819597 ) ) ;
#69573=CARTESIAN_POINT ( 'NONE',  ( 117.4688788178165737, -35.86077403649778716, 249.8927681330537780 ) ) ;
#69574=CARTESIAN_POINT ( 'NONE',  ( 172.5664832912729878, -27.82844715994070484, 258.9256252759120116 ) ) ;
#69575=LINE ( 'NONE', #83660, #25772 ) ;
#69576=CARTESIAN_POINT ( 'NONE',  ( 51.27381068362099370, -23.19206098993950604, -5.074374724088000832 ) ) ;
#69578=EDGE_CURVE ( 'NONE', #27916, #89573, #79671, .T. ) ;
#69580=EDGE_CURVE ( 'NONE', #67349, #20321, #51586, .T. ) ;
#69583=CARTESIAN_POINT ( 'NONE',  ( 97.67678136301120162, -41.13084272647608941, 211.6632443235309893 ) ) ;
#69584=ORIENTED_EDGE ( 'NONE', *, *, #48277, .T. ) ;
#69585=EDGE_LOOP ( 'NONE', ( #48460, #57258 ) ) ;
#69586=AXIS2_PLACEMENT_3D ( 'NONE', #63269, #15126, #21958 ) ;
#69587=CARTESIAN_POINT ( 'NONE',  ( 99.36575536895223593, -31.34657530650553880, 157.2606309249449623 ) ) ;
#69588=VECTOR ( 'NONE', #80127, 1000.000000000000000 ) ;
#69589=DIRECTION ( 'NONE',  ( 0.000000000000000000, 0.000000000000000000, -1.000000000000000000 ) ) ;
#69590=CARTESIAN_POINT ( 'NONE',  ( 114.6135591410776016, -41.37377328621888495, 14.81872616303997425 ) ) ;
#69592=ADVANCED_FACE ( 'NONE', ( #17967 ), #10705, .F. ) ;
#69594=VECTOR ( 'NONE', #39661, 1000.000000000000000 ) ;
#69596=CYLINDRICAL_SURFACE ( 'NONE', #55061, 0.5000000000000007772 ) ;
#69597=LINE ( 'NONE', #47784, #77838 ) ;
#69599=CARTESIAN_POINT ( 'NONE',  ( 116.8642987764957297, -41.79567201640977459, 243.4346728949589647 ) ) ;
#69600=DIRECTION ( 'NONE',  ( 1.000000000000000000, 0.000000000000000000, 0.000000000000000000 ) ) ;
#69601=ORIENTED_EDGE ( 'NONE', *, *, #5898, .T. ) ;
#69604=FACE_OUTER_BOUND ( 'NONE', #61555, .T. ) ;
#69605=CARTESIAN_POINT ( 'NONE',  ( 82.80376800125165460, -19.00431460297814468, 6.768845952122303444 ) ) ;
#69606=VECTOR ( 'NONE', #82933, 1000.000000000000000 ) ;
#69607=CARTESIAN_POINT ( 'NONE',  ( 97.92310196018878798, -40.78040932546785768, 122.6578565618004006 ) ) ;
#69611=CARTESIAN_POINT ( 'NONE',  ( 116.1963150171851851, -43.04653558477239272, 9.356577656862985037 ) ) ;
#69612=CARTESIAN_POINT ( 'NONE',  ( 96.80868943730629894, -40.84730494075294871, 251.6422919425777138 ) ) ;
#69613=VERTEX_POINT ( 'NONE', #51147 ) ;
#69616=CARTESIAN_POINT ( 'NONE',  ( 77.65458752640685702, -38.05177997653564859, 7.178113714831590997 ) ) ;
#69618=CARTESIAN_POINT ( 'NONE',  ( 111.2674639284623908, -45.80588075472486764, 167.9214246773950947 ) ) ;
#69620=CARTESIAN_POINT ( 'NONE',  ( 109.6406350139562136, -27.81487066565610888, 62.67094751244894724 ) ) ;
#69621=CARTESIAN_POINT ( 'NONE',  ( 108.3688181871424945, -47.72895317076035582, 158.6822919425779617 ) ) ;
#69626=ORIENTED_EDGE ( 'NONE', *, *, #21957, .F. ) ;
#69627=ORIENTED_EDGE ( 'NONE', *, *, #74187, .F. ) ;
#69629=ORIENTED_EDGE ( 'NONE', *, *, #83520, .F. ) ;
#69630=EDGE_LOOP ( 'NONE', ( #41801, #10420 ) ) ;
#69632=CARTESIAN_POINT ( 'NONE',  ( 115.2923595980251434, -39.02968425817515197, 98.03241982807698207 ) ) ;
#69633=CARTESIAN_POINT ( 'NONE',  ( 111.6181759772156994, -46.13308781976898842, 247.9356252759109509 ) ) ;
#69634=AXIS2_PLACEMENT_3D ( 'NONE', #22238, #30824, #71722 ) ;
#69635=CARTESIAN_POINT ( 'NONE',  ( 110.1310368924891350, -26.13358316477604504, 214.8403871806729342 ) ) ;
#69636=CARTESIAN_POINT ( 'NONE',  ( 96.97787942770426639, -32.27031107066119375, 51.98324432352996638 ) ) ;
#69637=CARTESIAN_POINT ( 'NONE',  ( 82.81648329127399677, -18.72944715994105636, -5.074374724089055100 ) ) ;
#69639=VECTOR ( 'NONE', #88340, 1000.000000000000000 ) ;
#69644=VECTOR ( 'NONE', #31193, 1000.000000000000000 ) ;
#69645=CARTESIAN_POINT ( 'NONE',  ( 107.9743429475490615, -26.39917242597363867, 109.9946728949599759 ) ) ;
#69646=CARTESIAN_POINT ( 'NONE',  ( 117.3100546213214699, -38.89183298362549834, 63.66133956162494911 ) ) ;
#69647=CARTESIAN_POINT ( 'NONE',  ( 110.7486471836621860, -26.25784018214204707, 254.8194347997204545 ) ) ;
#69648=EDGE_LOOP ( 'NONE', ( #38124, #60805, #29215, #61766 ) ) ;
#69649=CARTESIAN_POINT ( 'NONE',  ( 98.89873792621239090, -29.28182854020744230, 230.7261014663869503 ) ) ;
#69650=FACE_BOUND ( 'NONE', #31527, .T. ) ;
#69653=CARTESIAN_POINT ( 'NONE',  ( 116.3185177584062444, -32.94221225046054968, 100.1356252759109680 ) ) ;
#69657=CARTESIAN_POINT ( 'NONE',  ( 31.71315051185499811, -33.70561438052090608, -5.074374724088000832 ) ) ;
#69658=VECTOR ( 'NONE', #85953, 1000.000000000000000 ) ;
#69660=CYLINDRICAL_SURFACE ( 'NONE', #74969, 3.250000000000002665 ) ;
#69661=DIRECTION ( 'NONE',  ( 0.000000000000000000, 0.000000000000000000, 1.000000000000000000 ) ) ;
#69662=DIRECTION ( 'NONE',  ( 1.000000000000000078E-15, 0.000000000000000000, -1.000000000000000000 ) ) ;
#69663=ORIENTED_EDGE ( 'NONE', *, *, #79452, .T. ) ;
#69665=CARTESIAN_POINT ( 'NONE',  ( 115.3410742220599872, -45.24796585940374882, 268.1899109901965517 ) ) ;
#69666=CARTESIAN_POINT ( 'NONE',  ( 118.9175753851156401, -36.92810247848812821, 149.8127681330539644 ) ) ;
#69667=CARTESIAN_POINT ( 'NONE',  ( 97.77292256144662019, -40.53329279276322694, 7.635625275910939536 ) ) ;
#69668=AXIS2_PLACEMENT_3D ( 'NONE', #70179, #27059, #20248 ) ;
#69669=FACE_BOUND ( 'NONE', #47088, .T. ) ;
#69670=LINE ( 'NONE', #21072, #56601 ) ;
#69671=DIRECTION ( 'NONE',  ( -0.7071067811865197061, -0.7071067811865753283, -7.071067811865190357E-16 ) ) ;
#69675=ORIENTED_EDGE ( 'NONE', *, *, #65216, .T. ) ;
#69676=EDGE_CURVE ( 'NONE', #37713, #86716, #37372, .T. ) ;
#69677=DIRECTION ( 'NONE',  ( 0.000000000000000000, 1.000000000000000000, 0.000000000000000000 ) ) ;
#69679=AXIS2_PLACEMENT_3D ( 'NONE', #82928, #55165, #20687 ) ;
#69680=CARTESIAN_POINT ( 'NONE',  ( 102.8925193805077498, -44.76628084087394654, 166.6057531614099503 ) ) ;
#69681=ADVANCED_FACE ( 'NONE', ( #87030 ), #24795, .T. ) ;
#69683=ORIENTED_EDGE ( 'NONE', *, *, #39987, .F. ) ;
#69685=CARTESIAN_POINT ( 'NONE',  ( 105.7232414704440941, -24.98023492732646744, 156.1670538473399574 ) ) ;
#69686=CARTESIAN_POINT ( 'NONE',  ( 117.0724543456819902, -35.46712184163512660, 149.9277079111001854 ) ) ;
#69688=CARTESIAN_POINT ( 'NONE',  ( 97.33920838924730390, -34.06551626165290969, 87.11420987653328041 ) ) ;
#69689=EDGE_CURVE ( 'NONE', #77142, #46008, #47533, .T. ) ;
#69691=CARTESIAN_POINT ( 'NONE',  ( 86.06670390244796920, -58.72944715994112386, 198.9178068554149945 ) ) ;
#69692=LINE ( 'NONE', #20205, #19307 ) ;
#69693=CARTESIAN_POINT ( 'NONE',  ( 114.7602587138392920, -43.68247563549513046, 83.25372051400698581 ) ) ;
#69694=EDGE_LOOP ( 'NONE', ( #57546, #77543, #51332, #39756 ) ) ;
#69695=AXIS2_PLACEMENT_3D ( 'NONE', #21579, #69268, #35633 ) ;
#69697=VERTEX_POINT ( 'NONE', #7038 ) ;
#69698=ADVANCED_FACE ( 'NONE', ( #81573 ), #27246, .F. ) ;
#69699=CARTESIAN_POINT ( 'NONE',  ( 109.9481718979998277, -45.67217584368548700, 54.26824997256396443 ) ) ;
#69701=CARTESIAN_POINT ( 'NONE',  ( 98.80555182512732415, -41.96590078842027793, 182.7756252759109543 ) ) ;
#69703=CARTESIAN_POINT ( 'NONE',  ( 97.06103120714826105, -37.99613185989743869, 56.42650901886334935 ) ) ;
#69706=CYLINDRICAL_SURFACE ( 'NONE', #19945, 9.999999999999998224 ) ;
#69707=AXIS2_PLACEMENT_3D ( 'NONE', #84256, #35628, #22030 ) ;
#69709=DIRECTION ( 'NONE',  ( -1.665334536937733296E-13, -1.000000000000000000, 0.000000000000000000 ) ) ;
#69710=CARTESIAN_POINT ( 'NONE',  ( 113.9025887763448566, -28.07314977735658701, 124.5565776568629559 ) ) ;
#69711=ORIENTED_EDGE ( 'NONE', *, *, #82900, .F. ) ;
#69712=VERTEX_POINT ( 'NONE', #13408 ) ;
#69713=ADVANCED_FACE ( 'NONE', ( #88823 ), #19771, .F. ) ;
#69714=ORIENTED_EDGE ( 'NONE', *, *, #24481, .T. ) ;
#69715=VECTOR ( 'NONE', #66866, 1000.000000000000000 ) ;
#69718=CARTESIAN_POINT ( 'NONE',  ( 107.0664832912739399, -36.72944715994095333, 312.1356252759112522 ) ) ;
#69719=CARTESIAN_POINT ( 'NONE',  ( 100.1721853667017825, -41.09961673838238028, 184.5938046553059735 ) ) ;
#69722=CARTESIAN_POINT ( 'NONE',  ( 193.0374249753374443, -23.42844715993432558, 300.4678068554149490 ) ) ;
#69727=DIRECTION ( 'NONE',  ( 4.299999999999999979E-14, -1.000000000000000000, 4.400000000000000367E-29 ) ) ;
#69729=ORIENTED_EDGE ( 'NONE', *, *, #72456, .F. ) ;
#69730=CARTESIAN_POINT ( 'NONE',  ( 78.11989406983862239, -20.67261125154402990, 7.590611884336022186 ) ) ;
#69732=CARTESIAN_POINT ( 'NONE',  ( 98.31652346514815122, -35.14820314722400241, 237.6158690201829415 ) ) ;
#69734=ORIENTED_EDGE ( 'NONE', *, *, #42745, .F. ) ;
#69736=CARTESIAN_POINT ( 'NONE',  ( 172.5667039024480687, -42.82844715993500273, 300.4678068554149490 ) ) ;
#69740=FACE_OUTER_BOUND ( 'NONE', #17186, .T. ) ;
#69741=ORIENTED_EDGE ( 'NONE', *, *, #14214, .F. ) ;
#69742=VERTEX_POINT ( 'NONE', #1575 ) ;
#69744=CARTESIAN_POINT ( 'NONE',  ( 105.3241794147103008, -28.72650611001668608, 258.0652332267344491 ) ) ;
#69745=CARTESIAN_POINT ( 'NONE',  ( 103.1663722902654001, -27.03741444506403724, 130.3813395616259925 ) ) ;
#69746=CARTESIAN_POINT ( 'NONE',  ( 117.8338636819851644, -39.12263375953642708, 103.6403871806729455 ) ) ;
#69747=DIRECTION ( 'NONE',  ( 1.000000000000000000, 4.163336342344333240E-14, 0.000000000000000000 ) ) ;
#69748=DIRECTION ( 'NONE',  ( -1.000000000000000078E-15, 1.000000000000000083E-30, 1.000000000000000000 ) ) ;
#69749=CARTESIAN_POINT ( 'NONE',  ( 114.6054725695487946, -29.52902160936550047, 230.4327681330539690 ) ) ;
#69750=DIRECTION ( 'NONE',  ( 1.000000000000000000, 4.163336342344333240E-14, 0.000000000000000000 ) ) ;
#69751=DIRECTION ( 'NONE',  ( 1.000000000000000078E-15, -1.000000000000000083E-30, -1.000000000000000000 ) ) ;
#69755=ORIENTED_EDGE ( 'NONE', *, *, #23161, .T. ) ;
#69756=DIRECTION ( 'NONE',  ( -0.9254794337955620787, -0.3787978585227822492, 0.000000000000000000 ) ) ;
#69757=CONICAL_SURFACE ( 'NONE', #55263, 1.624999999999987566, 1.029744258676650093 ) ;
#69758=CARTESIAN_POINT ( 'NONE',  ( 103.2779695159621696, -27.47487189271723196, 136.3856721692480107 ) ) ;
#69760=EDGE_LOOP ( 'NONE', ( #23206, #83083, #49612, #87298, #25162, #37006, #60352, #56659 ) ) ;
#69761=CARTESIAN_POINT ( 'NONE',  ( 108.2767148518004490, -26.33900702273897565, 129.9841967044819739 ) ) ;
#69762=CARTESIAN_POINT ( 'NONE',  ( 98.35067341706619004, -31.65512452754220263, 255.9063942260654869 ) ) ;
#69765=CARTESIAN_POINT ( 'NONE',  ( 182.2420472961719895, -31.76306994223730840, -5.074374724088000832 ) ) ;
#69766=CARTESIAN_POINT ( 'NONE',  ( 98.12663683250418956, -41.21668256917149620, 56.69630050190792758 ) ) ;
#69767=CARTESIAN_POINT ( 'NONE',  ( 115.0380569359701326, -30.04493676975927485, 265.3813395616251682 ) ) ;
#69769=DIRECTION ( 'NONE',  ( 0.000000000000000000, 0.000000000000000000, -1.000000000000000000 ) ) ;
#69771=CARTESIAN_POINT ( 'NONE',  ( 134.0664832912740110, -41.22944715994101017, 4.925625275910997303 ) ) ;
#69772=CARTESIAN_POINT ( 'NONE',  ( 163.0667039024470171, -32.29483332968611364, -5.074374724088000832 ) ) ;
#69774=CYLINDRICAL_SURFACE ( 'NONE', #26032, 0.2500000000000002220 ) ;
#69776=CARTESIAN_POINT ( 'NONE',  ( 99.99420790045508056, -28.96206233275049158, 285.6641967044822650 ) ) ;
#69779=CARTESIAN_POINT ( 'NONE',  ( 102.9045757522767843, -27.10877478265368623, 155.4013395616249795 ) ) ;
#69780=CARTESIAN_POINT ( 'NONE',  ( 104.4907123320104461, -46.86782655419724364, 43.37848241876896083 ) ) ;
#69781=CARTESIAN_POINT ( 'NONE',  ( 96.69998679698829847, -35.27043030541812385, 177.2156252759109805 ) ) ;
#69782=CARTESIAN_POINT ( 'NONE',  ( 100.9546726858703920, -28.70702582103217182, 31.59395862158653046 ) ) ;
#69783=CARTESIAN_POINT ( 'NONE',  ( 113.2453581294647478, -28.75857153267794075, 100.5523746408958061 ) ) ;
#69785=CYLINDRICAL_SURFACE ( 'NONE', #32625, 0.4999999999999933387 ) ;
#69786=CYLINDRICAL_SURFACE ( 'NONE', #36554, 10.00000000000000888 ) ;
#69787=CARTESIAN_POINT ( 'NONE',  ( 41.56648329127399677, -9.303447159940999356, 261.0426252759119734 ) ) ;
#69788=ORIENTED_EDGE ( 'NONE', *, *, #66951, .T. ) ;
#69789=VECTOR ( 'NONE', #22195, 1000.000000000000000 ) ;
#69790=CARTESIAN_POINT ( 'NONE',  ( 172.5664832912740110, -27.82844715994070484, 263.6756252759120116 ) ) ;
#69792=ORIENTED_EDGE ( 'NONE', *, *, #53755, .T. ) ;
#69793=EDGE_CURVE ( 'NONE', #53364, #55247, #83884, .T. ) ;
#69798=CARTESIAN_POINT ( 'NONE',  ( 117.9791962420229794, -38.33460093242096178, 69.72229194257801055 ) ) ;
#69799=CARTESIAN_POINT ( 'NONE',  ( 41.56648329127399677, -9.303447159940999356, 196.8086252759119645 ) ) ;
#69800=AXIS2_PLACEMENT_3D ( 'NONE', #49962, #37252, #41019 ) ;
#69803=CARTESIAN_POINT ( 'NONE',  ( 96.60651355459405920, -37.15606806638657389, 157.3584824187679487 ) ) ;
#69804=CARTESIAN_POINT ( 'NONE',  ( 117.8597870418416562, -34.07357964055000821, 14.01848241876896317 ) ) ;
#69805=EDGE_LOOP ( 'NONE', ( #66792, #55775, #30936, #48344, #23193, #55510, #83183, #59543, #4162, #48472, #71267, #59933, #24076, #27029 ) ) ;
#69806=ORIENTED_EDGE ( 'NONE', *, *, #22224, .T. ) ;
#69807=VERTEX_POINT ( 'NONE', #78338 ) ;
#69810=CARTESIAN_POINT ( 'NONE',  ( 71.24162159452610865, 0.6420441417434794573, 540.9756252759101471 ) ) ;
#69811=LINE ( 'NONE', #7584, #88402 ) ;
#69813=CARTESIAN_POINT ( 'NONE',  ( 80.06648329127398256, -9.029447159941060619, 8.225625275910942946 ) ) ;
#69817=DIRECTION ( 'NONE',  ( -0.7071067811865197061, -0.7071067811865753283, -7.071067811865190357E-16 ) ) ;
#69818=AXIS2_PLACEMENT_3D ( 'NONE', #70015, #15052, #55454 ) ;
#69820=CARTESIAN_POINT ( 'NONE',  ( 112.0124476237221103, -28.73397683645135814, 289.6356252759109680 ) ) ;
#69821=PLANE ( 'NONE',  #87885 ) ;
#69823=ORIENTED_EDGE ( 'NONE', *, *, #4248, .F. ) ;
#69826=CARTESIAN_POINT ( 'NONE',  ( 113.4089301560035068, -41.86784124614906233, 86.10237608387694763 ) ) ;
#69827=VECTOR ( 'NONE', #57549, 1000.000000000000000 ) ;
#69829=DIRECTION ( 'NONE',  ( -0.7071067811865279218, 0.7071067811865670016, -2.899137802865041747E-29 ) ) ;
#69830=ORIENTED_EDGE ( 'NONE', *, *, #73179, .T. ) ;
#69831=ORIENTED_EDGE ( 'NONE', *, *, #61982, .T. ) ;
#69832=CARTESIAN_POINT ( 'NONE',  ( 79.05226586200586780, -34.17316201338598347, 8.065992442480940383 ) ) ;
#69833=ORIENTED_EDGE ( 'NONE', *, *, #67788, .F. ) ;
#69836=CARTESIAN_POINT ( 'NONE',  ( 105.7154773740255251, -46.72385839776377026, 68.46895861271767103 ) ) ;
#69837=CARTESIAN_POINT ( 'NONE',  ( 103.2835872187480533, -45.32980894545860906, 128.6663452106589887 ) ) ;
#69838=CARTESIAN_POINT ( 'NONE',  ( 99.65722331657703137, -39.76205027262535907, 10.08425333485812025 ) ) ;
#69840=CARTESIAN_POINT ( 'NONE',  ( 113.4285887376619968, -27.66253919562607422, 80.57753003781597556 ) ) ;
#69842=CARTESIAN_POINT ( 'NONE',  ( 112.0659116089343996, -45.48839626851365381, 83.98979194134383874 ) ) ;
#69845=VERTEX_POINT ( 'NONE', #56962 ) ;
#69847=CIRCLE ( 'NONE', #77114, 5.035202529042049235 ) ;
#69850=CARTESIAN_POINT ( 'NONE',  ( 116.7892270726677140, -35.66563809581925426, 278.9127681330543851 ) ) ;
#69851=CARTESIAN_POINT ( 'NONE',  ( 96.03095270115332482, -35.77956804193283347, 182.2461014663869889 ) ) ;
#69854=CARTESIAN_POINT ( 'NONE',  ( 117.6790090996954632, -39.81947568642139856, 134.5889586092439743 ) ) ;
#69856=LINE ( 'NONE', #8528, #11750 ) ;
#69859=ADVANCED_FACE ( 'NONE', ( #27918 ), #63342, .T. ) ;
#69865=CARTESIAN_POINT ( 'NONE',  ( 100.5506404981706510, -27.80068015945615656, 30.56610146638794134 ) ) ;
#69869=CARTESIAN_POINT ( 'NONE',  ( 101.2965385564679792, -30.39239502954603367, 285.0867055423626084 ) ) ;
#69871=CARTESIAN_POINT ( 'NONE',  ( 109.0680860650138300, -47.57644715601873742, 123.7337205140059666 ) ) ;
#69872=DIRECTION ( 'NONE',  ( 3.999999999999999995E-14, -1.000000000000000000, 4.100000000000000342E-29 ) ) ;
#69873=DIRECTION ( 'NONE',  ( -1.000000000000000000, 0.000000000000000000, 0.000000000000000000 ) ) ;
#69874=EDGE_LOOP ( 'NONE', ( #46541, #1316, #68555, #75277, #48798, #65504 ) ) ;
#69878=CARTESIAN_POINT ( 'NONE',  ( 136.6003823147690355, -35.66080131299383993, 2.811527311783425187 ) ) ;
#69881=CARTESIAN_POINT ( 'NONE',  ( 98.05257159168807846, -42.12399974224388188, 161.7556252759109725 ) ) ;
#69882=ORIENTED_EDGE ( 'NONE', *, *, #12979, .T. ) ;
#69883=FACE_OUTER_BOUND ( 'NONE', #44694, .T. ) ;
#69884=CARTESIAN_POINT ( 'NONE',  ( 118.0739042565516712, -35.49579832924209910, 229.9032443235299468 ) ) ;
#69885=CARTESIAN_POINT ( 'NONE',  ( 97.73362116697985869, -31.98701483920769206, 46.95276813305393659 ) ) ;
#69886=DIRECTION ( 'NONE',  ( -0.7071067811868642083, -0.7071067811862309371, -7.071067811868635707E-16 ) ) ;
#69887=VECTOR ( 'NONE', #46280, 1000.000000000000000 ) ;
#69888=CARTESIAN_POINT ( 'NONE',  ( 97.81461822720238786, -40.51595288653417981, 132.6359866545674890 ) ) ;
#69890=ORIENTED_EDGE ( 'NONE', *, *, #46666, .T. ) ;
#69891=AXIS2_PLACEMENT_3D ( 'NONE', #10636, #71987, #17461 ) ;
#69893=EDGE_CURVE ( 'NONE', #82764, #17557, #51587, .T. ) ;
#69894=VERTEX_POINT ( 'NONE', #57863 ) ;
#69895=EDGE_CURVE ( 'NONE', #67030, #74870, #52786, .T. ) ;
#69896=ORIENTED_EDGE ( 'NONE', *, *, #20194, .F. ) ;
#69897=EDGE_CURVE ( 'NONE', #18950, #8582, #53349, .T. ) ;
#69898=ORIENTED_EDGE ( 'NONE', *, *, #24256, .T. ) ;
#69899=DIRECTION ( 'NONE',  ( 0.000000000000000000, 1.000000000000000000, 0.000000000000000000 ) ) ;
#69900=CARTESIAN_POINT ( 'NONE',  ( 117.3348620442827865, -34.92864588493001321, 239.9641967044819637 ) ) ;
#69902=CARTESIAN_POINT ( 'NONE',  ( 136.8164482479830895, -18.55833207211816926, 3.101428811466735880 ) ) ;
#69904=EDGE_CURVE ( 'NONE', #1995, #45788, #65127, .T. ) ;
#69906=DIRECTION ( 'NONE',  ( 0.000000000000000000, 0.000000000000000000, -1.000000000000000000 ) ) ;
#69907=CARTESIAN_POINT ( 'NONE',  ( 142.0664832912739826, -8.729447159940995959, 14.92562527591100618 ) ) ;
#69908=CARTESIAN_POINT ( 'NONE',  ( 117.4065409050533617, -38.22262247076111663, 28.71276813305395592 ) ) ;
#69909=EDGE_LOOP ( 'NONE', ( #27095, #75334, #80675, #74221 ) ) ;
#69912=EDGE_CURVE ( 'NONE', #47987, #39785, #73309, .T. ) ;
#69913=VECTOR ( 'NONE', #80962, 1000.000000000000000 ) ;
#69916=CARTESIAN_POINT ( 'NONE',  ( 99.40370404213548738, -29.74227323812501211, 226.7261014663869503 ) ) ;
#69917=ADVANCED_FACE ( 'NONE', ( #75525 ), #82354, .F. ) ;
#69920=CARTESIAN_POINT ( 'NONE',  ( 114.1038288540492687, -43.56973530630599356, 94.21276813305296116 ) ) ;
#69921=CARTESIAN_POINT ( 'NONE',  ( 98.30749153155636577, -41.72877165996427351, 31.74000518241274804 ) ) ;
#69922=CARTESIAN_POINT ( 'NONE',  ( 103.2818408434572177, -27.47328781080362248, 21.38533937723293477 ) ) ;
#69923=ORIENTED_EDGE ( 'NONE', *, *, #33251, .F. ) ;
#69924=DIRECTION ( 'NONE',  ( 0.000000000000000000, 0.000000000000000000, 1.000000000000000000 ) ) ;
#69929=CARTESIAN_POINT ( 'NONE',  ( 110.2543409660563043, -27.89122963701645830, 246.2206309249449703 ) ) ;
#69930=CARTESIAN_POINT ( 'NONE',  ( 99.04406178633300328, -42.84125754617969051, 191.8439585998989685 ) ) ;
#69933=DIRECTION ( 'NONE',  ( 1.000000000000000000, 0.000000000000000000, 0.000000000000000000 ) ) ;
#69937=ORIENTED_EDGE ( 'NONE', *, *, #6692, .F. ) ;
#69938=CARTESIAN_POINT ( 'NONE',  ( 104.4906584979394211, -46.86803844812923359, 47.37848241876796607 ) ) ;
#69939=EDGE_LOOP ( 'NONE', ( #37655, #68951, #73870, #32556 ) ) ;
#69940=CARTESIAN_POINT ( 'NONE',  ( 112.8202834993214481, -29.45004372636961065, 272.3623760838771091 ) ) ;
#69942=CARTESIAN_POINT ( 'NONE',  ( 109.4488926988246646, -27.20905326525207357, 199.8813395616259925 ) ) ;
#69943=DIRECTION ( 'NONE',  ( 1.000000000000000000, 0.000000000000000000, 0.000000000000000000 ) ) ;
#69944=CARTESIAN_POINT ( 'NONE',  ( 95.05156358570199870, -41.69348830286664764, 289.6356252759107406 ) ) ;
#69945=DIRECTION ( 'NONE',  ( 1.110223024625155531E-13, -1.000000000000000000, 0.000000000000000000 ) ) ;
#69948=CARTESIAN_POINT ( 'NONE',  ( 61.56670390244639890, -23.42844715994043270, 129.9678068554150911 ) ) ;
#69949=CARTESIAN_POINT ( 'NONE',  ( 115.9437545354735306, -30.06674848629992880, 260.3508633711495008 ) ) ;
#69953=DIRECTION ( 'NONE',  ( 0.000000000000000000, 0.000000000000000000, 1.000000000000000000 ) ) ;
#69954=ORIENTED_EDGE ( 'NONE', *, *, #79427, .F. ) ;
#69955=CARTESIAN_POINT ( 'NONE',  ( 111.0993040117788979, -25.53357873718133320, 95.80133956162495679 ) ) ;
#69960=ORIENTED_EDGE ( 'NONE', *, *, #47730, .T. ) ;
#69961=CYLINDRICAL_SURFACE ( 'NONE', #44949, 10.00000000000000888 ) ;
#69962=CARTESIAN_POINT ( 'NONE',  ( 184.5667039024480118, -48.82844715994099971, 310.9178068554150514 ) ) ;
#69964=CARTESIAN_POINT ( 'NONE',  ( 63.06670390244794078, -40.32844715994017548, 300.4678068554150627 ) ) ;
#69965=LINE ( 'NONE', #54502, #22901 ) ;
#69966=CARTESIAN_POINT ( 'NONE',  ( 116.5562423158612972, -42.44168660689859962, 274.3832443235299365 ) ) ;
#69967=VECTOR ( 'NONE', #81232, 1000.000000000000000 ) ;
#69968=LINE ( 'NONE', #471, #55157 ) ;
#69969=ORIENTED_EDGE ( 'NONE', *, *, #86116, .T. ) ;
#69971=CARTESIAN_POINT ( 'NONE',  ( 80.48314995794039817, 12.92155284005802685, 349.2756252759109543 ) ) ;
#69972=VERTEX_POINT ( 'NONE', #53697 ) ;
#69973=EDGE_LOOP ( 'NONE', ( #15730, #69675 ) ) ;
#69974=VECTOR ( 'NONE', #10307, 1000.000000000000000 ) ;
#69975=EDGE_CURVE ( 'NONE', #76954, #67284, #4692, .T. ) ;
#69976=CARTESIAN_POINT ( 'NONE',  ( 81.55985452235577782, -21.04079274305108527, 1.981704437698954768 ) ) ;
#69978=CARTESIAN_POINT ( 'NONE',  ( 97.79631277754322127, -40.47965291819907918, 16.63237950705615731 ) ) ;
#69981=CARTESIAN_POINT ( 'NONE',  ( 112.5429177363308924, -43.28420096851815657, 192.5524198280769781 ) ) ;
#69983=CARTESIAN_POINT ( 'NONE',  ( 113.3411949225463502, -28.30449682957925717, 104.5670538473399347 ) ) ;
#69990=CARTESIAN_POINT ( 'NONE',  ( 97.07203916560013113, -35.37876108158648947, 262.2190116196141503 ) ) ;
#69991=ORIENTED_EDGE ( 'NONE', *, *, #87642, .F. ) ;
#69992=CARTESIAN_POINT ( 'NONE',  ( 165.6738106836030227, -28.98061976758901892, -5.074374724088000832 ) ) ;
#69996=ORIENTED_EDGE ( 'NONE', *, *, #36838, .F. ) ;
#69997=CARTESIAN_POINT ( 'NONE',  ( 95.32417067969559810, -34.95402877631575222, 71.20705384733993526 ) ) ;
#69999=FACE_OUTER_BOUND ( 'NONE', #89866, .T. ) ;
#70001=DIRECTION ( 'NONE',  ( 1.000000000000000000, 0.000000000000000000, 0.000000000000000000 ) ) ;
#70002=CARTESIAN_POINT ( 'NONE',  ( 132.8230071953907725, -16.27587548316543931, 1.868342134761751483 ) ) ;
#70003=ORIENTED_EDGE ( 'NONE', *, *, #72993, .T. ) ;
#70006=EDGE_CURVE ( 'NONE', #40462, #26689, #19214, .T. ) ;
#70007=CARTESIAN_POINT ( 'NONE',  ( 110.7480548206264785, -27.39964114457682598, 120.7761619811009126 ) ) ;
#70009=EDGE_CURVE ( 'NONE', #53062, #59219, #84119, .T. ) ;
#70011=CARTESIAN_POINT ( 'NONE',  ( 96.62018903270816850, -36.61901565639288236, 107.3184824187679567 ) ) ;
#70014=CARTESIAN_POINT ( 'NONE',  ( 51.42025729302574888, -31.94127993907664731, 117.4678068554150485 ) ) ;
#70015=CARTESIAN_POINT ( 'NONE',  ( 130.3998166246070127, 12.92155284005802685, 335.5992267699912190 ) ) ;
#70016=AXIS2_PLACEMENT_3D ( 'NONE', #17, #21356, #35412 ) ;
#70017=ORIENTED_EDGE ( 'NONE', *, *, #42607, .F. ) ;
#70019=CARTESIAN_POINT ( 'NONE',  ( 107.6167445103326230, -46.48501816386541208, 148.6213395616249784 ) ) ;
#70021=DIRECTION ( 'NONE',  ( 0.000000000000000000, 0.000000000000000000, -1.000000000000000000 ) ) ;
#70023=CARTESIAN_POINT ( 'NONE',  ( 104.8459308146384785, -26.52976224399709082, 256.2470538473397141 ) ) ;
#70024=CARTESIAN_POINT ( 'NONE',  ( 107.0664832912739399, -36.72944715994095333, 315.1356252759112522 ) ) ;
#70026=EDGE_CURVE ( 'NONE', #48723, #84365, #65901, .T. ) ;
#70027=CARTESIAN_POINT ( 'NONE',  ( 188.5667039024479834, -62.87844715994099687, 132.3428068554150343 ) ) ;
#70032=CARTESIAN_POINT ( 'NONE',  ( 99.06478422775786896, -31.10483629442210329, 205.8384824187689617 ) ) ;
#70033=ORIENTED_EDGE ( 'NONE', *, *, #70814, .T. ) ;
#70034=VERTEX_POINT ( 'NONE', #17763 ) ;
#70035=CARTESIAN_POINT ( 'NONE',  ( 100.2959224756171466, -44.18784923124425035, 153.4215833058969736 ) ) ;
#70037=CARTESIAN_POINT ( 'NONE',  ( 123.6837132603321692, -20.11243780205712639, 249.5838068554165261 ) ) ;
#70038=CARTESIAN_POINT ( 'NONE',  ( 103.4018642804673789, -27.34641595622759169, 16.80444044875395448 ) ) ;
#70039=DIRECTION ( 'NONE',  ( -1.000000000000000000, 1.011922027653136551E-15, 0.000000000000000000 ) ) ;
#70040=VECTOR ( 'NONE', #76017, 1000.000000000000000 ) ;
#70041=FACE_OUTER_BOUND ( 'NONE', #3813, .T. ) ;
#70043=DIRECTION ( 'NONE',  ( 5.512527431108029424E-15, -1.000000000000000000, 0.000000000000000000 ) ) ;
#70044=LINE ( 'NONE', #75962, #28474 ) ;
#70045=CARTESIAN_POINT ( 'NONE',  ( 98.91597900623158068, -29.29754952351876796, 230.7261014663869503 ) ) ;
#70047=VERTEX_POINT ( 'NONE', #38641 ) ;
#70048=ORIENTED_EDGE ( 'NONE', *, *, #86023, .F. ) ;
#70051=CARTESIAN_POINT ( 'NONE',  ( 99.50465472078816731, -43.30570863480165400, 122.8950840663260209 ) ) ;
#70053=EDGE_CURVE ( 'NONE', #41893, #21752, #78681, .T. ) ;
#70055=ORIENTED_EDGE ( 'NONE', *, *, #70728, .F. ) ;
#70056=CARTESIAN_POINT ( 'NONE',  ( 101.5861822943782755, -47.29253114347246623, 13.19562527591094891 ) ) ;
#70057=EDGE_CURVE ( 'NONE', #85412, #18386, #28747, .T. ) ;
#70058=CARTESIAN_POINT ( 'NONE',  ( 106.5673262220758772, -47.17821497701651623, 247.5384824187679556 ) ) ;
#70060=DIRECTION ( 'NONE',  ( -0.9254794337955620787, -0.3787978585227822492, 0.000000000000000000 ) ) ;
#70061=CARTESIAN_POINT ( 'NONE',  ( 90.44969454456439450, -20.11243780205712639, 249.5838068554174924 ) ) ;
#70063=CARTESIAN_POINT ( 'NONE',  ( 114.8864029495430685, -33.02137736771143750, 62.00904275054391945 ) ) ;
#70064=CARTESIAN_POINT ( 'NONE',  ( 108.2803420215754500, -47.73912846947793298, 153.6518157521009584 ) ) ;
#70066=ORIENTED_EDGE ( 'NONE', *, *, #64197, .T. ) ;
#70067=CARTESIAN_POINT ( 'NONE',  ( 182.4202572930269923, -31.94127993907680718, -5.074374724088000832 ) ) ;
#70069=VERTEX_POINT ( 'NONE', #38205 ) ;
#70071=EDGE_CURVE ( 'NONE', #7861, #84435, #40335, .T. ) ;
#70074=ORIENTED_EDGE ( 'NONE', *, *, #23681, .T. ) ;
#70075=DIRECTION ( 'NONE',  ( 1.000000000000000078E-15, -1.000000000000000083E-30, -1.000000000000000000 ) ) ;
#70077=CARTESIAN_POINT ( 'NONE',  ( 109.2815815313881558, -45.51044995646627456, 92.20765792331498290 ) ) ;
#70078=CARTESIAN_POINT ( 'NONE',  ( 105.8910851810002356, -47.14611527663348056, 282.4870538473393253 ) ) ;
#70079=CARTESIAN_POINT ( 'NONE',  ( 101.2129617469312564, -45.32973500739964834, 197.1013395616249966 ) ) ;
#70082=ORIENTED_EDGE ( 'NONE', *, *, #61804, .T. ) ;
#70083=CARTESIAN_POINT ( 'NONE',  ( 97.81169266289590780, -40.51741659614882707, 92.63571255866972365 ) ) ;
#70084=CARTESIAN_POINT ( 'NONE',  ( 93.94797395270801132, -35.60435878782501362, 293.6356252759106837 ) ) ;
#70085=CARTESIAN_POINT ( 'NONE',  ( 134.0664832912739826, -8.729447159941003065, 8.525625275911005829 ) ) ;
#70086=CARTESIAN_POINT ( 'NONE',  ( 114.2526777242401437, -43.36435822665426087, 123.2327681330539519 ) ) ;
#70087=AXIS2_PLACEMENT_3D ( 'NONE', #44836, #52078, #65296 ) ;
#70088=CARTESIAN_POINT ( 'NONE',  ( 96.61245533174189859, -37.29510205964861314, 76.36991099019697060 ) ) ;
#70089=CARTESIAN_POINT ( 'NONE',  ( 99.36439196449877898, -28.73628302914087840, 265.6746728949588032 ) ) ;
#70090=EDGE_LOOP ( 'NONE', ( #61648, #42871, #34953, #51791 ) ) ;
#70091=CARTESIAN_POINT ( 'NONE',  ( 96.12498142956854963, -35.16017202033504674, 226.2251490854349640 ) ) ;
#70092=CARTESIAN_POINT ( 'NONE',  ( 94.06648329127393993, -36.72944715994095333, 293.6356252759106837 ) ) ;
#70096=DIRECTION ( 'NONE',  ( -0.7071067811865259234, 0.7071067811865692221, -2.899137802865049595E-29 ) ) ;
#70097=FACE_OUTER_BOUND ( 'NONE', #75302, .T. ) ;
#70098=CARTESIAN_POINT ( 'NONE',  ( 167.6524903400756159, -49.32844715993520879, 129.9678068554150059 ) ) ;
#70104=CARTESIAN_POINT ( 'NONE',  ( 108.4174892294855681, -26.73503592422339992, 10.96895861100186309 ) ) ;
#70106=CARTESIAN_POINT ( 'NONE',  ( 165.6738106836044722, -28.98061976758450342, 193.9678068554149775 ) ) ;
#70107=DIRECTION ( 'NONE',  ( -0.000000000000000000, -0.000000000000000000, -1.000000000000000000 ) ) ;
#70109=DIRECTION ( 'NONE',  ( 3.999999999999999995E-14, -1.000000000000000000, 4.100000000000000342E-29 ) ) ;
#70110=CARTESIAN_POINT ( 'NONE',  ( 96.74139913992713957, -35.13602278645100796, 266.2041967044820581 ) ) ;
#70111=CARTESIAN_POINT ( 'NONE',  ( 113.3313291481109815, -45.06216520097333955, 139.0899109901969553 ) ) ;
#70112=CARTESIAN_POINT ( 'NONE',  ( 107.1956677504039135, -26.28336798021810239, 31.06705384733893283 ) ) ;
#70113=DIRECTION ( 'NONE',  ( 1.000000000000000000, 0.000000000000000000, 0.000000000000000000 ) ) ;
#70115=CARTESIAN_POINT ( 'NONE',  ( 97.81169607051373305, -40.51742273377266912, 46.63562653399714009 ) ) ;
#70116=CARTESIAN_POINT ( 'NONE',  ( 97.81170238817014706, -40.51743819009087844, 137.6355114220584994 ) ) ;
#70118=B_SPLINE_CURVE_WITH_KNOTS ( 'NONE', 3,
 ( #46453, #39650, #67353, #73277, #32842, #24252, #88282, #37881, #11055, #51922, #52793, #45546, #79679, #80563, #72842, #62680, #35408, #28604, #35864, #76311, #8173, #20904, #7280, #69504, #34966, #14546, #1362, #40098, #42660, #46899, #8631, #63583, #56292, #84500, #67814 ),
 .UNSPECIFIED., .F., .F.,
 ( 4, 2, 2, 1, 1, 2, 2, 2, 2, 2, 2, 1, 1, 2, 2, 2, 1, 1, 1, 2, 4 ),
 ( 0.3333434881890902091, 0.4166701562233744438, 0.4218780729755153280, 0.4270859897276562123, 0.4375018232319381473, 0.4583334902404970213, 0.4999968242576139366, 0.5208284912661723665, 0.5416601582747307964, 0.5624918252832892263, 0.5650957836593583083, 0.5676997420354273904, 0.5729076587875665538, 0.5833234922918473231, 0.6249868263089795040, 0.6275907846850493632, 0.6301947430611192225, 0.6354026598132580528, 0.6458184933175352693, 0.6562343268218123749, 0.6666501603260894804 ),
 .UNSPECIFIED. ) ;
#70119=ORIENTED_EDGE ( 'NONE', *, *, #47966, .F. ) ;
#70121=ORIENTED_EDGE ( 'NONE', *, *, #38614, .F. ) ;
#70122=CARTESIAN_POINT ( 'NONE',  ( 111.7477409549918690, -43.87381266066567775, 177.4609912566479579 ) ) ;
#70124=CYLINDRICAL_SURFACE ( 'NONE', #52894, 2.517500000000005844 ) ;
#70125=ORIENTED_EDGE ( 'NONE', *, *, #19055, .T. ) ;
#70128=CARTESIAN_POINT ( 'NONE',  ( 108.8451227504523189, -46.97957433935474825, 163.7127681330539701 ) ) ;
#70129=CARTESIAN_POINT ( 'NONE',  ( 176.7738106835049052, -48.62134037887551585, 180.4678068554150059 ) ) ;
#70131=CARTESIAN_POINT ( 'NONE',  ( 102.0674588022921228, -27.97026135298835925, 150.4901954177360039 ) ) ;
#70132=CARTESIAN_POINT ( 'NONE',  ( 110.4024638856497518, -27.29981427005776951, 85.80618083057217405 ) ) ;
#70134=DIRECTION ( 'NONE',  ( 0.9834602067019604377, 0.1811243270069963496, 0.000000000000000000 ) ) ;
#70135=CARTESIAN_POINT ( 'NONE',  ( 116.3624975636024317, -33.68846805112525544, 89.07848241876791917 ) ) ;
#70136=VERTEX_POINT ( 'NONE', #23705 ) ;
#70138=VERTEX_POINT ( 'NONE', #16431 ) ;
#70139=VECTOR ( 'NONE', #1024, 1000.000000000000000 ) ;
#70140=CARTESIAN_POINT ( 'NONE',  ( 109.8610415383596148, -27.05157811987473337, 61.28444044875497099 ) ) ;
#70142=CARTESIAN_POINT ( 'NONE',  ( 116.5710038106514759, -34.42130396933982439, 205.0156252759109634 ) ) ;
#70144=FACE_OUTER_BOUND ( 'NONE', #18854, .T. ) ;
#70145=DIRECTION ( 'NONE',  ( 6.524622321627019585E-16, 3.741823817616790462E-31, 1.000000000000000000 ) ) ;
#70146=FACE_OUTER_BOUND ( 'NONE', #84566, .T. ) ;
#70147=CARTESIAN_POINT ( 'NONE',  ( 31.56670390244800828, -33.35206098992711077, -5.074374724088000832 ) ) ;
#70148=DIRECTION ( 'NONE',  ( 0.000000000000000000, 0.000000000000000000, -1.000000000000000000 ) ) ;
#70149=CARTESIAN_POINT ( 'NONE',  ( 97.95167206076190780, -31.64175201202206011, 110.9213395616259703 ) ) ;
#70151=ORIENTED_EDGE ( 'NONE', *, *, #9230, .F. ) ;
#70152=ORIENTED_EDGE ( 'NONE', *, *, #31545, .F. ) ;
#70155=CARTESIAN_POINT ( 'NONE',  ( 97.60799287394519297, -39.98272528114131319, 131.5900899984870875 ) ) ;
#70156=DIRECTION ( 'NONE',  ( 1.000000000000000000, 4.299999999999999979E-14, 1.000000000000000078E-15 ) ) ;
#70157=CARTESIAN_POINT ( 'NONE',  ( 104.5243549119882829, -45.65320838865366682, 215.1738046553059860 ) ) ;
#70158=CIRCLE ( 'NONE', #49789, 9.571100913904368568 ) ;
#70160=AXIS2_PLACEMENT_3D ( 'NONE', #10424, #87619, #38127 ) ;
#70165=VERTEX_POINT ( 'NONE', #50484 ) ;
#70169=CARTESIAN_POINT ( 'NONE',  ( 63.56670390244824631, -47.82844715994016127, 300.4678068554150627 ) ) ;
#70170=CARTESIAN_POINT ( 'NONE',  ( 97.06047953529140671, -37.89159766150721964, 232.8501547344689584 ) ) ;
#70171=CARTESIAN_POINT ( 'NONE',  ( 86.98314995794039817, 12.92155284005802507, 349.2756252759109543 ) ) ;
#70172=EDGE_LOOP ( 'NONE', ( #67063, #56563, #13481, #74989, #57889 ) ) ;
#70173=DIRECTION ( 'NONE',  ( -0.7071067811734105257, 0.7071067811996846197, 0.000000000000000000 ) ) ;
#70175=ORIENTED_EDGE ( 'NONE', *, *, #42187, .T. ) ;
#70176=ORIENTED_EDGE ( 'NONE', *, *, #47418, .F. ) ;
#70177=AXIS2_PLACEMENT_3D ( 'NONE', #61209, #21235, #62108 ) ;
#70179=CARTESIAN_POINT ( 'NONE',  ( 162.7866693523289996, -36.02818131005891189, -5.074374724088000832 ) ) ;
#70180=AXIS2_PLACEMENT_3D ( 'NONE', #5330, #12143, #40730 ) ;
#70182=VERTEX_POINT ( 'NONE', #23273 ) ;
#70183=EDGE_CURVE ( 'NONE', #69535, #72716, #38914, .T. ) ;
#70184=CARTESIAN_POINT ( 'NONE',  ( 115.7079196686036653, -36.25352450022288764, 271.7004713219723726 ) ) ;
#70185=EDGE_CURVE ( 'NONE', #19998, #61434, #43250, .T. ) ;
#70186=AXIS2_PLACEMENT_3D ( 'NONE', #44979, #6240, #24116 ) ;
#70187=CARTESIAN_POINT ( 'NONE',  ( 113.0897370140187235, -28.19324317000061697, 129.5870538473399449 ) ) ;
#70188=CARTESIAN_POINT ( 'NONE',  ( 108.5348814579965904, -26.43029805172848867, 104.9641967044819779 ) ) ;
#70189=CARTESIAN_POINT ( 'NONE',  ( 116.4683302779955767, -39.73499081598242100, 249.5838068554167819 ) ) ;
#70190=PRESENTATION_STYLE_ASSIGNMENT (( #28861 ) ) ;
#70191=CARTESIAN_POINT ( 'NONE',  ( 118.0509465330791983, -35.49837129967784222, 229.9032443235299468 ) ) ;
#70192=FACE_OUTER_BOUND ( 'NONE', #26376, .T. ) ;
#70194=ORIENTED_EDGE ( 'NONE', *, *, #64256, .F. ) ;
#70195=CARTESIAN_POINT ( 'NONE',  ( 188.5667039024479834, -48.82844715994099971, 139.9678068554150059 ) ) ;
#70196=EDGE_CURVE ( 'NONE', #85915, #59995, #24138, .T. ) ;
#70197=VERTEX_POINT ( 'NONE', #50937 ) ;
#70198=ADVANCED_FACE ( 'NONE', ( #15991 ), #43671, .T. ) ;
#70200=CARTESIAN_POINT ( 'NONE',  ( 134.0664832912740110, -46.72944715994100306, 10.72562527591099801 ) ) ;
#70202=EDGE_CURVE ( 'NONE', #18115, #35754, #81027, .T. ) ;
#70203=DIRECTION ( 'NONE',  ( 1.907762142705490052E-15, 7.167082501179359715E-16, -1.000000000000000000 ) ) ;
#70204=ORIENTED_EDGE ( 'NONE', *, *, #73167, .F. ) ;
#70205=CARTESIAN_POINT ( 'NONE',  ( 97.61684652917979577, -30.99503764212949264, 125.8803871806719599 ) ) ;
#70206=CARTESIAN_POINT ( 'NONE',  ( 97.06097939450964418, -37.99593194579918531, 256.4272396045237201 ) ) ;
#70208=CYLINDRICAL_SURFACE ( 'NONE', #11643, 9.999999999999998224 ) ;
#70211=CARTESIAN_POINT ( 'NONE',  ( 107.0624707424859849, -46.75563725778415147, 57.57597174261474748 ) ) ;
#70212=CARTESIAN_POINT ( 'NONE',  ( 116.5858064714420976, -40.92601143571967270, 249.4956252759109532 ) ) ;
#70214=CARTESIAN_POINT ( 'NONE',  ( 97.81169822462854313, -40.51742973538109993, 111.6355314416972391 ) ) ;
#70216=CYLINDRICAL_SURFACE ( 'NONE', #87726, 0.2500000000000002220 ) ;
#70217=CARTESIAN_POINT ( 'NONE',  ( 25.56670390244797275, -48.82844715994099971, 137.2178068554150059 ) ) ;
#70219=CARTESIAN_POINT ( 'NONE',  ( 128.8897065959775432, -58.55267046464430791, -4.824374724089007138 ) ) ;
#70220=CARTESIAN_POINT ( 'NONE',  ( 118.3887371170988132, -33.06383674033636311, 284.0756252759109657 ) ) ;
#70222=CARTESIAN_POINT ( 'NONE',  ( 112.4976487814606685, -26.16836495570049337, 169.6984824187679521 ) ) ;
#70223=CARTESIAN_POINT ( 'NONE',  ( 117.4545169724989648, -37.95830395151629943, 49.73276813305393773 ) ) ;
#70224=CARTESIAN_POINT ( 'NONE',  ( 113.6415746488294047, -45.67179987042115386, 179.0689586092439640 ) ) ;
#70226=DIRECTION ( 'NONE',  ( 1.000000000000000078E-15, -1.000000000000000083E-30, -1.000000000000000000 ) ) ;
#70228=CARTESIAN_POINT ( 'NONE',  ( 172.5664832912729878, -27.57844715994070484, 318.9256252759120116 ) ) ;
#70229=CARTESIAN_POINT ( 'NONE',  ( 71.25416588882602298, -72.55705569728901594, 394.9756252759101471 ) ) ;
#70230=DIRECTION ( 'NONE',  ( 0.000000000000000000, 1.000000000000000000, 0.000000000000000000 ) ) ;
#70231=ORIENTED_EDGE ( 'NONE', *, *, #43628, .F. ) ;
#70232=VECTOR ( 'NONE', #46393, 1000.000000000000000 ) ;
#70234=AXIS2_PLACEMENT_3D ( 'NONE', #45920, #38239, #80943 ) ;
#70238=DIRECTION ( 'NONE',  ( -4.237773401492740281E-14, 1.000000000000000000, 0.000000000000000000 ) ) ;
#70240=CARTESIAN_POINT ( 'NONE',  ( 117.9659426345831719, -38.42225801833666310, 64.69181575210097890 ) ) ;
#70245=CARTESIAN_POINT ( 'NONE',  ( 118.9266961287330560, -37.70231105260669580, 184.7613395616249647 ) ) ;
#70246=EDGE_CURVE ( 'NONE', #24376, #55351, #49008, .T. ) ;
#70247=CARTESIAN_POINT ( 'NONE',  ( 106.1055101188695602, -45.24582830394255240, 281.9095626852197825 ) ) ;
#70248=ORIENTED_EDGE ( 'NONE', *, *, #56157, .T. ) ;
#70249=ORIENTED_EDGE ( 'NONE', *, *, #42568, .T. ) ;
#70251=ORIENTED_EDGE ( 'NONE', *, *, #25076, .F. ) ;
#70252=AXIS2_PLACEMENT_3D ( 'NONE', #27430, #33356, #47861 ) ;
#70254=VECTOR ( 'NONE', #39448, 1000.000000000000000 ) ;
#70255=DIRECTION ( 'NONE',  ( 1.000000000000000000, 0.000000000000000000, -1.147230458779309805E-16 ) ) ;
#70256=CARTESIAN_POINT ( 'NONE',  ( 97.81168148112675453, -40.51739256386586163, 162.6360428395636859 ) ) ;
#70257=CARTESIAN_POINT ( 'NONE',  ( 115.0898634087918850, -30.61888143515580296, 19.34376026548776650 ) ) ;
#70258=FACE_OUTER_BOUND ( 'NONE', #65328, .T. ) ;
#70263=CARTESIAN_POINT ( 'NONE',  ( 110.2773916389478188, -46.62487827714380018, 12.82705384733995402 ) ) ;
#70264=LINE ( 'NONE', #52341, #45834 ) ;
#70268=CARTESIAN_POINT ( 'NONE',  ( 103.8598393684536632, -44.23592174987565073, 90.07380465530594904 ) ) ;
#70269=DIRECTION ( 'NONE',  ( 0.7071067811865535679, -0.7071067811865415775, 7.071067811865543372E-16 ) ) ;
#70270=CARTESIAN_POINT ( 'NONE',  ( 99.09570907421795027, -30.55043175556566482, 45.80229194281738359 ) ) ;
#70271=EDGE_LOOP ( 'NONE', ( #9244, #5101 ) ) ;
#70273=DIRECTION ( 'NONE',  ( -0.9254794337955620787, -0.3787978585227822492, 0.000000000000000000 ) ) ;
#70274=VERTEX_POINT ( 'NONE', #18654 ) ;
#70276=CARTESIAN_POINT ( 'NONE',  ( 115.5299003720540014, -39.45574047089768754, 155.0101547344689550 ) ) ;
#70277=FACE_OUTER_BOUND ( 'NONE', #722, .T. ) ;
#70279=CARTESIAN_POINT ( 'NONE',  ( 112.5256494142567192, -27.82244069900259476, 90.63848241876793566 ) ) ;
#70280=CONICAL_SURFACE ( 'NONE', #29630, 11.57110091390437034, 0.7853981633974457255 ) ;
#70283=VECTOR ( 'NONE', #15928, 1000.000000000000000 ) ;
#70284=VERTEX_POINT ( 'NONE', #40434 ) ;
#70285=ORIENTED_EDGE ( 'NONE', *, *, #57102, .F. ) ;
#70289=DIRECTION ( 'NONE',  ( -0.9254794337955620787, -0.3787978585227822492, 0.000000000000000000 ) ) ;
#70290=VERTEX_POINT ( 'NONE', #74062 ) ;
#70291=CARTESIAN_POINT ( 'NONE',  ( 115.9265467165008232, -42.18176083994495684, 18.38705384733896153 ) ) ;
#70292=CARTESIAN_POINT ( 'NONE',  ( 117.4790109288255309, -40.50628101140208770, 169.5375300378159693 ) ) ;
#70294=DIRECTION ( 'NONE',  ( 2.056463827196271584E-15, -0.8571673007021100021, 0.5150380749100580413 ) ) ;
#70295=CARTESIAN_POINT ( 'NONE',  ( 111.7941755367341443, -25.86282203548705283, 130.7499109901969518 ) ) ;
#70296=DIRECTION ( 'NONE',  ( 0.7071067811989697471, 0.7071067811741252873, 7.071067811989691343E-16 ) ) ;
#70297=ORIENTED_EDGE ( 'NONE', *, *, #65282, .T. ) ;
#70298=DIRECTION ( 'NONE',  ( 0.7071067811866279529, -0.7071067811864671926, 7.071067811866286874E-16 ) ) ;
#70299=EDGE_CURVE ( 'NONE', #72137, #86716, #20003, .T. ) ;
#70309=CARTESIAN_POINT ( 'NONE',  ( 96.71451373887593661, -37.96385262316839260, 41.42133956162496844 ) ) ;
#70311=VECTOR ( 'NONE', #65178, 1000.000000000000000 ) ;
#70312=EDGE_CURVE ( 'NONE', #41323, #58627, #36076, .T. ) ;
#70313=CARTESIAN_POINT ( 'NONE',  ( 167.6524903400753601, -49.32844715993521589, 300.4678068554149490 ) ) ;
#70314=CARTESIAN_POINT ( 'NONE',  ( 116.7951252721156266, -39.38782978729904727, 74.61479194280059346 ) ) ;
#70315=CARTESIAN_POINT ( 'NONE',  ( 97.58158007118568378, -32.53714515026960896, 55.98324432352996638 ) ) ;
#70316=CARTESIAN_POINT ( 'NONE',  ( 98.34959472676385417, -31.65703098628569379, 110.9064992847184783 ) ) ;
#70317=CARTESIAN_POINT ( 'NONE',  ( 108.0049669398584911, -26.36739623290736390, 151.0041967044829505 ) ) ;
#70318=FACE_OUTER_BOUND ( 'NONE', #31700, .T. ) ;
#70320=ORIENTED_EDGE ( 'NONE', *, *, #19232, .F. ) ;
#70322=AXIS2_PLACEMENT_3D ( 'NONE', #159, #77362, #42369 ) ;
#70325=DIRECTION ( 'NONE',  ( 0.000000000000000000, 1.000000000000000000, 0.000000000000000000 ) ) ;
#70327=EDGE_CURVE ( 'NONE', #4991, #48663, #63635, .T. ) ;
#70328=DIRECTION ( 'NONE',  ( -0.7071067811865773267, 0.7071067811865178188, -7.071067811865781017E-16 ) ) ;
#70329=CARTESIAN_POINT ( 'NONE',  ( 117.3348906646497909, -34.51323323996641079, 183.9956252759109532 ) ) ;
#70330=ORIENTED_EDGE ( 'NONE', *, *, #79338, .T. ) ;
#70331=DIRECTION ( 'NONE',  ( 0.000000000000000000, 0.000000000000000000, 1.000000000000000000 ) ) ;
#70332=CARTESIAN_POINT ( 'NONE',  ( 98.51983665003312751, -30.72177789114069313, 201.8384824187679385 ) ) ;
#70333=CARTESIAN_POINT ( 'NONE',  ( 117.1483892680215888, -39.54869380112744892, 94.60991099019693706 ) ) ;
#70335=CARTESIAN_POINT ( 'NONE',  ( 115.8236631867570878, -31.72696035637653011, 190.2397867966467402 ) ) ;
#70336=EDGE_CURVE ( 'NONE', #59590, #65933, #76753, .T. ) ;
#70337=CARTESIAN_POINT ( 'NONE',  ( 165.3359832912740046, -36.32844715994100682, 342.9256252759119548 ) ) ;
#70338=ORIENTED_EDGE ( 'NONE', *, *, #29375, .T. ) ;
#70339=CIRCLE ( 'NONE', #89209, 7.499999999999992895 ) ;
#70340=ORIENTED_EDGE ( 'NONE', *, *, #43696, .T. ) ;
#70341=VERTEX_POINT ( 'NONE', #42652 ) ;
#70344=CARTESIAN_POINT ( 'NONE',  ( 105.6320745483020147, -47.05538338894268691, 253.4670538473393719 ) ) ;
#70345=DIRECTION ( 'NONE',  ( -1.000000000000000000, -4.299999999999999979E-14, -1.000000000000000078E-15 ) ) ;
#70349=LINE ( 'NONE', #8579, #73272 ) ;
#70351=CARTESIAN_POINT ( 'NONE',  ( 136.8164832912739826, -18.72944715994099951, 14.92562527591100263 ) ) ;
#70352=CARTESIAN_POINT ( 'NONE',  ( 112.1921266949303373, -27.58526089107821733, 34.66991099019695355 ) ) ;
#70353=ORIENTED_EDGE ( 'NONE', *, *, #78173, .T. ) ;
#70354=AXIS2_PLACEMENT_3D ( 'NONE', #76486, #41941, #41495 ) ;
#70356=CARTESIAN_POINT ( 'NONE',  ( 134.0664832912740110, -41.22944715994101017, 8.225625275910998013 ) ) ;
#70357=VECTOR ( 'NONE', #72565, 1000.000000000000000 ) ;
#70358=CARTESIAN_POINT ( 'NONE',  ( 99.09613892721601758, -30.54985836692837964, 16.80516855958618549 ) ) ;
#70360=CARTESIAN_POINT ( 'NONE',  ( 103.3362402991319584, -47.20309360805207177, 248.3041967044819387 ) ) ;
#70361=CYLINDRICAL_SURFACE ( 'NONE', #32707, 0.5000000000000197620 ) ;
#70362=CARTESIAN_POINT ( 'NONE',  ( 96.71010325458821910, -37.26253042779857338, 117.3794347997199594 ) ) ;
#70368=ORIENTED_EDGE ( 'NONE', *, *, #10532, .F. ) ;
#70370=CARTESIAN_POINT ( 'NONE',  ( 97.00631399252166887, -37.24296311215223909, 267.7987261630397029 ) ) ;
#70371=EDGE_CURVE ( 'NONE', #70652, #14566, #14537, .T. ) ;
#70373=CARTESIAN_POINT ( 'NONE',  ( 51.42025729304100423, -33.70561438051981185, -5.074374724088000832 ) ) ;
#70375=VECTOR ( 'NONE', #46087, 1000.000000000000000 ) ;
#70376=CARTESIAN_POINT ( 'NONE',  ( 102.0668027733616441, -27.97064593957984968, 140.4898149731944272 ) ) ;
#70378=CARTESIAN_POINT ( 'NONE',  ( 80.06648329127401098, -39.47944715994105991, 1.625625275910943746 ) ) ;
#70380=VERTEX_POINT ( 'NONE', #29057 ) ;
#70382=DIRECTION ( 'NONE',  ( 0.9254794337955621897, 0.3787978585227821382, 0.000000000000000000 ) ) ;
#70384=CARTESIAN_POINT ( 'NONE',  ( 115.6114045197296178, -28.51818617053012161, 39.43562527591099354 ) ) ;
#70386=CARTESIAN_POINT ( 'NONE',  ( 105.5338363264665986, -28.21170577469638729, 273.0242808457819592 ) ) ;
#70387=CIRCLE ( 'NONE', #18176, 0.5000000000000004441 ) ;
#70388=CARTESIAN_POINT ( 'NONE',  ( 109.6443389294615542, -46.47974508850531805, 127.7816520840981980 ) ) ;
#70389=CARTESIAN_POINT ( 'NONE',  ( 114.5468542906243243, -29.54732804739393615, 189.4232443235299570 ) ) ;
#70392=FACE_OUTER_BOUND ( 'NONE', #72695, .T. ) ;
#70393=PLANE ( 'NONE',  #43593 ) ;
#70395=EDGE_CURVE ( 'NONE', #27672, #5931, #14075, .T. ) ;
#70396=CARTESIAN_POINT ( 'NONE',  ( 96.49300521333343283, -40.10570368261699059, 277.5603871806730467 ) ) ;
#70397=CARTESIAN_POINT ( 'NONE',  ( 104.0320542673484852, -46.27522442963353200, 117.3334030146819202 ) ) ;
#70399=CARTESIAN_POINT ( 'NONE',  ( 141.8664832912740223, -71.52944715994085811, 394.9756252759100903 ) ) ;
#70400=EDGE_LOOP ( 'NONE', ( #2436, #4884 ) ) ;
#70401=CARTESIAN_POINT ( 'NONE',  ( 101.6557087385557736, -27.03816153323032268, 101.4937205140059575 ) ) ;
#70402=LINE ( 'NONE', #55394, #39582 ) ;
#70406=VECTOR ( 'NONE', #68770, 1000.000000000000000 ) ;
#70407=ORIENTED_EDGE ( 'NONE', *, *, #65658, .F. ) ;
#70409=EDGE_CURVE ( 'NONE', #66948, #34067, #41761, .T. ) ;
#70411=DIRECTION ( 'NONE',  ( 0.000000000000000000, 0.000000000000000000, 1.000000000000000000 ) ) ;
#70413=CARTESIAN_POINT ( 'NONE',  ( 97.33784628398525740, -34.07104680458591162, 267.1147904887237701 ) ) ;
#70414=DIRECTION ( 'NONE',  ( 1.000000000000000000, -3.885780586187990841E-13, 0.000000000000000000 ) ) ;
#70417=CARTESIAN_POINT ( 'NONE',  ( 106.2521435260052698, -26.30072798870746453, 21.13848241876792144 ) ) ;
#70419=ORIENTED_EDGE ( 'NONE', *, *, #58682, .F. ) ;
#70422=CARTESIAN_POINT ( 'NONE',  ( 113.1782915013152007, -44.75187050426813329, 43.09357499818941051 ) ) ;
#70423=VERTEX_POINT ( 'NONE', #77657 ) ;
#70424=ORIENTED_EDGE ( 'NONE', *, *, #55304, .T. ) ;
#70425=EDGE_CURVE ( 'NONE', #18492, #39136, #27373, .T. ) ;
#70426=CARTESIAN_POINT ( 'NONE',  ( 82.81648329127398256, -18.72944715994105636, 3.101481641215461327 ) ) ;
#70432=CARTESIAN_POINT ( 'NONE',  ( 102.4446420578519934, -44.51733865501087450, 206.5848007804579538 ) ) ;
#70433=FACE_OUTER_BOUND ( 'NONE', #65972, .T. ) ;
#70435=CARTESIAN_POINT ( 'NONE',  ( 112.5373769503831625, -27.80330641407773840, 94.63848241876793566 ) ) ;
#70436=ORIENTED_EDGE ( 'NONE', *, *, #36483, .F. ) ;
#70438=ORIENTED_EDGE ( 'NONE', *, *, #54800, .T. ) ;
#70439=CARTESIAN_POINT ( 'NONE',  ( 106.6049069045543405, -26.71869322362929822, 276.1132126703095082 ) ) ;
#70440=ORIENTED_EDGE ( 'NONE', *, *, #46264, .T. ) ;
#70441=LINE ( 'NONE', #64964, #88294 ) ;
#70446=CIRCLE ( 'NONE', #47192, 2.500000000000002220 ) ;
#70448=CARTESIAN_POINT ( 'NONE',  ( 118.0253644177900156, -38.34139182134431678, 73.72229194257801055 ) ) ;
#70449=AXIS2_PLACEMENT_3D ( 'NONE', #72372, #17840, #4215 ) ;
#70450=AXIS2_PLACEMENT_3D ( 'NONE', #10151, #43766, #65112 ) ;
#70452=AXIS2_PLACEMENT_3D ( 'NONE', #30416, #58113, #70869 ) ;
#70453=CARTESIAN_POINT ( 'NONE',  ( 105.7988705769415958, -26.72411980046145530, 165.1773442352779853 ) ) ;
#70456=CARTESIAN_POINT ( 'NONE',  ( 113.1782937596609457, -44.75186860166526515, 143.0939586080882577 ) ) ;
#70458=AXIS2_PLACEMENT_3D ( 'NONE', #36502, #78295, #76484 ) ;
#70460=DIRECTION ( 'NONE',  ( -4.237773401492740281E-14, 1.000000000000000000, 0.000000000000000000 ) ) ;
#70461=CIRCLE ( 'NONE', #73154, 0.5000000000000104361 ) ;
#70463=CARTESIAN_POINT ( 'NONE',  ( 108.9888594788934029, -47.63768604335348300, 118.7032443235299723 ) ) ;
#70464=DIRECTION ( 'NONE',  ( -1.000000000000000078E-15, -1.000000000000000083E-30, 1.000000000000000000 ) ) ;
#70465=LINE ( 'NONE', #84558, #57198 ) ;
#70466=ADVANCED_FACE ( 'NONE', ( #20454, #48124 ), #75858, .F. ) ;
#70468=AXIS2_PLACEMENT_3D ( 'NONE', #43531, #86230, #15850 ) ;
#70471=FACE_OUTER_BOUND ( 'NONE', #9118, .T. ) ;
#70472=CARTESIAN_POINT ( 'NONE',  ( 98.82386243697619932, -31.40279086140556331, 141.8699109901959616 ) ) ;
#70473=CARTESIAN_POINT ( 'NONE',  ( 123.6837132603318423, -20.11243780205705534, 239.5838068554170377 ) ) ;
#70475=CARTESIAN_POINT ( 'NONE',  ( 97.57986484199628308, -43.79006170206856297, 257.8356252759109566 ) ) ;
#70476=PLANE ( 'NONE',  #62852 ) ;
#70480=FACE_OUTER_BOUND ( 'NONE', #37871, .T. ) ;
#70482=CARTESIAN_POINT ( 'NONE',  ( 102.5357197525641766, -45.39752751535337438, 212.1927681330539599 ) ) ;
#70483=EDGE_LOOP ( 'NONE', ( #43816, #71388, #59843, #30389, #81349, #42789, #17774, #39646 ) ) ;
#70485=AXIS2_PLACEMENT_3D ( 'NONE', #62221, #8623, #82696 ) ;
#70486=CARTESIAN_POINT ( 'NONE',  ( 101.8133294234851860, -44.51716929413077395, 148.5234880678019351 ) ) ;
#70489=CARTESIAN_POINT ( 'NONE',  ( 110.6847694559308621, -28.64017749364363397, 21.17301187732595480 ) ) ;
#70490=VECTOR ( 'NONE', #26593, 1000.000000000000000 ) ;
#70491=FACE_OUTER_BOUND ( 'NONE', #24850, .T. ) ;
#70492=DIRECTION ( 'NONE',  ( 2.056463827196271584E-15, -0.8571673007021100021, 0.5150380749100580413 ) ) ;
#70493=LINE ( 'NONE', #29596, #22672 ) ;
#70494=CARTESIAN_POINT ( 'NONE',  ( 99.09570907225396752, -30.55043175805740674, 106.8022919430684539 ) ) ;
#70496=CARTESIAN_POINT ( 'NONE',  ( 98.05565822401619869, -44.38798742045811707, 226.8870538473399563 ) ) ;
#70497=CARTESIAN_POINT ( 'NONE',  ( 97.33770779590314248, -34.07148707886162953, 171.1142724482292863 ) ) ;
#70500=CARTESIAN_POINT ( 'NONE',  ( 117.0608945230788578, -38.08045312548524919, 88.71895860887195795 ) ) ;
#70502=CARTESIAN_POINT ( 'NONE',  ( 101.9936016578518974, -45.44608281785205861, 123.1551631644055220 ) ) ;
#70503=DIRECTION ( 'NONE',  ( 0.000000000000000000, 1.000000000000000000, 0.000000000000000000 ) ) ;
#70504=CARTESIAN_POINT ( 'NONE',  ( 106.5519926023875712, -26.37212682281792198, 41.12800622829093555 ) ) ;
#70505=CIRCLE ( 'NONE', #51605, 4.750000000000000888 ) ;
#70507=ORIENTED_EDGE ( 'NONE', *, *, #44793, .F. ) ;
#70508=AXIS2_PLACEMENT_3D ( 'NONE', #80988, #67320, #5110 ) ;
#70509=FACE_OUTER_BOUND ( 'NONE', #49311, .T. ) ;
#70510=CIRCLE ( 'NONE', #35674, 0.5000000000000004441 ) ;
#70511=CARTESIAN_POINT ( 'NONE',  ( 63.06670390244732971, -24.92844715994017690, 300.4678068554150627 ) ) ;
#70512=CARTESIAN_POINT ( 'NONE',  ( 97.16957671423683962, -40.00637722736999535, 241.5813395616249863 ) ) ;
#70513=EDGE_CURVE ( 'NONE', #27030, #21043, #49336, .T. ) ;
#70514=EDGE_LOOP ( 'NONE', ( #63111, #4107, #48318, #7316, #42585 ) ) ;
#70515=EDGE_CURVE ( 'NONE', #15623, #4781, #1805, .T. ) ;
#70517=LINE ( 'NONE', #40998, #26861 ) ;
#70518=EDGE_CURVE ( 'NONE', #73072, #25446, #50371, .T. ) ;
#70519=CARTESIAN_POINT ( 'NONE',  ( 116.3573301164176712, -40.55459570680316972, 168.5154237022636039 ) ) ;
#70520=CARTESIAN_POINT ( 'NONE',  ( 113.2960346059783774, -42.04690695427109404, 61.08237608387695161 ) ) ;
#70521=CARTESIAN_POINT ( 'NONE',  ( 96.02367466659750050, -35.86829477906547226, 187.2765776568629406 ) ) ;
#70522=CARTESIAN_POINT ( 'NONE',  ( 57.56670390244744340, -48.82844715994040286, 175.7178068554150911 ) ) ;
#70523=EDGE_LOOP ( 'NONE', ( #61880, #75507, #31656, #56050 ) ) ;
#70525=VECTOR ( 'NONE', #64443, 1000.000000000000000 ) ;
#70527=ORIENTED_EDGE ( 'NONE', *, *, #55173, .T. ) ;
#70528=ORIENTED_EDGE ( 'NONE', *, *, #3657, .F. ) ;
#70529=FACE_OUTER_BOUND ( 'NONE', #5263, .T. ) ;
#70531=ORIENTED_EDGE ( 'NONE', *, *, #11329, .F. ) ;
#70532=DIRECTION ( 'NONE',  ( 0.000000000000000000, 0.000000000000000000, -1.000000000000000000 ) ) ;
#70534=CARTESIAN_POINT ( 'NONE',  ( 108.0458233943899273, -25.31222262750819851, 322.3938544957129011 ) ) ;
#70535=EDGE_CURVE ( 'NONE', #84821, #8522, #30395, .T. ) ;
#70536=CARTESIAN_POINT ( 'NONE',  ( 99.71754419879584930, -32.37637629707774778, 85.32384839950596245 ) ) ;
#70537=CARTESIAN_POINT ( 'NONE',  ( 97.59524074137092953, -41.13874739096760891, 256.6727681330537507 ) ) ;
#70541=VERTEX_POINT ( 'NONE', #85385 ) ;
#70543=CYLINDRICAL_SURFACE ( 'NONE', #69586, 4.750000000000000888 ) ;
#70544=DIRECTION ( 'NONE',  ( -0.000000000000000000, -0.000000000000000000, -1.000000000000000000 ) ) ;
#70545=CARTESIAN_POINT ( 'NONE',  ( 117.1895451461017643, -38.97942580829906944, 103.6403871806739545 ) ) ;
#70546=CARTESIAN_POINT ( 'NONE',  ( 117.2525043769621362, -39.29786468180206782, 123.6299109901969615 ) ) ;
#70547=DIRECTION ( 'NONE',  ( 0.000000000000000000, 0.000000000000000000, 1.000000000000000000 ) ) ;
#70550=CARTESIAN_POINT ( 'NONE',  ( 104.1857688441879191, -26.67323559945603151, 225.2984824187679749 ) ) ;
#70554=CARTESIAN_POINT ( 'NONE',  ( 34.67381068362099228, -26.00627455219321860, -5.074374724088000832 ) ) ;
#70555=CARTESIAN_POINT ( 'NONE',  ( 41.56648329127398966, -27.57844715994070484, 138.9256252759119832 ) ) ;
#70558=CARTESIAN_POINT ( 'NONE',  ( 132.1654742078777360, -38.71744337671164971, 7.623533105443405233 ) ) ;
#70561=FACE_OUTER_BOUND ( 'NONE', #40490, .T. ) ;
#70562=DIRECTION ( 'NONE',  ( 0.000000000000000000, 0.000000000000000000, -1.000000000000000000 ) ) ;
#70564=CARTESIAN_POINT ( 'NONE',  ( 123.0664832912757163, -36.72944715993921960, -5.074374724089014244 ) ) ;
#70565=CARTESIAN_POINT ( 'NONE',  ( 99.52336843529489840, -29.45003914207232754, 250.7156252759109520 ) ) ;
#70566=CARTESIAN_POINT ( 'NONE',  ( 112.7801043229996338, -45.44936815460292934, 174.0384824187679556 ) ) ;
#70567=CARTESIAN_POINT ( 'NONE',  ( 96.51983850151567879, -40.19180362902228865, 282.5908633711491120 ) ) ;
#70568=VECTOR ( 'NONE', #11967, 999.9999999999997726 ) ;
#70569=DIRECTION ( 'NONE',  ( -0.000000000000000000, 1.000000000000000000, 0.000000000000000000 ) ) ;
#70571=CARTESIAN_POINT ( 'NONE',  ( 82.06789631128971507, -34.84294903900328677, 7.549690073101738008 ) ) ;
#70573=DIRECTION ( 'NONE',  ( 0.000000000000000000, 0.000000000000000000, -1.000000000000000000 ) ) ;
#70574=AXIS2_PLACEMENT_3D ( 'NONE', #76128, #13911, #40258 ) ;
#70576=EDGE_CURVE ( 'NONE', #87053, #29939, #58966, .T. ) ;
#70577=ORIENTED_EDGE ( 'NONE', *, *, #39315, .F. ) ;
#70580=CARTESIAN_POINT ( 'NONE',  ( 103.4754675462218927, -28.97956086136533926, 179.8438483995059869 ) ) ;
#70581=LINE ( 'NONE', #13819, #32637 ) ;
#70582=ORIENTED_EDGE ( 'NONE', *, *, #80901, .F. ) ;
#70583=LINE ( 'NONE', #34703, #27239 ) ;
#70584=CARTESIAN_POINT ( 'NONE',  ( 98.68348088377354088, -30.50934295487602199, 176.8184824187679567 ) ) ;
#70585=DIRECTION ( 'NONE',  ( 0.7071067811865473507, 0.000000000000000000, -0.7071067811865476838 ) ) ;
#70586=PLANE ( 'NONE',  #26925 ) ;
#70587=CARTESIAN_POINT ( 'NONE',  ( 102.1022249014249184, -28.02397532599129093, 86.48945707807658323 ) ) ;
#70588=CARTESIAN_POINT ( 'NONE',  ( 36.23715912545424089, -47.82818131006125384, 300.4678068554150059 ) ) ;
#70589=CYLINDRICAL_SURFACE ( 'NONE', #87512, 2.116999999999980009 ) ;
#70591=CARTESIAN_POINT ( 'NONE',  ( 100.7170190823676279, -45.85612711270997011, 87.09276813305393716 ) ) ;
#70593=ORIENTED_EDGE ( 'NONE', *, *, #50070, .F. ) ;
#70595=CARTESIAN_POINT ( 'NONE',  ( 116.3620231750148406, -38.09673052741934640, 70.15396425827796634 ) ) ;
#70596=ADVANCED_FACE ( 'NONE', ( #79904, #51706 ), #79456, .T. ) ;
#70598=CARTESIAN_POINT ( 'NONE',  ( 115.7764676695377517, -43.63945112744033850, 194.2927681330539542 ) ) ;
#70599=CARTESIAN_POINT ( 'NONE',  ( 116.3229784443844324, -32.93528945216412041, 94.13562527591096796 ) ) ;
#70600=DIRECTION ( 'NONE',  ( 1.000000000000000000, 4.163336342344333240E-14, 0.000000000000000000 ) ) ;
#70601=CARTESIAN_POINT ( 'NONE',  ( 80.06648329127399677, 0.2215528400590013880, 4.925625275911999168 ) ) ;
#70602=LINE ( 'NONE', #29709, #72143 ) ;
#70605=CARTESIAN_POINT ( 'NONE',  ( 117.2009162446675390, -42.82382785266567993, 128.3956252759109873 ) ) ;
#70607=ORIENTED_EDGE ( 'NONE', *, *, #42269, .T. ) ;
#70608=ORIENTED_EDGE ( 'NONE', *, *, #18724, .F. ) ;
#70611=CARTESIAN_POINT ( 'NONE',  ( 113.1782937644530307, -44.75186859791577376, 79.09395860856413663 ) ) ;
#70613=CARTESIAN_POINT ( 'NONE',  ( 115.2156275924750020, -36.25915663771239394, 226.6909475124489575 ) ) ;
#70615=LINE ( 'NONE', #15656, #24751 ) ;
#70616=CYLINDRICAL_SURFACE ( 'NONE', #8324, 9.999999999999998224 ) ;
#70619=ORIENTED_EDGE ( 'NONE', *, *, #7630, .F. ) ;
#70624=DIRECTION ( 'NONE',  ( 0.000000000000000000, 0.000000000000000000, -1.000000000000000000 ) ) ;
#70627=CARTESIAN_POINT ( 'NONE',  ( 100.1609931986295976, -31.17584605865120295, 237.2187261630399746 ) ) ;
#70628=CARTESIAN_POINT ( 'NONE',  ( 97.81186544543886896, -40.51730612966257183, 271.6361395295153898 ) ) ;
#70629=EDGE_LOOP ( 'NONE', ( #1319, #79358 ) ) ;
#70630=AXIS2_PLACEMENT_3D ( 'NONE', #77443, #17008, #43801 ) ;
#70631=B_SPLINE_CURVE_WITH_KNOTS ( 'NONE', 3,
 ( #66507, #4296, #31986, #25173, #43827, #9327, #16590, #64736, #2520, #53747, #74673, #67857, #12451, #41037, #26081, #54642, #47841, #88764, #26522, #81515, #12906, #40595, #11562, #87860, #54195, #68311, #19268, #34223, #32882, #46942, #39254, #60581, #88323, #53301, #39692, #12009, #67397, #68759, #73776, #75579, #18358, #6527, #82405, #32423, #40137, #46043, #61033, #5645, #18813, #33337, #60126, #25625, #47391, #13350, #61928, #81958, #5189, #46495, #61477, #6093, #89659, #20167, #27409, #4742, #19706, #66962, #81066, #74233, #33782, #75122, #89210, #26976, #80609, #20612, #28299, #62823, #36024, #83737, #62377, #21514, #21057, #35566 ),
 .UNSPECIFIED., .F., .F.,
 ( 4, 2, 2, 2, 2, 2, 2, 2, 2, 2, 2, 2, 2, 2, 2, 2, 2, 2, 2, 2, 2, 2, 2, 2, 2, 2, 2, 2, 2, 2, 2, 2, 2, 2, 2, 2, 2, 2, 2, 2, 4 ),
 ( 7.021675287307244464E-05, 0.0002385562018683249643, 0.0004068956508635774975, 0.0007435745488541031095, 0.001416932344835133408, 0.002763647936797193356, 0.004110363528759253086, 0.005457079120721313251, 0.006803794712683372548, 0.007477152508664412604, 0.008150510304645452661, 0.009497225896607553591, 0.01084394148856965626, 0.01219065708053175892, 0.01353737267249385812, 0.01488408826445596078, 0.01623080385641805998, 0.01892423504034226531, 0.02027095063230434716, 0.02161766622426642900, 0.02296438181622851432, 0.02431109740819059617, 0.02498445520417162669, 0.02565781300015265720, 0.02700452859211470436, 0.02835124418407675845, 0.02969795977603881601, 0.03104467536800087010, 0.03239139095996292766, 0.03306474875594395124, 0.03373810655192497482, 0.03508482214388704973, 0.03643153773584913158, 0.03777825332781119955, 0.03912496891977328140, 0.04047168451173535630, 0.04181840010369743815, 0.04249175789967847561, 0.04282843679766901168, 0.04299677624666430054, 0.04316511569565958245 ),
 .UNSPECIFIED. ) ;
#70632=DIRECTION ( 'NONE',  ( 1.000000000000000000, 4.299999999999999979E-14, 1.000000000000000078E-15 ) ) ;
#70633=CARTESIAN_POINT ( 'NONE',  ( 107.0664832912739399, -36.72944715994095333, 315.6356252759111953 ) ) ;
#70634=VERTEX_POINT ( 'NONE', #34292 ) ;
#70635=ORIENTED_EDGE ( 'NONE', *, *, #3874, .F. ) ;
#70637=CIRCLE ( 'NONE', #47382, 2.029999999999997140 ) ;
#70639=AXIS2_PLACEMENT_3D ( 'NONE', #8609, #57630, #70837 ) ;
#70640=EDGE_LOOP ( 'NONE', ( #15297, #46019, #47035, #59199 ) ) ;
#70641=ORIENTED_EDGE ( 'NONE', *, *, #3814, .F. ) ;
#70643=CARTESIAN_POINT ( 'NONE',  ( 101.0492827672293714, -31.21374014463884805, 273.5538046553056688 ) ) ;
#70644=CARTESIAN_POINT ( 'NONE',  ( 102.9045757522767843, -27.10877478265368623, 155.4013395616249795 ) ) ;
#70645=CARTESIAN_POINT ( 'NONE',  ( 96.66376384204015437, -36.61947630124858932, 111.3184824187679567 ) ) ;
#70646=LINE ( 'NONE', #36117, #21075 ) ;
#70649=CARTESIAN_POINT ( 'NONE',  ( 113.1000543987032785, -45.99065659369661319, 219.0480062282919960 ) ) ;
#70650=FACE_OUTER_BOUND ( 'NONE', #73050, .T. ) ;
#70651=CARTESIAN_POINT ( 'NONE',  ( 46.32460016641637424, -48.34074026909789268, 180.4678068554150911 ) ) ;
#70652=VERTEX_POINT ( 'NONE', #21128 ) ;
#70654=ORIENTED_EDGE ( 'NONE', *, *, #59885, .T. ) ;
#70658=CIRCLE ( 'NONE', #82272, 2.517499999999998739 ) ;
#70659=ORIENTED_EDGE ( 'NONE', *, *, #11540, .F. ) ;
#70660=CARTESIAN_POINT ( 'NONE',  ( 102.6975360555999259, -46.88284006984166297, 137.2651490854349561 ) ) ;
#70662=CARTESIAN_POINT ( 'NONE',  ( 136.2652213603992948, -35.07517613920733623, 7.387586420634884021 ) ) ;
#70663=DIRECTION ( 'NONE',  ( 1.000000000000000078E-15, -1.000000000000000083E-30, -1.000000000000000000 ) ) ;
#70664=DIRECTION ( 'NONE',  ( 8.568612280716163558E-05, -0.4999999926578935772, -0.8660254037844357100 ) ) ;
#70665=CARTESIAN_POINT ( 'NONE',  ( 93.56648329127393993, -36.72944715994093912, 311.6356252759112522 ) ) ;
#70666=CARTESIAN_POINT ( 'NONE',  ( 116.8642987764956160, -41.79567201640973195, 239.4346728949589647 ) ) ;
#70668=CARTESIAN_POINT ( 'NONE',  ( 107.0664832912739683, -25.27030990763060103, 305.0306255462182321 ) ) ;
#70669=FACE_OUTER_BOUND ( 'NONE', #87963, .T. ) ;
#70670=CYLINDRICAL_SURFACE ( 'NONE', #86316, 5.599999999999994316 ) ;
#70671=PLANE ( 'NONE',  #19861 ) ;
#70673=CARTESIAN_POINT ( 'NONE',  ( 118.1543649935527185, -36.20813824561556515, 268.8518157521014587 ) ) ;
#70676=CARTESIAN_POINT ( 'NONE',  ( 113.3446846601215441, -45.07992904040708737, 143.0899109901969553 ) ) ;
#70677=CARTESIAN_POINT ( 'NONE',  ( 110.5551769720564863, -46.59100632561725064, 33.84705384733993583 ) ) ;
#70678=CARTESIAN_POINT ( 'NONE',  ( 107.5678551521628492, -47.81755451042874228, 188.6003871806729535 ) ) ;
#70680=DIRECTION ( 'NONE',  ( 4.299999999999999979E-14, -1.000000000000000000, 4.400000000000000367E-29 ) ) ;
#70683=CARTESIAN_POINT ( 'NONE',  ( 120.3352449817834895, -37.86742168929413310, 299.5704287327187103 ) ) ;
#70685=ORIENTED_EDGE ( 'NONE', *, *, #22923, .T. ) ;
#70688=EDGE_CURVE ( 'NONE', #63748, #7464, #46216, .T. ) ;
#70690=VERTEX_POINT ( 'NONE', #59420 ) ;
#70692=ORIENTED_EDGE ( 'NONE', *, *, #40986, .T. ) ;
#70693=CARTESIAN_POINT ( 'NONE',  ( 100.9539191370902387, -46.85292318231929443, 48.14419670448194211 ) ) ;
#70694=CARTESIAN_POINT ( 'NONE',  ( 21.03689327557711763, -23.42844715994186089, 249.9678068554150059 ) ) ;
#70695=CARTESIAN_POINT ( 'NONE',  ( 20.03715912545637678, -24.42818131006202265, 193.9678068554150627 ) ) ;
#70696=CARTESIAN_POINT ( 'NONE',  ( 113.6418603426413938, -28.58344220020606130, 160.5356252759109736 ) ) ;
#70697=CIRCLE ( 'NONE', #37295, 0.4999999999999932832 ) ;
#70698=VECTOR ( 'NONE', #9478, 1000.000000000000000 ) ;
#70699=CARTESIAN_POINT ( 'NONE',  ( 107.8428746604417654, -27.05123223485975714, 264.4352769709337849 ) ) ;
#70700=ORIENTED_EDGE ( 'NONE', *, *, #28258, .F. ) ;
#70701=ORIENTED_EDGE ( 'NONE', *, *, #78966, .F. ) ;
#70702=ORIENTED_EDGE ( 'NONE', *, *, #17207, .T. ) ;
#70706=ORIENTED_EDGE ( 'NONE', *, *, #79687, .T. ) ;
#70707=CARTESIAN_POINT ( 'NONE',  ( 116.7951252717554098, -39.38782978876485430, 108.6147919426823734 ) ) ;
#70709=CIRCLE ( 'NONE', #47458, 37.00000000000000711 ) ;
#70712=CARTESIAN_POINT ( 'NONE',  ( 134.0664832912740110, 0.2215528400590013880, 4.925625275911999168 ) ) ;
#70713=DIRECTION ( 'NONE',  ( 0.000000000000000000, 0.000000000000000000, 1.000000000000000000 ) ) ;
#70714=CARTESIAN_POINT ( 'NONE',  ( 172.5664832912740110, 0.2215528400590013880, 138.9256252759119832 ) ) ;
#70716=CARTESIAN_POINT ( 'NONE',  ( 99.08262072259961428, -44.34008189452615056, 36.92038718067297509 ) ) ;
#70718=ADVANCED_FACE ( 'NONE', ( #33406 ), #82919, .F. ) ;
#70719=ORIENTED_EDGE ( 'NONE', *, *, #10486, .T. ) ;
#70721=EDGE_CURVE ( 'NONE', #15112, #50271, #17211, .T. ) ;
#70726=CARTESIAN_POINT ( 'NONE',  ( 112.5586783213544066, -42.80550525696455821, 130.9795189410199612 ) ) ;
#70727=CIRCLE ( 'NONE', #9766, 0.5000000000000004441 ) ;
#70728=EDGE_CURVE ( 'NONE', #13444, #89348, #66925, .T. ) ;
#70729=CARTESIAN_POINT ( 'NONE',  ( 97.81168844167092402, -40.51740470302234343, 181.6357138554620576 ) ) ;
#70732=ORIENTED_EDGE ( 'NONE', *, *, #36016, .F. ) ;
#70733=CARTESIAN_POINT ( 'NONE',  ( 115.0375080342936940, -42.90814572238593172, 138.3000974113143684 ) ) ;
#70734=ORIENTED_EDGE ( 'NONE', *, *, #44350, .F. ) ;
#70735=EDGE_LOOP ( 'NONE', ( #87240, #36064, #74147, #42447 ) ) ;
#70736=ADVANCED_FACE ( 'NONE', ( #61547 ), #75648, .T. ) ;
#70737=CARTESIAN_POINT ( 'NONE',  ( 103.7583319442197052, -28.50847317404091186, 126.8130118773259625 ) ) ;
#70739=CARTESIAN_POINT ( 'NONE',  ( 98.82287431334749783, -28.18163096472671469, 111.6870538473389587 ) ) ;
#70740=VECTOR ( 'NONE', #46059, 1000.000000000000000 ) ;
#70741=DIRECTION ( 'NONE',  ( 3.999999999999999995E-14, -1.000000000000000000, 4.100000000000000342E-29 ) ) ;
#70746=CARTESIAN_POINT ( 'NONE',  ( 118.0120547386033678, -38.42941975617429762, 68.69181575210198787 ) ) ;
#70747=ORIENTED_EDGE ( 'NONE', *, *, #8151, .F. ) ;
#70748=CARTESIAN_POINT ( 'NONE',  ( 117.4208826026019779, -36.15918394850536544, 273.8822919425783198 ) ) ;
#70749=CARTESIAN_POINT ( 'NONE',  ( 103.5350399278988078, -26.85989278392735002, 186.3499109901969746 ) ) ;
#70751=CARTESIAN_POINT ( 'NONE',  ( 107.0664832912748068, -36.72944715993923381, -5.074374724089029343 ) ) ;
#70752=CARTESIAN_POINT ( 'NONE',  ( 99.04385435236613944, -42.84094592217979169, 127.8439293676477462 ) ) ;
#70753=CARTESIAN_POINT ( 'NONE',  ( 95.77906782739819391, -40.33899944578667629, 127.5727681330539554 ) ) ;
#70755=EDGE_CURVE ( 'NONE', #5050, #26855, #36555, .T. ) ;
#70758=EDGE_CURVE ( 'NONE', #50262, #73333, #43341, .T. ) ;
#70759=CIRCLE ( 'NONE', #6878, 0.5000000000000004441 ) ;
#70760=VERTEX_POINT ( 'NONE', #64257 ) ;
#70761=DIRECTION ( 'NONE',  ( -1.000000000000000000, -2.422134843531340666E-15, 0.000000000000000000 ) ) ;
#70762=ORIENTED_EDGE ( 'NONE', *, *, #54903, .F. ) ;
#70764=VECTOR ( 'NONE', #57601, 1000.000000000000000 ) ;
#70766=AXIS2_PLACEMENT_3D ( 'NONE', #84227, #55121, #61956 ) ;
#70767=DIRECTION ( 'NONE',  ( 0.000000000000000000, 0.000000000000000000, 1.000000000000000000 ) ) ;
#70768=CARTESIAN_POINT ( 'NONE',  ( 116.3877942521162936, -31.98191425893181261, 44.20133956162491984 ) ) ;
#70769=CARTESIAN_POINT ( 'NONE',  ( 49.35211078756498893, -35.65087443492551245, -5.074374724088000832 ) ) ;
#70770=CARTESIAN_POINT ( 'NONE',  ( 101.3983180920321985, -48.92675847326103167, 9.425625275910963552 ) ) ;
#70772=CARTESIAN_POINT ( 'NONE',  ( 102.2761128416349123, -28.20209198692209185, 60.48419670448296159 ) ) ;
#70773=CARTESIAN_POINT ( 'NONE',  ( 97.12561475596668004, -37.99732759006241878, 111.4273445057939824 ) ) ;
#70774=CARTESIAN_POINT ( 'NONE',  ( 96.67182511810091228, -37.15340426533111895, 157.3584824187679487 ) ) ;
#70775=CARTESIAN_POINT ( 'NONE',  ( 168.5667039024483813, -48.82844715993517326, 249.9678068554149775 ) ) ;
#70776=CYLINDRICAL_SURFACE ( 'NONE', #35074, 4.874999999999990230 ) ;
#70778=DIRECTION ( 'NONE',  ( 0.000000000000000000, 0.000000000000000000, 1.000000000000000000 ) ) ;
#70779=AXIS2_PLACEMENT_3D ( 'NONE', #79782, #3899, #31596 ) ;
#70781=CARTESIAN_POINT ( 'NONE',  ( 172.5664832912740110, -18.82844715994099971, 318.9256252759120116 ) ) ;
#70782=VERTEX_POINT ( 'NONE', #85161 ) ;
#70783=VECTOR ( 'NONE', #43595, 1000.000000000000000 ) ;
#70785=CARTESIAN_POINT ( 'NONE',  ( 98.13053560861905567, -31.27458647820624549, 170.8899109901960003 ) ) ;
#70786=ORIENTED_EDGE ( 'NONE', *, *, #84686, .F. ) ;
#70788=CARTESIAN_POINT ( 'NONE',  ( 106.3003414554210764, -47.14819399153626023, 218.5184824187679453 ) ) ;
#70789=CARTESIAN_POINT ( 'NONE',  ( 117.0163018969640376, -33.47459087099611708, 85.07848241876791917 ) ) ;
#70794=LINE ( 'NONE', #35799, #64117 ) ;
#70797=VERTEX_POINT ( 'NONE', #49257 ) ;
#70798=VERTEX_POINT ( 'NONE', #1132 ) ;
#70799=PLANE ( 'NONE',  #59759 ) ;
#70800=CARTESIAN_POINT ( 'NONE',  ( 96.24939603668094890, -34.45687069020234361, 257.1737205140064475 ) ) ;
#70801=CARTESIAN_POINT ( 'NONE',  ( 97.12053416263984218, -35.23531894072210946, 251.2083665227183928 ) ) ;
#70802=CARTESIAN_POINT ( 'NONE',  ( 135.4870310422650732, -16.36767655970465540, 1.942446731291206596 ) ) ;
#70804=CARTESIAN_POINT ( 'NONE',  ( 25.56670390244797275, -48.82844715994099971, 139.9678068554150059 ) ) ;
#70807=CARTESIAN_POINT ( 'NONE',  ( 96.81178581975444786, -38.90419831550661911, 31.49276813305495892 ) ) ;
#70810=ORIENTED_EDGE ( 'NONE', *, *, #48335, .F. ) ;
#70811=EDGE_LOOP ( 'NONE', ( #5979, #44112, #61013, #53544 ) ) ;
#70812=DIRECTION ( 'NONE',  ( -1.000000000000000078E-15, -1.000000000000000083E-30, 1.000000000000000000 ) ) ;
#70813=CARTESIAN_POINT ( 'NONE',  ( 100.9553767296363702, -28.70647492237798559, 16.59715524421730137 ) ) ;
#70814=EDGE_CURVE ( 'NONE', #58395, #72856, #22932, .T. ) ;
#70815=CARTESIAN_POINT ( 'NONE',  ( 115.3604274781776411, -30.50455558986046256, 260.3508633711485345 ) ) ;
#70816=FACE_OUTER_BOUND ( 'NONE', #65410, .T. ) ;
#70818=CARTESIAN_POINT ( 'NONE',  ( 116.5394839232219510, -34.29517225379352396, 120.0270538473389479 ) ) ;
#70823=DIRECTION ( 'NONE',  ( 0.7071067811874278686, -0.7071067811856670549, 2.899137802861351288E-29 ) ) ;
#70825=CARTESIAN_POINT ( 'NONE',  ( 77.50946880809780737, -35.71735499139281700, 2.839545688279709434 ) ) ;
#70830=CARTESIAN_POINT ( 'NONE',  ( 111.0712550167563677, -29.58490437025668740, 32.48809036959193719 ) ) ;
#70832=VECTOR ( 'NONE', #44182, 1000.000000000000000 ) ;
#70833=CIRCLE ( 'NONE', #85370, 2.117000000000000881 ) ;
#70834=DIRECTION ( 'NONE',  ( 4.194175870806139918E-14, -1.000000000000000000, 0.000000000000000000 ) ) ;
#70836=CARTESIAN_POINT ( 'NONE',  ( 112.1393456466975636, -28.01282278429165729, 84.65645860877889106 ) ) ;
#70837=DIRECTION ( 'NONE',  ( -0.9254794337955620787, -0.3787978585227822492, 0.000000000000000000 ) ) ;
#70838=ORIENTED_EDGE ( 'NONE', *, *, #55348, .F. ) ;
#70839=DIRECTION ( 'NONE',  ( 2.900000000000000265E-14, -2.000000000000000155E-15, 1.000000000000000000 ) ) ;
#70841=CARTESIAN_POINT ( 'NONE',  ( 182.0374245136140701, -23.42844715993459559, 237.4678068554150059 ) ) ;
#70842=EDGE_LOOP ( 'NONE', ( #5286, #87455, #28388, #35604, #6876, #81872, #30971, #22037, #36684, #77748, #26279, #88819 ) ) ;
#70843=CARTESIAN_POINT ( 'NONE',  ( 117.4476241407275978, -37.68806341539836069, 78.75276813305399060 ) ) ;
#70845=CARTESIAN_POINT ( 'NONE',  ( 98.84295822536005005, -39.42912807745279480, 284.4090427505438470 ) ) ;
#70846=ADVANCED_FACE ( 'NONE', ( #22480 ), #35182, .T. ) ;
#70847=AXIS2_PLACEMENT_3D ( 'NONE', #51573, #59287, #44767 ) ;
#70848=LINE ( 'NONE', #7270, #2494 ) ;
#70849=CARTESIAN_POINT ( 'NONE',  ( 118.1473594538626486, -37.63838399483783093, 188.7613395616259595 ) ) ;
#70852=VECTOR ( 'NONE', #57174, 999.9999999999998863 ) ;
#70854=AXIS2_PLACEMENT_3D ( 'NONE', #36815, #16818, #15930 ) ;
#70856=CARTESIAN_POINT ( 'NONE',  ( 111.7585843298372197, -27.37117935058896379, 275.7070538473396937 ) ) ;
#70859=PLANE ( 'NONE',  #73398 ) ;
#70860=VERTEX_POINT ( 'NONE', #16112 ) ;
#70861=CARTESIAN_POINT ( 'NONE',  ( 108.7502231993919395, -25.75847702231262204, 140.9432443235299672 ) ) ;
#70863=ORIENTED_EDGE ( 'NONE', *, *, #79133, .F. ) ;
#70865=EDGE_LOOP ( 'NONE', ( #29441, #73642, #58757, #73965 ) ) ;
#70866=VECTOR ( 'NONE', #65489, 1000.000000000000114 ) ;
#70867=CARTESIAN_POINT ( 'NONE',  ( 105.7154772066486288, -46.72385837650929830, 122.4689585993907457 ) ) ;
#70869=DIRECTION ( 'NONE',  ( 0.000000000000000000, 0.000000000000000000, -1.000000000000000000 ) ) ;
#70872=CARTESIAN_POINT ( 'NONE',  ( 95.25919473906076007, -35.71823372881362957, 32.25848241876794020 ) ) ;
#70874=ADVANCED_FACE ( 'NONE', ( #62893 ), #38974, .F. ) ;
#70875=EDGE_LOOP ( 'NONE', ( #46343, #39480 ) ) ;
#70876=PLANE ( 'NONE',  #22507 ) ;
#70878=AXIS2_PLACEMENT_3D ( 'NONE', #62671, #84029, #15438 ) ;
#70882=ORIENTED_EDGE ( 'NONE', *, *, #47718, .T. ) ;
#70883=CARTESIAN_POINT ( 'NONE',  ( 81.24991378862624458, -21.21189172703844861, 1.845048092480171320 ) ) ;
#70884=CARTESIAN_POINT ( 'NONE',  ( 152.5667039024474718, -23.42844715993585325, 180.4678068554149775 ) ) ;
#70885=DIRECTION ( 'NONE',  ( 0.000000000000000000, 0.000000000000000000, 1.000000000000000000 ) ) ;
#70886=FACE_BOUND ( 'NONE', #80818, .T. ) ;
#70887=DIRECTION ( 'NONE',  ( 1.000000000000000078E-15, -1.000000000000000083E-30, -1.000000000000000000 ) ) ;
#70888=CARTESIAN_POINT ( 'NONE',  ( 109.6796103444932129, -28.56711482602328900, 234.2524198280769951 ) ) ;
#70891=CARTESIAN_POINT ( 'NONE',  ( 112.8260979389708183, -47.14365076028245483, 102.9784824187679817 ) ) ;
#70894=ORIENTED_EDGE ( 'NONE', *, *, #31629, .T. ) ;
#70896=CARTESIAN_POINT ( 'NONE',  ( 103.2784163218621529, -27.47468898029232065, 276.3856337844811719 ) ) ;
#70897=ORIENTED_EDGE ( 'NONE', *, *, #65386, .T. ) ;
#70898=AXIS2_PLACEMENT_3D ( 'NONE', #32534, #39793, #54752 ) ;
#70900=ORIENTED_EDGE ( 'NONE', *, *, #43175, .F. ) ;
#70901=DIRECTION ( 'NONE',  ( -3.999999999999999995E-14, 1.000000000000000000, -4.100000000000000342E-29 ) ) ;
#70903=VECTOR ( 'NONE', #8240, 1000.000000000000000 ) ;
#70904=LINE ( 'NONE', #21858, #82927 ) ;
#70906=CIRCLE ( 'NONE', #31707, 1.000000000000000888 ) ;
#70907=CARTESIAN_POINT ( 'NONE',  ( 117.6177984774595870, -42.17956309877360610, 93.44705384733897802 ) ) ;
#70909=LINE ( 'NONE', #16386, #40519 ) ;
#70910=DIRECTION ( 'NONE',  ( 1.000000000000000078E-15, -1.000000000000000083E-30, -1.000000000000000000 ) ) ;
#70912=EDGE_LOOP ( 'NONE', ( #60304, #32771, #19197, #82948, #7906 ) ) ;
#70914=CARTESIAN_POINT ( 'NONE',  ( 107.2978958415778123, -24.20855449189627251, 322.4523926293242653 ) ) ;
#70916=DIRECTION ( 'NONE',  ( -0.7071067811865165975, -0.7071067811865784369, -7.071067811865158803E-16 ) ) ;
#70917=CARTESIAN_POINT ( 'NONE',  ( 102.2923668651898339, -27.39740514546159389, 116.4527681330539650 ) ) ;
#70920=CARTESIAN_POINT ( 'NONE',  ( 116.3212776292296127, -32.94146857471318413, 287.6356252759109680 ) ) ;
#70923=B_SPLINE_CURVE_WITH_KNOTS ( 'NONE', 3,
 ( #5569, #68240, #55014, #60964, #26003, #81878, #82780, #19628, #46419, #74153, #5111, #20541, #6022, #61402, #88692, #4662, #26448, #26890 ),
 .UNSPECIFIED., .F., .F.,
 ( 4, 2, 2, 2, 2, 2, 2, 2, 4 ),
 ( 0.5000000005383744561, 0.5625000004710776214, 0.6250000004037807866, 0.6875000003364840628, 0.7500000002691872281, 0.8125000002018903933, 0.8750000001345936695, 0.9375000000672968348, 1.000000000000000000 ),
 .UNSPECIFIED. ) ;
#70925=EDGE_CURVE ( 'NONE', #26742, #44745, #10615, .T. ) ;
#70926=CARTESIAN_POINT ( 'NONE',  ( 167.2371591254544967, -47.82818131005522133, 180.4678068554150059 ) ) ;
#70927=EDGE_CURVE ( 'NONE', #11510, #56608, #17440, .T. ) ;
#70928=CARTESIAN_POINT ( 'NONE',  ( 98.56701561008813428, -30.78824967682752245, 156.8289586092439549 ) ) ;
#70929=VECTOR ( 'NONE', #814, 1000.000000000000000 ) ;
#70930=LINE ( 'NONE', #65868, #85007 ) ;
#70933=CARTESIAN_POINT ( 'NONE',  ( 117.4022237771661281, -37.57280582802024327, 34.77372051400595865 ) ) ;
#70934=CARTESIAN_POINT ( 'NONE',  ( 31.71315051185499811, -33.70561438052111214, -5.074374724088000832 ) ) ;
#70935=CARTESIAN_POINT ( 'NONE',  ( 142.8698897858160706, -0.9167816978817300289, 540.9756252759101471 ) ) ;
#70937=DIRECTION ( 'NONE',  ( -1.000000000000000078E-15, 1.000000000000000083E-30, 1.000000000000000000 ) ) ;
#70940=CARTESIAN_POINT ( 'NONE',  ( 115.3120223323506792, -44.18753462406608179, 233.2413395616259493 ) ) ;
#70941=ORIENTED_EDGE ( 'NONE', *, *, #10355, .T. ) ;
#70942=VERTEX_POINT ( 'NONE', #18774 ) ;
#70943=CIRCLE ( 'NONE', #65090, 2.029999999999997140 ) ;
#70944=CARTESIAN_POINT ( 'NONE',  ( 104.2961655698287302, -28.31198801876947613, 161.7615833058969486 ) ) ;
#70947=CARTESIAN_POINT ( 'NONE',  ( 104.0154917791352744, -27.12933488216606648, 51.75301187732594599 ) ) ;
#70949=EDGE_CURVE ( 'NONE', #74767, #6162, #13310, .T. ) ;
#70950=CARTESIAN_POINT ( 'NONE',  ( 142.8679068202682458, 10.65431904611001634, 542.9756252759101471 ) ) ;
#70952=CYLINDRICAL_SURFACE ( 'NONE', #21785, 2.517500000000005844 ) ;
#70953=DIRECTION ( 'NONE',  ( 1.387778780781444413E-14, -1.000000000000000000, 0.000000000000000000 ) ) ;
#70954=CARTESIAN_POINT ( 'NONE',  ( 96.93559702949573875, -34.21358363697170546, 276.1327681330537871 ) ) ;
#70957=ORIENTED_EDGE ( 'NONE', *, *, #40466, .T. ) ;
#70958=ADVANCED_FACE ( 'NONE', ( #89617 ), #18751, .F. ) ;
#70960=CARTESIAN_POINT ( 'NONE',  ( 123.6837132603321692, -53.34645651782491882, 249.5838068554164693 ) ) ;
#70962=CARTESIAN_POINT ( 'NONE',  ( 51.06648329127400388, 22.62155284005901024, 333.4006252759110112 ) ) ;
#70963=DIRECTION ( 'NONE',  ( 1.000000000000000078E-15, -1.000000000000000083E-30, -1.000000000000000000 ) ) ;
#70964=CARTESIAN_POINT ( 'NONE',  ( 117.5198883501232103, -40.51604253736888950, 19.54991099019698453 ) ) ;
#70966=LINE ( 'NONE', #76870, #62975 ) ;
#70967=VECTOR ( 'NONE', #41317, 1000.000000000000000 ) ;
#70968=ORIENTED_EDGE ( 'NONE', *, *, #70312, .F. ) ;
#70969=CARTESIAN_POINT ( 'NONE',  ( 168.5667039024480687, -48.82844715993497431, 300.4678068554149490 ) ) ;
#70970=DIRECTION ( 'NONE',  ( -1.000000000000000000, 0.000000000000000000, 0.000000000000000000 ) ) ;
#70971=CARTESIAN_POINT ( 'NONE',  ( 104.3243669996922307, -26.02151151870134171, 245.2880062282919482 ) ) ;
#70972=ORIENTED_EDGE ( 'NONE', *, *, #61563, .T. ) ;
#70975=CARTESIAN_POINT ( 'NONE',  ( 104.4085690792836942, -46.45823401906362449, 18.36525018442977952 ) ) ;
#70976=CARTESIAN_POINT ( 'NONE',  ( 116.3348466390194460, -36.28970630669515174, 116.6823760838769601 ) ) ;
#70977=CARTESIAN_POINT ( 'NONE',  ( 107.2435369062854420, -47.21027956138831883, 208.5899109901969837 ) ) ;
#70978=CARTESIAN_POINT ( 'NONE',  ( 83.06670390244796920, -64.87844715994098976, 201.9838068554149970 ) ) ;
#70979=EDGE_LOOP ( 'NONE', ( #76733, #53627 ) ) ;
#70980=VECTOR ( 'NONE', #50993, 1000.000000000000000 ) ;
#70982=FACE_OUTER_BOUND ( 'NONE', #15335, .T. ) ;
#70984=ORIENTED_EDGE ( 'NONE', *, *, #27242, .F. ) ;
#70985=CARTESIAN_POINT ( 'NONE',  ( 161.4809174648183614, -49.32844715993547879, 300.4678068554149490 ) ) ;
#70986=ORIENTED_EDGE ( 'NONE', *, *, #86417, .F. ) ;
#70987=ORIENTED_EDGE ( 'NONE', *, *, #84900, .F. ) ;
#70989=CARTESIAN_POINT ( 'NONE',  ( 113.2433028214677790, -28.75699364625837262, 24.55250987863361090 ) ) ;
#70991=CARTESIAN_POINT ( 'NONE',  ( 103.1716831446340166, -28.55367798840643090, 139.8648007804579549 ) ) ;
#70992=CARTESIAN_POINT ( 'NONE',  ( 112.5009111935468411, -46.38151608383146396, 257.9965776568635647 ) ) ;
#70993=CARTESIAN_POINT ( 'NONE',  ( 182.5667039024479550, -33.35206098992156143, 117.4678068554150627 ) ) ;
#70995=EDGE_CURVE ( 'NONE', #60117, #39460, #19227, .T. ) ;
#70998=CARTESIAN_POINT ( 'NONE',  ( 182.2420472961719895, -31.76306994223730840, 342.9256252759119548 ) ) ;
#70999=CARTESIAN_POINT ( 'NONE',  ( 41.56648329127399677, -9.303447159940999356, 18.92562527591200094 ) ) ;
#71000=VECTOR ( 'NONE', #1111, 1000.000000000000000 ) ;
#71001=EDGE_CURVE ( 'NONE', #89295, #70165, #19668, .T. ) ;
#71002=CARTESIAN_POINT ( 'NONE',  ( 96.65525155030036331, -37.83077348759547220, 126.4099109901969626 ) ) ;
#71003=CARTESIAN_POINT ( 'NONE',  ( 162.7131505118682639, -31.94127993907177299, 313.9678068554149490 ) ) ;
#71004=ORIENTED_EDGE ( 'NONE', *, *, #18951, .F. ) ;
#71005=CARTESIAN_POINT ( 'NONE',  ( 116.5366478410923463, -42.42989196264584706, 278.3832443235298797 ) ) ;
#71008=LINE ( 'NONE', #62821, #82793 ) ;
#71009=CARTESIAN_POINT ( 'NONE',  ( 80.06648329127399677, -8.729447159940999512, 7.443125275912000127 ) ) ;
#71011=DIRECTION ( 'NONE',  ( 0.7071067811566161820, 0.7071067812164789634, 0.000000000000000000 ) ) ;
#71016=FACE_OUTER_BOUND ( 'NONE', #5351, .T. ) ;
#71017=CARTESIAN_POINT ( 'NONE',  ( 107.0664832912739257, -52.57944715994094764, 302.7856252759109452 ) ) ;
#71021=LINE ( 'NONE', #14258, #8968 ) ;
#71022=CARTESIAN_POINT ( 'NONE',  ( 117.3567523603254159, -34.92480690411444044, 243.9641967044819637 ) ) ;
#71023=CARTESIAN_POINT ( 'NONE',  ( 116.8065287754011337, -43.47971597432173496, 159.3441967044829539 ) ) ;
#71024=CARTESIAN_POINT ( 'NONE',  ( 113.7840377202001036, -29.05235663984046823, 285.5032443235299979 ) ) ;
#71026=CARTESIAN_POINT ( 'NONE',  ( 104.4081006642920215, -46.45808914093545638, 47.36479194283237604 ) ) ;
#71027=CARTESIAN_POINT ( 'NONE',  ( 112.0658486739693274, -45.48843317147805720, 138.9897862770318113 ) ) ;
#71028=CIRCLE ( 'NONE', #59385, 3.250000000000002665 ) ;
#71029=AXIS2_PLACEMENT_3D ( 'NONE', #88287, #60087, #25586 ) ;
#71030=VERTEX_POINT ( 'NONE', #33300 ) ;
#71035=CARTESIAN_POINT ( 'NONE',  ( 101.2834890806669677, -28.93024170975123255, 185.0067055423629938 ) ) ;
#71036=VECTOR ( 'NONE', #45126, 1000.000000000000000 ) ;
#71039=DIRECTION ( 'NONE',  ( 0.000000000000000000, 0.000000000000000000, -1.000000000000000000 ) ) ;
#71040=ADVANCED_FACE ( 'NONE', ( #26933 ), #54601, .F. ) ;
#71041=CARTESIAN_POINT ( 'NONE',  ( 113.7366723824214318, -44.71300795807891149, 189.1299109901969757 ) ) ;
#71045=LINE ( 'NONE', #43300, #64602 ) ;
#71046=CARTESIAN_POINT ( 'NONE',  ( 110.9271686604937202, -27.50474214131384443, 85.76118691643459613 ) ) ;
#71050=AXIS2_PLACEMENT_3D ( 'NONE', #38113, #2715, #30411 ) ;
#71051=CARTESIAN_POINT ( 'NONE',  ( 112.7054497023526807, -28.73785826246136921, 129.5870538473399449 ) ) ;
#71054=CARTESIAN_POINT ( 'NONE',  ( 113.9863769398668296, -43.08488557356476889, 74.65491663922996679 ) ) ;
#71055=FACE_OUTER_BOUND ( 'NONE', #48398, .T. ) ;
#71057=CARTESIAN_POINT ( 'NONE',  ( 103.7602102885707467, -27.48919103108776341, 186.3499109901959798 ) ) ;
#71059=CARTESIAN_POINT ( 'NONE',  ( 100.9551113561145286, -28.70668612591127200, 55.59250746033355739 ) ) ;
#71060=CARTESIAN_POINT ( 'NONE',  ( 104.4899445637129674, -26.97881004783198122, 111.2818017522332781 ) ) ;
#71061=EDGE_CURVE ( 'NONE', #62271, #77006, #21469, .T. ) ;
#71066=CARTESIAN_POINT ( 'NONE',  ( 117.3423061886548879, -38.35306328171704848, 113.7013395616249767 ) ) ;
#71069=ORIENTED_EDGE ( 'NONE', *, *, #48300, .F. ) ;
#71072=CARTESIAN_POINT ( 'NONE',  ( 97.53195389500311308, -39.74930131913054510, 131.5705599381032584 ) ) ;
#71073=CARTESIAN_POINT ( 'NONE',  ( 112.0656190437874784, -45.48856781368362334, 103.9897653055920870 ) ) ;
#71074=CARTESIAN_POINT ( 'NONE',  ( 113.9479352111735295, -42.95371825284467349, 231.0595189410199453 ) ) ;
#71075=CIRCLE ( 'NONE', #34738, 2.517499999999998739 ) ;
#71077=CARTESIAN_POINT ( 'NONE',  ( 95.31140346374353101, -38.27925045402978554, 151.4299109901969871 ) ) ;
#71078=CARTESIAN_POINT ( 'NONE',  ( 62.03715912545828814, -47.82818131006021645, 249.9678068554150343 ) ) ;
#71079=ORIENTED_EDGE ( 'NONE', *, *, #16201, .F. ) ;
#71082=VECTOR ( 'NONE', #58296, 1000.000000000000000 ) ;
#71083=DIRECTION ( 'NONE',  ( -1.000000000000000078E-15, 0.000000000000000000, 1.000000000000000000 ) ) ;
#71084=ORIENTED_EDGE ( 'NONE', *, *, #13395, .F. ) ;
#71086=CARTESIAN_POINT ( 'NONE',  ( 78.16547420788155875, -20.71744337671388436, 7.623533105446029801 ) ) ;
#71087=DIRECTION ( 'NONE',  ( 8.755702086949183871E-16, 1.000000000000000000, 0.000000000000000000 ) ) ;
#71088=CARTESIAN_POINT ( 'NONE',  ( 111.5476492967639359, -29.48535330821865941, 286.0672975916113501 ) ) ;
#71089=AXIS2_PLACEMENT_3D ( 'NONE', #39708, #68778, #82871 ) ;
#71092=EDGE_CURVE ( 'NONE', #37008, #80917, #15557, .T. ) ;
#71093=CARTESIAN_POINT ( 'NONE',  ( 116.4917448565859104, -39.22821409912334190, 9.635625275910937759 ) ) ;
#71094=CARTESIAN_POINT ( 'NONE',  ( 165.9667039024459996, -26.71338133339301635, 117.4678068554150485 ) ) ;
#71095=ORIENTED_EDGE ( 'NONE', *, *, #57983, .T. ) ;
#71097=ORIENTED_EDGE ( 'NONE', *, *, #67191, .T. ) ;
#71098=CARTESIAN_POINT ( 'NONE',  ( 117.0877018078255389, -37.67114210324087509, 113.7515134788750970 ) ) ;
#71101=EDGE_CURVE ( 'NONE', #26573, #81352, #57919, .T. ) ;
#71102=CARTESIAN_POINT ( 'NONE',  ( 114.2324904129858112, -40.69568343359240714, 261.2423760838772182 ) ) ;
#71103=VECTOR ( 'NONE', #83703, 1000.000000000000000 ) ;
#71104=CARTESIAN_POINT ( 'NONE',  ( 109.4503794976336764, -25.91221646008812840, 179.8918157521019339 ) ) ;
#71105=CARTESIAN_POINT ( 'NONE',  ( 96.03721982003239077, -36.58408020053186505, 156.3280062282919687 ) ) ;
#71106=CARTESIAN_POINT ( 'NONE',  ( 103.8197751496740011, -48.12653019911325458, 213.3556252759109668 ) ) ;
#71108=CARTESIAN_POINT ( 'NONE',  ( 75.31670390244798341, -67.87844715994100397, 58.80080685541479824 ) ) ;
#71109=ORIENTED_EDGE ( 'NONE', *, *, #63218, .F. ) ;
#71113=CIRCLE ( 'NONE', #45003, 0.2999999999999943823 ) ;
#71115=CARTESIAN_POINT ( 'NONE',  ( 110.5134301196510620, -26.84384026877932072, 209.8099109901969541 ) ) ;
#71116=ORIENTED_EDGE ( 'NONE', *, *, #70299, .T. ) ;
#71117=CARTESIAN_POINT ( 'NONE',  ( 99.42196222650996162, -27.67359991961172128, 150.6356252759109680 ) ) ;
#71119=CARTESIAN_POINT ( 'NONE',  ( 29.56648329127400388, 15.62155284005900491, 323.8756252759109202 ) ) ;
#71121=CARTESIAN_POINT ( 'NONE',  ( 165.6738106836211557, -26.00627455218794637, 237.4678068554150059 ) ) ;
#71122=CARTESIAN_POINT ( 'NONE',  ( 116.3173461584868278, -32.93718857426866720, 59.13562527591098217 ) ) ;
#71123=CARTESIAN_POINT ( 'NONE',  ( 99.41296134609930846, -28.78668791560525975, 261.6746728949588032 ) ) ;
#71124=DIRECTION ( 'NONE',  ( 0.7071067811865165975, 0.7071067811865784369, 7.071067811865470403E-16 ) ) ;
#71126=VECTOR ( 'NONE', #74231, 1000.000000000000114 ) ;
#71128=DIRECTION ( 'NONE',  ( 5.512527431108029424E-15, -1.000000000000000000, 0.000000000000000000 ) ) ;
#71129=CARTESIAN_POINT ( 'NONE',  ( 116.3136297247243078, -32.94478793390952376, 255.1356252759109395 ) ) ;
#71130=FACE_OUTER_BOUND ( 'NONE', #13977, .T. ) ;
#71131=CARTESIAN_POINT ( 'NONE',  ( 115.4962543148458423, -35.12635383809098499, 195.5838068554167535 ) ) ;
#71134=CARTESIAN_POINT ( 'NONE',  ( 117.4794452684060104, -40.50643855513092007, 173.5375300378159693 ) ) ;
#71135=CARTESIAN_POINT ( 'NONE',  ( 114.3531094850664260, -44.18515411228707279, 69.19276813305397411 ) ) ;
#71136=CARTESIAN_POINT ( 'NONE',  ( 103.7092163704185026, -26.14992651007402813, 201.3089586092439731 ) ) ;
#71138=CYLINDRICAL_SURFACE ( 'NONE', #56179, 1.000000000000000888 ) ;
#71139=CIRCLE ( 'NONE', #44970, 0.5000000000000004441 ) ;
#71140=FACE_OUTER_BOUND ( 'NONE', #62532, .T. ) ;
#71143=CARTESIAN_POINT ( 'NONE',  ( 69.68306499799194853, -72.55732494037970071, 540.9756252759101471 ) ) ;
#71145=LINE ( 'NONE', #27995, #48458 ) ;
#71146=ORIENTED_EDGE ( 'NONE', *, *, #65095, .F. ) ;
#71147=VERTEX_POINT ( 'NONE', #42774 ) ;
#71148=EDGE_CURVE ( 'NONE', #84501, #67129, #8288, .T. ) ;
#71150=LINE ( 'NONE', #19962, #13981 ) ;
#71151=EDGE_LOOP ( 'NONE', ( #52375, #80650, #80243, #40338 ) ) ;
#71153=CARTESIAN_POINT ( 'NONE',  ( 96.66376384204026806, -36.61947630124858932, 107.3184824187679567 ) ) ;
#71154=CYLINDRICAL_SURFACE ( 'NONE', #81683, 2.517500000000005844 ) ;
#71155=ADVANCED_FACE ( 'NONE', ( #35984 ), #14658, .T. ) ;
#71157=DIRECTION ( 'NONE',  ( 0.4214249218767882055, 0.9068632946707806397, 4.214249218767890910E-16 ) ) ;
#71160=CARTESIAN_POINT ( 'NONE',  ( 102.1671273105904447, -43.72604531649727733, 281.5124198280768155 ) ) ;
#71162=ORIENTED_EDGE ( 'NONE', *, *, #74070, .F. ) ;
#71163=CIRCLE ( 'NONE', #10257, 10.00000000000002665 ) ;
#71165=CARTESIAN_POINT ( 'NONE',  ( 105.7154773345749135, -46.72385839275415265, 107.4689586095794738 ) ) ;
#71166=FACE_OUTER_BOUND ( 'NONE', #44088, .T. ) ;
#71167=CYLINDRICAL_SURFACE ( 'NONE', #5667, 2.500000000000002220 ) ;
#71168=DIRECTION ( 'NONE',  ( 1.000000000000000078E-15, -1.000000000000000083E-30, -1.000000000000000000 ) ) ;
#71169=LINE ( 'NONE', #28929, #30192 ) ;
#71170=CARTESIAN_POINT ( 'NONE',  ( 97.39127856926108961, -39.27846915049015308, 52.53132659260805326 ) ) ;
#71175=EDGE_CURVE ( 'NONE', #37060, #72283, #84344, .T. ) ;
#71176=CARTESIAN_POINT ( 'NONE',  ( 97.82554479137630210, -33.52525840161893456, 286.0613395616258572 ) ) ;
#71177=EDGE_LOOP ( 'NONE', ( #57542, #4630, #68397, #50892, #62730, #62891, #51266, #50728, #86544 ) ) ;
#71180=CARTESIAN_POINT ( 'NONE',  ( 103.5819438468105744, -44.65149928713079674, 130.0528522743539668 ) ) ;
#71183=CYLINDRICAL_SURFACE ( 'NONE', #3906, 0.5000000000000197620 ) ;
#71184=ORIENTED_EDGE ( 'NONE', *, *, #79800, .T. ) ;
#71185=ORIENTED_EDGE ( 'NONE', *, *, #72502, .F. ) ;
#71186=CARTESIAN_POINT ( 'NONE',  ( 105.7156386614864658, -46.72388412106460720, 137.4669372650166679 ) ) ;
#71187=VECTOR ( 'NONE', #12472, 1000.000000000000000 ) ;
#71189=ORIENTED_EDGE ( 'NONE', *, *, #54497, .T. ) ;
#71190=CARTESIAN_POINT ( 'NONE',  ( 117.1402439185659006, -36.89830975172036887, 150.2444404487539487 ) ) ;
#71191=DIRECTION ( 'NONE',  ( -0.7071067811734105257, 0.7071067811996846197, 0.000000000000000000 ) ) ;
#71192=CARTESIAN_POINT ( 'NONE',  ( 114.5831001172654595, -44.03558617456690172, 94.21276813305395592 ) ) ;
#71193=ADVANCED_FACE ( 'NONE', ( #73630 ), #86379, .T. ) ;
#71194=CARTESIAN_POINT ( 'NONE',  ( 110.8549378340421470, -45.98404676291230686, 17.88566530162140467 ) ) ;
#71197=EDGE_LOOP ( 'NONE', ( #8598, #72487, #74042, #85499 ) ) ;
#71199=CARTESIAN_POINT ( 'NONE',  ( 108.4620505914581798, -44.77196653648033475, 165.5309475124489609 ) ) ;
#71200=CARTESIAN_POINT ( 'NONE',  ( 107.8700610081582738, -26.31308374369285730, 70.01562527591099183 ) ) ;
#71202=CARTESIAN_POINT ( 'NONE',  ( 115.4270991047691410, -42.97960947038953350, 28.31562527591097123 ) ) ;
#71203=CARTESIAN_POINT ( 'NONE',  ( 114.1394676070193839, -29.04113448922185370, 195.4841967044819739 ) ) ;
#71204=DIRECTION ( 'NONE',  ( 1.000000000000000078E-15, -1.000000000000000083E-30, -1.000000000000000000 ) ) ;
#71206=CARTESIAN_POINT ( 'NONE',  ( 98.45631125714150755, -42.66967193002393088, 122.8070538473389490 ) ) ;
#71207=AXIS2_PLACEMENT_3D ( 'NONE', #3448, #31584, #86575 ) ;
#71209=VERTEX_POINT ( 'NONE', #24155 ) ;
#71210=DIRECTION ( 'NONE',  ( -1.907762142705490052E-15, -7.167082501179359715E-16, 1.000000000000000000 ) ) ;
#71211=CIRCLE ( 'NONE', #87149, 1.000000000000000888 ) ;
#71212=CIRCLE ( 'NONE', #82820, 0.5000000000000004441 ) ;
#71214=CARTESIAN_POINT ( 'NONE',  ( 97.81930656603341845, -40.53598742125645060, 132.6376059489711849 ) ) ;
#71216=ORIENTED_EDGE ( 'NONE', *, *, #69265, .F. ) ;
#71217=AXIS2_PLACEMENT_3D ( 'NONE', #52191, #4526, #79954 ) ;
#71219=EDGE_CURVE ( 'NONE', #39785, #32919, #53867, .T. ) ;
#71220=CARTESIAN_POINT ( 'NONE',  ( 116.3212776292296127, -32.94146857471318413, 287.6356252759109680 ) ) ;
#71221=CARTESIAN_POINT ( 'NONE',  ( 118.0757533234433083, -37.71689883586016379, 33.74324432352998571 ) ) ;
#71223=CARTESIAN_POINT ( 'NONE',  ( 97.81170986510684884, -40.51745644794008427, 172.6354259520616097 ) ) ;
#71224=DIRECTION ( 'NONE',  ( 1.000000000000000000, 1.199348956600846523E-15, 0.000000000000000000 ) ) ;
#71225=CARTESIAN_POINT ( 'NONE',  ( 115.0831197249980420, -29.02584261466826021, 39.43562527591099354 ) ) ;
#71226=CARTESIAN_POINT ( 'NONE',  ( 97.81002727075654946, -40.51336424107649492, 111.6352756744173007 ) ) ;
#71227=CARTESIAN_POINT ( 'NONE',  ( 116.7861719071672155, -43.46560779248400763, 159.3441967044829539 ) ) ;
#71228=DIRECTION ( 'NONE',  ( -1.000000000000000000, -4.299999999999999979E-14, -1.000000000000000078E-15 ) ) ;
#71229=LINE ( 'NONE', #23090, #82965 ) ;
#71230=ORIENTED_EDGE ( 'NONE', *, *, #57696, .T. ) ;
#71231=B_SPLINE_CURVE_WITH_KNOTS ( 'NONE', 3,
 ( #70628, #36102, #43796, #7947, #9297, #51493, #1138, #17003, #22940, #77894, #36999, #86054, #2928, #16119, #64264, #56982, #42894, #2485 ),
 .UNSPECIFIED., .F., .F.,
 ( 4, 2, 2, 2, 2, 2, 2, 2, 4 ),
 ( 0.4999999768783345844, 0.5624999797685428238, 0.6249999826587508966, 0.6874999855489591916, 0.7499999884391672644, 0.8124999913293755593, 0.8749999942195836322, 0.9374999971097919271, 1.000000000000000000 ),
 .UNSPECIFIED. ) ;
#71233=CARTESIAN_POINT ( 'NONE',  ( 33.92127028473603900, -29.73316016639542170, 342.9256252759109884 ) ) ;
#71235=CARTESIAN_POINT ( 'NONE',  ( 100.1253875378072848, -39.57043109886186727, 0.4256252759109631079 ) ) ;
#71238=EDGE_CURVE ( 'NONE', #25358, #83795, #23286, .T. ) ;
#71239=CARTESIAN_POINT ( 'NONE',  ( 77.31648329127399677, -18.72944715994106346, 6.749768910606400496 ) ) ;
#71240=CARTESIAN_POINT ( 'NONE',  ( 117.4576385420935338, -35.45251388149282690, 193.9241967044829664 ) ) ;
#71241=ORIENTED_EDGE ( 'NONE', *, *, #51808, .F. ) ;
#71243=CARTESIAN_POINT ( 'NONE',  ( 118.0636334930051987, -35.40736804548507877, 234.9337205140059552 ) ) ;
#71244=CARTESIAN_POINT ( 'NONE',  ( 108.9932425643425802, -47.01927604342903777, 78.72419670448194040 ) ) ;
#71246=CARTESIAN_POINT ( 'NONE',  ( 97.31590013278544404, -39.30611206075547415, 192.5313402528328481 ) ) ;
#71249=ADVANCED_FACE ( 'NONE', ( #10076 ), #44120, .F. ) ;
#71250=ORIENTED_EDGE ( 'NONE', *, *, #32250, .F. ) ;
#71252=ORIENTED_EDGE ( 'NONE', *, *, #22738, .F. ) ;
#71255=CARTESIAN_POINT ( 'NONE',  ( 130.3998166246070127, 12.92155284005802685, 336.5756252759110225 ) ) ;
#71256=CARTESIAN_POINT ( 'NONE',  ( 96.77275252345162926, -34.86922145964237529, 237.1841967044819626 ) ) ;
#71258=CARTESIAN_POINT ( 'NONE',  ( 131.8592257737628586, -35.08568546291017043, 2.471387922376259816 ) ) ;
#71259=EDGE_CURVE ( 'NONE', #80300, #62557, #1324, .T. ) ;
#71260=CARTESIAN_POINT ( 'NONE',  ( 179.1667039024460166, -28.27351298637280408, -5.074374724088000832 ) ) ;
#71263=AXIS2_PLACEMENT_3D ( 'NONE', #58673, #3732, #32314 ) ;
#71264=CARTESIAN_POINT ( 'NONE',  ( 116.7906267970580103, -31.42506456344890964, 24.21181575210196257 ) ) ;
#71267=ORIENTED_EDGE ( 'NONE', *, *, #45425, .F. ) ;
#71268=VECTOR ( 'NONE', #3268, 1000.000000000000000 ) ;
#71271=CARTESIAN_POINT ( 'NONE',  ( 99.85651329999866732, -30.12038005271842422, 271.7356252759109907 ) ) ;
#71272=LINE ( 'NONE', #1322, #55962 ) ;
#71274=CARTESIAN_POINT ( 'NONE',  ( 107.9743429475490615, -26.39917242597376301, 105.9946728949579864 ) ) ;
#71276=CARTESIAN_POINT ( 'NONE',  ( 104.4076007111484614, -46.45794255853319754, 27.36475074168719601 ) ) ;
#71278=ORIENTED_EDGE ( 'NONE', *, *, #59034, .T. ) ;
#71283=CARTESIAN_POINT ( 'NONE',  ( 107.1674220045319288, -28.56736792770730560, 32.88523322673398042 ) ) ;
#71285=DIRECTION ( 'NONE',  ( 1.639958061481212836E-42, -4.100000000000000342E-29, -1.000000000000000000 ) ) ;
#71287=VECTOR ( 'NONE', #38574, 1000.000000000000000 ) ;
#71288=CARTESIAN_POINT ( 'NONE',  ( 51.06648329127400388, -8.350947159940998787, 333.4006252759120343 ) ) ;
#71290=CARTESIAN_POINT ( 'NONE',  ( 141.8164832912739826, -9.833000550534297446, 14.92562527591100618 ) ) ;
#71292=VERTEX_POINT ( 'NONE', #81371 ) ;
#71293=CARTESIAN_POINT ( 'NONE',  ( 117.1066318038510303, -39.53701698219273908, 98.60991099019594230 ) ) ;
#71294=ORIENTED_EDGE ( 'NONE', *, *, #10203, .T. ) ;
#71295=CARTESIAN_POINT ( 'NONE',  ( 115.2801527212906336, -32.91522314707135166, 58.58289601855292972 ) ) ;
#71298=CARTESIAN_POINT ( 'NONE',  ( 96.72778144249456034, -35.92320320382069099, 191.2765776568639922 ) ) ;
#71299=CARTESIAN_POINT ( 'NONE',  ( 142.8698897858160706, -0.9167816978817300289, 542.9756252759101471 ) ) ;
#71300=DIRECTION ( 'NONE',  ( -1.000000000000000000, -3.999999999999999995E-14, 4.193851878741028267E-47 ) ) ;
#71302=CARTESIAN_POINT ( 'NONE',  ( 151.0371591254582597, -46.82818131005593187, 300.4678068554149490 ) ) ;
#71303=CARTESIAN_POINT ( 'NONE',  ( 110.2908372810403819, -46.66631795110420455, 8.827053847339950465 ) ) ;
#71304=ORIENTED_EDGE ( 'NONE', *, *, #26906, .T. ) ;
#71306=ORIENTED_EDGE ( 'NONE', *, *, #68276, .T. ) ;
#71307=CARTESIAN_POINT ( 'NONE',  ( 117.7479605218750862, -39.74664297364158472, 139.6194347997199827 ) ) ;
#71308=DIRECTION ( 'NONE',  ( 0.000000000000000000, 0.000000000000000000, -1.000000000000000000 ) ) ;
#71313=CIRCLE ( 'NONE', #16203, 3.299999999999999822 ) ;
#71314=CARTESIAN_POINT ( 'NONE',  ( 107.0667039024467329, -53.45944715994091467, 195.5838068554169524 ) ) ;
#71315=DIRECTION ( 'NONE',  ( -2.900000000000000265E-14, 2.000000000000000155E-15, -1.000000000000000000 ) ) ;
#71317=DIRECTION ( 'NONE',  ( 1.907762142705490052E-15, 7.167082501179359715E-16, -1.000000000000000000 ) ) ;
#71318=FACE_OUTER_BOUND ( 'NONE', #79253, .T. ) ;
#71319=CARTESIAN_POINT ( 'NONE',  ( 104.2409529242390391, -46.76432966167102023, 18.35848241876792031 ) ) ;
#71322=DIRECTION ( 'NONE',  ( 0.000000000000000000, 0.000000000000000000, -1.000000000000000000 ) ) ;
#71323=DIRECTION ( 'NONE',  ( 9.351236661543306751E-17, -3.725950533538267725E-29, -1.000000000000000000 ) ) ;
#71324=VERTEX_POINT ( 'NONE', #54050 ) ;
#71330=EDGE_CURVE ( 'NONE', #5931, #83484, #49140, .T. ) ;
#71333=CARTESIAN_POINT ( 'NONE',  ( 99.66831329903114067, -43.01734891331329891, 226.3095626852189639 ) ) ;
#71334=FACE_OUTER_BOUND ( 'NONE', #60522, .T. ) ;
#71335=CARTESIAN_POINT ( 'NONE',  ( 100.4250012405661607, -28.72198927997979823, 36.62705384733894221 ) ) ;
#71336=LINE ( 'NONE', #58134, #45124 ) ;
#71337=CARTESIAN_POINT ( 'NONE',  ( 102.9537058647788967, -46.35710148923402585, 92.25562527591097250 ) ) ;
#71338=ORIENTED_EDGE ( 'NONE', *, *, #17352, .T. ) ;
#71339=CARTESIAN_POINT ( 'NONE',  ( 131.3333327974766576, -19.08363404519706208, 6.775960187534563417 ) ) ;
#71341=EDGE_CURVE ( 'NONE', #21246, #75279, #12934, .T. ) ;
#71342=CARTESIAN_POINT ( 'NONE',  ( 194.0667039024480118, -40.32844715993407902, 249.9678068554149775 ) ) ;
#71343=CARTESIAN_POINT ( 'NONE',  ( 25.56670390244797275, -58.35344715994099829, 257.2178068554150059 ) ) ;
#71344=VERTEX_POINT ( 'NONE', #25935 ) ;
#71345=EDGE_CURVE ( 'NONE', #57944, #83877, #60893, .T. ) ;
#71346=EDGE_CURVE ( 'NONE', #4781, #48555, #44806, .T. ) ;
#71347=CARTESIAN_POINT ( 'NONE',  ( 32.06670390244579494, -32.29483332968550258, 117.4678068554150485 ) ) ;
#71348=VERTEX_POINT ( 'NONE', #12306 ) ;
#71349=CARTESIAN_POINT ( 'NONE',  ( 107.0664832912739683, -18.82844715994099971, 199.5838068554169809 ) ) ;
#71350=DIRECTION ( 'NONE',  ( 1.000000000000000000, 4.299999999999999979E-14, 1.000000000000000078E-15 ) ) ;
#71351=AXIS2_PLACEMENT_3D ( 'NONE', #44617, #39046, #25873 ) ;
#71352=ADVANCED_FACE ( 'NONE', ( #13648 ), #32282, .F. ) ;
#71353=FACE_OUTER_BOUND ( 'NONE', #48171, .T. ) ;
#71354=EDGE_CURVE ( 'NONE', #54231, #38331, #53972, .T. ) ;
#71355=ORIENTED_EDGE ( 'NONE', *, *, #20372, .T. ) ;
#71356=CARTESIAN_POINT ( 'NONE',  ( 100.2843123851674960, -46.47809700006297362, 87.09276813305393716 ) ) ;
#71358=EDGE_CURVE ( 'NONE', #25435, #1233, #60435, .T. ) ;
#71359=CARTESIAN_POINT ( 'NONE',  ( 141.8164832912740394, -45.62589376934770513, -5.074374724088994704 ) ) ;
#71360=DIRECTION ( 'NONE',  ( 1.000000000000000078E-15, -1.000000000000000000, 0.000000000000000000 ) ) ;
#71361=CARTESIAN_POINT ( 'NONE',  ( 61.67078992371376245, -0.9290567490904538817, 542.9756252759101471 ) ) ;
#71363=AXIS2_PLACEMENT_3D ( 'NONE', #39474, #73998, #11777 ) ;
#71364=EDGE_CURVE ( 'NONE', #34865, #36283, #39553, .T. ) ;
#71366=CARTESIAN_POINT ( 'NONE',  ( 80.06648281188262217, -21.47944715903999224, 8.225259175037979986 ) ) ;
#71367=AXIS2_PLACEMENT_3D ( 'NONE', #40039, #87310, #13247 ) ;
#71370=CARTESIAN_POINT ( 'NONE',  ( 181.8764988495240118, -33.54226604284930602, 342.9256252759119548 ) ) ;
#71372=CARTESIAN_POINT ( 'NONE',  ( 41.56648329127399677, -18.82844715994099971, 318.9256252759120116 ) ) ;
#71373=VERTEX_POINT ( 'NONE', #77227 ) ;
#71375=CARTESIAN_POINT ( 'NONE',  ( 106.9806506443342755, -46.50983917909364607, 183.5699109901959787 ) ) ;
#71377=ORIENTED_EDGE ( 'NONE', *, *, #25991, .F. ) ;
#71379=CARTESIAN_POINT ( 'NONE',  ( 111.0600676159102278, -27.80113716328034457, 20.74133956162494030 ) ) ;
#71380=DIRECTION ( 'NONE',  ( 0.9834602067019598826, 0.1811243270069988198, 0.000000000000000000 ) ) ;
#71382=EDGE_CURVE ( 'NONE', #17509, #21135, #72391, .T. ) ;
#71383=CARTESIAN_POINT ( 'NONE',  ( 108.3314583620718849, -46.73508509281070644, 12.67747797925112963 ) ) ;
#71385=DIRECTION ( 'NONE',  ( 1.000000000000000078E-15, 0.000000000000000000, -1.000000000000000000 ) ) ;
#71386=EDGE_CURVE ( 'NONE', #1463, #231, #1371, .T. ) ;
#71387=CARTESIAN_POINT ( 'NONE',  ( 97.32398421004032230, -35.86507053846867166, 231.2556252759109725 ) ) ;
#71388=ORIENTED_EDGE ( 'NONE', *, *, #13480, .T. ) ;
#71389=CIRCLE ( 'NONE', #72795, 2.500000000000002220 ) ;
#71390=VERTEX_POINT ( 'NONE', #69962 ) ;
#71391=CARTESIAN_POINT ( 'NONE',  ( 99.72946911866242203, -30.86048229651775543, 192.2092023535159626 ) ) ;
#71393=DIRECTION ( 'NONE',  ( 0.000000000000000000, 0.000000000000000000, 1.000000000000000000 ) ) ;
#71394=CARTESIAN_POINT ( 'NONE',  ( 109.9481718979998277, -45.67217584368548700, 54.26824997256396443 ) ) ;
#71396=DIRECTION ( 'NONE',  ( -1.000000000000000078E-15, 1.000000000000000083E-30, 1.000000000000000000 ) ) ;
#71400=FACE_OUTER_BOUND ( 'NONE', #59309, .T. ) ;
#71401=CARTESIAN_POINT ( 'NONE',  ( 112.4005920293390233, -46.38403708128156921, 252.9661014663871583 ) ) ;
#71402=CYLINDRICAL_SURFACE ( 'NONE', #60510, 5.599999999999994316 ) ;
#71403=ORIENTED_EDGE ( 'NONE', *, *, #6345, .F. ) ;
#71405=VECTOR ( 'NONE', #15761, 1000.000000000000000 ) ;
#71406=CARTESIAN_POINT ( 'NONE',  ( 115.7831076680295723, -41.80230951391620664, 83.40645860891918062 ) ) ;
#71411=CARTESIAN_POINT ( 'NONE',  ( 107.1874307469290244, -26.94942635195924652, 31.06705384733893283 ) ) ;
#71412=DIRECTION ( 'NONE',  ( -2.127927463864879951E-15, 0.000000000000000000, -1.000000000000000000 ) ) ;
#71413=EDGE_LOOP ( 'NONE', ( #44325, #73818, #16278, #62686 ) ) ;
#71414=VECTOR ( 'NONE', #1719, 999.9999999999998863 ) ;
#71415=CARTESIAN_POINT ( 'NONE',  ( 118.1215414109737196, -37.72100569522838498, 29.74324432352998215 ) ) ;
#71416=CARTESIAN_POINT ( 'NONE',  ( 167.2371591254542693, -47.82818131005522844, 300.4678068554149490 ) ) ;
#71417=CARTESIAN_POINT ( 'NONE',  ( 100.5838780899822922, -28.49162262467549667, 15.60705384733995871 ) ) ;
#71419=CIRCLE ( 'NONE', #84528, 13.31747058675099993 ) ;
#71421=CARTESIAN_POINT ( 'NONE',  ( 142.8838050580813785, -82.11588141944044139, 394.9756252759102040 ) ) ;
#71424=CARTESIAN_POINT ( 'NONE',  ( 109.4870457054322941, -44.52499740455228761, 95.63380465530596553 ) ) ;
#71425=CARTESIAN_POINT ( 'NONE',  ( 112.2157656529268763, -45.81911987206276393, 208.9870538473389558 ) ) ;
#71428=DIRECTION ( 'NONE',  ( 4.299999999999999979E-14, -1.000000000000000000, 4.400000000000000367E-29 ) ) ;
#71435=DIRECTION ( 'NONE',  ( 0.7071067811989676377, 0.7071067811741275078, 7.071067811989670636E-16 ) ) ;
#71436=EDGE_CURVE ( 'NONE', #38972, #22588, #6279, .T. ) ;
#71438=DIRECTION ( 'NONE',  ( 1.000000000000000078E-15, -1.000000000000000083E-30, -1.000000000000000000 ) ) ;
#71439=CARTESIAN_POINT ( 'NONE',  ( 115.1410662219050067, -33.85660664540706222, 113.5209912566479744 ) ) ;
#71440=CARTESIAN_POINT ( 'NONE',  ( 96.95731234646120811, -39.36592712812080208, 276.5299109901967540 ) ) ;
#71441=EDGE_CURVE ( 'NONE', #80932, #72917, #82584, .T. ) ;
#71442=AXIS2_PLACEMENT_3D ( 'NONE', #86220, #58057, #2663 ) ;
#71443=CARTESIAN_POINT ( 'NONE',  ( 180.2143765759489895, -35.91149509761070391, -5.074374724088000832 ) ) ;
#71444=ORIENTED_EDGE ( 'NONE', *, *, #75330, .F. ) ;
#71446=ORIENTED_EDGE ( 'NONE', *, *, #70196, .T. ) ;
#71450=ADVANCED_FACE ( 'NONE', ( #56761 ), #50392, .F. ) ;
#71451=AXIS2_PLACEMENT_3D ( 'NONE', #70511, #82479, #19333 ) ;
#71452=CARTESIAN_POINT ( 'NONE',  ( 117.4075167370973958, -38.36336677748749224, 113.7013395616249767 ) ) ;
#71453=CARTESIAN_POINT ( 'NONE',  ( 182.4202572930407769, -33.70561438051400671, 237.4678068554150059 ) ) ;
#71454=ORIENTED_EDGE ( 'NONE', *, *, #60852, .T. ) ;
#71456=CARTESIAN_POINT ( 'NONE',  ( 106.2268934648462420, -47.75097955688366369, 267.5280062282920994 ) ) ;
#71457=CARTESIAN_POINT ( 'NONE',  ( 90.44969454456405344, -21.37118780205715396, 218.8274735512160589 ) ) ;
#71458=DIRECTION ( 'NONE',  ( 9.002638163713000033E-13, -1.000000000000000000, 4.100000000000000342E-29 ) ) ;
#71463=CARTESIAN_POINT ( 'NONE',  ( 57.56670390244744340, -48.82844715994040286, 173.2178068554150911 ) ) ;
#71464=CARTESIAN_POINT ( 'NONE',  ( 131.3164832912740110, -36.72944715994100306, 6.749768910606454675 ) ) ;
#71466=CARTESIAN_POINT ( 'NONE',  ( 97.31584373246833763, -39.30597606293734714, 12.53145861429736030 ) ) ;
#71467=CARTESIAN_POINT ( 'NONE',  ( 117.0609946685736276, -38.07974641096466684, 163.7188594754593964 ) ) ;
#71468=VECTOR ( 'NONE', #71518, 1000.000000000000000 ) ;
#71469=EDGE_CURVE ( 'NONE', #53210, #37453, #84509, .T. ) ;
#71470=DIRECTION ( 'NONE',  ( -0.9963424814100680926, 0.08544974978095698503, 0.000000000000000000 ) ) ;
#71472=CARTESIAN_POINT ( 'NONE',  ( 116.1589316287842735, -31.54115767207924748, 289.2384824187681716 ) ) ;
#71473=CARTESIAN_POINT ( 'NONE',  ( 102.9671325615611437, -26.46449201736525225, 171.3908633711489813 ) ) ;
#71474=CARTESIAN_POINT ( 'NONE',  ( 118.2318068709390815, -40.77392476355825579, 19.54991099019698453 ) ) ;
#71476=CARTESIAN_POINT ( 'NONE',  ( 82.60054997757750073, -35.66120003907148117, 7.039521718173837428 ) ) ;
#71477=CARTESIAN_POINT ( 'NONE',  ( 82.41744075320353602, -35.29868422066351030, 2.608896314039987452 ) ) ;
#71479=AXIS2_PLACEMENT_3D ( 'NONE', #89196, #41905, #1040 ) ;
#71480=VERTEX_POINT ( 'NONE', #8639 ) ;
#71481=DIRECTION ( 'NONE',  ( 4.299999999999999979E-14, -1.000000000000000000, 0.000000000000000000 ) ) ;
#71484=CARTESIAN_POINT ( 'NONE',  ( 100.7170190823677132, -45.85612711270987774, 83.09276813305294240 ) ) ;
#71487=CARTESIAN_POINT ( 'NONE',  ( 117.0607673848196839, -38.08134988825185729, 49.71888720434603215 ) ) ;
#71488=CARTESIAN_POINT ( 'NONE',  ( 117.9098725419244005, -34.70837513311213485, 199.9851490854349549 ) ) ;
#71489=CARTESIAN_POINT ( 'NONE',  ( 126.8897065959774295, -54.55267237199291230, 14.92562527591099020 ) ) ;
#71490=DIRECTION ( 'NONE',  ( 0.000000000000000000, 1.000000000000000000, 1.541976423090495239E-15 ) ) ;
#71491=CARTESIAN_POINT ( 'NONE',  ( 107.0664832912739968, -36.72944715994100306, 277.6356252759110248 ) ) ;
#71492=CARTESIAN_POINT ( 'NONE',  ( 114.4222700328740245, -29.92353839607118715, 85.42008522968446016 ) ) ;
#71495=DIRECTION ( 'NONE',  ( 0.000000000000000000, 0.000000000000000000, -1.000000000000000000 ) ) ;
#71497=CARTESIAN_POINT ( 'NONE',  ( 114.0519814166327563, -29.87813257090970609, 149.4441967044829767 ) ) ;
#71498=EDGE_LOOP ( 'NONE', ( #48787, #80671, #9926, #86165 ) ) ;
#71499=ORIENTED_EDGE ( 'NONE', *, *, #55856, .T. ) ;
#71500=CARTESIAN_POINT ( 'NONE',  ( 103.8469135698534416, -45.55616208374542708, 93.71777378208700782 ) ) ;
#71501=FACE_OUTER_BOUND ( 'NONE', #80702, .T. ) ;
#71502=CARTESIAN_POINT ( 'NONE',  ( 109.1965444620390286, -27.18343884754229833, 220.9013395616249795 ) ) ;
#71504=DIRECTION ( 'NONE',  ( 1.000000000000000000, 2.999999999999999839E-15, 1.000000000000000078E-15 ) ) ;
#71505=CARTESIAN_POINT ( 'NONE',  ( 108.4174825185799733, -26.73503487134302503, 110.9692457430530652 ) ) ;
#71506=FACE_OUTER_BOUND ( 'NONE', #80123, .T. ) ;
#71507=CIRCLE ( 'NONE', #88933, 2.749999999999974687 ) ;
#71509=CARTESIAN_POINT ( 'NONE',  ( 46.83715912545337545, -47.82818131006086304, 193.9678068554150911 ) ) ;
#71510=CARTESIAN_POINT ( 'NONE',  ( 98.87380182923577365, -30.31772012733808808, 155.7984824187679465 ) ) ;
#71511=ORIENTED_EDGE ( 'NONE', *, *, #70409, .F. ) ;
#71513=EDGE_LOOP ( 'NONE', ( #83001, #10016, #15238, #50875 ) ) ;
#71514=ADVANCED_FACE ( 'NONE', ( #58111 ), #78587, .F. ) ;
#71517=CARTESIAN_POINT ( 'NONE',  ( 97.39142042132525035, -39.27900364432255742, 131.5314998150807639 ) ) ;
#71518=DIRECTION ( 'NONE',  ( 0.000000000000000000, 1.000000000000000000, 0.000000000000000000 ) ) ;
#71519=CARTESIAN_POINT ( 'NONE',  ( 99.99635294717694478, -42.73853927783394369, 224.7052332267339807 ) ) ;
#71521=EDGE_CURVE ( 'NONE', #31761, #30540, #37225, .T. ) ;
#71522=CARTESIAN_POINT ( 'NONE',  ( 116.7951241094207830, -39.38783451605569752, 269.6147915599842122 ) ) ;
#71523=CARTESIAN_POINT ( 'NONE',  ( 117.4874684240972300, -40.41484487456647656, 178.5680062282919778 ) ) ;
#71526=ORIENTED_EDGE ( 'NONE', *, *, #51904, .T. ) ;
#71530=VERTEX_POINT ( 'NONE', #64930 ) ;
#71531=CYLINDRICAL_SURFACE ( 'NONE', #30427, 3.000000000000002665 ) ;
#71533=CARTESIAN_POINT ( 'NONE',  ( 104.9598549460505126, -28.12176414095025834, 281.6987261630399644 ) ) ;
#71536=CARTESIAN_POINT ( 'NONE',  ( 107.5239001228424058, -44.99862095125077133, 9.635625275910943088 ) ) ;
#71538=ORIENTED_EDGE ( 'NONE', *, *, #40949, .F. ) ;
#71539=EDGE_LOOP ( 'NONE', ( #53379, #16916, #66273, #45009 ) ) ;
#71541=CARTESIAN_POINT ( 'NONE',  ( 98.04155473296256673, -41.04193254465488394, 111.6812086568694440 ) ) ;
#71542=ORIENTED_EDGE ( 'NONE', *, *, #59303, .T. ) ;
#71543=VERTEX_POINT ( 'NONE', #24052 ) ;
#71544=AXIS2_PLACEMENT_3D ( 'NONE', #72321, #88195, #80936 ) ;
#71545=ADVANCED_FACE ( 'NONE', ( #23180 ), #17234, .T. ) ;
#71546=EDGE_CURVE ( 'NONE', #52594, #11728, #51273, .T. ) ;
#71547=AXIS2_PLACEMENT_3D ( 'NONE', #79616, #10995, #17816 ) ;
#71548=CARTESIAN_POINT ( 'NONE',  ( 116.0863591824327443, -37.53846460971577415, 33.16575316141096152 ) ) ;
#71549=CARTESIAN_POINT ( 'NONE',  ( 102.8350101556302434, -46.28146260531957523, 177.2441967044819648 ) ) ;
#71550=EDGE_CURVE ( 'NONE', #87063, #70690, #71755, .T. ) ;
#71551=CARTESIAN_POINT ( 'NONE',  ( 104.9672558511365992, -25.09151557957600076, 125.2184824187689856 ) ) ;
#71552=CARTESIAN_POINT ( 'NONE',  ( 96.13817600250692408, -35.07231702426307152, 217.1946728949589840 ) ) ;
#71553=CARTESIAN_POINT ( 'NONE',  ( 115.7832353055570280, -41.80209406143853812, 99.40770611954226865 ) ) ;
#71557=EDGE_CURVE ( 'NONE', #71147, #70860, #29969, .T. ) ;
#71560=CARTESIAN_POINT ( 'NONE',  ( 114.9985205141181837, -29.89647917087096118, 184.3927681330539770 ) ) ;
#71561=ORIENTED_EDGE ( 'NONE', *, *, #49361, .F. ) ;
#71562=CARTESIAN_POINT ( 'NONE',  ( 108.3661291232776023, -47.70624136733754028, 162.6822919425769669 ) ) ;
#71563=LINE ( 'NONE', #9324, #22495 ) ;
#71564=CARTESIAN_POINT ( 'NONE',  ( 135.6272734918642868, -34.46583755400483540, 7.833212107639223376 ) ) ;
#71565=LINE ( 'NONE', #22515, #15203 ) ;
#71567=DIRECTION ( 'NONE',  ( -4.093947403305260305E-16, 1.000000000000000000, -6.162975822039159109E-32 ) ) ;
#71568=CARTESIAN_POINT ( 'NONE',  ( 108.0121126588926046, -24.94157235513516468, 261.0127681330534415 ) ) ;
#71570=CARTESIAN_POINT ( 'NONE',  ( 165.6738106836030227, -28.98061976758901537, 342.9256252759109884 ) ) ;
#71572=CARTESIAN_POINT ( 'NONE',  ( 97.81373435033219721, -40.51654435448209313, 87.63515866765291662 ) ) ;
#71575=CARTESIAN_POINT ( 'NONE',  ( 97.33784130303931192, -34.07106455859420890, 257.1147919449370534 ) ) ;
#71577=CARTESIAN_POINT ( 'NONE',  ( 111.9759329535769297, -43.13121445202460791, 195.5838068554168103 ) ) ;
#71578=ORIENTED_EDGE ( 'NONE', *, *, #77485, .T. ) ;
#71580=CARTESIAN_POINT ( 'NONE',  ( 109.8619129364321481, -26.66307059906275612, 174.8613395616249591 ) ) ;
#71581=CARTESIAN_POINT ( 'NONE',  ( 104.0427601340384030, -47.36105469373795529, 63.36800622829197494 ) ) ;
#71582=CARTESIAN_POINT ( 'NONE',  ( 103.6242938494280423, -26.17725164406494542, 206.3394347997209763 ) ) ;
#71584=DIRECTION ( 'NONE',  ( -4.237773401492740281E-14, 1.000000000000000000, 0.000000000000000000 ) ) ;
#71585=DIRECTION ( 'NONE',  ( 0.7071067811861728725, -0.7071067811869222730, 0.000000000000000000 ) ) ;
#71588=PLANE ( 'NONE',  #15136 ) ;
#71589=EDGE_LOOP ( 'NONE', ( #59626, #67694, #81445, #30276 ) ) ;
#71591=LINE ( 'NONE', #80188, #38428 ) ;
#71592=VERTEX_POINT ( 'NONE', #79474 ) ;
#71593=ORIENTED_EDGE ( 'NONE', *, *, #11756, .T. ) ;
#71594=CARTESIAN_POINT ( 'NONE',  ( 98.64819939953339656, -38.17465580927972724, 90.88384839950496996 ) ) ;
#71597=CARTESIAN_POINT ( 'NONE',  ( 116.9541756933414263, -33.49491404195861577, 85.07848241876791917 ) ) ;
#71599=DIRECTION ( 'NONE',  ( 1.000000000000000078E-15, -1.000000000000000083E-30, -1.000000000000000000 ) ) ;
#71600=CARTESIAN_POINT ( 'NONE',  ( 100.9546728288143527, -28.70702571419132809, 176.5939586075147929 ) ) ;
#71601=EDGE_CURVE ( 'NONE', #42662, #5137, #52117, .T. ) ;
#71602=CARTESIAN_POINT ( 'NONE',  ( 112.5987260342905358, -28.66361022110268308, 44.59848241876795782 ) ) ;
#71603=VERTEX_POINT ( 'NONE', #64490 ) ;
#71605=ORIENTED_EDGE ( 'NONE', *, *, #52115, .F. ) ;
#71606=AXIS2_PLACEMENT_3D ( 'NONE', #35685, #56574, #1638 ) ;
#71609=CARTESIAN_POINT ( 'NONE',  ( 97.06107109598296745, -37.99641195321030551, 117.4272919417498144 ) ) ;
#71610=VECTOR ( 'NONE', #1837, 1000.000000000000000 ) ;
#71613=CARTESIAN_POINT ( 'NONE',  ( 108.4182074779043603, -26.73512707025641433, 50.97033420604262943 ) ) ;
#71616=CARTESIAN_POINT ( 'NONE',  ( 104.7644060343265409, -46.87484541886973943, 72.39848241876795498 ) ) ;
#71618=CARTESIAN_POINT ( 'NONE',  ( 116.3251852747984003, -32.94148267319277323, 269.1356252759109680 ) ) ;
#71620=CARTESIAN_POINT ( 'NONE',  ( 99.95702547362903090, -40.74009991652987139, 134.5538046553059530 ) ) ;
#71621=ADVANCED_FACE ( 'NONE', ( #57660 ), #28459, .T. ) ;
#71622=AXIS2_PLACEMENT_3D ( 'NONE', #5928, #33617, #61312 ) ;
#71624=LINE ( 'NONE', #16651, #48477 ) ;
#71626=VERTEX_POINT ( 'NONE', #2113 ) ;
#71627=EDGE_LOOP ( 'NONE', ( #57334, #31524 ) ) ;
#71628=DIRECTION ( 'NONE',  ( 0.000000000000000000, 0.000000000000000000, 1.000000000000000000 ) ) ;
#71632=CARTESIAN_POINT ( 'NONE',  ( 115.3361691346596558, -39.99662111280561305, 189.9587261630399553 ) ) ;
#71633=DIRECTION ( 'NONE',  ( 1.000000000000000000, 4.299999999999999979E-14, 1.000000000000000078E-15 ) ) ;
#71634=CARTESIAN_POINT ( 'NONE',  ( 107.9474582775578568, -25.68820226555254749, 111.0251490854349754 ) ) ;
#71635=CARTESIAN_POINT ( 'NONE',  ( 105.7995185650176779, -26.72403495711487764, 120.1772919364191665 ) ) ;
#71636=VECTOR ( 'NONE', #40323, 1000.000000000000000 ) ;
#71637=CARTESIAN_POINT ( 'NONE',  ( 98.30753417424557483, -41.72887546278693094, 82.73979193999794290 ) ) ;
#71638=VERTEX_POINT ( 'NONE', #29377 ) ;
#71640=ORIENTED_EDGE ( 'NONE', *, *, #49136, .T. ) ;
#71642=CARTESIAN_POINT ( 'NONE',  ( 108.3259390676978455, -28.66449228317154763, 187.7709475124489700 ) ) ;
#71643=CARTESIAN_POINT ( 'NONE',  ( 98.57199122844706096, -43.83852907894476658, 71.86895860924397539 ) ) ;
#71644=ORIENTED_EDGE ( 'NONE', *, *, #51013, .T. ) ;
#71645=ADVANCED_FACE ( 'NONE', ( #1674 ), #78434, .T. ) ;
#71646=CARTESIAN_POINT ( 'NONE',  ( 106.2538455105912050, -26.32252419718678027, 25.13848241876792855 ) ) ;
#71647=CARTESIAN_POINT ( 'NONE',  ( 99.27233432241882838, -29.77326281039884037, 186.7470538473389752 ) ) ;
#71648=DIRECTION ( 'NONE',  ( 1.000000000000000078E-15, 1.000000000000000083E-30, -1.000000000000000000 ) ) ;
#71650=EDGE_CURVE ( 'NONE', #3324, #53629, #79727, .T. ) ;
#71651=CARTESIAN_POINT ( 'NONE',  ( 114.7713543040237454, -44.65465650488444993, 114.2022919425779719 ) ) ;
#71653=ORIENTED_EDGE ( 'NONE', *, *, #21949, .F. ) ;
#71655=EDGE_CURVE ( 'NONE', #42544, #19998, #49345, .T. ) ;
#71656=ORIENTED_EDGE ( 'NONE', *, *, #56713, .F. ) ;
#71658=DIRECTION ( 'NONE',  ( 6.745093096447288888E-17, 1.000000000000000000, 0.000000000000000000 ) ) ;
#71659=VERTEX_POINT ( 'NONE', #42524 ) ;
#71662=CARTESIAN_POINT ( 'NONE',  ( 108.1495617321014748, -26.75831605517002387, 130.9904251009939173 ) ) ;
#71663=CARTESIAN_POINT ( 'NONE',  ( 97.28826076399516865, -33.11373220042904109, 66.04419670448297097 ) ) ;
#71666=CARTESIAN_POINT ( 'NONE',  ( 163.0667039024470171, -33.35206098992711077, -5.074374724088000832 ) ) ;
#71667=CARTESIAN_POINT ( 'NONE',  ( 115.7831076719501056, -41.80230950688442704, 74.40645860955640956 ) ) ;
#71668=CARTESIAN_POINT ( 'NONE',  ( 112.4622727538958884, -27.87370092883236694, 49.62895860924398761 ) ) ;
#71669=CARTESIAN_POINT ( 'NONE',  ( 105.7992162164682384, -26.72406929376951723, 110.1773159172848722 ) ) ;
#71670=CARTESIAN_POINT ( 'NONE',  ( 114.4965984691700953, -29.44205611023144087, 145.4441967044819819 ) ) ;
#71671=CARTESIAN_POINT ( 'NONE',  ( 116.3173461584868278, -32.93718857426866720, 59.13562527591098217 ) ) ;
#71673=ADVANCED_FACE ( 'NONE', ( #71166 ), #77076, .F. ) ;
#71674=ORIENTED_EDGE ( 'NONE', *, *, #42801, .T. ) ;
#71678=LINE ( 'NONE', #57580, #72333 ) ;
#71679=CARTESIAN_POINT ( 'NONE',  ( 107.2439172579031919, -47.23279478401654075, 212.5899109901969837 ) ) ;
#71681=DIRECTION ( 'NONE',  ( -1.000000000000000000, -5.512527431108013646E-15, 0.000000000000000000 ) ) ;
#71682=CARTESIAN_POINT ( 'NONE',  ( 98.92566635982139189, -30.18235936901480443, 236.7870538473399336 ) ) ;
#71683=CARTESIAN_POINT ( 'NONE',  ( 98.11234142011190329, -43.28847465721014487, 102.8175300378159847 ) ) ;
#71685=CARTESIAN_POINT ( 'NONE',  ( 116.3231543710223121, -32.93883412237410369, 190.1356252759109680 ) ) ;
#71688=VECTOR ( 'NONE', #49586, 1000.000000000000000 ) ;
#71690=AXIS2_PLACEMENT_3D ( 'NONE', #68422, #81622, #12560 ) ;
#71694=EDGE_LOOP ( 'NONE', ( #20910, #49694, #34358, #28947 ) ) ;
#71696=CARTESIAN_POINT ( 'NONE',  ( 100.1387811872355371, -44.51978932219680019, 262.9984824187678782 ) ) ;
#71701=DIRECTION ( 'NONE',  ( 1.000000000000000078E-15, 1.000000000000000083E-30, -1.000000000000000000 ) ) ;
#71702=ADVANCED_FACE ( 'NONE', ( #84356, #14858 ), #63436, .T. ) ;
#71703=CARTESIAN_POINT ( 'NONE',  ( 101.0745446329174655, -30.64234581064881269, 225.1181341137909442 ) ) ;
#71705=VERTEX_POINT ( 'NONE', #22566 ) ;
#71706=ORIENTED_EDGE ( 'NONE', *, *, #54056, .T. ) ;
#71709=CARTESIAN_POINT ( 'NONE',  ( 107.9555263298577188, -25.64695713395855137, 261.0127681330532710 ) ) ;
#71710=CARTESIAN_POINT ( 'NONE',  ( 180.3521107875703535, -35.65087443489212404, 237.4678068554150059 ) ) ;
#71711=CARTESIAN_POINT ( 'NONE',  ( 98.15811136316406760, -31.42099212808723863, 126.9108633711489915 ) ) ;
#71714=LINE ( 'NONE', #56721, #87882 ) ;
#71715=LINE ( 'NONE', #56722, #8530 ) ;
#71718=CARTESIAN_POINT ( 'NONE',  ( 105.5764564592757466, -44.77785207962899250, 10.24809036959195652 ) ) ;
#71720=EDGE_CURVE ( 'NONE', #5050, #28392, #50240, .T. ) ;
#71722=DIRECTION ( 'NONE',  ( 0.7071067811866516006, -0.7071067811864434338, 0.000000000000000000 ) ) ;
#71723=AXIS2_PLACEMENT_3D ( 'NONE', #62607, #6304, #33997 ) ;
#71724=DIRECTION ( 'NONE',  ( 0.000000000000000000, 0.000000000000000000, 1.000000000000000000 ) ) ;
#71727=DIRECTION ( 'NONE',  ( 1.000000000000000078E-15, -1.000000000000000083E-30, -1.000000000000000000 ) ) ;
#71728=DIRECTION ( 'NONE',  ( 0.000000000000000000, 0.000000000000000000, 1.000000000000000000 ) ) ;
#71729=VERTEX_POINT ( 'NONE', #8485 ) ;
#71730=CARTESIAN_POINT ( 'NONE',  ( 104.0426969376867987, -47.36127689622573200, 67.36800622829191809 ) ) ;
#71731=EDGE_LOOP ( 'NONE', ( #9395, #49030, #30160, #57426 ) ) ;
#71732=CARTESIAN_POINT ( 'NONE',  ( 102.8831062096190436, -29.28260300185988996, 59.90670554236199052 ) ) ;
#71734=CARTESIAN_POINT ( 'NONE',  ( 111.4018971211722544, -45.77100106855414197, 88.93158766652720715 ) ) ;
#71735=CARTESIAN_POINT ( 'NONE',  ( 103.5852769812406535, -44.87864842379759978, 88.68729759161098514 ) ) ;
#71737=CARTESIAN_POINT ( 'NONE',  ( 49.16670390244745192, -28.27351298637373489, 313.9678068554150059 ) ) ;
#71738=CARTESIAN_POINT ( 'NONE',  ( 22.49563609058251146, -67.87844715994100397, 307.9888746672805269 ) ) ;
#71739=CARTESIAN_POINT ( 'NONE',  ( 111.0094172226674374, -46.42718045843506047, 278.8841967044824059 ) ) ;
#71741=VERTEX_POINT ( 'NONE', #43874 ) ;
#71743=VECTOR ( 'NONE', #43866, 1000.000000000000114 ) ;
#71745=CARTESIAN_POINT ( 'NONE',  ( 108.2828737166157964, -47.76209090725709672, 153.6518157521009584 ) ) ;
#71746=DIRECTION ( 'NONE',  ( 1.000000000000000000, 4.299999999999999979E-14, 1.000000000000000078E-15 ) ) ;
#71747=VECTOR ( 'NONE', #31895, 1000.000000000000000 ) ;
#71748=AXIS2_PLACEMENT_3D ( 'NONE', #6779, #66422, #34479 ) ;
#71750=EDGE_LOOP ( 'NONE', ( #85595, #17245, #83898, #8985 ) ) ;
#71752=EDGE_LOOP ( 'NONE', ( #21939, #71992, #19500, #3275 ) ) ;
#71755=LINE ( 'NONE', #9522, #7224 ) ;
#71756=CARTESIAN_POINT ( 'NONE',  ( 114.9950743857441608, -30.04541929558963886, 224.3718157521019521 ) ) ;
#71757=CARTESIAN_POINT ( 'NONE',  ( 41.56648329127499153, -36.32844715994070839, 14.17562527591199917 ) ) ;
#71758=CARTESIAN_POINT ( 'NONE',  ( 31.56670390244621771, -32.29483332968584364, 193.9678068554150911 ) ) ;
#71759=CYLINDRICAL_SURFACE ( 'NONE', #60602, 3.249999999999975131 ) ;
#71760=EDGE_CURVE ( 'NONE', #56062, #14566, #7134, .T. ) ;
#71761=CARTESIAN_POINT ( 'NONE',  ( 99.76212870471702843, -44.21728614272981872, 17.96133956162493206 ) ) ;
#71764=CARTESIAN_POINT ( 'NONE',  ( 116.3153332067577850, -32.94059133099460723, 170.1356252759109680 ) ) ;
#71767=CARTESIAN_POINT ( 'NONE',  ( 82.10314251156495402, -20.57949487819488255, 2.327894807232544938 ) ) ;
#71769=CARTESIAN_POINT ( 'NONE',  ( 110.2492204789523242, -26.78788743924345184, 234.8299109901969643 ) ) ;
#71770=DIRECTION ( 'NONE',  ( -4.299999999999999979E-14, 1.000000000000000000, -4.400000000000000367E-29 ) ) ;
#71771=FACE_BOUND ( 'NONE', #2693, .T. ) ;
#71773=CARTESIAN_POINT ( 'NONE',  ( 115.1107970995275736, -40.88897666221423322, 242.8571817328389670 ) ) ;
#71774=CYLINDRICAL_SURFACE ( 'NONE', #82389, 2.517499999999998739 ) ;
#71775=CARTESIAN_POINT ( 'NONE',  ( 96.20032699425235023, -38.62430069186628856, 42.45181575210199298 ) ) ;
#71777=CARTESIAN_POINT ( 'NONE',  ( 113.8852007176727028, -44.67373811025045427, 108.1413395616249744 ) ) ;
#71779=CARTESIAN_POINT ( 'NONE',  ( 131.7480217999322747, -20.20859666167233470, 7.273989459504827337 ) ) ;
#71781=ORIENTED_EDGE ( 'NONE', *, *, #2228, .T. ) ;
#71782=CARTESIAN_POINT ( 'NONE',  ( 83.06670390244796920, -61.87844715994100397, 231.5838068554150198 ) ) ;
#71784=CARTESIAN_POINT ( 'NONE',  ( 112.7628927828184402, -28.45360054538134520, 275.5965050139159302 ) ) ;
#71785=ORIENTED_EDGE ( 'NONE', *, *, #45616, .T. ) ;
#71786=DIRECTION ( 'NONE',  ( 0.000000000000000000, 0.000000000000000000, -1.000000000000000000 ) ) ;
#71787=ORIENTED_EDGE ( 'NONE', *, *, #84269, .T. ) ;
#71788=CARTESIAN_POINT ( 'NONE',  ( 194.0371591254572650, -24.42818131005417825, 313.9678068554149490 ) ) ;
#71789=FACE_OUTER_BOUND ( 'NONE', #25321, .T. ) ;
#71790=DIRECTION ( 'NONE',  ( 0.000000000000000000, 0.000000000000000000, -1.000000000000000000 ) ) ;
#71792=CARTESIAN_POINT ( 'NONE',  ( 103.2708046866033129, -47.13561192255075838, 97.28610146638693834 ) ) ;
#71794=AXIS2_PLACEMENT_3D ( 'NONE', #45276, #72994, #10761 ) ;
#71795=CARTESIAN_POINT ( 'NONE',  ( 188.5667039024486087, -48.82844715993430640, 137.2178068554150059 ) ) ;
#71796=CARTESIAN_POINT ( 'NONE',  ( 165.6738106836030227, -28.98061976758901892, -5.074374724088000832 ) ) ;
#71798=ORIENTED_EDGE ( 'NONE', *, *, #67275, .F. ) ;
#71801=DIRECTION ( 'NONE',  ( 0.000000000000000000, 1.000000000000000000, 0.000000000000000000 ) ) ;
#71802=DIRECTION ( 'NONE',  ( 0.000000000000000000, 0.000000000000000000, 1.000000000000000000 ) ) ;
#71803=FACE_OUTER_BOUND ( 'NONE', #4269, .T. ) ;
#71804=LINE ( 'NONE', #78192, #15200 ) ;
#71805=LINE ( 'NONE', #78644, #59596 ) ;
#71807=ORIENTED_EDGE ( 'NONE', *, *, #16992, .T. ) ;
#71808=AXIS2_PLACEMENT_3D ( 'NONE', #52652, #87663, #26326 ) ;
#71809=TOROIDAL_SURFACE ( 'NONE', #5077, 11.75000000000000000, 2.125000000000000000 ) ;
#71812=CARTESIAN_POINT ( 'NONE',  ( 98.51953950620418254, -30.85675296092865239, 161.8594347997199918 ) ) ;
#71813=CARTESIAN_POINT ( 'NONE',  ( 71.06648329127399677, -18.82844715994099971, 284.9256252759119548 ) ) ;
#71814=ORIENTED_EDGE ( 'NONE', *, *, #18304, .F. ) ;
#71815=VECTOR ( 'NONE', #13474, 1000.000000000000000 ) ;
#71816=VECTOR ( 'NONE', #34144, 1000.000000000000000 ) ;
#71817=CARTESIAN_POINT ( 'NONE',  ( 98.36549455146196408, -40.29075363668730603, 7.635625275910939536 ) ) ;
#71818=FACE_BOUND ( 'NONE', #34417, .T. ) ;
#71820=PLANE ( 'NONE',  #12284 ) ;
#71821=CARTESIAN_POINT ( 'NONE',  ( 108.4186682723848634, -26.73518572642002411, 29.96909420486912268 ) ) ;
#71822=CARTESIAN_POINT ( 'NONE',  ( 97.44287158780957725, -40.59272077381807975, 251.6422919425783675 ) ) ;
#71823=EDGE_LOOP ( 'NONE', ( #77462, #68221, #88699, #25720 ) ) ;
#71824=ORIENTED_EDGE ( 'NONE', *, *, #88887, .T. ) ;
#71826=CARTESIAN_POINT ( 'NONE',  ( 102.0804048320179618, -44.05524405925518039, 193.5330118773259755 ) ) ;
#71828=ADVANCED_FACE ( 'NONE', ( #55686 ), #42969, .T. ) ;
#71829=CARTESIAN_POINT ( 'NONE',  ( 114.3297541623348224, -29.74979092151301074, 35.86729759161094933 ) ) ;
#71832=CARTESIAN_POINT ( 'NONE',  ( 112.1393456441725931, -28.01282278273417603, 79.65645860901210540 ) ) ;
#71833=B_SPLINE_CURVE_WITH_KNOTS ( 'NONE', 3,
 ( #37198, #64901, #58076, #85814, #23583, #31257, #12173, #74847, #39857, #53465, #67578, #52570, #66677, #88029, #74395, #4461, #18074, #45322, #68026, #81677, #40310, #80776, #45762, #46211, #73490, #11266, #87137, #38968, #73040, #87580, #46667, #4007, #32596, #25337, #12623, #25794, #66219 ),
 .UNSPECIFIED., .F., .F.,
 ( 4, 2, 2, 1, 2, 2, 2, 1, 1, 2, 2, 2, 2, 1, 2, 2, 2, 1, 1, 1, 2, 4 ),
 ( 0.6666501603261554276, 0.6874845253057836336, 0.6926931165506905463, 0.6979017077955975701, 0.7083188902854107294, 0.7499876202446639217, 0.7525919158671158238, 0.7551962114895677258, 0.7604048027344691985, 0.7708219852242721437, 0.7916563502038780342, 0.8124907151834839247, 0.8176993064283852863, 0.8229078976732865369, 0.8333250801630887050, 0.8749938101222999309, 0.8775981057447522771, 0.8802024013672045122, 0.8854109926121092045, 0.8958281751019185890, 0.9166625400815370250, 1.000000000000000000 ),
 .UNSPECIFIED. ) ;
#71834=EDGE_CURVE ( 'NONE', #82808, #52812, #69811, .T. ) ;
#71835=DIRECTION ( 'NONE',  ( 0.000000000000000000, 0.000000000000000000, -1.000000000000000000 ) ) ;
#71837=CARTESIAN_POINT ( 'NONE',  ( 172.5664832912729878, -27.82844715994070484, 315.9256252759120116 ) ) ;
#71838=DIRECTION ( 'NONE',  ( 0.7071067811866516006, -0.7071067811864434338, 0.000000000000000000 ) ) ;
#71839=CARTESIAN_POINT ( 'NONE',  ( 110.7254274611716056, -26.32387412717027786, 254.8194347997205682 ) ) ;
#71841=ORIENTED_EDGE ( 'NONE', *, *, #71092, .F. ) ;
#71842=EDGE_CURVE ( 'NONE', #39081, #83239, #37444, .T. ) ;
#71844=CARTESIAN_POINT ( 'NONE',  ( 104.4081006514864924, -46.45808913754018477, 82.36479194178809848 ) ) ;
#71847=FACE_BOUND ( 'NONE', #83355, .T. ) ;
#71848=EDGE_CURVE ( 'NONE', #40542, #45509, #68105, .T. ) ;
#71850=CARTESIAN_POINT ( 'NONE',  ( 105.5226833586260966, -46.38761039419742360, 33.44991099019595282 ) ) ;
#71851=CARTESIAN_POINT ( 'NONE',  ( 19.56670390244796920, -48.82844715994099971, 310.9178068554150514 ) ) ;
#71853=CARTESIAN_POINT ( 'NONE',  ( 117.1334281162953346, -32.05460809866745109, 55.16038718067301261 ) ) ;
#71856=CARTESIAN_POINT ( 'NONE',  ( 96.91416677013903325, -34.20826173260762459, 276.1327681330537871 ) ) ;
#71857=ORIENTED_EDGE ( 'NONE', *, *, #43102, .F. ) ;
#71858=CARTESIAN_POINT ( 'NONE',  ( 21.03715912545824551, -47.82818131006186491, 300.4678068554150059 ) ) ;
#71859=PLANE ( 'NONE',  #22547 ) ;
#71860=DIRECTION ( 'NONE',  ( 0.000000000000000000, 0.000000000000000000, 1.000000000000000000 ) ) ;
#71861=ADVANCED_FACE ( 'NONE', ( #29745, #9739 ), #56530, .F. ) ;
#71862=CARTESIAN_POINT ( 'NONE',  ( 98.42956409136928642, -40.12054696651731689, 94.44237608387695104 ) ) ;
#71863=CARTESIAN_POINT ( 'NONE',  ( 110.0582552220427175, -26.06480902925029497, 215.8708633711489711 ) ) ;
#71864=CARTESIAN_POINT ( 'NONE',  ( 182.0374245136140132, -23.42844715993459559, 313.9678068554149490 ) ) ;
#71865=EDGE_LOOP ( 'NONE', ( #49486, #53951 ) ) ;
#71866=CARTESIAN_POINT ( 'NONE',  ( 37.03715912545433042, -48.62818131006122258, 249.9678068554150343 ) ) ;
#71868=EDGE_LOOP ( 'NONE', ( #89854, #57877, #42695, #68385 ) ) ;
#71869=CIRCLE ( 'NONE', #89252, 2.117000000000000881 ) ;
#71870=VECTOR ( 'NONE', #27893, 1000.000000000000000 ) ;
#71871=DIRECTION ( 'NONE',  ( 0.000000000000000000, -1.000000000000000000, 0.000000000000000000 ) ) ;
#71872=VECTOR ( 'NONE', #14744, 1000.000000000000000 ) ;
#71873=ORIENTED_EDGE ( 'NONE', *, *, #59471, .F. ) ;
#71874=ORIENTED_EDGE ( 'NONE', *, *, #55118, .F. ) ;
#71877=CARTESIAN_POINT ( 'NONE',  ( 115.7741036766735618, -31.77434046802498457, 40.23810575919497978 ) ) ;
#71878=CARTESIAN_POINT ( 'NONE',  ( 98.57243884988349691, -37.62796858414048273, 125.8324198280769650 ) ) ;
#71879=CARTESIAN_POINT ( 'NONE',  ( 111.8742750991676758, -46.04467666623092015, 272.9556252759110180 ) ) ;
#71880=EDGE_CURVE ( 'NONE', #36969, #51954, #89907, .T. ) ;
#71881=EDGE_CURVE ( 'NONE', #65168, #46193, #71231, .T. ) ;
#71883=ORIENTED_EDGE ( 'NONE', *, *, #53660, .T. ) ;
#71886=DIRECTION ( 'NONE',  ( 1.387778780781444492E-15, 0.000000000000000000, -1.000000000000000000 ) ) ;
#71887=VERTEX_POINT ( 'NONE', #50160 ) ;
#71891=DIRECTION ( 'NONE',  ( 1.000000000000000078E-15, -1.000000000000000000, 0.000000000000000000 ) ) ;
#71895=CARTESIAN_POINT ( 'NONE',  ( 116.2188219837490522, -41.79507674895632618, 263.4241967044824833 ) ) ;
#71896=CARTESIAN_POINT ( 'NONE',  ( 118.1291538054787509, -37.63212066291781355, 34.77372051400695341 ) ) ;
#71898=CARTESIAN_POINT ( 'NONE',  ( 31.90335556477799628, -33.89581943344391135, -5.074374724088000832 ) ) ;
#71902=FACE_OUTER_BOUND ( 'NONE', #37466, .T. ) ;
#71903=FACE_OUTER_BOUND ( 'NONE', #1979, .T. ) ;
#71904=CARTESIAN_POINT ( 'NONE',  ( 83.06670390244796920, -61.87844715994100397, 234.8338068554150198 ) ) ;
#71905=DIRECTION ( 'NONE',  ( 0.000000000000000000, 0.000000000000000000, 1.000000000000000000 ) ) ;
#71907=CARTESIAN_POINT ( 'NONE',  ( 168.3664380525667639, -48.62818131005477795, 300.4678068554149490 ) ) ;
#71908=CARTESIAN_POINT ( 'NONE',  ( 33.96670390244699433, -26.71338133339301635, 342.9256252759119548 ) ) ;
#71909=CARTESIAN_POINT ( 'NONE',  ( 116.1968789481791191, -43.04691504047773520, 13.35657765686298859 ) ) ;
#71910=CARTESIAN_POINT ( 'NONE',  ( 98.66592356458792779, -30.49631559909255074, 176.8184824187679567 ) ) ;
#71911=CARTESIAN_POINT ( 'NONE',  ( 96.90588099414922851, -39.15831928773680914, 52.51276813305394597 ) ) ;
#71912=CARTESIAN_POINT ( 'NONE',  ( 83.73314995793998605, 12.92155284005730387, 355.9756252759109998 ) ) ;
#71913=CARTESIAN_POINT ( 'NONE',  ( 172.5664832912729878, -27.57844715994070484, 321.9256252759120116 ) ) ;
#71914=CARTESIAN_POINT ( 'NONE',  ( 82.16842210270093005, -34.94667169166114462, 2.376609173395129115 ) ) ;
#71915=CIRCLE ( 'NONE', #67560, 0.5000000000000073275 ) ;
#71916=VERTEX_POINT ( 'NONE', #16555 ) ;
#71919=CARTESIAN_POINT ( 'NONE',  ( 116.1466984671187248, -33.09446055034466383, 50.12991099019598096 ) ) ;
#71920=CARTESIAN_POINT ( 'NONE',  ( 29.56648329127298069, -71.37844715994266664, 342.9256252759109884 ) ) ;
#71923=CARTESIAN_POINT ( 'NONE',  ( 108.6716496925947126, -26.45072611336629720, 185.9527681330539792 ) ) ;
#71925=CARTESIAN_POINT ( 'NONE',  ( 97.86673084626464458, -40.64958532137394087, 146.6470202068057063 ) ) ;
#71928=CARTESIAN_POINT ( 'NONE',  ( 182.2300522401173168, -33.89581943343755910, 237.4678068554150059 ) ) ;
#71929=CARTESIAN_POINT ( 'NONE',  ( 108.3313117362001492, -46.73510236842512455, 97.67716632620181372 ) ) ;
#71930=CARTESIAN_POINT ( 'NONE',  ( 107.3174176841070846, -26.95189801805063823, 120.0556252759109555 ) ) ;
#71931=EDGE_LOOP ( 'NONE', ( #50749, #40855, #44297, #31491 ) ) ;
#71932=ORIENTED_EDGE ( 'NONE', *, *, #74991, .F. ) ;
#71933=VECTOR ( 'NONE', #69924, 1000.000000000000000 ) ;
#71934=CARTESIAN_POINT ( 'NONE',  ( 98.33263373320089329, -38.22883053613415427, 87.89301187732596077 ) ) ;
#71935=CIRCLE ( 'NONE', #18231, 16.00000000000000000 ) ;
#71939=CARTESIAN_POINT ( 'NONE',  ( 99.44473759953889669, -30.59981194223820467, 236.7870538473389388 ) ) ;
#71940=CARTESIAN_POINT ( 'NONE',  ( 83.56670390244801183, -36.72944715994108122, 219.5838068554169809 ) ) ;
#71941=VECTOR ( 'NONE', #34841, 1000.000000000000000 ) ;
#71942=CARTESIAN_POINT ( 'NONE',  ( 46.03715912545342093, -48.62818131006090283, 193.9678068554150911 ) ) ;
#71943=CARTESIAN_POINT ( 'NONE',  ( 116.3212776292293569, -32.94146857471253753, 110.1356252759109822 ) ) ;
#71944=EDGE_CURVE ( 'NONE', #39083, #40784, #28846, .T. ) ;
#71945=LINE ( 'NONE', #78773, #1140 ) ;
#71946=EDGE_CURVE ( 'NONE', #64140, #83074, #22047, .T. ) ;
#71949=CARTESIAN_POINT ( 'NONE',  ( 108.5866130067098538, -47.05677245125747277, 142.6927681330539883 ) ) ;
#71950=VERTEX_POINT ( 'NONE', #53264 ) ;
#71953=EDGE_CURVE ( 'NONE', #42074, #69327, #17881, .T. ) ;
#71954=CARTESIAN_POINT ( 'NONE',  ( 165.9667039024459996, -28.27351298637401200, -5.074374724088000832 ) ) ;
#71955=CARTESIAN_POINT ( 'NONE',  ( 77.45963244950117144, -17.85248396558682416, 2.902015641458085771 ) ) ;
#71957=LINE ( 'NONE', #9723, #71468 ) ;
#71959=CARTESIAN_POINT ( 'NONE',  ( 102.0474437309886184, -43.16675777147634108, 229.8680903695919540 ) ) ;
#71960=EDGE_CURVE ( 'NONE', #63602, #83432, #18326, .T. ) ;
#71961=CARTESIAN_POINT ( 'NONE',  ( 177.0664832912740110, 12.92155284005802685, 335.5992267699913327 ) ) ;
#71962=AXIS2_PLACEMENT_3D ( 'NONE', #17728, #88564, #11351 ) ;
#71963=EDGE_CURVE ( 'NONE', #26343, #61899, #33278, .T. ) ;
#71964=CARTESIAN_POINT ( 'NONE',  ( 117.9487373648833426, -34.79150140969374405, 198.9546728949589749 ) ) ;
#71965=CYLINDRICAL_SURFACE ( 'NONE', #2496, 3.299999999999999822 ) ;
#71968=VERTEX_POINT ( 'NONE', #59208 ) ;
#71969=CARTESIAN_POINT ( 'NONE',  ( 117.0679413654940646, -37.57840742081197050, 64.75943071796990580 ) ) ;
#71970=ORIENTED_EDGE ( 'NONE', *, *, #19617, .T. ) ;
#71972=CARTESIAN_POINT ( 'NONE',  ( 49.35211078756945824, -35.65087443489821339, 117.4678068554150485 ) ) ;
#71973=ADVANCED_FACE ( 'NONE', ( #25591 ), #73935, .F. ) ;
#71974=CARTESIAN_POINT ( 'NONE',  ( 114.4012193684849734, -41.70236635182605056, 269.7844404487540260 ) ) ;
#71976=ORIENTED_EDGE ( 'NONE', *, *, #30359, .F. ) ;
#71977=CARTESIAN_POINT ( 'NONE',  ( 116.3568090314797132, -39.36905942218098176, 9.635625275910941312 ) ) ;
#71981=CARTESIAN_POINT ( 'NONE',  ( 108.3335591113261245, -46.73484676085423217, 112.6773436138281141 ) ) ;
#71983=ORIENTED_EDGE ( 'NONE', *, *, #27353, .T. ) ;
#71984=CARTESIAN_POINT ( 'NONE',  ( 115.6248209149117940, -37.18450138507482450, 18.20670554236297889 ) ) ;
#71985=CARTESIAN_POINT ( 'NONE',  ( 108.0089373620841826, -26.32355773090834816, 155.0041967044819557 ) ) ;
#71986=CARTESIAN_POINT ( 'NONE',  ( 114.2249171546291677, -45.12625265263336871, 153.1508633711489722 ) ) ;
#71987=DIRECTION ( 'NONE',  ( 0.000000000000000000, 1.000000000000000000, 0.000000000000000000 ) ) ;
#71988=CARTESIAN_POINT ( 'NONE',  ( 97.61538875609650745, -41.12936756086440226, 252.6727681330536655 ) ) ;
#71990=CARTESIAN_POINT ( 'NONE',  ( 188.5667039024482392, -48.82844715993431350, 295.7178068554150059 ) ) ;
#71991=CARTESIAN_POINT ( 'NONE',  ( 107.0664832912748068, -36.72944715993923381, -5.074374724089029343 ) ) ;
#71992=ORIENTED_EDGE ( 'NONE', *, *, #56339, .F. ) ;
#71993=EDGE_CURVE ( 'NONE', #71968, #74301, #73288, .T. ) ;
#71995=EDGE_CURVE ( 'NONE', #34216, #34233, #10075, .T. ) ;
#71996=CIRCLE ( 'NONE', #22668, 2.500000000000002220 ) ;
#71997=AXIS2_PLACEMENT_3D ( 'NONE', #14588, #44387, #65299 ) ;
#71998=CARTESIAN_POINT ( 'NONE',  ( 109.6166107820099569, -26.53883167775938645, 199.8813395616249977 ) ) ;
#72000=CIRCLE ( 'NONE', #19793, 2.030000000000003801 ) ;
#72001=CARTESIAN_POINT ( 'NONE',  ( 114.3440588962603215, -29.21527388614784115, 174.4641967044819637 ) ) ;
#72002=DIRECTION ( 'NONE',  ( 0.9825752044328148749, 0.1858654557302456822, 0.000000000000000000 ) ) ;
#72004=CARTESIAN_POINT ( 'NONE',  ( 136.1934021726305275, -34.98608769072284730, 7.448832051633326401 ) ) ;
#72008=CARTESIAN_POINT ( 'NONE',  ( 115.3963619165045458, -41.85549553236474196, 14.38705384733895976 ) ) ;
#72009=DIRECTION ( 'NONE',  ( 0.000000000000000000, 0.000000000000000000, -1.000000000000000000 ) ) ;
#72010=CARTESIAN_POINT ( 'NONE',  ( 80.06648329127402519, -36.72944715994107412, -5.074374724089057764 ) ) ;
#72013=CARTESIAN_POINT ( 'NONE',  ( 104.4899544351757612, -26.97880758891392006, 256.2814586106100592 ) ) ;
#72014=CARTESIAN_POINT ( 'NONE',  ( 131.0667039024480403, -42.21678055153905262, 207.5838068554170377 ) ) ;
#72015=CARTESIAN_POINT ( 'NONE',  ( 115.2539372359732255, -38.22674572785330582, 195.5838068554167251 ) ) ;
#72016=VERTEX_POINT ( 'NONE', #86940 ) ;
#72017=CARTESIAN_POINT ( 'NONE',  ( 126.8164832912740110, -54.62589567669621005, 14.92562527591099020 ) ) ;
#72018=CARTESIAN_POINT ( 'NONE',  ( 102.6741928909662391, -27.25030431863982372, 180.4213395616249898 ) ) ;
#72019=CARTESIAN_POINT ( 'NONE',  ( 118.8426969166518319, -35.40452897077508965, 79.91562527591095488 ) ) ;
#72020=CARTESIAN_POINT ( 'NONE',  ( 98.39890672360048995, -29.79614961819730468, 191.7775300378159784 ) ) ;
#72023=VECTOR ( 'NONE', #74208, 1000.000000000000000 ) ;
#72025=CARTESIAN_POINT ( 'NONE',  ( 112.2334563547038755, -45.33745837553901481, 39.00654346520547477 ) ) ;
#72026=CARTESIAN_POINT ( 'NONE',  ( 126.8164832912739826, -36.72944715994101017, 14.92562527591099020 ) ) ;
#72027=DIRECTION ( 'NONE',  ( 1.000000000000000078E-15, -1.000000000000000083E-30, -1.000000000000000000 ) ) ;
#72028=ORIENTED_EDGE ( 'NONE', *, *, #37246, .F. ) ;
#72029=CARTESIAN_POINT ( 'NONE',  ( 181.5667039024459939, -18.82844715994031048, -5.074374724088000832 ) ) ;
#72030=ORIENTED_EDGE ( 'NONE', *, *, #44285, .T. ) ;
#72031=EDGE_LOOP ( 'NONE', ( #19343, #45119 ) ) ;
#72032=CARTESIAN_POINT ( 'NONE',  ( 112.7360809596688966, -29.66769577629168353, 118.9486103042669782 ) ) ;
#72034=VERTEX_POINT ( 'NONE', #46463 ) ;
#72035=CARTESIAN_POINT ( 'NONE',  ( 98.11562048848820439, -31.42749274529986536, 81.90133956162493689 ) ) ;
#72037=CARTESIAN_POINT ( 'NONE',  ( 77.53592152231050250, -17.65293368212969227, 7.043713522541727556 ) ) ;
#72038=DIRECTION ( 'NONE',  ( 1.000000000000000000, 0.000000000000000000, 9.462128050782575008E-16 ) ) ;
#72039=CARTESIAN_POINT ( 'NONE',  ( 111.0600676157742726, -27.80113716294804505, 24.74133956162494030 ) ) ;
#72041=EDGE_CURVE ( 'NONE', #48350, #83417, #72418, .T. ) ;
#72044=CARTESIAN_POINT ( 'NONE',  ( 50.96943157743499597, -34.03355364505720360, -5.074374724088000832 ) ) ;
#72046=DIRECTION ( 'NONE',  ( 0.000000000000000000, 0.000000000000000000, -1.000000000000000000 ) ) ;
#72050=CARTESIAN_POINT ( 'NONE',  ( 115.0895152844205143, -30.61842842605814496, 50.34448410232288040 ) ) ;
#72051=EDGE_CURVE ( 'NONE', #4843, #37315, #3372, .T. ) ;
#72052=CARTESIAN_POINT ( 'NONE',  ( 45.77381068363443006, -48.62134037875091508, 180.4678068554150911 ) ) ;
#72053=EDGE_CURVE ( 'NONE', #13427, #4391, #76852, .T. ) ;
#72055=CARTESIAN_POINT ( 'NONE',  ( 97.82856912889580769, -29.34641599088746133, 45.78991099019697231 ) ) ;
#72056=ORIENTED_EDGE ( 'NONE', *, *, #71842, .F. ) ;
#72057=EDGE_CURVE ( 'NONE', #42074, #59810, #81224, .T. ) ;
#72058=PLANE ( 'NONE',  #60370 ) ;
#72060=AXIS2_PLACEMENT_3D ( 'NONE', #39767, #66131, #40214 ) ;
#72062=CARTESIAN_POINT ( 'NONE',  ( 113.0492235774716363, -42.98306560958572931, 110.9899951314959594 ) ) ;
#72063=EDGE_CURVE ( 'NONE', #42164, #37640, #53604, .T. ) ;
#72064=CIRCLE ( 'NONE', #54633, 0.5000000000000004441 ) ;
#72066=CIRCLE ( 'NONE', #38711, 1.000000000000000888 ) ;
#72067=CARTESIAN_POINT ( 'NONE',  ( 97.79840183623460348, -40.48482318767148769, 96.63282328633124507 ) ) ;
#72069=DIRECTION ( 'NONE',  ( 0.000000000000000000, 0.000000000000000000, 1.000000000000000000 ) ) ;
#72070=ORIENTED_EDGE ( 'NONE', *, *, #17692, .T. ) ;
#72074=ORIENTED_EDGE ( 'NONE', *, *, #12159, .F. ) ;
#72075=EDGE_CURVE ( 'NONE', #17322, #45997, #17445, .T. ) ;
#72076=CARTESIAN_POINT ( 'NONE',  ( 104.9381124493903457, -46.57529615900893560, 178.8387261630399507 ) ) ;
#72079=CARTESIAN_POINT ( 'NONE',  ( 97.77490566832175034, -42.75910828249967466, 142.7965776568629508 ) ) ;
#72081=CARTESIAN_POINT ( 'NONE',  ( 100.8874678619102241, -44.70022135782634365, 83.05229194033439910 ) ) ;
#72082=VERTEX_POINT ( 'NONE', #11523 ) ;
#72084=ORIENTED_EDGE ( 'NONE', *, *, #9001, .F. ) ;
#72085=CARTESIAN_POINT ( 'NONE',  ( 107.9397346479727418, -44.84530559174715592, 200.4795189410199612 ) ) ;
#72086=CARTESIAN_POINT ( 'NONE',  ( 118.8678016624199358, -35.40170448615204890, 83.91562527591095488 ) ) ;
#72088=CARTESIAN_POINT ( 'NONE',  ( 96.20032699425225076, -38.62430069186631698, 46.45181575210094138 ) ) ;
#72089=CARTESIAN_POINT ( 'NONE',  ( 111.7740190377046758, -28.54012605827362137, 249.5838068554168956 ) ) ;
#72090=CARTESIAN_POINT ( 'NONE',  ( 107.0664832912739968, -18.82844715994099971, 168.9256252759119832 ) ) ;
#72091=DIRECTION ( 'NONE',  ( -4.299999999999999979E-14, 1.000000000000000000, 0.000000000000000000 ) ) ;
#72092=CARTESIAN_POINT ( 'NONE',  ( 114.5275249938671465, -28.57771476791114296, 150.4746728949579619 ) ) ;
#72093=FACE_OUTER_BOUND ( 'NONE', #82378, .T. ) ;
#72099=ADVANCED_FACE ( 'NONE', ( #52801 ), #80575, .T. ) ;
#72101=VECTOR ( 'NONE', #20403, 1000.000000000000000 ) ;
#72103=CARTESIAN_POINT ( 'NONE',  ( 97.43481369731881614, -33.83398838518805007, 132.0936288413114141 ) ) ;
#72104=CARTESIAN_POINT ( 'NONE',  ( 103.4771249150381749, -25.43533399052049049, 55.32133956162594046 ) ) ;
#72106=DIRECTION ( 'NONE',  ( 0.000000000000000000, 0.000000000000000000, 1.000000000000000000 ) ) ;
#72107=CARTESIAN_POINT ( 'NONE',  ( 112.0659116278142164, -45.48839625744306403, 73.98979194306805596 ) ) ;
#72108=CARTESIAN_POINT ( 'NONE',  ( 116.6363502066643321, -38.74961609181406175, 63.66133956162595098 ) ) ;
#72110=CARTESIAN_POINT ( 'NONE',  ( 117.0023065291008066, -39.93004192841230804, 154.5784824187679476 ) ) ;
#72113=EDGE_LOOP ( 'NONE', ( #20304, #24793, #69734, #10780 ) ) ;
#72115=CARTESIAN_POINT ( 'NONE',  ( 22.49541547940852126, 22.69262065192448574, 328.6381252759109088 ) ) ;
#72117=FACE_OUTER_BOUND ( 'NONE', #46489, .T. ) ;
#72119=CARTESIAN_POINT ( 'NONE',  ( 117.2401079361024898, -34.25881411750412298, 209.0156252759109634 ) ) ;
#72120=ORIENTED_EDGE ( 'NONE', *, *, #48527, .T. ) ;
#72121=CIRCLE ( 'NONE', #56138, 9.999999999999998224 ) ;
#72122=CARTESIAN_POINT ( 'NONE',  ( 97.80799470936521800, -40.50839083839967714, 146.6348481252984755 ) ) ;
#72123=CARTESIAN_POINT ( 'NONE',  ( 96.22678813199759418, -34.45212096497557042, 257.1737205140064475 ) ) ;
#72124=CARTESIAN_POINT ( 'NONE',  ( 104.2021517265174992, -25.17926459036136322, 86.26991099019699050 ) ) ;
#72126=CARTESIAN_POINT ( 'NONE',  ( 97.81399931465544739, -40.51646775427786196, 252.6355816051047896 ) ) ;
#72127=CARTESIAN_POINT ( 'NONE',  ( 63.03715912545646205, -24.42818131006026761, 116.4678068554151054 ) ) ;
#72128=DIRECTION ( 'NONE',  ( 1.000000000000000078E-15, -1.000000000000000000, 0.000000000000000000 ) ) ;
#72129=CARTESIAN_POINT ( 'NONE',  ( 117.0720556136961648, -35.46381013733837051, 264.9274461759231372 ) ) ;
#72132=VECTOR ( 'NONE', #66402, 1000.000000000000000 ) ;
#72133=VECTOR ( 'NONE', #4917, 1000.000000000000000 ) ;
#72134=AXIS2_PLACEMENT_3D ( 'NONE', #65135, #84711, #78345 ) ;
#72136=ORIENTED_EDGE ( 'NONE', *, *, #7082, .F. ) ;
#72137=VERTEX_POINT ( 'NONE', #12877 ) ;
#72139=CARTESIAN_POINT ( 'NONE',  ( 111.4803918977840169, -26.59589994751270936, 280.7375300378156453 ) ) ;
#72140=DIRECTION ( 'NONE',  ( 0.8571673007021115565, -0.5150380749100554878, 7.521945815882500121E-16 ) ) ;
#72141=DIRECTION ( 'NONE',  ( 0.000000000000000000, 0.000000000000000000, -1.000000000000000000 ) ) ;
#72143=VECTOR ( 'NONE', #84693, 1000.000000000000114 ) ;
#72144=DIRECTION ( 'NONE',  ( 1.000000000000000078E-15, -1.000000000000000000, 0.000000000000000000 ) ) ;
#72147=TOROIDAL_SURFACE ( 'NONE', #40212, 15.69999999999999929, 0.2999999999999999889 ) ;
#72148=CARTESIAN_POINT ( 'NONE',  ( 113.5483862797134549, -30.40508126489656604, 193.8762293518859678 ) ) ;
#72149=VERTEX_POINT ( 'NONE', #40105 ) ;
#72150=ORIENTED_EDGE ( 'NONE', *, *, #60276, .F. ) ;
#72151=ORIENTED_EDGE ( 'NONE', *, *, #25161, .F. ) ;
#72152=FACE_OUTER_BOUND ( 'NONE', #19848, .T. ) ;
#72153=CARTESIAN_POINT ( 'NONE',  ( 48.45959712127140051, -26.00627455219179751, 193.9678068554150911 ) ) ;
#72154=CARTESIAN_POINT ( 'NONE',  ( 96.91794407517411969, -34.59732685048010126, 257.1737205140059928 ) ) ;
#72155=EDGE_CURVE ( 'NONE', #77070, #5714, #67822, .T. ) ;
#72156=CARTESIAN_POINT ( 'NONE',  ( 172.5667039024478129, -36.32844715993500273, 300.4678068554149490 ) ) ;
#72157=EDGE_CURVE ( 'NONE', #34504, #43897, #54608, .T. ) ;
#72158=FACE_OUTER_BOUND ( 'NONE', #63349, .T. ) ;
#72159=DIRECTION ( 'NONE',  ( 0.000000000000000000, 0.000000000000000000, -1.000000000000000000 ) ) ;
#72161=EDGE_CURVE ( 'NONE', #18505, #69050, #565, .T. ) ;
#72162=CARTESIAN_POINT ( 'NONE',  ( 78.82300719538731926, -34.27587548317108457, 1.868342134763057549 ) ) ;
#72163=ORIENTED_EDGE ( 'NONE', *, *, #75229, .F. ) ;
#72164=DIRECTION ( 'NONE',  ( 9.351236661543306751E-17, -3.725950533538267725E-29, -1.000000000000000000 ) ) ;
#72165=CARTESIAN_POINT ( 'NONE',  ( 106.4288663150950214, -28.56390168778064975, 22.95666179816197072 ) ) ;
#72172=PLANE ( 'NONE',  #65341 ) ;
#72173=DIRECTION ( 'NONE',  ( 1.000000000000000000, 0.000000000000000000, 0.000000000000000000 ) ) ;
#72174=ORIENTED_EDGE ( 'NONE', *, *, #76847, .F. ) ;
#72175=CARTESIAN_POINT ( 'NONE',  ( 115.2074362016368099, -44.20634311780637660, 78.22324432352995416 ) ) ;
#72177=CARTESIAN_POINT ( 'NONE',  ( 101.6136182267745056, -30.15507309768812050, 40.04956268521897300 ) ) ;
#72178=CARTESIAN_POINT ( 'NONE',  ( 114.6397582406955422, -43.29253298239483172, 89.25751118873346002 ) ) ;
#72179=CARTESIAN_POINT ( 'NONE',  ( 109.2913206311583707, -45.85778897805103327, 84.18634521065892784 ) ) ;
#72180=CARTESIAN_POINT ( 'NONE',  ( 109.6420608605809406, -46.48032619938765464, 13.78138133162124568 ) ) ;
#72182=CIRCLE ( 'NONE', #33008, 13.44999999999999396 ) ;
#72184=CARTESIAN_POINT ( 'NONE',  ( 101.5975885682485398, -47.27054607199826819, 13.19562527591094891 ) ) ;
#72187=DIRECTION ( 'NONE',  ( 0.9825752044328147639, 0.1858654557302462929, 0.000000000000000000 ) ) ;
#72190=CARTESIAN_POINT ( 'NONE',  ( 114.2834173682332732, -44.31288860877327807, 154.1813395616249807 ) ) ;
#72191=AXIS2_PLACEMENT_3D ( 'NONE', #63313, #71039, #29248 ) ;
#72193=EDGE_LOOP ( 'NONE', ( #4978, #67910, #76518, #61610 ) ) ;
#72194=VERTEX_POINT ( 'NONE', #33751 ) ;
#72195=CARTESIAN_POINT ( 'NONE',  ( 33.91903122894598965, -35.91149509761181235, -5.074374724088000832 ) ) ;
#72196=CIRCLE ( 'NONE', #40481, 2.117000000000000881 ) ;
#72197=CARTESIAN_POINT ( 'NONE',  ( 25.56670390244797275, -65.37844715994100397, 298.0928068554150627 ) ) ;
#72198=CARTESIAN_POINT ( 'NONE',  ( 117.1144258088630750, -31.97015794161411861, 214.1784824187679419 ) ) ;
#72199=DIRECTION ( 'NONE',  ( 0.000000000000000000, 1.000000000000000000, 0.000000000000000000 ) ) ;
#72200=CYLINDRICAL_SURFACE ( 'NONE', #8955, 2.116999999999993776 ) ;
#72201=DIRECTION ( 'NONE',  ( 4.194175870806139918E-14, -1.000000000000000000, 0.000000000000000000 ) ) ;
#72202=CARTESIAN_POINT ( 'NONE',  ( 96.83360046493686468, -38.89957200400883863, 27.49276813305395706 ) ) ;
#72203=DIRECTION ( 'NONE',  ( -1.000000000000000078E-15, 1.000000000000000000, 0.000000000000000000 ) ) ;
#72204=ORIENTED_EDGE ( 'NONE', *, *, #12811, .F. ) ;
#72205=AXIS2_PLACEMENT_3D ( 'NONE', #85309, #50757, #38025 ) ;
#72206=CARTESIAN_POINT ( 'NONE',  ( 97.33770338515772380, -34.07162276509023258, 172.1147621535543806 ) ) ;
#72207=VECTOR ( 'NONE', #61416, 1000.000000000000000 ) ;
#72210=EDGE_CURVE ( 'NONE', #65745, #58445, #75433, .T. ) ;
#72212=VECTOR ( 'NONE', #4448, 1000.000000000000000 ) ;
#72214=LINE ( 'NONE', #38561, #54173 ) ;
#72215=CARTESIAN_POINT ( 'NONE',  ( 95.31970492887376167, -38.09378048407036488, 236.4184824187679510 ) ) ;
#72217=FACE_OUTER_BOUND ( 'NONE', #51731, .T. ) ;
#72218=PLANE ( 'NONE',  #57713 ) ;
#72219=CARTESIAN_POINT ( 'NONE',  ( 115.8412394166662835, -32.57321297090945933, 213.6009912566489675 ) ) ;
#72221=CARTESIAN_POINT ( 'NONE',  ( 107.6057229598026197, -48.54288983744045538, 38.61276813305397582 ) ) ;
#72223=CARTESIAN_POINT ( 'NONE',  ( 114.1106629025095458, -44.52247787522302502, 133.1613395616249989 ) ) ;
#72225=CARTESIAN_POINT ( 'NONE',  ( 25.56670390244797275, -58.35344715994099829, 254.4678068554150343 ) ) ;
#72226=VERTEX_POINT ( 'NONE', #89171 ) ;
#72228=CARTESIAN_POINT ( 'NONE',  ( 72.31648329127401098, -45.72944715994106701, 14.92562527591093691 ) ) ;
#72229=CARTESIAN_POINT ( 'NONE',  ( 108.6469982457124104, -26.82183733066701237, 275.9507284248297765 ) ) ;
#72230=ORIENTED_EDGE ( 'NONE', *, *, #19235, .T. ) ;
#72231=DIRECTION ( 'NONE',  ( 0.000000000000000000, 0.000000000000000000, 1.000000000000000000 ) ) ;
#72232=VERTEX_POINT ( 'NONE', #6488 ) ;
#72234=DIRECTION ( 'NONE',  ( 0.000000000000000000, 0.000000000000000000, -1.000000000000000000 ) ) ;
#72235=AXIS2_PLACEMENT_3D ( 'NONE', #56006, #70569, #56467 ) ;
#72236=CARTESIAN_POINT ( 'NONE',  ( 88.17226027475707895, -14.72944715994102616, 249.5838068554175777 ) ) ;
#72237=ORIENTED_EDGE ( 'NONE', *, *, #12167, .F. ) ;
#72239=CARTESIAN_POINT ( 'NONE',  ( 110.1645224859485808, -46.70684747839494833, 97.81562527591097478 ) ) ;
#72241=CARTESIAN_POINT ( 'NONE',  ( 97.12558202918494032, -37.99705770278674066, 166.4273231845742487 ) ) ;
#72242=DIRECTION ( 'NONE',  ( 1.000000000000000000, 4.163336342344333240E-14, 0.000000000000000000 ) ) ;
#72243=CARTESIAN_POINT ( 'NONE',  ( 97.81169952324414396, -40.51743120087827776, 141.6355106266202313 ) ) ;
#72248=ORIENTED_CLOSED_SHELL ( 'NONE', *, #1014, .F. );
#72249=AXIS2_PLACEMENT_3D ( 'NONE', #73539, #65824, #17252 ) ;
#72252=DIRECTION ( 'NONE',  ( 0.000000000000000000, 0.000000000000000000, 1.000000000000000000 ) ) ;
#72253=VECTOR ( 'NONE', #27437, 999.9999999999998863 ) ;
#72255=VECTOR ( 'NONE', #50429, 1000.000000000000000 ) ;
#72257=CARTESIAN_POINT ( 'NONE',  ( 164.9190312289449878, -35.91149509761181235, 117.4678068554150627 ) ) ;
#72258=CARTESIAN_POINT ( 'NONE',  ( 97.98063455390173715, -41.72806076336409120, 172.7146728949579710 ) ) ;
#72260=LINE ( 'NONE', #64106, #8081 ) ;
#72261=ORIENTED_EDGE ( 'NONE', *, *, #66836, .F. ) ;
#72263=CARTESIAN_POINT ( 'NONE',  ( 106.6352542858682284, -26.36832623700844280, 36.09753003781596448 ) ) ;
#72264=LINE ( 'NONE', #1880, #65764 ) ;
#72266=EDGE_CURVE ( 'NONE', #28799, #6003, #29012, .T. ) ;
#72267=LINE ( 'NONE', #30479, #18107 ) ;
#72268=AXIS2_PLACEMENT_3D ( 'NONE', #75274, #34367, #82996 ) ;
#72269=ORIENTED_EDGE ( 'NONE', *, *, #77180, .F. ) ;
#72271=EDGE_CURVE ( 'NONE', #33917, #58383, #26941, .T. ) ;
#72272=AXIS2_PLACEMENT_3D ( 'NONE', #28580, #84476, #1792 ) ;
#72273=CARTESIAN_POINT ( 'NONE',  ( 110.0587659310071729, -27.38278898179161658, 234.8299109901969643 ) ) ;
#72274=EDGE_LOOP ( 'NONE', ( #42106, #36971, #11389, #79469 ) ) ;
#72275=ORIENTED_EDGE ( 'NONE', *, *, #26955, .F. ) ;
#72276=CARTESIAN_POINT ( 'NONE',  ( 112.7482059764288778, -43.52991081625548020, 189.5615833058969883 ) ) ;
#72277=CARTESIAN_POINT ( 'NONE',  ( 127.1498166246059753, 12.92155284005802862, 355.9756252759109998 ) ) ;
#72278=CARTESIAN_POINT ( 'NONE',  ( 111.4141554795631492, -28.97316737322958957, 31.10158330589696263 ) ) ;
#72280=PLANE ( 'NONE',  #43135 ) ;
#72283=VERTEX_POINT ( 'NONE', #75545 ) ;
#72286=EDGE_CURVE ( 'NONE', #82640, #35753, #75982, .T. ) ;
#72288=CARTESIAN_POINT ( 'NONE',  ( 112.4780167374716058, -46.34085331822173970, 257.9965776568635647 ) ) ;
#72289=CARTESIAN_POINT ( 'NONE',  ( 116.3212776292303090, -32.94146857471486811, 175.1356252759109680 ) ) ;
#72290=EDGE_LOOP ( 'NONE', ( #43818, #70719 ) ) ;
#72291=CARTESIAN_POINT ( 'NONE',  ( 115.0372575036200828, -42.90846257047583379, 83.30229194220611078 ) ) ;
#72295=CIRCLE ( 'NONE', #54876, 4.750000000000004441 ) ;
#72296=AXIS2_PLACEMENT_3D ( 'NONE', #45796, #59876, #65808 ) ;
#72297=CARTESIAN_POINT ( 'NONE',  ( 112.2265052985635236, -45.83807782717671131, 208.9870538473389558 ) ) ;
#72300=CARTESIAN_POINT ( 'NONE',  ( 97.31101637507774171, -32.83472251844465717, 37.02419670448292521 ) ) ;
#72301=CARTESIAN_POINT ( 'NONE',  ( 20.03715912545637678, -24.42818131006202265, 193.9678068554150627 ) ) ;
#72302=CARTESIAN_POINT ( 'NONE',  ( 109.2120108049357299, -48.38436871983039111, 277.7213395616254843 ) ) ;
#72304=CARTESIAN_POINT ( 'NONE',  ( 82.41744075321345520, -17.29868422067037770, 2.608896314050102472 ) ) ;
#72306=CARTESIAN_POINT ( 'NONE',  ( 62.03742497533745137, -23.42844715994041849, 313.9678068554150059 ) ) ;
#72307=CARTESIAN_POINT ( 'NONE',  ( 102.9084262957273097, -29.13922403623678292, 98.28142370292496821 ) ) ;
#72308=CARTESIAN_POINT ( 'NONE',  ( 103.2957022058525780, -26.98683617215391806, 211.3699109901969848 ) ) ;
#72309=CARTESIAN_POINT ( 'NONE',  ( 77.31648329127398256, -18.72944715994106346, 14.92562527591094046 ) ) ;
#72311=ORIENTED_EDGE ( 'NONE', *, *, #1919, .T. ) ;
#72312=FACE_OUTER_BOUND ( 'NONE', #30056, .T. ) ;
#72314=ORIENTED_EDGE ( 'NONE', *, *, #39133, .F. ) ;
#72316=CIRCLE ( 'NONE', #33141, 5.800000000000000711 ) ;
#72317=VECTOR ( 'NONE', #29790, 999.9999999999998863 ) ;
#72320=VERTEX_POINT ( 'NONE', #55058 ) ;
#72321=CARTESIAN_POINT ( 'NONE',  ( 163.0664832912739826, 25.62155284005901379, 333.4006252759110112 ) ) ;
#72322=EDGE_CURVE ( 'NONE', #62403, #30864, #50784, .T. ) ;
#72323=CARTESIAN_POINT ( 'NONE',  ( 115.0870504499182374, -30.61523282038012184, 24.34419833761608487 ) ) ;
#72324=CARTESIAN_POINT ( 'NONE',  ( 97.81853004928629503, -39.68680891125094234, 130.9952769709339577 ) ) ;
#72325=CARTESIAN_POINT ( 'NONE',  ( 114.8522965031571630, -43.72857415363870359, 38.24419670448192221 ) ) ;
#72327=CARTESIAN_POINT ( 'NONE',  ( 172.5664832912740110, -36.32844715994070839, 263.6756252759120116 ) ) ;
#72329=AXIS2_PLACEMENT_3D ( 'NONE', #31138, #3444, #3001 ) ;
#72330=CARTESIAN_POINT ( 'NONE',  ( 116.3168070826688876, -32.94156582961523583, 135.1356252759109680 ) ) ;
#72332=LINE ( 'NONE', #57335, #33398 ) ;
#72333=VECTOR ( 'NONE', #58035, 999.9999999999998863 ) ;
#72334=PLANE ( 'NONE',  #3779 ) ;
#72335=CARTESIAN_POINT ( 'NONE',  ( 37.06648329127298780, 12.92155284005730387, 355.9756252759109998 ) ) ;
#72336=DIRECTION ( 'NONE',  ( 1.000000000000000078E-15, -1.000000000000000083E-30, -1.000000000000000000 ) ) ;
#72337=ORIENTED_EDGE ( 'NONE', *, *, #27025, .F. ) ;
#72338=EDGE_CURVE ( 'NONE', #11985, #25266, #31902, .T. ) ;
#72340=CARTESIAN_POINT ( 'NONE',  ( 105.1090048964814940, -25.85068961359000284, 275.2061014663871674 ) ) ;
#72341=CARTESIAN_POINT ( 'NONE',  ( 95.20983985305964836, -35.71400682071400468, 32.25848241876794020 ) ) ;
#72342=CARTESIAN_POINT ( 'NONE',  ( 117.0608945233633165, -38.08045312270508731, 119.7189586090938036 ) ) ;
#72343=CARTESIAN_POINT ( 'NONE',  ( 151.0371591254575208, -24.42818131005592264, 180.4678068554149775 ) ) ;
#72345=DIRECTION ( 'NONE',  ( -0.8571673007021110013, 1.917331853055865018E-16, 0.5150380749100563760 ) ) ;
#72346=CYLINDRICAL_SURFACE ( 'NONE', #263, 3.299999999999997158 ) ;
#72347=LINE ( 'NONE', #16047, #22317 ) ;
#72348=AXIS2_PLACEMENT_3D ( 'NONE', #16684, #4395, #38445 ) ;
#72349=DIRECTION ( 'NONE',  ( -0.7071067811865506814, 0.7071067811865443531, -7.071067811865500971E-16 ) ) ;
#72350=CARTESIAN_POINT ( 'NONE',  ( 131.0667039024480118, -67.87844715994100397, 213.1838068554149856 ) ) ;
#72352=EDGE_CURVE ( 'NONE', #7662, #21135, #88732, .T. ) ;
#72353=DIRECTION ( 'NONE',  ( 0.000000000000000000, 0.000000000000000000, -1.000000000000000000 ) ) ;
#72354=CARTESIAN_POINT ( 'NONE',  ( 116.5143565283028266, -32.21898467494469998, 19.18133956162493092 ) ) ;
#72355=CARTESIAN_POINT ( 'NONE',  ( 113.6144894440835031, -28.61735105040022376, 160.5356252759109736 ) ) ;
#72356=CARTESIAN_POINT ( 'NONE',  ( 103.5915305487281302, -46.58145011825330783, 53.30705384733997221 ) ) ;
#72357=LINE ( 'NONE', #45068, #84181 ) ;
#72358=CARTESIAN_POINT ( 'NONE',  ( 162.8913605087221015, -31.76306994223262947, 313.9678068554149490 ) ) ;
#72359=CARTESIAN_POINT ( 'NONE',  ( 25.56670390244808644, -42.82844715994167473, 254.7178068554150059 ) ) ;
#72360=CIRCLE ( 'NONE', #4204, 1.571100913904360796 ) ;
#72362=ORIENTED_EDGE ( 'NONE', *, *, #56232, .F. ) ;
#72363=DIRECTION ( 'NONE',  ( 1.000000000000000078E-15, 0.000000000000000000, -1.000000000000000000 ) ) ;
#72364=ORIENTED_EDGE ( 'NONE', *, *, #24762, .F. ) ;
#72365=CARTESIAN_POINT ( 'NONE',  ( 102.2761128416349692, -28.20209198692217356, 56.48419670448195973 ) ) ;
#72366=DIRECTION ( 'NONE',  ( 0.000000000000000000, 0.000000000000000000, -1.000000000000000000 ) ) ;
#72367=ORIENTED_EDGE ( 'NONE', *, *, #13480, .F. ) ;
#72368=CARTESIAN_POINT ( 'NONE',  ( 80.48314995794042659, 12.92155284005802685, 336.5756252759109657 ) ) ;
#72369=CARTESIAN_POINT ( 'NONE',  ( 96.06973772670292533, -35.87188691900273341, 187.2765776568629406 ) ) ;
#72371=CARTESIAN_POINT ( 'NONE',  ( 99.50487655220703687, -43.30595522777451123, 146.8960869441339412 ) ) ;
#72372=CARTESIAN_POINT ( 'NONE',  ( 149.4512091874902922, -60.54365471797113685, 361.9756252759100335 ) ) ;
#72373=EDGE_CURVE ( 'NONE', #47593, #29714, #39170, .T. ) ;
#72374=CARTESIAN_POINT ( 'NONE',  ( 98.34985890484145443, -31.65658482251759054, 46.90645861040638209 ) ) ;
#72375=AXIS2_PLACEMENT_3D ( 'NONE', #79170, #2855, #30555 ) ;
#72376=DIRECTION ( 'NONE',  ( -0.000000000000000000, 1.000000000000000000, 0.000000000000000000 ) ) ;
#72377=CARTESIAN_POINT ( 'NONE',  ( 97.92335910827921452, -40.78098889029146079, 96.65840926232698394 ) ) ;
#72378=CARTESIAN_POINT ( 'NONE',  ( 114.2526777242401437, -43.36435822665426087, 123.2327681330539519 ) ) ;
#72379=ORIENTED_EDGE ( 'NONE', *, *, #36290, .T. ) ;
#72380=EDGE_LOOP ( 'NONE', ( #41715, #41077, #37164, #31073 ) ) ;
#72381=AXIS2_PLACEMENT_3D ( 'NONE', #62980, #1675, #36641 ) ;
#72382=CARTESIAN_POINT ( 'NONE',  ( 99.64559906019141522, -41.57287113897975672, 98.21872616303994619 ) ) ;
#72384=CARTESIAN_POINT ( 'NONE',  ( 97.48942487598456808, -34.74365074496814998, 212.1641967044819808 ) ) ;
#72385=DIRECTION ( 'NONE',  ( 1.000000000000000000, 0.000000000000000000, 0.000000000000000000 ) ) ;
#72386=FACE_OUTER_BOUND ( 'NONE', #47566, .T. ) ;
#72390=EDGE_CURVE ( 'NONE', #75837, #61357, #9629, .T. ) ;
#72391=CIRCLE ( 'NONE', #5673, 4.750000000000000888 ) ;
#72396=CARTESIAN_POINT ( 'NONE',  ( 112.4747680694540861, -26.21285726233885427, 169.6984824187679521 ) ) ;
#72399=ADVANCED_FACE ( 'NONE', ( #16448 ), #65041, .F. ) ;
#72402=CARTESIAN_POINT ( 'NONE',  ( 104.4899545160106129, -26.97880756856109841, 151.2814586040433653 ) ) ;
#72405=DIRECTION ( 'NONE',  ( 0.000000000000000000, 0.000000000000000000, -1.000000000000000000 ) ) ;
#72406=CARTESIAN_POINT ( 'NONE',  ( 117.0608820234855756, -38.08057516226932648, 104.7189489036250762 ) ) ;
#72408=CARTESIAN_POINT ( 'NONE',  ( 117.4139541310910175, -35.45788210829842058, 193.9241967044829664 ) ) ;
#72409=LINE ( 'NONE', #31053, #19786 ) ;
#72410=EDGE_LOOP ( 'NONE', ( #60758, #83780, #57065, #21096 ) ) ;
#72411=ORIENTED_EDGE ( 'NONE', *, *, #83569, .T. ) ;
#72412=ORIENTED_EDGE ( 'NONE', *, *, #47004, .T. ) ;
#72414=CARTESIAN_POINT ( 'NONE',  ( 116.9529224355460428, -35.09431523556290244, 64.95720187668048595 ) ) ;
#72415=FACE_OUTER_BOUND ( 'NONE', #19791, .T. ) ;
#72416=CARTESIAN_POINT ( 'NONE',  ( 133.4132809338266554, -34.05633243510674646, 8.161687850942930922 ) ) ;
#72417=CARTESIAN_POINT ( 'NONE',  ( 115.9514134386872826, -36.57345012324869060, 285.2730118773255867 ) ) ;
#72418=LINE ( 'NONE', #65589, #84076 ) ;
#72420=CARTESIAN_POINT ( 'NONE',  ( 111.5136026189559715, -44.03072630541131360, 9.635625275910941312 ) ) ;
#72424=CARTESIAN_POINT ( 'NONE',  ( 112.3881417993268883, -45.21006700246557841, 113.0223899637873615 ) ) ;
#72427=EDGE_CURVE ( 'NONE', #63148, #54616, #42779, .T. ) ;
#72428=CARTESIAN_POINT ( 'NONE',  ( 105.0857350373783561, -45.56626257478142605, 26.81146744712498275 ) ) ;
#72429=CARTESIAN_POINT ( 'NONE',  ( 96.03049237414208505, -35.77952841945960216, 186.2461014663869889 ) ) ;
#72430=CARTESIAN_POINT ( 'NONE',  ( 113.8292797163802561, -28.77778007523021842, 139.5156252759109634 ) ) ;
#72431=FACE_OUTER_BOUND ( 'NONE', #12316, .T. ) ;
#72432=CARTESIAN_POINT ( 'NONE',  ( 110.7330907359209107, -26.30208074597294754, 250.8194347997206819 ) ) ;
#72433=CARTESIAN_POINT ( 'NONE',  ( 115.0374028803999238, -42.90827821187051683, 99.30364407749972600 ) ) ;
#72435=ORIENTED_EDGE ( 'NONE', *, *, #32785, .T. ) ;
#72436=VECTOR ( 'NONE', #24534, 1000.000000000000000 ) ;
#72437=VERTEX_POINT ( 'NONE', #71864 ) ;
#72438=AXIS2_PLACEMENT_3D ( 'NONE', #78496, #49852, #15809 ) ;
#72439=CARTESIAN_POINT ( 'NONE',  ( 99.25559070964938257, -29.75831933708737864, 190.7470538473399415 ) ) ;
#72440=EDGE_LOOP ( 'NONE', ( #89474, #85036, #29088, #4471, #16347 ) ) ;
#72441=ADVANCED_FACE ( 'NONE', ( #2378 ), #64157, .F. ) ;
#72442=CARTESIAN_POINT ( 'NONE',  ( 113.6146262985763258, -28.61718150614917633, 164.5356252759109736 ) ) ;
#72443=CARTESIAN_POINT ( 'NONE',  ( 162.7866693523289996, -36.02818131005891189, 342.9256252759119548 ) ) ;
#72444=DIRECTION ( 'NONE',  ( 0.000000000000000000, 0.000000000000000000, 1.000000000000000000 ) ) ;
#72445=CARTESIAN_POINT ( 'NONE',  ( 51.06648329127400388, 0.2215528400590083269, 333.4006252759110112 ) ) ;
#72447=PLANE ( 'NONE',  #33137 ) ;
#72449=CARTESIAN_POINT ( 'NONE',  ( 111.8803037788896262, -27.54327565145516488, 10.68038718067199078 ) ) ;
#72450=FACE_OUTER_BOUND ( 'NONE', #69273, .T. ) ;
#72451=CARTESIAN_POINT ( 'NONE',  ( 142.8821648370247885, -72.54478064608022692, 361.9756252759100335 ) ) ;
#72452=CARTESIAN_POINT ( 'NONE',  ( 100.9529263512021231, -28.70839242353804011, 271.5937037379645176 ) ) ;
#72453=EDGE_CURVE ( 'NONE', #3527, #39861, #4364, .T. ) ;
#72454=DIRECTION ( 'NONE',  ( 0.000000000000000000, 0.000000000000000000, 1.000000000000000000 ) ) ;
#72456=EDGE_CURVE ( 'NONE', #18132, #16891, #21474, .T. ) ;
#72458=CARTESIAN_POINT ( 'NONE',  ( 115.5237354892296793, -35.57185660929852133, 195.5838068554167535 ) ) ;
#72461=CARTESIAN_POINT ( 'NONE',  ( 136.2679348343054926, -20.38027623201341143, 7.385026757011662113 ) ) ;
#72462=CARTESIAN_POINT ( 'NONE',  ( 103.5348926201861985, -26.85948109348520418, 190.3499109901969746 ) ) ;
#72463=CARTESIAN_POINT ( 'NONE',  ( 117.0537825276303749, -31.99364369613817161, 60.19086337114898555 ) ) ;
#72464=CARTESIAN_POINT ( 'NONE',  ( 97.99904154034810233, -44.43610744809739543, 222.8870538473399563 ) ) ;
#72466=CIRCLE ( 'NONE', #56490, 0.1499999999999973577 ) ;
#72467=DIRECTION ( 'NONE',  ( -0.7071067811865758834, 0.7071067811865192621, -7.071067811865765240E-16 ) ) ;
#72468=CARTESIAN_POINT ( 'NONE',  ( 193.0371591254582881, -47.82818131005411999, 300.4678068554149490 ) ) ;
#72469=CARTESIAN_POINT ( 'NONE',  ( 97.80893753052176010, -40.51861053356429920, 37.63533870039827178 ) ) ;
#72471=LINE ( 'NONE', #57936, #68320 ) ;
#72473=CARTESIAN_POINT ( 'NONE',  ( 97.06381610791373760, -37.34192999475997254, 66.37606947914083833 ) ) ;
#72477=CARTESIAN_POINT ( 'NONE',  ( 102.7155009198991280, -28.78705314239651969, 99.88575316140996563 ) ) ;
#72479=VERTEX_POINT ( 'NONE', #29625 ) ;
#72480=CARTESIAN_POINT ( 'NONE',  ( 114.6914383512287543, -44.69963429152225132, 109.1718157521009687 ) ) ;
#72481=ADVANCED_FACE ( 'NONE', ( #57313 ), #85060, .F. ) ;
#72482=CYLINDRICAL_SURFACE ( 'NONE', #52695, 2.500000000000002220 ) ;
#72485=CARTESIAN_POINT ( 'NONE',  ( 104.4899544686384445, -26.97880758048861338, 176.2814586078853836 ) ) ;
#72486=CARTESIAN_POINT ( 'NONE',  ( 97.72045520820927322, -39.61305636501506910, 21.56419670448295278 ) ) ;
#72487=ORIENTED_EDGE ( 'NONE', *, *, #46853, .T. ) ;
#72488=VECTOR ( 'NONE', #66445, 1000.000000000000000 ) ;
#72489=ORIENTED_EDGE ( 'NONE', *, *, #28165, .T. ) ;
#72492=CARTESIAN_POINT ( 'NONE',  ( 182.0374245136140132, -23.42844715993459559, 313.9678068554149490 ) ) ;
#72494=CARTESIAN_POINT ( 'NONE',  ( 29.77381068363397887, -48.62134037875510018, 129.9678068554150627 ) ) ;
#72497=CARTESIAN_POINT ( 'NONE',  ( 97.80830042520018708, -40.50914691106578402, 52.63449809795601197 ) ) ;
#72499=CIRCLE ( 'NONE', #50767, 2.030000000000003801 ) ;
#72500=EDGE_CURVE ( 'NONE', #14741, #18083, #8723, .T. ) ;
#72502=EDGE_CURVE ( 'NONE', #65852, #73636, #49603, .T. ) ;
#72503=CARTESIAN_POINT ( 'NONE',  ( 117.0329088946583624, -32.00354160957719074, 64.19086337114899266 ) ) ;
#72504=ORIENTED_EDGE ( 'NONE', *, *, #21918, .F. ) ;
#72505=ORIENTED_EDGE ( 'NONE', *, *, #62402, .F. ) ;
#72506=EDGE_CURVE ( 'NONE', #73586, #44183, #24161, .T. ) ;
#72509=DIRECTION ( 'NONE',  ( 0.1811243268507065352, -0.9834602067307444129, 0.000000000000000000 ) ) ;
#72510=EDGE_CURVE ( 'NONE', #22204, #48918, #45459, .T. ) ;
#72511=CARTESIAN_POINT ( 'NONE',  ( 97.81170051792484799, -40.51743816602341752, 61.63542871443850402 ) ) ;
#72512=CARTESIAN_POINT ( 'NONE',  ( 100.0846959373945566, -41.84369885408329992, 104.6357094172109470 ) ) ;
#72513=AXIS2_PLACEMENT_3D ( 'NONE', #1174, #70664, #62490 ) ;
#72514=CIRCLE ( 'NONE', #33328, 2.517500000000005844 ) ;
#72515=CARTESIAN_POINT ( 'NONE',  ( 51.06648329127400388, -0.2185775633790978945, 335.9181252759120184 ) ) ;
#72517=EDGE_LOOP ( 'NONE', ( #47695, #23682, #23168, #55167 ) ) ;
#72518=ORIENTED_EDGE ( 'NONE', *, *, #48110, .F. ) ;
#72521=ORIENTED_EDGE ( 'NONE', *, *, #68228, .T. ) ;
#72523=CARTESIAN_POINT ( 'NONE',  ( 107.4908894006829172, -46.11541567637532069, 189.0320594963729661 ) ) ;
#72525=AXIS2_PLACEMENT_3D ( 'NONE', #56077, #35652, #55170 ) ;
#72526=CARTESIAN_POINT ( 'NONE',  ( 112.1306244020896941, -47.47080300746646486, 133.9270538473399768 ) ) ;
#72527=DIRECTION ( 'NONE',  ( 0.000000000000000000, 0.000000000000000000, 1.000000000000000000 ) ) ;
#72528=CARTESIAN_POINT ( 'NONE',  ( 98.15099476832955361, -41.26164693790821048, 16.70074034222754733 ) ) ;
#72530=ORIENTED_EDGE ( 'NONE', *, *, #47718, .F. ) ;
#72531=ORIENTED_EDGE ( 'NONE', *, *, #50469, .F. ) ;
#72533=CARTESIAN_POINT ( 'NONE',  ( 112.5929834642309117, -30.72215809952430376, 197.3023760838769647 ) ) ;
#72534=CARTESIAN_POINT ( 'NONE',  ( 106.9270552135175620, -26.24760940922973163, 60.08705384733897858 ) ) ;
#72535=ORIENTED_EDGE ( 'NONE', *, *, #52027, .T. ) ;
#72536=CARTESIAN_POINT ( 'NONE',  ( 116.3681181406587370, -31.99193570193495262, 44.20133956162491984 ) ) ;
#72537=CYLINDRICAL_SURFACE ( 'NONE', #31237, 2.117000000000007987 ) ;
#72538=CARTESIAN_POINT ( 'NONE',  ( 172.5667039024480118, -36.32844715993499563, 193.9678068554150059 ) ) ;
#72540=CARTESIAN_POINT ( 'NONE',  ( 117.0231160686283687, -39.93674523842013713, 154.5784824187679476 ) ) ;
#72541=CARTESIAN_POINT ( 'NONE',  ( 116.8171228658513741, -34.15291831898669273, 264.0314586093876414 ) ) ;
#72543=CARTESIAN_POINT ( 'NONE',  ( 179.1667039024460166, -28.27351298637280408, -5.074374724088000832 ) ) ;
#72545=CARTESIAN_POINT ( 'NONE',  ( 167.2371591254545535, -47.82818131005522133, 129.9678068554149775 ) ) ;
#72547=VECTOR ( 'NONE', #34949, 1000.000000000000000 ) ;
#72548=ORIENTED_EDGE ( 'NONE', *, *, #49696, .F. ) ;
#72549=DIRECTION ( 'NONE',  ( 0.9068632946707805287, -0.4214249218767882055, 8.839355291601567287E-16 ) ) ;
#72551=CARTESIAN_POINT ( 'NONE',  ( 107.3210346550871179, -25.67891364084480799, 75.04610146638695767 ) ) ;
#72552=CARTESIAN_POINT ( 'NONE',  ( 32.16397622746000451, -34.03355364505800651, -5.074374724088000832 ) ) ;
#72555=CARTESIAN_POINT ( 'NONE',  ( 98.30753419713312269, -41.72887550236994514, 72.73979194360303779 ) ) ;
#72557=CARTESIAN_POINT ( 'NONE',  ( 115.5638989210038119, -29.55965564860105843, 74.38419670448293175 ) ) ;
#72558=PLANE ( 'NONE',  #5591 ) ;
#72559=CARTESIAN_POINT ( 'NONE',  ( 117.2701380961605651, -34.52720868313124924, 179.9956252759109532 ) ) ;
#72561=LINE ( 'NONE', #23533, #80105 ) ;
#72562=VERTEX_POINT ( 'NONE', #31397 ) ;
#72563=CARTESIAN_POINT ( 'NONE',  ( 25.56670390244744695, -48.82844715994178841, 173.2178068554150627 ) ) ;
#72564=ADVANCED_FACE ( 'NONE', ( #25484 ), #58649, .T. ) ;
#72565=DIRECTION ( 'NONE',  ( -0.000000000000000000, -0.000000000000000000, -1.000000000000000000 ) ) ;
#72566=DIRECTION ( 'NONE',  ( -3.360405532702990443E-14, 1.000000000000000000, 0.000000000000000000 ) ) ;
#72567=AXIS2_PLACEMENT_3D ( 'NONE', #37384, #52306, #59149 ) ;
#72570=CARTESIAN_POINT ( 'NONE',  ( 113.1256532486054880, -46.02994946121840769, 223.0480062282919675 ) ) ;
#72572=CARTESIAN_POINT ( 'NONE',  ( 116.3212776292272537, -32.94146857470742162, 144.1356252759109680 ) ) ;
#72573=CARTESIAN_POINT ( 'NONE',  ( 117.5131067102741582, -36.80237174509009179, 259.8213395616249386 ) ) ;
#72574=CARTESIAN_POINT ( 'NONE',  ( 98.42032043187158763, -42.69450228079005427, 122.8070538473389490 ) ) ;
#72575=CARTESIAN_POINT ( 'NONE',  ( 164.9212702847350158, -29.73316016639540749, -5.074374724088000832 ) ) ;
#72576=CARTESIAN_POINT ( 'NONE',  ( 82.31791107858728651, -38.31136518418592374, 7.339178645746792462 ) ) ;
#72577=CARTESIAN_POINT ( 'NONE',  ( 51.56670390244899238, -32.29483332968450782, 342.9256252759119548 ) ) ;
#72578=CARTESIAN_POINT ( 'NONE',  ( 180.2143765759489895, -35.91149509761070391, 117.4678068554150627 ) ) ;
#72579=EDGE_LOOP ( 'NONE', ( #87296, #3817, #60292, #64436 ) ) ;
#72580=CIRCLE ( 'NONE', #76908, 3.299999999999999822 ) ;
#72581=ADVANCED_FACE ( 'NONE', ( #18672 ), #45022, .F. ) ;
#72582=ORIENTED_EDGE ( 'NONE', *, *, #45303, .F. ) ;
#72585=VECTOR ( 'NONE', #22721, 1000.000000000000000 ) ;
#72587=DIRECTION ( 'NONE',  ( 3.999999999999999995E-14, -1.000000000000000000, 4.100000000000000342E-29 ) ) ;
#72588=CARTESIAN_POINT ( 'NONE',  ( 96.97881741550158097, -39.36031858868991407, 272.5299109901966972 ) ) ;
#72590=DIRECTION ( 'NONE',  ( 0.7071067812158990940, 0.7071067811571960515, 0.000000000000000000 ) ) ;
#72595=DIRECTION ( 'NONE',  ( 0.000000000000000000, 0.000000000000000000, 1.000000000000000000 ) ) ;
#72596=CARTESIAN_POINT ( 'NONE',  ( 101.7992505034292350, -28.57304559719056058, 219.9552769709339657 ) ) ;
#72597=ORIENTED_EDGE ( 'NONE', *, *, #11015, .F. ) ;
#72599=EDGE_LOOP ( 'NONE', ( #73629, #35872 ) ) ;
#72602=CARTESIAN_POINT ( 'NONE',  ( 110.8602461355434912, -45.98187261348512322, 182.8861217718651915 ) ) ;
#72603=DIRECTION ( 'NONE',  ( 1.000000000000000000, 1.261617073437676668E-15, 9.462128050782575008E-16 ) ) ;
#72604=CARTESIAN_POINT ( 'NONE',  ( 95.96284676697312932, -37.29622633765301032, 267.3670538473388092 ) ) ;
#72605=AXIS2_PLACEMENT_3D ( 'NONE', #87383, #19236, #88295 ) ;
#72607=CARTESIAN_POINT ( 'NONE',  ( 193.0374249753374443, -23.42844715993432558, 313.9678068554149490 ) ) ;
#72608=CYLINDRICAL_SURFACE ( 'NONE', #63427, 9.999999999999998224 ) ;
#72609=ORIENTED_EDGE ( 'NONE', *, *, #33229, .T. ) ;
#72610=PLANE ( 'NONE',  #57861 ) ;
#72613=VECTOR ( 'NONE', #59410, 1000.000000000000000 ) ;
#72614=LINE ( 'NONE', #10377, #78617 ) ;
#72615=CARTESIAN_POINT ( 'NONE',  ( 100.8629568432159260, -42.03472619363567730, 29.70809036959193250 ) ) ;
#72616=CARTESIAN_POINT ( 'NONE',  ( 80.06648329127399677, -18.72944715994105991, -5.074374724089057764 ) ) ;
#72617=DIRECTION ( 'NONE',  ( -0.9825752044165969590, -0.1858654558159821002, 0.000000000000000000 ) ) ;
#72618=CYLINDRICAL_SURFACE ( 'NONE', #41498, 1.000000000000000888 ) ;
#72620=CARTESIAN_POINT ( 'NONE',  ( 50.56670390244696733, -18.82844715994099971, 330.9332325604117955 ) ) ;
#72622=ORIENTED_EDGE ( 'NONE', *, *, #78150, .F. ) ;
#72623=CARTESIAN_POINT ( 'NONE',  ( 96.79149040999978126, -38.49340627261485537, 91.46133956162493917 ) ) ;
#72624=ORIENTED_EDGE ( 'NONE', *, *, #63540, .F. ) ;
#72625=CARTESIAN_POINT ( 'NONE',  ( 114.1180452634077369, -42.41171291218270767, 42.69718173283898466 ) ) ;
#72628=CARTESIAN_POINT ( 'NONE',  ( 104.6418561626188364, -26.95233673609813962, 86.70158330589694629 ) ) ;
#72630=CARTESIAN_POINT ( 'NONE',  ( 99.04396218797715790, -42.84110790024666926, 12.84394456308144328 ) ) ;
#72632=CARTESIAN_POINT ( 'NONE',  ( 90.06648329127389729, -36.72944715993924802, 14.92562527591095289 ) ) ;
#72633=CARTESIAN_POINT ( 'NONE',  ( 101.3723308891022157, -27.97080072976544685, 21.53562527591096298 ) ) ;
#72634=VECTOR ( 'NONE', #84539, 1000.000000000000000 ) ;
#72635=DIRECTION ( 'NONE',  ( 0.000000000000000000, 1.000000000000000000, 0.000000000000000000 ) ) ;
#72636=EDGE_LOOP ( 'NONE', ( #60531, #86259, #69072, #15813 ) ) ;
#72641=VERTEX_POINT ( 'NONE', #10957 ) ;
#72643=CIRCLE ( 'NONE', #79917, 1.000000000000000888 ) ;
#72645=CARTESIAN_POINT ( 'NONE',  ( 112.7271506738796347, -45.41826929060063378, 223.0480062282919675 ) ) ;
#72646=CARTESIAN_POINT ( 'NONE',  ( 107.4535518903492033, -26.65157354815539748, 125.0442608526201838 ) ) ;
#72648=CARTESIAN_POINT ( 'NONE',  ( 109.9110140596799425, -46.79572638734455126, 68.79562527591099297 ) ) ;
#72651=CARTESIAN_POINT ( 'NONE',  ( 99.09516693519820763, -30.55115414915417560, 171.8022944752187016 ) ) ;
#72652=CARTESIAN_POINT ( 'NONE',  ( 184.5667039024480118, -67.87844715994100397, 300.9178068554150514 ) ) ;
#72653=ORIENTED_EDGE ( 'NONE', *, *, #4444, .F. ) ;
#72654=B_SPLINE_CURVE_WITH_KNOTS ( 'NONE', 3,
 ( #63581, #77217, #22256, #7716, #83143, #35406, #63124, #70397, #62676, #64033, #1811, #55835, #451, #28143, #1360, #29509, #57191, #304, #89809, #54790, #41173, #82555, #60720, #19403, #40287, #83427, #20316, #34363 ),
 .UNSPECIFIED., .F., .F.,
 ( 4, 2, 2, 2, 2, 2, 2, 2, 2, 2, 2, 2, 2, 4 ),
 ( 0.5000628611168262960, 0.5625550034772225372, 0.6250471458376188894, 0.6875392881980151305, 0.7187853593782136397, 0.7500314305584121488, 0.7812775017386106580, 0.8125235729188091671, 0.8437696440990075653, 0.8750157152792059634, 0.9062617864594044725, 0.9375078576396029817, 0.9687539288198014908, 1.000000000000000000 ),
 .UNSPECIFIED. ) ;
#72655=DIRECTION ( 'NONE',  ( 0.000000000000000000, 1.000000000000000000, 0.000000000000000000 ) ) ;
#72656=CARTESIAN_POINT ( 'NONE',  ( 134.0664832912739826, -18.72944715994100306, -5.074374724089001809 ) ) ;
#72657=CARTESIAN_POINT ( 'NONE',  ( 115.4423046205436947, -29.55243945206539280, 229.4022919425779605 ) ) ;
#72658=CARTESIAN_POINT ( 'NONE',  ( 48.79742451362081823, -36.32844715994077944, 237.4678068554150059 ) ) ;
#72660=FACE_BOUND ( 'NONE', #60332, .T. ) ;
#72661=CARTESIAN_POINT ( 'NONE',  ( 80.06648329127401098, -39.47944715994105991, 1.625625275910943746 ) ) ;
#72663=CARTESIAN_POINT ( 'NONE',  ( 101.0745446329174655, -30.64234581064881269, 225.1181341137909442 ) ) ;
#72665=CARTESIAN_POINT ( 'NONE',  ( 102.9796410358630254, -46.29638950891617100, 88.25562527591095829 ) ) ;
#72667=CARTESIAN_POINT ( 'NONE',  ( 113.9459708190624241, -28.01821676562244789, 124.5565776568629559 ) ) ;
#72670=ORIENTED_EDGE ( 'NONE', *, *, #2635, .F. ) ;
#72673=EDGE_CURVE ( 'NONE', #82826, #11696, #24553, .T. ) ;
#72674=DIRECTION ( 'NONE',  ( 1.000000000000000000, 0.000000000000000000, 0.000000000000000000 ) ) ;
#72677=ORIENTED_EDGE ( 'NONE', *, *, #19389, .F. ) ;
#72679=ADVANCED_FACE ( 'NONE', ( #13214 ), #75882, .T. ) ;
#72681=CYLINDRICAL_SURFACE ( 'NONE', #36398, 9.999999999999998224 ) ;
#72686=ADVANCED_FACE ( 'NONE', ( #41336 ), #48591, .T. ) ;
#72688=CARTESIAN_POINT ( 'NONE',  ( 117.8983839226775387, -39.04577396070462214, 108.6708633711489824 ) ) ;
#72690=CARTESIAN_POINT ( 'NONE',  ( 97.79831359961421811, -40.48460542285404529, 166.6328045679836691 ) ) ;
#72695=EDGE_LOOP ( 'NONE', ( #26209, #79818, #37222, #73607 ) ) ;
#72696=DIRECTION ( 'NONE',  ( -1.000000000000000000, -2.756263715554006823E-15, 0.000000000000000000 ) ) ;
#72697=DIRECTION ( 'NONE',  ( -1.000000000000000000, -4.299999999999999979E-14, -1.000000000000000078E-15 ) ) ;
#72698=DIRECTION ( 'NONE',  ( 0.000000000000000000, 0.000000000000000000, 1.000000000000000000 ) ) ;
#72700=CARTESIAN_POINT ( 'NONE',  ( 116.7602698800575212, -34.01575108322786889, 250.0437193735734525 ) ) ;
#72702=LINE ( 'NONE', #16398, #79946 ) ;
#72705=CARTESIAN_POINT ( 'NONE',  ( 172.5664832912740110, -9.303447159940999356, 198.9256252759119832 ) ) ;
#72706=CARTESIAN_POINT ( 'NONE',  ( 104.7173522264389618, -47.59653351925012288, 178.4070538473389718 ) ) ;
#72707=AXIS2_PLACEMENT_3D ( 'NONE', #88067, #19461, #89865 ) ;
#72708=CARTESIAN_POINT ( 'NONE',  ( 51.27381068362099370, -23.19206098993950604, 342.9256252759119548 ) ) ;
#72710=CARTESIAN_POINT ( 'NONE',  ( 110.2470682213182300, -46.59973918892927003, 53.83657765686300678 ) ) ;
#72711=CYLINDRICAL_SURFACE ( 'NONE', #64666, 2.030000000001869864 ) ;
#72715=ORIENTED_EDGE ( 'NONE', *, *, #33758, .F. ) ;
#72716=VERTEX_POINT ( 'NONE', #74983 ) ;
#72717=EDGE_CURVE ( 'NONE', #48829, #85625, #68177, .T. ) ;
#72718=CARTESIAN_POINT ( 'NONE',  ( 102.7466871476783581, -44.50128676613118728, 183.6044404487539623 ) ) ;
#72721=DIRECTION ( 'NONE',  ( 0.7071067708032326982, 0.0001211784769794325652, 0.7071067811865484609 ) ) ;
#72723=VERTEX_POINT ( 'NONE', #20026 ) ;
#72724=CARTESIAN_POINT ( 'NONE',  ( 62.03742497533654188, -23.42844715994041493, 180.4678068554151196 ) ) ;
#72725=CARTESIAN_POINT ( 'NONE',  ( 172.5664832912729878, -27.57844715994070484, 78.92562527591199739 ) ) ;
#72727=CARTESIAN_POINT ( 'NONE',  ( 116.5858064714421829, -40.92601143571970823, 253.4956252759109532 ) ) ;
#72730=DIRECTION ( 'NONE',  ( 1.000000000000000078E-15, -1.000000000000000083E-30, -1.000000000000000000 ) ) ;
#72731=DIRECTION ( 'NONE',  ( 0.000000000000000000, 0.000000000000000000, 1.000000000000000000 ) ) ;
#72732=FACE_BOUND ( 'NONE', #58610, .T. ) ;
#72735=CARTESIAN_POINT ( 'NONE',  ( 101.3810039469494200, -45.56196318943892010, 218.1213395616249784 ) ) ;
#72736=CARTESIAN_POINT ( 'NONE',  ( 130.5667039024480118, -36.72944715994093912, 218.8274735512161158 ) ) ;
#72738=CIRCLE ( 'NONE', #33570, 2.550000000000006040 ) ;
#72740=CARTESIAN_POINT ( 'NONE',  ( 106.6049252239556608, -25.63961115983148176, 36.09753003781596448 ) ) ;
#72742=CARTESIAN_POINT ( 'NONE',  ( 106.8364329414440874, -47.15221585624544787, 272.5584824187680510 ) ) ;
#72745=CARTESIAN_POINT ( 'NONE',  ( 79.31518617683019556, -39.40257939794701514, 8.160477455080144438 ) ) ;
#72746=CARTESIAN_POINT ( 'NONE',  ( 100.8875449613382358, -44.70030174540323742, 18.05248020336808779 ) ) ;
#72748=CARTESIAN_POINT ( 'NONE',  ( 100.6392880577574687, -41.80624237711439406, 89.67666179816296790 ) ) ;
#72749=CARTESIAN_POINT ( 'NONE',  ( 97.90015701271006776, -41.74100594024375965, 217.7241967044829494 ) ) ;
#72750=VECTOR ( 'NONE', #16748, 1000.000000000000114 ) ;
#72751=DIRECTION ( 'NONE',  ( 0.000000000000000000, 0.000000000000000000, 1.000000000000000000 ) ) ;
#72754=ORIENTED_EDGE ( 'NONE', *, *, #55245, .T. ) ;
#72761=CARTESIAN_POINT ( 'NONE',  ( 104.5239601885372309, -27.05251041699375136, 41.28092177733371670 ) ) ;
#72762=ADVANCED_FACE ( 'NONE', ( #27276 ), #54951, .F. ) ;
#72763=CARTESIAN_POINT ( 'NONE',  ( 107.7867742379091567, -27.70205266993799142, 114.4476579233149636 ) ) ;
#72764=VECTOR ( 'NONE', #34098, 1000.000000000000000 ) ;
#72765=CARTESIAN_POINT ( 'NONE',  ( 97.75295786963341982, -40.54146432227403807, 11.63562527591094309 ) ) ;
#72769=EDGE_CURVE ( 'NONE', #24182, #20410, #12767, .T. ) ;
#72770=AXIS2_PLACEMENT_3D ( 'NONE', #8899, #37033, #59683 ) ;
#72771=ORIENTED_EDGE ( 'NONE', *, *, #87405, .T. ) ;
#72773=EDGE_CURVE ( 'NONE', #19408, #44789, #5505, .T. ) ;
#72774=ORIENTED_EDGE ( 'NONE', *, *, #15796, .F. ) ;
#72775=CARTESIAN_POINT ( 'NONE',  ( 102.5037471771102986, -27.80297507283301428, 166.4518860084373557 ) ) ;
#72776=CARTESIAN_POINT ( 'NONE',  ( 114.0075790447407087, -33.88846322102013175, 0.4256252759109769856 ) ) ;
#72778=DIRECTION ( 'NONE',  ( 3.999999999999999995E-14, -1.000000000000000000, 4.100000000000000342E-29 ) ) ;
#72779=ORIENTED_EDGE ( 'NONE', *, *, #40222, .T. ) ;
#72780=CARTESIAN_POINT ( 'NONE',  ( 115.0549195170180639, -30.03079676387787345, 269.3813395616251682 ) ) ;
#72781=CARTESIAN_POINT ( 'NONE',  ( 105.4141053104174830, -47.06688527371949249, 33.44991099019695469 ) ) ;
#72783=CARTESIAN_POINT ( 'NONE',  ( 162.8913605087222436, -31.76306994223276092, 313.9678068554149490 ) ) ;
#72784=FACE_OUTER_BOUND ( 'NONE', #32810, .T. ) ;
#72787=DIRECTION ( 'NONE',  ( 1.000000000000000000, 4.299999999999999979E-14, 1.000000000000000078E-15 ) ) ;
#72790=CARTESIAN_POINT ( 'NONE',  ( 97.81136857603131318, -40.51756142711754194, 161.6353372277744143 ) ) ;
#72792=CARTESIAN_POINT ( 'NONE',  ( 116.7680724212777079, -31.33574231247038355, 29.24229194257799236 ) ) ;
#72793=CARTESIAN_POINT ( 'NONE',  ( 106.4836140971313654, -24.89327890070114435, 191.1156252759109861 ) ) ;
#72794=CARTESIAN_POINT ( 'NONE',  ( 112.8297475082234484, -27.27058933724656953, 45.62895860924398761 ) ) ;
#72795=AXIS2_PLACEMENT_3D ( 'NONE', #49869, #21751, #63974 ) ;
#72796=DIRECTION ( 'NONE',  ( 0.000000000000000000, 0.000000000000000000, 1.000000000000000000 ) ) ;
#72797=CARTESIAN_POINT ( 'NONE',  ( 179.4595971212889935, -28.98061976758940617, 342.9256252759119548 ) ) ;
#72798=CARTESIAN_POINT ( 'NONE',  ( 134.0664832912740110, -36.72944715994100306, -5.074374724089001809 ) ) ;
#72801=LINE ( 'NONE', #11008, #79587 ) ;
#72803=CARTESIAN_POINT ( 'NONE',  ( 99.11394507416773081, -43.38496525699387973, 67.86895860924396118 ) ) ;
#72805=ORIENTED_EDGE ( 'NONE', *, *, #66702, .F. ) ;
#72806=CARTESIAN_POINT ( 'NONE',  ( 115.7827153205794133, -41.80297204315836268, 49.40639791532688463 ) ) ;
#72807=CARTESIAN_POINT ( 'NONE',  ( 97.11708974113240345, -41.49110554365059045, 212.6937205140059461 ) ) ;
#72808=DIRECTION ( 'NONE',  ( -1.000000000000000000, -3.999999999999999995E-14, -1.000000000000000078E-15 ) ) ;
#72809=CARTESIAN_POINT ( 'NONE',  ( 99.08981748339620310, -42.79584291293824805, 146.8439966323671513 ) ) ;
#72811=CARTESIAN_POINT ( 'NONE',  ( 163.2449138992999735, -32.11662333284611748, -5.074374724088000832 ) ) ;
#72812=DIRECTION ( 'NONE',  ( 0.7071067811739274456, -0.7071067811991676999, 0.000000000000000000 ) ) ;
#72813=FACE_OUTER_BOUND ( 'NONE', #69939, .T. ) ;
#72814=CARTESIAN_POINT ( 'NONE',  ( 96.47668441219802560, -40.11591174724604514, 131.5727681330539554 ) ) ;
#72815=ORIENTED_EDGE ( 'NONE', *, *, #79294, .T. ) ;
#72817=ADVANCED_FACE ( 'NONE', ( #62695 ), #57211, .F. ) ;
#72818=CARTESIAN_POINT ( 'NONE',  ( 97.69004538871082843, -40.41090301495324155, 93.05586902018298190 ) ) ;
#72820=DIRECTION ( 'NONE',  ( 0.7071067811865449082, 0.7071067811865501263, 7.071067811865448709E-16 ) ) ;
#72821=CARTESIAN_POINT ( 'NONE',  ( 105.2318265017784000, -27.12228994480481248, 231.2270538473389649 ) ) ;
#72822=DIRECTION ( 'NONE',  ( 0.000000000000000000, 1.000000000000000000, 0.000000000000000000 ) ) ;
#72823=DIRECTION ( 'NONE',  ( 0.000000000000000000, 1.000000000000000000, 0.000000000000000000 ) ) ;
#72824=DIRECTION ( 'NONE',  ( 0.000000000000000000, -1.000000000000000000, 0.000000000000000000 ) ) ;
#72828=PLANE ( 'NONE',  #84105 ) ;
#72830=CARTESIAN_POINT ( 'NONE',  ( 117.7567108552515265, -34.01230579303179979, 169.0365776568629599 ) ) ;
#72831=ORIENTED_EDGE ( 'NONE', *, *, #44117, .T. ) ;
#72832=AXIS2_PLACEMENT_3D ( 'NONE', #80501, #39148, #60020 ) ;
#72833=EDGE_LOOP ( 'NONE', ( #33836, #84912 ) ) ;
#72834=AXIS2_PLACEMENT_3D ( 'NONE', #37991, #29403, #37107 ) ;
#72837=CARTESIAN_POINT ( 'NONE',  ( 138.8167039024479834, -57.40094715994099772, 35.51780685541480409 ) ) ;
#72838=CARTESIAN_POINT ( 'NONE',  ( 97.81169951533574647, -40.51743117454552134, 102.6356342116286413 ) ) ;
#72840=CARTESIAN_POINT ( 'NONE',  ( 141.9629299006807344, -9.772340378754462265, -5.074374724088959177 ) ) ;
#72841=CARTESIAN_POINT ( 'NONE',  ( 103.5423316596719445, -26.88027146080960961, 190.3499109901969746 ) ) ;
#72842=CARTESIAN_POINT ( 'NONE',  ( 136.3179110785846149, -38.31136518418494319, 7.339178645749313112 ) ) ;
#72843=ORIENTED_EDGE ( 'NONE', *, *, #6641, .F. ) ;
#72844=EDGE_LOOP ( 'NONE', ( #3241, #87612, #7252, #77634 ) ) ;
#72845=ORIENTED_EDGE ( 'NONE', *, *, #17301, .T. ) ;
#72847=CARTESIAN_POINT ( 'NONE',  ( 130.5667039024479834, -36.72944715994100306, 239.5838068554162987 ) ) ;
#72848=CARTESIAN_POINT ( 'NONE',  ( 132.2214349158019502, -34.68812225915852565, 7.662832107304482498 ) ) ;
#72849=CARTESIAN_POINT ( 'NONE',  ( 110.4041361119612930, -44.93847832680074106, 279.3158690201827881 ) ) ;
#72850=EDGE_CURVE ( 'NONE', #8395, #8413, #69968, .T. ) ;
#72851=CARTESIAN_POINT ( 'NONE',  ( 50.97905606905900555, -31.62489322948711035, -5.074374724088000832 ) ) ;
#72856=VERTEX_POINT ( 'NONE', #28166 ) ;
#72857=ORIENTED_EDGE ( 'NONE', *, *, #37347, .F. ) ;
#72858=CIRCLE ( 'NONE', #48197, 1.000000000000000888 ) ;
#72860=ORIENTED_EDGE ( 'NONE', *, *, #2836, .T. ) ;
#72861=ORIENTED_EDGE ( 'NONE', *, *, #3650, .F. ) ;
#72862=CARTESIAN_POINT ( 'NONE',  ( 102.0657985602879592, -27.97123491610240720, 156.4896842834733661 ) ) ;
#72863=CARTESIAN_POINT ( 'NONE',  ( 98.56159230830689921, -41.41319107723295900, 26.14956268521895311 ) ) ;
#72864=CARTESIAN_POINT ( 'NONE',  ( 99.06899620534126427, -29.95238561887155981, 215.7670538473399517 ) ) ;
#72865=CARTESIAN_POINT ( 'NONE',  ( 102.6254653968535990, -46.82603978519644272, 132.2346728949579528 ) ) ;
#72867=CARTESIAN_POINT ( 'NONE',  ( 105.7763715259175257, -26.38449191207581634, 266.1756252759109884 ) ) ;
#72868=CARTESIAN_POINT ( 'NONE',  ( 109.6431669551641477, -46.48004783680506335, 98.78305064256221613 ) ) ;
#72869=EDGE_CURVE ( 'NONE', #628, #59432, #27638, .T. ) ;
#72872=CIRCLE ( 'NONE', #77232, 9.571100913904354357 ) ;
#72873=VERTEX_POINT ( 'NONE', #28621 ) ;
#72875=CARTESIAN_POINT ( 'NONE',  ( 115.2864439380202271, -30.18849607537921997, 244.3613395616249875 ) ) ;
#72876=ORIENTED_EDGE ( 'NONE', *, *, #67127, .T. ) ;
#72877=CARTESIAN_POINT ( 'NONE',  ( 108.0069521509713297, -26.34547698190780451, 155.0041967044819557 ) ) ;
#72880=FACE_OUTER_BOUND ( 'NONE', #47116, .T. ) ;
#72882=DIRECTION ( 'NONE',  ( 0.7071067811865473507, 0.7071067811865476838, 0.000000000000000000 ) ) ;
#72884=CARTESIAN_POINT ( 'NONE',  ( 111.7292870705843342, -27.42961193919087748, 275.7070538473395800 ) ) ;
#72885=DIRECTION ( 'NONE',  ( 0.000000000000000000, 0.000000000000000000, -1.000000000000000000 ) ) ;
#72886=LINE ( 'NONE', #31990, #72940 ) ;
#72890=DIRECTION ( 'NONE',  ( 5.512527431108029424E-15, -1.000000000000000000, 0.000000000000000000 ) ) ;
#72891=EDGE_CURVE ( 'NONE', #34937, #29192, #29975, .T. ) ;
#72893=CARTESIAN_POINT ( 'NONE',  ( 107.0664832912739968, -36.72944715994100306, 287.6356252759109680 ) ) ;
#72894=CARTESIAN_POINT ( 'NONE',  ( 98.65276261104773425, -37.10273558558598239, 195.5838068554173788 ) ) ;
#72895=VERTEX_POINT ( 'NONE', #8644 ) ;
#72897=CARTESIAN_POINT ( 'NONE',  ( 96.03049237414208505, -35.77952841945960216, 186.2461014663869889 ) ) ;
#72898=CARTESIAN_POINT ( 'NONE',  ( 111.9288574835248511, -27.50774424443475397, 55.68991099019693536 ) ) ;
#72899=CARTESIAN_POINT ( 'NONE',  ( 99.72256515790628839, -29.26889448616327982, 221.6956252759109702 ) ) ;
#72900=DIRECTION ( 'NONE',  ( 1.000000000000000078E-15, -1.000000000000000083E-30, -1.000000000000000000 ) ) ;
#72901=CARTESIAN_POINT ( 'NONE',  ( 53.56670390244828184, -48.82844715994055917, 300.4678068554150059 ) ) ;
#72902=DIRECTION ( 'NONE',  ( 0.000000000000000000, 1.000000000000000000, 0.000000000000000000 ) ) ;
#72903=CARTESIAN_POINT ( 'NONE',  ( 117.0747869972543782, -37.01281407854411043, 39.80368068565672246 ) ) ;
#72905=DIRECTION ( 'NONE',  ( -0.7071067812159698152, -0.7071067811571253303, -7.071067812159691855E-16 ) ) ;
#72906=CARTESIAN_POINT ( 'NONE',  ( 36.23715912545429063, -47.82818131006125384, 237.4678068554150059 ) ) ;
#72908=EDGE_LOOP ( 'NONE', ( #84718, #46143, #26160, #14768, #87249, #39067 ) ) ;
#72909=CARTESIAN_POINT ( 'NONE',  ( 109.5993548714604060, -44.88669505861042808, 97.23813411379100557 ) ) ;
#72912=CARTESIAN_POINT ( 'NONE',  ( 103.2867953297129873, -47.09177226061134292, 93.28610146638693834 ) ) ;
#72914=LINE ( 'NONE', #10682, #32617 ) ;
#72915=CARTESIAN_POINT ( 'NONE',  ( 108.4174892645027910, -26.73503592953050045, 175.9689586082560027 ) ) ;
#72916=CARTESIAN_POINT ( 'NONE',  ( 97.00695627739551696, -39.24785929248557892, 16.53372051400697629 ) ) ;
#72917=VERTEX_POINT ( 'NONE', #49947 ) ;
#72918=VERTEX_POINT ( 'NONE', #8188 ) ;
#72920=VECTOR ( 'NONE', #2369, 1000.000000000000000 ) ;
#72921=CARTESIAN_POINT ( 'NONE',  ( 124.9629318080292393, -56.47944715994101728, -5.074374724089012467 ) ) ;
#72922=CARTESIAN_POINT ( 'NONE',  ( 107.0664832912748068, -36.72944715993923381, -5.074374724089029343 ) ) ;
#72924=DIRECTION ( 'NONE',  ( -1.000000000000000000, -4.299999999999999979E-14, -1.000000000000000078E-15 ) ) ;
#72927=LINE ( 'NONE', #38403, #76480 ) ;
#72929=CARTESIAN_POINT ( 'NONE',  ( 99.31004196827748842, -43.71529311364911763, 56.90991099019593236 ) ) ;
#72934=CARTESIAN_POINT ( 'NONE',  ( 106.6465955684521418, -26.33791012980835333, 322.9014499992877631 ) ) ;
#72935=CARTESIAN_POINT ( 'NONE',  ( 115.4711811475381467, -34.66499115051416169, 161.8242808457819706 ) ) ;
#72936=CIRCLE ( 'NONE', #35267, 2.750000000000002665 ) ;
#72937=EDGE_CURVE ( 'NONE', #23005, #5529, #35880, .T. ) ;
#72938=EDGE_CURVE ( 'NONE', #15987, #16664, #36341, .T. ) ;
#72939=B_SPLINE_CURVE_WITH_KNOTS ( 'NONE', 3,
 ( #46229, #67595, #76997, #4923, #53936, #73964, #11742, #88942, #81694, #47127, #14779, #83817, #39440, #88051, #80795, #21134, #21591, #87596 ),
 .UNSPECIFIED., .F., .F.,
 ( 4, 2, 2, 2, 2, 2, 2, 2, 4 ),
 ( 0.4999639890268276488, 0.5624684903984742412, 0.6249729917701207782, 0.6874774931417673152, 0.7499819945134138521, 0.8124864958850603891, 0.8749909972567069261, 0.9374954986283534630, 1.000000000000000000 ),
 .UNSPECIFIED. ) ;
#72940=VECTOR ( 'NONE', #17042, 1000.000000000000000 ) ;
#72941=CARTESIAN_POINT ( 'NONE',  ( 87.31648329127403940, -54.62589567669624557, -5.074374724089048883 ) ) ;
#72942=ORIENTED_EDGE ( 'NONE', *, *, #60384, .T. ) ;
#72943=ORIENTED_EDGE ( 'NONE', *, *, #84881, .T. ) ;
#72945=DIRECTION ( 'NONE',  ( 1.000000000000000078E-15, 1.000000000000000083E-30, -1.000000000000000000 ) ) ;
#72946=ORIENTED_EDGE ( 'NONE', *, *, #42702, .T. ) ;
#72949=EDGE_CURVE ( 'NONE', #16561, #36943, #13128, .T. ) ;
#72950=CARTESIAN_POINT ( 'NONE',  ( 116.1725082674369816, -34.41496348756209755, 165.4682499725639957 ) ) ;
#72951=EDGE_CURVE ( 'NONE', #51499, #14684, #20392, .T. ) ;
#72952=CARTESIAN_POINT ( 'NONE',  ( 136.8164832912740110, -36.72944715994100306, -5.074374724088999145 ) ) ;
#72953=CARTESIAN_POINT ( 'NONE',  ( 97.81170242524891023, -40.51743837274789684, 121.6354095930283137 ) ) ;
#72955=CARTESIAN_POINT ( 'NONE',  ( 97.92338993004062786, -40.78105876605869184, 16.65841519439857876 ) ) ;
#72957=AXIS2_PLACEMENT_3D ( 'NONE', #59033, #71801, #30463 ) ;
#72959=ORIENTED_EDGE ( 'NONE', *, *, #76438, .F. ) ;
#72961=CARTESIAN_POINT ( 'NONE',  ( 100.8178804068425904, -31.43438811971037339, 213.5852332267339762 ) ) ;
#72962=AXIS2_PLACEMENT_3D ( 'NONE', #21544, #49668, #34705 ) ;
#72963=CARTESIAN_POINT ( 'NONE',  ( 103.2708046866033129, -47.13561192255075838, 97.28610146638693834 ) ) ;
#72964=CARTESIAN_POINT ( 'NONE',  ( 110.3650187231686743, -47.25482062520524096, 52.80610146638697699 ) ) ;
#72965=CARTESIAN_POINT ( 'NONE',  ( 112.7690144390553257, -28.67084679305116524, 249.5838068554166682 ) ) ;
#72968=CARTESIAN_POINT ( 'NONE',  ( 98.09065366798802188, -42.10120877535955231, 157.7556252759109725 ) ) ;
#72969=EDGE_CURVE ( 'NONE', #52054, #49269, #36334, .T. ) ;
#72970=DIRECTION ( 'NONE',  ( 0.7071067811865160424, 0.7071067811865791031, 0.000000000000000000 ) ) ;
#72971=ORIENTED_EDGE ( 'NONE', *, *, #26899, .T. ) ;
#72972=FACE_OUTER_BOUND ( 'NONE', #79793, .T. ) ;
#72973=ORIENTED_EDGE ( 'NONE', *, *, #35833, .T. ) ;
#72974=EDGE_LOOP ( 'NONE', ( #705, #53899, #13858, #36131 ) ) ;
#72977=ORIENTED_EDGE ( 'NONE', *, *, #69580, .T. ) ;
#72979=DIRECTION ( 'NONE',  ( 2.900000000000000265E-14, -2.000000000000000155E-15, 1.000000000000000000 ) ) ;
#72981=CARTESIAN_POINT ( 'NONE',  ( 105.9042722318897063, -26.76946864612742871, 131.1688829675021850 ) ) ;
#72982=CARTESIAN_POINT ( 'NONE',  ( 100.9409889914183225, -46.87433776650586736, 52.14419670448194921 ) ) ;
#72983=LINE ( 'NONE', #67066, #73613 ) ;
#72984=CARTESIAN_POINT ( 'NONE',  ( 164.9190312289458120, -35.91149509760592906, 237.4678068554150059 ) ) ;
#72985=LINE ( 'NONE', #79382, #28152 ) ;
#72986=CARTESIAN_POINT ( 'NONE',  ( 98.65123886609826798, -31.74476095556097377, 85.90133956162593165 ) ) ;
#72987=CARTESIAN_POINT ( 'NONE',  ( 72.06648329127401098, -45.72944715994106701, 14.67562527591093513 ) ) ;
#72988=CARTESIAN_POINT ( 'NONE',  ( 117.0473132972741013, -39.66401662079133672, 179.5984824187679294 ) ) ;
#72989=CARTESIAN_POINT ( 'NONE',  ( 104.4871046023747141, -26.97959138088134168, 60.28169211698992314 ) ) ;
#72990=CARTESIAN_POINT ( 'NONE',  ( 51.56670390244899949, -32.29483332968430886, 342.9256252759109884 ) ) ;
#72991=EDGE_LOOP ( 'NONE', ( #35590, #28586 ) ) ;
#72992=CARTESIAN_POINT ( 'NONE',  ( 19.56670390244824631, -47.82844715994191631, 300.4678068554150059 ) ) ;
#72993=EDGE_CURVE ( 'NONE', #79585, #19595, #18114, .T. ) ;
#72994=DIRECTION ( 'NONE',  ( -1.175184669632759901E-16, 1.000000000000000000, 2.000000000000003705E-15 ) ) ;
#72996=FACE_OUTER_BOUND ( 'NONE', #15745, .T. ) ;
#72997=EDGE_CURVE ( 'NONE', #42899, #88172, #44918, .T. ) ;
#72998=CARTESIAN_POINT ( 'NONE',  ( 48.16670390244701139, -26.71338133339251542, -5.074374724088000832 ) ) ;
#72999=CARTESIAN_POINT ( 'NONE',  ( 117.2706010548463667, -41.09852764615815346, 213.5165776568629781 ) ) ;
#73000=ORIENTED_EDGE ( 'NONE', *, *, #22707, .F. ) ;
#73001=CARTESIAN_POINT ( 'NONE',  ( 97.81070293921875702, -40.51501671228320589, 146.6354177189882932 ) ) ;
#73002=CARTESIAN_POINT ( 'NONE',  ( 97.20328444759655895, -40.27860260594448505, 262.6013395616254797 ) ) ;
#73003=CARTESIAN_POINT ( 'NONE',  ( 108.9928688995437653, -47.66043690685247469, 118.7032443235299723 ) ) ;
#73004=EDGE_CURVE ( 'NONE', #57751, #75328, #10415, .T. ) ;
#73005=CARTESIAN_POINT ( 'NONE',  ( 113.2492937776126922, -28.76157751642139360, 250.5554876614661737 ) ) ;
#73006=CARTESIAN_POINT ( 'NONE',  ( 82.56634656606027534, -37.87725565066433120, 7.080220459961196866 ) ) ;
#73008=LINE ( 'NONE', #79852, #3229 ) ;
#73009=ORIENTED_EDGE ( 'NONE', *, *, #41909, .F. ) ;
#73012=ORIENTED_EDGE ( 'NONE', *, *, #78679, .T. ) ;
#73013=ORIENTED_EDGE ( 'NONE', *, *, #38150, .T. ) ;
#73014=ORIENTED_EDGE ( 'NONE', *, *, #37541, .T. ) ;
#73015=CARTESIAN_POINT ( 'NONE',  ( 113.1782937634553576, -44.75186859869646838, 73.09395860846349535 ) ) ;
#73016=CARTESIAN_POINT ( 'NONE',  ( 116.3171286962602267, -41.53660429022799150, 284.4441967044824082 ) ) ;
#73018=CARTESIAN_POINT ( 'NONE',  ( 132.9420963948878125, -34.21971364483388811, 1.822997995688940165 ) ) ;
#73019=CARTESIAN_POINT ( 'NONE',  ( 80.06648329127399677, 0.2215528400590013880, 293.6356252759119911 ) ) ;
#73021=CARTESIAN_POINT ( 'NONE',  ( 103.9834678596679538, -28.76382429851063449, 214.7924198280769872 ) ) ;
#73025=CARTESIAN_POINT ( 'NONE',  ( 107.0664832912739968, -18.82844715994099971, 168.9256252759119832 ) ) ;
#73027=DIRECTION ( 'NONE',  ( 0.7071067811989676377, 0.7071067811741275078, 7.071067811989670636E-16 ) ) ;
#73028=CYLINDRICAL_SURFACE ( 'NONE', #62012, 2.117000000000007987 ) ;
#73029=CARTESIAN_POINT ( 'NONE',  ( 98.59875070808803343, -39.34206841476268579, 17.99586902018296541 ) ) ;
#73032=CARTESIAN_POINT ( 'NONE',  ( 50.97905606903279363, -31.62489322948217918, 193.9678068554150911 ) ) ;
#73033=FACE_OUTER_BOUND ( 'NONE', #45657, .T. ) ;
#73035=CYLINDRICAL_SURFACE ( 'NONE', #9827, 0.4999999999999933387 ) ;
#73037=LINE ( 'NONE', #30379, #72750 ) ;
#73038=CARTESIAN_POINT ( 'NONE',  ( 106.6371065190374452, -28.08557299187883061, 42.94618560768698501 ) ) ;
#73040=CARTESIAN_POINT ( 'NONE',  ( 135.6272734918656511, -16.46583755400462579, 7.833212107638488853 ) ) ;
#73041=EDGE_CURVE ( 'NONE', #52002, #15093, #8305, .T. ) ;
#73042=CYLINDRICAL_SURFACE ( 'NONE', #69354, 0.5000000000000197620 ) ;
#73044=ORIENTED_EDGE ( 'NONE', *, *, #49056, .F. ) ;
#73048=VERTEX_POINT ( 'NONE', #85849 ) ;
#73049=CARTESIAN_POINT ( 'NONE',  ( 113.9865487620526920, -28.11017913222394071, 119.5261014663869474 ) ) ;
#73050=EDGE_LOOP ( 'NONE', ( #71403, #24309, #56474, #87011 ) ) ;
#73051=CARTESIAN_POINT ( 'NONE',  ( 98.78342310422263495, -33.06835657602663758, 55.40575316140994033 ) ) ;
#73052=EDGE_CURVE ( 'NONE', #79236, #4014, #52160, .T. ) ;
#73054=CARTESIAN_POINT ( 'NONE',  ( 97.10642131522254772, -35.22350214559244819, 67.63872616303994789 ) ) ;
#73056=EDGE_CURVE ( 'NONE', #26477, #57212, #73078, .T. ) ;
#73058=CYLINDRICAL_SURFACE ( 'NONE', #13530, 0.5000000000000004441 ) ;
#73059=CARTESIAN_POINT ( 'NONE',  ( 116.7902211891048694, -31.42528581690661582, 20.21181575210195902 ) ) ;
#73062=ORIENTED_EDGE ( 'NONE', *, *, #72057, .T. ) ;
#73063=VECTOR ( 'NONE', #43725, 1000.000000000000000 ) ;
#73064=CARTESIAN_POINT ( 'NONE',  ( 25.56670390244797275, -62.87844715994099687, 178.0928068554149775 ) ) ;
#73065=ORIENTED_EDGE ( 'NONE', *, *, #24099, .T. ) ;
#73068=VERTEX_POINT ( 'NONE', #4042 ) ;
#73071=DIRECTION ( 'NONE',  ( 0.000000000000000000, 0.000000000000000000, 1.000000000000000000 ) ) ;
#73072=VERTEX_POINT ( 'NONE', #11759 ) ;
#73073=CARTESIAN_POINT ( 'NONE',  ( 101.0349934672010903, -27.38958028709080139, 220.5327681330539633 ) ) ;
#73074=DIRECTION ( 'NONE',  ( 0.000000000000000000, 0.000000000000000000, -1.000000000000000000 ) ) ;
#73076=CARTESIAN_POINT ( 'NONE',  ( 106.5180998683148488, -25.68982506017174927, 41.12800622829193742 ) ) ;
#73077=ADVANCED_FACE ( 'NONE', ( #27615 ), #47145, .T. ) ;
#73078=LINE ( 'NONE', #79027, #61017 ) ;
#73080=CARTESIAN_POINT ( 'NONE',  ( 103.2795865501787773, -27.47421004149664014, 171.3855331769660495 ) ) ;
#73081=CARTESIAN_POINT ( 'NONE',  ( 90.44969454456439450, -53.34645651782491882, 249.5838068554174640 ) ) ;
#73082=ADVANCED_FACE ( 'NONE', ( #67156 ), #10195, .T. ) ;
#73083=ORIENTED_EDGE ( 'NONE', *, *, #80691, .F. ) ;
#73085=VECTOR ( 'NONE', #65215, 1000.000000000000000 ) ;
#73086=CARTESIAN_POINT ( 'NONE',  ( 72.06648329127399677, -9.729447159941065237, -4.824374724089063982 ) ) ;
#73087=CARTESIAN_POINT ( 'NONE',  ( 112.4005920293390233, -46.38403708128156921, 252.9661014663871583 ) ) ;
#73088=DIRECTION ( 'NONE',  ( 1.000000000000000078E-15, -1.000000000000000083E-30, -1.000000000000000000 ) ) ;
#73089=AXIS2_PLACEMENT_3D ( 'NONE', #39362, #17585, #3065 ) ;
#73090=CARTESIAN_POINT ( 'NONE',  ( 188.5667039024479834, -62.87844715994099687, 298.0928068554150627 ) ) ;
#73091=CARTESIAN_POINT ( 'NONE',  ( 77.40046754268347229, -37.42701295173601039, 2.979899338979277612 ) ) ;
#73092=CARTESIAN_POINT ( 'NONE',  ( 116.1125752699382048, -36.30413522796790460, 268.2743245899816884 ) ) ;
#73093=CARTESIAN_POINT ( 'NONE',  ( 143.0664832912740110, -18.82844715994099971, -5.074374724088000832 ) ) ;
#73094=CARTESIAN_POINT ( 'NONE',  ( 117.9659426345831719, -38.42225801833666310, 64.69181575210097890 ) ) ;
#73096=CARTESIAN_POINT ( 'NONE',  ( 95.73117830242222226, -40.35431382354642693, 131.5727681330539554 ) ) ;
#73097=EDGE_LOOP ( 'NONE', ( #20293, #47893 ) ) ;
#73099=ORIENTED_EDGE ( 'NONE', *, *, #7749, .F. ) ;
#73100=LINE ( 'NONE', #36006, #49655 ) ;
#73102=DIRECTION ( 'NONE',  ( 1.000000000000000000, 8.673617379883546378E-16, 9.757819552368989676E-16 ) ) ;
#73107=CARTESIAN_POINT ( 'NONE',  ( 101.7334424669833339, -26.99437863453528408, 100.4632443235299633 ) ) ;
#73112=DIRECTION ( 'NONE',  ( 0.000000000000000000, 0.000000000000000000, 1.000000000000000000 ) ) ;
#73113=ORIENTED_EDGE ( 'NONE', *, *, #23367, .T. ) ;
#73114=CARTESIAN_POINT ( 'NONE',  ( 108.0362122550155135, -25.69517931502184993, 109.9946728949589811 ) ) ;
#73115=FACE_OUTER_BOUND ( 'NONE', #43460, .T. ) ;
#73117=ORIENTED_EDGE ( 'NONE', *, *, #47105, .F. ) ;
#73122=DIRECTION ( 'NONE',  ( -0.7071067811865175967, -0.7071067811865774377, -7.071067811865168663E-16 ) ) ;
#73124=CARTESIAN_POINT ( 'NONE',  ( 138.8167039024479834, -50.82844715994100682, 60.91780685541480267 ) ) ;
#73126=EDGE_CURVE ( 'NONE', #834, #35753, #1523, .T. ) ;
#73127=ORIENTED_EDGE ( 'NONE', *, *, #82576, .T. ) ;
#73128=VECTOR ( 'NONE', #84077, 1000.000000000000000 ) ;
#73129=PLANE ( 'NONE',  #20118 ) ;
#73130=CARTESIAN_POINT ( 'NONE',  ( 96.72778144249465981, -35.92320320382071230, 187.2765776568629406 ) ) ;
#73132=ORIENTED_EDGE ( 'NONE', *, *, #23752, .T. ) ;
#73133=CARTESIAN_POINT ( 'NONE',  ( 101.5072281473882612, -27.97539281467255279, 61.51467289495899138 ) ) ;
#73134=CARTESIAN_POINT ( 'NONE',  ( 99.50486818388880295, -43.30594552113949192, 51.89608593702373440 ) ) ;
#73136=CARTESIAN_POINT ( 'NONE',  ( 116.3201356630459884, -32.94258242523766711, 69.13562527591093954 ) ) ;
#73137=ORIENTED_EDGE ( 'NONE', *, *, #60123, .F. ) ;
#73138=CYLINDRICAL_SURFACE ( 'NONE', #67499, 11.45913725231036118 ) ;
#73139=ORIENTED_EDGE ( 'NONE', *, *, #47418, .T. ) ;
#73140=ORIENTED_EDGE ( 'NONE', *, *, #30594, .T. ) ;
#73141=EDGE_CURVE ( 'NONE', #50262, #38273, #55298, .T. ) ;
#73142=CARTESIAN_POINT ( 'NONE',  ( 100.4550560919867479, -30.82882778563945791, 187.1787261630399541 ) ) ;
#73143=CARTESIAN_POINT ( 'NONE',  ( 117.0614819080372655, -38.07633510806910948, 54.71886380986607890 ) ) ;
#73144=AXIS2_PLACEMENT_3D ( 'NONE', #49827, #28494, #48464 ) ;
#73146=AXIS2_PLACEMENT_3D ( 'NONE', #21626, #42037, #1631 ) ;
#73147=EDGE_CURVE ( 'NONE', #13607, #20681, #11518, .T. ) ;
#73149=DIRECTION ( 'NONE',  ( 0.000000000000000000, 1.000000000000000000, 0.000000000000000000 ) ) ;
#73152=VERTEX_POINT ( 'NONE', #40792 ) ;
#73154=AXIS2_PLACEMENT_3D ( 'NONE', #26554, #27447, #46971 ) ;
#73155=EDGE_CURVE ( 'NONE', #31941, #47853, #61235, .T. ) ;
#73156=CARTESIAN_POINT ( 'NONE',  ( 97.31317918327525263, -38.96105433417827157, 37.50518654075179370 ) ) ;
#73157=ORIENTED_EDGE ( 'NONE', *, *, #55287, .F. ) ;
#73158=CARTESIAN_POINT ( 'NONE',  ( 101.6088808140983417, -47.24878093606274376, 17.19562527591095247 ) ) ;
#73161=ADVANCED_FACE ( 'NONE', ( #53500 ), #81266, .T. ) ;
#73164=CARTESIAN_POINT ( 'NONE',  ( 46.48091746482045750, -49.32844715994088602, 180.4678068554150911 ) ) ;
#73165=CARTESIAN_POINT ( 'NONE',  ( 101.3252678580387709, -46.22870732629148449, 198.1318157521009482 ) ) ;
#73167=EDGE_CURVE ( 'NONE', #82506, #32225, #68513, .T. ) ;
#73169=CARTESIAN_POINT ( 'NONE',  ( 107.8717034087400322, -26.29179415218835913, 66.01562527591097762 ) ) ;
#73170=CARTESIAN_POINT ( 'NONE',  ( 87.31648329127401098, -46.47944715994105280, 14.92562527591095112 ) ) ;
#73171=ORIENTED_EDGE ( 'NONE', *, *, #45905, .F. ) ;
#73172=ORIENTED_EDGE ( 'NONE', *, *, #38401, .F. ) ;
#73173=EDGE_CURVE ( 'NONE', #26208, #71209, #63959, .T. ) ;
#73174=CARTESIAN_POINT ( 'NONE',  ( 78.26014418490360924, -38.80290789369995252, 7.687431601936923542 ) ) ;
#73175=CARTESIAN_POINT ( 'NONE',  ( 107.0664832912748068, -36.72944715993923381, -5.074374724089029343 ) ) ;
#73176=DIRECTION ( 'NONE',  ( 3.999999999999999995E-14, -1.000000000000000000, 4.100000000000000342E-29 ) ) ;
#73177=CARTESIAN_POINT ( 'NONE',  ( 111.7725766154891431, -30.05993356141850015, 127.4052332267339693 ) ) ;
#73178=CARTESIAN_POINT ( 'NONE',  ( 95.27050013873164858, -38.09949539013453546, 232.4184824187679794 ) ) ;
#73179=EDGE_CURVE ( 'NONE', #38559, #39595, #69856, .T. ) ;
#73182=CARTESIAN_POINT ( 'NONE',  ( 135.9140641843650315, -38.77438500682884381, 2.186796636972260011 ) ) ;
#73185=AXIS2_PLACEMENT_3D ( 'NONE', #68781, #13812, #56010 ) ;
#73186=DIRECTION ( 'NONE',  ( -1.000000000000000078E-15, 1.000000000000000083E-30, 1.000000000000000000 ) ) ;
#73187=ORIENTED_EDGE ( 'NONE', *, *, #54204, .F. ) ;
#73189=CARTESIAN_POINT ( 'NONE',  ( 59.67079009362632291, -0.9310397146383332379, 396.9756252759102040 ) ) ;
#73192=CARTESIAN_POINT ( 'NONE',  ( 77.31648329127399677, -18.72944715994106346, -5.074374724089059541 ) ) ;
#73193=CARTESIAN_POINT ( 'NONE',  ( 102.0031328989874027, -44.23578847709845263, 151.5143245899819817 ) ) ;
#73194=CARTESIAN_POINT ( 'NONE',  ( 96.79018504364255193, -38.90877927100929412, 31.49276813305495892 ) ) ;
#73196=DIRECTION ( 'NONE',  ( 1.147230458779309805E-16, 3.204747427460360459E-31, 1.000000000000000000 ) ) ;
#73199=ORIENTED_EDGE ( 'NONE', *, *, #68336, .T. ) ;
#73200=CARTESIAN_POINT ( 'NONE',  ( 97.79399791629339234, -40.47395449460485395, 167.6321610181374524 ) ) ;
#73201=DIRECTION ( 'NONE',  ( 0.000000000000000000, 0.000000000000000000, -1.000000000000000000 ) ) ;
#73203=CARTESIAN_POINT ( 'NONE',  ( 97.81847504816714434, -40.53396937462733973, 131.6370481833811255 ) ) ;
#73205=AXIS2_PLACEMENT_3D ( 'NONE', #1666, #64771, #29366 ) ;
#73206=ORIENTED_EDGE ( 'NONE', *, *, #3076, .T. ) ;
#73207=CARTESIAN_POINT ( 'NONE',  ( 96.81178581975444786, -38.90419831550661911, 31.49276813305495892 ) ) ;
#73208=CIRCLE ( 'NONE', #22401, 2.517500000000005844 ) ;
#73209=CARTESIAN_POINT ( 'NONE',  ( 100.4377198651835101, -44.85950937921091253, 8.032768133053981074 ) ) ;
#73210=VECTOR ( 'NONE', #77622, 1000.000000000000000 ) ;
#73213=CARTESIAN_POINT ( 'NONE',  ( 107.0664832912750057, -36.72944715993903486, 9.125625275910969947 ) ) ;
#73214=CARTESIAN_POINT ( 'NONE',  ( 184.5667039024483813, -48.82844715993448403, 249.9678068554149775 ) ) ;
#73217=AXIS2_PLACEMENT_3D ( 'NONE', #86427, #65517, #16044 ) ;
#73218=CARTESIAN_POINT ( 'NONE',  ( 152.5667039024469602, -23.42844715993586036, 300.4678068554149490 ) ) ;
#73220=EDGE_CURVE ( 'NONE', #36065, #2851, #50281, .T. ) ;
#73221=CARTESIAN_POINT ( 'NONE',  ( 106.5157732221739195, -25.64298685704507363, 45.12800622829193742 ) ) ;
#73222=CARTESIAN_POINT ( 'NONE',  ( 97.76247233159546113, -41.51031662465626937, 192.7041967044819728 ) ) ;
#73223=CARTESIAN_POINT ( 'NONE',  ( 114.8356066511136504, -43.71357066064707197, 34.24419670448197905 ) ) ;
#73224=DIRECTION ( 'NONE',  ( 1.000000000000000000, 4.299999999999999979E-14, 1.000000000000000078E-15 ) ) ;
#73226=CARTESIAN_POINT ( 'NONE',  ( 107.0664832912739968, -36.72944715994100306, 9.635625275910941312 ) ) ;
#73228=AXIS2_PLACEMENT_3D ( 'NONE', #6090, #26518, #61472 ) ;
#73229=ORIENTED_EDGE ( 'NONE', *, *, #21601, .T. ) ;
#73231=VERTEX_POINT ( 'NONE', #69409 ) ;
#73232=CARTESIAN_POINT ( 'NONE',  ( 102.0418483691416895, -28.29933337693059414, 81.50419670448194154 ) ) ;
#73233=DIRECTION ( 'NONE',  ( 0.000000000000000000, 0.000000000000000000, 1.000000000000000000 ) ) ;
#73234=ORIENTED_EDGE ( 'NONE', *, *, #34101, .T. ) ;
#73235=DIRECTION ( 'NONE',  ( 0.000000000000000000, 0.000000000000000000, -1.000000000000000000 ) ) ;
#73236=CARTESIAN_POINT ( 'NONE',  ( 109.3321198358311932, -26.57584895156214699, 220.9013395616249795 ) ) ;
#73238=CARTESIAN_POINT ( 'NONE',  ( 116.3221839001005264, -32.94216875276463696, 149.1356252759109680 ) ) ;
#73240=CARTESIAN_POINT ( 'NONE',  ( 78.13314995793999174, 12.92155284005730387, 358.9756252759109998 ) ) ;
#73242=CARTESIAN_POINT ( 'NONE',  ( 131.7155263566431813, -38.16021090637521951, 2.608895778950927724 ) ) ;
#73244=CARTESIAN_POINT ( 'NONE',  ( 104.0088209277215583, -27.43890701233894092, 165.3299109901969643 ) ) ;
#73245=ORIENTED_EDGE ( 'NONE', *, *, #61698, .T. ) ;
#73246=VERTEX_POINT ( 'NONE', #42128 ) ;
#73248=CARTESIAN_POINT ( 'NONE',  ( 101.3137116872897820, -44.99844491211269570, 83.52444044875394979 ) ) ;
#73250=CARTESIAN_POINT ( 'NONE',  ( 97.67678136301130110, -41.13084272647604678, 207.6632443235299661 ) ) ;
#73253=DIRECTION ( 'NONE',  ( 0.000000000000000000, 1.000000000000000000, 0.000000000000000000 ) ) ;
#73257=CARTESIAN_POINT ( 'NONE',  ( 177.0371591254543659, -48.62818131005480637, 237.4678068554150059 ) ) ;
#73258=EDGE_CURVE ( 'NONE', #58668, #32600, #43638, .T. ) ;
#73259=DIRECTION ( 'NONE',  ( -0.9254794337955620787, -0.3787978585227822492, 0.000000000000000000 ) ) ;
#73260=CARTESIAN_POINT ( 'NONE',  ( 102.9757002774701959, -26.48594595611781344, 175.3908633711489813 ) ) ;
#73263=ORIENTED_EDGE ( 'NONE', *, *, #60978, .F. ) ;
#73264=ADVANCED_FACE ( 'NONE', ( #8984 ), #808, .T. ) ;
#73266=CARTESIAN_POINT ( 'NONE',  ( 97.31584368152388720, -39.30597586568408985, 152.5314585983696531 ) ) ;
#73267=CARTESIAN_POINT ( 'NONE',  ( 51.06648329127400388, 19.62155284005901024, 336.6506252759110112 ) ) ;
#73269=CIRCLE ( 'NONE', #84916, 1.000000000000000888 ) ;
#73272=VECTOR ( 'NONE', #69456, 1000.000000000000000 ) ;
#73273=CARTESIAN_POINT ( 'NONE',  ( 141.8164832912740110, -9.833000550534297446, -5.074374724088994704 ) ) ;
#73274=CIRCLE ( 'NONE', #38451, 3.600000000000000089 ) ;
#73275=AXIS2_PLACEMENT_3D ( 'NONE', #25480, #10953, #25936 ) ;
#73276=CARTESIAN_POINT ( 'NONE',  ( 117.7793243111075157, -34.00655811778471360, 169.0365776568629599 ) ) ;
#73277=CARTESIAN_POINT ( 'NONE',  ( 135.1909174281129538, -39.23916151080251069, 8.028235474617126499 ) ) ;
#73279=VERTEX_POINT ( 'NONE', #83945 ) ;
#73282=AXIS2_PLACEMENT_3D ( 'NONE', #51658, #66637, #45288 ) ;
#73284=CARTESIAN_POINT ( 'NONE',  ( 95.35945913470564506, -35.72541260001472097, 298.1356252759109680 ) ) ;
#73286=CARTESIAN_POINT ( 'NONE',  ( 116.2008526694824582, -35.09873344310054932, 46.78523322673494533 ) ) ;
#73287=AXIS2_PLACEMENT_3D ( 'NONE', #14501, #77617, #856 ) ;
#73288=LINE ( 'NONE', #11977, #71036 ) ;
#73290=AXIS2_PLACEMENT_3D ( 'NONE', #35141, #48306, #21540 ) ;
#73295=DIRECTION ( 'NONE',  ( 1.000000000000000000, 4.163336342344347755E-14, 0.000000000000000000 ) ) ;
#73297=ORIENTED_EDGE ( 'NONE', *, *, #67633, .T. ) ;
#73299=AXIS2_PLACEMENT_3D ( 'NONE', #58261, #58693, #30117 ) ;
#73300=CARTESIAN_POINT ( 'NONE',  ( 102.4109068130577356, -29.56832019646944687, 24.95813411379099733 ) ) ;
#73301=CARTESIAN_POINT ( 'NONE',  ( 117.2137812332333766, -41.17104435167765075, 208.4861014663869696 ) ) ;
#73302=CARTESIAN_POINT ( 'NONE',  ( 96.06973772670281164, -35.87188691900273341, 191.2765776568629690 ) ) ;
#73304=CARTESIAN_POINT ( 'NONE',  ( 99.33320739591177073, -28.83195234130426243, 266.7051490854347549 ) ) ;
#73306=CYLINDRICAL_SURFACE ( 'NONE', #46789, 2.117000000000000881 ) ;
#73307=VERTEX_POINT ( 'NONE', #35765 ) ;
#73309=B_SPLINE_CURVE_WITH_KNOTS ( 'NONE', 3,
 ( #16985, #36975, #85597, #31482, #80115, #23376, #71955, #37424, #51045, #16537, #34166, #20114, #26473, #74178, #39642, #47343, #11505, #75071, #55040, #39199, #82804, #60989, #88716, #26031, #74618, #88273, #68267, #6048, #32373, #66909 ),
 .UNSPECIFIED., .F., .F.,
 ( 4, 2, 2, 2, 1, 2, 2, 2, 2, 2, 2, 2, 1, 2, 2, 4 ),
 ( 0.000000000000000000, 0.1249999999999997780, 0.1875000000000007772, 0.2187500000000001110, 0.2343749999999997780, 0.2421874999999996392, 0.2499999999999995282, 0.3749999999999976685, 0.4374999999999936717, 0.4999999999999896749, 0.6249999999999764633, 0.6874999999999692468, 0.7187499999999694689, 0.7343749999999699130, 0.7499999999999704681, 1.000000000000000000 ),
 .UNSPECIFIED. ) ;
#73310=EDGE_CURVE ( 'NONE', #11858, #26048, #14679, .T. ) ;
#73311=B_SPLINE_CURVE_WITH_KNOTS ( 'NONE', 3,
 ( #54190, #89205, #76009, #13784, #81953, #26971, #54638, #20162, #68752, #39688, #5183, #6522, #41470, #32877, #60577, #64620, #35111, #43717 ),
 .UNSPECIFIED., .F., .F.,
 ( 4, 2, 2, 2, 2, 2, 2, 2, 4 ),
 ( 0.000000000000000000, 0.06250000025565728701, 0.1250000005113145740, 0.1875000007669718749, 0.2500000010226291480, 0.3125000012782864212, 0.3750000015339437498, 0.4375000017896010229, 0.5000000020452582961 ),
 .UNSPECIFIED. ) ;
#73312=CIRCLE ( 'NONE', #19636, 3.249999999999975131 ) ;
#73313=CARTESIAN_POINT ( 'NONE',  ( 97.81362638013557387, -40.52215668197012377, 111.6360318040896829 ) ) ;
#73314=CARTESIAN_POINT ( 'NONE',  ( 106.8507020815961397, -47.82747951245497831, 227.5489586092439538 ) ) ;
#73316=CARTESIAN_POINT ( 'NONE',  ( 117.9487373648833426, -34.79150140969374405, 198.9546728949589749 ) ) ;
#73318=AXIS2_PLACEMENT_3D ( 'NONE', #61040, #88771, #26529 ) ;
#73319=CYLINDRICAL_SURFACE ( 'NONE', #4235, 1.000000000002049694 ) ;
#73320=EDGE_CURVE ( 'NONE', #23215, #87708, #5924, .T. ) ;
#73321=CARTESIAN_POINT ( 'NONE',  ( 31.78666935232998725, -36.02818131005891189, -5.074374724088000832 ) ) ;
#73325=CARTESIAN_POINT ( 'NONE',  ( 96.55902551080276908, -40.08462249002850086, 277.5603871806729899 ) ) ;
#73326=CARTESIAN_POINT ( 'NONE',  ( 63.03715912545646205, -24.89890238295017255, 129.9678068554150911 ) ) ;
#73327=CARTESIAN_POINT ( 'NONE',  ( 182.5667039024459939, -22.48495420874030515, -5.074374724088000832 ) ) ;
#73330=CARTESIAN_POINT ( 'NONE',  ( 21.03715912545829170, -47.82818131006186491, 249.9678068554150059 ) ) ;
#73331=DIRECTION ( 'NONE',  ( -0.9254794337955620787, -0.3787978585227822492, 0.000000000000000000 ) ) ;
#73333=VERTEX_POINT ( 'NONE', #15791 ) ;
#73334=CARTESIAN_POINT ( 'NONE',  ( 136.4105765916308144, -20.17027654743777276, 7.249284792654901111 ) ) ;
#73335=CARTESIAN_POINT ( 'NONE',  ( 109.3633609874958523, -25.89340572475189006, 184.9222919425779708 ) ) ;
#73336=CARTESIAN_POINT ( 'NONE',  ( 106.0764678730365063, -48.53853201145131635, 108.5099109901969712 ) ) ;
#73337=CARTESIAN_POINT ( 'NONE',  ( 95.24589774366052097, -38.10235284316662074, 232.4184824187679794 ) ) ;
#73338=CARTESIAN_POINT ( 'NONE',  ( 63.56670390244828184, -47.82844715994016127, 249.9678068554150343 ) ) ;
#73339=LINE ( 'NONE', #11112, #21400 ) ;
#73340=DIRECTION ( 'NONE',  ( -1.000000000000000000, -3.360405532702990443E-14, 0.000000000000000000 ) ) ;
#73341=CARTESIAN_POINT ( 'NONE',  ( 97.82515122448313605, -40.55016472165671360, 37.63815125684190832 ) ) ;
#73343=DIRECTION ( 'NONE',  ( 1.000000000000000000, 4.163336342344333240E-14, 0.000000000000000000 ) ) ;
#73345=AXIS2_PLACEMENT_3D ( 'NONE', #32249, #5458, #59945 ) ;
#73346=EDGE_CURVE ( 'NONE', #41277, #86596, #33240, .T. ) ;
#73347=AXIS2_PLACEMENT_3D ( 'NONE', #44639, #3329, #16958 ) ;
#73348=CIRCLE ( 'NONE', #3712, 5.499999999999999112 ) ;
#73349=VECTOR ( 'NONE', #37227, 1000.000000000000000 ) ;
#73351=ORIENTED_EDGE ( 'NONE', *, *, #35302, .T. ) ;
#73352=VECTOR ( 'NONE', #67417, 1000.000000000000000 ) ;
#73353=CARTESIAN_POINT ( 'NONE',  ( 103.9632409301644316, -45.23724106753869734, 96.70861030426696914 ) ) ;
#73355=ORIENTED_EDGE ( 'NONE', *, *, #86284, .T. ) ;
#73356=CARTESIAN_POINT ( 'NONE',  ( 117.2009162446674395, -42.82382785266563019, 124.3956252759109731 ) ) ;
#73359=CARTESIAN_POINT ( 'NONE',  ( 78.80082187617267664, -16.28157759251482517, 7.978179524063404138 ) ) ;
#73360=CARTESIAN_POINT ( 'NONE',  ( 165.9667039024459996, -28.27351298637401200, 117.4678068554150485 ) ) ;
#73362=AXIS2_PLACEMENT_3D ( 'NONE', #38175, #57722, #9583 ) ;
#73363=CARTESIAN_POINT ( 'NONE',  ( 101.3216544293209864, -28.81361639883581205, 75.57562527591093726 ) ) ;
#73367=DIRECTION ( 'NONE',  ( -1.000000000000000078E-15, 1.000000000000000083E-30, 1.000000000000000000 ) ) ;
#73368=CARTESIAN_POINT ( 'NONE',  ( 117.2073019650708261, -38.89799087863979565, 104.6708633711489824 ) ) ;
#73369=CARTESIAN_POINT ( 'NONE',  ( 51.56670390244772761, -33.35206098992764367, 237.4678068554150059 ) ) ;
#73370=CIRCLE ( 'NONE', #55970, 2.117000000000007987 ) ;
#73371=DIRECTION ( 'NONE',  ( 0.000000000000000000, 0.000000000000000000, 1.000000000000000000 ) ) ;
#73374=DIRECTION ( 'NONE',  ( -0.7071067708032375831, -0.0001211784769794317250, 0.7071067811865434649 ) ) ;
#73376=CARTESIAN_POINT ( 'NONE',  ( 62.03715912545754207, -47.82818131006020934, 129.9678068554150911 ) ) ;
#73377=CARTESIAN_POINT ( 'NONE',  ( 110.4495079430909641, -47.22796928374267367, 57.83657765686300678 ) ) ;
#73378=ORIENTED_EDGE ( 'NONE', *, *, #29306, .F. ) ;
#73381=EDGE_CURVE ( 'NONE', #58445, #61346, #86617, .T. ) ;
#73383=CARTESIAN_POINT ( 'NONE',  ( 31.78666935232898894, -29.62846900982320264, 342.9256252759119548 ) ) ;
#73385=CARTESIAN_POINT ( 'NONE',  ( 115.3759468638744181, -39.14889752855258820, 136.4071379886389650 ) ) ;
#73386=VECTOR ( 'NONE', #57989, 1000.000000000000000 ) ;
#73389=ORIENTED_EDGE ( 'NONE', *, *, #89579, .T. ) ;
#73390=ADVANCED_FACE ( 'NONE', ( #45682 ), #78478, .T. ) ;
#73393=ORIENTED_EDGE ( 'NONE', *, *, #9489, .T. ) ;
#73394=EDGE_CURVE ( 'NONE', #53017, #12546, #16679, .T. ) ;
#73396=CARTESIAN_POINT ( 'NONE',  ( 115.5247806442692422, -34.08644044406323559, 170.4987261630399473 ) ) ;
#73397=PLANE ( 'NONE',  #32720 ) ;
#73398=AXIS2_PLACEMENT_3D ( 'NONE', #33296, #49482, #42223 ) ;
#73399=FACE_OUTER_BOUND ( 'NONE', #56097, .T. ) ;
#73405=AXIS2_PLACEMENT_3D ( 'NONE', #31367, #17750, #79995 ) ;
#73408=CARTESIAN_POINT ( 'NONE',  ( 115.1674193411231784, -35.52216783720512439, 216.7623760838769726 ) ) ;
#73409=CARTESIAN_POINT ( 'NONE',  ( 103.1971861921166038, -46.47197777470199753, 117.2756252759109543 ) ) ;
#73410=CARTESIAN_POINT ( 'NONE',  ( 99.31004196827748842, -43.71529311364911763, 56.90991099019593236 ) ) ;
#73411=CARTESIAN_POINT ( 'NONE',  ( 105.7135912305062391, -46.72357220724894233, 252.4691331623911594 ) ) ;
#73412=FACE_OUTER_BOUND ( 'NONE', #13847, .T. ) ;
#73413=CARTESIAN_POINT ( 'NONE',  ( 107.5312500490845053, -25.27893178259700591, 323.2150800290978623 ) ) ;
#73414=CARTESIAN_POINT ( 'NONE',  ( 102.8440116971490852, -46.26114276377411016, 173.2441967044829596 ) ) ;
#73418=ORIENTED_EDGE ( 'NONE', *, *, #50310, .T. ) ;
#73419=ORIENTED_EDGE ( 'NONE', *, *, #13852, .T. ) ;
#73420=CARTESIAN_POINT ( 'NONE',  ( 128.0667039024480118, -50.82844715994100682, 310.9178068554150514 ) ) ;
#73422=VECTOR ( 'NONE', #58068, 1000.000000000000000 ) ;
#73423=EDGE_LOOP ( 'NONE', ( #65316, #55513, #51846, #16502, #88833, #13199, #23936, #71230, #50438, #36835, #61059, #72845, #53185, #61184 ) ) ;
#73426=CARTESIAN_POINT ( 'NONE',  ( 110.4252027303417663, -27.27630697421929540, 130.8049591708739854 ) ) ;
#73427=CARTESIAN_POINT ( 'NONE',  ( 104.4906584979394211, -46.86803844812923359, 47.37848241876796607 ) ) ;
#73428=CARTESIAN_POINT ( 'NONE',  ( 46.83715912545343940, -47.82818131006086304, 129.9678068554150911 ) ) ;
#73429=VECTOR ( 'NONE', #44751, 999.9999999999998863 ) ;
#73433=CARTESIAN_POINT ( 'NONE',  ( 114.1038288540493539, -43.56973530630605751, 98.21276813305496489 ) ) ;
#73435=CARTESIAN_POINT ( 'NONE',  ( 95.43233898611183008, -38.84956357215551037, 197.4699109901969791 ) ) ;
#73436=CARTESIAN_POINT ( 'NONE',  ( 115.0858478210553102, -30.61367454548772926, 59.34435376945771168 ) ) ;
#73437=DIRECTION ( 'NONE',  ( 0.7071067811869283792, -0.7071067811861665442, 7.071067811869291448E-16 ) ) ;
#73438=ORIENTED_EDGE ( 'NONE', *, *, #50801, .T. ) ;
#73440=DIRECTION ( 'NONE',  ( -4.299999999999999979E-14, 1.000000000000000000, -4.400000000000000367E-29 ) ) ;
#73442=DIRECTION ( 'NONE',  ( -0.000000000000000000, 1.000000000000000000, 0.000000000000000000 ) ) ;
#73443=CARTESIAN_POINT ( 'NONE',  ( 116.4168962126584717, -41.43863437684461104, 203.4556252759109611 ) ) ;
#73445=CARTESIAN_POINT ( 'NONE',  ( 97.70664662319364879, -40.25154480828024361, 146.6128751502485841 ) ) ;
#73446=CARTESIAN_POINT ( 'NONE',  ( 100.4653332305737905, -44.82571634032018437, 8.032768133053981074 ) ) ;
#73447=CARTESIAN_POINT ( 'NONE',  ( 102.2824096876565108, -27.37794169069978523, 116.4527681330539650 ) ) ;
#73449=CARTESIAN_POINT ( 'NONE',  ( 82.80376803119651186, -37.00431460296900354, 6.768845908774068221 ) ) ;
#73454=ORIENTED_EDGE ( 'NONE', *, *, #81140, .F. ) ;
#73455=ORIENTED_EDGE ( 'NONE', *, *, #34723, .T. ) ;
#73456=VERTEX_POINT ( 'NONE', #23514 ) ;
#73457=CARTESIAN_POINT ( 'NONE',  ( 115.0372575016916556, -42.90846257304766453, 73.30229194195298703 ) ) ;
#73458=CARTESIAN_POINT ( 'NONE',  ( 115.3234718241651535, -45.22984455807579707, 264.1899109901965517 ) ) ;
#73459=DIRECTION ( 'NONE',  ( 6.524622321627019585E-16, 3.741823817616790462E-31, 1.000000000000000000 ) ) ;
#73462=ADVANCED_FACE ( 'NONE', ( #72093 ), #32077, .T. ) ;
#73466=CARTESIAN_POINT ( 'NONE',  ( 102.4446420578519934, -44.51733865501087450, 206.5848007804579538 ) ) ;
#73467=ORIENTED_EDGE ( 'NONE', *, *, #1151, .F. ) ;
#73469=CIRCLE ( 'NONE', #69136, 3.299999999999997158 ) ;
#73470=VERTEX_POINT ( 'NONE', #51623 ) ;
#73471=TOROIDAL_SURFACE ( 'NONE', #34305, 15.69999999999999929, 0.2999999999999999889 ) ;
#73472=VECTOR ( 'NONE', #66450, 1000.000000000000000 ) ;
#73473=DIRECTION ( 'NONE',  ( 1.000000000000000078E-15, -1.000000000000000083E-30, -1.000000000000000000 ) ) ;
#73475=DIRECTION ( 'NONE',  ( -4.237773401492740281E-14, 1.000000000000000000, 0.000000000000000000 ) ) ;
#73478=CARTESIAN_POINT ( 'NONE',  ( 100.3180865808431719, -43.26669944020724756, 38.38253568684996253 ) ) ;
#73480=CARTESIAN_POINT ( 'NONE',  ( 113.2433229834693975, -28.75700906242621357, 174.5525078777224621 ) ) ;
#73481=EDGE_CURVE ( 'NONE', #8582, #18961, #3486, .T. ) ;
#73482=DIRECTION ( 'NONE',  ( 0.000000000000000000, 0.000000000000000000, -1.000000000000000000 ) ) ;
#73483=ORIENTED_EDGE ( 'NONE', *, *, #26131, .T. ) ;
#73484=CARTESIAN_POINT ( 'NONE',  ( 110.2707404709723846, -27.22220358462151779, 55.81764542590168077 ) ) ;
#73486=AXIS2_PLACEMENT_3D ( 'NONE', #10526, #11876, #80034 ) ;
#73487=DIRECTION ( 'NONE',  ( -1.000000000000000000, -4.299999999999999979E-14, -9.351236661543306751E-17 ) ) ;
#73488=CARTESIAN_POINT ( 'NONE',  ( 106.7065939435451440, -28.08240114970028856, 37.91570941720995336 ) ) ;
#73489=CLOSED_SHELL ( 'NONE', ( #47727, #16369, #24698, #48115, #81105, #53124, #25832, #75275, #2120, #2417 ) ) ;
#73490=CARTESIAN_POINT ( 'NONE',  ( 136.0678963113202258, -16.84294903903614937, 7.549690073078446417 ) ) ;
#73492=CARTESIAN_POINT ( 'NONE',  ( 107.0664832912739541, -36.72944715994095333, 305.0306255462182321 ) ) ;
#73493=LINE ( 'NONE', #53467, #74972 ) ;
#73496=ADVANCED_FACE ( 'NONE', ( #45250 ), #10736, .T. ) ;
#73497=PLANE ( 'NONE',  #39685 ) ;
#73498=VERTEX_POINT ( 'NONE', #51177 ) ;
#73499=CARTESIAN_POINT ( 'NONE',  ( 117.2223540064780991, -42.83671953415140621, 128.3956252759109873 ) ) ;
#73502=CARTESIAN_POINT ( 'NONE',  ( 107.2750367832685043, -27.67576416532946126, 74.46861030426799744 ) ) ;
#73503=EDGE_CURVE ( 'NONE', #71292, #79308, #72643, .T. ) ;
#73504=CARTESIAN_POINT ( 'NONE',  ( 162.7131505118539962, -33.70561438052111214, -5.074374724088000832 ) ) ;
#73505=CARTESIAN_POINT ( 'NONE',  ( 115.5559677222042154, -32.70388140663459353, 60.62253568684894134 ) ) ;
#73509=CARTESIAN_POINT ( 'NONE',  ( 117.4061096064183971, -38.22256018827695101, 24.71276813305395237 ) ) ;
#73510=VECTOR ( 'NONE', #71458, 1000.000000000000000 ) ;
#73511=LINE ( 'NONE', #3580, #28015 ) ;
#73513=CARTESIAN_POINT ( 'NONE',  ( 113.1781050883711544, -44.75200969554006747, 258.0938408987704520 ) ) ;
#73514=ORIENTED_EDGE ( 'NONE', *, *, #87758, .T. ) ;
#73516=VERTEX_POINT ( 'NONE', #13001 ) ;
#73517=VERTEX_POINT ( 'NONE', #32976 ) ;
#73519=CARTESIAN_POINT ( 'NONE',  ( 104.0204373342842388, -47.42213563049719482, 217.3556252759109668 ) ) ;
#73520=DIRECTION ( 'NONE',  ( -0.000000000000000000, -0.000000000000000000, -1.000000000000000000 ) ) ;
#73522=B_SPLINE_CURVE_WITH_KNOTS ( 'NONE', 3,
 ( #385, #26743, #5422, #12684, #61701, #6308, #61263, #41256, #47622, #14015, #68089, #89434, #5875, #33117, #62609, #82185, #19941, #34898 ),
 .UNSPECIFIED., .F., .F.,
 ( 4, 2, 2, 2, 2, 2, 2, 2, 4 ),
 ( 0.4999434485927969907, 0.5624505175186973460, 0.6249575864445977569, 0.6874646553704981677, 0.7499717242963985786, 0.8124787932222989895, 0.8749858621481992893, 0.9374929310740995891, 1.000000000000000000 ),
 .UNSPECIFIED. ) ;
#73523=CARTESIAN_POINT ( 'NONE',  ( 99.29379691555868703, -43.72992423520055638, 52.90991099019698396 ) ) ;
#73524=CARTESIAN_POINT ( 'NONE',  ( 116.3212776292295842, -32.94146857471309886, 45.13562527591097506 ) ) ;
#73526=CARTESIAN_POINT ( 'NONE',  ( 115.8256479356252555, -31.73037971375361366, 114.2402245575558055 ) ) ;
#73528=DIRECTION ( 'NONE',  ( 0.000000000000000000, 1.000000000000000000, 0.000000000000000000 ) ) ;
#73529=ORIENTED_EDGE ( 'NONE', *, *, #79906, .T. ) ;
#73530=AXIS2_PLACEMENT_3D ( 'NONE', #50544, #78734, #8332 ) ;
#73531=DIRECTION ( 'NONE',  ( -4.299999999999999979E-14, 1.000000000000000000, -4.400000000000000367E-29 ) ) ;
#73532=AXIS2_PLACEMENT_3D ( 'NONE', #74959, #12743, #54482 ) ;
#73533=CARTESIAN_POINT ( 'NONE',  ( 108.3314314236784384, -46.73508782468640277, 113.6779012139213449 ) ) ;
#73534=CARTESIAN_POINT ( 'NONE',  ( 103.9458437887065827, -26.80522050874817808, 250.3184824187678714 ) ) ;
#73536=CONICAL_SURFACE ( 'NONE', #8259, 1.258750000000002922, 1.029744258676650093 ) ;
#73537=EDGE_CURVE ( 'NONE', #42076, #34742, #20442, .T. ) ;
#73538=CARTESIAN_POINT ( 'NONE',  ( 163.0664832912739826, 19.62155284005901024, 339.0006252759110339 ) ) ;
#73539=CARTESIAN_POINT ( 'NONE',  ( 83.56670559755329464, -36.73837296219065252, 239.5838068554176914 ) ) ;
#73540=CARTESIAN_POINT ( 'NONE',  ( 115.6071762752661130, -36.01623928086704041, 253.3152769709339793 ) ) ;
#73542=CARTESIAN_POINT ( 'NONE',  ( 101.7220374796297335, -27.76276858577408291, 81.50419670448295051 ) ) ;
#73544=CARTESIAN_POINT ( 'NONE',  ( 97.53097521295029537, -31.04728477963730171, 130.9108633711489915 ) ) ;
#73545=ORIENTED_EDGE ( 'NONE', *, *, #59881, .T. ) ;
#73551=CARTESIAN_POINT ( 'NONE',  ( 135.7052281011855541, -34.51875982969371393, 2.060081176883824305 ) ) ;
#73553=CARTESIAN_POINT ( 'NONE',  ( 164.9212702847357548, -29.73316016638997894, 313.9678068554149490 ) ) ;
#73554=CARTESIAN_POINT ( 'NONE',  ( 97.18391573584769105, -31.67496972499959895, 95.96229194257799122 ) ) ;
#73555=EDGE_LOOP ( 'NONE', ( #28308, #36557 ) ) ;
#73559=DIRECTION ( 'NONE',  ( -0.8571673007021084478, -0.5150380749100604838, -8.571673007021083688E-16 ) ) ;
#73560=VERTEX_POINT ( 'NONE', #40231 ) ;
#73561=AXIS2_PLACEMENT_3D ( 'NONE', #46882, #34162, #81010 ) ;
#73562=CARTESIAN_POINT ( 'NONE',  ( 109.5136938427377373, -46.88609643433851915, 132.7641967044819751 ) ) ;
#73563=EDGE_CURVE ( 'NONE', #10086, #74993, #68850, .T. ) ;
#73565=DIRECTION ( 'NONE',  ( -0.7071067812162665778, -0.7071067811568285677, -6.612322856132800227E-17 ) ) ;
#73570=ORIENTED_EDGE ( 'NONE', *, *, #4979, .F. ) ;
#73571=FACE_OUTER_BOUND ( 'NONE', #62461, .T. ) ;
#73572=LINE ( 'NONE', #44963, #51231 ) ;
#73573=DIRECTION ( 'NONE',  ( 0.000000000000000000, 0.000000000000000000, -1.000000000000000000 ) ) ;
#73574=EDGE_CURVE ( 'NONE', #83432, #58568, #37413, .T. ) ;
#73578=CARTESIAN_POINT ( 'NONE',  ( 90.44969454456416713, -50.82895651782500579, 219.5838068554169809 ) ) ;
#73582=DIRECTION ( 'NONE',  ( 0.000000000000000000, 0.000000000000000000, -1.000000000000000000 ) ) ;
#73583=EDGE_CURVE ( 'NONE', #3527, #27939, #40726, .T. ) ;
#73584=CARTESIAN_POINT ( 'NONE',  ( 115.8019334949657804, -41.12891815432276843, 199.4556252759109611 ) ) ;
#73585=CARTESIAN_POINT ( 'NONE',  ( 107.0664832912750057, -36.72944715993903486, 0.4256252759109709349 ) ) ;
#73586=VERTEX_POINT ( 'NONE', #47031 ) ;
#73587=CARTESIAN_POINT ( 'NONE',  ( 113.0644005321300227, -46.09090919705343481, 64.02991099019594401 ) ) ;
#73588=CARTESIAN_POINT ( 'NONE',  ( 110.8542690866539004, -45.98432040429123902, 52.88560783171133295 ) ) ;
#73591=DIRECTION ( 'NONE',  ( -1.000000000000000000, -4.012088370409549976E-14, 0.000000000000000000 ) ) ;
#73593=FACE_OUTER_BOUND ( 'NONE', #48542, .T. ) ;
#73594=VECTOR ( 'NONE', #19357, 1000.000000000000000 ) ;
#73596=ORIENTED_EDGE ( 'NONE', *, *, #52522, .T. ) ;
#73597=CARTESIAN_POINT ( 'NONE',  ( 110.9273191204289191, -44.70580129652318391, 244.3672975916109635 ) ) ;
#73600=VECTOR ( 'NONE', #45333, 1000.000000000000114 ) ;
#73603=DIRECTION ( 'NONE',  ( -0.9254794337955620787, -0.3787978585227822492, 0.000000000000000000 ) ) ;
#73604=EDGE_LOOP ( 'NONE', ( #6235, #8937, #30817, #66827, #57216, #6582, #34337, #79138 ) ) ;
#73607=ORIENTED_EDGE ( 'NONE', *, *, #35385, .T. ) ;
#73608=CARTESIAN_POINT ( 'NONE',  ( 116.7272869458707305, -31.35841744470506498, 29.24229194257799236 ) ) ;
#73609=ORIENTED_EDGE ( 'NONE', *, *, #34266, .F. ) ;
#73611=CARTESIAN_POINT ( 'NONE',  ( 106.0563433008199752, -28.62948770221197137, 267.9938046553056665 ) ) ;
#73613=VECTOR ( 'NONE', #31647, 1000.000000000000000 ) ;
#73614=FACE_OUTER_BOUND ( 'NONE', #10384, .T. ) ;
#73616=CARTESIAN_POINT ( 'NONE',  ( 37.56670390244716629, -48.82844715994106366, 180.4678068554150911 ) ) ;
#73619=ADVANCED_FACE ( 'NONE', ( #75219 ), #26612, .T. ) ;
#73621=CARTESIAN_POINT ( 'NONE',  ( 116.8983464293968524, -40.32492306460803633, 214.5470538473389581 ) ) ;
#73622=CARTESIAN_POINT ( 'NONE',  ( 182.5667039024480118, -32.29483332968450782, 117.4678068554150627 ) ) ;
#73623=AXIS2_PLACEMENT_3D ( 'NONE', #32135, #10798, #52557 ) ;
#73625=CARTESIAN_POINT ( 'NONE',  ( 110.1708544452211100, -46.72723989065711692, 93.81562527591097478 ) ) ;
#73629=ORIENTED_EDGE ( 'NONE', *, *, #2548, .T. ) ;
#73630=FACE_OUTER_BOUND ( 'NONE', #79359, .T. ) ;
#73631=PLANE ( 'NONE',  #73275 ) ;
#73632=CARTESIAN_POINT ( 'NONE',  ( 117.0724204941129472, -35.46684028317002202, 153.9277302053984897 ) ) ;
#73633=CARTESIAN_POINT ( 'NONE',  ( 99.66770068389166681, -32.23957622922084454, 123.6985665600679738 ) ) ;
#73634=CARTESIAN_POINT ( 'NONE',  ( 104.3186933571878399, -25.99935600364358024, 241.2880062282919482 ) ) ;
#73636=VERTEX_POINT ( 'NONE', #35209 ) ;
#73637=CARTESIAN_POINT ( 'NONE',  ( 136.6144450028905055, -37.76411817600060772, 2.828498113172214445 ) ) ;
#73639=AXIS2_PLACEMENT_3D ( 'NONE', #47410, #76481, #55109 ) ;
#73640=ORIENTED_EDGE ( 'NONE', *, *, #35530, .F. ) ;
#73641=CARTESIAN_POINT ( 'NONE',  ( 83.56670390244799762, -36.72944715994108122, 239.5838068554169809 ) ) ;
#73642=ORIENTED_EDGE ( 'NONE', *, *, #74185, .T. ) ;
#73643=ORIENTED_EDGE ( 'NONE', *, *, #49136, .F. ) ;
#73645=FACE_OUTER_BOUND ( 'NONE', #15226, .T. ) ;
#73647=CARTESIAN_POINT ( 'NONE',  ( 112.3908963168805712, -43.44530362507355647, 167.5324198280769963 ) ) ;
#73648=CARTESIAN_POINT ( 'NONE',  ( 96.61485869678695337, -32.99094118449985302, 26.06514908543494613 ) ) ;
#73649=LINE ( 'NONE', #60001, #39369 ) ;
#73651=CARTESIAN_POINT ( 'NONE',  ( 141.0667039024479834, -58.72944715994110254, 310.9178068554150514 ) ) ;
#73652=VERTEX_POINT ( 'NONE', #42464 ) ;
#73653=DIRECTION ( 'NONE',  ( 1.000000000000000078E-15, -1.000000000000000083E-30, -1.000000000000000000 ) ) ;
#73654=EDGE_LOOP ( 'NONE', ( #15513, #76861, #28695, #1271 ) ) ;
#73655=DIRECTION ( 'NONE',  ( -1.000000000000000000, -2.756263715554006823E-15, 0.000000000000000000 ) ) ;
#73656=VECTOR ( 'NONE', #70887, 1000.000000000000000 ) ;
#73657=CARTESIAN_POINT ( 'NONE',  ( 105.9716693386988311, -11.55321978063677690, 320.5359728645732389 ) ) ;
#73658=DIRECTION ( 'NONE',  ( -2.900000000000000265E-14, 2.000000000000000155E-15, -1.000000000000000000 ) ) ;
#73659=EDGE_CURVE ( 'NONE', #72873, #8213, #34772, .T. ) ;
#73660=AXIS2_PLACEMENT_3D ( 'NONE', #58924, #29913, #64429 ) ;
#73661=FACE_OUTER_BOUND ( 'NONE', #51939, .T. ) ;
#73662=ORIENTED_EDGE ( 'NONE', *, *, #67522, .F. ) ;
#73664=CARTESIAN_POINT ( 'NONE',  ( 96.32141381413643444, -39.41948438522342713, 16.53372051400597798 ) ) ;
#73665=CARTESIAN_POINT ( 'NONE',  ( 107.6091111025649809, -48.61711588689897212, 38.61276813305397582 ) ) ;
#73667=EDGE_CURVE ( 'NONE', #54028, #73279, #8425, .T. ) ;
#73670=CARTESIAN_POINT ( 'NONE',  ( 97.06107015462058030, -37.99640499814212546, 147.4278258600957940 ) ) ;
#73671=EDGE_CURVE ( 'NONE', #22054, #18083, #48372, .T. ) ;
#73673=CARTESIAN_POINT ( 'NONE',  ( 132.8222787434396253, -39.18254450372684516, 7.982620440119482019 ) ) ;
#73674=VECTOR ( 'NONE', #41637, 1000.000000000000000 ) ;
#73676=DIRECTION ( 'NONE',  ( 0.000000000000000000, 1.000000000000000000, 0.000000000000000000 ) ) ;
#73677=VECTOR ( 'NONE', #49961, 1000.000000000000000 ) ;
#73679=EDGE_CURVE ( 'NONE', #23550, #40647, #27955, .T. ) ;
#73681=CARTESIAN_POINT ( 'NONE',  ( 97.03298259997053776, -33.74021148472603215, 31.09562527591097592 ) ) ;
#73682=CARTESIAN_POINT ( 'NONE',  ( 101.4046705256369734, -45.52519664383009257, 218.1213395616249784 ) ) ;
#73683=CARTESIAN_POINT ( 'NONE',  ( 110.3788355960759162, -47.29890920647816444, 48.80610146638797175 ) ) ;
#73686=CARTESIAN_POINT ( 'NONE',  ( 117.0715322531006990, -35.45947498896153860, 173.9259864712019521 ) ) ;
#73687=CARTESIAN_POINT ( 'NONE',  ( 188.5667039024479834, -48.82844715994099971, 137.2178068554150059 ) ) ;
#73689=VECTOR ( 'NONE', #59728, 1000.000000000000000 ) ;
#73694=ADVANCED_FACE ( 'NONE', ( #76106 ), #1660, .T. ) ;
#73695=CARTESIAN_POINT ( 'NONE',  ( 103.4440497394146092, -45.85039829771042719, 113.2756252759109827 ) ) ;
#73696=AXIS2_PLACEMENT_3D ( 'NONE', #76328, #26827, #62697 ) ;
#73698=VERTEX_POINT ( 'NONE', #43364 ) ;
#73699=CARTESIAN_POINT ( 'NONE',  ( 106.3035372762157493, -47.10473409126645805, 218.5184824187679453 ) ) ;
#73705=DIRECTION ( 'NONE',  ( -0.7071067811865774377, 0.7071067811865175967, -7.071067811865782003E-16 ) ) ;
#73707=CARTESIAN_POINT ( 'NONE',  ( 116.4020974974656042, -33.81230083437810663, 174.0670538473399347 ) ) ;
#73711=CARTESIAN_POINT ( 'NONE',  ( 103.7583319442197052, -28.50847317404091186, 126.8130118773259625 ) ) ;
#73712=CARTESIAN_POINT ( 'NONE',  ( 41.56670390244801894, -27.57844715994070484, -5.074374724088000832 ) ) ;
#73713=CARTESIAN_POINT ( 'NONE',  ( 101.2327472597882263, -44.62129728587211730, 253.0699109901961492 ) ) ;
#73715=DIRECTION ( 'NONE',  ( -1.000000000000000000, 0.000000000000000000, 0.000000000000000000 ) ) ;
#73717=DIRECTION ( 'NONE',  ( 1.000000000000000078E-15, -1.000000000000000083E-30, -1.000000000000000000 ) ) ;
#73718=DIRECTION ( 'NONE',  ( 0.000000000000000000, 0.000000000000000000, -1.000000000000000000 ) ) ;
#73719=PLANE ( 'NONE',  #66693 ) ;
#73721=CARTESIAN_POINT ( 'NONE',  ( 117.3921119255897452, -35.46056622170122097, 193.9241967044829664 ) ) ;
#73728=ADVANCED_FACE ( 'NONE', ( #62920 ), #22066, .T. ) ;
#73731=VECTOR ( 'NONE', #78621, 1000.000000000000000 ) ;
#73732=CARTESIAN_POINT ( 'NONE',  ( 117.0604406654448582, -38.08365174049107083, 63.71870391512912590 ) ) ;
#73733=CARTESIAN_POINT ( 'NONE',  ( 106.9404395787681352, -47.78219344473501451, 232.5794347997199907 ) ) ;
#73734=CARTESIAN_POINT ( 'NONE',  ( 107.0664832912739968, -36.72944715994100306, 287.6356252759109680 ) ) ;
#73735=ORIENTED_EDGE ( 'NONE', *, *, #88496, .T. ) ;
#73738=CARTESIAN_POINT ( 'NONE',  ( 86.06670390244796920, -48.82844715994099971, 250.9178068554150514 ) ) ;
#73739=CARTESIAN_POINT ( 'NONE',  ( 104.8541313898159757, -44.58662387026339502, 20.17666179816296435 ) ) ;
#73741=DIRECTION ( 'NONE',  ( 1.000000000000000000, 0.000000000000000000, 0.000000000000000000 ) ) ;
#73742=VERTEX_POINT ( 'NONE', #55184 ) ;
#73743=ADVANCED_FACE ( 'NONE', ( #84743 ), #28864, .T. ) ;
#73747=CARTESIAN_POINT ( 'NONE',  ( 81.36335724985904960, -16.30134337669397127, 7.962481652680392763 ) ) ;
#73749=ORIENTED_EDGE ( 'NONE', *, *, #37152, .T. ) ;
#73750=ADVANCED_FACE ( 'NONE', ( #82945 ), #28400, .T. ) ;
#73751=DIRECTION ( 'NONE',  ( 1.000000000000000078E-15, -1.000000000000000083E-30, -1.000000000000000000 ) ) ;
#73752=VERTEX_POINT ( 'NONE', #71108 ) ;
#73754=CARTESIAN_POINT ( 'NONE',  ( 163.5667039024460223, -18.82844715994111340, -5.074374724088000832 ) ) ;
#73755=AXIS2_PLACEMENT_3D ( 'NONE', #20373, #89414, #27172 ) ;
#73756=CARTESIAN_POINT ( 'NONE',  ( 113.0365282982730264, -42.83802263516175657, 72.61527697093394806 ) ) ;
#73757=CARTESIAN_POINT ( 'NONE',  ( 98.41658590534017037, -29.81029140585139814, 195.7775300378159784 ) ) ;
#73758=CARTESIAN_POINT ( 'NONE',  ( 109.8501361970267425, -26.70547878262030395, 174.8613395616249591 ) ) ;
#73759=CARTESIAN_POINT ( 'NONE',  ( 101.1175715082527660, -44.88412347719182804, 22.07575109432372074 ) ) ;
#73760=CARTESIAN_POINT ( 'NONE',  ( 106.8364377494367403, -47.15199802307920152, 268.5584824187679374 ) ) ;
#73761=CARTESIAN_POINT ( 'NONE',  ( 128.0667039024480118, -50.82844715994100682, 10.91780685541499807 ) ) ;
#73763=ORIENTED_EDGE ( 'NONE', *, *, #82972, .T. ) ;
#73765=CIRCLE ( 'NONE', #21532, 3.250000000000002665 ) ;
#73766=AXIS2_PLACEMENT_3D ( 'NONE', #78979, #52996, #31698 ) ;
#73768=CARTESIAN_POINT ( 'NONE',  ( 117.5184129516626257, -36.12626193255995588, 228.8727681330539667 ) ) ;
#73769=ORIENTED_EDGE ( 'NONE', *, *, #9684, .F. ) ;
#73770=CARTESIAN_POINT ( 'NONE',  ( 98.26116833961376074, -42.31097554054522902, 186.7756252759109543 ) ) ;
#73771=CARTESIAN_POINT ( 'NONE',  ( 172.5664832912729878, -18.82844715994071194, 18.92562527591200094 ) ) ;
#73773=CARTESIAN_POINT ( 'NONE',  ( 177.8371591254543489, -47.82818131005478079, 237.4678068554150059 ) ) ;
#73774=CARTESIAN_POINT ( 'NONE',  ( 80.06648329127399677, -18.72944715994105991, -5.074374724089057764 ) ) ;
#73775=EDGE_CURVE ( 'NONE', #56608, #84350, #49286, .T. ) ;
#73776=CARTESIAN_POINT ( 'NONE',  ( 110.8744162906118333, -29.68297622160992688, 277.6356252759108543 ) ) ;
#73777=DIRECTION ( 'NONE',  ( 0.000000000000000000, 1.000000000000000000, 0.000000000000000000 ) ) ;
#73778=CARTESIAN_POINT ( 'NONE',  ( 97.81170986510684884, -40.51745644794008427, 172.6354259520616097 ) ) ;
#73781=DIRECTION ( 'NONE',  ( 0.7071067811869283792, -0.7071067811861665442, 7.071067811868979848E-16 ) ) ;
#73783=CARTESIAN_POINT ( 'NONE',  ( 53.35959712126227572, -48.62134037875156878, 300.4678068554150059 ) ) ;
#73786=DIRECTION ( 'NONE',  ( -1.000000000000000078E-15, 1.000000000000000083E-30, 1.000000000000000000 ) ) ;
#73787=ORIENTED_EDGE ( 'NONE', *, *, #89495, .T. ) ;
#73788=AXIS2_PLACEMENT_3D ( 'NONE', #77930, #8896, #72882 ) ;
#73789=EDGE_CURVE ( 'NONE', #85398, #73516, #16833, .T. ) ;
#73790=DIRECTION ( 'NONE',  ( 0.7071067811865779928, -0.7071067811865171526, 7.071067811865786933E-16 ) ) ;
#73791=CARTESIAN_POINT ( 'NONE',  ( 112.4658351597014843, -45.71473303307890035, 238.0070538473389377 ) ) ;
#73792=CARTESIAN_POINT ( 'NONE',  ( 98.20239980326637408, -43.33262854484335946, 107.8480062282919647 ) ) ;
#73793=CARTESIAN_POINT ( 'NONE',  ( 113.1252749404788034, -46.02936877844707197, 219.0480062282919960 ) ) ;
#73794=DIRECTION ( 'NONE',  ( 0.000000000000000000, 1.000000000000000000, 0.000000000000000000 ) ) ;
#73795=DIRECTION ( 'NONE',  ( 0.000000000000000000, 0.000000000000000000, -1.000000000000000000 ) ) ;
#73796=CARTESIAN_POINT ( 'NONE',  ( 188.5667039024479834, -67.87844715994100397, 293.2178068554150627 ) ) ;
#73799=CARTESIAN_POINT ( 'NONE',  ( 132.9844404253379366, -21.25772566032916799, 1.807989669955668122 ) ) ;
#73800=AXIS2_PLACEMENT_3D ( 'NONE', #80076, #4652, #32338 ) ;
#73802=VERTEX_POINT ( 'NONE', #71990 ) ;
#73804=EDGE_CURVE ( 'NONE', #12675, #20444, #73649, .T. ) ;
#73805=CARTESIAN_POINT ( 'NONE',  ( 102.9824767429641525, -29.22764064321736299, 144.8952769709339634 ) ) ;
#73806=AXIS2_PLACEMENT_3D ( 'NONE', #14982, #20896, #49474 ) ;
#73808=ORIENTED_EDGE ( 'NONE', *, *, #43712, .T. ) ;
#73809=CARTESIAN_POINT ( 'NONE',  ( 113.2453749487971209, -28.75857822357426130, 89.55142878775579618 ) ) ;
#73810=CARTESIAN_POINT ( 'NONE',  ( 109.0680860650138300, -47.57644715601873742, 123.7337205140059666 ) ) ;
#73812=CARTESIAN_POINT ( 'NONE',  ( 79.41328093382365694, -16.05633243510679264, 8.161687850942282552 ) ) ;
#73813=DIRECTION ( 'NONE',  ( 0.000000000000000000, 0.000000000000000000, 1.000000000000000000 ) ) ;
#73814=CARTESIAN_POINT ( 'NONE',  ( 152.0368932755770288, -23.42844715993588522, 313.9678068554149490 ) ) ;
#73816=CARTESIAN_POINT ( 'NONE',  ( 116.0809032858471852, -32.84949784884745583, 79.14991099019697174 ) ) ;
#73817=VERTEX_POINT ( 'NONE', #85636 ) ;
#73818=ORIENTED_EDGE ( 'NONE', *, *, #32996, .F. ) ;
#73821=CARTESIAN_POINT ( 'NONE',  ( 103.2980200187117816, -27.06831524915196141, 166.3603871806719496 ) ) ;
#73823=CARTESIAN_POINT ( 'NONE',  ( 96.06648329127393993, -36.72944715994093912, 312.6356252759112522 ) ) ;
#73825=VECTOR ( 'NONE', #5405, 1000.000000000000000 ) ;
#73827=DIRECTION ( 'NONE',  ( 0.000000000000000000, 0.000000000000000000, -1.000000000000000000 ) ) ;
#73829=CARTESIAN_POINT ( 'NONE',  ( 97.28692064948100438, -31.62807703868913833, 90.93181575210196854 ) ) ;
#73830=EDGE_LOOP ( 'NONE', ( #65059, #12721, #50386, #38231 ) ) ;
#73831=VERTEX_POINT ( 'NONE', #86073 ) ;
#73834=DIRECTION ( 'NONE',  ( -4.237773401492740281E-14, 1.000000000000000000, 0.000000000000000000 ) ) ;
#73836=CARTESIAN_POINT ( 'NONE',  ( 108.3793409795780036, -28.17508408765456096, 142.7614237029239632 ) ) ;
#73842=DIRECTION ( 'NONE',  ( 0.000000000000000000, 0.000000000000000000, 1.000000000000000000 ) ) ;
#73844=ORIENTED_EDGE ( 'NONE', *, *, #57285, .T. ) ;
#73846=CARTESIAN_POINT ( 'NONE',  ( 114.9579445475069264, -42.99008164810605592, 194.7244404487539668 ) ) ;
#73848=LINE ( 'NONE', #39327, #26413 ) ;
#73852=VERTEX_POINT ( 'NONE', #18688 ) ;
#73854=ORIENTED_EDGE ( 'NONE', *, *, #15423, .F. ) ;
#73856=ORIENTED_EDGE ( 'NONE', *, *, #60966, .F. ) ;
#73857=ORIENTED_EDGE ( 'NONE', *, *, #81140, .T. ) ;
#73858=CARTESIAN_POINT ( 'NONE',  ( 113.6383730011278601, -31.09817814777808564, 227.2204713219719565 ) ) ;
#73860=CARTESIAN_POINT ( 'NONE',  ( 117.8983839226775387, -39.04577396070462214, 108.6708633711489824 ) ) ;
#73861=CARTESIAN_POINT ( 'NONE',  ( 98.73996931189270754, -42.96625968561445319, 66.83848241876793850 ) ) ;
#73862=CARTESIAN_POINT ( 'NONE',  ( 116.3186249068845939, -32.94868901192853627, 254.1356252759109395 ) ) ;
#73863=CARTESIAN_POINT ( 'NONE',  ( 193.0371591254586292, -47.82818131005411999, 180.4678068554150343 ) ) ;
#73864=CARTESIAN_POINT ( 'NONE',  ( 36.65249034007530327, -49.32844715994124130, 300.4678068554150059 ) ) ;
#73866=CARTESIAN_POINT ( 'NONE',  ( 99.10138041440774259, -45.50374834597938900, 152.9899109901969894 ) ) ;
#73867=CARTESIAN_POINT ( 'NONE',  ( 107.8173249548519692, -46.71069529603006032, 277.6356222035115024 ) ) ;
#73868=ORIENTED_EDGE ( 'NONE', *, *, #46506, .F. ) ;
#73869=DIRECTION ( 'NONE',  ( -1.000000000000000078E-15, 0.000000000000000000, -1.000000000000000000 ) ) ;
#73870=ORIENTED_EDGE ( 'NONE', *, *, #37087, .F. ) ;
#73871=ORIENTED_EDGE ( 'NONE', *, *, #52036, .T. ) ;
#73873=CARTESIAN_POINT ( 'NONE',  ( 134.0664832912740110, -8.350947159940998787, 308.6356252759119911 ) ) ;
#73874=CARTESIAN_POINT ( 'NONE',  ( 90.44969454456413871, -50.82895651782494895, 239.5838068554169809 ) ) ;
#73875=ORIENTED_EDGE ( 'NONE', *, *, #25159, .F. ) ;
#73878=CARTESIAN_POINT ( 'NONE',  ( 115.0372574989604288, -42.90846257669011976, 178.3022919417056471 ) ) ;
#73879=CARTESIAN_POINT ( 'NONE',  ( 108.5379876179846264, -26.40851185940291046, 104.9641967044819779 ) ) ;
#73881=CARTESIAN_POINT ( 'NONE',  ( 180.2143765759489895, -35.91149509761070391, -5.074374724088000832 ) ) ;
#73882=DIRECTION ( 'NONE',  ( 0.000000000000000000, 0.000000000000000000, -1.000000000000000000 ) ) ;
#73883=CARTESIAN_POINT ( 'NONE',  ( 109.5220866130624984, -46.80460460589471694, 87.75467289495897205 ) ) ;
#73885=CARTESIAN_POINT ( 'NONE',  ( 109.8501361970267425, -26.70547878262040342, 170.8613395616249591 ) ) ;
#73886=CARTESIAN_POINT ( 'NONE',  ( 97.06115785756830405, -37.99686386286577999, 61.42732787508487036 ) ) ;
#73889=ORIENTED_EDGE ( 'NONE', *, *, #18534, .T. ) ;
#73891=CARTESIAN_POINT ( 'NONE',  ( 177.4809174648213741, -49.32844715993478957, 300.4678068554149490 ) ) ;
#73892=EDGE_CURVE ( 'NONE', #61198, #61470, #51514, .T. ) ;
#73893=LINE ( 'NONE', #46162, #65928 ) ;
#73895=CARTESIAN_POINT ( 'NONE',  ( 115.8270178786686841, -31.73274795042722829, 134.2399272767322884 ) ) ;
#73897=CARTESIAN_POINT ( 'NONE',  ( 117.3784280654263341, -34.92100556036569259, 243.9641967044819637 ) ) ;
#73900=CARTESIAN_POINT ( 'NONE',  ( 102.0668330567940387, -27.97062182092777149, 145.4898119003854902 ) ) ;
#73901=CARTESIAN_POINT ( 'NONE',  ( 106.8359569501641744, -47.17378133968975362, 268.5584824187679374 ) ) ;
#73902=CARTESIAN_POINT ( 'NONE',  ( 108.7502231993919395, -25.75847702231262204, 140.9432443235299672 ) ) ;
#73905=CIRCLE ( 'NONE', #27477, 16.72999999999999332 ) ;
#73907=CARTESIAN_POINT ( 'NONE',  ( 116.8174729601854835, -34.15427434069496115, 265.0316169617216815 ) ) ;
#73908=ORIENTED_EDGE ( 'NONE', *, *, #33170, .T. ) ;
#73909=B_SPLINE_CURVE_WITH_KNOTS ( 'NONE', 3,
 ( #19477, #13122, #40806, #68076, #54411, #40362, #20386, #48056, #74445, #19027, #68528, #76230, #48488, #82174, #12671, #47160, #34439, #41242, #7198, #19929, #6740, #67625, #82625, #46714, #12220, #26288, #13557, #89424, #6296, #68973, #14004 ),
 .UNSPECIFIED., .F., .F.,
 ( 4, 2, 2, 2, 2, 2, 2, 2, 2, 2, 2, 2, 1, 1, 1, 2, 4 ),
 ( 0.000000000000000000, 0.03125570353835087356, 0.06251140707670174712, 0.09376711061505262068, 0.1250228141534034942, 0.1875342212301058242, 0.2500456283068081542, 0.3125570353835104842, 0.3750684424602129807, 0.4375798495369154217, 0.4688355530752666422, 0.4844634048444423358, 0.4922773307290300160, 0.4961842936713238839, 0.4981377751424709288, 0.4991145158780446733, 0.5000912566136184179 ),
 .UNSPECIFIED. ) ;
#73910=VERTEX_POINT ( 'NONE', #75001 ) ;
#73911=ORIENTED_EDGE ( 'NONE', *, *, #31923, .F. ) ;
#73912=ADVANCED_FACE ( 'NONE', ( #48167 ), #33218, .T. ) ;
#73913=CONICAL_SURFACE ( 'NONE', #76831, 1.258750000000002922, 1.029744258676650093 ) ;
#73914=ORIENTED_EDGE ( 'NONE', *, *, #84383, .F. ) ;
#73916=CARTESIAN_POINT ( 'NONE',  ( 117.4658636684176543, -37.01502254527064650, 39.80419670448193159 ) ) ;
#73917=FACE_OUTER_BOUND ( 'NONE', #36814, .T. ) ;
#73918=EDGE_CURVE ( 'NONE', #31858, #87649, #5998, .T. ) ;
#73920=AXIS2_PLACEMENT_3D ( 'NONE', #12582, #68886, #290 ) ;
#73921=CARTESIAN_POINT ( 'NONE',  ( 41.56648329127399677, -18.82844715994099971, 138.9256252759119832 ) ) ;
#73922=CARTESIAN_POINT ( 'NONE',  ( 116.3181333158508295, -32.94392590426259204, 50.13562527591097506 ) ) ;
#73923=CARTESIAN_POINT ( 'NONE',  ( 115.1439687268531600, -40.82418761129420659, 247.8876579233149755 ) ) ;
#73924=VERTEX_POINT ( 'NONE', #48607 ) ;
#73930=CARTESIAN_POINT ( 'NONE',  ( 109.6431719188696263, -46.48004672784288260, 102.7812855322859917 ) ) ;
#73932=CARTESIAN_POINT ( 'NONE',  ( 107.0664832912739541, -22.72944715994095688, 312.1356252759112522 ) ) ;
#73933=CARTESIAN_POINT ( 'NONE',  ( 102.2363890476183599, -29.29987999758196793, 21.96729759161197748 ) ) ;
#73935=CONICAL_SURFACE ( 'NONE', #34764, 5.799999999999998934, 0.7853981633974369547 ) ;
#73936=CARTESIAN_POINT ( 'NONE',  ( 105.7976179630505413, -26.72429355889029168, 175.1774430963942848 ) ) ;
#73938=CARTESIAN_POINT ( 'NONE',  ( 116.7002268312856188, -35.03994406823839114, 243.9641967044829585 ) ) ;
#73940=ORIENTED_EDGE ( 'NONE', *, *, #60133, .T. ) ;
#73941=DIRECTION ( 'NONE',  ( 4.299999999999999979E-14, -1.000000000000000000, 0.000000000000000000 ) ) ;
#73942=CIRCLE ( 'NONE', #43451, 15.99999999999999822 ) ;
#73943=LINE ( 'NONE', #60294, #69967 ) ;
#73944=ADVANCED_FACE ( 'NONE', ( #89085 ), #83621, .T. ) ;
#73945=CARTESIAN_POINT ( 'NONE',  ( 109.0838521367681864, -44.63893190664380484, 45.59380465530593796 ) ) ;
#73947=EDGE_CURVE ( 'NONE', #79544, #88157, #344, .T. ) ;
#73951=ORIENTED_EDGE ( 'NONE', *, *, #66702, .T. ) ;
#73952=LINE ( 'NONE', #32157, #63922 ) ;
#73955=CARTESIAN_POINT ( 'NONE',  ( 96.02342237304465300, -37.20891875426686823, 116.3489586092439652 ) ) ;
#73956=VERTEX_POINT ( 'NONE', #13669 ) ;
#73957=CARTESIAN_POINT ( 'NONE',  ( 100.1685590971342776, -42.59726720982692427, 76.32194363760098099 ) ) ;
#73958=LINE ( 'NONE', #25348, #79407 ) ;
#73959=CARTESIAN_POINT ( 'NONE',  ( 113.4424924140864590, -42.92691738999312889, 94.64444044875396855 ) ) ;
#73962=AXIS2_PLACEMENT_3D ( 'NONE', #74610, #18300, #12389 ) ;
#73963=CARTESIAN_POINT ( 'NONE',  ( 115.4621199703947241, -43.00579008905405232, 24.31562527591096767 ) ) ;
#73964=CARTESIAN_POINT ( 'NONE',  ( 98.34995908937969489, -31.65640510623499893, 181.9069259909072969 ) ) ;
#73965=ORIENTED_EDGE ( 'NONE', *, *, #87736, .F. ) ;
#73970=ORIENTED_EDGE ( 'NONE', *, *, #61069, .F. ) ;
#73972=DIRECTION ( 'NONE',  ( 0.000000000000000000, 1.000000000000000000, 2.000000000000000155E-15 ) ) ;
#73973=ORIENTED_EDGE ( 'NONE', *, *, #14668, .T. ) ;
#73974=CARTESIAN_POINT ( 'NONE',  ( 116.7002268312856188, -35.03994406823839114, 243.9641967044829585 ) ) ;
#73975=CARTESIAN_POINT ( 'NONE',  ( 112.0074966433228099, -27.97083403899759801, 124.6671618762774187 ) ) ;
#73976=CARTESIAN_POINT ( 'NONE',  ( 101.9936208482194075, -45.44607148560456267, 188.1564586008105664 ) ) ;
#73977=CARTESIAN_POINT ( 'NONE',  ( 105.9884228536615609, -26.36024887173286757, 46.15848241876796720 ) ) ;
#73978=CARTESIAN_POINT ( 'NONE',  ( 112.1429027457822656, -28.01486178590806730, 95.65578064394281910 ) ) ;
#73979=ORIENTED_EDGE ( 'NONE', *, *, #61756, .F. ) ;
#73982=EDGE_CURVE ( 'NONE', #10572, #49269, #40477, .T. ) ;
#73983=CARTESIAN_POINT ( 'NONE',  ( 71.24025061656124080, 8.642044024269685210, 542.9756252759101471 ) ) ;
#73984=EDGE_LOOP ( 'NONE', ( #45238, #58337, #22898, #30334 ) ) ;
#73985=AXIS2_PLACEMENT_3D ( 'NONE', #85079, #50072, #49621 ) ;
#73986=CARTESIAN_POINT ( 'NONE',  ( 134.0664832912740110, 0.2215528400590013880, 296.1531252759119752 ) ) ;
#73988=CARTESIAN_POINT ( 'NONE',  ( 109.9831304889623027, -26.74336511273919115, 259.8499109901965767 ) ) ;
#73989=DIRECTION ( 'NONE',  ( 0.000000000000000000, -1.000000000000000000, 0.000000000000000000 ) ) ;
#73990=CARTESIAN_POINT ( 'NONE',  ( 72.31648329127396835, -9.833000550534366724, 14.92562527591093691 ) ) ;
#73991=CARTESIAN_POINT ( 'NONE',  ( 78.80082187616059741, -39.17731672735968118, 1.873071027762776453 ) ) ;
#73992=CARTESIAN_POINT ( 'NONE',  ( 106.3060546692423145, -45.75354925581387278, 261.9200388756959796 ) ) ;
#73993=CARTESIAN_POINT ( 'NONE',  ( 63.03715912545740707, -46.82818131006017381, 117.4678068554150485 ) ) ;
#73994=CARTESIAN_POINT ( 'NONE',  ( 116.1047473792919504, -29.10330858331350612, 70.38419670448192278 ) ) ;
#73996=CARTESIAN_POINT ( 'NONE',  ( 117.6255004633147507, -33.30599276614662330, 134.0880062282919880 ) ) ;
#73998=DIRECTION ( 'NONE',  ( 0.000000000000000000, 1.000000000000000000, 0.000000000000000000 ) ) ;
#74000=CARTESIAN_POINT ( 'NONE',  ( 57.56670390244747892, -48.82844715994040286, 137.2178068554150911 ) ) ;
#74001=DIRECTION ( 'NONE',  ( 1.000000000000000078E-15, -1.000000000000000000, 0.000000000000000000 ) ) ;
#74003=FACE_OUTER_BOUND ( 'NONE', #85531, .T. ) ;
#74006=CARTESIAN_POINT ( 'NONE',  ( 97.80412552530029302, -40.49889735345233532, 51.63403232301700996 ) ) ;
#74007=CARTESIAN_POINT ( 'NONE',  ( 108.0109225731970213, -26.30163847990888826, 155.0041967044819557 ) ) ;
#74008=ORIENTED_EDGE ( 'NONE', *, *, #515, .T. ) ;
#74009=DIRECTION ( 'NONE',  ( 0.7071067811864656383, 0.7071067811866295072, 7.071067811864650974E-16 ) ) ;
#74010=VECTOR ( 'NONE', #24518, 1000.000000000000000 ) ;
#74012=DIRECTION ( 'NONE',  ( 0.000000000000000000, 0.000000000000000000, -1.000000000000000000 ) ) ;
#74015=CARTESIAN_POINT ( 'NONE',  ( 103.1663722902654001, -27.03741444506403724, 130.3813395616259925 ) ) ;
#74019=EDGE_LOOP ( 'NONE', ( #32390, #4605, #49609, #70762 ) ) ;
#74020=VECTOR ( 'NONE', #26079, 1000.000000000000000 ) ;
#74021=EDGE_CURVE ( 'NONE', #44052, #73924, #40917, .T. ) ;
#74023=CARTESIAN_POINT ( 'NONE',  ( 32.24491389930098251, -32.11662333284611748, -5.074374724088000832 ) ) ;
#74025=EDGE_CURVE ( 'NONE', #53911, #37008, #54969, .T. ) ;
#74026=CARTESIAN_POINT ( 'NONE',  ( 116.7951252645493128, -39.38782981807234052, 158.6147919403088906 ) ) ;
#74027=CARTESIAN_POINT ( 'NONE',  ( 162.5667039024470171, -33.35206098992711077, -5.074374724088000832 ) ) ;
#74028=LINE ( 'NONE', #87219, #53714 ) ;
#74031=VECTOR ( 'NONE', #9059, 1000.000000000000000 ) ;
#74032=EDGE_LOOP ( 'NONE', ( #21908, #31135, #78749, #78972 ) ) ;
#74033=CARTESIAN_POINT ( 'NONE',  ( 59.67079009362632291, -0.9310397146383332379, 540.9756252759101471 ) ) ;
#74034=CARTESIAN_POINT ( 'NONE',  ( 98.33750497493211640, -41.21483588869658377, 192.7041967044819728 ) ) ;
#74035=PLANE ( 'NONE',  #25447 ) ;
#74036=VERTEX_POINT ( 'NONE', #82736 ) ;
#74037=CARTESIAN_POINT ( 'NONE',  ( 117.2535196871929770, -41.18324016912737306, 54.49848241876692612 ) ) ;
#74038=CARTESIAN_POINT ( 'NONE',  ( 112.0515904353014065, -45.40454050051200596, 52.99152818533465137 ) ) ;
#74040=CARTESIAN_POINT ( 'NONE',  ( 97.80782893958210877, -40.50798467304517914, 22.63481380566990708 ) ) ;
#74041=AXIS2_PLACEMENT_3D ( 'NONE', #36041, #63755, #7888 ) ;
#74042=ORIENTED_EDGE ( 'NONE', *, *, #34828, .F. ) ;
#74044=ORIENTED_EDGE ( 'NONE', *, *, #18301, .F. ) ;
#74046=CARTESIAN_POINT ( 'NONE',  ( 114.7070687854681807, -41.21829243659817621, 234.8358690201829404 ) ) ;
#74048=CARTESIAN_POINT ( 'NONE',  ( 164.7830935719599381, -29.99615139350823867, 342.9256252759109884 ) ) ;
#74051=AXIS2_PLACEMENT_3D ( 'NONE', #33089, #67610, #54844 ) ;
#74052=DIRECTION ( 'NONE',  ( 0.000000000000000000, 0.000000000000000000, -1.000000000000000000 ) ) ;
#74053=EDGE_LOOP ( 'NONE', ( #88994, #26652, #37154, #22964 ) ) ;
#74057=CARTESIAN_POINT ( 'NONE',  ( 97.10456541990245682, -39.80308206185652864, 21.56419670448195092 ) ) ;
#74060=CARTESIAN_POINT ( 'NONE',  ( 114.2324904129858112, -40.69568343359240714, 261.2423760838772182 ) ) ;
#74062=CARTESIAN_POINT ( 'NONE',  ( 48.45959712129000252, -28.98061976758940617, 237.4678068554150059 ) ) ;
#74063=AXIS2_PLACEMENT_3D ( 'NONE', #75576, #46492, #68307 ) ;
#74064=DIRECTION ( 'NONE',  ( 1.000000000000000078E-15, -1.000000000000000083E-30, -1.000000000000000000 ) ) ;
#74065=FACE_OUTER_BOUND ( 'NONE', #29642, .T. ) ;
#74066=CARTESIAN_POINT ( 'NONE',  ( 96.81585423491817721, -34.60398634006848795, 212.1641967044819808 ) ) ;
#74068=VERTEX_POINT ( 'NONE', #55427 ) ;
#74069=CARTESIAN_POINT ( 'NONE',  ( 106.6586400085135438, -26.26872808310278629, 81.10705384733896040 ) ) ;
#74070=EDGE_CURVE ( 'NONE', #18008, #28336, #20501, .T. ) ;
#74072=ORIENTED_EDGE ( 'NONE', *, *, #5625, .T. ) ;
#74075=ORIENTED_EDGE ( 'NONE', *, *, #27222, .F. ) ;
#74081=CARTESIAN_POINT ( 'NONE',  ( 115.7813752605596420, -41.80523413302275770, 153.4069233405687100 ) ) ;
#74082=CARTESIAN_POINT ( 'NONE',  ( 112.8963470814680932, -31.01156847455079912, 147.2623760838769726 ) ) ;
#74083=CARTESIAN_POINT ( 'NONE',  ( 118.0636334930051987, -35.40736804548507877, 234.9337205140059552 ) ) ;
#74084=EDGE_CURVE ( 'NONE', #34812, #72137, #19583, .T. ) ;
#74086=VERTEX_POINT ( 'NONE', #35903 ) ;
#74088=EDGE_CURVE ( 'NONE', #12758, #2876, #2295, .T. ) ;
#74090=ORIENTED_EDGE ( 'NONE', *, *, #72390, .F. ) ;
#74091=VERTEX_POINT ( 'NONE', #43152 ) ;
#74092=EDGE_CURVE ( 'NONE', #36659, #60843, #8210, .T. ) ;
#74094=AXIS2_PLACEMENT_3D ( 'NONE', #16894, #64152, #10079 ) ;
#74095=DIRECTION ( 'NONE',  ( -1.000000000000000078E-15, 0.000000000000000000, 1.000000000000000000 ) ) ;
#74096=ORIENTED_EDGE ( 'NONE', *, *, #76222, .F. ) ;
#74100=ADVANCED_FACE ( 'NONE', ( #43600 ), #1847, .T. ) ;
#74102=CARTESIAN_POINT ( 'NONE',  ( 115.3083805796901373, -34.38525866856544866, 148.4695626852189605 ) ) ;
#74103=CARTESIAN_POINT ( 'NONE',  ( 98.38709084977145380, -42.09077886617859576, 11.76800622829193799 ) ) ;
#74109=ORIENTED_EDGE ( 'NONE', *, *, #54678, .F. ) ;
#74110=CIRCLE ( 'NONE', #42191, 2.500000000000002220 ) ;
#74113=CARTESIAN_POINT ( 'NONE',  ( 119.2637946045970097, -42.39761235918182791, 6.826283056785802827 ) ) ;
#74119=EDGE_LOOP ( 'NONE', ( #62795, #54635 ) ) ;
#74120=CARTESIAN_POINT ( 'NONE',  ( 106.2504075017224210, -26.27849585604564098, 25.13848241876792855 ) ) ;
#74121=CARTESIAN_POINT ( 'NONE',  ( 98.55462967347544634, -43.85305904914448405, 67.86895860924497015 ) ) ;
#74124=CARTESIAN_POINT ( 'NONE',  ( 184.5664832912740110, 15.62155284005900491, 323.8756252759109202 ) ) ;
#74125=CARTESIAN_POINT ( 'NONE',  ( 115.0889146834008585, -30.61764965368201175, 145.3442830127359571 ) ) ;
#74126=CARTESIAN_POINT ( 'NONE',  ( 105.8444747722200674, -25.33565403619829226, 322.4846826458744431 ) ) ;
#74127=CARTESIAN_POINT ( 'NONE',  ( 34.33598329127499227, -36.32844715994100682, -5.074374724088000832 ) ) ;
#74128=VECTOR ( 'NONE', #14344, 1000.000000000000000 ) ;
#74129=EDGE_CURVE ( 'NONE', #51804, #79942, #26332, .T. ) ;
#74130=DIRECTION ( 'NONE',  ( -1.000000000000000000, -6.055337108828351666E-16, 0.000000000000000000 ) ) ;
#74131=EDGE_CURVE ( 'NONE', #3441, #53911, #15483, .T. ) ;
#74133=EDGE_CURVE ( 'NONE', #76782, #28502, #69847, .T. ) ;
#74136=CARTESIAN_POINT ( 'NONE',  ( 112.7657546104280044, -27.20415503536211688, 54.65943479971996055 ) ) ;
#74137=CARTESIAN_POINT ( 'NONE',  ( 110.0520154068402263, -26.08705182471624795, 215.8708633711489711 ) ) ;
#74138=CARTESIAN_POINT ( 'NONE',  ( 101.6996507173639088, -27.72520905039313632, 81.50419670448295051 ) ) ;
#74141=DIRECTION ( 'NONE',  ( 1.000000000000000000, 0.000000000000000000, 0.000000000000000000 ) ) ;
#74145=CARTESIAN_POINT ( 'NONE',  ( 102.8368274790083490, -27.91052165842139487, 91.43276813305296002 ) ) ;
#74147=ORIENTED_EDGE ( 'NONE', *, *, #5807, .T. ) ;
#74149=CARTESIAN_POINT ( 'NONE',  ( 98.95962429139169103, -30.20966935044063462, 236.7870538473399336 ) ) ;
#74150=CARTESIAN_POINT ( 'NONE',  ( 48.45959712127301344, -26.00627455219131789, -5.074374724088000832 ) ) ;
#74151=LINE ( 'NONE', #18279, #31856 ) ;
#74153=CARTESIAN_POINT ( 'NONE',  ( 104.4899544671745844, -26.97880758085721808, 81.28145860801052436 ) ) ;
#74157=CARTESIAN_POINT ( 'NONE',  ( 116.2045471004838078, -43.06251688283441581, 163.3441967044829823 ) ) ;
#74158=VERTEX_POINT ( 'NONE', #77252 ) ;
#74160=CARTESIAN_POINT ( 'NONE',  ( 113.5773531717103282, -42.74084067657960162, 119.6644404487539646 ) ) ;
#74161=AXIS2_PLACEMENT_3D ( 'NONE', #3160, #71317, #9085 ) ;
#74162=CARTESIAN_POINT ( 'NONE',  ( 41.56648329127398966, -18.82844715994071194, 78.92562527591199739 ) ) ;
#74163=CARTESIAN_POINT ( 'NONE',  ( 114.5610390845466071, -30.44493693613353358, 265.3813395616247135 ) ) ;
#74164=CARTESIAN_POINT ( 'NONE',  ( 194.5664832912739826, 12.92155284005902516, 333.4006252759108975 ) ) ;
#74165=CARTESIAN_POINT ( 'NONE',  ( 130.5667039024480118, -36.72944715994093912, 218.8274735512161158 ) ) ;
#74167=CARTESIAN_POINT ( 'NONE',  ( 116.3212776292297406, -32.94146857471347545, 140.1356252759109680 ) ) ;
#74169=CARTESIAN_POINT ( 'NONE',  ( 29.56648329127298069, -81.37844715994266664, 361.9756252759109998 ) ) ;
#74172=CARTESIAN_POINT ( 'NONE',  ( 117.9257662994440494, -34.79559216868040039, 198.9546728949589749 ) ) ;
#74173=DIRECTION ( 'NONE',  ( 0.000000000000000000, 0.000000000000000000, 1.000000000000000000 ) ) ;
#74174=EDGE_LOOP ( 'NONE', ( #82138, #29257 ) ) ;
#74176=VECTOR ( 'NONE', #55691, 1000.000000000000000 ) ;
#74178=CARTESIAN_POINT ( 'NONE',  ( 77.66889017811094220, -17.37024878619161683, 2.654395752941510978 ) ) ;
#74179=LINE ( 'NONE', #53247, #38875 ) ;
#74181=AXIS2_PLACEMENT_3D ( 'NONE', #19385, #68880, #46621 ) ;
#74182=CARTESIAN_POINT ( 'NONE',  ( 108.4139369173698242, -26.73458070908401041, 94.96924584189345353 ) ) ;
#74183=VERTEX_POINT ( 'NONE', #29100 ) ;
#74185=EDGE_CURVE ( 'NONE', #18386, #87456, #22745, .T. ) ;
#74186=CARTESIAN_POINT ( 'NONE',  ( 107.2431713256043224, -47.18863871633809026, 212.5899109901969837 ) ) ;
#74187=EDGE_CURVE ( 'NONE', #15780, #73586, #24381, .T. ) ;
#74195=DIRECTION ( 'NONE',  ( -1.000000000000000000, 0.000000000000000000, -1.000000000000000078E-15 ) ) ;
#74196=AXIS2_PLACEMENT_3D ( 'NONE', #88874, #40703, #61149 ) ;
#74197=CARTESIAN_POINT ( 'NONE',  ( 99.45988105884268293, -33.69262468827373169, 38.84237608387697094 ) ) ;
#74198=CARTESIAN_POINT ( 'NONE',  ( 111.8040564975826356, -25.84011059577494152, 130.7499109901969518 ) ) ;
#74199=EDGE_CURVE ( 'NONE', #19039, #25006, #17259, .T. ) ;
#74201=ORIENTED_EDGE ( 'NONE', *, *, #70688, .T. ) ;
#74204=CARTESIAN_POINT ( 'NONE',  ( 80.06648329127401098, -33.97944715994105991, 1.625625275910943746 ) ) ;
#74206=ORIENTED_EDGE ( 'NONE', *, *, #80515, .F. ) ;
#74207=EDGE_CURVE ( 'NONE', #8128, #27831, #10876, .T. ) ;
#74208=DIRECTION ( 'NONE',  ( -4.237773401492740281E-14, 1.000000000000000000, 0.000000000000000000 ) ) ;
#74209=VERTEX_POINT ( 'NONE', #31762 ) ;
#74210=ORIENTED_EDGE ( 'NONE', *, *, #22350, .T. ) ;
#74211=PLANE ( 'NONE',  #58651 ) ;
#74212=EDGE_CURVE ( 'NONE', #38962, #48829, #59458, .T. ) ;
#74213=CARTESIAN_POINT ( 'NONE',  ( 114.9961339231967798, -33.55505389859023069, 53.55241982807695678 ) ) ;
#74214=CARTESIAN_POINT ( 'NONE',  ( 117.7991783922927738, -31.64581934375353711, 214.1784824187679419 ) ) ;
#74215=CIRCLE ( 'NONE', #43726, 6.571100913904396990 ) ;
#74216=CARTESIAN_POINT ( 'NONE',  ( 113.5515132932711566, -44.90922781482916548, 168.1099109901969939 ) ) ;
#74217=CARTESIAN_POINT ( 'NONE',  ( 104.8309510432842444, -46.56975234077351189, 22.39971745899171651 ) ) ;
#74218=CARTESIAN_POINT ( 'NONE',  ( 115.4270991047690558, -42.97960947038945534, 24.31562527591096767 ) ) ;
#74219=PLANE ( 'NONE',  #62277 ) ;
#74221=ORIENTED_EDGE ( 'NONE', *, *, #80774, .T. ) ;
#74223=AXIS2_PLACEMENT_3D ( 'NONE', #57701, #23648, #36376 ) ;
#74224=EDGE_CURVE ( 'NONE', #20434, #30630, #66922, .T. ) ;
#74225=AXIS2_PLACEMENT_3D ( 'NONE', #68404, #27951, #77456 ) ;
#74227=CARTESIAN_POINT ( 'NONE',  ( 107.5119097530387933, -47.18928756557821202, 237.6099109901969655 ) ) ;
#74229=CARTESIAN_POINT ( 'NONE',  ( 98.53748378420890219, -30.73418253943381728, 205.8384824187679669 ) ) ;
#74230=DIRECTION ( 'NONE',  ( 1.000000000000000000, 3.999999999999999995E-14, 1.000000000000000078E-15 ) ) ;
#74231=DIRECTION ( 'NONE',  ( -0.7071067811865171526, -0.7071067811865779928, 2.899137802864853973E-29 ) ) ;
#74232=DIRECTION ( 'NONE',  ( 0.000000000000000000, 1.000000000000000000, 0.000000000000000000 ) ) ;
#74233=CARTESIAN_POINT ( 'NONE',  ( 111.9228550121644190, -44.05463541751552725, 277.6356252759109680 ) ) ;
#74234=CARTESIAN_POINT ( 'NONE',  ( 144.4532657278588204, -72.54451140298851897, 540.9756252759101471 ) ) ;
#74235=PLANE ( 'NONE',  #39433 ) ;
#74238=LINE ( 'NONE', #164, #84965 ) ;
#74239=CARTESIAN_POINT ( 'NONE',  ( 180.2121375201597573, -29.73316016638934300, 237.4678068554150059 ) ) ;
#74240=DIRECTION ( 'NONE',  ( -2.999999999999999839E-15, 1.000000000000000000, -2.999999999999999900E-30 ) ) ;
#74241=AXIS2_PLACEMENT_3D ( 'NONE', #37412, #30153, #65116 ) ;
#74244=ORIENTED_EDGE ( 'NONE', *, *, #70371, .T. ) ;
#74245=DIRECTION ( 'NONE',  ( 1.000000000000000078E-15, 0.000000000000000000, 1.000000000000000000 ) ) ;
#74246=CARTESIAN_POINT ( 'NONE',  ( 97.89977465614410335, -41.74121498826879417, 221.7241967044819546 ) ) ;
#74247=CARTESIAN_POINT ( 'NONE',  ( 109.2549746569086437, -46.95841770046993702, 103.7441967044829880 ) ) ;
#74248=CARTESIAN_POINT ( 'NONE',  ( 117.4559332992660075, -35.18111149946130922, 214.9441967044829767 ) ) ;
#74249=CARTESIAN_POINT ( 'NONE',  ( 152.0368932755772562, -23.42844715993587812, 193.9678068554149775 ) ) ;
#74253=LINE ( 'NONE', #12027, #73352 ) ;
#74254=CARTESIAN_POINT ( 'NONE',  ( 46.83715912545344651, -47.82818131006087015, 117.4678068554150485 ) ) ;
#74257=VECTOR ( 'NONE', #86708, 1000.000000000000000 ) ;
#74258=ORIENTED_EDGE ( 'NONE', *, *, #17102, .F. ) ;
#74259=ORIENTED_EDGE ( 'NONE', *, *, #87339, .F. ) ;
#74260=CARTESIAN_POINT ( 'NONE',  ( 112.6791402994794709, -29.62235551608389628, 123.9790864947439815 ) ) ;
#74261=CARTESIAN_POINT ( 'NONE',  ( 180.3521107875639871, -35.65087443492551245, 117.4678068554150627 ) ) ;
#74263=CARTESIAN_POINT ( 'NONE',  ( 97.06107483254703538, -37.99643385399256346, 91.42643104473111748 ) ) ;
#74264=CARTESIAN_POINT ( 'NONE',  ( 103.1828028919049984, -27.07824557232550688, 126.3813395616259783 ) ) ;
#74265=CARTESIAN_POINT ( 'NONE',  ( 25.56670390244797275, -62.87844715994099687, 290.4678068554150627 ) ) ;
#74266=AXIS2_PLACEMENT_3D ( 'NONE', #51862, #30110, #31431 ) ;
#74267=DIRECTION ( 'NONE',  ( 1.000000000000000000, 0.000000000000000000, 0.000000000000000000 ) ) ;
#74268=ADVANCED_FACE ( 'NONE', ( #18582 ), #46262, .F. ) ;
#74271=CARTESIAN_POINT ( 'NONE',  ( 100.8874678906910418, -44.70022137984270927, 108.0522919431911788 ) ) ;
#74272=CARTESIAN_POINT ( 'NONE',  ( 103.6990349130722251, -26.13358598113143216, 55.32133956162594046 ) ) ;
#74273=ORIENTED_EDGE ( 'NONE', *, *, #50225, .F. ) ;
#74275=VERTEX_POINT ( 'NONE', #60351 ) ;
#74276=EDGE_CURVE ( 'NONE', #18505, #40389, #56804, .T. ) ;
#74277=CARTESIAN_POINT ( 'NONE',  ( 177.8371591254543489, -47.82818131005477369, 249.9678068554149775 ) ) ;
#74278=CARTESIAN_POINT ( 'NONE',  ( 116.2045471004837083, -43.06251688283437318, 159.3441967044819592 ) ) ;
#74279=DIRECTION ( 'NONE',  ( 0.7071067811865473507, 0.000000000000000000, -0.7071067811865476838 ) ) ;
#74280=CARTESIAN_POINT ( 'NONE',  ( 163.1543517358360020, -31.62489322948790971, -5.074374724088000832 ) ) ;
#74283=CARTESIAN_POINT ( 'NONE',  ( 118.5256205435843526, -36.72944715994100306, 311.6356252759112522 ) ) ;
#74284=CARTESIAN_POINT ( 'NONE',  ( 99.04403034142228535, -42.84121029749736920, 177.8439541681125036 ) ) ;
#74285=CARTESIAN_POINT ( 'NONE',  ( 117.9791962420231073, -38.33460093242097599, 73.72229194257801055 ) ) ;
#74286=VERTEX_POINT ( 'NONE', #44493 ) ;
#74287=ORIENTED_EDGE ( 'NONE', *, *, #21524, .T. ) ;
#74290=VECTOR ( 'NONE', #43501, 1000.000000000000000 ) ;
#74291=DIRECTION ( 'NONE',  ( 0.000000000000000000, 0.000000000000000000, 1.000000000000000000 ) ) ;
#74292=CARTESIAN_POINT ( 'NONE',  ( 98.91056109567942656, -37.06209505544900651, 159.1766617981629679 ) ) ;
#74293=EDGE_CURVE ( 'NONE', #89909, #61092, #9996, .T. ) ;
#74294=ADVANCED_FACE ( 'NONE', ( #58567 ), #86297, .T. ) ;
#74295=EDGE_CURVE ( 'NONE', #67028, #14919, #69427, .T. ) ;
#74301=VERTEX_POINT ( 'NONE', #88539 ) ;
#74304=DIRECTION ( 'NONE',  ( -0.04216478779797398074, 0.9991106698809455455, 0.000000000000000000 ) ) ;
#74306=CARTESIAN_POINT ( 'NONE',  ( 109.9841060568515729, -28.36190534590500434, 206.2415833058969667 ) ) ;
#74307=EDGE_CURVE ( 'NONE', #41305, #25889, #20827, .T. ) ;
#74308=CARTESIAN_POINT ( 'NONE',  ( 51.56670390244676128, -33.35206098992666313, 193.9678068554150911 ) ) ;
#74309=CARTESIAN_POINT ( 'NONE',  ( 116.3216177720312317, -32.94249360885015676, 184.1356252759109680 ) ) ;
#74310=CYLINDRICAL_SURFACE ( 'NONE', #66253, 3.299999999999999822 ) ;
#74312=EDGE_LOOP ( 'NONE', ( #8630, #5713, #88620, #79301 ) ) ;
#74313=EDGE_CURVE ( 'NONE', #42339, #4876, #38002, .T. ) ;
#74314=AXIS2_PLACEMENT_3D ( 'NONE', #54290, #73869, #52931 ) ;
#74315=VERTEX_POINT ( 'NONE', #41692 ) ;
#74317=EDGE_CURVE ( 'NONE', #66479, #5006, #14008, .T. ) ;
#74318=AXIS2_PLACEMENT_3D ( 'NONE', #77934, #1636, #15258 ) ;
#74319=CARTESIAN_POINT ( 'NONE',  ( 114.4736784013144586, -40.22460793573437599, 226.2938046553059621 ) ) ;
#74320=CARTESIAN_POINT ( 'NONE',  ( 107.6042850712483698, -26.26048674992130572, 95.03562527591097364 ) ) ;
#74321=CARTESIAN_POINT ( 'NONE',  ( 96.94236579736387682, -32.35154040576531997, 61.01372051400599616 ) ) ;
#74322=CARTESIAN_POINT ( 'NONE',  ( 109.4816866186930326, -44.79096458540936254, 249.5838068554168672 ) ) ;
#74324=CYLINDRICAL_SURFACE ( 'NONE', #57643, 0.2500000000000002220 ) ;
#74325=CARTESIAN_POINT ( 'NONE',  ( 117.9325828832643026, -34.70414220975756336, 199.9851490854349549 ) ) ;
#74327=ORIENTED_EDGE ( 'NONE', *, *, #27845, .T. ) ;
#74328=LINE ( 'NONE', #33430, #85941 ) ;
#74330=VERTEX_POINT ( 'NONE', #47614 ) ;
#74331=DIRECTION ( 'NONE',  ( -6.524622321627019585E-16, -4.013151879589939944E-16, -1.000000000000000000 ) ) ;
#74332=EDGE_LOOP ( 'NONE', ( #77790, #61771 ) ) ;
#74333=CARTESIAN_POINT ( 'NONE',  ( 87.17003668186750076, -46.62589376934784013, -5.074374724089000033 ) ) ;
#74334=CARTESIAN_POINT ( 'NONE',  ( 116.7951252695739868, -39.38782979763659853, 178.6147919420326673 ) ) ;
#74335=CARTESIAN_POINT ( 'NONE',  ( 117.3389957193927131, -32.64844533837379004, 99.13943479972098771 ) ) ;
#74336=DIRECTION ( 'NONE',  ( 0.000000000000000000, 0.000000000000000000, 1.000000000000000000 ) ) ;
#74339=DIRECTION ( 'NONE',  ( -4.299999999999999979E-14, 1.000000000000000000, -4.400000000000000367E-29 ) ) ;
#74340=FACE_OUTER_BOUND ( 'NONE', #78677, .T. ) ;
#74341=CARTESIAN_POINT ( 'NONE',  ( 98.18688568738953393, -31.30898482519909365, 166.8899109901969950 ) ) ;
#74342=PLANE ( 'NONE',  #74196 ) ;
#74345=FACE_OUTER_BOUND ( 'NONE', #67786, .T. ) ;
#74348=CARTESIAN_POINT ( 'NONE',  ( 97.07198307494437017, -35.37891590512482054, 136.2191293735547788 ) ) ;
#74350=CARTESIAN_POINT ( 'NONE',  ( 96.97388998173752839, -33.94624283173551049, 251.1127681330538337 ) ) ;
#74352=CARTESIAN_POINT ( 'NONE',  ( 114.7884511584987024, -30.33054135350295866, 194.3769663851998928 ) ) ;
#74353=CARTESIAN_POINT ( 'NONE',  ( 111.0012107362514939, -46.40699640104500645, 278.8841967044824059 ) ) ;
#74354=CARTESIAN_POINT ( 'NONE',  ( 95.98172161192206886, -37.30002307145830542, 117.3794347997199594 ) ) ;
#74359=FACE_OUTER_BOUND ( 'NONE', #70172, .T. ) ;
#74360=CARTESIAN_POINT ( 'NONE',  ( 108.4174892948216211, -26.73503593412567625, 189.9689586058460122 ) ) ;
#74362=ORIENTED_EDGE ( 'NONE', *, *, #28451, .F. ) ;
#74363=AXIS2_PLACEMENT_3D ( 'NONE', #15552, #43227, #32947 ) ;
#74364=EDGE_LOOP ( 'NONE', ( #77218, #31964, #59153, #7951 ) ) ;
#74365=ORIENTED_EDGE ( 'NONE', *, *, #18307, .F. ) ;
#74366=EDGE_LOOP ( 'NONE', ( #78452, #78306, #53226, #81593, #20770, #1491 ) ) ;
#74367=FACE_BOUND ( 'NONE', #80075, .T. ) ;
#74368=CARTESIAN_POINT ( 'NONE',  ( 96.36668125800727580, -39.40815171121896299, 12.53372051400597442 ) ) ;
#74370=CARTESIAN_POINT ( 'NONE',  ( 133.6895842087618291, -33.97944715994099596, 1.625625275910995704 ) ) ;
#74371=VECTOR ( 'NONE', #26475, 1000.000000000000114 ) ;
#74373=CARTESIAN_POINT ( 'NONE',  ( 131.0667039024480118, -58.72944715994093201, 207.5838068554149913 ) ) ;
#74375=CARTESIAN_POINT ( 'NONE',  ( 99.32305605351064060, -40.33436967443800825, 256.0952769709339236 ) ) ;
#74376=ORIENTED_EDGE ( 'NONE', *, *, #9279, .F. ) ;
#74377=ORIENTED_EDGE ( 'NONE', *, *, #84383, .T. ) ;
#74378=ORIENTED_EDGE ( 'NONE', *, *, #46897, .T. ) ;
#74381=FACE_OUTER_BOUND ( 'NONE', #28570, .T. ) ;
#74382=CARTESIAN_POINT ( 'NONE',  ( 20.03715912545644073, -24.42818131006202265, 129.9678068554150627 ) ) ;
#74383=CARTESIAN_POINT ( 'NONE',  ( 25.56670390244719115, -42.82844715994178131, 173.2178068554150627 ) ) ;
#74384=CARTESIAN_POINT ( 'NONE',  ( 116.3114837287122754, -32.94280867712679850, 274.1356252759109680 ) ) ;
#74385=CARTESIAN_POINT ( 'NONE',  ( 97.95230308628410398, -39.01119097033267025, 12.96539282970593554 ) ) ;
#74388=CARTESIAN_POINT ( 'NONE',  ( 99.09505096938842428, -30.55130953284144724, 175.8023783150660790 ) ) ;
#74389=CARTESIAN_POINT ( 'NONE',  ( 105.9660763718858618, -46.48152545022894344, 282.4870538473400643 ) ) ;
#74390=CARTESIAN_POINT ( 'NONE',  ( 51.06648329127400388, 12.92155284005902516, 333.4006252759110112 ) ) ;
#74392=CARTESIAN_POINT ( 'NONE',  ( 21.56670390244696733, -23.42844715994183957, 300.4678068554150059 ) ) ;
#74393=DIRECTION ( 'NONE',  ( 0.9068632946707807507, -0.4214249218767881500, 1.031805784967618114E-15 ) ) ;
#74394=CARTESIAN_POINT ( 'NONE',  ( 115.6184857618795121, -38.05767108254817543, 66.50999513149596964 ) ) ;
#74395=CARTESIAN_POINT ( 'NONE',  ( 136.5456844410148278, -17.53793914064988257, 7.103892432643784005 ) ) ;
#74396=DIRECTION ( 'NONE',  ( 0.000000000000000000, 0.000000000000000000, -1.000000000000000000 ) ) ;
#74397=EDGE_CURVE ( 'NONE', #89511, #28842, #23504, .T. ) ;
#74398=CARTESIAN_POINT ( 'NONE',  ( 112.0658116054833897, -45.48845209930474454, 193.9897506056947236 ) ) ;
#74399=ORIENTED_EDGE ( 'NONE', *, *, #17869, .F. ) ;
#74400=CARTESIAN_POINT ( 'NONE',  ( 161.4809174648185603, -48.32844715993547169, 180.4678068554150059 ) ) ;
#74401=DIRECTION ( 'NONE',  ( -0.7071067811865274777, 0.7071067811865675568, -7.071067811865283048E-16 ) ) ;
#74402=VECTOR ( 'NONE', #5221, 1000.000000000000000 ) ;
#74404=ORIENTED_EDGE ( 'NONE', *, *, #33890, .F. ) ;
#74405=CARTESIAN_POINT ( 'NONE',  ( 96.69902036285651548, -37.82614351231516281, 126.4099109901969626 ) ) ;
#74408=CARTESIAN_POINT ( 'NONE',  ( 116.0152812585483275, -38.11929796734737863, 68.11432458998100969 ) ) ;
#74410=CARTESIAN_POINT ( 'NONE',  ( 111.9416332874190090, -45.54441269975540507, 99.41015473446796591 ) ) ;
#74414=CARTESIAN_POINT ( 'NONE',  ( 97.60264960697516301, -32.22222542080420027, 71.97276813305397525 ) ) ;
#74416=AXIS2_PLACEMENT_3D ( 'NONE', #3585, #31281, #58539 ) ;
#74417=CARTESIAN_POINT ( 'NONE',  ( 108.3332793974000765, -46.73487859761686991, 257.6771670143646702 ) ) ;
#74418=ORIENTED_EDGE ( 'NONE', *, *, #77656, .F. ) ;
#74419=DIRECTION ( 'NONE',  ( 1.000000000000000078E-15, -1.000000000000000083E-30, -1.000000000000000000 ) ) ;
#74423=LINE ( 'NONE', #60778, #597 ) ;
#74425=CARTESIAN_POINT ( 'NONE',  ( 101.2327472597881552, -44.62129728587218835, 257.0699109901973998 ) ) ;
#74426=CARTESIAN_POINT ( 'NONE',  ( 113.8576076518026383, -28.74447221003411812, 135.5156252759109634 ) ) ;
#74427=DIRECTION ( 'NONE',  ( 0.000000000000000000, -1.000000000000000000, 0.000000000000000000 ) ) ;
#74428=CARTESIAN_POINT ( 'NONE',  ( 107.0664832912739968, 19.62155284005901024, 333.4006252759110112 ) ) ;
#74429=CARTESIAN_POINT ( 'NONE',  ( 104.7595845749942782, -46.89609389129499561, 68.39848241876794077 ) ) ;
#74430=CARTESIAN_POINT ( 'NONE',  ( 115.8279189686416828, -31.73432177683753608, 95.23967231875141692 ) ) ;
#74431=ORIENTED_EDGE ( 'NONE', *, *, #13406, .T. ) ;
#74433=CARTESIAN_POINT ( 'NONE',  ( 105.7157274140183603, -46.72389631486497308, 158.4687971658879349 ) ) ;
#74438=CARTESIAN_POINT ( 'NONE',  ( 105.1635383257858507, -47.00901688944614421, 12.42991099019596923 ) ) ;
#74439=CARTESIAN_POINT ( 'NONE',  ( 194.0371591254573218, -24.42818131005417825, 249.9678068554149775 ) ) ;
#74440=CIRCLE ( 'NONE', #33845, 0.5000000000000197620 ) ;
#74442=CARTESIAN_POINT ( 'NONE',  ( 79.32178306375476495, -39.37853523628606212, 1.709393643967942245 ) ) ;
#74443=CARTESIAN_POINT ( 'NONE',  ( 99.27767200979357654, -42.52643314540505060, 261.2581341137909590 ) ) ;
#74444=TOROIDAL_SURFACE ( 'NONE', #9160, 11.75000000000000000, 2.125000000000000000 ) ;
#74445=CARTESIAN_POINT ( 'NONE',  ( 110.6885610099060244, -27.38152249298925867, 99.78298386793977670 ) ) ;
#74446=CARTESIAN_POINT ( 'NONE',  ( 116.2124334422529870, -31.77159869865918296, 65.22133956162595325 ) ) ;
#74448=CARTESIAN_POINT ( 'NONE',  ( 111.4357194830650002, -47.79916136671457849, 172.8756252759109771 ) ) ;
#74452=CARTESIAN_POINT ( 'NONE',  ( 41.56648329127499153, -32.07844715994070839, 83.67562527591201160 ) ) ;
#74454=CARTESIAN_POINT ( 'NONE',  ( 131.0667039024480118, -61.87844715994100397, 231.5838068554150198 ) ) ;
#74457=CARTESIAN_POINT ( 'NONE',  ( 95.73117830242222226, -40.35431382354642693, 131.5727681330539554 ) ) ;
#74458=ORIENTED_EDGE ( 'NONE', *, *, #6065, .F. ) ;
#74460=DIRECTION ( 'NONE',  ( -4.554376769437570034E-14, 1.000000000000000000, 0.000000000000000000 ) ) ;
#74463=DIRECTION ( 'NONE',  ( 0.000000000000000000, 0.000000000000000000, 1.000000000000000000 ) ) ;
#74464=DIRECTION ( 'NONE',  ( -3.999999999999999995E-14, 1.000000000000000000, -4.100000000000000342E-29 ) ) ;
#74465=ORIENTED_EDGE ( 'NONE', *, *, #41697, .F. ) ;
#74467=VECTOR ( 'NONE', #70460, 1000.000000000000000 ) ;
#74469=DIRECTION ( 'NONE',  ( -2.900000000000000265E-14, 2.000000000000000155E-15, -1.000000000000000000 ) ) ;
#74471=ORIENTED_EDGE ( 'NONE', *, *, #74921, .F. ) ;
#74472=AXIS2_PLACEMENT_3D ( 'NONE', #70934, #29139, #37743 ) ;
#74473=ORIENTED_EDGE ( 'NONE', *, *, #78649, .F. ) ;
#74476=CARTESIAN_POINT ( 'NONE',  ( 97.81170669197712186, -40.51744871389600178, 156.6352702525290681 ) ) ;
#74477=LINE ( 'NONE', #31344, #28443 ) ;
#74478=DIRECTION ( 'NONE',  ( -0.7071067811866279529, 0.7071067811864671926, -7.071067811866286874E-16 ) ) ;
#74480=LINE ( 'NONE', #33140, #12415 ) ;
#74482=ORIENTED_EDGE ( 'NONE', *, *, #12159, .T. ) ;
#74483=ADVANCED_FACE ( 'NONE', ( #27189 ), #12676, .F. ) ;
#74484=DIRECTION ( 'NONE',  ( 0.7071067811865453523, 0.000000000000000000, 0.7071067811865496822 ) ) ;
#74485=CARTESIAN_POINT ( 'NONE',  ( 116.5710038106514759, -34.42130396933982439, 205.0156252759109634 ) ) ;
#74486=DIRECTION ( 'NONE',  ( -1.000000000000000078E-15, 1.000000000000000083E-30, 1.000000000000000000 ) ) ;
#74487=ORIENTED_EDGE ( 'NONE', *, *, #62322, .F. ) ;
#74488=CARTESIAN_POINT ( 'NONE',  ( 115.1932381579439948, -43.17108053757041830, 44.30514908543392494 ) ) ;
#74489=CARTESIAN_POINT ( 'NONE',  ( 111.2436683438683644, -45.81674569873502634, 52.91934373813153769 ) ) ;
#74493=CARTESIAN_POINT ( 'NONE',  ( 116.3148031259206192, -32.94054721833379062, 24.13562527591095375 ) ) ;
#74496=CARTESIAN_POINT ( 'NONE',  ( 100.8499323319230854, -30.41416626502819298, 222.1272975916109544 ) ) ;
#74498=DIRECTION ( 'NONE',  ( -0.7071067811734105257, 0.7071067811996846197, 0.000000000000000000 ) ) ;
#74500=AXIS2_PLACEMENT_3D ( 'NONE', #934, #50863, #29535 ) ;
#74502=CARTESIAN_POINT ( 'NONE',  ( 82.74959284958354999, -37.33856210725883784, 3.004220725470468256 ) ) ;
#74507=CARTESIAN_POINT ( 'NONE',  ( 115.4447846419100472, -42.99283068281499709, 28.31562527591097123 ) ) ;
#74508=ORIENTED_EDGE ( 'NONE', *, *, #58271, .T. ) ;
#74511=CARTESIAN_POINT ( 'NONE',  ( 114.7858077920586908, -40.64262416812939449, 246.2833284648299639 ) ) ;
#74512=FACE_OUTER_BOUND ( 'NONE', #69760, .T. ) ;
#74513=CARTESIAN_POINT ( 'NONE',  ( 108.2029444874846007, -47.03713394308636708, 157.6518157521019532 ) ) ;
#74515=CARTESIAN_POINT ( 'NONE',  ( 151.0371591254585724, -46.82818131005582529, 180.4678068554149775 ) ) ;
#74516=LINE ( 'NONE', #12296, #46282 ) ;
#74517=CARTESIAN_POINT ( 'NONE',  ( 115.8125398181975783, -30.97623284308500757, 250.2899109901966028 ) ) ;
#74519=ORIENTED_EDGE ( 'NONE', *, *, #12279, .T. ) ;
#74520=CIRCLE ( 'NONE', #87562, 11.57110091390434192 ) ;
#74521=CARTESIAN_POINT ( 'NONE',  ( 104.0301208637212369, -47.40549519127628031, 63.36800622829197494 ) ) ;
#74522=DIRECTION ( 'NONE',  ( 0.000000000000000000, 0.000000000000000000, 1.000000000000000000 ) ) ;
#74524=ORIENTED_EDGE ( 'NONE', *, *, #65899, .T. ) ;
#74525=EDGE_LOOP ( 'NONE', ( #71278, #68644, #22277, #88463 ) ) ;
#74528=CIRCLE ( 'NONE', #78897, 0.5000000000000197620 ) ;
#74529=DIRECTION ( 'NONE',  ( 1.000000000000000078E-15, -1.000000000000000000, 0.000000000000000000 ) ) ;
#74530=CYLINDRICAL_SURFACE ( 'NONE', #21033, 2.517499999999998739 ) ;
#74531=EDGE_CURVE ( 'NONE', #20097, #36440, #14918, .T. ) ;
#74533=CARTESIAN_POINT ( 'NONE',  ( 108.9785397593094132, -44.66504833944034658, 130.5823760838769658 ) ) ;
#74534=CARTESIAN_POINT ( 'NONE',  ( 98.92566635982139189, -30.18235936901480443, 236.7870538473399336 ) ) ;
#74535=CARTESIAN_POINT ( 'NONE',  ( 188.5667039024484097, -48.82844715993431350, 254.7178068554150059 ) ) ;
#74538=CARTESIAN_POINT ( 'NONE',  ( 41.56648329127399677, -9.303447159940999356, 318.9256252759120116 ) ) ;
#74540=ORIENTED_EDGE ( 'NONE', *, *, #86610, .F. ) ;
#74541=PLANE ( 'NONE',  #37321 ) ;
#74542=ORIENTED_EDGE ( 'NONE', *, *, #7445, .F. ) ;
#74545=DIRECTION ( 'NONE',  ( -1.000000000000000078E-15, 1.000000000000000083E-30, 1.000000000000000000 ) ) ;
#74546=DIRECTION ( 'NONE',  ( 0.000000000000000000, 0.000000000000000000, 1.000000000000000000 ) ) ;
#74547=CARTESIAN_POINT ( 'NONE',  ( 110.6311418553464279, -45.76071711580824086, 172.2981341137909794 ) ) ;
#74548=CARTESIAN_POINT ( 'NONE',  ( 103.9442172157761917, -47.38141121271982570, 62.33753003781600199 ) ) ;
#74550=VERTEX_POINT ( 'NONE', #21273 ) ;
#74551=CARTESIAN_POINT ( 'NONE',  ( 107.0620278373210539, -36.73691869758540207, 394.9756252759100903 ) ) ;
#74552=ORIENTED_EDGE ( 'NONE', *, *, #88719, .T. ) ;
#74554=ORIENTED_EDGE ( 'NONE', *, *, #13852, .F. ) ;
#74557=CARTESIAN_POINT ( 'NONE',  ( 104.4073079673720343, -46.45785698206038461, 132.3648020700444761 ) ) ;
#74561=CARTESIAN_POINT ( 'NONE',  ( 111.3322245453084918, -27.19268589797737334, 24.74133956162494030 ) ) ;
#74562=CARTESIAN_POINT ( 'NONE',  ( 112.7653987728015323, -27.20474975302890996, 50.65943479972101215 ) ) ;
#74565=DIRECTION ( 'NONE',  ( 0.000000000000000000, 1.000000000000000000, 0.000000000000000000 ) ) ;
#74566=CARTESIAN_POINT ( 'NONE',  ( 194.0371591254585155, -46.82818131005407736, 117.4678068554150627 ) ) ;
#74568=CARTESIAN_POINT ( 'NONE',  ( 99.09571505209436282, -30.55042394618130785, 146.8027630058878401 ) ) ;
#74569=CARTESIAN_POINT ( 'NONE',  ( 149.4409906032288404, -0.9156555935619370423, 361.9756252759100335 ) ) ;
#74570=CARTESIAN_POINT ( 'NONE',  ( 51.56670390244899238, -32.29483332968450782, -5.074374724088000832 ) ) ;
#74572=ORIENTED_EDGE ( 'NONE', *, *, #70755, .F. ) ;
#74573=CARTESIAN_POINT ( 'NONE',  ( 99.03195499373370581, -44.38837911315224716, 36.92038718067297509 ) ) ;
#74574=CARTESIAN_POINT ( 'NONE',  ( 106.3019393658184129, -47.12646404140136269, 218.5184824187679453 ) ) ;
#74575=CARTESIAN_POINT ( 'NONE',  ( 116.1426067713721437, -29.07136428874337142, 70.38419670448192278 ) ) ;
#74577=CARTESIAN_POINT ( 'NONE',  ( 85.24325998657074877, -58.55267046464445002, -5.074374724089052435 ) ) ;
#74578=DIRECTION ( 'NONE',  ( 0.000000000000000000, 0.000000000000000000, -1.000000000000000000 ) ) ;
#74579=VECTOR ( 'NONE', #43437, 999.9999999999998863 ) ;
#74580=EDGE_CURVE ( 'NONE', #3629, #60265, #42584, .T. ) ;
#74581=VECTOR ( 'NONE', #72027, 1000.000000000000000 ) ;
#74582=CIRCLE ( 'NONE', #87622, 0.5000000000000004441 ) ;
#74583=CARTESIAN_POINT ( 'NONE',  ( 165.3359832912740046, -36.32844715994100682, -5.074374724088000832 ) ) ;
#74585=CARTESIAN_POINT ( 'NONE',  ( 98.75024281215311817, -42.92452016420547523, 107.8480062282919647 ) ) ;
#74589=CARTESIAN_POINT ( 'NONE',  ( 103.9458437887066111, -26.80522050874827755, 246.3184824187679567 ) ) ;
#74590=CARTESIAN_POINT ( 'NONE',  ( 108.3324760767353609, -46.73498777622212685, 253.6793502017058586 ) ) ;
#74591=CARTESIAN_POINT ( 'NONE',  ( 107.0664832912739968, -36.72944715994100306, 293.2242906452868851 ) ) ;
#74594=ADVANCED_FACE ( 'NONE', ( #83962, #64403 ), #37146, .F. ) ;
#74597=DIRECTION ( 'NONE',  ( 0.000000000000000000, 1.000000000000000000, 0.000000000000000000 ) ) ;
#74598=CARTESIAN_POINT ( 'NONE',  ( 114.0663967180213803, -29.08153105160599949, 154.4746728949589851 ) ) ;
#74600=ORIENTED_EDGE ( 'NONE', *, *, #71650, .T. ) ;
#74601=EDGE_CURVE ( 'NONE', #52429, #89126, #84459, .T. ) ;
#74602=CARTESIAN_POINT ( 'NONE',  ( 108.1315353547809224, -45.52682987947058280, 114.1044404487549571 ) ) ;
#74603=DIRECTION ( 'NONE',  ( 1.000000000000000078E-15, -1.000000000000000083E-30, -1.000000000000000000 ) ) ;
#74604=CARTESIAN_POINT ( 'NONE',  ( 112.1541913332956284, -45.76570811864959154, 253.9965776568629110 ) ) ;
#74605=CYLINDRICAL_SURFACE ( 'NONE', #36083, 2.116999999999980009 ) ;
#74606=FACE_OUTER_BOUND ( 'NONE', #37165, .T. ) ;
#74607=ADVANCED_FACE ( 'NONE', ( #9002 ), #8548, .F. ) ;
#74608=DIRECTION ( 'NONE',  ( -9.073094938289460781E-13, -1.000000000000000000, 0.000000000000000000 ) ) ;
#74609=CARTESIAN_POINT ( 'NONE',  ( 107.0664832912739968, -36.72944715994100306, 287.6356252759109680 ) ) ;
#74610=CARTESIAN_POINT ( 'NONE',  ( 134.0664832912740110, -36.72944715994100306, -5.074374724089001809 ) ) ;
#74611=LINE ( 'NONE', #33730, #80683 ) ;
#74612=CARTESIAN_POINT ( 'NONE',  ( 112.7681627534586681, -45.43114336468926950, 178.0384824187679556 ) ) ;
#74613=DIRECTION ( 'NONE',  ( 0.000000000000000000, 1.000000000000000000, 0.000000000000000000 ) ) ;
#74614=EDGE_LOOP ( 'NONE', ( #42827, #86712, #62681, #54544 ) ) ;
#74616=VERTEX_POINT ( 'NONE', #15369 ) ;
#74618=CARTESIAN_POINT ( 'NONE',  ( 78.88305248757605170, -16.24700279812641668, 1.845048209621644952 ) ) ;
#74619=CARTESIAN_POINT ( 'NONE',  ( 107.0664832912739541, -23.08981143457874197, 302.6356252759109680 ) ) ;
#74621=VECTOR ( 'NONE', #57707, 1000.000000000000000 ) ;
#74622=LINE ( 'NONE', #12400, #42661 ) ;
#74623=ORIENTED_EDGE ( 'NONE', *, *, #55826, .T. ) ;
#74624=CARTESIAN_POINT ( 'NONE',  ( 112.0640814316657412, -45.48941673008675224, 62.98962639481060677 ) ) ;
#74627=CARTESIAN_POINT ( 'NONE',  ( 110.1375194624030769, -26.11116931986236267, 214.8403871806729342 ) ) ;
#74628=DIRECTION ( 'NONE',  ( 0.000000000000000000, 0.000000000000000000, 1.000000000000000000 ) ) ;
#74630=ADVANCED_FACE ( 'NONE', ( #21733 ), #85317, .F. ) ;
#74631=DIRECTION ( 'NONE',  ( 3.999999999999999995E-14, -1.000000000000000000, 4.100000000000000342E-29 ) ) ;
#74633=ADVANCED_FACE ( 'NONE', ( #28518 ), #70776, .F. ) ;
#74634=CARTESIAN_POINT ( 'NONE',  ( 72.06648329127386887, -9.729447159941003065, 14.82207188531764430 ) ) ;
#74635=EDGE_CURVE ( 'NONE', #13404, #36163, #49405, .T. ) ;
#74636=CARTESIAN_POINT ( 'NONE',  ( 114.3647906391003630, -33.01227106732497418, 42.01951894101996032 ) ) ;
#74637=CARTESIAN_POINT ( 'NONE',  ( 108.2792189108890568, -26.31750842948725122, 125.9841967044819597 ) ) ;
#74638=CARTESIAN_POINT ( 'NONE',  ( 19.56670390244739721, -25.42844715994192129, 249.9678068554150059 ) ) ;
#74639=VERTEX_POINT ( 'NONE', #84862 ) ;
#74640=EDGE_CURVE ( 'NONE', #42455, #52237, #71229, .T. ) ;
#74641=DIRECTION ( 'NONE',  ( 0.000000000000000000, 0.000000000000000000, -1.000000000000000000 ) ) ;
#74642=CARTESIAN_POINT ( 'NONE',  ( 82.67897566168218759, -17.84952872353950681, 6.945088388038879401 ) ) ;
#74646=AXIS2_PLACEMENT_3D ( 'NONE', #25531, #53204, #80973 ) ;
#74648=AXIS2_PLACEMENT_3D ( 'NONE', #63538, #42622, #84901 ) ;
#74650=ORIENTED_EDGE ( 'NONE', *, *, #79577, .F. ) ;
#74652=AXIS2_PLACEMENT_3D ( 'NONE', #41473, #81514, #13349 ) ;
#74653=CARTESIAN_POINT ( 'NONE',  ( 107.7234663162357151, -28.21331511381966806, 69.43813411379096578 ) ) ;
#74654=AXIS2_PLACEMENT_3D ( 'NONE', #10550, #3740, #31430 ) ;
#74655=CARTESIAN_POINT ( 'NONE',  ( 113.0381276193345883, -46.05869713813741129, 218.0175300378159591 ) ) ;
#74656=AXIS2_PLACEMENT_3D ( 'NONE', #11366, #12719, #18175 ) ;
#74657=CARTESIAN_POINT ( 'NONE',  ( 98.02603654163375779, -30.41010087969369735, 160.8289586092449497 ) ) ;
#74658=DIRECTION ( 'NONE',  ( -0.7071067812162665778, -0.7071067811568285677, 2.899137802742881592E-29 ) ) ;
#74659=CARTESIAN_POINT ( 'NONE',  ( 105.3240584539683482, -26.47319898023377149, 11.20991099019697046 ) ) ;
#74661=CARTESIAN_POINT ( 'NONE',  ( 193.0371591254582881, -47.82818131005411999, 300.4678068554149490 ) ) ;
#74663=ORIENTED_EDGE ( 'NONE', *, *, #41356, .T. ) ;
#74664=CARTESIAN_POINT ( 'NONE',  ( 97.81192379525968761, -40.51799951135461697, 111.6356742260152402 ) ) ;
#74665=CARTESIAN_POINT ( 'NONE',  ( 96.72907894039983034, -34.86132901292410224, 241.1841967044819626 ) ) ;
#74667=CARTESIAN_POINT ( 'NONE',  ( 99.08584233156592802, -29.96666100724374715, 215.7670538473399517 ) ) ;
#74668=PLANE ( 'NONE',  #37010 ) ;
#74671=CARTESIAN_POINT ( 'NONE',  ( 46.83715912545339677, -47.82818131006086304, 180.4678068554150911 ) ) ;
#74673=CARTESIAN_POINT ( 'NONE',  ( 98.00685971283303388, -38.32702420013065137, 277.6356252759115932 ) ) ;
#74674=LINE ( 'NONE', #46496, #670 ) ;
#74677=LINE ( 'NONE', #40599, #45483 ) ;
#74678=LINE ( 'NONE', #41043, #10948 ) ;
#74679=DIRECTION ( 'NONE',  ( -0.9825752044165969590, -0.1858654558159821002, 0.000000000000000000 ) ) ;
#74680=LINE ( 'NONE', #6535, #68043 ) ;
#74682=EDGE_LOOP ( 'NONE', ( #57078, #65224, #42161, #8669, #14843, #22714, #76658, #43749, #1622, #70972, #74572, #64604 ) ) ;
#74684=CARTESIAN_POINT ( 'NONE',  ( 95.27000809083011745, -38.09955253919518015, 236.4184824187679510 ) ) ;
#74685=CARTESIAN_POINT ( 'NONE',  ( 107.6031410145815528, -26.28275719304336633, 91.03562527591097364 ) ) ;
#74686=CARTESIAN_POINT ( 'NONE',  ( 95.18190931754610062, -37.33608887137841492, 267.3670538473396618 ) ) ;
#74687=CARTESIAN_POINT ( 'NONE',  ( 49.21437657594998427, -35.91149509761070391, -5.074374724088000832 ) ) ;
#74688=PLANE ( 'NONE',  #46063 ) ;
#74690=CARTESIAN_POINT ( 'NONE',  ( 116.3214877775586018, -32.94188667902410117, 30.13562527591096085 ) ) ;
#74691=DIRECTION ( 'NONE',  ( -1.000000000000000000, 0.000000000000000000, 0.000000000000000000 ) ) ;
#74692=VECTOR ( 'NONE', #40158, 1000.000000000000000 ) ;
#74693=CARTESIAN_POINT ( 'NONE',  ( 133.0080215814340647, -21.26771232012911383, 1.799893082727315186 ) ) ;
#74694=ADVANCED_FACE ( 'NONE', ( #55755 ), #83502, .F. ) ;
#74695=CIRCLE ( 'NONE', #35517, 0.4999999999999932832 ) ;
#74696=EDGE_LOOP ( 'NONE', ( #22914, #58934, #38795, #14952, #54232 ) ) ;
#74699=CARTESIAN_POINT ( 'NONE',  ( 108.3628298334300268, -27.77214277553820665, 149.3962293518869444 ) ) ;
#74704=CARTESIAN_POINT ( 'NONE',  ( 116.7751801856527152, -32.99181816784840748, 135.1184824187679396 ) ) ;
#74705=CYLINDRICAL_SURFACE ( 'NONE', #30901, 9.999999999999998224 ) ;
#74709=CARTESIAN_POINT ( 'NONE',  ( 21.03689327557613709, -23.42844715994197813, 193.9678068554150627 ) ) ;
#74710=CARTESIAN_POINT ( 'NONE',  ( 108.3334481003509779, -46.73485935324176666, 108.6772919430070914 ) ) ;
#74711=CARTESIAN_POINT ( 'NONE',  ( 112.4079628628857677, -28.49644221148687251, 69.61848241876894861 ) ) ;
#74712=ORIENTED_EDGE ( 'NONE', *, *, #76438, .T. ) ;
#74713=ORIENTED_EDGE ( 'NONE', *, *, #62063, .T. ) ;
#74714=ORIENTED_EDGE ( 'NONE', *, *, #62831, .F. ) ;
#74715=ADVANCED_FACE ( 'NONE', ( #58025 ), #59794, .T. ) ;
#74717=DIRECTION ( 'NONE',  ( 0.000000000000000000, 0.000000000000000000, -1.000000000000000000 ) ) ;
#74719=CARTESIAN_POINT ( 'NONE',  ( 108.6395843534182291, -26.47938140272626484, 140.9432443235289725 ) ) ;
#74720=DIRECTION ( 'NONE',  ( 1.000000000000000000, 0.000000000000000000, 0.000000000000000000 ) ) ;
#74721=VECTOR ( 'NONE', #7829, 1000.000000000000000 ) ;
#74725=VECTOR ( 'NONE', #22101, 1000.000000000000000 ) ;
#74726=DIRECTION ( 'NONE',  ( 1.000000000000000000, 0.000000000000000000, 0.000000000000000000 ) ) ;
#74727=CARTESIAN_POINT ( 'NONE',  ( 142.8687636814963184, 5.654319119531125537, 543.8623766218582887 ) ) ;
#74729=CARTESIAN_POINT ( 'NONE',  ( 96.66103594285301881, -37.56076609107802255, 101.3899109901969524 ) ) ;
#74731=ADVANCED_FACE ( 'NONE', ( #58900 ), #24908, .F. ) ;
#74736=AXIS2_PLACEMENT_3D ( 'NONE', #42287, #62744, #77283 ) ;
#74737=CARTESIAN_POINT ( 'NONE',  ( 105.6960798208838384, -45.90617939248504342, 145.2766617981629622 ) ) ;
#74738=AXIS2_PLACEMENT_3D ( 'NONE', #16937, #44616, #64198 ) ;
#74742=DIRECTION ( 'NONE',  ( -0.000000000000000000, -0.000000000000000000, -1.000000000000000000 ) ) ;
#74743=CARTESIAN_POINT ( 'NONE',  ( 136.6493805748345380, -19.67376371870151175, 2.871651383882735331 ) ) ;
#74744=ORIENTED_EDGE ( 'NONE', *, *, #3845, .T. ) ;
#74745=ORIENTED_EDGE ( 'NONE', *, *, #89621, .T. ) ;
#74746=LINE ( 'NONE', #12524, #54958 ) ;
#74748=CARTESIAN_POINT ( 'NONE',  ( 109.2250051346758113, -28.10373483931914151, 196.3130118773259767 ) ) ;
#74749=EDGE_CURVE ( 'NONE', #65895, #85412, #72561, .T. ) ;
#74750=LINE ( 'NONE', #67036, #21143 ) ;
#74752=CARTESIAN_POINT ( 'NONE',  ( 134.0664832912740110, -46.72944715994100306, 4.925625275910997303 ) ) ;
#74754=ORIENTED_EDGE ( 'NONE', *, *, #30409, .T. ) ;
#74757=VERTEX_POINT ( 'NONE', #4411 ) ;
#74759=CARTESIAN_POINT ( 'NONE',  ( 100.7056284991137289, -31.61385801203766377, 238.6052332267339580 ) ) ;
#74760=CARTESIAN_POINT ( 'NONE',  ( 95.46334413863738177, -34.19939227723602926, 106.1556252759109640 ) ) ;
#74761=CARTESIAN_POINT ( 'NONE',  ( 109.9050689397999889, -46.77468768478704675, 72.79562527591099297 ) ) ;
#74762=CARTESIAN_POINT ( 'NONE',  ( 101.0001179910210141, -41.97448653419763787, 249.5838068554172366 ) ) ;
#74763=CARTESIAN_POINT ( 'NONE',  ( 131.4524275574068497, -17.85322059724320454, 6.943211687812105737 ) ) ;
#74764=CARTESIAN_POINT ( 'NONE',  ( 188.5667039024484950, -42.82844715993430640, 139.7178068554150059 ) ) ;
#74765=CARTESIAN_POINT ( 'NONE',  ( 114.8139851684208992, -29.70110827795256014, 205.4127681330539872 ) ) ;
#74767=VERTEX_POINT ( 'NONE', #78937 ) ;
#74770=ORIENTED_EDGE ( 'NONE', *, *, #27357, .T. ) ;
#74774=DIRECTION ( 'NONE',  ( 0.7071067811864656383, 0.7071067811866295072, 7.071067811864650974E-16 ) ) ;
#74777=CARTESIAN_POINT ( 'NONE',  ( 100.9531696234827933, -28.70820207419374626, 91.59410946087238869 ) ) ;
#74778=CARTESIAN_POINT ( 'NONE',  ( 97.93239114460148187, -31.63098981178377755, 110.9213395616259703 ) ) ;
#74779=CARTESIAN_POINT ( 'NONE',  ( 115.8281814637101377, -31.73477629227051366, 254.2397833965958114 ) ) ;
#74780=DIRECTION ( 'NONE',  ( -1.000000000000000000, -4.299999999999999979E-14, -1.000000000000000078E-15 ) ) ;
#74781=DIRECTION ( 'NONE',  ( 0.000000000000000000, 0.000000000000000000, 1.000000000000000000 ) ) ;
#74782=CARTESIAN_POINT ( 'NONE',  ( 112.0659116166449536, -45.48839626399238512, 143.9897919420481287 ) ) ;
#74783=DIRECTION ( 'NONE',  ( 0.7071067811865491270, -0.7071067811865459074, 7.071067811865492096E-16 ) ) ;
#74784=CARTESIAN_POINT ( 'NONE',  ( 117.7539631054256972, -31.66723592997637482, 210.1784824187679703 ) ) ;
#74787=VERTEX_POINT ( 'NONE', #72990 ) ;
#74789=AXIS2_PLACEMENT_3D ( 'NONE', #16171, #49321, #43850 ) ;
#74792=VECTOR ( 'NONE', #72595, 1000.000000000000000 ) ;
#74794=CARTESIAN_POINT ( 'NONE',  ( 105.6259887305572676, -47.09919361126699044, 257.4670538473392298 ) ) ;
#74797=CARTESIAN_POINT ( 'NONE',  ( 105.1635842947561343, -47.00881719185149876, 8.429910990196965770 ) ) ;
#74798=CARTESIAN_POINT ( 'NONE',  ( 103.7937703862009613, -26.78548768338485075, 161.3299109901969643 ) ) ;
#74799=DIRECTION ( 'NONE',  ( 1.000000000000000078E-15, -1.000000000000000083E-30, -1.000000000000000000 ) ) ;
#74800=DIRECTION ( 'NONE',  ( 1.000000000000000078E-15, 1.000000000000000083E-30, -1.000000000000000000 ) ) ;
#74802=EDGE_CURVE ( 'NONE', #54909, #22054, #71419, .T. ) ;
#74805=DIRECTION ( 'NONE',  ( -1.000000000000000078E-15, 0.000000000000000000, 1.000000000000000000 ) ) ;
#74806=DIRECTION ( 'NONE',  ( 1.071939472051879986E-15, 0.000000000000000000, 1.000000000000000000 ) ) ;
#74807=ORIENTED_EDGE ( 'NONE', *, *, #4865, .F. ) ;
#74808=VECTOR ( 'NONE', #72698, 1000.000000000000000 ) ;
#74809=EDGE_CURVE ( 'NONE', #47917, #32414, #38463, .T. ) ;
#74810=VERTEX_POINT ( 'NONE', #18023 ) ;
#74811=EDGE_CURVE ( 'NONE', #25056, #55605, #3954, .T. ) ;
#74816=CARTESIAN_POINT ( 'NONE',  ( 115.4270991047690558, -42.97960947038945534, 24.31562527591096767 ) ) ;
#74817=DIRECTION ( 'NONE',  ( 1.000000000000000078E-15, 1.000000000000000083E-30, -1.000000000000000000 ) ) ;
#74819=EDGE_CURVE ( 'NONE', #77225, #71373, #30811, .T. ) ;
#74820=CARTESIAN_POINT ( 'NONE',  ( 194.5667039024482960, -47.82844715993405771, 300.4678068554149490 ) ) ;
#74822=CARTESIAN_POINT ( 'NONE',  ( 106.6575247680289777, -45.29010455595041407, 246.9609912566479579 ) ) ;
#74823=ORIENTED_EDGE ( 'NONE', *, *, #5508, .F. ) ;
#74825=AXIS2_PLACEMENT_3D ( 'NONE', #58996, #86736, #24507 ) ;
#74827=EDGE_CURVE ( 'NONE', #61623, #15987, #80280, .T. ) ;
#74828=DIRECTION ( 'NONE',  ( -1.000000000000000000, -4.299999999999999979E-14, -1.000000000000000078E-15 ) ) ;
#74831=CARTESIAN_POINT ( 'NONE',  ( 50.96943157743500308, -34.03355364505722491, 342.9256252759109884 ) ) ;
#74832=DIRECTION ( 'NONE',  ( 0.000000000000000000, 0.000000000000000000, 1.000000000000000000 ) ) ;
#74833=CARTESIAN_POINT ( 'NONE',  ( 110.0319707555399447, -45.11204900458633915, 34.27872616304095033 ) ) ;
#74834=ADVANCED_FACE ( 'NONE', ( #11210 ), #32097, .F. ) ;
#74837=CARTESIAN_POINT ( 'NONE',  ( 112.3177584634463244, -44.98096486020163098, 263.0270538473400279 ) ) ;
#74838=DIRECTION ( 'NONE',  ( 0.000000000000000000, 0.000000000000000000, 1.000000000000000000 ) ) ;
#74841=LINE ( 'NONE', #26678, #73674 ) ;
#74842=CARTESIAN_POINT ( 'NONE',  ( 180.3521107875639871, -35.65087443492551245, 193.9678068554150059 ) ) ;
#74843=CARTESIAN_POINT ( 'NONE',  ( 102.2704046875766579, -44.67259270758150080, 49.96237608387698970 ) ) ;
#74844=CIRCLE ( 'NONE', #25550, 9.571100913904325935 ) ;
#74845=CIRCLE ( 'NONE', #70508, 9.571100913904340146 ) ;
#74847=CARTESIAN_POINT ( 'NONE',  ( 136.7727304466921510, -18.23917853420268287, 6.814128304789858426 ) ) ;
#74849=CYLINDRICAL_SURFACE ( 'NONE', #65002, 12.99999999999999822 ) ;
#74850=CARTESIAN_POINT ( 'NONE',  ( 177.4809174648214309, -49.32844715993478957, 249.9678068554149775 ) ) ;
#74851=ORIENTED_EDGE ( 'NONE', *, *, #26180, .T. ) ;
#74852=CARTESIAN_POINT ( 'NONE',  ( 25.56670390244745050, -48.82844715994178841, 170.7178068554150627 ) ) ;
#74853=ORIENTED_EDGE ( 'NONE', *, *, #60442, .T. ) ;
#74854=CARTESIAN_POINT ( 'NONE',  ( 101.5007711604877159, -27.91412646590841362, 110.5241967044819944 ) ) ;
#74855=VERTEX_POINT ( 'NONE', #26190 ) ;
#74856=CARTESIAN_POINT ( 'NONE',  ( 106.7337219657603100, -28.19449539544314476, 84.52956268522000016 ) ) ;
#74857=CARTESIAN_POINT ( 'NONE',  ( 97.81171347387959258, -40.51745984142272761, 22.63530404563221410 ) ) ;
#74858=CARTESIAN_POINT ( 'NONE',  ( 102.5524010923236915, -28.48932656383806972, 96.89491663923000431 ) ) ;
#74859=CARTESIAN_POINT ( 'NONE',  ( 167.7413838386819123, -48.33240602328260849, 180.4678068554150059 ) ) ;
#74860=ADVANCED_FACE ( 'NONE', ( #53859 ), #55206, .F. ) ;
#74862=CIRCLE ( 'NONE', #6707, 4.750000000000004441 ) ;
#74863=CARTESIAN_POINT ( 'NONE',  ( 117.9472974416529638, -41.48656121291797660, 54.49848241876792088 ) ) ;
#74865=CARTESIAN_POINT ( 'NONE',  ( 117.0719393226367515, -35.46284531538225337, 258.9272565253700122 ) ) ;
#74866=VERTEX_POINT ( 'NONE', #62042 ) ;
#74867=CARTESIAN_POINT ( 'NONE',  ( 77.31651901074906164, -18.90078909148962083, 3.101427792080710955 ) ) ;
#74868=EDGE_LOOP ( 'NONE', ( #5506, #34149, #41395, #1449, #60055, #73418 ) ) ;
#74870=VERTEX_POINT ( 'NONE', #61587 ) ;
#74872=ORIENTED_EDGE ( 'NONE', *, *, #65498, .F. ) ;
#74873=CARTESIAN_POINT ( 'NONE',  ( 96.02263050233423769, -38.01213896886783061, 236.4184824187689458 ) ) ;
#74874=CARTESIAN_POINT ( 'NONE',  ( 98.83948440537673719, -30.29086274794821065, 151.7984824187679465 ) ) ;
#74876=CARTESIAN_POINT ( 'NONE',  ( 113.1762138295820961, -44.75342279309901983, 129.0937539895759869 ) ) ;
#74877=CARTESIAN_POINT ( 'NONE',  ( 96.65662162753720565, -37.29271227441797265, 72.36991099019596163 ) ) ;
#74879=ORIENTED_EDGE ( 'NONE', *, *, #26338, .T. ) ;
#74880=DIRECTION ( 'NONE',  ( 0.000000000000000000, 0.000000000000000000, -1.000000000000000000 ) ) ;
#74881=EDGE_CURVE ( 'NONE', #66717, #51052, #32993, .T. ) ;
#74882=CARTESIAN_POINT ( 'NONE',  ( 116.7952875727523576, -39.38725125411153272, 159.6146818031017744 ) ) ;
#74885=EDGE_CURVE ( 'NONE', #59669, #71638, #88876, .T. ) ;
#74887=LINE ( 'NONE', #88528, #68735 ) ;
#74888=CARTESIAN_POINT ( 'NONE',  ( 117.4080659314679025, -35.59792815749687378, 278.9127681330539872 ) ) ;
#74891=DIRECTION ( 'NONE',  ( 0.000000000000000000, 0.000000000000000000, 1.000000000000000000 ) ) ;
#74892=CARTESIAN_POINT ( 'NONE',  ( 101.4801710200817126, -30.26808144278882651, 260.0667055423624561 ) ) ;
#74894=CARTESIAN_POINT ( 'NONE',  ( 114.0075736764522389, -28.98025818340847692, 110.4956252759109816 ) ) ;
#74896=CARTESIAN_POINT ( 'NONE',  ( 114.3747829841801149, -29.18355094256887838, 174.4641967044819637 ) ) ;
#74899=ORIENTED_EDGE ( 'NONE', *, *, #60728, .T. ) ;
#74900=FACE_OUTER_BOUND ( 'NONE', #75196, .T. ) ;
#74901=CARTESIAN_POINT ( 'NONE',  ( 141.0664832912740394, -46.72944715994099596, 14.67562527591100441 ) ) ;
#74905=CARTESIAN_POINT ( 'NONE',  ( 113.8721965385452677, -28.72731865945801744, 139.5156252759109634 ) ) ;
#74908=VECTOR ( 'NONE', #60534, 1000.000000000000000 ) ;
#74912=AXIS2_PLACEMENT_3D ( 'NONE', #40981, #49121, #75519 ) ;
#74921=EDGE_CURVE ( 'NONE', #49976, #6901, #4852, .T. ) ;
#74923=ORIENTED_EDGE ( 'NONE', *, *, #44066, .T. ) ;
#74924=LINE ( 'NONE', #48973, #45232 ) ;
#74926=CARTESIAN_POINT ( 'NONE',  ( 105.7154772392229063, -46.72385838064575125, 157.4689586019844683 ) ) ;
#74928=EDGE_CURVE ( 'NONE', #18950, #84106, #67514, .T. ) ;
#74929=CARTESIAN_POINT ( 'NONE',  ( 100.9545475257521332, -28.70712375422630558, 105.5939711813188495 ) ) ;
#74931=CARTESIAN_POINT ( 'NONE',  ( 97.07202417197602529, -35.37877911891951044, 181.2189852412958260 ) ) ;
#74932=VERTEX_POINT ( 'NONE', #34336 ) ;
#74934=DIRECTION ( 'NONE',  ( 1.000000000000000078E-15, -1.000000000000000083E-30, -1.000000000000000000 ) ) ;
#74935=CARTESIAN_POINT ( 'NONE',  ( 98.96845470676157674, -30.25173782105014197, 191.7775300378149836 ) ) ;
#74936=EDGE_CURVE ( 'NONE', #37298, #42164, #46610, .T. ) ;
#74937=CARTESIAN_POINT ( 'NONE',  ( 31.56670390244700641, -22.48495420874110806, 342.9256252759109884 ) ) ;
#74938=ORIENTED_EDGE ( 'NONE', *, *, #37476, .F. ) ;
#74939=CARTESIAN_POINT ( 'NONE',  ( 103.2241971045484519, -45.72390501747104707, 88.25562527591095829 ) ) ;
#74940=DIRECTION ( 'NONE',  ( 0.9242245927363033076, 0.3818493186865918321, 0.000000000000000000 ) ) ;
#74941=LINE ( 'NONE', #67218, #83358 ) ;
#74942=FACE_OUTER_BOUND ( 'NONE', #48528, .T. ) ;
#74944=CYLINDRICAL_SURFACE ( 'NONE', #39945, 29.00000000000000000 ) ;
#74945=EDGE_LOOP ( 'NONE', ( #26596, #10641 ) ) ;
#74946=VERTEX_POINT ( 'NONE', #40704 ) ;
#74947=CARTESIAN_POINT ( 'NONE',  ( 114.0241607691103809, -31.19294522270855907, 240.7930118773259665 ) ) ;
#74948=CARTESIAN_POINT ( 'NONE',  ( 101.9940466514257622, -45.44635550110415068, 53.15612750292554267 ) ) ;
#74951=CARTESIAN_POINT ( 'NONE',  ( 81.91406418435974501, -38.77438500683208389, 2.186796636968284080 ) ) ;
#74952=ORIENTED_EDGE ( 'NONE', *, *, #41999, .T. ) ;
#74956=CARTESIAN_POINT ( 'NONE',  ( 97.79211192542227593, -40.52543860420435351, 11.63562527591094309 ) ) ;
#74958=CARTESIAN_POINT ( 'NONE',  ( 102.1978417368446657, -43.31572210571547998, 254.8880903695915947 ) ) ;
#74959=CARTESIAN_POINT ( 'NONE',  ( 184.5667039024480118, -48.82844715994099971, 300.9178068554150514 ) ) ;
#74960=CARTESIAN_POINT ( 'NONE',  ( 116.2961327041338535, -39.96626766897450977, 133.5584824187689605 ) ) ;
#74963=CIRCLE ( 'NONE', #72060, 11.45913725231036118 ) ;
#74966=CARTESIAN_POINT ( 'NONE',  ( 107.5118819425545951, -47.18863449879560079, 233.6099109901969655 ) ) ;
#74967=DIRECTION ( 'NONE',  ( -1.000000000000000000, 0.000000000000000000, 0.000000000000000000 ) ) ;
#74969=AXIS2_PLACEMENT_3D ( 'NONE', #13798, #75586, #68319 ) ;
#74970=CARTESIAN_POINT ( 'NONE',  ( 117.0955297935745705, -31.97384786926005873, 60.19086337114898555 ) ) ;
#74971=CARTESIAN_POINT ( 'NONE',  ( 172.5664832912740110, -32.07844715994070839, 134.1756252759119832 ) ) ;
#74972=VECTOR ( 'NONE', #69829, 1000.000000000000114 ) ;
#74975=ORIENTED_EDGE ( 'NONE', *, *, #26423, .F. ) ;
#74976=ORIENTED_EDGE ( 'NONE', *, *, #66675, .T. ) ;
#74977=CARTESIAN_POINT ( 'NONE',  ( 108.4153923495580898, -26.73476988454487469, 159.9688923623228050 ) ) ;
#74978=CARTESIAN_POINT ( 'NONE',  ( 141.0235900724605074, -8.833000550534283235, -5.074374724088999145 ) ) ;
#74979=DIRECTION ( 'NONE',  ( -0.7071067811865453523, -0.7071067811865496822, -7.071067811865460542E-16 ) ) ;
#74980=FACE_OUTER_BOUND ( 'NONE', #67082, .T. ) ;
#74981=CARTESIAN_POINT ( 'NONE',  ( 112.4302714532559548, -29.93748856177429118, 122.3747570362579751 ) ) ;
#74982=CARTESIAN_POINT ( 'NONE',  ( 115.3407290770031324, -45.24761053976980918, 264.1899109901965517 ) ) ;
#74983=CARTESIAN_POINT ( 'NONE',  ( 41.56648329127381203, -27.82844715994070484, 261.9256252759120116 ) ) ;
#74984=ORIENTED_EDGE ( 'NONE', *, *, #54097, .F. ) ;
#74986=CIRCLE ( 'NONE', #35816, 5.599999999999994316 ) ;
#74987=CARTESIAN_POINT ( 'NONE',  ( 97.80889870804310249, -40.51851473143300097, 41.63518016758125384 ) ) ;
#74989=ORIENTED_EDGE ( 'NONE', *, *, #71469, .F. ) ;
#74991=EDGE_CURVE ( 'NONE', #74036, #68275, #29337, .T. ) ;
#74992=FACE_OUTER_BOUND ( 'NONE', #69909, .T. ) ;
#74993=VERTEX_POINT ( 'NONE', #13458 ) ;
#74994=ORIENTED_EDGE ( 'NONE', *, *, #9797, .F. ) ;
#74995=PLANE ( 'NONE',  #457 ) ;
#74997=CARTESIAN_POINT ( 'NONE',  ( 177.0371591254546217, -48.62818131005479927, 117.4678068554150485 ) ) ;
#74998=CYLINDRICAL_SURFACE ( 'NONE', #80880, 2.030000000001311644 ) ;
#74999=CARTESIAN_POINT ( 'NONE',  ( 115.4591718486505698, -35.14231982251399700, 158.3981341137909737 ) ) ;
#75000=CARTESIAN_POINT ( 'NONE',  ( 96.91385697446291658, -32.24201331651869396, 55.98324432352897162 ) ) ;
#75001=CARTESIAN_POINT ( 'NONE',  ( 181.9694315774339941, -34.03355364505720360, 117.4678068554150627 ) ) ;
#75002=ORIENTED_EDGE ( 'NONE', *, *, #57479, .F. ) ;
#75004=ORIENTED_EDGE ( 'NONE', *, *, #61297, .F. ) ;
#75009=CARTESIAN_POINT ( 'NONE',  ( 98.38052710835017933, -41.69545545435574496, 131.7398046494048742 ) ) ;
#75011=FACE_OUTER_BOUND ( 'NONE', #27889, .T. ) ;
#75013=CARTESIAN_POINT ( 'NONE',  ( 117.5190927476815119, -36.54584727635032237, 288.8413395616252615 ) ) ;
#75014=CARTESIAN_POINT ( 'NONE',  ( 117.4907998085504062, -37.69205034685562339, 74.75276813305397638 ) ) ;
#75015=CARTESIAN_POINT ( 'NONE',  ( 86.06670390244796920, -58.72944715994110254, 10.91780685541499807 ) ) ;
#75017=CARTESIAN_POINT ( 'NONE',  ( 97.81219807385008380, -40.51719912245609123, 147.6362401243850115 ) ) ;
#75018=DIRECTION ( 'NONE',  ( 0.000000000000000000, 0.000000000000000000, 1.000000000000000000 ) ) ;
#75020=EDGE_CURVE ( 'NONE', #56128, #15112, #53990, .T. ) ;
#75025=ORIENTED_EDGE ( 'NONE', *, *, #61073, .F. ) ;
#75026=CARTESIAN_POINT ( 'NONE',  ( 107.1959452681378053, -26.26092741545045328, 35.06705384733893283 ) ) ;
#75027=CARTESIAN_POINT ( 'NONE',  ( 97.52247766716473620, -32.48101032970659219, 96.99276813305395706 ) ) ;
#75029=CIRCLE ( 'NONE', #85169, 3.250000000000002665 ) ;
#75030=VECTOR ( 'NONE', #33603, 1000.000000000000000 ) ;
#75031=CARTESIAN_POINT ( 'NONE',  ( 97.81480632908598238, -40.51613010894325839, 171.6358981596145270 ) ) ;
#75038=ORIENTED_EDGE ( 'NONE', *, *, #70995, .F. ) ;
#75039=CARTESIAN_POINT ( 'NONE',  ( 101.8448680821487642, -28.45912855063591351, 106.5241967044819944 ) ) ;
#75042=VERTEX_POINT ( 'NONE', #70214 ) ;
#75043=CARTESIAN_POINT ( 'NONE',  ( 99.76842024043818924, -29.31547782932927859, 221.6956252759109702 ) ) ;
#75044=DIRECTION ( 'NONE',  ( 9.912705577010326536E-16, 1.000000000000000000, 0.000000000000000000 ) ) ;
#75047=CARTESIAN_POINT ( 'NONE',  ( 19.56648329127400032, 0.2215528400590083269, 323.8756252759109202 ) ) ;
#75048=CARTESIAN_POINT ( 'NONE',  ( 116.3212776292295842, -32.94146857471309886, 45.13562527591097506 ) ) ;
#75049=CIRCLE ( 'NONE', #5421, 2.999999999999947153 ) ;
#75050=FACE_OUTER_BOUND ( 'NONE', #29294, .T. ) ;
#75053=CARTESIAN_POINT ( 'NONE',  ( 108.8290724220007348, -27.07506712556656936, 164.9327681330539690 ) ) ;
#75055=ORIENTED_EDGE ( 'NONE', *, *, #27144, .T. ) ;
#75056=CARTESIAN_POINT ( 'NONE',  ( 103.0662520580798116, -44.63681263099613972, 123.6358690201829802 ) ) ;
#75057=AXIS2_PLACEMENT_3D ( 'NONE', #83841, #62480, #42030 ) ;
#75058=PLANE ( 'NONE',  #52941 ) ;
#75059=CARTESIAN_POINT ( 'NONE',  ( 95.96284676697312932, -37.29622633765301032, 267.3670538473388092 ) ) ;
#75060=CARTESIAN_POINT ( 'NONE',  ( 52.65249034007741358, -48.32844715994062312, 180.4678068554151196 ) ) ;
#75064=DIRECTION ( 'NONE',  ( 0.000000000000000000, -1.000000000000000000, 0.000000000000000000 ) ) ;
#75066=CARTESIAN_POINT ( 'NONE',  ( 116.3579325164319869, -41.40893824611053020, 203.4556252759109611 ) ) ;
#75067=DIRECTION ( 'NONE',  ( 1.639958061481212836E-42, -4.100000000000000342E-29, -1.000000000000000000 ) ) ;
#75068=ORIENTED_EDGE ( 'NONE', *, *, #71842, .T. ) ;
#75069=ORIENTED_EDGE ( 'NONE', *, *, #15350, .F. ) ;
#75071=CARTESIAN_POINT ( 'NONE',  ( 78.02982435611156120, -16.87939921900763096, 2.327894594457669886 ) ) ;
#75072=CARTESIAN_POINT ( 'NONE',  ( 97.33789672108279944, -34.07083907252764021, 186.1152661070771046 ) ) ;
#75073=DIRECTION ( 'NONE',  ( 1.000000000000000000, 4.163336342344333240E-14, 0.000000000000000000 ) ) ;
#75076=ORIENTED_EDGE ( 'NONE', *, *, #89848, .F. ) ;
#75079=CARTESIAN_POINT ( 'NONE',  ( 113.0255487838780937, -46.03904575001691768, 218.0175300378159591 ) ) ;
#75080=EDGE_LOOP ( 'NONE', ( #15060, #46562 ) ) ;
#75082=FACE_OUTER_BOUND ( 'NONE', #44801, .T. ) ;
#75084=CARTESIAN_POINT ( 'NONE',  ( 115.2453386458995652, -37.16432389609550313, 16.60237608387699026 ) ) ;
#75085=CARTESIAN_POINT ( 'NONE',  ( 97.40507707138063154, -42.14631300639911160, 177.7451490854349743 ) ) ;
#75086=DIRECTION ( 'NONE',  ( -4.237773401492740281E-14, 1.000000000000000000, 0.000000000000000000 ) ) ;
#75087=VERTEX_POINT ( 'NONE', #35684 ) ;
#75088=VECTOR ( 'NONE', #18238, 1000.000000000000000 ) ;
#75089=PLANE ( 'NONE',  #65397 ) ;
#75090=CARTESIAN_POINT ( 'NONE',  ( 109.3070416278940797, -46.56271945438447801, 67.75589170717483967 ) ) ;
#75094=VECTOR ( 'NONE', #13821, 1000.000000000000000 ) ;
#75095=CARTESIAN_POINT ( 'NONE',  ( 33.91903122894498779, -35.91149509761220315, -5.074374724088000832 ) ) ;
#75096=ORIENTED_EDGE ( 'NONE', *, *, #59724, .T. ) ;
#75097=ORIENTED_EDGE ( 'NONE', *, *, #63727, .T. ) ;
#75098=PLANE ( 'NONE',  #6292 ) ;
#75099=CARTESIAN_POINT ( 'NONE',  ( 106.9524907322914089, -28.15978509997144741, 59.50956268521995440 ) ) ;
#75100=CARTESIAN_POINT ( 'NONE',  ( 99.52336843529489840, -29.45003914207232754, 250.7156252759109520 ) ) ;
#75102=CARTESIAN_POINT ( 'NONE',  ( 98.68348088377346983, -30.50934295487596515, 180.8184824187679567 ) ) ;
#75103=CARTESIAN_POINT ( 'NONE',  ( 116.3148031259206192, -32.94054721833379062, 24.13562527591095375 ) ) ;
#75104=CARTESIAN_POINT ( 'NONE',  ( 97.81168895331678925, -40.51742574516946860, 7.635625275910939536 ) ) ;
#75106=DIRECTION ( 'NONE',  ( 2.999999999999999839E-15, -1.000000000000000000, 2.999999999999999900E-30 ) ) ;
#75108=ADVANCED_FACE ( 'NONE', ( #62494 ), #8901, .T. ) ;
#75110=AXIS2_PLACEMENT_3D ( 'NONE', #1455, #539, #29152 ) ;
#75111=CIRCLE ( 'NONE', #86729, 9.571100913904423635 ) ;
#75112=AXIS2_PLACEMENT_3D ( 'NONE', #47762, #35039, #21885 ) ;
#75113=DIRECTION ( 'NONE',  ( 0.9242245927363033076, 0.3818493186865917766, 0.000000000000000000 ) ) ;
#75114=CARTESIAN_POINT ( 'NONE',  ( 118.1283360304583994, -32.34034571477864262, 249.1270538473389706 ) ) ;
#75116=CARTESIAN_POINT ( 'NONE',  ( 110.1375194624030769, -26.11116931986236267, 214.8403871806729342 ) ) ;
#75117=DIRECTION ( 'NONE',  ( 0.9999999853157766072, 0.0001713722456127401463, -9.999999853157767620E-16 ) ) ;
#75120=CARTESIAN_POINT ( 'NONE',  ( 97.81280325506480722, -40.52014819707925852, 22.63585978562170453 ) ) ;
#75122=CARTESIAN_POINT ( 'NONE',  ( 110.8530203762849169, -44.87085336317501572, 277.6356252759111953 ) ) ;
#75123=LINE ( 'NONE', #34224, #41304 ) ;
#75124=CARTESIAN_POINT ( 'NONE',  ( 116.8171287662699456, -34.15293273489836423, 175.0314573698340439 ) ) ;
#75125=DIRECTION ( 'NONE',  ( 0.9999999853157766072, 0.0001713722456127401463, -9.999999853157767620E-16 ) ) ;
#75126=LINE ( 'NONE', #46048, #46978 ) ;
#75127=CARTESIAN_POINT ( 'NONE',  ( 188.5667039024479834, -62.87844715994099687, 293.2178068554150627 ) ) ;
#75128=CARTESIAN_POINT ( 'NONE',  ( 97.80889870804310249, -40.51851473143300097, 41.63518016758125384 ) ) ;
#75130=CARTESIAN_POINT ( 'NONE',  ( 112.1393456453461681, -28.01282278345784604, 75.65645860890421659 ) ) ;
#75133=CARTESIAN_POINT ( 'NONE',  ( 136.8037680012526494, -19.00431460297267350, 6.768845952120934761 ) ) ;
#75134=CARTESIAN_POINT ( 'NONE',  ( 100.6426946765138695, -44.96845825347062231, 232.0499109901969632 ) ) ;
#75135=CARTESIAN_POINT ( 'NONE',  ( 117.3638278218041364, -38.35646377537064211, 109.7013395616249767 ) ) ;
#75136=CARTESIAN_POINT ( 'NONE',  ( 99.30088202768328642, -28.79894053213705973, 266.7051490854347549 ) ) ;
#75137=CARTESIAN_POINT ( 'NONE',  ( 51.23005224011598102, -33.89581943344511217, -5.074374724088000832 ) ) ;
#75139=VECTOR ( 'NONE', #68268, 1000.000000000000000 ) ;
#75140=LINE ( 'NONE', #6544, #68148 ) ;
#75141=CARTESIAN_POINT ( 'NONE',  ( 89.10937460273895283, -56.62589376934769092, -5.074374724089016020 ) ) ;
#75142=PLANE ( 'NONE',  #39260 ) ;
#75143=AXIS2_PLACEMENT_3D ( 'NONE', #82870, #34240, #60596 ) ;
#75144=CARTESIAN_POINT ( 'NONE',  ( 131.5441285970359218, -19.82508440162534669, 2.797770139039466031 ) ) ;
#75145=ORIENTED_EDGE ( 'NONE', *, *, #65870, .F. ) ;
#75147=CARTESIAN_POINT ( 'NONE',  ( 103.4202683135912650, -45.01906637089264507, 131.6571817328389784 ) ) ;
#75149=CARTESIAN_POINT ( 'NONE',  ( 97.81252181335722184, -40.51708140359354360, 276.6353344664656220 ) ) ;
#75150=ORIENTED_EDGE ( 'NONE', *, *, #15855, .T. ) ;
#75151=CARTESIAN_POINT ( 'NONE',  ( 99.09566894039866725, -30.55048508729688095, 90.80073160410523769 ) ) ;
#75152=CARTESIAN_POINT ( 'NONE',  ( 113.9719413768824126, -28.12837331961977938, 115.5261014663869474 ) ) ;
#75153=CARTESIAN_POINT ( 'NONE',  ( 138.8664832912739939, -71.52944715994085811, 361.9756252759100335 ) ) ;
#75156=FACE_OUTER_BOUND ( 'NONE', #19875, .T. ) ;
#75158=DIRECTION ( 'NONE',  ( 1.000000000000000078E-15, 1.000000000000000083E-30, -1.000000000000000000 ) ) ;
#75159=EDGE_CURVE ( 'NONE', #30367, #71324, #14876, .T. ) ;
#75160=AXIS2_PLACEMENT_3D ( 'NONE', #44486, #85424, #16804 ) ;
#75161=CARTESIAN_POINT ( 'NONE',  ( 114.5308976578478735, -43.10096916487051288, 63.26419670448296984 ) ) ;
#75162=ORIENTED_EDGE ( 'NONE', *, *, #52906, .F. ) ;
#75164=ORIENTED_EDGE ( 'NONE', *, *, #72850, .F. ) ;
#75165=AXIS2_PLACEMENT_3D ( 'NONE', #61951, #69677, #35136 ) ;
#75166=AXIS2_PLACEMENT_3D ( 'NONE', #59470, #2753, #51311 ) ;
#75167=CARTESIAN_POINT ( 'NONE',  ( 114.0075790447407087, -33.88846322102013175, 9.635625275910941312 ) ) ;
#75169=CARTESIAN_POINT ( 'NONE',  ( 113.8091913586853821, -43.81457933525486936, 154.1813395616249807 ) ) ;
#75173=LINE ( 'NONE', #33832, #18433 ) ;
#75174=AXIS2_PLACEMENT_3D ( 'NONE', #49241, #62881, #43779 ) ;
#75176=DIRECTION ( 'NONE',  ( 0.000000000000000000, 0.000000000000000000, -1.000000000000000000 ) ) ;
#75177=CARTESIAN_POINT ( 'NONE',  ( 108.5348814579965904, -26.43029805172848867, 104.9641967044819779 ) ) ;
#75180=ORIENTED_EDGE ( 'NONE', *, *, #62433, .T. ) ;
#75181=AXIS2_PLACEMENT_3D ( 'NONE', #69251, #76057, #35613 ) ;
#75187=CARTESIAN_POINT ( 'NONE',  ( 100.9764986820135420, -31.29420903488464845, 188.5652332267349607 ) ) ;
#75189=CARTESIAN_POINT ( 'NONE',  ( 100.9551459015743262, -28.70665567104044058, 26.59337149677223877 ) ) ;
#75191=ORIENTED_EDGE ( 'NONE', *, *, #52062, .F. ) ;
#75192=ORIENTED_EDGE ( 'NONE', *, *, #33758, .T. ) ;
#75193=CIRCLE ( 'NONE', #36029, 0.5000000000000004441 ) ;
#75194=DIRECTION ( 'NONE',  ( 1.000000000000000000, 4.163336342344333240E-14, 0.000000000000000000 ) ) ;
#75195=CARTESIAN_POINT ( 'NONE',  ( 136.6235172543038630, -19.74149216370141247, 2.839569540204845310 ) ) ;
#75196=EDGE_LOOP ( 'NONE', ( #57980, #53225, #88922, #65656 ) ) ;
#75197=ORIENTED_EDGE ( 'NONE', *, *, #37003, .F. ) ;
#75198=CARTESIAN_POINT ( 'NONE',  ( 164.7812970173289955, -35.65087443492610930, -5.074374724088000832 ) ) ;
#75199=CARTESIAN_POINT ( 'NONE',  ( 100.8499323319230854, -30.41416626502819298, 222.1272975916109544 ) ) ;
#75200=CIRCLE ( 'NONE', #50552, 5.599999999999994316 ) ;
#75201=FACE_OUTER_BOUND ( 'NONE', #58228, .T. ) ;
#75202=CIRCLE ( 'NONE', #60655, 0.5000000000000004441 ) ;
#75205=ORIENTED_EDGE ( 'NONE', *, *, #28775, .F. ) ;
#75207=CARTESIAN_POINT ( 'NONE',  ( 20.03715912545739997, -46.82818131006202123, 129.9678068554150627 ) ) ;
#75208=VERTEX_POINT ( 'NONE', #69320 ) ;
#75210=EDGE_CURVE ( 'NONE', #66199, #10278, #23573, .T. ) ;
#75211=CARTESIAN_POINT ( 'NONE',  ( 101.3402310731127329, -30.91225182618282830, 223.5138046553059894 ) ) ;
#75213=CARTESIAN_POINT ( 'NONE',  ( 113.8578909311569305, -28.74413913138208088, 139.5156252759109634 ) ) ;
#75214=CARTESIAN_POINT ( 'NONE',  ( 99.51750086509213133, -43.88776608678593760, 81.92991099019597812 ) ) ;
#75215=CARTESIAN_POINT ( 'NONE',  ( 104.5384893572752958, -28.65942663403409441, 249.5838068554171514 ) ) ;
#75216=CARTESIAN_POINT ( 'NONE',  ( 132.6459363690132705, -16.36767598606458307, 7.908804215160404993 ) ) ;
#75218=CARTESIAN_POINT ( 'NONE',  ( 100.0081584303796944, -27.21027357624165788, 181.5841967044829630 ) ) ;
#75219=FACE_OUTER_BOUND ( 'NONE', #52019, .T. ) ;
#75220=VERTEX_POINT ( 'NONE', #70668 ) ;
#75221=DIRECTION ( 'NONE',  ( 0.7071067811865969777, -0.7071067811864980568, 0.000000000000000000 ) ) ;
#75222=EDGE_CURVE ( 'NONE', #19595, #3377, #76583, .T. ) ;
#75223=VERTEX_POINT ( 'NONE', #84758 ) ;
#75224=AXIS2_PLACEMENT_3D ( 'NONE', #37590, #38460, #80277 ) ;
#75225=ADVANCED_FACE ( 'NONE', ( #14365 ), #24738, .F. ) ;
#75226=ORIENTED_EDGE ( 'NONE', *, *, #68961, .F. ) ;
#75228=ORIENTED_EDGE ( 'NONE', *, *, #21279, .F. ) ;
#75229=EDGE_CURVE ( 'NONE', #48612, #1618, #16594, .T. ) ;
#75230=AXIS2_PLACEMENT_3D ( 'NONE', #15510, #77280, #35934 ) ;
#75232=AXIS2_PLACEMENT_3D ( 'NONE', #28714, #62775, #62332 ) ;
#75233=CARTESIAN_POINT ( 'NONE',  ( 112.5143773164265184, -27.84083190490108706, 94.63848241876793566 ) ) ;
#75235=EDGE_CURVE ( 'NONE', #64226, #11834, #10653, .T. ) ;
#75238=CARTESIAN_POINT ( 'NONE',  ( 98.30753418359370244, -41.72887547895405902, 142.7397919414705427 ) ) ;
#75240=CARTESIAN_POINT ( 'NONE',  ( 117.4525030917817645, -36.13006561810995976, 224.8727681330539667 ) ) ;
#75243=VERTEX_POINT ( 'NONE', #51095 ) ;
#75244=AXIS2_PLACEMENT_3D ( 'NONE', #8622, #83138, #69943 ) ;
#75246=LINE ( 'NONE', #47952, #50038 ) ;
#75247=CARTESIAN_POINT ( 'NONE',  ( 88.17226027475679473, -58.72944715994100306, 239.5838068554174924 ) ) ;
#75249=CIRCLE ( 'NONE', #60763, 4.750000000000004441 ) ;
#75250=CARTESIAN_POINT ( 'NONE',  ( 48.85858412958099706, -30.08671355700241179, -5.074374724088000832 ) ) ;
#75251=CARTESIAN_POINT ( 'NONE',  ( 107.2500105196458549, -24.83007258495691616, 230.0641967044819580 ) ) ;
#75252=VERTEX_POINT ( 'NONE', #65183 ) ;
#75253=CARTESIAN_POINT ( 'NONE',  ( 102.3835747273358550, -27.86123704493403963, 195.4630013769998982 ) ) ;
#75254=CARTESIAN_POINT ( 'NONE',  ( 99.76212870471702843, -44.21728614272981872, 17.96133956162493206 ) ) ;
#75255=CARTESIAN_POINT ( 'NONE',  ( 101.9507351169249887, -46.57965624409947480, 163.1832443235299763 ) ) ;
#75256=CARTESIAN_POINT ( 'NONE',  ( 179.1667039024473809, -26.71338133338671739, 313.9678068554149490 ) ) ;
#75257=CARTESIAN_POINT ( 'NONE',  ( 97.70650136287245857, -40.25115876428171191, 102.6128377541471650 ) ) ;
#75259=CARTESIAN_POINT ( 'NONE',  ( 152.0368932755770857, -23.42844715993588522, 249.9678068554149490 ) ) ;
#75260=FACE_OUTER_BOUND ( 'NONE', #31213, .T. ) ;
#75264=EDGE_LOOP ( 'NONE', ( #73640, #3669, #53419, #88652 ) ) ;
#75265=AXIS2_PLACEMENT_3D ( 'NONE', #72652, #73528, #24501 ) ;
#75266=EDGE_CURVE ( 'NONE', #36163, #89471, #36603, .T. ) ;
#75267=ORIENTED_EDGE ( 'NONE', *, *, #56966, .F. ) ;
#75269=CARTESIAN_POINT ( 'NONE',  ( 99.08262072259969955, -44.34008189452608661, 32.92038718067297509 ) ) ;
#75271=EDGE_CURVE ( 'NONE', #5447, #74330, #78834, .T. ) ;
#75272=ADVANCED_FACE ( 'NONE', ( #2962 ), #58362, .T. ) ;
#75274=CARTESIAN_POINT ( 'NONE',  ( 107.0664832912750057, -36.72944715993903486, 0.4256252759109709349 ) ) ;
#75275=ADVANCED_FACE ( 'NONE', ( #45163 ), #56993, .F. ) ;
#75276=CARTESIAN_POINT ( 'NONE',  ( 114.8173571680961231, -40.38677627709480333, 227.8981341137909453 ) ) ;
#75277=ORIENTED_EDGE ( 'NONE', *, *, #73503, .F. ) ;
#75279=VERTEX_POINT ( 'NONE', #71570 ) ;
#75280=DIRECTION ( 'NONE',  ( -2.999999999999999839E-15, 1.000000000000000000, -2.999999999999999900E-30 ) ) ;
#75281=CARTESIAN_POINT ( 'NONE',  ( 101.9936758543545636, -45.44610597658563478, 102.1565380991941652 ) ) ;
#75282=LINE ( 'NONE', #47991, #9185 ) ;
#75283=FACE_OUTER_BOUND ( 'NONE', #64079, .T. ) ;
#75284=CARTESIAN_POINT ( 'NONE',  ( 184.5667039024485518, -48.82844715993447693, 180.4678068554150343 ) ) ;
#75285=DIRECTION ( 'NONE',  ( 1.000000000000000000, 4.163336342344333240E-14, 0.000000000000000000 ) ) ;
#75286=CARTESIAN_POINT ( 'NONE',  ( 109.8085987287837497, -27.34093086507531112, 259.8499109901970314 ) ) ;
#75288=EDGE_LOOP ( 'NONE', ( #15151, #15830, #38882, #70407 ) ) ;
#75289=AXIS2_PLACEMENT_3D ( 'NONE', #88662, #39587, #32781 ) ;
#75290=CARTESIAN_POINT ( 'NONE',  ( 194.0371591254584587, -46.82818131005407736, 193.9678068554150343 ) ) ;
#75293=CARTESIAN_POINT ( 'NONE',  ( 113.4874516948114547, -42.53221286317273098, 81.07189989340096758 ) ) ;
#75294=AXIS2_PLACEMENT_3D ( 'NONE', #32134, #73475, #58940 ) ;
#75295=VECTOR ( 'NONE', #15883, 1000.000000000000000 ) ;
#75296=CARTESIAN_POINT ( 'NONE',  ( 109.7231921452033276, -27.00035804852990751, 129.8649303482066273 ) ) ;
#75297=CARTESIAN_POINT ( 'NONE',  ( 165.6738106836207578, -26.00627455218829809, 313.9678068554149490 ) ) ;
#75298=CARTESIAN_POINT ( 'NONE',  ( 115.0889047237290157, -30.61763667965946212, 44.34395860927426014 ) ) ;
#75299=ORIENTED_EDGE ( 'NONE', *, *, #21739, .F. ) ;
#75301=CARTESIAN_POINT ( 'NONE',  ( 91.06648329127391150, -36.72944715993925513, -4.074374724089044442 ) ) ;
#75302=EDGE_LOOP ( 'NONE', ( #19797, #62062, #80136, #49006, #53615, #67472 ) ) ;
#75303=CARTESIAN_POINT ( 'NONE',  ( 96.67071733825032709, -35.94615501309311156, 146.2670538473399517 ) ) ;
#75304=VERTEX_POINT ( 'NONE', #65624 ) ;
#75305=LINE ( 'NONE', #25807, #72133 ) ;
#75306=CARTESIAN_POINT ( 'NONE',  ( 108.9267623252842441, -45.42435897675616019, 104.1758690201829722 ) ) ;
#75310=CARTESIAN_POINT ( 'NONE',  ( 96.93562038266055936, -32.25163268508860881, 51.98324432352996638 ) ) ;
#75311=DIRECTION ( 'NONE',  ( -1.000000000000000078E-15, 0.000000000000000000, 1.000000000000000000 ) ) ;
#75312=EDGE_LOOP ( 'NONE', ( #17171, #16948, #84947, #8972 ) ) ;
#75316=EDGE_CURVE ( 'NONE', #85451, #52659, #72886, .T. ) ;
#75317=ADVANCED_FACE ( 'NONE', ( #59684 ), #87416, .T. ) ;
#75321=ORIENTED_EDGE ( 'NONE', *, *, #35, .F. ) ;
#75322=CARTESIAN_POINT ( 'NONE',  ( 109.7813264909552515, -47.51098736074730766, 242.7727681330539724 ) ) ;
#75323=CARTESIAN_POINT ( 'NONE',  ( 97.98816800684205930, -30.38363046389439859, 156.8289586092439549 ) ) ;
#75326=CARTESIAN_POINT ( 'NONE',  ( 101.7559735582952953, -27.03550746236556890, 96.46324432352997746 ) ) ;
#75327=DIRECTION ( 'NONE',  ( -1.000000000000000000, -4.510281037539694659E-14, 0.000000000000000000 ) ) ;
#75328=VERTEX_POINT ( 'NONE', #57916 ) ;
#75329=DIRECTION ( 'NONE',  ( 0.7071067811873675835, 0.7071067811857274510, 7.071067811873668640E-16 ) ) ;
#75330=EDGE_CURVE ( 'NONE', #56272, #84121, #37924, .T. ) ;
#75332=LINE ( 'NONE', #40351, #78198 ) ;
#75333=CONICAL_SURFACE ( 'NONE', #36177, 9.571100913904395213, 0.7853981633974522758 ) ;
#75334=ORIENTED_EDGE ( 'NONE', *, *, #27032, .F. ) ;
#75336=FACE_OUTER_BOUND ( 'NONE', #22042, .T. ) ;
#75337=CARTESIAN_POINT ( 'NONE',  ( 87.06648329127403940, -46.72944715994105280, -4.824374724089049771 ) ) ;
#75338=CARTESIAN_POINT ( 'NONE',  ( 111.7637953458032172, -46.71243375810367837, 287.9146728949587555 ) ) ;
#75339=DIRECTION ( 'NONE',  ( -0.7071067811578587436, 0.7071067812152364018, 0.000000000000000000 ) ) ;
#75340=CARTESIAN_POINT ( 'NONE',  ( 33.96670390244661775, -28.27351298637442056, 117.4678068554150485 ) ) ;
#75341=CARTESIAN_POINT ( 'NONE',  ( 108.3355664562415939, -46.73461849300061743, 92.67825729137430812 ) ) ;
#75342=CARTESIAN_POINT ( 'NONE',  ( 111.8651074766111861, -28.16866562884735004, 34.66991099019695355 ) ) ;
#75343=DIRECTION ( 'NONE',  ( 0.000000000000000000, 0.000000000000000000, -1.000000000000000000 ) ) ;
#75344=CARTESIAN_POINT ( 'NONE',  ( 117.8527506973082524, -39.03601561205230297, 104.6708633711489824 ) ) ;
#75345=DIRECTION ( 'NONE',  ( 0.7071067811865067165, 0.7071067811865883179, 7.071067811865061181E-16 ) ) ;
#75346=CARTESIAN_POINT ( 'NONE',  ( 116.7015053437751959, -40.82493444377960401, 168.5070538473399608 ) ) ;
#75347=CARTESIAN_POINT ( 'NONE',  ( 125.0664851986225159, -56.47944715994101728, 14.92562527591098842 ) ) ;
#75350=CARTESIAN_POINT ( 'NONE',  ( 107.0664832912739968, 0.2215528400590013880, 168.9256252759119832 ) ) ;
#75351=CARTESIAN_POINT ( 'NONE',  ( 136.1684221027065576, -34.94667169167191645, 2.376609173399411912 ) ) ;
#75355=DIRECTION ( 'NONE',  ( -0.7071067811869841124, 0.7071067811861110330, 0.000000000000000000 ) ) ;
#75356=CARTESIAN_POINT ( 'NONE',  ( 117.7240352459720043, -39.83258586197658246, 138.5889586092439743 ) ) ;
#75357=EDGE_LOOP ( 'NONE', ( #67724, #54116, #29371, #40448 ) ) ;
#75358=CARTESIAN_POINT ( 'NONE',  ( 141.0667039024479834, -58.35344715994099829, 310.9178068554150514 ) ) ;
#75360=LINE ( 'NONE', #68096, #18396 ) ;
#75361=EDGE_CURVE ( 'NONE', #47693, #49032, #12013, .T. ) ;
#75364=VERTEX_POINT ( 'NONE', #75582 ) ;
#75365=VECTOR ( 'NONE', #29295, 1000.000000000000000 ) ;
#75367=VERTEX_POINT ( 'NONE', #19271 ) ;
#75368=ORIENTED_EDGE ( 'NONE', *, *, #48277, .F. ) ;
#75369=VECTOR ( 'NONE', #77521, 1000.000000000000000 ) ;
#75373=CARTESIAN_POINT ( 'NONE',  ( 107.0664832912739968, -36.72944715994100306, 287.6356252759109680 ) ) ;
#75375=CARTESIAN_POINT ( 'NONE',  ( 63.03715912545736444, -24.42818131006027826, 237.4678068554150059 ) ) ;
#75378=CARTESIAN_POINT ( 'NONE',  ( 19.56670390244796920, -67.87844715994100397, 310.9178068554150514 ) ) ;
#75380=CARTESIAN_POINT ( 'NONE',  ( 97.79833369891507289, -40.48465503131496490, 181.6328088241103274 ) ) ;
#75382=ORIENTED_EDGE ( 'NONE', *, *, #2430, .F. ) ;
#75383=AXIS2_PLACEMENT_3D ( 'NONE', #66878, #46416, #11477 ) ;
#75384=DIRECTION ( 'NONE',  ( 4.299999999999999979E-14, -1.000000000000000000, 4.400000000000000367E-29 ) ) ;
#75385=DIRECTION ( 'NONE',  ( 9.351236661543306751E-17, -3.725950533538267725E-29, -1.000000000000000000 ) ) ;
#75386=CARTESIAN_POINT ( 'NONE',  ( 101.0525363619397581, -44.44280425155404401, 228.0499109901959400 ) ) ;
#75391=CARTESIAN_POINT ( 'NONE',  ( 99.36524671511907059, -42.81259845621065807, 87.85848241876792031 ) ) ;
#75393=FACE_OUTER_BOUND ( 'NONE', #85834, .T. ) ;
#75394=CARTESIAN_POINT ( 'NONE',  ( 103.2777341875169554, -27.47496823152900802, 21.38569241147085620 ) ) ;
#75395=ORIENTED_EDGE ( 'NONE', *, *, #72266, .T. ) ;
#75397=DIRECTION ( 'NONE',  ( 0.000000000000000000, 1.000000000000000000, 2.000000000000000155E-15 ) ) ;
#75398=EDGE_LOOP ( 'NONE', ( #83190, #30988, #7314, #72151 ) ) ;
#75399=VERTEX_POINT ( 'NONE', #82408 ) ;
#75401=CARTESIAN_POINT ( 'NONE',  ( 106.6421946519922983, -45.61100719954815474, 243.9701547344679682 ) ) ;
#75403=DIRECTION ( 'NONE',  ( 1.000000000000000000, 4.163336342344333240E-14, 0.000000000000000000 ) ) ;
#75404=CARTESIAN_POINT ( 'NONE',  ( 115.0885484784128465, -30.61717473208839735, 139.3440046732524138 ) ) ;
#75405=DIRECTION ( 'NONE',  ( 0.000000000000000000, 1.000000000000000000, 0.000000000000000000 ) ) ;
#75406=CARTESIAN_POINT ( 'NONE',  ( 81.36878785332568498, -39.15209318185590348, 1.893168666199420924 ) ) ;
#75410=CARTESIAN_POINT ( 'NONE',  ( 115.7817158473913253, -41.80465924930165755, 184.4068246429673366 ) ) ;
#75411=EDGE_LOOP ( 'NONE', ( #8115, #64259 ) ) ;
#75412=CARTESIAN_POINT ( 'NONE',  ( 109.6430426817424433, -46.83134659365198615, 47.77562527591094721 ) ) ;
#75414=CARTESIAN_POINT ( 'NONE',  ( 113.5315931691687439, -43.38514287343249265, 266.0080903695914003 ) ) ;
#75415=VECTOR ( 'NONE', #89677, 1000.000000000000000 ) ;
#75417=CARTESIAN_POINT ( 'NONE',  ( 117.0231039428183522, -39.62849705588583760, 138.5889586092449690 ) ) ;
#75419=DIRECTION ( 'NONE',  ( 0.000000000000000000, 0.000000000000000000, -1.000000000000000000 ) ) ;
#75420=DIRECTION ( 'NONE',  ( -4.237773401492740281E-14, 1.000000000000000000, 0.000000000000000000 ) ) ;
#75422=CARTESIAN_POINT ( 'NONE',  ( 117.5342389965484386, -35.85531600229182914, 249.8927681330537780 ) ) ;
#75423=FACE_OUTER_BOUND ( 'NONE', #85638, .T. ) ;
#75424=AXIS2_PLACEMENT_3D ( 'NONE', #79378, #37136, #58451 ) ;
#75426=CARTESIAN_POINT ( 'NONE',  ( 113.9455412938869330, -28.01876065682782624, 120.5565776568639507 ) ) ;
#75429=ORIENTED_EDGE ( 'NONE', *, *, #57171, .F. ) ;
#75432=ORIENTED_EDGE ( 'NONE', *, *, #63647, .F. ) ;
#75433=CIRCLE ( 'NONE', #81288, 1.000000000000000888 ) ;
#75435=DIRECTION ( 'NONE',  ( 0.000000000000000000, 0.000000000000000000, 1.000000000000000000 ) ) ;
#75438=LINE ( 'NONE', #84049, #180 ) ;
#75440=CARTESIAN_POINT ( 'NONE',  ( 112.8577109034250583, -30.29807625619018197, 157.3233284648299559 ) ) ;
#75441=CARTESIAN_POINT ( 'NONE',  ( 97.54012738755939438, -43.81963713510241121, 257.8356252759109566 ) ) ;
#75442=CARTESIAN_POINT ( 'NONE',  ( 99.50452936416800753, -43.30555000397543353, 57.89599405887542360 ) ) ;
#75443=ORIENTED_EDGE ( 'NONE', *, *, #10316, .T. ) ;
#75445=AXIS2_PLACEMENT_3D ( 'NONE', #18586, #46266, #74001 ) ;
#75446=DIRECTION ( 'NONE',  ( 0.000000000000000000, 0.000000000000000000, -1.000000000000000000 ) ) ;
#75449=EDGE_CURVE ( 'NONE', #39918, #14767, #6530, .T. ) ;
#75451=ORIENTED_EDGE ( 'NONE', *, *, #76222, .T. ) ;
#75453=DIRECTION ( 'NONE',  ( -2.999999999999999839E-15, 1.000000000000000000, -2.999999999999999900E-30 ) ) ;
#75454=DIRECTION ( 'NONE',  ( 1.000000000000000078E-15, -1.000000000000000083E-30, -1.000000000000000000 ) ) ;
#75456=DIRECTION ( 'NONE',  ( -1.000000000000000078E-15, 0.000000000000000000, -1.000000000000000000 ) ) ;
#75457=ADVANCED_FACE ( 'NONE', ( #88768 ), #32885, .T. ) ;
#75458=VECTOR ( 'NONE', #87409, 1000.000000000000000 ) ;
#75459=CARTESIAN_POINT ( 'NONE',  ( 98.52747904795083400, -36.52563780154032003, 195.7295626852199462 ) ) ;
#75460=CARTESIAN_POINT ( 'NONE',  ( 117.1340566916381789, -32.05431620389533265, 59.16038718067295576 ) ) ;
#75461=DIRECTION ( 'NONE',  ( 1.000000000000000000, 0.000000000000000000, 0.000000000000000000 ) ) ;
#75465=CARTESIAN_POINT ( 'NONE',  ( 87.17003668186664811, -54.68655584847640228, 14.92562527591100618 ) ) ;
#75466=ORIENTED_EDGE ( 'NONE', *, *, #50855, .T. ) ;
#75467=CARTESIAN_POINT ( 'NONE',  ( 115.5207272689788027, -31.29719706063076856, 165.2807688001713018 ) ) ;
#75469=FACE_OUTER_BOUND ( 'NONE', #80458, .T. ) ;
#75470=CIRCLE ( 'NONE', #36301, 2.500000000000002220 ) ;
#75472=ORIENTED_EDGE ( 'NONE', *, *, #578, .T. ) ;
#75473=CARTESIAN_POINT ( 'NONE',  ( 112.7537747436706184, -27.22417719680832704, 54.65943479971996055 ) ) ;
#75475=DIRECTION ( 'NONE',  ( 1.000000000000000000, 0.000000000000000000, -0.000000000000000000 ) ) ;
#75476=FACE_OUTER_BOUND ( 'NONE', #55046, .T. ) ;
#75477=CARTESIAN_POINT ( 'NONE',  ( 131.5918432679227408, -17.51852171454203244, 2.740177351677692830 ) ) ;
#75478=ORIENTED_EDGE ( 'NONE', *, *, #26118, .F. ) ;
#75480=CARTESIAN_POINT ( 'NONE',  ( 97.06871944863306112, -35.59214294076518570, 122.2351737579207054 ) ) ;
#75482=VECTOR ( 'NONE', #62397, 1000.000000000000000 ) ;
#75483=DIRECTION ( 'NONE',  ( -1.000000000000000000, -3.360405532702990443E-14, 0.000000000000000000 ) ) ;
#75485=CARTESIAN_POINT ( 'NONE',  ( 113.3277443033378376, -28.32255675095946046, 100.5670538473389684 ) ) ;
#75487=DIRECTION ( 'NONE',  ( 4.299999999999999979E-14, -1.000000000000000000, 4.400000000000000367E-29 ) ) ;
#75488=EDGE_CURVE ( 'NONE', #18807, #5538, #34226, .T. ) ;
#75491=DIRECTION ( 'NONE',  ( 0.000000000000000000, 0.000000000000000000, -1.000000000000000000 ) ) ;
#75493=CARTESIAN_POINT ( 'NONE',  ( 107.9488082096507213, -26.98745991040269487, 151.0041967044819557 ) ) ;
#75494=VECTOR ( 'NONE', #56767, 1000.000000000000000 ) ;
#75496=ORIENTED_EDGE ( 'NONE', *, *, #67321, .F. ) ;
#75497=CARTESIAN_POINT ( 'NONE',  ( 99.41296134609930846, -28.78668791560525975, 261.6746728949588032 ) ) ;
#75498=CARTESIAN_POINT ( 'NONE',  ( 156.5667039024483813, -48.82844715993569196, 257.2178068554149490 ) ) ;
#75500=CARTESIAN_POINT ( 'NONE',  ( 90.44969454456439450, -53.34645651782491882, 249.5838068554174640 ) ) ;
#75501=FACE_OUTER_BOUND ( 'NONE', #2477, .T. ) ;
#75505=CARTESIAN_POINT ( 'NONE',  ( 103.9298229712113653, -26.84510867568817716, 205.3089586092449679 ) ) ;
#75506=ORIENTED_EDGE ( 'NONE', *, *, #68136, .F. ) ;
#75507=ORIENTED_EDGE ( 'NONE', *, *, #56785, .F. ) ;
#75508=CARTESIAN_POINT ( 'NONE',  ( 98.25403324269851169, -37.66165033158306130, 122.8415833058969469 ) ) ;
#75509=ADVANCED_FACE ( 'NONE', ( #52839 ), #46498, .T. ) ;
#75511=CARTESIAN_POINT ( 'NONE',  ( 115.2782656938782821, -32.16401669718150202, 25.67396425827794815 ) ) ;
#75512=LINE ( 'NONE', #5581, #4175 ) ;
#75513=DIRECTION ( 'NONE',  ( -1.042183321081676705E-15, -1.000000000000000000, 0.000000000000000000 ) ) ;
#75515=PLANE ( 'NONE',  #69284 ) ;
#75516=CARTESIAN_POINT ( 'NONE',  ( 33.91903122894498779, -35.91149509761220315, -5.074374724088000832 ) ) ;
#75518=CARTESIAN_POINT ( 'NONE',  ( 100.9546728069516917, -28.70702573053221585, 106.5939586096738054 ) ) ;
#75519=DIRECTION ( 'NONE',  ( -0.9254794337955620787, -0.3787978585227822492, 0.000000000000000000 ) ) ;
#75520=CARTESIAN_POINT ( 'NONE',  ( 96.69582475441069391, -35.54038568221476879, 206.2356252759109623 ) ) ;
#75522=ORIENTED_EDGE ( 'NONE', *, *, #10565, .F. ) ;
#75525=FACE_OUTER_BOUND ( 'NONE', #84729, .T. ) ;
#75526=CARTESIAN_POINT ( 'NONE',  ( 116.7956972015441863, -39.38580969979880564, 124.6137336630641812 ) ) ;
#75528=VECTOR ( 'NONE', #29493, 1000.000000000000000 ) ;
#75529=DIRECTION ( 'NONE',  ( -0.7071067811865794361, 0.7071067811865157093, -7.071067811865803697E-16 ) ) ;
#75531=CARTESIAN_POINT ( 'NONE',  ( 104.4070190479019118, -46.45777198906507977, 62.36470280596612525 ) ) ;
#75532=CARTESIAN_POINT ( 'NONE',  ( 112.2051334037466432, -45.80035149650004200, 212.9870538473389558 ) ) ;
#75539=CARTESIAN_POINT ( 'NONE',  ( 115.9631861912839241, -41.36764275679356473, 168.4441829924387264 ) ) ;
#75541=CARTESIAN_POINT ( 'NONE',  ( 116.2870986197744969, -35.69205421237206366, 81.73380465530594563 ) ) ;
#75542=CARTESIAN_POINT ( 'NONE',  ( 114.9815172128508465, -29.91112648151817410, 180.3927681330539770 ) ) ;
#75543=VECTOR ( 'NONE', #88567, 1000.000000000000000 ) ;
#75544=CIRCLE ( 'NONE', #11935, 10.00000000000000888 ) ;
#75545=CARTESIAN_POINT ( 'NONE',  ( 80.06648281188265059, -39.47944715903999224, 8.225259175037734849 ) ) ;
#75546=ORIENTED_EDGE ( 'NONE', *, *, #55726, .F. ) ;
#75547=EDGE_CURVE ( 'NONE', #11858, #87811, #68314, .T. ) ;
#75549=CARTESIAN_POINT ( 'NONE',  ( 105.4091548812398855, -46.67577557997189786, 67.44613915122781123 ) ) ;
#75558=CARTESIAN_POINT ( 'NONE',  ( 114.4871815801477624, -30.46814820527590228, 73.80670554236196779 ) ) ;
#75560=CARTESIAN_POINT ( 'NONE',  ( 116.9463234969885974, -41.73785994705047386, 248.4651490854349731 ) ) ;
#75561=CARTESIAN_POINT ( 'NONE',  ( 115.3705510513157861, -30.46277945167181045, 219.3413395616249773 ) ) ;
#75562=CYLINDRICAL_SURFACE ( 'NONE', #49014, 3.000000000000002665 ) ;
#75563=CARTESIAN_POINT ( 'NONE',  ( 113.7560087186648730, -29.08427257552855494, 285.5032443235299979 ) ) ;
#75566=CARTESIAN_POINT ( 'NONE',  ( 181.8884939055940038, -32.11662333284530746, -5.074374724088000832 ) ) ;
#75567=VECTOR ( 'NONE', #88974, 1000.000000000000000 ) ;
#75570=CARTESIAN_POINT ( 'NONE',  ( 114.7041265136728612, -43.74408836545399737, 78.22324432353094892 ) ) ;
#75571=CARTESIAN_POINT ( 'NONE',  ( 96.74811198265052781, -38.50085326290480481, 91.46133956162493917 ) ) ;
#75572=CARTESIAN_POINT ( 'NONE',  ( 97.18209604296552584, -40.28622700274314639, 266.6013395616253661 ) ) ;
#75573=ORIENTED_EDGE ( 'NONE', *, *, #9397, .F. ) ;
#75574=CARTESIAN_POINT ( 'NONE',  ( 116.8576245982602870, -40.31003124190988274, 218.5470538473399529 ) ) ;
#75575=CARTESIAN_POINT ( 'NONE',  ( 172.5664832912740110, -32.07844715994070839, 198.9256252759119832 ) ) ;
#75576=CARTESIAN_POINT ( 'NONE',  ( 141.8664832912729992, -71.52944715994142655, 352.4506252759077825 ) ) ;
#75577=CARTESIAN_POINT ( 'NONE',  ( 118.5256205435843100, -36.72944715994100306, 309.2406250056037038 ) ) ;
#75579=CARTESIAN_POINT ( 'NONE',  ( 111.6409576225383802, -30.15385841292844304, 277.6356252759107974 ) ) ;
#75581=CARTESIAN_POINT ( 'NONE',  ( 112.0657623353423560, -45.48848379642200257, 173.9897783938763780 ) ) ;
#75582=CARTESIAN_POINT ( 'NONE',  ( 160.5667039024426970, -48.82844715994099971, 249.9678068554149775 ) ) ;
#75583=DIRECTION ( 'NONE',  ( 1.000000000000000000, 0.000000000000000000, 0.000000000000000000 ) ) ;
#75584=CIRCLE ( 'NONE', #24804, 2.517499999999998739 ) ;
#75585=LINE ( 'NONE', #82860, #3696 ) ;
#75586=DIRECTION ( 'NONE',  ( 1.907762142705490052E-15, 7.167082501179359715E-16, -1.000000000000000000 ) ) ;
#75587=VECTOR ( 'NONE', #74806, 1000.000000000000000 ) ;
#75591=DIRECTION ( 'NONE',  ( 0.9999999853157766072, 0.0001713722456134972175, 0.000000000000000000 ) ) ;
#75592=CARTESIAN_POINT ( 'NONE',  ( 100.8099727397313217, -45.87009904342127697, 242.1108633711489517 ) ) ;
#75593=CARTESIAN_POINT ( 'NONE',  ( 117.5808906079046352, -33.32045621506634347, 130.0880062282919880 ) ) ;
#75594=CARTESIAN_POINT ( 'NONE',  ( 97.18271318096459765, -40.28600493293344442, 262.6013395616255934 ) ) ;
#75595=B_SPLINE_CURVE_WITH_KNOTS ( 'NONE', 3,
 ( #61856, #9480, #22680, #37192, #64007, #29482, #50353, #57165, #85808, #70825, #64896, #30377, #9050, #36749, #36297, #57622, #78092, #15859, #43982, #15417, #64448, #89593, #78982, #72162, #41412, #51241, #8600, #82790, #6907, #84468 ),
 .UNSPECIFIED., .F., .F.,
 ( 4, 2, 2, 2, 1, 2, 2, 2, 2, 2, 2, 2, 1, 2, 2, 4 ),
 ( 0.000000000000000000, 0.1250000000000416889, 0.1875000000000625333, 0.2187500000000721367, 0.2343750000000751343, 0.2421875000000783817, 0.2500000000000816014, 0.3750000000000487943, 0.4375000000000323630, 0.5000000000000159872, 0.6249999999999775735, 0.6874999999999630296, 0.7187499999999547029, 0.7343749999999505951, 0.7499999999999464873, 1.000000000000000000 ),
 .UNSPECIFIED. ) ;
#75596=CARTESIAN_POINT ( 'NONE',  ( 180.2143765759489895, -35.91149509761070391, 342.9256252759119548 ) ) ;
#75599=CARTESIAN_POINT ( 'NONE',  ( 83.73314995794039817, 12.92155284005802685, 349.2756252759109543 ) ) ;
#75600=ADVANCED_FACE ( 'NONE', ( #28302 ), #49187, .T. ) ;
#75602=CYLINDRICAL_SURFACE ( 'NONE', #89232, 2.030000000001807248 ) ;
#75603=CIRCLE ( 'NONE', #20488, 12.99999999999999822 ) ;
#75606=ORIENTED_EDGE ( 'NONE', *, *, #72673, .F. ) ;
#75607=CARTESIAN_POINT ( 'NONE',  ( 97.43556672503765981, -37.99919831760565359, 150.8524198280769895 ) ) ;
#75610=CARTESIAN_POINT ( 'NONE',  ( 115.0888006782553248, -30.61750168745167855, 89.34348336381457045 ) ) ;
#75611=CARTESIAN_POINT ( 'NONE',  ( 114.4473569665853603, -28.53271593493113301, 155.5051490854349652 ) ) ;
#75612=FACE_OUTER_BOUND ( 'NONE', #23591, .T. ) ;
#75614=CIRCLE ( 'NONE', #8908, 2.117000000000007987 ) ;
#75616=CARTESIAN_POINT ( 'NONE',  ( 48.85858412958099706, -30.08671355700241179, -5.074374724088000832 ) ) ;
#75617=CARTESIAN_POINT ( 'NONE',  ( 106.1376555893193228, -47.80867374849579221, 112.5099109901969712 ) ) ;
#75619=EDGE_LOOP ( 'NONE', ( #24048, #81123, #54246, #13966 ) ) ;
#75620=CIRCLE ( 'NONE', #6051, 1.000000000000000888 ) ;
#75621=VERTEX_POINT ( 'NONE', #83293 ) ;
#75623=CARTESIAN_POINT ( 'NONE',  ( 46.48091746482131015, -48.32844715994084339, 249.9678068554150343 ) ) ;
#75624=CARTESIAN_POINT ( 'NONE',  ( 98.64540312569894809, -41.76920806142280185, 157.7556252759109725 ) ) ;
#75626=CARTESIAN_POINT ( 'NONE',  ( 63.06670390244794078, -40.32844715994017548, 300.4678068554150627 ) ) ;
#75627=CYLINDRICAL_SURFACE ( 'NONE', #4544, 5.499999999999999112 ) ;
#75629=DIRECTION ( 'NONE',  ( -0.9254794337955620787, -0.3787978585227822492, 0.000000000000000000 ) ) ;
#75630=DIRECTION ( 'NONE',  ( 3.999999999999999995E-14, -1.000000000000000000, 4.100000000000000342E-29 ) ) ;
#75632=CARTESIAN_POINT ( 'NONE',  ( 100.3128846869252726, -46.43702735306955276, 87.09276813305393716 ) ) ;
#75633=EDGE_LOOP ( 'NONE', ( #43072, #39473, #31295, #33649, #21586, #65448 ) ) ;
#75635=CIRCLE ( 'NONE', #65503, 4.750000000000004441 ) ;
#75636=VERTEX_POINT ( 'NONE', #83741 ) ;
#75638=CARTESIAN_POINT ( 'NONE',  ( 107.0667039024479834, -36.72944715994099596, 239.5838068554170093 ) ) ;
#75641=CARTESIAN_POINT ( 'NONE',  ( 115.2258025850914862, -39.61500320815195408, 176.3861856076869685 ) ) ;
#75642=CARTESIAN_POINT ( 'NONE',  ( 25.56670390244748248, -48.82844715994178841, 137.2178068554150627 ) ) ;
#75643=ORIENTED_EDGE ( 'NONE', *, *, #28796, .F. ) ;
#75645=ORIENTED_EDGE ( 'NONE', *, *, #28736, .T. ) ;
#75646=FACE_OUTER_BOUND ( 'NONE', #30009, .T. ) ;
#75648=PLANE ( 'NONE',  #4170 ) ;
#75650=EDGE_LOOP ( 'NONE', ( #14272, #64762, #68051, #67498 ) ) ;
#75651=DIRECTION ( 'NONE',  ( 0.000000000000000000, 0.000000000000000000, -1.000000000000000000 ) ) ;
#75653=CARTESIAN_POINT ( 'NONE',  ( 106.4165995140572250, -45.56720307917569102, 218.9501547344689527 ) ) ;
#75658=ORIENTED_EDGE ( 'NONE', *, *, #3684, .T. ) ;
#75659=ORIENTED_EDGE ( 'NONE', *, *, #33890, .T. ) ;
#75661=ORIENTED_EDGE ( 'NONE', *, *, #61345, .F. ) ;
#75664=CARTESIAN_POINT ( 'NONE',  ( 97.84965203270614609, -37.79993896977983070, 234.2366617981629702 ) ) ;
#75665=CARTESIAN_POINT ( 'NONE',  ( 102.3504518276437523, -46.05175434220414132, 127.2041967044829960 ) ) ;
#75666=CARTESIAN_POINT ( 'NONE',  ( 116.9011659702704264, -33.23038410113876040, 114.0984824187679720 ) ) ;
#75667=CARTESIAN_POINT ( 'NONE',  ( 105.8091682078810294, -28.24967526344544311, 249.5838068554170377 ) ) ;
#75668=ADVANCED_FACE ( 'NONE', ( #28773 ), #21972, .T. ) ;
#75669=DIRECTION ( 'NONE',  ( 1.000000000000000000, 4.299999999999999979E-14, 1.000000000000000078E-15 ) ) ;
#75670=CARTESIAN_POINT ( 'NONE',  ( 107.5657681238088941, -47.77139876010166830, 188.6003871806729535 ) ) ;
#75672=ORIENTED_EDGE ( 'NONE', *, *, #84160, .F. ) ;
#75674=EDGE_LOOP ( 'NONE', ( #64018, #57937, #68853, #3912 ) ) ;
#75675=CIRCLE ( 'NONE', #35061, 2.517500000000000071 ) ;
#75676=ORIENTED_EDGE ( 'NONE', *, *, #20497, .T. ) ;
#75677=CARTESIAN_POINT ( 'NONE',  ( 188.5667039024483245, -42.82844715993430640, 170.7178068554150059 ) ) ;
#75681=CARTESIAN_POINT ( 'NONE',  ( 97.26623355869948284, -31.61728591124570542, 90.93181575210196854 ) ) ;
#75683=CARTESIAN_POINT ( 'NONE',  ( 107.0664832912739968, 12.92155284005902516, 336.6506252759110112 ) ) ;
#75687=CARTESIAN_POINT ( 'NONE',  ( 98.05565822401628395, -44.38798742045805312, 222.8870538473399563 ) ) ;
#75689=DIRECTION ( 'NONE',  ( 5.512527431108029424E-15, -1.000000000000000000, 0.000000000000000000 ) ) ;
#75691=AXIS2_PLACEMENT_3D ( 'NONE', #65724, #52515, #79387 ) ;
#75692=CARTESIAN_POINT ( 'NONE',  ( 107.0667039024467186, -36.72944715994091069, 195.5838068554169809 ) ) ;
#75693=DIRECTION ( 'NONE',  ( 0.7071067811864661934, 0.7071067811866289521, 7.071067811864966518E-16 ) ) ;
#75694=CARTESIAN_POINT ( 'NONE',  ( 82.81648329127399677, -18.72944715994105636, -5.074374724089055100 ) ) ;
#75695=VECTOR ( 'NONE', #6202, 1000.000000000000000 ) ;
#75696=LINE ( 'NONE', #12573, #56360 ) ;
#75697=CARTESIAN_POINT ( 'NONE',  ( 95.24515967180828113, -38.10243856675759133, 236.4184824187679510 ) ) ;
#75699=CARTESIAN_POINT ( 'NONE',  ( 72.06648329127401098, -45.72944715994106701, 14.92562527591093691 ) ) ;
#75700=CARTESIAN_POINT ( 'NONE',  ( 99.66888285774223277, -46.01973906766702527, 122.0413395616249659 ) ) ;
#75701=CARTESIAN_POINT ( 'NONE',  ( 105.9884228536615609, -26.36024887173286757, 46.15848241876796720 ) ) ;
#75702=CARTESIAN_POINT ( 'NONE',  ( 117.8238795360118445, -33.99523349031771602, 165.0365776568629315 ) ) ;
#75707=DIRECTION ( 'NONE',  ( 4.299999999999999979E-14, -1.000000000000000000, 4.400000000000000367E-29 ) ) ;
#75709=VERTEX_POINT ( 'NONE', #14700 ) ;
#75711=VERTEX_POINT ( 'NONE', #77364 ) ;
#75713=ORIENTED_EDGE ( 'NONE', *, *, #82913, .F. ) ;
#75714=DIRECTION ( 'NONE',  ( 0.000000000000000000, 0.000000000000000000, 1.000000000000000000 ) ) ;
#75715=CARTESIAN_POINT ( 'NONE',  ( 99.16013801855510224, -43.49098322490559809, 27.88991099019694175 ) ) ;
#75716=DIRECTION ( 'NONE',  ( 4.299999999999999979E-14, -1.000000000000000000, 4.400000000000000367E-29 ) ) ;
#75717=LINE ( 'NONE', #13487, #16630 ) ;
#75719=VECTOR ( 'NONE', #52636, 1000.000000000000000 ) ;
#75720=CARTESIAN_POINT ( 'NONE',  ( 104.8198721574821803, -27.95645401395800533, 244.7105150661719790 ) ) ;
#75722=VERTEX_POINT ( 'NONE', #64191 ) ;
#75723=ORIENTED_EDGE ( 'NONE', *, *, #32291, .T. ) ;
#75725=LINE ( 'NONE', #26666, #26859 ) ;
#75726=CARTESIAN_POINT ( 'NONE',  ( 115.0374107822371030, -42.90826833801408213, 103.3020634734001391 ) ) ;
#75727=CARTESIAN_POINT ( 'NONE',  ( 165.2725846195380086, -35.55794170701810941, 342.9256252759119548 ) ) ;
#75732=CARTESIAN_POINT ( 'NONE',  ( 104.4882414327378939, -26.97927861161949181, 175.2815989661729077 ) ) ;
#75733=CARTESIAN_POINT ( 'NONE',  ( 110.5064767540468296, -26.94654216138279068, 254.8194347997213640 ) ) ;
#75734=FACE_OUTER_BOUND ( 'NONE', #31187, .T. ) ;
#75735=EDGE_CURVE ( 'NONE', #83669, #28614, #82855, .T. ) ;
#75736=CIRCLE ( 'NONE', #22136, 2.517500000000005844 ) ;
#75738=EDGE_CURVE ( 'NONE', #12019, #21182, #81667, .T. ) ;
#75739=DIRECTION ( 'NONE',  ( 0.000000000000000000, 0.000000000000000000, -1.000000000000000000 ) ) ;
#75741=CARTESIAN_POINT ( 'NONE',  ( 101.7674321979440606, -44.34626990135510738, 84.91094751244793315 ) ) ;
#75743=EDGE_CURVE ( 'NONE', #40273, #87723, #42456, .T. ) ;
#75745=EDGE_CURVE ( 'NONE', #56522, #623, #77821, .T. ) ;
#75748=LINE ( 'NONE', #13516, #61925 ) ;
#75749=ORIENTED_EDGE ( 'NONE', *, *, #13399, .F. ) ;
#75750=CARTESIAN_POINT ( 'NONE',  ( 107.0664832912739399, -36.72944715994095333, 293.1356252759106837 ) ) ;
#75752=CARTESIAN_POINT ( 'NONE',  ( 117.0333688383452397, -30.31836458025946968, 144.2813395616249750 ) ) ;
#75753=ORIENTED_EDGE ( 'NONE', *, *, #40782, .T. ) ;
#75754=VECTOR ( 'NONE', #72345, 1000.000000000000000 ) ;
#75755=EDGE_CURVE ( 'NONE', #46083, #78070, #75813, .T. ) ;
#75756=CARTESIAN_POINT ( 'NONE',  ( 98.30753422232200478, -41.72887554593309289, 67.73979194757066580 ) ) ;
#75757=CARTESIAN_POINT ( 'NONE',  ( 100.7916921807572379, -44.60965664144636378, 118.4730118773259733 ) ) ;
#75758=DIRECTION ( 'NONE',  ( 1.000000000000000000, 0.000000000000000000, 0.000000000000000000 ) ) ;
#75760=CARTESIAN_POINT ( 'NONE',  ( 110.3609615670502535, -25.32029891922833897, 60.85276813305395649 ) ) ;
#75761=DIRECTION ( 'NONE',  ( 0.7071067811865295871, -0.7071067811865655584, 7.071067811865303756E-16 ) ) ;
#75763=DIRECTION ( 'NONE',  ( 0.000000000000000000, 1.000000000000000000, 0.000000000000000000 ) ) ;
#75765=VERTEX_POINT ( 'NONE', #23757 ) ;
#75767=CIRCLE ( 'NONE', #14891, 4.874999999999990230 ) ;
#75768=LINE ( 'NONE', #62574, #45504 ) ;
#75769=ORIENTED_EDGE ( 'NONE', *, *, #58686, .F. ) ;
#75770=CARTESIAN_POINT ( 'NONE',  ( 99.44473759953881142, -30.59981194223813361, 240.7870538473399620 ) ) ;
#75771=CARTESIAN_POINT ( 'NONE',  ( 114.4782738979392747, -28.49838154746453256, 155.5051490854349652 ) ) ;
#75773=CARTESIAN_POINT ( 'NONE',  ( 107.0664832912750057, -36.72944715993903486, 6.826283056785790393 ) ) ;
#75774=DIRECTION ( 'NONE',  ( 0.7071067811865295871, -0.7071067811865655584, 7.071067811864992156E-16 ) ) ;
#75775=CARTESIAN_POINT ( 'NONE',  ( 99.50169031327072844, -43.90275843488763741, 77.92991099019597812 ) ) ;
#75776=CARTESIAN_POINT ( 'NONE',  ( 97.31576093318726350, -39.30577132596791046, 97.53168462105917058 ) ) ;
#75777=EDGE_CURVE ( 'NONE', #66733, #43936, #30558, .T. ) ;
#75779=CARTESIAN_POINT ( 'NONE',  ( 179.7974245136200011, -36.32844715994040996, -5.074374724088000832 ) ) ;
#75780=ADVANCED_FACE ( 'NONE', ( #16046 ), #50989, .T. ) ;
#75781=CARTESIAN_POINT ( 'NONE',  ( 108.3337614075856692, -46.73482379084396143, 158.6771398271995679 ) ) ;
#75782=ORIENTED_EDGE ( 'NONE', *, *, #88496, .F. ) ;
#75783=VECTOR ( 'NONE', #9392, 1000.000000000000000 ) ;
#75786=CARTESIAN_POINT ( 'NONE',  ( 97.24442698086039627, -40.26379795196659472, 266.6013395616254797 ) ) ;
#75787=CARTESIAN_POINT ( 'NONE',  ( 37.35959712144330780, -48.62134037893607541, 129.9678068554150911 ) ) ;
#75788=CARTESIAN_POINT ( 'NONE',  ( 31.78666935232867630, -29.62846900982351528, 117.4678068554150485 ) ) ;
#75789=CARTESIAN_POINT ( 'NONE',  ( 105.7171716027695112, -46.72411491083433077, 92.46978268234177278 ) ) ;
#75790=CARTESIAN_POINT ( 'NONE',  ( 97.33063403691424753, -33.15845143124434458, 21.03467289495897319 ) ) ;
#75791=DIRECTION ( 'NONE',  ( 0.0001713722456120069274, -0.9999999853157766072, 0.000000000000000000 ) ) ;
#75792=CARTESIAN_POINT ( 'NONE',  ( 108.2741602056595269, -26.36093993100608657, 125.9841967044819597 ) ) ;
#75794=CARTESIAN_POINT ( 'NONE',  ( 102.0297551351921044, -46.62107256275958633, 172.2137205140059564 ) ) ;
#75796=EDGE_LOOP ( 'NONE', ( #29677, #3415, #7568, #34661 ) ) ;
#75797=CARTESIAN_POINT ( 'NONE',  ( 107.0664832912739968, -36.72944715994100306, 287.6356252759109680 ) ) ;
#75798=CYLINDRICAL_SURFACE ( 'NONE', #29085, 2.117000000000000881 ) ;
#75799=CARTESIAN_POINT ( 'NONE',  ( 136.6805397534846520, -35.85322261660486731, 2.908039740961550823 ) ) ;
#75802=CARTESIAN_POINT ( 'NONE',  ( 163.1543517358360020, -31.62489322948790971, -5.074374724088000832 ) ) ;
#75803=CARTESIAN_POINT ( 'NONE',  ( 108.5962597759698127, -47.12230983477568458, 142.6927681330539883 ) ) ;
#75810=CIRCLE ( 'NONE', #35194, 2.750000000000002665 ) ;
#75811=ORIENTED_EDGE ( 'NONE', *, *, #19643, .F. ) ;
#75813=CIRCLE ( 'NONE', #36656, 14.00000000000000888 ) ;
#75814=ORIENTED_EDGE ( 'NONE', *, *, #53027, .F. ) ;
#75815=CYLINDRICAL_SURFACE ( 'NONE', #6113, 2.030000000001872529 ) ;
#75817=CARTESIAN_POINT ( 'NONE',  ( 73.17003668186733023, -46.47944715994106701, -5.074374724089063982 ) ) ;
#75819=CARTESIAN_POINT ( 'NONE',  ( 177.0371591254543091, -48.62818131005480637, 313.9678068554149490 ) ) ;
#75820=CARTESIAN_POINT ( 'NONE',  ( 188.5667039024480971, -42.82844715993431350, 290.7178068554150059 ) ) ;
#75822=ORIENTED_EDGE ( 'NONE', *, *, #82236, .T. ) ;
#75823=LINE ( 'NONE', #13597, #664 ) ;
#75824=DIRECTION ( 'NONE',  ( 1.000000000000000000, 1.261617073437676668E-15, 1.261617073437676668E-15 ) ) ;
#75826=CARTESIAN_POINT ( 'NONE',  ( 118.0655259830058270, -38.35211242607483939, 219.7099109901959935 ) ) ;
#75827=DIRECTION ( 'NONE',  ( -4.237773401492740281E-14, 1.000000000000000000, 0.000000000000000000 ) ) ;
#75828=ADVANCED_FACE ( 'NONE', ( #71903 ), #74444, .T. ) ;
#75830=CARTESIAN_POINT ( 'NONE',  ( 107.2219638487720488, -26.36052190073626988, 76.07657765686298035 ) ) ;
#75831=DIRECTION ( 'NONE',  ( 0.000000000000000000, 0.000000000000000000, -1.000000000000000000 ) ) ;
#75832=CARTESIAN_POINT ( 'NONE',  ( 115.7800367298386419, -31.78559340308600412, 20.23709803735599877 ) ) ;
#75833=ADVANCED_FACE ( 'NONE', ( #85095 ), #22864, .F. ) ;
#75835=CARTESIAN_POINT ( 'NONE',  ( 127.1498166246070269, 12.92155284005802685, 336.5756252759110225 ) ) ;
#75836=ADVANCED_FACE ( 'NONE', ( #85986 ), #72346, .F. ) ;
#75837=VERTEX_POINT ( 'NONE', #3304 ) ;
#75838=EDGE_LOOP ( 'NONE', ( #59764, #878, #32117, #74482 ) ) ;
#75840=CARTESIAN_POINT ( 'NONE',  ( 104.4082965424966147, -28.27590814835049926, 246.7501547344679693 ) ) ;
#75842=VECTOR ( 'NONE', #51268, 1000.000000000000000 ) ;
#75843=CYLINDRICAL_SURFACE ( 'NONE', #53005, 7.499999999999996447 ) ;
#75845=EDGE_CURVE ( 'NONE', #51458, #10458, #31432, .T. ) ;
#75846=CYLINDRICAL_SURFACE ( 'NONE', #11240, 2.116999999999993776 ) ;
#75848=EDGE_LOOP ( 'NONE', ( #24692, #16869, #50268, #36378, #43156 ) ) ;
#75852=CARTESIAN_POINT ( 'NONE',  ( 97.77227622453175115, -32.00665715170008951, 50.95276813305294183 ) ) ;
#75854=CARTESIAN_POINT ( 'NONE',  ( 115.1807610290764075, -35.84162759104140150, 276.7309475124485516 ) ) ;
#75856=CARTESIAN_POINT ( 'NONE',  ( 97.81286927418427979, -40.51761286958078756, 126.6352223400343746 ) ) ;
#75857=CARTESIAN_POINT ( 'NONE',  ( 102.6819511611810753, -27.33185899950643005, 135.4118157521019441 ) ) ;
#75858=PLANE ( 'NONE',  #88285 ) ;
#75859=CARTESIAN_POINT ( 'NONE',  ( 131.0667039024480118, -58.72944715994093201, 207.5838068554149913 ) ) ;
#75860=LINE ( 'NONE', #54486, #70967 ) ;
#75862=ADVANCED_FACE ( 'NONE', ( #78282 ), #2411, .F. ) ;
#75863=CARTESIAN_POINT ( 'NONE',  ( 97.12841500021716001, -40.02000613830777098, 237.5813395616249579 ) ) ;
#75865=CARTESIAN_POINT ( 'NONE',  ( 162.5667039024470171, -33.35206098992711077, 193.9678068554150059 ) ) ;
#75867=AXIS2_PLACEMENT_3D ( 'NONE', #80386, #3618, #11324 ) ;
#75868=ORIENTED_EDGE ( 'NONE', *, *, #18105, .F. ) ;
#75869=CARTESIAN_POINT ( 'NONE',  ( 114.8035609388329021, -44.68778416175712920, 114.2022919425779719 ) ) ;
#75872=ORIENTED_EDGE ( 'NONE', *, *, #13962, .F. ) ;
#75873=ORIENTED_EDGE ( 'NONE', *, *, #41022, .F. ) ;
#75876=DIRECTION ( 'NONE',  ( 0.000000000000000000, 0.000000000000000000, -1.000000000000000000 ) ) ;
#75879=DIRECTION ( 'NONE',  ( -0.7071067811865613395, 0.7071067811865336949, -7.071067811865620286E-16 ) ) ;
#75880=CARTESIAN_POINT ( 'NONE',  ( 98.91056109567942656, -37.06209505544900651, 159.1766617981629679 ) ) ;
#75881=CARTESIAN_POINT ( 'NONE',  ( 106.1364166314141499, -47.76666518589912869, 258.4975300378158636 ) ) ;
#75882=CYLINDRICAL_SURFACE ( 'NONE', #8790, 0.5000000000000004441 ) ;
#75883=EDGE_CURVE ( 'NONE', #39354, #33468, #57808, .T. ) ;
#75884=ORIENTED_EDGE ( 'NONE', *, *, #24103, .T. ) ;
#75886=EDGE_CURVE ( 'NONE', #22170, #86967, #52739, .T. ) ;
#75887=CARTESIAN_POINT ( 'NONE',  ( 107.0664832912739399, -36.72944715994095333, 293.6356252759106837 ) ) ;
#75888=ORIENTED_EDGE ( 'NONE', *, *, #64992, .T. ) ;
#75890=DIRECTION ( 'NONE',  ( 1.000000000000000078E-15, -1.000000000000000083E-30, -1.000000000000000000 ) ) ;
#75891=VECTOR ( 'NONE', #60595, 1000.000000000000000 ) ;
#75892=ORIENTED_EDGE ( 'NONE', *, *, #57852, .F. ) ;
#75893=LINE ( 'NONE', #68633, #65741 ) ;
#75894=CARTESIAN_POINT ( 'NONE',  ( 115.0888988976580976, -30.61762792753790663, 14.34395942819159941 ) ) ;
#75895=B_SPLINE_CURVE_WITH_KNOTS ( 'NONE', 3,
 ( #70115, #63756, #29239, #56923, #15613, #71026, #24207, #31005, #65962, #10561, #86439, #30125, #51437, #51874, #17385, #10125, #52748, #59150 ),
 .UNSPECIFIED., .F., .F.,
 ( 4, 2, 2, 2, 2, 2, 2, 2, 4 ),
 ( 0.5000000000719210247, 0.5625000000629308827, 0.6250000000539407408, 0.6875000000449507098, 0.7500000000359605679, 0.8125000000269704259, 0.8750000000179802839, 0.9375000000089901420, 1.000000000000000000 ),
 .UNSPECIFIED. ) ;
#75896=DIRECTION ( 'NONE',  ( 1.907762142705490052E-15, 7.167082501179359715E-16, -1.000000000000000000 ) ) ;
#75897=LINE ( 'NONE', #6849, #89627 ) ;
#75898=CARTESIAN_POINT ( 'NONE',  ( 113.5483862797134549, -30.40508126489656604, 193.8762293518859678 ) ) ;
#75899=CARTESIAN_POINT ( 'NONE',  ( 109.9230826530363743, -46.83843495353658426, 72.79562527591099297 ) ) ;
#75900=DIRECTION ( 'NONE',  ( 0.000000000000000000, 0.000000000000000000, -1.000000000000000000 ) ) ;
#75902=AXIS2_PLACEMENT_3D ( 'NONE', #26887, #61399, #89575 ) ;
#75903=LINE ( 'NONE', #82290, #89100 ) ;
#75905=CARTESIAN_POINT ( 'NONE',  ( 112.1380301845968290, -28.01206920712143500, 260.6564718618365646 ) ) ;
#75906=VERTEX_POINT ( 'NONE', #18259 ) ;
#75907=DIRECTION ( 'NONE',  ( 0.000000000000000000, 1.000000000000000000, 0.000000000000000000 ) ) ;
#75909=CIRCLE ( 'NONE', #81695, 17.00000000000090239 ) ;
#75910=EDGE_CURVE ( 'NONE', #72232, #89279, #12554, .T. ) ;
#75911=DIRECTION ( 'NONE',  ( 1.000000000000000000, 4.272717921125132861E-14, 0.000000000000000000 ) ) ;
#75912=ORIENTED_EDGE ( 'NONE', *, *, #60973, .T. ) ;
#75913=CARTESIAN_POINT ( 'NONE',  ( 96.89953391513134306, -32.33301889150666142, 61.01372051400599616 ) ) ;
#75918=CARTESIAN_POINT ( 'NONE',  ( 131.4450127212694781, -17.89730640218637703, 2.921034946745714844 ) ) ;
#75919=EDGE_LOOP ( 'NONE', ( #30130, #30735, #9645, #40837 ) ) ;
#75922=DIRECTION ( 'NONE',  ( 1.000000000000000000, 0.000000000000000000, 0.000000000000000000 ) ) ;
#75923=ORIENTED_EDGE ( 'NONE', *, *, #12697, .F. ) ;
#75924=CARTESIAN_POINT ( 'NONE',  ( 98.31807308660266642, -42.43931386104045345, 97.78705384733993355 ) ) ;
#75925=PLANE ( 'NONE',  #76974 ) ;
#75926=DIRECTION ( 'NONE',  ( 1.000000000000000078E-15, -1.000000000000000083E-30, -1.000000000000000000 ) ) ;
#75928=EDGE_CURVE ( 'NONE', #89348, #67268, #11905, .T. ) ;
#75930=AXIS2_PLACEMENT_3D ( 'NONE', #37242, #57219, #43589 ) ;
#75931=EDGE_CURVE ( 'NONE', #69462, #60854, #51029, .T. ) ;
#75934=EDGE_CURVE ( 'NONE', #43691, #228, #87479, .T. ) ;
#75935=CARTESIAN_POINT ( 'NONE',  ( 116.5042510202518571, -34.04512512578506289, 145.0470538473389581 ) ) ;
#75936=DIRECTION ( 'NONE',  ( -1.000000000000000000, -4.554376769437570034E-14, 0.000000000000000000 ) ) ;
#75939=CARTESIAN_POINT ( 'NONE',  ( 109.2074818670226222, -48.35976665079980563, 273.7213395616252569 ) ) ;
#75940=DIRECTION ( 'NONE',  ( -4.299999999999999979E-14, 1.000000000000000000, -4.400000000000000367E-29 ) ) ;
#75944=DIRECTION ( 'NONE',  ( 1.639958061481212836E-42, -4.100000000000000342E-29, -1.000000000000000000 ) ) ;
#75947=CARTESIAN_POINT ( 'NONE',  ( 104.0204373342842388, -47.42213563049719482, 217.3556252759109668 ) ) ;
#75948=ORIENTED_EDGE ( 'NONE', *, *, #11129, .T. ) ;
#75950=CARTESIAN_POINT ( 'NONE',  ( 115.5247806442692422, -34.08644044406323559, 170.4987261630399473 ) ) ;
#75953=CARTESIAN_POINT ( 'NONE',  ( 114.1881255536272022, -42.05338753103387717, 24.74729759161198217 ) ) ;
#75954=CARTESIAN_POINT ( 'NONE',  ( 97.80396793100808850, -40.49851008571629762, 57.63399943843067774 ) ) ;
#75957=EDGE_CURVE ( 'NONE', #70274, #63468, #86258, .T. ) ;
#75960=VECTOR ( 'NONE', #28756, 1000.000000000000000 ) ;
#75962=CARTESIAN_POINT ( 'NONE',  ( 152.0368932755773130, -23.42844715993587812, 129.9678068554149775 ) ) ;
#75963=CARTESIAN_POINT ( 'NONE',  ( 98.95962429139160577, -30.20966935044058488, 240.7870538473399620 ) ) ;
#75964=CARTESIAN_POINT ( 'NONE',  ( 109.7260104821493485, -27.00109994382369649, 169.8639692407531925 ) ) ;
#75967=ADVANCED_FACE ( 'NONE', ( #30844 ), #4025, .T. ) ;
#75971=CYLINDRICAL_SURFACE ( 'NONE', #21620, 16.00000000000090239 ) ;
#75973=VERTEX_POINT ( 'NONE', #24924 ) ;
#75975=CARTESIAN_POINT ( 'NONE',  ( 101.6505379212622699, -45.63756515480785225, 247.1413395616249602 ) ) ;
#75978=CARTESIAN_POINT ( 'NONE',  ( 107.3864418959535527, -26.30668689864625875, 322.4523926293242653 ) ) ;
#75979=CARTESIAN_POINT ( 'NONE',  ( 109.6422649569531416, -46.48027517605736136, 167.7814222378137288 ) ) ;
#75980=CARTESIAN_POINT ( 'NONE',  ( 114.9159532999967723, -33.08434830970520579, 56.97856656006794651 ) ) ;
#75981=CARTESIAN_POINT ( 'NONE',  ( 97.93745859118190822, -30.45679909449765432, 161.8594347997199918 ) ) ;
#75982=LINE ( 'NONE', #55505, #60892 ) ;
#75983=ORIENTED_EDGE ( 'NONE', *, *, #13090, .T. ) ;
#75985=DIRECTION ( 'NONE',  ( 0.7071067811861728725, -0.7071067811869222730, 0.000000000000000000 ) ) ;
#75988=AXIS2_PLACEMENT_3D ( 'NONE', #18710, #88666, #72787 ) ;
#75990=ORIENTED_EDGE ( 'NONE', *, *, #33598, .F. ) ;
#75992=FACE_OUTER_BOUND ( 'NONE', #54912, .T. ) ;
#75993=AXIS2_PLACEMENT_3D ( 'NONE', #77343, #14682, #55975 ) ;
#75994=CARTESIAN_POINT ( 'NONE',  ( 99.58293739761768393, -32.55228987500129278, 110.3438483995049495 ) ) ;
#75995=CARTESIAN_POINT ( 'NONE',  ( 115.5353962700893788, -29.58991257470437120, 224.3718157521009573 ) ) ;
#75996=CARTESIAN_POINT ( 'NONE',  ( 104.4591861284129948, -26.65816784528755790, 200.2784824187679362 ) ) ;
#75997=CARTESIAN_POINT ( 'NONE',  ( 117.3629797429380659, -38.21633193987522503, 24.71276813305395237 ) ) ;
#75998=CARTESIAN_POINT ( 'NONE',  ( 48.45959712128969699, -28.98061976758959801, 193.9678068554150911 ) ) ;
#75999=CARTESIAN_POINT ( 'NONE',  ( 98.30745363658094504, -41.72867870133166690, 92.73977502107145199 ) ) ;
#76000=EDGE_CURVE ( 'NONE', #25675, #10962, #58533, .T. ) ;
#76002=CARTESIAN_POINT ( 'NONE',  ( 112.7054497023526807, -28.73785826246136921, 129.5870538473399449 ) ) ;
#76004=CARTESIAN_POINT ( 'NONE',  ( 104.7497970125497204, -46.93922829031851762, 72.39848241876795498 ) ) ;
#76005=CARTESIAN_POINT ( 'NONE',  ( 101.6276731664663089, -45.67517298127779668, 247.1413395616249602 ) ) ;
#76008=CARTESIAN_POINT ( 'NONE',  ( 115.2518872279481030, -30.21599423016839836, 244.3613395616249875 ) ) ;
#76009=CARTESIAN_POINT ( 'NONE',  ( 115.0889047178942661, -30.61763667089422469, 34.34395861009651441 ) ) ;
#76010=CARTESIAN_POINT ( 'NONE',  ( 41.56648329127499153, -27.82844715994070484, 23.67562527591200094 ) ) ;
#76014=DIRECTION ( 'NONE',  ( 0.7071067811571405404, 0.7071067812159546051, 0.000000000000000000 ) ) ;
#76015=DIRECTION ( 'NONE',  ( -3.999999999999999995E-14, 1.000000000000000000, -4.100000000000000342E-29 ) ) ;
#76016=PLANE ( 'NONE',  #84463 ) ;
#76017=DIRECTION ( 'NONE',  ( 0.000000000000000000, 0.000000000000000000, 1.000000000000000000 ) ) ;
#76018=CARTESIAN_POINT ( 'NONE',  ( 46.83715912545343940, -47.82818131006086304, 129.9678068554150911 ) ) ;
#76022=CYLINDRICAL_SURFACE ( 'NONE', #78253, 3.299999999999999822 ) ;
#76023=CARTESIAN_POINT ( 'NONE',  ( 97.31584372647238013, -39.30597603972135801, 261.5314586125417122 ) ) ;
#76024=ORIENTED_EDGE ( 'NONE', *, *, #38346, .T. ) ;
#76025=FACE_OUTER_BOUND ( 'NONE', #53491, .T. ) ;
#76026=CARTESIAN_POINT ( 'NONE',  ( 111.8742750991676758, -46.04467666623092015, 272.9556252759110180 ) ) ;
#76027=CARTESIAN_POINT ( 'NONE',  ( 100.8865061632069882, -45.89117093204367137, 148.0918157521009562 ) ) ;
#76028=CARTESIAN_POINT ( 'NONE',  ( 117.5342389965484386, -35.85531600229182914, 249.8927681330537780 ) ) ;
#76033=FACE_OUTER_BOUND ( 'NONE', #8301, .T. ) ;
#76035=CARTESIAN_POINT ( 'NONE',  ( 128.0667039024480118, -58.72944715994112386, 198.9178068554149945 ) ) ;
#76037=EDGE_CURVE ( 'NONE', #80917, #82312, #38986, .T. ) ;
#76038=CARTESIAN_POINT ( 'NONE',  ( 112.4311324297980406, -44.02555639339375659, 182.4914674471249612 ) ) ;
#76040=ORIENTED_EDGE ( 'NONE', *, *, #80627, .T. ) ;
#76041=DIRECTION ( 'NONE',  ( 0.000000000000000000, 0.000000000000000000, -1.000000000000000000 ) ) ;
#76042=EDGE_CURVE ( 'NONE', #12758, #17652, #65794, .T. ) ;
#76043=CARTESIAN_POINT ( 'NONE',  ( 108.2752786314947286, -47.69320359391959840, 153.6518157521009584 ) ) ;
#76044=DIRECTION ( 'NONE',  ( 0.000000000000000000, 0.000000000000000000, -1.000000000000000000 ) ) ;
#76048=CARTESIAN_POINT ( 'NONE',  ( 97.81168895331838087, -40.51742574516882200, 287.6356252759109680 ) ) ;
#76049=CARTESIAN_POINT ( 'NONE',  ( 108.8666348730871221, -46.34312957481634498, 82.72419670448294937 ) ) ;
#76051=ORIENTED_EDGE ( 'NONE', *, *, #76054, .T. ) ;
#76052=ORIENTED_EDGE ( 'NONE', *, *, #62679, .F. ) ;
#76053=CIRCLE ( 'NONE', #15179, 13.99999999999999822 ) ;
#76054=EDGE_CURVE ( 'NONE', #48698, #19610, #9962, .T. ) ;
#76055=CYLINDRICAL_SURFACE ( 'NONE', #21103, 10.04999999999999361 ) ;
#76056=CARTESIAN_POINT ( 'NONE',  ( 109.4488926988246504, -27.20905326525217660, 195.8813395616249977 ) ) ;
#76057=DIRECTION ( 'NONE',  ( 0.000000000000000000, 0.000000000000000000, -1.000000000000000000 ) ) ;
#76058=AXIS2_PLACEMENT_3D ( 'NONE', #46267, #65837, #4521 ) ;
#76060=DIRECTION ( 'NONE',  ( 0.000000000000000000, 1.000000000000000000, 0.000000000000000000 ) ) ;
#76061=EDGE_CURVE ( 'NONE', #35213, #26343, #10399, .T. ) ;
#76063=FACE_OUTER_BOUND ( 'NONE', #32525, .T. ) ;
#76065=CARTESIAN_POINT ( 'NONE',  ( 102.4028819069269218, -26.73371583578772004, 135.4118157521009493 ) ) ;
#76067=EDGE_LOOP ( 'NONE', ( #76778, #294, #12536, #79451 ) ) ;
#76068=ORIENTED_EDGE ( 'NONE', *, *, #5223, .T. ) ;
#76069=DIRECTION ( 'NONE',  ( 4.825893423866870279E-33, 0.000000000000000000, -1.000000000000000000 ) ) ;
#76072=CARTESIAN_POINT ( 'NONE',  ( 108.3259390676978455, -28.66449228317154763, 187.7709475124489700 ) ) ;
#76073=CIRCLE ( 'NONE', #55682, 2.517500000000005844 ) ;
#76077=CIRCLE ( 'NONE', #2115, 3.249999999999975131 ) ;
#76078=LINE ( 'NONE', #27038, #15594 ) ;
#76080=VERTEX_POINT ( 'NONE', #38104 ) ;
#76085=ORIENTED_EDGE ( 'NONE', *, *, #86846, .F. ) ;
#76087=CARTESIAN_POINT ( 'NONE',  ( 77.76764265987219460, -20.23887630717950259, 7.293197373621064905 ) ) ;
#76088=CARTESIAN_POINT ( 'NONE',  ( 106.2775494337459037, -46.09182447052010190, 258.9292023535161889 ) ) ;
#76090=EDGE_CURVE ( 'NONE', #70, #43353, #73511, .T. ) ;
#76091=DIRECTION ( 'NONE',  ( 0.000000000000000000, 0.000000000000000000, 1.000000000000000000 ) ) ;
#76093=ORIENTED_EDGE ( 'NONE', *, *, #83241, .F. ) ;
#76094=ORIENTED_EDGE ( 'NONE', *, *, #46308, .T. ) ;
#76095=DIRECTION ( 'NONE',  ( 1.639958061481212836E-42, -4.100000000000000342E-29, -1.000000000000000000 ) ) ;
#76097=VERTEX_POINT ( 'NONE', #4482 ) ;
#76099=CARTESIAN_POINT ( 'NONE',  ( 98.84295822536005005, -39.42912807745279480, 284.4090427505438470 ) ) ;
#76100=CARTESIAN_POINT ( 'NONE',  ( 102.2921677216391174, -27.39701587636625391, 120.4527681330539792 ) ) ;
#76101=CARTESIAN_POINT ( 'NONE',  ( 102.9796410358629828, -46.29638950891627047, 92.25562527591097250 ) ) ;
#76102=CARTESIAN_POINT ( 'NONE',  ( 108.5950374404567071, -44.93858127607868624, 249.5838068554168387 ) ) ;
#76103=CARTESIAN_POINT ( 'NONE',  ( 131.5325842222575830, -17.66080143920384771, 7.039723185229114222 ) ) ;
#76104=CARTESIAN_POINT ( 'NONE',  ( 113.7506423937859807, -44.72972868871420360, 189.1299109901969757 ) ) ;
#76106=FACE_OUTER_BOUND ( 'NONE', #82646, .T. ) ;
#76107=ORIENTED_EDGE ( 'NONE', *, *, #64014, .F. ) ;
#76108=LINE ( 'NONE', #77019, #17769 ) ;
#76111=CARTESIAN_POINT ( 'NONE',  ( 51.34673845256598668, -36.02818131005800950, -5.074374724088000832 ) ) ;
#76115=CARTESIAN_POINT ( 'NONE',  ( 97.98636869442889008, -41.85180495037556625, 136.7356252759109623 ) ) ;
#76117=VECTOR ( 'NONE', #23431, 1000.000000000000000 ) ;
#76118=LINE ( 'NONE', #61144, #39128 ) ;
#76119=CARTESIAN_POINT ( 'NONE',  ( 168.3664380525673607, -48.62818131005418110, 300.4678068554149490 ) ) ;
#76120=DIRECTION ( 'NONE',  ( 1.000000000000000078E-15, -1.000000000000000083E-30, -1.000000000000000000 ) ) ;
#76122=CARTESIAN_POINT ( 'NONE',  ( 118.7655994573050577, -38.45539276985793720, 219.7099109901969882 ) ) ;
#76123=DIRECTION ( 'NONE',  ( 0.000000000000000000, 0.000000000000000000, -1.000000000000000000 ) ) ;
#76124=DIRECTION ( 'NONE',  ( -0.000000000000000000, -0.000000000000000000, -1.000000000000000000 ) ) ;
#76125=ORIENTED_EDGE ( 'NONE', *, *, #29283, .F. ) ;
#76126=DIRECTION ( 'NONE',  ( 1.000000000000000078E-15, -1.000000000000000000, 0.000000000000000000 ) ) ;
#76128=CARTESIAN_POINT ( 'NONE',  ( 107.0664832912739968, -36.72944715994100306, 294.6356252759106837 ) ) ;
#76130=CARTESIAN_POINT ( 'NONE',  ( 106.5394234437989667, -24.24056378642895737, 322.0356252759110021 ) ) ;
#76131=VERTEX_POINT ( 'NONE', #58971 ) ;
#76132=DIRECTION ( 'NONE',  ( -1.000000000000000078E-15, 1.000000000000000083E-30, 1.000000000000000000 ) ) ;
#76133=CARTESIAN_POINT ( 'NONE',  ( 96.64877318785802629, -35.94450158219160585, 146.2670538473399517 ) ) ;
#76134=CARTESIAN_POINT ( 'NONE',  ( 111.3231501057927346, -27.21297328954094041, 20.74133956162494030 ) ) ;
#76135=CARTESIAN_POINT ( 'NONE',  ( 103.0329776526464087, -26.38883157761164000, 166.3603871806729444 ) ) ;
#76136=DIRECTION ( 'NONE',  ( 0.000000000000000000, 0.000000000000000000, -1.000000000000000000 ) ) ;
#76137=CARTESIAN_POINT ( 'NONE',  ( 194.5664832912739826, -18.82844715994099971, 342.9256252759119548 ) ) ;
#76139=DIRECTION ( 'NONE',  ( 1.000000000000000000, 3.083952846180989689E-15, 1.541976423090494844E-15 ) ) ;
#76140=DIRECTION ( 'NONE',  ( 1.387778780781444413E-14, -1.000000000000000000, 0.000000000000000000 ) ) ;
#76141=FACE_OUTER_BOUND ( 'NONE', #75848, .T. ) ;
#76144=VECTOR ( 'NONE', #19064, 1000.000000000000000 ) ;
#76145=CIRCLE ( 'NONE', #45695, 1.000000000000000888 ) ;
#76147=ORIENTED_EDGE ( 'NONE', *, *, #18724, .T. ) ;
#76148=ORIENTED_EDGE ( 'NONE', *, *, #50054, .T. ) ;
#76149=EDGE_CURVE ( 'NONE', #56141, #77917, #18094, .T. ) ;
#76150=TOROIDAL_SURFACE ( 'NONE', #68897, 7.799999999999999822, 0.2999999999999999889 ) ;
#76151=VECTOR ( 'NONE', #27785, 1000.000000000000000 ) ;
#76153=CARTESIAN_POINT ( 'NONE',  ( 83.06670390244796920, -61.87844715994100397, 231.5838068554150198 ) ) ;
#76154=CARTESIAN_POINT ( 'NONE',  ( 99.51750086509218818, -43.88776608678588786, 77.92991099019597812 ) ) ;
#76155=CARTESIAN_POINT ( 'NONE',  ( 138.8167039024479834, -57.40094715994099772, 63.03480685541479289 ) ) ;
#76158=CARTESIAN_POINT ( 'NONE',  ( 117.5007279078441655, -40.51415819784174488, 169.5375300378159693 ) ) ;
#76161=VECTOR ( 'NONE', #76381, 1000.000000000000000 ) ;
#76162=CARTESIAN_POINT ( 'NONE',  ( 110.9972015515846238, -44.34532242709460093, 272.3781341137911909 ) ) ;
#76163=ORIENTED_EDGE ( 'NONE', *, *, #13072, .F. ) ;
#76166=DIRECTION ( 'NONE',  ( 4.299999999999999979E-14, -1.000000000000000000, 0.000000000000000000 ) ) ;
#76167=CARTESIAN_POINT ( 'NONE',  ( 126.0667039024479550, -14.72944715994094977, 199.5838068554170093 ) ) ;
#76169=VECTOR ( 'NONE', #23421, 1000.000000000000114 ) ;
#76170=DIRECTION ( 'NONE',  ( -1.000000000000000078E-15, 1.000000000000000083E-30, 1.000000000000000000 ) ) ;
#76173=EDGE_CURVE ( 'NONE', #54590, #32962, #14325, .T. ) ;
#76176=CARTESIAN_POINT ( 'NONE',  ( 106.2538455105912050, -26.32252419718678027, 25.13848241876792855 ) ) ;
#76177=CARTESIAN_POINT ( 'NONE',  ( 71.24076473329810710, 5.642044068322332961, 394.9756252759101471 ) ) ;
#76178=ORIENTED_EDGE ( 'NONE', *, *, #63517, .T. ) ;
#76179=CARTESIAN_POINT ( 'NONE',  ( 97.81136857581559241, -40.51756142658395987, 157.6353372204761456 ) ) ;
#76180=DIRECTION ( 'NONE',  ( 0.000000000000000000, 0.000000000000000000, -1.000000000000000000 ) ) ;
#76181=CARTESIAN_POINT ( 'NONE',  ( 97.89197038913195570, -35.34227587553755257, 69.02523322673498285 ) ) ;
#76182=VECTOR ( 'NONE', #31406, 1000.000000000000000 ) ;
#76183=AXIS2_PLACEMENT_3D ( 'NONE', #2966, #72454, #51971 ) ;
#76185=CARTESIAN_POINT ( 'NONE',  ( 51.06648329127400388, 12.92155284005902516, 333.4006252759110112 ) ) ;
#76186=ORIENTED_EDGE ( 'NONE', *, *, #85613, .F. ) ;
#76188=CARTESIAN_POINT ( 'NONE',  ( 78.80082187618229739, -34.28157759250729697, 7.978179524066798756 ) ) ;
#76190=CARTESIAN_POINT ( 'NONE',  ( 98.85647153018690858, -30.30415715074617111, 155.7984824187679465 ) ) ;
#76191=ORIENTED_EDGE ( 'NONE', *, *, #40466, .F. ) ;
#76192=CARTESIAN_POINT ( 'NONE',  ( 100.8874679282520788, -44.70022140857566484, 68.05229194691942496 ) ) ;
#76193=CARTESIAN_POINT ( 'NONE',  ( 99.18485448662231363, -41.84413841198986006, 143.2282499725629634 ) ) ;
#76195=DIRECTION ( 'NONE',  ( 1.000000000000000078E-15, -1.000000000000000083E-30, -1.000000000000000000 ) ) ;
#76196=CARTESIAN_POINT ( 'NONE',  ( 117.4762281475856724, -37.96087228405902181, 49.73276813305393773 ) ) ;
#76198=AXIS2_PLACEMENT_3D ( 'NONE', #29144, #71385, #57275 ) ;
#76200=CARTESIAN_POINT ( 'NONE',  ( 48.79742451361987321, -36.32844715994078655, 193.9678068554150911 ) ) ;
#76201=AXIS2_PLACEMENT_3D ( 'NONE', #65989, #2895, #16085 ) ;
#76203=EDGE_LOOP ( 'NONE', ( #5709, #4250, #51086, #59372 ) ) ;
#76206=AXIS2_PLACEMENT_3D ( 'NONE', #13037, #26646, #41159 ) ;
#76207=CARTESIAN_POINT ( 'NONE',  ( 107.0664832912739968, -36.72944715994100306, 287.6356252759109680 ) ) ;
#76209=CARTESIAN_POINT ( 'NONE',  ( 100.4593435015893164, -29.47291325643525184, 285.6641967044828334 ) ) ;
#76210=CARTESIAN_POINT ( 'NONE',  ( 97.96758126215280527, -41.86240348953004542, 132.7356252759109623 ) ) ;
#76211=LINE ( 'NONE', #88954, #64059 ) ;
#76213=CARTESIAN_POINT ( 'NONE',  ( 113.5060836576900272, -28.53103057085638383, 75.54705384733995288 ) ) ;
#76214=CARTESIAN_POINT ( 'NONE',  ( 104.4081006910507341, -46.45808914803028955, 262.3647919450149288 ) ) ;
#76216=AXIS2_PLACEMENT_3D ( 'NONE', #37626, #71701, #29466 ) ;
#76218=CARTESIAN_POINT ( 'NONE',  ( 109.6433497169441722, -46.48000174799164341, 158.7813111578553844 ) ) ;
#76219=CONICAL_SURFACE ( 'NONE', #79163, 1.624999999999987566, 1.029744258676650093 ) ;
#76222=EDGE_CURVE ( 'NONE', #29668, #36866, #72939, .T. ) ;
#76223=DIRECTION ( 'NONE',  ( -4.237773401492740281E-14, 1.000000000000000000, 0.000000000000000000 ) ) ;
#76224=CARTESIAN_POINT ( 'NONE',  ( 100.4109522542116650, -28.70505079160765760, 40.62705384733894221 ) ) ;
#76226=VECTOR ( 'NONE', #3309, 1000.000000000000000 ) ;
#76227=DIRECTION ( 'NONE',  ( 9.351236661543306751E-17, -3.725950533538267725E-29, -1.000000000000000000 ) ) ;
#76228=CARTESIAN_POINT ( 'NONE',  ( 115.0393671692859101, -42.90578492219520967, 93.30325341284572005 ) ) ;
#76229=CARTESIAN_POINT ( 'NONE',  ( 115.3963617111076445, -41.85549503053864839, 18.38705384734096171 ) ) ;
#76230=CARTESIAN_POINT ( 'NONE',  ( 104.5295158156824584, -26.96092172908695161, 100.2802235910898787 ) ) ;
#76231=CARTESIAN_POINT ( 'NONE',  ( 107.3333893024683903, -26.32957087652229689, 116.0556252759109555 ) ) ;
#76233=CARTESIAN_POINT ( 'NONE',  ( 101.7470617766046956, -45.74667603143129924, 162.1527681330539679 ) ) ;
#76234=DIRECTION ( 'NONE',  ( 1.000000000000000000, 1.000000000000000078E-15, 1.000000000000000078E-15 ) ) ;
#76235=ORIENTED_EDGE ( 'NONE', *, *, #82838, .F. ) ;
#76236=DIRECTION ( 'NONE',  ( 0.000000000000000000, 0.000000000000000000, -1.000000000000000000 ) ) ;
#76240=VERTEX_POINT ( 'NONE', #26695 ) ;
#76241=EDGE_CURVE ( 'NONE', #76131, #78184, #5373, .T. ) ;
#76244=CARTESIAN_POINT ( 'NONE',  ( 117.0593108693811786, -33.60693806652478344, 174.0670538473389399 ) ) ;
#76247=CARTESIAN_POINT ( 'NONE',  ( 106.9401787849546537, -47.80506239865356122, 228.5794347997199907 ) ) ;
#76252=ORIENTED_EDGE ( 'NONE', *, *, #78750, .T. ) ;
#76253=EDGE_CURVE ( 'NONE', #4135, #14684, #46685, .T. ) ;
#76257=DIRECTION ( 'NONE',  ( 1.000000000000000000, 3.999999999999999995E-14, 1.000000000000000078E-15 ) ) ;
#76258=CARTESIAN_POINT ( 'NONE',  ( 97.16978355702093495, -40.00630874038032658, 237.5813395616249579 ) ) ;
#76261=ADVANCED_FACE ( 'NONE', ( #39874 ), #13503, .F. ) ;
#76262=DIRECTION ( 'NONE',  ( -1.000000000000000078E-15, -1.000000000000000083E-30, 1.000000000000000000 ) ) ;
#76264=CARTESIAN_POINT ( 'NONE',  ( 33.92127028473601769, -29.73316016639540749, -5.074374724088000832 ) ) ;
#76265=CARTESIAN_POINT ( 'NONE',  ( 104.7307148508592007, -47.55717207929887991, 32.41943479972098174 ) ) ;
#76268=EDGE_LOOP ( 'NONE', ( #72314, #40951, #48425, #46327 ) ) ;
#76270=VECTOR ( 'NONE', #15527, 1000.000000000000000 ) ;
#76274=CARTESIAN_POINT ( 'NONE',  ( 116.3159835831961857, -41.41832011455023377, 244.4651490854349731 ) ) ;
#76275=CARTESIAN_POINT ( 'NONE',  ( 31.56670390244800117, -32.29483332968611364, 342.9256252759109884 ) ) ;
#76276=ADVANCED_FACE ( 'NONE', ( #32613 ), #40325, .T. ) ;
#76277=CARTESIAN_POINT ( 'NONE',  ( 102.0418483691416895, -28.29933337693059414, 81.50419670448194154 ) ) ;
#76278=CARTESIAN_POINT ( 'NONE',  ( 177.0371591254543091, -48.62818131005480637, 313.9678068554149490 ) ) ;
#76282=ORIENTED_EDGE ( 'NONE', *, *, #38037, .T. ) ;
#76283=CARTESIAN_POINT ( 'NONE',  ( 177.0664832912730162, 12.92155284005730387, 361.9756252759109998 ) ) ;
#76285=ORIENTED_EDGE ( 'NONE', *, *, #73982, .T. ) ;
#76289=CARTESIAN_POINT ( 'NONE',  ( 116.4516747918435300, -36.28819209217700603, 265.2834880678017839 ) ) ;
#76290=DIRECTION ( 'NONE',  ( 1.000000000000000000, 4.237773401492740281E-14, 0.000000000000000000 ) ) ;
#76292=CIRCLE ( 'NONE', #54470, 0.5000000000000004441 ) ;
#76293=CARTESIAN_POINT ( 'NONE',  ( 98.34985892274558239, -31.65658479228161681, 85.90645860766178998 ) ) ;
#76297=CARTESIAN_POINT ( 'NONE',  ( 104.4070256631273850, -46.45777391140720169, 183.3652439674835932 ) ) ;
#76299=CARTESIAN_POINT ( 'NONE',  ( 106.6068369155051698, -25.68554329116653534, 40.09753003781596448 ) ) ;
#76300=VERTEX_POINT ( 'NONE', #46701 ) ;
#76301=CARTESIAN_POINT ( 'NONE',  ( 99.09762411907954061, -31.97621503831505407, 278.7166617981628178 ) ) ;
#76302=CARTESIAN_POINT ( 'NONE',  ( 115.7840093042128018, -41.80077732092177456, 128.4066342822487456 ) ) ;
#76303=CARTESIAN_POINT ( 'NONE',  ( 113.1634500054122583, -44.41975088505045477, 168.1099109901969939 ) ) ;
#76305=LINE ( 'NONE', #1355, #62164 ) ;
#76306=LINE ( 'NONE', #40877, #17273 ) ;
#76308=CARTESIAN_POINT ( 'NONE',  ( 116.0926836276447460, -42.03234139191665975, 234.4041967044819899 ) ) ;
#76310=ORIENTED_EDGE ( 'NONE', *, *, #88777, .F. ) ;
#76311=CARTESIAN_POINT ( 'NONE',  ( 136.5146477271286187, -37.98222059078806012, 7.138441653514234098 ) ) ;
#76312=ORIENTED_EDGE ( 'NONE', *, *, #86270, .T. ) ;
#76313=CARTESIAN_POINT ( 'NONE',  ( 117.1483892680215888, -39.54869380112744892, 94.60991099019693706 ) ) ;
#76316=VERTEX_POINT ( 'NONE', #53502 ) ;
#76317=ORIENTED_EDGE ( 'NONE', *, *, #86522, .F. ) ;
#76320=FACE_OUTER_BOUND ( 'NONE', #21199, .T. ) ;
#76321=DIRECTION ( 'NONE',  ( 1.000000000000000000, 0.000000000000000000, 0.000000000000000000 ) ) ;
#76322=CARTESIAN_POINT ( 'NONE',  ( 100.6382899380647871, -31.69863749346629689, 153.6166617981629656 ) ) ;
#76323=CARTESIAN_POINT ( 'NONE',  ( 112.6753912189806073, -45.54292608213916793, 259.0270538473393458 ) ) ;
#76324=CARTESIAN_POINT ( 'NONE',  ( 97.82520644204963389, -40.55030899666594024, 57.63845489205286299 ) ) ;
#76325=ORIENTED_EDGE ( 'NONE', *, *, #10608, .F. ) ;
#76327=AXIS2_PLACEMENT_3D ( 'NONE', #29961, #59428, #23169 ) ;
#76328=CARTESIAN_POINT ( 'NONE',  ( 107.0664832912739968, -18.82844715994099971, 168.9256252759119832 ) ) ;
#76331=CIRCLE ( 'NONE', #19728, 9.999999999999994671 ) ;
#76332=CIRCLE ( 'NONE', #77901, 2.750000000000002665 ) ;
#76333=DIRECTION ( 'NONE',  ( 1.000000000000000078E-15, -1.000000000000000083E-30, -1.000000000000000000 ) ) ;
#76335=EDGE_CURVE ( 'NONE', #54231, #82906, #88522, .T. ) ;
#76336=DIRECTION ( 'NONE',  ( 0.000000000000000000, 0.000000000000000000, -1.000000000000000000 ) ) ;
#76337=CARTESIAN_POINT ( 'NONE',  ( 97.80833607050627165, -40.50923396610764371, 16.63492042907981272 ) ) ;
#76338=AXIS2_PLACEMENT_3D ( 'NONE', #16423, #64568, #4119 ) ;
#76339=EDGE_CURVE ( 'NONE', #53860, #59559, #68515, .T. ) ;
#76340=CARTESIAN_POINT ( 'NONE',  ( 162.7131505118539962, -33.70561438052090608, -5.074374724088000832 ) ) ;
#76341=DIRECTION ( 'NONE',  ( -1.000000000000000078E-15, 1.000000000000000083E-30, 1.000000000000000000 ) ) ;
#76342=CARTESIAN_POINT ( 'NONE',  ( 98.15635076299318484, -32.87196533591951919, 210.4238483995049762 ) ) ;
#76343=CARTESIAN_POINT ( 'NONE',  ( 104.0299312746664526, -47.40616179873944702, 67.36800622829191809 ) ) ;
#76345=ORIENTED_EDGE ( 'NONE', *, *, #20696, .T. ) ;
#76346=EDGE_CURVE ( 'NONE', #30351, #58675, #53986, .T. ) ;
#76349=ADVANCED_FACE ( 'NONE', ( #32184 ), #67612, .T. ) ;
#76353=CARTESIAN_POINT ( 'NONE',  ( 116.3175913315759402, -32.94491325663879877, 165.1356252759109680 ) ) ;
#76354=FACE_OUTER_BOUND ( 'NONE', #8355, .T. ) ;
#76355=CARTESIAN_POINT ( 'NONE',  ( 97.81252181392954981, -40.51708140501057187, 272.6353344860016819 ) ) ;
#76358=CARTESIAN_POINT ( 'NONE',  ( 83.06670390244796920, -61.87844715994100397, 213.1838068554149856 ) ) ;
#76359=VERTEX_POINT ( 'NONE', #26277 ) ;
#76360=CARTESIAN_POINT ( 'NONE',  ( 118.0120547386033678, -38.42941975617429762, 68.69181575210198787 ) ) ;
#76364=CARTESIAN_POINT ( 'NONE',  ( 91.42390633313587500, -35.38788608837992911, 293.9356252759109793 ) ) ;
#76366=CARTESIAN_POINT ( 'NONE',  ( 163.0959832912772356, -23.42844715993520310, 193.9678068554149775 ) ) ;
#76368=ORIENTED_EDGE ( 'NONE', *, *, #71960, .F. ) ;
#76369=LINE ( 'NONE', #21867, #35865 ) ;
#76370=EDGE_CURVE ( 'NONE', #36669, #3392, #67158, .T. ) ;
#76371=LINE ( 'NONE', #28202, #31283 ) ;
#76373=ORIENTED_EDGE ( 'NONE', *, *, #21621, .F. ) ;
#76374=CARTESIAN_POINT ( 'NONE',  ( 98.18387371117843543, -43.34642931133835475, 107.8480062282919647 ) ) ;
#76377=CARTESIAN_POINT ( 'NONE',  ( 130.5667039024480118, -36.72944715994093912, 219.5838068554170093 ) ) ;
#76379=ORIENTED_EDGE ( 'NONE', *, *, #34478, .T. ) ;
#76380=CARTESIAN_POINT ( 'NONE',  ( 98.98846131648984681, -42.30253745798191289, 122.8070538473389490 ) ) ;
#76381=DIRECTION ( 'NONE',  ( 0.7071067811864980568, 0.7071067811865969777, 0.000000000000000000 ) ) ;
#76383=CARTESIAN_POINT ( 'NONE',  ( 100.2615012876618295, -45.41023301258249489, 273.0594347997205773 ) ) ;
#76384=CARTESIAN_POINT ( 'NONE',  ( 97.81455683053849270, -40.52442650171994387, 252.6361864024953547 ) ) ;
#76385=CARTESIAN_POINT ( 'NONE',  ( 131.0667039024480118, -42.21678055153905262, 231.5838068554170093 ) ) ;
#76387=FACE_OUTER_BOUND ( 'NONE', #49024, .T. ) ;
#76389=CARTESIAN_POINT ( 'NONE',  ( 131.0667039024480118, -58.72944715994098175, 231.5838068554150198 ) ) ;
#76390=CARTESIAN_POINT ( 'NONE',  ( 180.1667039024460166, -28.27351298637340093, -5.074374724088000832 ) ) ;
#76391=EDGE_CURVE ( 'NONE', #19911, #68206, #52603, .T. ) ;
#76392=AXIS2_PLACEMENT_3D ( 'NONE', #87833, #4264, #3816 ) ;
#76393=CARTESIAN_POINT ( 'NONE',  ( 117.2610056464983899, -34.82931580038571440, 203.9851490854349549 ) ) ;
#76395=EDGE_LOOP ( 'NONE', ( #83275, #54167, #82178, #35492 ) ) ;
#76396=CARTESIAN_POINT ( 'NONE',  ( 115.9244277637092040, -39.86207309682762912, 174.9996785439919904 ) ) ;
#76397=AXIS2_PLACEMENT_3D ( 'NONE', #33344, #82412, #61041 ) ;
#76400=CARTESIAN_POINT ( 'NONE',  ( 116.7892270756567967, -35.66563809766837778, 274.9127681330532482 ) ) ;
#76401=CIRCLE ( 'NONE', #88013, 3.000000000000002665 ) ;
#76402=CARTESIAN_POINT ( 'NONE',  ( 134.0664832912740110, -8.729447159940999512, 296.1531252759119752 ) ) ;
#76403=CARTESIAN_POINT ( 'NONE',  ( 112.0652091731003139, -45.48878794064455633, 267.9899078305007833 ) ) ;
#76406=CARTESIAN_POINT ( 'NONE',  ( 163.1543517358360020, -31.62489322948790971, -5.074374724088000832 ) ) ;
#76407=CARTESIAN_POINT ( 'NONE',  ( 114.5897159479186342, -29.54407062678533791, 234.4327681330539690 ) ) ;
#76408=CARTESIAN_POINT ( 'NONE',  ( 32.24491389929970353, -32.11662333284649407, 193.9678068554150911 ) ) ;
#76411=LINE ( 'NONE', #14188, #44480 ) ;
#76414=LINE ( 'NONE', #89608, #18679 ) ;
#76416=LINE ( 'NONE', #47793, #28147 ) ;
#76417=CLOSED_SHELL ( 'NONE', ( #34398, #65164, #52398, #8682 ) ) ;
#76418=ORIENTED_EDGE ( 'NONE', *, *, #18499, .F. ) ;
#76419=CARTESIAN_POINT ( 'NONE',  ( 116.5137666388868780, -32.21926627522912412, 15.18133956162492915 ) ) ;
#76420=CARTESIAN_POINT ( 'NONE',  ( 100.1386363970297992, -44.51995214173314963, 266.9984824187679919 ) ) ;
#76422=CARTESIAN_POINT ( 'NONE',  ( 77.55551418447849699, -37.85480617631969835, 7.067502061087529874 ) ) ;
#76423=DIRECTION ( 'NONE',  ( -0.7071067811985215501, 0.7071067811745735954, 0.000000000000000000 ) ) ;
#76424=CARTESIAN_POINT ( 'NONE',  ( 41.56648329127499153, -32.07844715994070839, 14.17562527591199917 ) ) ;
#76425=CARTESIAN_POINT ( 'NONE',  ( 114.6445280793269603, -33.69580855137893138, 51.94809036959197357 ) ) ;
#76426=CARTESIAN_POINT ( 'NONE',  ( 117.0891209002388678, -39.67630891660421355, 179.5984824187679294 ) ) ;
#76428=ORIENTED_EDGE ( 'NONE', *, *, #20201, .T. ) ;
#76429=CARTESIAN_POINT ( 'NONE',  ( 37.03715912545433042, -48.62818131006122258, 249.9678068554150343 ) ) ;
#76432=ORIENTED_EDGE ( 'NONE', *, *, #27705, .T. ) ;
#76433=PLANE ( 'NONE',  #34324 ) ;
#76434=ORIENTED_EDGE ( 'NONE', *, *, #4468, .T. ) ;
#76435=EDGE_LOOP ( 'NONE', ( #86694, #8922 ) ) ;
#76437=EDGE_CURVE ( 'NONE', #38582, #11954, #12654, .T. ) ;
#76438=EDGE_CURVE ( 'NONE', #39122, #33219, #80364, .T. ) ;
#76439=CARTESIAN_POINT ( 'NONE',  ( 103.3727720482000620, -29.02797788616916108, 94.85527697093499455 ) ) ;
#76440=CARTESIAN_POINT ( 'NONE',  ( 106.5662725644766908, -47.20027100765710060, 247.5384824187679556 ) ) ;
#76442=CARTESIAN_POINT ( 'NONE',  ( 112.1942863616536386, -45.78120396183496155, 212.9870538473389558 ) ) ;
#76443=CARTESIAN_POINT ( 'NONE',  ( 117.0705705820183482, -32.08379757587637471, 55.16038718067301261 ) ) ;
#76446=EDGE_CURVE ( 'NONE', #72723, #76939, #13110, .T. ) ;
#76447=EDGE_LOOP ( 'NONE', ( #49406, #89176, #34965, #25477 ) ) ;
#76448=CARTESIAN_POINT ( 'NONE',  ( 108.3334480733278866, -46.73485935691606841, 177.6772919410516351 ) ) ;
#76449=AXIS2_PLACEMENT_3D ( 'NONE', #29033, #56718, #12651 ) ;
#76451=CARTESIAN_POINT ( 'NONE',  ( 181.9790560690580037, -31.62489322948711035, 117.4678068554150627 ) ) ;
#76452=EDGE_CURVE ( 'NONE', #50846, #1932, #54399, .T. ) ;
#76453=CARTESIAN_POINT ( 'NONE',  ( 104.2906771502715628, -46.10805769451172864, 107.3470538473399500 ) ) ;
#76454=CARTESIAN_POINT ( 'NONE',  ( 103.8276485124378183, -46.72253193893131140, 82.32705384733995402 ) ) ;
#76456=CARTESIAN_POINT ( 'NONE',  ( 100.1483249706684546, -45.40999835672980112, 272.0289586092442278 ) ) ;
#76458=AXIS2_PLACEMENT_3D ( 'NONE', #73504, #32607, #80789 ) ;
#76459=CARTESIAN_POINT ( 'NONE',  ( 97.16957671423683962, -40.00637722736999535, 241.5813395616249863 ) ) ;
#76460=CARTESIAN_POINT ( 'NONE',  ( 29.56670390244743629, -48.82844715994161078, 180.4678068554150911 ) ) ;
#76462=CARTESIAN_POINT ( 'NONE',  ( 98.54762029648411215, -41.97692828339373960, 22.76579877019573672 ) ) ;
#76468=EDGE_CURVE ( 'NONE', #76300, #83795, #43481, .T. ) ;
#76469=FACE_OUTER_BOUND ( 'NONE', #26796, .T. ) ;
#76474=CARTESIAN_POINT ( 'NONE',  ( 102.0670549394996840, -27.97049807078126094, 260.4897919444414924 ) ) ;
#76476=PLANE ( 'NONE',  #23498 ) ;
#76477=CARTESIAN_POINT ( 'NONE',  ( 100.1240125862563275, -44.53639691489608765, 266.9984824187678782 ) ) ;
#76478=CARTESIAN_POINT ( 'NONE',  ( 96.01412018463531695, -36.58377574468403282, 152.3280062282919971 ) ) ;
#76479=CARTESIAN_POINT ( 'NONE',  ( 106.8354761508916226, -47.19556465630029862, 268.5584824187679374 ) ) ;
#76480=VECTOR ( 'NONE', #66108, 1000.000000000000000 ) ;
#76481=DIRECTION ( 'NONE',  ( 0.000000000000000000, 1.000000000000000000, 0.000000000000000000 ) ) ;
#76482=AXIS2_PLACEMENT_3D ( 'NONE', #88637, #47263, #48598 ) ;
#76483=LINE ( 'NONE', #43285, #75482 ) ;
#76484=DIRECTION ( 'NONE',  ( 1.000000000000000000, 1.271620792853953879E-14, 0.000000000000000000 ) ) ;
#76485=CARTESIAN_POINT ( 'NONE',  ( 97.81939108931598525, -40.53620304804683627, 137.6372407434755019 ) ) ;
#76486=CARTESIAN_POINT ( 'NONE',  ( 142.8821648370247885, -72.54478064608022692, 361.9756252759100335 ) ) ;
#76487=VECTOR ( 'NONE', #66339, 1000.000000000000000 ) ;
#76488=ORIENTED_EDGE ( 'NONE', *, *, #578, .F. ) ;
#76489=LINE ( 'NONE', #59820, #67897 ) ;
#76490=ORIENTED_EDGE ( 'NONE', *, *, #5919, .T. ) ;
#76491=CARTESIAN_POINT ( 'NONE',  ( 115.4591718486505698, -35.14231982251399700, 158.3981341137909737 ) ) ;
#76494=CYLINDRICAL_SURFACE ( 'NONE', #15655, 9.999999999999998224 ) ;
#76495=CARTESIAN_POINT ( 'NONE',  ( 108.0049669398584911, -26.36739623290736390, 151.0041967044829505 ) ) ;
#76496=PLANE ( 'NONE',  #54079 ) ;
#76498=CARTESIAN_POINT ( 'NONE',  ( 100.4979874790370644, -29.16083011470633224, 86.64560808839608796 ) ) ;
#76499=DIRECTION ( 'NONE',  ( -1.000000000000000078E-15, 1.000000000000000083E-30, 1.000000000000000000 ) ) ;
#76500=DIRECTION ( 'NONE',  ( 0.000000000000000000, 0.000000000000000000, -1.000000000000000000 ) ) ;
#76502=CARTESIAN_POINT ( 'NONE',  ( 104.0406618471960201, -46.06530165129709076, 82.32705384733995402 ) ) ;
#76504=VERTEX_POINT ( 'NONE', #83948 ) ;
#76506=VERTEX_POINT ( 'NONE', #62135 ) ;
#76507=CARTESIAN_POINT ( 'NONE',  ( 104.0154917791352744, -27.12933488216606648, 51.75301187732594599 ) ) ;
#76509=CARTESIAN_POINT ( 'NONE',  ( 99.07755742602716964, -44.46178485432842109, 187.9384824187679612 ) ) ;
#76512=DIRECTION ( 'NONE',  ( 0.000000000000000000, 1.000000000000000000, 0.000000000000000000 ) ) ;
#76513=CARTESIAN_POINT ( 'NONE',  ( 116.3212776292296127, -32.94146857471318413, 287.6356252759109680 ) ) ;
#76516=CARTESIAN_POINT ( 'NONE',  ( 114.6914383512288254, -44.69963429152232237, 113.1718157521009687 ) ) ;
#76517=ORIENTED_EDGE ( 'NONE', *, *, #69111, .F. ) ;
#76518=ORIENTED_EDGE ( 'NONE', *, *, #37865, .T. ) ;
#76520=ADVANCED_FACE ( 'NONE', ( #13992 ), #69412, .T. ) ;
#76523=VECTOR ( 'NONE', #55866, 1000.000000000000000 ) ;
#76525=CARTESIAN_POINT ( 'NONE',  ( 106.9948502263972188, -44.89183619263916825, 185.3880903695919642 ) ) ;
#76529=CYLINDRICAL_SURFACE ( 'NONE', #18911, 2.517499999999998739 ) ;
#76530=DIRECTION ( 'NONE',  ( 0.7071067811865157093, 0.7071067811865794361, 7.071067811865148942E-16 ) ) ;
#76532=EDGE_LOOP ( 'NONE', ( #48984, #5895, #36205, #38249 ) ) ;
#76535=CARTESIAN_POINT ( 'NONE',  ( 136.6144450028906192, -19.76411817599922216, 2.828498113172279727 ) ) ;
#76536=VERTEX_POINT ( 'NONE', #14901 ) ;
#76538=CARTESIAN_POINT ( 'NONE',  ( 34.67381068360452900, -28.98061976759034764, 237.4678068554150059 ) ) ;
#76539=CARTESIAN_POINT ( 'NONE',  ( 98.10010861879410982, -32.13871408278030373, 242.3815833058969815 ) ) ;
#76540=AXIS2_PLACEMENT_3D ( 'NONE', #3497, #11203, #65286 ) ;
#76542=VERTEX_POINT ( 'NONE', #812 ) ;
#76545=DIRECTION ( 'NONE',  ( 0.000000000000000000, 0.000000000000000000, -1.000000000000000000 ) ) ;
#76548=ORIENTED_EDGE ( 'NONE', *, *, #11947, .F. ) ;
#76552=ORIENTED_EDGE ( 'NONE', *, *, #17586, .T. ) ;
#76553=EDGE_CURVE ( 'NONE', #37760, #45213, #7628, .T. ) ;
#76555=CARTESIAN_POINT ( 'NONE',  ( 115.2503885696571047, -36.58558574821132936, 286.6595189410200533 ) ) ;
#76556=CARTESIAN_POINT ( 'NONE',  ( 109.5136938427377373, -46.88609643433851915, 132.7641967044819751 ) ) ;
#76558=CARTESIAN_POINT ( 'NONE',  ( 114.7552509866192452, -44.63809267644818135, 118.2022919425779719 ) ) ;
#76559=DIRECTION ( 'NONE',  ( 0.000000000000000000, 1.000000000000000000, 0.000000000000000000 ) ) ;
#76560=CARTESIAN_POINT ( 'NONE',  ( 52.65249034007746332, -49.32844715994061602, 180.4678068554151196 ) ) ;
#76561=CARTESIAN_POINT ( 'NONE',  ( 117.4742555207853059, -36.12881027634428222, 224.8727681330539667 ) ) ;
#76562=DIRECTION ( 'NONE',  ( -0.7071067811567173234, 0.7071067812163779331, 0.000000000000000000 ) ) ;
#76566=ORIENTED_EDGE ( 'NONE', *, *, #6590, .F. ) ;
#76568=EDGE_LOOP ( 'NONE', ( #84749, #7605, #74244, #85716 ) ) ;
#76571=VECTOR ( 'NONE', #41780, 1000.000000000000000 ) ;
#76572=CARTESIAN_POINT ( 'NONE',  ( 97.39130545576651343, -39.27856786311136261, 137.5314412799998536 ) ) ;
#76574=EDGE_LOOP ( 'NONE', ( #56509, #82269 ) ) ;
#76575=CARTESIAN_POINT ( 'NONE',  ( 99.05404782812107101, -43.39937282746017644, 116.8784824187679732 ) ) ;
#76577=CARTESIAN_POINT ( 'NONE',  ( 138.8167039024479834, -67.87844715994100397, 33.40080685541480676 ) ) ;
#76579=FACE_BOUND ( 'NONE', #26360, .T. ) ;
#76580=DIRECTION ( 'NONE',  ( -0.9825752044165969590, -0.1858654558159821002, 0.000000000000000000 ) ) ;
#76581=CARTESIAN_POINT ( 'NONE',  ( 104.1918496689535090, -26.69446299336411599, 221.2984824187679465 ) ) ;
#76583=LINE ( 'NONE', #273, #58363 ) ;
#76584=ADVANCED_FACE ( 'NONE', ( #63938 ), #34425, .T. ) ;
#76588=CARTESIAN_POINT ( 'NONE',  ( 107.0664832912750057, -36.72944715993903486, 0.7256252759109708128 ) ) ;
#76589=DIRECTION ( 'NONE',  ( -0.9834602067153815907, -0.1811243269341220596, 0.000000000000000000 ) ) ;
#76590=CARTESIAN_POINT ( 'NONE',  ( 104.5776654613874683, -26.56013282928604724, 285.2670538473396391 ) ) ;
#76593=CARTESIAN_POINT ( 'NONE',  ( 97.72652769937234041, -42.68433437468970482, 141.7661014663869707 ) ) ;
#76594=CARTESIAN_POINT ( 'NONE',  ( 99.98074987894446508, -44.37633341885192095, 42.98133956162492098 ) ) ;
#76595=CARTESIAN_POINT ( 'NONE',  ( 102.6652156630552355, -27.23093027504711117, 176.4213395616249898 ) ) ;
#76596=AXIS2_PLACEMENT_3D ( 'NONE', #29538, #23200, #35896 ) ;
#76597=DIRECTION ( 'NONE',  ( -2.900000000000000265E-14, 2.000000000000000155E-15, -1.000000000000000000 ) ) ;
#76598=CARTESIAN_POINT ( 'NONE',  ( 97.75828880830677292, -40.38464125964823381, 102.6242338216369774 ) ) ;
#76599=CARTESIAN_POINT ( 'NONE',  ( 182.0667039024469886, -33.35206098992630075, 342.9256252759119548 ) ) ;
#76601=DIRECTION ( 'NONE',  ( -1.000000000000000078E-15, 1.000000000000000083E-30, 1.000000000000000000 ) ) ;
#76604=DIRECTION ( 'NONE',  ( 0.000000000000000000, 0.000000000000000000, -1.000000000000000000 ) ) ;
#76606=CIRCLE ( 'NONE', #37431, 1.000000000000000888 ) ;
#76610=ORIENTED_EDGE ( 'NONE', *, *, #60747, .T. ) ;
#76611=CARTESIAN_POINT ( 'NONE',  ( 96.36089708107968477, -41.75325360632972149, 57.67562527591096710 ) ) ;
#76614=CYLINDRICAL_SURFACE ( 'NONE', #12272, 9.999999999999998224 ) ;
#76615=CARTESIAN_POINT ( 'NONE',  ( 101.9507351169249887, -46.57965624409947480, 163.1832443235299763 ) ) ;
#76616=VECTOR ( 'NONE', #53920, 1000.000000000000000 ) ;
#76618=CARTESIAN_POINT ( 'NONE',  ( 116.3037889147421424, -33.73884459347697629, 283.4981341137910249 ) ) ;
#76619=VERTEX_POINT ( 'NONE', #65274 ) ;
#76621=ORIENTED_EDGE ( 'NONE', *, *, #57003, .F. ) ;
#76622=DIRECTION ( 'NONE',  ( 2.900000000000000265E-14, -2.000000000000000155E-15, 1.000000000000000000 ) ) ;
#76623=DIRECTION ( 'NONE',  ( 1.000000000000000078E-15, -1.000000000000000083E-30, -1.000000000000000000 ) ) ;
#76624=CARTESIAN_POINT ( 'NONE',  ( 156.5667039024483529, -48.82844715993569196, 295.7178068554149490 ) ) ;
#76625=CARTESIAN_POINT ( 'NONE',  ( 98.35015076301363024, -31.65606670507391840, 20.90547850657702611 ) ) ;
#76630=CARTESIAN_POINT ( 'NONE',  ( 87.06648329127403940, -56.72944715994104570, -5.074374724089050659 ) ) ;
#76631=CARTESIAN_POINT ( 'NONE',  ( 99.77739493559400330, -44.20163642594134501, 21.96133956162593748 ) ) ;
#76632=CARTESIAN_POINT ( 'NONE',  ( 29.56648329127298069, -71.37844715994266664, 361.9756252759109998 ) ) ;
#76634=CARTESIAN_POINT ( 'NONE',  ( 181.8764988495240118, -33.54226604284930602, -5.074374724088000832 ) ) ;
#76636=LINE ( 'NONE', #43433, #26449 ) ;
#76637=CARTESIAN_POINT ( 'NONE',  ( 107.2657893863845260, -28.07721033202879113, 72.86428084578200526 ) ) ;
#76639=DIRECTION ( 'NONE',  ( 1.000000000000000078E-15, 0.000000000000000000, 1.000000000000000000 ) ) ;
#76640=PLANE ( 'NONE',  #58997 ) ;
#76641=ORIENTED_EDGE ( 'NONE', *, *, #35434, .F. ) ;
#76642=ORIENTED_EDGE ( 'NONE', *, *, #38096, .T. ) ;
#76643=DIRECTION ( 'NONE',  ( 1.000000000000000078E-15, 0.000000000000000000, 1.000000000000000000 ) ) ;
#76645=ORIENTED_EDGE ( 'NONE', *, *, #51403, .F. ) ;
#76647=CARTESIAN_POINT ( 'NONE',  ( 115.0372575196810061, -42.90846254905609669, 69.30229194431436213 ) ) ;
#76648=CARTESIAN_POINT ( 'NONE',  ( 108.0961452412413166, -46.06846630830715128, 154.0834880678019374 ) ) ;
#76651=CARTESIAN_POINT ( 'NONE',  ( 116.6182342972125809, -29.67350615900649657, 105.3327681330539463 ) ) ;
#76658=ORIENTED_EDGE ( 'NONE', *, *, #25364, .T. ) ;
#76659=EDGE_CURVE ( 'NONE', #18961, #43071, #9416, .T. ) ;
#76662=ORIENTED_EDGE ( 'NONE', *, *, #57972, .F. ) ;
#76663=ADVANCED_FACE ( 'NONE', ( #72972 ), #85296, .T. ) ;
#76664=CARTESIAN_POINT ( 'NONE',  ( 113.3428377330624954, -29.55695056567750711, 289.5032443235305664 ) ) ;
#76665=CARTESIAN_POINT ( 'NONE',  ( 98.41694670496758590, -29.81058001376278099, 191.7775300378159784 ) ) ;
#76666=DIRECTION ( 'NONE',  ( -4.299999999999999979E-14, 1.000000000000000000, -4.400000000000000367E-29 ) ) ;
#76668=EDGE_CURVE ( 'NONE', #14129, #73307, #37128, .T. ) ;
#76669=CARTESIAN_POINT ( 'NONE',  ( 96.64197643737422538, -36.61924597882073584, 107.3184824187679567 ) ) ;
#76670=CARTESIAN_POINT ( 'NONE',  ( 116.7951252736160086, -39.38782978119709810, 263.6147919432945059 ) ) ;
#76673=CARTESIAN_POINT ( 'NONE',  ( 97.33763774114136424, -34.07177809286157810, 116.1163881612916384 ) ) ;
#76677=ORIENTED_EDGE ( 'NONE', *, *, #39846, .T. ) ;
#76679=CARTESIAN_POINT ( 'NONE',  ( 89.33314995793998037, 12.92155284005730387, 358.9756252759109998 ) ) ;
#76680=CARTESIAN_POINT ( 'NONE',  ( 102.7552189479022928, -25.69072042043729098, 20.37276813305294354 ) ) ;
#76682=CARTESIAN_POINT ( 'NONE',  ( 141.0664832912739826, -8.729447159940995959, 14.67562527591100441 ) ) ;
#76683=CARTESIAN_POINT ( 'NONE',  ( 45.76696975232854925, -48.62818131006066835, 300.4678068554150059 ) ) ;
#76684=CARTESIAN_POINT ( 'NONE',  ( 111.1466539572802787, -45.61852150023370456, 27.91848241876893155 ) ) ;
#76685=CARTESIAN_POINT ( 'NONE',  ( 97.78504508517835347, -40.45176323166522536, 111.6299858404451300 ) ) ;
#76686=CARTESIAN_POINT ( 'NONE',  ( 98.47671751366520709, -30.86049585540216711, 116.8499109901969604 ) ) ;
#76688=DIRECTION ( 'NONE',  ( -4.299999999999999979E-14, 1.000000000000000000, -4.400000000000000367E-29 ) ) ;
#76690=ORIENTED_EDGE ( 'NONE', *, *, #52841, .T. ) ;
#76691=LINE ( 'NONE', #43036, #33772 ) ;
#76694=DIRECTION ( 'NONE',  ( 0.9068632946707805287, -0.4214249218767880389, 9.068632946707802473E-16 ) ) ;
#76695=ORIENTED_EDGE ( 'NONE', *, *, #56459, .F. ) ;
#76697=CARTESIAN_POINT ( 'NONE',  ( 102.0297551351921044, -46.62107256275958633, 172.2137205140059564 ) ) ;
#76698=ORIENTED_EDGE ( 'NONE', *, *, #74885, .T. ) ;
#76699=CYLINDRICAL_SURFACE ( 'NONE', #5986, 2.030000000002086580 ) ;
#76700=CARTESIAN_POINT ( 'NONE',  ( 117.7987307161850907, -31.64603138916173464, 210.1784824187679703 ) ) ;
#76701=CARTESIAN_POINT ( 'NONE',  ( 110.4707641138770668, -47.29393344369797347, 53.83657765686300678 ) ) ;
#76704=VECTOR ( 'NONE', #45315, 1000.000000000000000 ) ;
#76706=VERTEX_POINT ( 'NONE', #3054 ) ;
#76707=ORIENTED_EDGE ( 'NONE', *, *, #76874, .F. ) ;
#76710=FACE_OUTER_BOUND ( 'NONE', #35715, .T. ) ;
#76711=CARTESIAN_POINT ( 'NONE',  ( 116.5266666817545627, -41.19333145446972821, 224.4756252759109714 ) ) ;
#76715=FACE_OUTER_BOUND ( 'NONE', #21145, .T. ) ;
#76716=CARTESIAN_POINT ( 'NONE',  ( 41.56648329127398966, -27.57844715994070484, 135.9256252759119832 ) ) ;
#76717=DIRECTION ( 'NONE',  ( 0.000000000000000000, 0.000000000000000000, 1.000000000000000000 ) ) ;
#76718=EDGE_CURVE ( 'NONE', #68380, #47694, #22076, .T. ) ;
#76719=CARTESIAN_POINT ( 'NONE',  ( 106.5169308145888607, -25.66629059357601506, 45.12800622829193742 ) ) ;
#76720=VERTEX_POINT ( 'NONE', #3488 ) ;
#76721=VECTOR ( 'NONE', #82320, 1000.000000000000000 ) ;
#76723=EDGE_LOOP ( 'NONE', ( #79911, #26121, #45629, #5775 ) ) ;
#76726=CARTESIAN_POINT ( 'NONE',  ( 116.2779988688839552, -41.49250982992358416, 239.4346728949579699 ) ) ;
#76727=CARTESIAN_POINT ( 'NONE',  ( 182.4202572930400095, -33.70561438051981185, -5.074374724088000832 ) ) ;
#76729=CARTESIAN_POINT ( 'NONE',  ( 116.7343647603065619, -32.97833357388816466, 90.10895860924395606 ) ) ;
#76730=DIRECTION ( 'NONE',  ( 0.000000000000000000, 0.000000000000000000, -1.000000000000000000 ) ) ;
#76733=ORIENTED_EDGE ( 'NONE', *, *, #89297, .F. ) ;
#76734=CARTESIAN_POINT ( 'NONE',  ( 172.5664832912740110, -18.82844715994099971, 141.0426252759120018 ) ) ;
#76736=EDGE_LOOP ( 'NONE', ( #3939, #45307 ) ) ;
#76738=CARTESIAN_POINT ( 'NONE',  ( 114.4699299399979395, -31.85941057575024971, 250.7215833058968997 ) ) ;
#76741=CARTESIAN_POINT ( 'NONE',  ( 99.09558145272080765, -30.55060196207903900, 140.8023086913604232 ) ) ;
#76742=DIRECTION ( 'NONE',  ( -1.000000000000000078E-15, 0.000000000000000000, -1.000000000000000000 ) ) ;
#76748=CARTESIAN_POINT ( 'NONE',  ( 95.25894796463062164, -35.71821259427313322, 36.25848241876794731 ) ) ;
#76750=CARTESIAN_POINT ( 'NONE',  ( 99.16797791762762415, -38.78938375721887155, 274.3480903695913184 ) ) ;
#76751=CARTESIAN_POINT ( 'NONE',  ( 97.81168895331838087, -40.51742574516882200, 287.6356252759109680 ) ) ;
#76752=CARTESIAN_POINT ( 'NONE',  ( 114.4888877093246293, -29.48743791597849651, 194.4537205140069318 ) ) ;
#76753=LINE ( 'NONE', #55829, #14298 ) ;
#76757=VECTOR ( 'NONE', #21564, 1000.000000000000000 ) ;
#76758=CARTESIAN_POINT ( 'NONE',  ( 105.3167593786310903, -26.43023667424511913, 11.20991099019697046 ) ) ;
#76759=LINE ( 'NONE', #34964, #45631 ) ;
#76760=ORIENTED_EDGE ( 'NONE', *, *, #62995, .T. ) ;
#76761=CARTESIAN_POINT ( 'NONE',  ( 147.9173672921288869, -72.54391775211570348, 542.9756252759101471 ) ) ;
#76763=CARTESIAN_POINT ( 'NONE',  ( 116.9629591039797845, -33.20839883953882321, 110.0984824187679578 ) ) ;
#76765=ORIENTED_EDGE ( 'NONE', *, *, #15989, .F. ) ;
#76768=ORIENTED_EDGE ( 'NONE', *, *, #79758, .F. ) ;
#76769=CARTESIAN_POINT ( 'NONE',  ( 62.03742497533659872, -23.42844715994045401, 117.4678068554150485 ) ) ;
#76772=DIRECTION ( 'NONE',  ( -0.7071067811865475727, 0.000000000000000000, -0.7071067811865475727 ) ) ;
#76774=EDGE_CURVE ( 'NONE', #52430, #7253, #52056, .T. ) ;
#76775=CARTESIAN_POINT ( 'NONE',  ( 108.9290709455192570, -28.27771998284391231, 177.7099951314959583 ) ) ;
#76776=CARTESIAN_POINT ( 'NONE',  ( 97.59563580048326514, -41.13856347273024738, 252.6727681330536655 ) ) ;
#76777=CARTESIAN_POINT ( 'NONE',  ( 188.5667039024479834, -65.37844715994100397, 288.3428068554150059 ) ) ;
#76778=ORIENTED_EDGE ( 'NONE', *, *, #74021, .F. ) ;
#76781=DIRECTION ( 'NONE',  ( 0.000000000000000000, 0.000000000000000000, -1.000000000000000000 ) ) ;
#76782=VERTEX_POINT ( 'NONE', #29420 ) ;
#76787=CARTESIAN_POINT ( 'NONE',  ( 162.9033555647770015, -33.89581943344391135, -5.074374724088000832 ) ) ;
#76790=CARTESIAN_POINT ( 'NONE',  ( 149.4430470701762772, -12.91565541735124256, 394.9756252759100903 ) ) ;
#76791=CARTESIAN_POINT ( 'NONE',  ( 107.9802517323619355, -45.22186489331556203, 202.0838483995049728 ) ) ;
#76792=CARTESIAN_POINT ( 'NONE',  ( 103.3467460430879612, -47.18776626161088927, 102.3165776568629752 ) ) ;
#76794=CARTESIAN_POINT ( 'NONE',  ( 131.4622572338305986, -19.61690131752980903, 6.952852217890792552 ) ) ;
#76795=ADVANCED_FACE ( 'NONE', ( #50283 ), #11937, .F. ) ;
#76799=CARTESIAN_POINT ( 'NONE',  ( 130.0664832912740110, -18.82844715994099971, 199.5838068554170093 ) ) ;
#76801=CARTESIAN_POINT ( 'NONE',  ( 99.09532346176355588, -30.55094594719723133, 261.8023343508735366 ) ) ;
#76802=ORIENTED_EDGE ( 'NONE', *, *, #13308, .F. ) ;
#76805=FACE_BOUND ( 'NONE', #69973, .T. ) ;
#76806=CARTESIAN_POINT ( 'NONE',  ( 73.06648329127358465, -8.729447159940534107, -4.970821333494978234 ) ) ;
#76808=ORIENTED_EDGE ( 'NONE', *, *, #81057, .F. ) ;
#76809=CARTESIAN_POINT ( 'NONE',  ( 96.90545716317438973, -39.15842060370329847, 56.51276813305394597 ) ) ;
#76815=ORIENTED_EDGE ( 'NONE', *, *, #20878, .F. ) ;
#76816=VECTOR ( 'NONE', #32987, 1000.000000000000000 ) ;
#76817=LINE ( 'NONE', #43172, #63432 ) ;
#76819=DIRECTION ( 'NONE',  ( 0.9999999853157766072, 0.0001713722456127291416, -9.999999853157765648E-16 ) ) ;
#76821=CARTESIAN_POINT ( 'NONE',  ( 99.03746950336261534, -43.41317339962571253, 112.8784824187679732 ) ) ;
#76822=LINE ( 'NONE', #69563, #11680 ) ;
#76824=DIRECTION ( 'NONE',  ( -4.237773401492740281E-14, 1.000000000000000000, 0.000000000000000000 ) ) ;
#76825=AXIS2_PLACEMENT_3D ( 'NONE', #26466, #60518, #25562 ) ;
#76826=VERTEX_POINT ( 'NONE', #39781 ) ;
#76828=CARTESIAN_POINT ( 'NONE',  ( 97.31342953368671544, -35.99458159538090030, 142.2670538473389570 ) ) ;
#76829=CYLINDRICAL_SURFACE ( 'NONE', #2197, 9.999999999999998224 ) ;
#76831=AXIS2_PLACEMENT_3D ( 'NONE', #74165, #6035, #47331 ) ;
#76832=CARTESIAN_POINT ( 'NONE',  ( 100.1919508713739759, -45.35525880799009713, 268.0289586092443415 ) ) ;
#76834=FACE_OUTER_BOUND ( 'NONE', #82917, .T. ) ;
#76835=CARTESIAN_POINT ( 'NONE',  ( 82.81648064515530905, -18.72944715939135207, 6.749772901088279653 ) ) ;
#76837=CIRCLE ( 'NONE', #88457, 11.57110091390439699 ) ;
#76839=FACE_OUTER_BOUND ( 'NONE', #49528, .T. ) ;
#76840=CARTESIAN_POINT ( 'NONE',  ( 115.7764676695378512, -43.63945112744040955, 198.2927681330539542 ) ) ;
#76842=VERTEX_POINT ( 'NONE', #53392 ) ;
#76844=CARTESIAN_POINT ( 'NONE',  ( 117.1402439185659006, -36.89830975172036887, 150.2444404487539487 ) ) ;
#76846=DIRECTION ( 'NONE',  ( -2.900000000000000265E-14, 2.000000000000000155E-15, -1.000000000000000000 ) ) ;
#76847=EDGE_CURVE ( 'NONE', #53694, #29605, #32978, .T. ) ;
#76848=CARTESIAN_POINT ( 'NONE',  ( 116.8725690376871569, -36.55701438716827312, 284.8413395616245793 ) ) ;
#76849=CARTESIAN_POINT ( 'NONE',  ( 37.36643805256671413, -48.62818131006081046, 300.4678068554150059 ) ) ;
#76850=EDGE_CURVE ( 'NONE', #73636, #59995, #59336, .T. ) ;
#76851=CARTESIAN_POINT ( 'NONE',  ( 117.0720588755466025, -35.46383719571640825, 268.9274440218657105 ) ) ;
#76852=CIRCLE ( 'NONE', #30444, 2.117000000000007987 ) ;
#76855=CYLINDRICAL_SURFACE ( 'NONE', #82676, 7.499999999999996447 ) ;
#76856=CARTESIAN_POINT ( 'NONE',  ( 90.44969454456408187, -53.34645651782490461, 239.5838068554174356 ) ) ;
#76858=CARTESIAN_POINT ( 'NONE',  ( 97.07914014679025172, -41.41098531455293141, 211.6632443235299945 ) ) ;
#76859=DIRECTION ( 'NONE',  ( 1.000000000000000000, 4.163336342344333240E-14, 0.000000000000000000 ) ) ;
#76860=ORIENTED_EDGE ( 'NONE', *, *, #68466, .F. ) ;
#76861=ORIENTED_EDGE ( 'NONE', *, *, #62829, .T. ) ;
#76862=EDGE_CURVE ( 'NONE', #50856, #2257, #3259, .T. ) ;
#76866=AXIS2_PLACEMENT_3D ( 'NONE', #69292, #61556, #89293 ) ;
#76867=DIRECTION ( 'NONE',  ( 0.000000000000000000, 0.000000000000000000, 1.000000000000000000 ) ) ;
#76870=CARTESIAN_POINT ( 'NONE',  ( 165.6738106836199904, -26.00627455219321860, -5.074374724088000832 ) ) ;
#76871=EDGE_CURVE ( 'NONE', #17132, #19112, #81160, .T. ) ;
#76874=EDGE_CURVE ( 'NONE', #48829, #38962, #55417, .T. ) ;
#76875=CARTESIAN_POINT ( 'NONE',  ( 118.0818320075808856, -32.35879749485835788, 249.1270538473389706 ) ) ;
#76877=CIRCLE ( 'NONE', #7242, 2.517500000000005844 ) ;
#76878=CARTESIAN_POINT ( 'NONE',  ( 176.7669697523282935, -48.62818131005432321, 300.4678068554149490 ) ) ;
#76879=CARTESIAN_POINT ( 'NONE',  ( 29.56670390244828184, -48.82844715994152551, 300.4678068554150059 ) ) ;
#76880=DIRECTION ( 'NONE',  ( 0.000000000000000000, 0.000000000000000000, -1.000000000000000000 ) ) ;
#76881=ADVANCED_FACE ( 'NONE', ( #4834 ), #80258, .T. ) ;
#76882=CARTESIAN_POINT ( 'NONE',  ( 115.5682441604615178, -40.44643428488449644, 56.31666179816296847 ) ) ;
#76883=CARTESIAN_POINT ( 'NONE',  ( 102.8351866564443924, -46.28106417705388509, 173.2441967044829596 ) ) ;
#76885=ORIENTED_EDGE ( 'NONE', *, *, #89380, .F. ) ;
#76886=FACE_BOUND ( 'NONE', #87694, .T. ) ;
#76887=VECTOR ( 'NONE', #38196, 1000.000000000000000 ) ;
#76889=EDGE_LOOP ( 'NONE', ( #26845, #67631, #73875, #52720 ) ) ;
#76891=ORIENTED_EDGE ( 'NONE', *, *, #59421, .F. ) ;
#76892=ORIENTED_EDGE ( 'NONE', *, *, #30816, .F. ) ;
#76894=LINE ( 'NONE', #12093, #73594 ) ;
#76895=CARTESIAN_POINT ( 'NONE',  ( 98.06318007301436523, -37.70576754076741821, 80.82289601855296723 ) ) ;
#76896=CARTESIAN_POINT ( 'NONE',  ( 96.75420216176078725, -40.77324476150559462, 246.6118157521009664 ) ) ;
#76897=EDGE_CURVE ( 'NONE', #84365, #17889, #18906, .T. ) ;
#76898=CARTESIAN_POINT ( 'NONE',  ( 117.2062538965840304, -41.07097622818930915, 213.5165776568629781 ) ) ;
#76900=DIRECTION ( 'NONE',  ( 0.7071067811865491270, -0.7071067811865459074, 7.071067811865492096E-16 ) ) ;
#76904=DIRECTION ( 'NONE',  ( 0.7071067811571405404, 0.7071067812159546051, 0.000000000000000000 ) ) ;
#76905=EDGE_CURVE ( 'NONE', #86581, #29066, #74328, .T. ) ;
#76908=AXIS2_PLACEMENT_3D ( 'NONE', #3290, #44594, #50526 ) ;
#76909=CARTESIAN_POINT ( 'NONE',  ( 114.2951562036313646, -44.16484043540982185, 118.2022919425779719 ) ) ;
#76910=CARTESIAN_POINT ( 'NONE',  ( 97.24697957573494023, -33.09846756419045022, 66.04419670448297097 ) ) ;
#76911=CARTESIAN_POINT ( 'NONE',  ( 105.7708979221677197, -26.34060099707374292, 270.1756252759109884 ) ) ;
#76912=ORIENTED_EDGE ( 'NONE', *, *, #26557, .T. ) ;
#76913=CARTESIAN_POINT ( 'NONE',  ( 114.6056301357651819, -29.52887111919123697, 234.4327681330539690 ) ) ;
#76914=CARTESIAN_POINT ( 'NONE',  ( 107.0664832912739399, -48.47944715994096043, 307.1356252759109680 ) ) ;
#76916=CARTESIAN_POINT ( 'NONE',  ( 116.3244028009478797, -32.94573790848593120, 95.13562527591096796 ) ) ;
#76917=CARTESIAN_POINT ( 'NONE',  ( 62.03715912545739286, -47.82818131006020934, 180.4678068554151196 ) ) ;
#76918=CARTESIAN_POINT ( 'NONE',  ( 126.0667039024479266, -14.72944715994094977, 239.5838068554170377 ) ) ;
#76926=CARTESIAN_POINT ( 'NONE',  ( 98.34985888773255169, -31.65658485141074152, 11.90645861297915076 ) ) ;
#76927=DIRECTION ( 'NONE',  ( 0.000000000000000000, 0.000000000000000000, 1.000000000000000000 ) ) ;
#76928=CARTESIAN_POINT ( 'NONE',  ( 116.3135889066590636, -32.94480564983713577, 259.1356252759109680 ) ) ;
#76931=CARTESIAN_POINT ( 'NONE',  ( 101.2817000042767148, -26.35783695576231267, 255.4813395616251626 ) ) ;
#76932=CARTESIAN_POINT ( 'NONE',  ( 113.0769238478409449, -28.21140209294909695, 125.5870538473399591 ) ) ;
#76933=CARTESIAN_POINT ( 'NONE',  ( 104.7308122791112908, -47.55672043936114335, 28.41943479971997988 ) ) ;
#76934=VECTOR ( 'NONE', #18136, 1000.000000000000000 ) ;
#76935=DIRECTION ( 'NONE',  ( 0.000000000000000000, -1.000000000000000000, 0.000000000000000000 ) ) ;
#76936=CARTESIAN_POINT ( 'NONE',  ( 113.7762091862918226, -33.98316268565083220, -2.114374724089040924 ) ) ;
#76937=CARTESIAN_POINT ( 'NONE',  ( 82.79786375350262517, -36.40984252624630102, 6.777538624683718815 ) ) ;
#76939=VERTEX_POINT ( 'NONE', #18004 ) ;
#76940=CARTESIAN_POINT ( 'NONE',  ( 124.7998166246059810, 12.92155284005730387, 361.9756252759109998 ) ) ;
#76943=CARTESIAN_POINT ( 'NONE',  ( 99.77605516222793369, -32.27907757783855658, 170.3124198280769974 ) ) ;
#76946=LINE ( 'NONE', #7454, #37361 ) ;
#76947=CARTESIAN_POINT ( 'NONE',  ( 117.4654710391979222, -40.40706546494229201, 174.5680062282919778 ) ) ;
#76949=CARTESIAN_POINT ( 'NONE',  ( 99.09591451443299093, -30.55015794387348649, 150.8027366674846235 ) ) ;
#76950=DIRECTION ( 'NONE',  ( 0.000000000000000000, 1.000000000000000000, 0.000000000000000000 ) ) ;
#76953=CARTESIAN_POINT ( 'NONE',  ( 113.4367438382844284, -44.15125393826594546, 108.1413395616259692 ) ) ;
#76954=VERTEX_POINT ( 'NONE', #87064 ) ;
#76957=VERTEX_POINT ( 'NONE', #11189 ) ;
#76958=CARTESIAN_POINT ( 'NONE',  ( 111.1996377132626748, -28.89074107182586815, 56.12158330589694799 ) ) ;
#76959=CARTESIAN_POINT ( 'NONE',  ( 45.76696975232782449, -48.62818131005837330, 249.9678068554150343 ) ) ;
#76960=CARTESIAN_POINT ( 'NONE',  ( 101.7740290765682829, -45.64733444449320388, 203.1622919425769567 ) ) ;
#76964=CARTESIAN_POINT ( 'NONE',  ( 188.5667039024479834, -48.82844715994099971, 137.2178068554150059 ) ) ;
#76965=ADVANCED_FACE ( 'NONE', ( #47933 ), #48374, .F. ) ;
#76967=EDGE_CURVE ( 'NONE', #34717, #28582, #88790, .T. ) ;
#76970=CARTESIAN_POINT ( 'NONE',  ( 95.69905522618344662, -33.46911247776736786, 141.1041967044829732 ) ) ;
#76972=ORIENTED_EDGE ( 'NONE', *, *, #80664, .F. ) ;
#76973=VERTEX_POINT ( 'NONE', #70195 ) ;
#76974=AXIS2_PLACEMENT_3D ( 'NONE', #77275, #1870, #35925 ) ;
#76975=EDGE_CURVE ( 'NONE', #48113, #10930, #76108, .T. ) ;
#76976=EDGE_CURVE ( 'NONE', #4752, #82826, #56090, .T. ) ;
#76979=CARTESIAN_POINT ( 'NONE',  ( 116.3254862984629909, -32.93730789470958342, 129.1356252759109680 ) ) ;
#76980=DIRECTION ( 'NONE',  ( -0.7071067811865774377, 0.7071067811865175967, -7.071067811865782003E-16 ) ) ;
#76981=CARTESIAN_POINT ( 'NONE',  ( 107.5268921225462719, -45.37172398690709230, 195.4490427505439811 ) ) ;
#76983=EDGE_CURVE ( 'NONE', #30351, #5575, #14799, .T. ) ;
#76984=FACE_OUTER_BOUND ( 'NONE', #6777, .T. ) ;
#76986=CARTESIAN_POINT ( 'NONE',  ( 97.81193178031652735, -40.51732023384165160, 27.63604381180012837 ) ) ;
#76991=CARTESIAN_POINT ( 'NONE',  ( 150.5667039024473866, -25.42844715993594562, 249.9678068554149490 ) ) ;
#76993=VERTEX_POINT ( 'NONE', #37464 ) ;
#76994=LINE ( 'NONE', #36099, #79713 ) ;
#76996=CARTESIAN_POINT ( 'NONE',  ( 111.6101215911791087, -44.95330735676063938, 249.3977737820869720 ) ) ;
#76997=CARTESIAN_POINT ( 'NONE',  ( 97.06105994701182738, -37.99635423742223850, 182.4277913507199003 ) ) ;
#76999=DIRECTION ( 'NONE',  ( 6.831565154159360295E-14, -1.000000000000000000, 0.000000000000000000 ) ) ;
#77004=FACE_OUTER_BOUND ( 'NONE', #2202, .T. ) ;
#77006=VERTEX_POINT ( 'NONE', #15239 ) ;
#77007=AXIS2_PLACEMENT_3D ( 'NONE', #82823, #48252, #75985 ) ;
#77008=CARTESIAN_POINT ( 'NONE',  ( 110.8229109585819003, -44.00762958608321895, 270.7738046553057529 ) ) ;
#77009=CARTESIAN_POINT ( 'NONE',  ( 108.5930441862165026, -47.10046404026961397, 142.6927681330539883 ) ) ;
#77010=AXIS2_PLACEMENT_3D ( 'NONE', #73226, #31896, #66413 ) ;
#77011=CARTESIAN_POINT ( 'NONE',  ( 117.3173117416417739, -32.65705981835808558, 99.13943479972098771 ) ) ;
#77013=( NAMED_UNIT ( * ) SI_UNIT ( $, .STERADIAN. ) SOLID_ANGLE_UNIT ( ) );
#77014=CARTESIAN_POINT ( 'NONE',  ( 100.6376613383881704, -26.77430457650146423, 216.5327681330539633 ) ) ;
#77016=VECTOR ( 'NONE', #3520, 1000.000000000000000 ) ;
#77018=ORIENTED_EDGE ( 'NONE', *, *, #1095, .F. ) ;
#77019=CARTESIAN_POINT ( 'NONE',  ( 116.3212776292296127, -32.94146857471318413, 287.6356252759109680 ) ) ;
#77021=EDGE_CURVE ( 'NONE', #71887, #40190, #80155, .T. ) ;
#77022=ORIENTED_EDGE ( 'NONE', *, *, #49924, .F. ) ;
#77023=DIRECTION ( 'NONE',  ( 0.000000000000000000, 0.000000000000000000, 1.000000000000000000 ) ) ;
#77025=AXIS2_PLACEMENT_3D ( 'NONE', #53184, #32776, #53636 ) ;
#77026=CARTESIAN_POINT ( 'NONE',  ( 97.33776833833610453, -34.07136034921212797, 137.1147412179166736 ) ) ;
#77027=CIRCLE ( 'NONE', #52333, 2.116999999999993776 ) ;
#77029=CARTESIAN_POINT ( 'NONE',  ( 114.1752211786757414, -45.19379553418442441, 148.1203871806719405 ) ) ;
#77030=DIRECTION ( 'NONE',  ( 1.000000000000000078E-15, 1.000000000000000083E-30, -1.000000000000000000 ) ) ;
#77032=CARTESIAN_POINT ( 'NONE',  ( 80.06648329127399677, -15.97944715994105813, 1.625625275910943746 ) ) ;
#77035=CARTESIAN_POINT ( 'NONE',  ( 115.8883252675856994, -30.10835006627626953, 260.3508633711493871 ) ) ;
#77039=FACE_OUTER_BOUND ( 'NONE', #46110, .T. ) ;
#77040=CARTESIAN_POINT ( 'NONE',  ( 109.6430121502607733, -46.48008672978578204, 258.7814586108584081 ) ) ;
#77042=AXIS2_PLACEMENT_3D ( 'NONE', #24875, #45729, #60268 ) ;
#77043=CARTESIAN_POINT ( 'NONE',  ( 112.8265051076421770, -28.69573459919405067, 195.5838068554226368 ) ) ;
#77044=ORIENTED_EDGE ( 'NONE', *, *, #50630, .F. ) ;
#77045=CARTESIAN_POINT ( 'NONE',  ( 51.56670390244699576, -19.82844715994031048, -5.074374724088000832 ) ) ;
#77046=CARTESIAN_POINT ( 'NONE',  ( 97.93707779058323126, -30.45653744243544736, 165.8594347997199634 ) ) ;
#77047=CARTESIAN_POINT ( 'NONE',  ( 111.4154404335798745, -46.20410067450679037, 23.91848241876792969 ) ) ;
#77048=CARTESIAN_POINT ( 'NONE',  ( 110.7114656039092893, -48.05751922203765503, 203.8241967044819489 ) ) ;
#77053=DIRECTION ( 'NONE',  ( 0.000000000000000000, 0.000000000000000000, -1.000000000000000000 ) ) ;
#77055=ORIENTED_EDGE ( 'NONE', *, *, #20921, .F. ) ;
#77057=EDGE_CURVE ( 'NONE', #4931, #55131, #63839, .T. ) ;
#77058=FACE_BOUND ( 'NONE', #85362, .T. ) ;
#77061=VECTOR ( 'NONE', #89411, 1000.000000000000114 ) ;
#77062=FACE_OUTER_BOUND ( 'NONE', #46070, .T. ) ;
#77063=VERTEX_POINT ( 'NONE', #57901 ) ;
#77064=CARTESIAN_POINT ( 'NONE',  ( 101.9712125536871383, -27.65933791914800111, 56.48419670448296159 ) ) ;
#77067=CARTESIAN_POINT ( 'NONE',  ( 48.79742451362098166, -36.32844715994040996, 237.4678068554150059 ) ) ;
#77068=CARTESIAN_POINT ( 'NONE',  ( 113.5922599384962552, -44.96062289245586641, 164.1099109901969655 ) ) ;
#77069=CARTESIAN_POINT ( 'NONE',  ( 105.4627246288800109, -27.81649992262058646, 274.6286103042674540 ) ) ;
#77070=VERTEX_POINT ( 'NONE', #22504 ) ;
#77072=ORIENTED_EDGE ( 'NONE', *, *, #20083, .F. ) ;
#77073=ORIENTED_EDGE ( 'NONE', *, *, #87977, .T. ) ;
#77075=CARTESIAN_POINT ( 'NONE',  ( 125.0664851986225443, -56.72944715994101728, -4.824374724089012467 ) ) ;
#77076=PLANE ( 'NONE',  #56479 ) ;
#77077=DIRECTION ( 'NONE',  ( 0.7071067812164788524, -0.7071067811566160710, 0.000000000000000000 ) ) ;
#77078=CARTESIAN_POINT ( 'NONE',  ( 100.9546728043249573, -28.70702573249558753, 75.59395860993166139 ) ) ;
#77080=EDGE_CURVE ( 'NONE', #37453, #14129, #9761, .T. ) ;
#77083=PLANE ( 'NONE',  #83423 ) ;
#77084=VECTOR ( 'NONE', #23234, 1000.000000000000000 ) ;
#77086=DIRECTION ( 'NONE',  ( 0.000000000000000000, -1.000000000000000000, 0.000000000000000000 ) ) ;
#77087=CARTESIAN_POINT ( 'NONE',  ( 115.4270991047691410, -42.97960947038953350, 28.31562527591097123 ) ) ;
#77089=ORIENTED_EDGE ( 'NONE', *, *, #81503, .F. ) ;
#77091=CARTESIAN_POINT ( 'NONE',  ( 188.5667039024479834, -62.87844715994099687, 173.2178068554149775 ) ) ;
#77093=CYLINDRICAL_SURFACE ( 'NONE', #58347, 0.9999999999999800160 ) ;
#77094=CARTESIAN_POINT ( 'NONE',  ( 109.2937122495728772, -44.61120707852311540, 70.61380465530497474 ) ) ;
#77095=EDGE_CURVE ( 'NONE', #7923, #50110, #45580, .T. ) ;
#77096=AXIS2_PLACEMENT_3D ( 'NONE', #49495, #85408, #36338 ) ;
#77099=FACE_OUTER_BOUND ( 'NONE', #3708, .T. ) ;
#77100=ORIENTED_EDGE ( 'NONE', *, *, #14236, .T. ) ;
#77102=DIRECTION ( 'NONE',  ( 0.000000000000000000, 0.000000000000000000, -1.000000000000000000 ) ) ;
#77104=ORIENTED_EDGE ( 'NONE', *, *, #8261, .F. ) ;
#77105=AXIS2_PLACEMENT_3D ( 'NONE', #61522, #76512, #14296 ) ;
#77106=CARTESIAN_POINT ( 'NONE',  ( 108.3613424580152724, -45.52634895430261253, 139.1244404487539725 ) ) ;
#77107=LINE ( 'NONE', #6263, #54744 ) ;
#77108=CARTESIAN_POINT ( 'NONE',  ( 101.6669702799278525, -27.05833217848093497, 101.4937205140059575 ) ) ;
#77112=ORIENTED_EDGE ( 'NONE', *, *, #43289, .T. ) ;
#77114=AXIS2_PLACEMENT_3D ( 'NONE', #1396, #57230, #35445 ) ;
#77115=DIRECTION ( 'NONE',  ( 0.000000000000000000, 0.000000000000000000, -1.000000000000000000 ) ) ;
#77117=CARTESIAN_POINT ( 'NONE',  ( 101.4562478665867928, -44.74122718545263666, 282.0899109901972110 ) ) ;
#77118=CARTESIAN_POINT ( 'NONE',  ( 117.8014899757583578, -34.00092425788908912, 165.0365776568629315 ) ) ;
#77119=CARTESIAN_POINT ( 'NONE',  ( 107.0664832912739968, -8.729447159940999512, 17.92562527591199739 ) ) ;
#77121=CARTESIAN_POINT ( 'NONE',  ( 117.1635299909640082, -34.13481127188234865, 120.0270538473389479 ) ) ;
#77124=VERTEX_POINT ( 'NONE', #53735 ) ;
#77125=DIRECTION ( 'NONE',  ( 0.7071067811868710917, -0.7071067811862240537, 0.000000000000000000 ) ) ;
#77128=EDGE_CURVE ( 'NONE', #36943, #16561, #75810, .T. ) ;
#77129=ORIENTED_EDGE ( 'NONE', *, *, #49317, .F. ) ;
#77132=CARTESIAN_POINT ( 'NONE',  ( 34.27258461953793045, -35.55794170701850732, 117.4678068554150485 ) ) ;
#77133=CARTESIAN_POINT ( 'NONE',  ( 114.0907319755898186, -46.27410096495736269, 33.08133956162495792 ) ) ;
#77137=CARTESIAN_POINT ( 'NONE',  ( 114.5003125304781122, -32.48770244606883040, 288.6609912566482308 ) ) ;
#77138=CARTESIAN_POINT ( 'NONE',  ( 97.81169822462854313, -40.51742973538109993, 111.6355314416972391 ) ) ;
#77139=CARTESIAN_POINT ( 'NONE',  ( 107.6517678568360452, -47.10594642807011923, 148.6213395616249784 ) ) ;
#77141=DIRECTION ( 'NONE',  ( 0.7071067811869279351, -0.7071067811861670993, 2.899137802863401107E-29 ) ) ;
#77142=VERTEX_POINT ( 'NONE', #59667 ) ;
#77144=VECTOR ( 'NONE', #28198, 1000.000000000000000 ) ;
#77148=LINE ( 'NONE', #11216, #5683 ) ;
#77149=CARTESIAN_POINT ( 'NONE',  ( 118.9274366748948069, -37.70237179777471681, 188.7613395616259595 ) ) ;
#77150=VERTEX_POINT ( 'NONE', #17464 ) ;
#77152=CARTESIAN_POINT ( 'NONE',  ( 96.10234264863321130, -35.15692507338371087, 222.2251490854349640 ) ) ;
#77153=CARTESIAN_POINT ( 'NONE',  ( 110.8100519147795922, -46.50588177123592715, 58.86705384733998159 ) ) ;
#77157=CARTESIAN_POINT ( 'NONE',  ( 113.1782937761293653, -44.75186858878011265, 78.09395860973531001 ) ) ;
#77158=ORIENTED_EDGE ( 'NONE', *, *, #44959, .F. ) ;
#77159=AXIS2_PLACEMENT_3D ( 'NONE', #62020, #41124, #75669 ) ;
#77160=EDGE_CURVE ( 'NONE', #62011, #41091, #86957, .T. ) ;
#77162=ORIENTED_EDGE ( 'NONE', *, *, #43007, .T. ) ;
#77166=CARTESIAN_POINT ( 'NONE',  ( 106.9404422130490815, -47.78196244520037084, 228.5794347997199907 ) ) ;
#77169=AXIS2_PLACEMENT_3D ( 'NONE', #85587, #58297, #79661 ) ;
#77170=LINE ( 'NONE', #49886, #13397 ) ;
#77172=CARTESIAN_POINT ( 'NONE',  ( 25.56670390244734747, -48.82844715994178841, 139.7178068554150627 ) ) ;
#77173=CARTESIAN_POINT ( 'NONE',  ( 101.1290945223330198, -28.09024711436062915, 50.55562527591095545 ) ) ;
#77175=VECTOR ( 'NONE', #43510, 1000.000000000000000 ) ;
#77176=VERTEX_POINT ( 'NONE', #46927 ) ;
#77177=FACE_OUTER_BOUND ( 'NONE', #14457, .T. ) ;
#77178=CARTESIAN_POINT ( 'NONE',  ( 98.35016245627538467, -31.65604021423551373, 16.90910402984798111 ) ) ;
#77179=CARTESIAN_POINT ( 'NONE',  ( 100.2051353121705546, -29.75912871662447756, 221.6956252759109702 ) ) ;
#77180=EDGE_CURVE ( 'NONE', #59590, #69306, #61023, .T. ) ;
#77181=AXIS2_PLACEMENT_3D ( 'NONE', #7645, #43935, #1283 ) ;
#77182=CYLINDRICAL_SURFACE ( 'NONE', #58830, 3.000000000000002665 ) ;
#77183=CARTESIAN_POINT ( 'NONE',  ( 114.2526777242400726, -43.36435822665418982, 119.2327681330529714 ) ) ;
#77185=CYLINDRICAL_SURFACE ( 'NONE', #18289, 9.999999999999998224 ) ;
#77186=EDGE_CURVE ( 'NONE', #52268, #78070, #45308, .T. ) ;
#77190=DIRECTION ( 'NONE',  ( -0.7071067811865794361, 0.7071067811865157093, -7.071067811865803697E-16 ) ) ;
#77191=VECTOR ( 'NONE', #87488, 1000.000000000000000 ) ;
#77196=CARTESIAN_POINT ( 'NONE',  ( 105.9698521113164844, -27.93594508925886188, 266.6072975916113705 ) ) ;
#77197=CARTESIAN_POINT ( 'NONE',  ( 116.8171228685551313, -34.15291832559168483, 194.0314586088195199 ) ) ;
#77199=CARTESIAN_POINT ( 'NONE',  ( 100.9546728245577469, -28.70702571737296793, 85.59395860794109012 ) ) ;
#77200=ADVANCED_FACE ( 'NONE', ( #5633 ), #18799, .F. ) ;
#77203=DIRECTION ( 'NONE',  ( 0.000000000000000000, 0.000000000000000000, 1.000000000000000000 ) ) ;
#77206=CARTESIAN_POINT ( 'NONE',  ( 99.06573214631099233, -44.35618096740151373, 36.92038718067297509 ) ) ;
#77208=CARTESIAN_POINT ( 'NONE',  ( 110.5540359372802328, -28.93245362646326768, 24.16384839950497110 ) ) ;
#77209=DIRECTION ( 'NONE',  ( 0.000000000000000000, 0.000000000000000000, -1.000000000000000000 ) ) ;
#77210=CARTESIAN_POINT ( 'NONE',  ( 114.4768422515204946, -30.34587328852055066, 184.3927681330539770 ) ) ;
#77213=DIRECTION ( 'NONE',  ( 0.9254794337955621897, 0.3787978585227821382, 0.000000000000000000 ) ) ;
#77215=CARTESIAN_POINT ( 'NONE',  ( 167.2371591254544967, -47.82818131005522133, 180.4678068554150059 ) ) ;
#77216=CARTESIAN_POINT ( 'NONE',  ( 118.3880299729056276, -33.06406546148816261, 280.0756252759109657 ) ) ;
#77217=CARTESIAN_POINT ( 'NONE',  ( 98.06462366603227565, -41.13538585706373851, 116.6892862011573584 ) ) ;
#77218=ORIENTED_EDGE ( 'NONE', *, *, #15228, .F. ) ;
#77220=ORIENTED_EDGE ( 'NONE', *, *, #41619, .F. ) ;
#77221=CARTESIAN_POINT ( 'NONE',  ( 108.5441076757828398, -26.36558658937538269, 100.9641967044829727 ) ) ;
#77224=ORIENTED_EDGE ( 'NONE', *, *, #63000, .T. ) ;
#77225=VERTEX_POINT ( 'NONE', #10639 ) ;
#77226=CARTESIAN_POINT ( 'NONE',  ( 108.3334479865492455, -46.73485936871515634, 122.6772919339558143 ) ) ;
#77227=CARTESIAN_POINT ( 'NONE',  ( 41.56648329127381203, -18.82844715994071194, 81.92562527591194055 ) ) ;
#77230=DIRECTION ( 'NONE',  ( 0.000000000000000000, 0.000000000000000000, 1.000000000000000000 ) ) ;
#77231=CARTESIAN_POINT ( 'NONE',  ( 114.8194029112656551, -43.69900416259703491, 34.24419670448197905 ) ) ;
#77232=AXIS2_PLACEMENT_3D ( 'NONE', #83913, #21683, #49357 ) ;
#77235=DIRECTION ( 'NONE',  ( 0.7071067811865671127, 0.7071067811865279218, 7.071067811865664660E-16 ) ) ;
#77236=CARTESIAN_POINT ( 'NONE',  ( 116.7951261054197118, -39.38782728827160895, 43.61448311080118856 ) ) ;
#77237=EDGE_CURVE ( 'NONE', #42340, #45263, #38343, .T. ) ;
#77238=ORIENTED_EDGE ( 'NONE', *, *, #73155, .T. ) ;
#77239=VERTEX_POINT ( 'NONE', #26509 ) ;
#77241=CARTESIAN_POINT ( 'NONE',  ( 82.68803181460158669, -19.56139158947832613, 2.921136715972032505 ) ) ;
#77242=CARTESIAN_POINT ( 'NONE',  ( 105.8881231706732962, -26.36991942434103819, 322.4846826458744431 ) ) ;
#77243=LINE ( 'NONE', #1838, #79189 ) ;
#77244=ADVANCED_FACE ( 'NONE', ( #79709 ), #73306, .F. ) ;
#77247=CARTESIAN_POINT ( 'NONE',  ( 99.44356389104279970, -40.64648710652873831, 196.1267055423629699 ) ) ;
#77250=CARTESIAN_POINT ( 'NONE',  ( 96.74811198265052781, -38.50085326290480481, 91.46133956162493917 ) ) ;
#77252=CARTESIAN_POINT ( 'NONE',  ( 84.06648329127399677, -18.82844715994099971, 284.9256252759119548 ) ) ;
#77254=FACE_OUTER_BOUND ( 'NONE', #45105, .T. ) ;
#77255=ORIENTED_EDGE ( 'NONE', *, *, #11939, .T. ) ;
#77257=ORIENTED_EDGE ( 'NONE', *, *, #54903, .T. ) ;
#77258=DIRECTION ( 'NONE',  ( 1.000000000000000000, 4.299999999999999979E-14, 1.000000000000000078E-15 ) ) ;
#77261=LINE ( 'NONE', #84984, #33566 ) ;
#77262=ORIENTED_EDGE ( 'NONE', *, *, #50413, .T. ) ;
#77264=CARTESIAN_POINT ( 'NONE',  ( 110.3789737648050107, -47.29935009229100729, 52.80610146638697699 ) ) ;
#77265=CARTESIAN_POINT ( 'NONE',  ( 84.06648329127399677, -18.82844715994099971, 284.9256252759119548 ) ) ;
#77267=DIRECTION ( 'NONE',  ( 1.000000000000000078E-15, -1.000000000000000083E-30, -1.000000000000000000 ) ) ;
#77268=CARTESIAN_POINT ( 'NONE',  ( 25.56670390244797275, -62.87844715994099687, 134.4678068554150059 ) ) ;
#77269=EDGE_LOOP ( 'NONE', ( #55350, #54596, #55132, #54342 ) ) ;
#77271=CARTESIAN_POINT ( 'NONE',  ( 179.8608231853567645, -35.55794170701179269, 313.9678068554149490 ) ) ;
#77272=FACE_OUTER_BOUND ( 'NONE', #22289, .T. ) ;
#77273=CARTESIAN_POINT ( 'NONE',  ( 25.56670390244731550, -42.82844715994178131, 175.7178068554150627 ) ) ;
#77274=CARTESIAN_POINT ( 'NONE',  ( 118.9284187910711665, -36.16665333732972698, 114.8641967044819694 ) ) ;
#77275=CARTESIAN_POINT ( 'NONE',  ( 41.56670390244689628, -36.32844715994109208, 180.4678068554150911 ) ) ;
#77276=FACE_BOUND ( 'NONE', #39606, .T. ) ;
#77277=CARTESIAN_POINT ( 'NONE',  ( 80.54920390244805617, -51.22944715994108833, 207.5838068554169809 ) ) ;
#77278=AXIS2_PLACEMENT_3D ( 'NONE', #71416, #9179, #36878 ) ;
#77279=ORIENTED_EDGE ( 'NONE', *, *, #84511, .F. ) ;
#77280=DIRECTION ( 'NONE',  ( 0.000000000000000000, 0.000000000000000000, 1.000000000000000000 ) ) ;
#77281=CARTESIAN_POINT ( 'NONE',  ( 109.3575602964533289, -46.23809593081413993, 128.7641967044819751 ) ) ;
#77282=EDGE_CURVE ( 'NONE', #64418, #29598, #16351, .T. ) ;
#77283=DIRECTION ( 'NONE',  ( -1.000000000000000000, -2.756263715554006823E-15, 0.000000000000000000 ) ) ;
#77285=CARTESIAN_POINT ( 'NONE',  ( 104.5933598291445605, -26.62426044571802208, 281.2670538473395823 ) ) ;
#77286=FACE_OUTER_BOUND ( 'NONE', #62504, .T. ) ;
#77287=DIRECTION ( 'NONE',  ( 1.000000000000000078E-15, -1.000000000000000083E-30, -1.000000000000000000 ) ) ;
#77292=CARTESIAN_POINT ( 'NONE',  ( 116.3289480479917017, -32.94026123176625731, 29.13562527591096085 ) ) ;
#77293=CARTESIAN_POINT ( 'NONE',  ( 101.7025241355416796, -45.60450926735023813, 202.1318157521019430 ) ) ;
#77294=ORIENTED_EDGE ( 'NONE', *, *, #38203, .T. ) ;
#77295=ORIENTED_EDGE ( 'NONE', *, *, #43370, .F. ) ;
#77296=CARTESIAN_POINT ( 'NONE',  ( 102.5639289776614191, -44.36196183098122958, 158.5844404487539805 ) ) ;
#77299=CARTESIAN_POINT ( 'NONE',  ( 116.8454820155364331, -34.32316206775963963, 10.45015473446897403 ) ) ;
#77303=EDGE_CURVE ( 'NONE', #20681, #14785, #32711, .T. ) ;
#77305=CARTESIAN_POINT ( 'NONE',  ( 102.0670549556952409, -27.97049806174883813, 106.4897919429764244 ) ) ;
#77306=DIRECTION ( 'NONE',  ( 0.000000000000000000, 1.000000000000000000, 0.000000000000000000 ) ) ;
#77308=CARTESIAN_POINT ( 'NONE',  ( 103.8265608274144256, -48.10271009292828381, 217.3556252759109668 ) ) ;
#77309=CARTESIAN_POINT ( 'NONE',  ( 97.31322288428147260, -38.96126826842726132, 171.5055204312964747 ) ) ;
#77312=CARTESIAN_POINT ( 'NONE',  ( 109.6430121157968074, -46.48008673925917833, 87.78145860803415701 ) ) ;
#77314=CARTESIAN_POINT ( 'NONE',  ( 115.7840308798700022, -41.80076151575822507, 124.4051493520911720 ) ) ;
#77316=CARTESIAN_POINT ( 'NONE',  ( 99.61812512063050917, -43.94476044465307751, 37.95086337114900488 ) ) ;
#77318=EDGE_LOOP ( 'NONE', ( #25820, #47723, #4431, #7032 ) ) ;
#77319=PLANE ( 'NONE',  #58207 ) ;
#77320=DIRECTION ( 'NONE',  ( 0.000000000000000000, 1.000000000000000000, 0.000000000000000000 ) ) ;
#77321=CARTESIAN_POINT ( 'NONE',  ( 115.7763152052227156, -31.00006163510664337, 254.2899109901966028 ) ) ;
#77323=CIRCLE ( 'NONE', #55497, 10.00000000000000711 ) ;
#77326=LINE ( 'NONE', #76424, #70139 ) ;
#77327=CARTESIAN_POINT ( 'NONE',  ( 99.67188489287487130, -33.20771423803368094, 73.79094751244896599 ) ) ;
#77328=CARTESIAN_POINT ( 'NONE',  ( 97.03730526165486481, -41.43059529571826261, 207.6632443235299661 ) ) ;
#77330=ORIENTED_EDGE ( 'NONE', *, *, #42997, .F. ) ;
#77331=DIRECTION ( 'NONE',  ( 0.000000000000000000, 0.000000000000000000, 1.000000000000000000 ) ) ;
#77334=AXIS2_PLACEMENT_3D ( 'NONE', #21245, #68943, #48917 ) ;
#77337=EDGE_LOOP ( 'NONE', ( #38900, #14316 ) ) ;
#77339=EDGE_CURVE ( 'NONE', #60265, #89871, #35098, .T. ) ;
#77340=CARTESIAN_POINT ( 'NONE',  ( 105.8444747722200674, -25.33565403619829226, 322.4846826458744431 ) ) ;
#77341=CARTESIAN_POINT ( 'NONE',  ( 107.5061752250017264, -28.17031325930595642, 94.45813411379100444 ) ) ;
#77342=CARTESIAN_POINT ( 'NONE',  ( 100.0090739042524604, -28.97838942479177149, 285.6641967044823787 ) ) ;
#77343=CARTESIAN_POINT ( 'NONE',  ( 141.0667039024479834, -48.82844715994099971, 250.9178068554160461 ) ) ;
#77345=ORIENTED_EDGE ( 'NONE', *, *, #88046, .T. ) ;
#77346=ORIENTED_EDGE ( 'NONE', *, *, #3130, .F. ) ;
#77348=DIRECTION ( 'NONE',  ( 0.000000000000000000, 1.000000000000000000, 0.000000000000000000 ) ) ;
#77349=DIRECTION ( 'NONE',  ( 0.000000000000000000, 1.000000000000000000, 0.000000000000000000 ) ) ;
#77350=CARTESIAN_POINT ( 'NONE',  ( 116.5825849560772411, -39.12894369053753252, 123.6299109901969615 ) ) ;
#77351=AXIS2_PLACEMENT_3D ( 'NONE', #72992, #58463, #58027 ) ;
#77352=CARTESIAN_POINT ( 'NONE',  ( 113.4422559937560777, -27.64306140573813408, 84.57753003781698453 ) ) ;
#77354=VERTEX_POINT ( 'NONE', #61912 ) ;
#77356=CARTESIAN_POINT ( 'NONE',  ( 103.9392425780951754, -26.78422740453794404, 250.3184824187678714 ) ) ;
#77357=CARTESIAN_POINT ( 'NONE',  ( 131.0667039024480118, -58.35344715994099829, 207.5838068554149913 ) ) ;
#77358=VECTOR ( 'NONE', #70075, 1000.000000000000000 ) ;
#77360=DIRECTION ( 'NONE',  ( 1.000000000000000000, 4.299999999999999979E-14, 1.000000000000000078E-15 ) ) ;
#77362=DIRECTION ( 'NONE',  ( 4.299999999999999979E-14, -1.000000000000000000, 4.400000000000000367E-29 ) ) ;
#77364=CARTESIAN_POINT ( 'NONE',  ( 143.0664832912740110, -8.729447159940999512, 323.8756252759120002 ) ) ;
#77368=ADVANCED_FACE ( 'NONE', ( #47375 ), #27941, .F. ) ;
#77370=CARTESIAN_POINT ( 'NONE',  ( 31.71315051185499811, -33.70561438052090608, -5.074374724088000832 ) ) ;
#77371=ORIENTED_EDGE ( 'NONE', *, *, #36129, .T. ) ;
#77373=LINE ( 'NONE', #70564, #24905 ) ;
#77374=CARTESIAN_POINT ( 'NONE',  ( 105.6290166497307581, -47.07739640705644035, 257.4670538473392298 ) ) ;
#77375=CARTESIAN_POINT ( 'NONE',  ( 108.7432144037193922, -25.80414517310806488, 140.9432443235299672 ) ) ;
#77376=CARTESIAN_POINT ( 'NONE',  ( 104.2350475155005114, -46.78530274442771031, 18.35848241876792031 ) ) ;
#77377=B_SPLINE_CURVE_WITH_KNOTS ( 'NONE', 3,
 ( #88468, #22123, #35720, #43420, #8025, #84355, #71165, #63435, #49791, #48883, #63896, #21211, #77973, #70707, #9370, #15747, #77519, #1221 ),
 .UNSPECIFIED., .F., .F.,
 ( 4, 2, 2, 2, 2, 2, 2, 2, 4 ),
 ( 0.4999969828548403439, 0.5624973599979853356, 0.6249977371411302718, 0.6874981142842752080, 0.7499984914274202552, 0.8124988685705651914, 0.8749992457137101276, 0.9374996228568550638, 1.000000000000000000 ),
 .UNSPECIFIED. ) ;
#77378=FACE_BOUND ( 'NONE', #47570, .T. ) ;
#77380=DIRECTION ( 'NONE',  ( 1.000000000000000078E-15, 0.000000000000000000, -1.000000000000000000 ) ) ;
#77381=CARTESIAN_POINT ( 'NONE',  ( 115.0372256488966087, -42.90850505318414321, 139.3022878054204909 ) ) ;
#77382=VECTOR ( 'NONE', #42277, 1000.000000000000000 ) ;
#77383=EDGE_CURVE ( 'NONE', #88283, #84681, #40582, .T. ) ;
#77385=CARTESIAN_POINT ( 'NONE',  ( 97.81286927418427979, -40.51761286958078756, 126.6352223400343746 ) ) ;
#77386=ORIENTED_EDGE ( 'NONE', *, *, #78657, .T. ) ;
#77387=CARTESIAN_POINT ( 'NONE',  ( 108.6057327191364976, -28.29838476132584191, 164.3552769709339714 ) ) ;
#77390=VECTOR ( 'NONE', #43298, 1000.000000000000000 ) ;
#77392=CARTESIAN_POINT ( 'NONE',  ( 107.9164806882189254, -47.13338536194948603, 173.6413395616249886 ) ) ;
#77393=CARTESIAN_POINT ( 'NONE',  ( 115.7812633450314053, -41.80542298390999179, 149.4069061460392049 ) ) ;
#77395=EDGE_CURVE ( 'NONE', #40665, #58734, #33721, .T. ) ;
#77396=CARTESIAN_POINT ( 'NONE',  ( 49.21213752015946596, -29.73316016639569526, 313.9678068554150059 ) ) ;
#77397=DIRECTION ( 'NONE',  ( 0.000000000000000000, 1.000000000000000000, 0.000000000000000000 ) ) ;
#77398=DIRECTION ( 'NONE',  ( -1.000000000000000078E-15, 1.000000000000000083E-30, 1.000000000000000000 ) ) ;
#77399=CARTESIAN_POINT ( 'NONE',  ( 101.8448680821487073, -28.45912855063583891, 110.5241967044829892 ) ) ;
#77403=CIRCLE ( 'NONE', #41133, 5.500000000000000888 ) ;
#77404=CARTESIAN_POINT ( 'NONE',  ( 102.7262891916532084, -29.00345248032369483, 56.91586902018297423 ) ) ;
#77406=CARTESIAN_POINT ( 'NONE',  ( 116.7860849611260647, -31.33117650353040062, 175.2299109901959753 ) ) ;
#77411=ADVANCED_FACE ( 'NONE', ( #27397 ), #68300, .F. ) ;
#77412=FACE_OUTER_BOUND ( 'NONE', #67604, .T. ) ;
#77415=CARTESIAN_POINT ( 'NONE',  ( 104.9672558511365992, -25.09151557957600076, 125.2184824187689856 ) ) ;
#77417=ORIENTED_EDGE ( 'NONE', *, *, #5307, .T. ) ;
#77418=ORIENTED_EDGE ( 'NONE', *, *, #4004, .T. ) ;
#77422=EDGE_CURVE ( 'NONE', #66156, #71950, #86300, .T. ) ;
#77423=CARTESIAN_POINT ( 'NONE',  ( 115.7831076670964876, -41.80230951558946373, 79.40645860876814766 ) ) ;
#77425=CARTESIAN_POINT ( 'NONE',  ( 99.49937927431119533, -39.79027430526630127, 204.4509475124479536 ) ) ;
#77426=VECTOR ( 'NONE', #53413, 1000.000000000000000 ) ;
#77427=CARTESIAN_POINT ( 'NONE',  ( 177.4809174648215730, -49.32844715993478246, 180.4678068554150059 ) ) ;
#77429=DIRECTION ( 'NONE',  ( -1.907762142705490052E-15, -7.167082501179359715E-16, 1.000000000000000000 ) ) ;
#77430=ORIENTED_EDGE ( 'NONE', *, *, #10985, .F. ) ;
#77432=ORIENTED_EDGE ( 'NONE', *, *, #54677, .F. ) ;
#77434=ORIENTED_EDGE ( 'NONE', *, *, #56129, .F. ) ;
#77435=EDGE_LOOP ( 'NONE', ( #48179, #28491, #75672, #9855, #40147 ) ) ;
#77437=B_SPLINE_CURVE_WITH_KNOTS ( 'NONE', 3,
 ( #2661, #23117, #52544, #31230, #51221, #17178, #23996, #44861, #43513, #16282, #65749, #31682, #2208, #59378, #58055, #71258, #3535, #87110, #58926, #86664, #24438, #79865, #85785, #29914, #23556, #45298, #73018, #24878, #74370, #67547 ),
 .UNSPECIFIED., .F., .F.,
 ( 4, 2, 2, 2, 1, 2, 2, 2, 2, 2, 2, 2, 1, 2, 2, 4 ),
 ( 0.000000000000000000, 0.1249999999999328315, 0.1874999999998993028, 0.2187499999998844258, 0.2343749999998752109, 0.2421874999998733236, 0.2499999999998714362, 0.3749999999998946953, 0.4374999999999019118, 0.4999999999999091838, 0.6249999999999314992, 0.6874999999999480416, 0.7187499999999479305, 0.7343749999999469313, 0.7499999999999458211, 1.000000000000000000 ),
 .UNSPECIFIED. ) ;
#77439=CARTESIAN_POINT ( 'NONE',  ( 110.2543409660563043, -27.89122963701645830, 246.2206309249449703 ) ) ;
#77440=DIRECTION ( 'NONE',  ( 0.0001713722456120069274, -0.9999999853157766072, -0.000000000000000000 ) ) ;
#77442=DIRECTION ( 'NONE',  ( 1.000000000000000000, 0.000000000000000000, 0.000000000000000000 ) ) ;
#77443=CARTESIAN_POINT ( 'NONE',  ( 188.5667039024486087, -48.82844715993430640, 137.2178068554150059 ) ) ;
#77446=AXIS2_PLACEMENT_3D ( 'NONE', #3131, #2244, #85377 ) ;
#77447=CARTESIAN_POINT ( 'NONE',  ( 98.38059522467183626, -41.69557667784989974, 111.7398153013165540 ) ) ;
#77449=ORIENTED_EDGE ( 'NONE', *, *, #26965, .F. ) ;
#77450=ORIENTED_EDGE ( 'NONE', *, *, #2132, .T. ) ;
#77451=CARTESIAN_POINT ( 'NONE',  ( 110.5225122084979574, -28.79501634926980458, 282.5557094172103803 ) ) ;
#77453=CARTESIAN_POINT ( 'NONE',  ( 98.83914123113804351, -30.29059417415423638, 155.7984824187679465 ) ) ;
#77454=CARTESIAN_POINT ( 'NONE',  ( 114.7100688122353063, -43.78666090992615523, 123.2327681330539519 ) ) ;
#77455=CARTESIAN_POINT ( 'NONE',  ( 116.3463703120535513, -39.80474152520470454, 249.5838068554169524 ) ) ;
#77456=DIRECTION ( 'NONE',  ( -1.000000000000000000, 0.000000000000000000, 2.775557561562892929E-14 ) ) ;
#77457=CARTESIAN_POINT ( 'NONE',  ( 105.1109661324377811, -26.48940614006117755, 231.2270538473399597 ) ) ;
#77459=DIRECTION ( 'NONE',  ( -1.045284632676476099E-16, -0.1045284632676476005, -0.9945218953682739560 ) ) ;
#77462=ORIENTED_EDGE ( 'NONE', *, *, #82656, .F. ) ;
#77464=DIRECTION ( 'NONE',  ( -0.7071067811864697461, -0.7071067811866252883, -7.071067811864691403E-16 ) ) ;
#77465=ORIENTED_EDGE ( 'NONE', *, *, #43633, .T. ) ;
#77467=CARTESIAN_POINT ( 'NONE',  ( 103.1745875910851851, -27.05783000869472588, 130.3813395616259925 ) ) ;
#77469=CARTESIAN_POINT ( 'NONE',  ( 135.5068622967102385, -34.38644903112312079, 7.895285856723117668 ) ) ;
#77471=EDGE_CURVE ( 'NONE', #20143, #40854, #73100, .T. ) ;
#77474=CARTESIAN_POINT ( 'NONE',  ( 106.1402962346845982, -47.72062544595559785, 258.4975300378158636 ) ) ;
#77479=LINE ( 'NONE', #22524, #45671 ) ;
#77481=EDGE_CURVE ( 'NONE', #11825, #65478, #395, .T. ) ;
#77482=DIRECTION ( 'NONE',  ( 1.000000000000000000, 1.000000000000000078E-15, 1.000000000000000078E-15 ) ) ;
#77483=CARTESIAN_POINT ( 'NONE',  ( 115.9443088281525149, -30.06633247050010382, 264.3508633711492735 ) ) ;
#77484=ORIENTED_EDGE ( 'NONE', *, *, #15787, .T. ) ;
#77485=EDGE_CURVE ( 'NONE', #26619, #62403, #17261, .T. ) ;
#77486=PLANE ( 'NONE',  #4548 ) ;
#77487=CARTESIAN_POINT ( 'NONE',  ( 117.8235219141173218, -34.08718286818967158, 164.0061014663869798 ) ) ;
#77488=CARTESIAN_POINT ( 'NONE',  ( 116.7699407904022451, -31.43634848722146202, 20.21181575210195902 ) ) ;
#77489=CARTESIAN_POINT ( 'NONE',  ( 104.5521338839504608, -48.36083399734661725, 178.4070538473399665 ) ) ;
#77491=CARTESIAN_POINT ( 'NONE',  ( 20.03715912545641231, -24.95799193693202156, 180.4678068554150911 ) ) ;
#77493=CARTESIAN_POINT ( 'NONE',  ( 164.9667039024476196, -26.71338133338732135, 193.9678068554149775 ) ) ;
#77494=CARTESIAN_POINT ( 'NONE',  ( 97.33784131618190827, -34.07106451174902162, 71.11479194109409718 ) ) ;
#77495=LINE ( 'NONE', #15275, #17745 ) ;
#77497=ORIENTED_EDGE ( 'NONE', *, *, #29306, .T. ) ;
#77498=ADVANCED_FACE ( 'NONE', ( #65406 ), #66735, .T. ) ;
#77500=DIRECTION ( 'NONE',  ( -1.000000000000000000, -4.299999999999999979E-14, -1.000000000000000078E-15 ) ) ;
#77504=ORIENTED_EDGE ( 'NONE', *, *, #6503, .T. ) ;
#77507=CARTESIAN_POINT ( 'NONE',  ( 100.9560042165379770, -28.30978499293933126, 71.57562527591099411 ) ) ;
#77509=EDGE_CURVE ( 'NONE', #12725, #23895, #58477, .T. ) ;
#77510=CARTESIAN_POINT ( 'NONE',  ( 71.24189083761808661, -0.9290567490904538817, 542.9756252759101471 ) ) ;
#77511=CARTESIAN_POINT ( 'NONE',  ( 102.8263616157396854, -46.30098559033366001, 173.2441967044829596 ) ) ;
#77512=CARTESIAN_POINT ( 'NONE',  ( 114.8253727231603136, -41.39981172478538696, 277.8057531614101663 ) ) ;
#77514=ORIENTED_EDGE ( 'NONE', *, *, #68047, .T. ) ;
#77516=VECTOR ( 'NONE', #62333, 1000.000000000000000 ) ;
#77519=CARTESIAN_POINT ( 'NONE',  ( 116.8171228664334365, -34.15291832040662712, 109.0314586092652576 ) ) ;
#77520=AXIS2_PLACEMENT_3D ( 'NONE', #37051, #23446, #9793 ) ;
#77521=DIRECTION ( 'NONE',  ( -1.000000000000000078E-15, 1.000000000000000083E-30, 1.000000000000000000 ) ) ;
#77522=CARTESIAN_POINT ( 'NONE',  ( 180.2143765759500127, -35.91149509760546010, 313.9678068554149490 ) ) ;
#77523=CARTESIAN_POINT ( 'NONE',  ( 108.4186602322921829, -26.73518583127572512, 19.96809642925226669 ) ) ;
#77527=AXIS2_PLACEMENT_3D ( 'NONE', #53219, #88247, #89578 ) ;
#77528=DIRECTION ( 'NONE',  ( 0.7071067811865506814, -0.7071067811865443531, 7.071067811865500971E-16 ) ) ;
#77529=CARTESIAN_POINT ( 'NONE',  ( 104.2468583329775669, -46.74335657891444384, 22.35848241876792031 ) ) ;
#77531=VERTEX_POINT ( 'NONE', #28749 ) ;
#77533=DIRECTION ( 'NONE',  ( 1.000000000000000000, 0.000000000000000000, 0.000000000000000000 ) ) ;
#77535=CARTESIAN_POINT ( 'NONE',  ( 50.96943157740508923, -34.03355364506504799, 117.4678068554150485 ) ) ;
#77536=CARTESIAN_POINT ( 'NONE',  ( 112.4302714532559548, -29.93748856177429118, 122.3747570362579751 ) ) ;
#77537=PLANE ( 'NONE',  #7860 ) ;
#77538=CARTESIAN_POINT ( 'NONE',  ( 176.7738106835696499, -48.62134037881071436, 129.9678068554150059 ) ) ;
#77541=CARTESIAN_POINT ( 'NONE',  ( 116.7952593538610131, -39.38735379887159382, 138.6131012738933634 ) ) ;
#77543=ORIENTED_EDGE ( 'NONE', *, *, #49083, .T. ) ;
#77544=CARTESIAN_POINT ( 'NONE',  ( 102.5639289776614191, -44.36196183098122958, 158.5844404487539805 ) ) ;
#77546=CARTESIAN_POINT ( 'NONE',  ( 97.91349202876114077, -31.62044072442156306, 106.9213395616259703 ) ) ;
#77548=CYLINDRICAL_SURFACE ( 'NONE', #41547, 0.2500000000000002220 ) ;
#77550=( BOUNDED_CURVE ( )  B_SPLINE_CURVE ( 3, ( #60999, #74634, #5149, #11521 ),
 .UNSPECIFIED., .F., .T. ) 
 B_SPLINE_CURVE_WITH_KNOTS ( ( 4, 4 ),
 ( 1.488040654385104793E-11, 1.570796326813557631 ),
 .UNSPECIFIED. ) 
 CURVE ( )  GEOMETRIC_REPRESENTATION_ITEM ( )  RATIONAL_B_SPLINE_CURVE ( ( 1.000000000000000000, 0.8047378541234737614, 0.8047378541234737614, 1.000000000000000000 ) ) 
 REPRESENTATION_ITEM ( '' )  );
#77551=VECTOR ( 'NONE', #63962, 1000.000000000000000 ) ;
#77552=EDGE_LOOP ( 'NONE', ( #34099, #56844, #25743, #62436 ) ) ;
#77554=CARTESIAN_POINT ( 'NONE',  ( 115.5918606122963439, -42.76801532637115599, 53.33562527591095659 ) ) ;
#77556=CARTESIAN_POINT ( 'NONE',  ( 118.5467753794659842, -33.90456151647278205, 14.01848241876796308 ) ) ;
#77557=CARTESIAN_POINT ( 'NONE',  ( 96.72156277063432128, -35.27346698316355145, 177.2156252759109805 ) ) ;
#77560=CARTESIAN_POINT ( 'NONE',  ( 118.9036788419121962, -36.16782713317093112, 114.8641967044819694 ) ) ;
#77561=DIRECTION ( 'NONE',  ( 0.000000000000000000, 0.000000000000000000, 1.000000000000000000 ) ) ;
#77563=CARTESIAN_POINT ( 'NONE',  ( 97.53211280107056780, -39.74980392530692086, 116.5710736105993135 ) ) ;
#77565=CARTESIAN_POINT ( 'NONE',  ( 98.54769938335446966, -41.97705865527272096, 132.7663827518260575 ) ) ;
#77566=ORIENTED_EDGE ( 'NONE', *, *, #57648, .F. ) ;
#77568=ORIENTED_EDGE ( 'NONE', *, *, #77940, .F. ) ;
#77569=CARTESIAN_POINT ( 'NONE',  ( 137.8897065959776000, -5.906223855237799469, -4.824374724088998256 ) ) ;
#77570=CIRCLE ( 'NONE', #64480, 2.116999999999993776 ) ;
#77571=CIRCLE ( 'NONE', #6498, 2.500000000000002220 ) ;
#77573=CARTESIAN_POINT ( 'NONE',  ( 118.2087526870871415, -40.76557371769158777, 23.54991099019593292 ) ) ;
#77577=FACE_OUTER_BOUND ( 'NONE', #13574, .T. ) ;
#77578=CARTESIAN_POINT ( 'NONE',  ( 188.5667039024479834, -65.37844715994100397, 298.0928068554150627 ) ) ;
#77580=CARTESIAN_POINT ( 'NONE',  ( 97.95204982468527533, -33.09064556074055474, 41.02419670448293232 ) ) ;
#77581=CARTESIAN_POINT ( 'NONE',  ( 102.0667094465962919, -27.97069076498398132, 110.4898230829296466 ) ) ;
#77582=CARTESIAN_POINT ( 'NONE',  ( 95.69905522618357452, -33.46911247776740339, 137.1041967044819501 ) ) ;
#77583=CYLINDRICAL_SURFACE ( 'NONE', #36412, 2.500000000000002220 ) ;
#77584=CARTESIAN_POINT ( 'NONE',  ( 172.5664832912740110, -9.303447159940999356, 318.9256252759120116 ) ) ;
#77585=ORIENTED_EDGE ( 'NONE', *, *, #13962, .T. ) ;
#77586=DIRECTION ( 'NONE',  ( 0.7071067811865535679, -0.7071067811865415775, 7.071067811865543372E-16 ) ) ;
#77587=AXIS2_PLACEMENT_3D ( 'NONE', #49107, #41841, #13716 ) ;
#77588=ADVANCED_FACE ( 'NONE', ( #67179 ), #1889, .F. ) ;
#77592=EDGE_CURVE ( 'NONE', #58734, #40665, #55527, .T. ) ;
#77594=CARTESIAN_POINT ( 'NONE',  ( 117.8461808354131080, -34.08161713018977679, 164.0061014663869798 ) ) ;
#77595=ORIENTED_EDGE ( 'NONE', *, *, #73667, .T. ) ;
#77596=CARTESIAN_POINT ( 'NONE',  ( 71.25443513191777356, -74.12815658812309039, 540.9756252759101471 ) ) ;
#77597=CARTESIAN_POINT ( 'NONE',  ( 117.2133579748808927, -41.17085908628773439, 204.4861014663869696 ) ) ;
#77598=CARTESIAN_POINT ( 'NONE',  ( 106.6586400085135438, -26.26872808310278629, 81.10705384733896040 ) ) ;
#77599=CARTESIAN_POINT ( 'NONE',  ( 31.56670390244700641, -22.48495420874110806, 342.9256252759119548 ) ) ;
#77600=DIRECTION ( 'NONE',  ( 0.000000000000000000, 0.000000000000000000, -1.000000000000000000 ) ) ;
#77601=CARTESIAN_POINT ( 'NONE',  ( 117.0718954850710389, -35.46248235502250168, 78.92729194267583637 ) ) ;
#77602=EDGE_LOOP ( 'NONE', ( #54921, #69629, #22915, #57491 ) ) ;
#77606=VERTEX_POINT ( 'NONE', #53520 ) ;
#77610=LINE ( 'NONE', #16724, #77175 ) ;
#77611=CARTESIAN_POINT ( 'NONE',  ( 109.9892391005685255, -26.72245031140752758, 255.8499109901966051 ) ) ;
#77613=CARTESIAN_POINT ( 'NONE',  ( 136.5183630979287557, -17.48272428402880863, 2.716753546994847834 ) ) ;
#77614=EDGE_CURVE ( 'NONE', #46964, #89573, #6302, .T. ) ;
#77617=DIRECTION ( 'NONE',  ( 1.000000000000000000, 0.000000000000000000, -7.723290606088049820E-15 ) ) ;
#77618=CARTESIAN_POINT ( 'NONE',  ( 116.4074703635738075, -31.97189281592868682, 44.20133956162491984 ) ) ;
#77620=VECTOR ( 'NONE', #30683, 1000.000000000000000 ) ;
#77622=DIRECTION ( 'NONE',  ( -4.237773401492740281E-14, 1.000000000000000000, 0.000000000000000000 ) ) ;
#77625=CARTESIAN_POINT ( 'NONE',  ( 109.0793648129487678, -47.66380996059997699, 273.7213395616246885 ) ) ;
#77627=CARTESIAN_POINT ( 'NONE',  ( 98.99072789581764198, -31.21169308021403310, 116.8499109901959514 ) ) ;
#77628=CARTESIAN_POINT ( 'NONE',  ( 33.96670390244745619, -26.71338133339334320, 237.4678068554150059 ) ) ;
#77629=LINE ( 'NONE', #43979, #25681 ) ;
#77631=DIRECTION ( 'NONE',  ( 0.000000000000000000, 0.000000000000000000, -1.000000000000000000 ) ) ;
#77632=CARTESIAN_POINT ( 'NONE',  ( 97.39134470890573425, -39.27871236491387918, 57.53145266978995664 ) ) ;
#77634=ORIENTED_EDGE ( 'NONE', *, *, #56255, .F. ) ;
#77635=EDGE_CURVE ( 'NONE', #43132, #29159, #48062, .T. ) ;
#77637=CARTESIAN_POINT ( 'NONE',  ( 116.4478251454372923, -36.21277458701120366, 270.3139642582781335 ) ) ;
#77640=VECTOR ( 'NONE', #56704, 1000.000000000000000 ) ;
#77641=VECTOR ( 'NONE', #74828, 1000.000000000000000 ) ;
#77642=CYLINDRICAL_SURFACE ( 'NONE', #2922, 5.599999999999994316 ) ;
#77643=VECTOR ( 'NONE', #16004, 1000.000000000000000 ) ;
#77644=DIRECTION ( 'NONE',  ( 0.000000000000000000, -1.000000000000000000, 0.000000000000000000 ) ) ;
#77649=CARTESIAN_POINT ( 'NONE',  ( 107.0664832912739968, -0.7548456658612000547, 333.4006252759120343 ) ) ;
#77650=ORIENTED_EDGE ( 'NONE', *, *, #49686, .F. ) ;
#77651=CARTESIAN_POINT ( 'NONE',  ( 116.6749405801447921, -32.59381477748385691, 79.14991099019697174 ) ) ;
#77653=CARTESIAN_POINT ( 'NONE',  ( 101.0492827672293714, -31.21374014463884805, 273.5538046553056688 ) ) ;
#77654=CARTESIAN_POINT ( 'NONE',  ( 98.30786778252010549, -41.72947753537307847, 126.7394794444259247 ) ) ;
#77655=CARTESIAN_POINT ( 'NONE',  ( 116.8431970675092515, -40.18699730018606431, 178.5680062282919778 ) ) ;
#77656=EDGE_CURVE ( 'NONE', #54421, #25056, #81716, .T. ) ;
#77657=CARTESIAN_POINT ( 'NONE',  ( 134.0664832912739826, -8.729447159941003065, 1.325625275910988554 ) ) ;
#77658=PLANE ( 'NONE',  #70485 ) ;
#77661=CARTESIAN_POINT ( 'NONE',  ( 97.18271318096459765, -40.28600493293344442, 262.6013395616255934 ) ) ;
#77666=VERTEX_POINT ( 'NONE', #46265 ) ;
#77667=CARTESIAN_POINT ( 'NONE',  ( 113.3575164265628672, -45.09699625868619677, 139.0899109901969553 ) ) ;
#77668=CARTESIAN_POINT ( 'NONE',  ( 79.05226586199776762, -21.28573230649618608, 1.785258109343569100 ) ) ;
#77669=ORIENTED_EDGE ( 'NONE', *, *, #47690, .F. ) ;
#77670=AXIS2_PLACEMENT_3D ( 'NONE', #1515, #29217, #56903 ) ;
#77672=ORIENTED_EDGE ( 'NONE', *, *, #51917, .F. ) ;
#77673=DIRECTION ( 'NONE',  ( 1.000000000000000078E-15, 1.000000000000000083E-30, -1.000000000000000000 ) ) ;
#77675=FACE_OUTER_BOUND ( 'NONE', #63340, .T. ) ;
#77676=DIRECTION ( 'NONE',  ( 0.000000000000000000, 0.000000000000000000, 1.000000000000000000 ) ) ;
#77677=CARTESIAN_POINT ( 'NONE',  ( 168.0371591254546217, -48.62818131005519007, 129.9678068554150059 ) ) ;
#77678=CARTESIAN_POINT ( 'NONE',  ( 112.1812230000633832, -27.60471316448668588, 30.66991099019694644 ) ) ;
#77679=DIRECTION ( 'NONE',  ( 0.000000000000000000, 1.000000000000000000, 0.000000000000000000 ) ) ;
#77681=CARTESIAN_POINT ( 'NONE',  ( 126.9629299006806775, -54.68655584847609674, -5.074374724088952959 ) ) ;
#77682=DIRECTION ( 'NONE',  ( -0.7071067811855900054, -0.7071067811875051401, 0.000000000000000000 ) ) ;
#77686=CARTESIAN_POINT ( 'NONE',  ( 82.46407580265253046, -20.08864647352212174, 2.654395117675909965 ) ) ;
#77688=CIRCLE ( 'NONE', #32676, 2.517499999999998739 ) ;
#77689=DIRECTION ( 'NONE',  ( 0.000000000000000000, 0.000000000000000000, -1.000000000000000000 ) ) ;
#77694=CARTESIAN_POINT ( 'NONE',  ( 97.42200983434074146, -37.84960760947268454, 235.8409912566479818 ) ) ;
#77695=CARTESIAN_POINT ( 'NONE',  ( 20.03715912545730760, -24.42818131006189830, 300.4678068554150059 ) ) ;
#77697=CARTESIAN_POINT ( 'NONE',  ( 96.59500279541983048, -37.56604165528066375, 101.3899109901969524 ) ) ;
#77701=ADVANCED_FACE ( 'NONE', ( #46722, #33112 ), #19484, .F. ) ;
#77702=CARTESIAN_POINT ( 'NONE',  ( 97.81169160209351787, -40.51741184665055329, 67.63577596198375375 ) ) ;
#77705=DIRECTION ( 'NONE',  ( 0.000000000000000000, 1.000000000000000000, 0.000000000000000000 ) ) ;
#77706=EDGE_CURVE ( 'NONE', #40317, #24929, #22202, .T. ) ;
#77708=DIRECTION ( 'NONE',  ( 1.000000000000000078E-15, 0.000000000000000000, -1.000000000000000000 ) ) ;
#77709=CARTESIAN_POINT ( 'NONE',  ( 115.7844980097995062, -41.79996075137723466, 274.4062243839134112 ) ) ;
#77713=CARTESIAN_POINT ( 'NONE',  ( 117.3753987692272602, -38.63066374137464720, 88.68133956162493803 ) ) ;
#77718=CARTESIAN_POINT ( 'NONE',  ( 25.56670390244797275, -62.87844715994099687, 137.2178068554150059 ) ) ;
#77720=CARTESIAN_POINT ( 'NONE',  ( 83.56670559755329464, -33.43837296219065536, 239.5838068554176914 ) ) ;
#77722=VERTEX_POINT ( 'NONE', #26296 ) ;
#77725=DIRECTION ( 'NONE',  ( 1.000000000000000000, 4.163336342344333240E-14, 0.000000000000000000 ) ) ;
#77726=CARTESIAN_POINT ( 'NONE',  ( 25.56670390244797275, -58.35344715994099829, 137.2178068554150059 ) ) ;
#77727=CIRCLE ( 'NONE', #42874, 0.4999999999999989453 ) ;
#77728=CARTESIAN_POINT ( 'NONE',  ( 46.03715912545343514, -48.62818131006090283, 180.4678068554150911 ) ) ;
#77729=CARTESIAN_POINT ( 'NONE',  ( 97.55141575199942849, -31.05946519635597269, 126.9108633711489915 ) ) ;
#77730=CARTESIAN_POINT ( 'NONE',  ( 163.0959832912742797, -23.42844715993517113, 117.4678068554150485 ) ) ;
#77731=DIRECTION ( 'NONE',  ( -1.000000000000000078E-15, 1.000000000000000083E-30, 1.000000000000000000 ) ) ;
#77733=TOROIDAL_SURFACE ( 'NONE', #89341, 11.75000000000000000, 2.550000000000000266 ) ;
#77734=ORIENTED_EDGE ( 'NONE', *, *, #50920, .T. ) ;
#77736=CARTESIAN_POINT ( 'NONE',  ( 181.9694315774339941, -34.03355364505720360, -5.074374724088000832 ) ) ;
#77737=CARTESIAN_POINT ( 'NONE',  ( 103.2980200187117816, -27.06831524915196141, 166.3603871806719496 ) ) ;
#77738=DIRECTION ( 'NONE',  ( 0.000000000000000000, 0.000000000000000000, 1.000000000000000000 ) ) ;
#77740=CARTESIAN_POINT ( 'NONE',  ( 117.3951115944450123, -37.65585020919950665, 29.74324432352998215 ) ) ;
#77742=DIRECTION ( 'NONE',  ( 0.000000000000000000, 1.000000000000000000, 0.000000000000000000 ) ) ;
#77745=CARTESIAN_POINT ( 'NONE',  ( 46.03715912545427358, -48.62818131006086020, 300.4678068554150059 ) ) ;
#77746=CARTESIAN_POINT ( 'NONE',  ( 113.3831382903590992, -27.58002901871518020, 239.5956252759109759 ) ) ;
#77748=ORIENTED_EDGE ( 'NONE', *, *, #27242, .T. ) ;
#77749=ADVANCED_FACE ( 'NONE', ( #74900 ), #68534, .T. ) ;
#77750=CARTESIAN_POINT ( 'NONE',  ( 115.7125814391468737, -38.67428926243481158, 145.0815833058969702 ) ) ;
#77752=CARTESIAN_POINT ( 'NONE',  ( 97.02995690277612084, -35.86988738539728416, 32.69015473446795994 ) ) ;
#77754=EDGE_CURVE ( 'NONE', #593, #17048, #40370, .T. ) ;
#77758=DIRECTION ( 'NONE',  ( 0.000000000000000000, 0.000000000000000000, 1.000000000000000000 ) ) ;
#77759=CARTESIAN_POINT ( 'NONE',  ( 114.3996560367811810, -27.45190519937920470, 274.5441967044824878 ) ) ;
#77761=ORIENTED_EDGE ( 'NONE', *, *, #69032, .T. ) ;
#77762=ORIENTED_EDGE ( 'NONE', *, *, #80984, .F. ) ;
#77764=CARTESIAN_POINT ( 'NONE',  ( 82.67951041502472265, -19.60592655296214204, 6.943955837755186877 ) ) ;
#77765=DIRECTION ( 'NONE',  ( 0.000000000000000000, 1.000000000000000000, 0.000000000000000000 ) ) ;
#77767=AXIS2_PLACEMENT_3D ( 'NONE', #41769, #28146, #55837 ) ;
#77768=CARTESIAN_POINT ( 'NONE',  ( 97.35451824726690973, -37.88753622196094284, 37.42133956162496844 ) ) ;
#77769=CIRCLE ( 'NONE', #38587, 2.517499999999998739 ) ;
#77771=ORIENTED_EDGE ( 'NONE', *, *, #5094, .T. ) ;
#77778=CARTESIAN_POINT ( 'NONE',  ( 107.5100371804366688, -47.14531440222233272, 237.6099109901969655 ) ) ;
#77780=DIRECTION ( 'NONE',  ( 1.000000000000000000, 0.000000000000000000, -0.000000000000000000 ) ) ;
#77781=CARTESIAN_POINT ( 'NONE',  ( 182.6664832912729821, 12.92155284005730387, 361.9756252759109998 ) ) ;
#77783=CARTESIAN_POINT ( 'NONE',  ( 100.6253115865833365, -30.05058211904245624, 113.5052332267339779 ) ) ;
#77784=CARTESIAN_POINT ( 'NONE',  ( 114.9943830143096335, -28.99422824087939432, 190.4537205140059655 ) ) ;
#77788=DIRECTION ( 'NONE',  ( 0.000000000000000000, -1.000000000000000000, 0.000000000000000000 ) ) ;
#77789=VERTEX_POINT ( 'NONE', #22633 ) ;
#77790=ORIENTED_EDGE ( 'NONE', *, *, #18924, .T. ) ;
#77791=CYLINDRICAL_SURFACE ( 'NONE', #51690, 2.517500000000005844 ) ;
#77792=ORIENTED_EDGE ( 'NONE', *, *, #36957, .F. ) ;
#77793=ORIENTED_EDGE ( 'NONE', *, *, #21092, .T. ) ;
#77794=CARTESIAN_POINT ( 'NONE',  ( 25.56670390244797275, -62.87844715994099687, 259.9678068554150059 ) ) ;
#77796=CARTESIAN_POINT ( 'NONE',  ( 116.3148031259206192, -32.94054721833379062, 24.13562527591095375 ) ) ;
#77798=CARTESIAN_POINT ( 'NONE',  ( 99.91372553312717741, -41.39787175238471661, 101.2095626852199644 ) ) ;
#77799=CARTESIAN_POINT ( 'NONE',  ( 105.0173152498862947, -25.84384494483574102, 280.2365776568630622 ) ) ;
#77800=ADVANCED_FACE ( 'NONE', ( #28520 ), #56213, .F. ) ;
#77801=DIRECTION ( 'NONE',  ( -0.9963424814100680926, 0.08544974978095698503, 0.000000000000000000 ) ) ;
#77804=ORIENTED_EDGE ( 'NONE', *, *, #24195, .F. ) ;
#77805=EDGE_CURVE ( 'NONE', #58818, #43667, #84864, .T. ) ;
#77806=ORIENTED_EDGE ( 'NONE', *, *, #12387, .F. ) ;
#77807=DIRECTION ( 'NONE',  ( 0.000000000000000000, 0.000000000000000000, -1.000000000000000000 ) ) ;
#77810=CARTESIAN_POINT ( 'NONE',  ( 97.57695254711111943, -30.97082841205668657, 125.8803871806719599 ) ) ;
#77811=DIRECTION ( 'NONE',  ( 1.000000000000000078E-15, -1.000000000000000083E-30, -1.000000000000000000 ) ) ;
#77814=CARTESIAN_POINT ( 'NONE',  ( 111.7391504816189212, -27.40993963462091543, 279.7070538473396937 ) ) ;
#77815=CARTESIAN_POINT ( 'NONE',  ( 83.56670390244799762, -36.72944715994108122, 239.5838068554169809 ) ) ;
#77816=DIRECTION ( 'NONE',  ( 0.000000000000000000, 1.000000000000000000, 0.000000000000000000 ) ) ;
#77821=LINE ( 'NONE', #15599, #25036 ) ;
#77822=CARTESIAN_POINT ( 'NONE',  ( 132.4924365228324916, -38.98954602992306917, 7.829737527538009445 ) ) ;
#77828=CARTESIAN_POINT ( 'NONE',  ( 107.0664832912739399, -36.72944715994095333, 302.4856252759109907 ) ) ;
#77831=CARTESIAN_POINT ( 'NONE',  ( 115.9788024870550061, -30.15175701148841725, 259.3203871806730945 ) ) ;
#77832=CARTESIAN_POINT ( 'NONE',  ( 107.9182609186041333, -47.15517531916538019, 173.6413395616249886 ) ) ;
#77833=CARTESIAN_POINT ( 'NONE',  ( 99.99465048579469340, -28.96254792738658779, 281.6641967044822650 ) ) ;
#77834=AXIS2_PLACEMENT_3D ( 'NONE', #87049, #31616, #53824 ) ;
#77835=CARTESIAN_POINT ( 'NONE',  ( 63.56670390244714497, -40.82844715994014706, 129.9678068554150911 ) ) ;
#77836=CARTESIAN_POINT ( 'NONE',  ( 80.43833865489237667, -33.97944715994105991, 8.225625275910944723 ) ) ;
#77837=CARTESIAN_POINT ( 'NONE',  ( 113.1782416917127705, -44.75190934023923006, 139.0939534517803793 ) ) ;
#77838=VECTOR ( 'NONE', #14183, 1000.000000000000000 ) ;
#77841=CIRCLE ( 'NONE', #38654, 2.030000000001869864 ) ;
#77843=DIRECTION ( 'NONE',  ( 1.000000000000000000, 4.299999999999999979E-14, 1.000000000000000078E-15 ) ) ;
#77845=CARTESIAN_POINT ( 'NONE',  ( 98.53214291706959216, -37.07752924029257713, 160.7809912566479511 ) ) ;
#77846=CARTESIAN_POINT ( 'NONE',  ( 117.0727434263538669, -35.46952932352849075, 188.9273346943833758 ) ) ;
#77847=ORIENTED_EDGE ( 'NONE', *, *, #72993, .F. ) ;
#77848=CARTESIAN_POINT ( 'NONE',  ( 37.35959712144463651, -48.62134037893550698, 249.9678068554150343 ) ) ;
#77849=CARTESIAN_POINT ( 'NONE',  ( 98.39792771585426578, -29.90889243069713288, 196.8080062282919869 ) ) ;
#77851=CARTESIAN_POINT ( 'NONE',  ( 29.56648329127298069, -81.37844715994266664, 342.9256252759109884 ) ) ;
#77852=CARTESIAN_POINT ( 'NONE',  ( 108.4238121438592231, -26.80045362567452472, 85.96918707036505225 ) ) ;
#77854=CARTESIAN_POINT ( 'NONE',  ( 97.81360741897486832, -40.52211042289001597, 96.63602782802603031 ) ) ;
#77855=VECTOR ( 'NONE', #5621, 1000.000000000000000 ) ;
#77856=CARTESIAN_POINT ( 'NONE',  ( 108.4956486572523744, -46.43878675094428843, 142.6927681330539883 ) ) ;
#77857=VERTEX_POINT ( 'NONE', #7204 ) ;
#77860=CARTESIAN_POINT ( 'NONE',  ( 111.9059958850653800, -29.27014106345288624, 66.05015473446795227 ) ) ;
#77861=VECTOR ( 'NONE', #88416, 1000.000000000000000 ) ;
#77863=CARTESIAN_POINT ( 'NONE',  ( 99.76930146980372172, -30.21680002102814555, 186.7470538473389752 ) ) ;
#77867=EDGE_CURVE ( 'NONE', #71530, #64390, #6747, .T. ) ;
#77871=CARTESIAN_POINT ( 'NONE',  ( 117.1882713363357169, -39.28166824301213467, 123.6299109901969615 ) ) ;
#77872=ORIENTED_EDGE ( 'NONE', *, *, #20769, .F. ) ;
#77874=ORIENTED_EDGE ( 'NONE', *, *, #10203, .F. ) ;
#77877=FACE_OUTER_BOUND ( 'NONE', #11694, .T. ) ;
#77878=CARTESIAN_POINT ( 'NONE',  ( 99.25992742994408502, -40.46556956555936324, 214.5118998934009653 ) ) ;
#77881=DIRECTION ( 'NONE',  ( 0.000000000000000000, 0.000000000000000000, 1.000000000000000000 ) ) ;
#77882=CARTESIAN_POINT ( 'NONE',  ( 114.1752211786757414, -45.19379553418442441, 148.1203871806719405 ) ) ;
#77883=CARTESIAN_POINT ( 'NONE',  ( 134.0664832912740110, -8.729447159940999512, 308.6356252759119911 ) ) ;
#77884=VERTEX_POINT ( 'NONE', #8551 ) ;
#77885=EDGE_LOOP ( 'NONE', ( #85711, #20246, #5244, #25912, #83325 ) ) ;
#77886=ORIENTED_EDGE ( 'NONE', *, *, #5701, .F. ) ;
#77887=DIRECTION ( 'NONE',  ( 4.299999999999999979E-14, -1.000000000000000000, 0.000000000000000000 ) ) ;
#77890=DIRECTION ( 'NONE',  ( -1.000000000000000000, -6.193183223602000661E-14, -1.000000000000000078E-15 ) ) ;
#77891=FACE_OUTER_BOUND ( 'NONE', #84725, .T. ) ;
#77892=CARTESIAN_POINT ( 'NONE',  ( 101.9834712436270507, -43.98831800240917289, 278.5215833058970247 ) ) ;
#77893=EDGE_CURVE ( 'NONE', #35637, #24486, #72936, .T. ) ;
#77894=CARTESIAN_POINT ( 'NONE',  ( 112.0659110422256930, -45.48839660081501535, 272.9897918895903217 ) ) ;
#77895=VERTEX_POINT ( 'NONE', #83075 ) ;
#77897=CARTESIAN_POINT ( 'NONE',  ( 115.4645620972963513, -40.57776935811419605, 9.635625275910941312 ) ) ;
#77898=CYLINDRICAL_SURFACE ( 'NONE', #27117, 2.500000000000002220 ) ;
#77901=AXIS2_PLACEMENT_3D ( 'NONE', #279, #27977, #55652 ) ;
#77902=CIRCLE ( 'NONE', #73532, 10.00000000000002487 ) ;
#77903=CARTESIAN_POINT ( 'NONE',  ( 98.15101777340095168, -41.26169252765487272, 111.7007443023918825 ) ) ;
#77904=CIRCLE ( 'NONE', #66263, 9.571100913904423635 ) ;
#77905=ORIENTED_EDGE ( 'NONE', *, *, #29504, .F. ) ;
#77906=ORIENTED_EDGE ( 'NONE', *, *, #75229, .T. ) ;
#77908=CARTESIAN_POINT ( 'NONE',  ( 105.5338363264665986, -28.21170577469638729, 273.0242808457819592 ) ) ;
#77909=CARTESIAN_POINT ( 'NONE',  ( 97.93707779058323126, -30.45653744243544736, 165.8594347997199634 ) ) ;
#77910=CARTESIAN_POINT ( 'NONE',  ( 99.43809884604145566, -27.69271567064627604, 150.6356252759109680 ) ) ;
#77912=FACE_OUTER_BOUND ( 'NONE', #33015, .T. ) ;
#77913=CARTESIAN_POINT ( 'NONE',  ( 110.1374552785425323, -26.11139123911904036, 210.8403871806729626 ) ) ;
#77916=DIRECTION ( 'NONE',  ( -0.7071067811864671926, -0.7071067811866279529, -6.612322855854137577E-17 ) ) ;
#77917=VERTEX_POINT ( 'NONE', #49857 ) ;
#77920=ORIENTED_EDGE ( 'NONE', *, *, #29310, .T. ) ;
#77923=VECTOR ( 'NONE', #34323, 1000.000000000000000 ) ;
#77924=CARTESIAN_POINT ( 'NONE',  ( 96.00724586008001893, -35.77752748456175169, 186.2461014663869889 ) ) ;
#77925=ORIENTED_EDGE ( 'NONE', *, *, #37926, .F. ) ;
#77926=CARTESIAN_POINT ( 'NONE',  ( 113.9170494572507266, -28.05483877344520849, 124.5565776568629559 ) ) ;
#77930=CARTESIAN_POINT ( 'NONE',  ( 184.5664832912740110, 15.62155284005900491, 323.8756252759109202 ) ) ;
#77931=CARTESIAN_POINT ( 'NONE',  ( 116.9441839019826261, -38.62175960871475411, 58.67575922383635145 ) ) ;
#77932=CARTESIAN_POINT ( 'NONE',  ( 96.27200394136428940, -34.46162041542912391, 257.1737205140064475 ) ) ;
#77934=CARTESIAN_POINT ( 'NONE',  ( 188.5667039024485518, -48.82844715993430640, 173.2178068554150059 ) ) ;
#77936=EDGE_CURVE ( 'NONE', #1366, #20465, #14920, .T. ) ;
#77937=CARTESIAN_POINT ( 'NONE',  ( 90.44969454456403923, -20.11243780205715481, 239.5838068554169809 ) ) ;
#77938=EDGE_CURVE ( 'NONE', #69845, #13929, #48948, .T. ) ;
#77939=CARTESIAN_POINT ( 'NONE',  ( 99.09570906053022554, -30.55043177293176981, 256.8022919445643879 ) ) ;
#77940=EDGE_CURVE ( 'NONE', #46193, #5603, #76691, .T. ) ;
#77941=CARTESIAN_POINT ( 'NONE',  ( 172.5664832912729878, -27.82844715994070484, 198.9256252759119832 ) ) ;
#77942=CARTESIAN_POINT ( 'NONE',  ( 99.30039714715974242, -28.79844535499942637, 270.7051490854347549 ) ) ;
#77943=ORIENTED_EDGE ( 'NONE', *, *, #61297, .T. ) ;
#77945=CARTESIAN_POINT ( 'NONE',  ( 108.8526476014722277, -47.02293932800507292, 167.7127681330539701 ) ) ;
#77946=CARTESIAN_POINT ( 'NONE',  ( 99.50169031327072844, -43.90275843488763741, 77.92991099019597812 ) ) ;
#77947=CARTESIAN_POINT ( 'NONE',  ( 113.1808386317757282, -26.52034477659904610, 200.6470538473399756 ) ) ;
#77948=ADVANCED_FACE ( 'NONE', ( #50766 ), #16704, .T. ) ;
#77950=CARTESIAN_POINT ( 'NONE',  ( 163.1639762274590169, -34.03355364505800651, -5.074374724088000832 ) ) ;
#77953=CARTESIAN_POINT ( 'NONE',  ( 112.1393456458850579, -28.01282278379046886, 69.65645860885391016 ) ) ;
#77956=AXIS2_PLACEMENT_3D ( 'NONE', #63409, #71584, #43398 ) ;
#77957=PLANE ( 'NONE',  #45543 ) ;
#77958=ORIENTED_EDGE ( 'NONE', *, *, #80192, .F. ) ;
#77962=CARTESIAN_POINT ( 'NONE',  ( 96.97787942770426639, -32.27031107066119375, 51.98324432352996638 ) ) ;
#77963=CARTESIAN_POINT ( 'NONE',  ( 25.56670390244797275, -62.87844715994099687, 257.2178068554150059 ) ) ;
#77964=DIRECTION ( 'NONE',  ( 0.7071067811865449082, 0.7071067811865501263, 7.071067811865448709E-16 ) ) ;
#77967=CARTESIAN_POINT ( 'NONE',  ( 113.6113952709150396, -31.24125447920927101, 268.8038483995053411 ) ) ;
#77971=VECTOR ( 'NONE', #80506, 1000.000000000000000 ) ;
#77973=CARTESIAN_POINT ( 'NONE',  ( 115.7831076709258582, -41.80230950872173423, 108.4064586093909384 ) ) ;
#77974=DIRECTION ( 'NONE',  ( -1.147230458779309805E-16, 0.000000000000000000, -1.000000000000000000 ) ) ;
#77976=CARTESIAN_POINT ( 'NONE',  ( 112.1388153513013037, -28.01251898142565011, 160.6565068732068937 ) ) ;
#77977=CARTESIAN_POINT ( 'NONE',  ( 97.07211725179735140, -35.37804438830692533, 21.21817328746602982 ) ) ;
#77980=EDGE_CURVE ( 'NONE', #66368, #6493, #4804, .T. ) ;
#77981=DIRECTION ( 'NONE',  ( -1.000000000000000000, 0.000000000000000000, 0.000000000000000000 ) ) ;
#77982=DIRECTION ( 'NONE',  ( 1.705911707540438309E-29, 0.7071067811865391350, -0.7071067811865560104 ) ) ;
#77983=CARTESIAN_POINT ( 'NONE',  ( 116.4547782460827250, -32.24742764444978604, 19.18133956162493092 ) ) ;
#77985=VECTOR ( 'NONE', #55308, 1000.000000000000000 ) ;
#77986=CARTESIAN_POINT ( 'NONE',  ( 98.34985944185039841, -31.65658391562952545, 270.9064585273550847 ) ) ;
#77987=VECTOR ( 'NONE', #17752, 1000.000000000000000 ) ;
#77988=AXIS2_PLACEMENT_3D ( 'NONE', #9422, #72979, #52938 ) ;
#77989=DIRECTION ( 'NONE',  ( -0.0001713722456120069274, 0.9999999853157766072, 0.000000000000000000 ) ) ;
#77990=CARTESIAN_POINT ( 'NONE',  ( 115.0182259351703777, -41.51125854152899564, 126.2138046553059638 ) ) ;
#77994=CARTESIAN_POINT ( 'NONE',  ( 116.3229784443844324, -32.93528945216412041, 94.13562527591096796 ) ) ;
#77998=EDGE_CURVE ( 'NONE', #15487, #20374, #54110, .T. ) ;
#77999=CARTESIAN_POINT ( 'NONE',  ( 109.6432586217883909, -46.48002561855553694, 137.7791137709158988 ) ) ;
#78000=VERTEX_POINT ( 'NONE', #71233 ) ;
#78003=CARTESIAN_POINT ( 'NONE',  ( 103.0256836488564716, -28.24720316769774797, 136.8739642582779652 ) ) ;
#78004=ADVANCED_FACE ( 'NONE', ( #3508 ), #31205, .T. ) ;
#78006=CARTESIAN_POINT ( 'NONE',  ( 103.2709630098024576, -47.13517786649186547, 93.28610146638693834 ) ) ;
#78008=EDGE_CURVE ( 'NONE', #48239, #47446, #26513, .T. ) ;
#78009=CARTESIAN_POINT ( 'NONE',  ( 113.6855641942755142, -44.25381336270734067, 18.15052713635613557 ) ) ;
#78010=VERTEX_POINT ( 'NONE', #58902 ) ;
#78011=EDGE_CURVE ( 'NONE', #89277, #48723, #9004, .T. ) ;
#78013=VERTEX_POINT ( 'NONE', #85764 ) ;
#78015=CARTESIAN_POINT ( 'NONE',  ( 103.8344565422589767, -46.70152647745319996, 82.32705384733995402 ) ) ;
#78016=ORIENTED_EDGE ( 'NONE', *, *, #83207, .T. ) ;
#78017=CARTESIAN_POINT ( 'NONE',  ( 97.37192905580960200, -32.85904099757679830, 41.02419670448193045 ) ) ;
#78018=CARTESIAN_POINT ( 'NONE',  ( 98.24294948823698803, -42.32252413779357170, 182.7756252759109543 ) ) ;
#78020=CARTESIAN_POINT ( 'NONE',  ( 92.82872956494375671, -30.11307588647346023, 0.7256252759109567130 ) ) ;
#78022=CARTESIAN_POINT ( 'NONE',  ( 99.05421528594702352, -43.39923342774125814, 112.8784824187679732 ) ) ;
#78025=ORIENTED_EDGE ( 'NONE', *, *, #71346, .T. ) ;
#78026=CARTESIAN_POINT ( 'NONE',  ( 130.3998166246070127, 12.92155284005802685, 335.5992267699912190 ) ) ;
#78027=AXIS2_PLACEMENT_3D ( 'NONE', #39569, #19580, #33215 ) ;
#78028=VERTEX_POINT ( 'NONE', #51646 ) ;
#78029=CARTESIAN_POINT ( 'NONE',  ( 22.49563609058250435, -67.87844715994100397, 13.84673904354932361 ) ) ;
#78030=VERTEX_POINT ( 'NONE', #17151 ) ;
#78034=AXIS2_PLACEMENT_3D ( 'NONE', #46381, #66847, #81407 ) ;
#78035=LINE ( 'NONE', #83491, #66718 ) ;
#78036=CARTESIAN_POINT ( 'NONE',  ( 112.1173730388400287, -26.89747643418222722, 19.71086337114896736 ) ) ;
#78040=CARTESIAN_POINT ( 'NONE',  ( 101.3196941207356758, -46.24713579373447914, 52.14419670448295108 ) ) ;
#78041=CARTESIAN_POINT ( 'NONE',  ( 97.79845349656991971, -40.48495068833381083, 111.6328342125843989 ) ) ;
#78042=CARTESIAN_POINT ( 'NONE',  ( 103.8142050530422864, -26.84757730287823563, 161.3299109901969643 ) ) ;
#78043=CARTESIAN_POINT ( 'NONE',  ( 112.1393456392507630, -28.01282277969801626, 70.65645860946722223 ) ) ;
#78047=EDGE_CURVE ( 'NONE', #22553, #32339, #2183, .T. ) ;
#78048=VECTOR ( 'NONE', #61636, 1000.000000000000000 ) ;
#78051=EDGE_CURVE ( 'NONE', #29424, #61339, #30985, .T. ) ;
#78052=ORIENTED_EDGE ( 'NONE', *, *, #75449, .F. ) ;
#78054=AXIS2_PLACEMENT_3D ( 'NONE', #88748, #87395, #25155 ) ;
#78055=LINE ( 'NONE', #36255, #66472 ) ;
#78056=CARTESIAN_POINT ( 'NONE',  ( 114.3747829841801149, -29.18355094256887838, 174.4641967044819637 ) ) ;
#78057=ORIENTED_EDGE ( 'NONE', *, *, #52928, .T. ) ;
#78058=PLANE ( 'NONE',  #29191 ) ;
#78059=CARTESIAN_POINT ( 'NONE',  ( 107.2435369062854420, -47.21027956138831883, 208.5899109901969837 ) ) ;
#78060=CARTESIAN_POINT ( 'NONE',  ( 112.8257383337702606, -47.14300054286279362, 98.97848241876793907 ) ) ;
#78061=AXIS2_PLACEMENT_3D ( 'NONE', #2685, #31259, #9056 ) ;
#78062=EDGE_CURVE ( 'NONE', #23208, #86726, #38034, .T. ) ;
#78064=VECTOR ( 'NONE', #88651, 1000.000000000000000 ) ;
#78065=CARTESIAN_POINT ( 'NONE',  ( 156.5667039024483245, -42.82844715993568485, 170.7178068554149775 ) ) ;
#78067=ORIENTED_EDGE ( 'NONE', *, *, #77706, .F. ) ;
#78070=VERTEX_POINT ( 'NONE', #9437 ) ;
#78071=VERTEX_POINT ( 'NONE', #37148 ) ;
#78073=CARTESIAN_POINT ( 'NONE',  ( 118.0406971908402340, -35.41012545131285094, 234.9337205140059552 ) ) ;
#78076=CARTESIAN_POINT ( 'NONE',  ( 25.56670390244797275, -67.87844715994100397, 173.2178068554149775 ) ) ;
#78079=CARTESIAN_POINT ( 'NONE',  ( 101.3720933679328482, -27.97043537882594322, 25.53562527591096654 ) ) ;
#78084=LINE ( 'NONE', #36738, #35475 ) ;
#78086=CARTESIAN_POINT ( 'NONE',  ( 111.4826097991074079, -46.11499196468592743, 283.9146728949579597 ) ) ;
#78087=PLANE ( 'NONE',  #70468 ) ;
#78088=CARTESIAN_POINT ( 'NONE',  ( 114.2951562036312936, -44.16484043540973659, 114.2022919425769771 ) ) ;
#78090=ORIENTED_EDGE ( 'NONE', *, *, #16458, .F. ) ;
#78092=CARTESIAN_POINT ( 'NONE',  ( 77.96925277058818438, -34.94806367530411251, 2.376725340801996378 ) ) ;
#78093=EDGE_LOOP ( 'NONE', ( #42467, #16981, #34009, #73139 ) ) ;
#78095=CARTESIAN_POINT ( 'NONE',  ( 111.0839405624553251, -29.06298261359865975, 12.49856656006798161 ) ) ;
#78097=VECTOR ( 'NONE', #28189, 1000.000000000000000 ) ;
#78099=CARTESIAN_POINT ( 'NONE',  ( 107.0667039024479834, -36.72944715994100306, 239.5838068554170093 ) ) ;
#78100=EDGE_CURVE ( 'NONE', #67129, #85840, #52670, .T. ) ;
#78104=ORIENTED_EDGE ( 'NONE', *, *, #19410, .F. ) ;
#78105=DIRECTION ( 'NONE',  ( 0.000000000000000000, 1.000000000000000000, 0.000000000000000000 ) ) ;
#78106=VECTOR ( 'NONE', #3795, 1000.000000000000000 ) ;
#78107=EDGE_CURVE ( 'NONE', #22201, #38380, #33893, .T. ) ;
#78108=DIRECTION ( 'NONE',  ( 1.000000000000000000, 4.299999999999999979E-14, 1.000000000000000078E-15 ) ) ;
#78109=ORIENTED_EDGE ( 'NONE', *, *, #73775, .T. ) ;
#78110=CARTESIAN_POINT ( 'NONE',  ( 100.9430784815160251, -28.29197455274081463, 75.57562527591093726 ) ) ;
#78111=B_SPLINE_CURVE_WITH_KNOTS ( 'NONE', 3,
 ( #45777, #4475, #68934, #55715, #34856, #48909, #76647, #69388, #14433, #33951, #42110, #69836, #83034, #68494, #76192, #27596, #75756, #20788 ),
 .UNSPECIFIED., .F., .F.,
 ( 4, 2, 2, 2, 2, 2, 2, 2, 4 ),
 ( 0.000000000000000000, 0.06249999986974735799, 0.1249999997394947160, 0.1874999996092420740, 0.2499999994789894320, 0.3124999993487367900, 0.3749999992184841480, 0.4374999990882315060, 0.4999999989579788640 ),
 .UNSPECIFIED. ) ;
#78113=CARTESIAN_POINT ( 'NONE',  ( 111.8977291718574065, -29.68564172797395528, 44.02099125664899049 ) ) ;
#78115=ADVANCED_FACE ( 'NONE', ( #12116 ), #61391, .T. ) ;
#78116=LINE ( 'NONE', #58527, #66329 ) ;
#78117=CARTESIAN_POINT ( 'NONE',  ( 111.1483613326457913, -47.07112276671761464, 172.8756252759109771 ) ) ;
#78119=FACE_OUTER_BOUND ( 'NONE', #20938, .T. ) ;
#78120=AXIS2_PLACEMENT_3D ( 'NONE', #80658, #11611, #24787 ) ;
#78121=FACE_OUTER_BOUND ( 'NONE', #21814, .T. ) ;
#78124=CARTESIAN_POINT ( 'NONE',  ( 96.51983850151567879, -40.19180362902228865, 282.5908633711491120 ) ) ;
#78129=CARTESIAN_POINT ( 'NONE',  ( 98.24414503606394078, -31.02815815664761345, 141.8699109901969564 ) ) ;
#78130=CARTESIAN_POINT ( 'NONE',  ( 116.3212776292296127, -32.94146857471318413, 287.6356252759109680 ) ) ;
#78133=EDGE_CURVE ( 'NONE', #86269, #66733, #47507, .T. ) ;
#78135=CIRCLE ( 'NONE', #38936, 0.5000000000000004441 ) ;
#78136=FACE_OUTER_BOUND ( 'NONE', #77552, .T. ) ;
#78139=PLANE ( 'NONE',  #78599 ) ;
#78141=CARTESIAN_POINT ( 'NONE',  ( 97.79230575738172604, -40.52535926896634777, 7.635625275910939536 ) ) ;
#78142=ADVANCED_FACE ( 'NONE', ( #74345 ), #32540, .F. ) ;
#78143=DIRECTION ( 'NONE',  ( 0.000000000000000000, 1.000000000000000000, 0.000000000000000000 ) ) ;
#78145=CARTESIAN_POINT ( 'NONE',  ( 108.6169522717627700, -26.81698160835030365, 170.9531425218682159 ) ) ;
#78146=AXIS2_PLACEMENT_3D ( 'NONE', #78231, #44108, #32726 ) ;
#78148=ORIENTED_EDGE ( 'NONE', *, *, #23886, .F. ) ;
#78149=VECTOR ( 'NONE', #27009, 1000.000000000000000 ) ;
#78150=EDGE_CURVE ( 'NONE', #12059, #41030, #88963, .T. ) ;
#78152=CARTESIAN_POINT ( 'NONE',  ( 90.44969454456413871, -53.34645651782494724, 239.5838068554169809 ) ) ;
#78153=DIRECTION ( 'NONE',  ( 1.000000000000000000, 0.000000000000000000, 0.000000000000000000 ) ) ;
#78157=CARTESIAN_POINT ( 'NONE',  ( 113.9904334582008545, -30.89236017996071837, 223.7943245899819829 ) ) ;
#78158=DIRECTION ( 'NONE',  ( 0.000000000000000000, 0.000000000000000000, -1.000000000000000000 ) ) ;
#78159=CARTESIAN_POINT ( 'NONE',  ( 105.9906760191434358, -26.38192068051327510, 46.15848241876796720 ) ) ;
#78161=CARTESIAN_POINT ( 'NONE',  ( 115.2418052506917832, -44.23790868596334747, 78.22324432352995416 ) ) ;
#78163=DIRECTION ( 'NONE',  ( -0.7071067812159675947, -0.7071067811571274397, -7.071067812159669175E-16 ) ) ;
#78164=ORIENTED_EDGE ( 'NONE', *, *, #27687, .F. ) ;
#78165=CARTESIAN_POINT ( 'NONE',  ( 104.4899544225926604, -26.97880759208219104, 66.28145861163227437 ) ) ;
#78166=CARTESIAN_POINT ( 'NONE',  ( 103.2772504383587915, -27.47516629124199383, 276.3857340133070011 ) ) ;
#78167=EDGE_LOOP ( 'NONE', ( #66884, #27031, #24446, #48996 ) ) ;
#78173=EDGE_CURVE ( 'NONE', #36895, #49620, #18471, .T. ) ;
#78174=DIRECTION ( 'NONE',  ( 0.000000000000000000, 0.000000000000000000, -1.000000000000000000 ) ) ;
#78175=VECTOR ( 'NONE', #29573, 1000.000000000000000 ) ;
#78176=DIRECTION ( 'NONE',  ( -1.000000000000000000, 6.036837696399408848E-13, 0.000000000000000000 ) ) ;
#78179=CARTESIAN_POINT ( 'NONE',  ( 117.4695374193713775, -37.69008693337416815, 78.75276813305399060 ) ) ;
#78181=CARTESIAN_POINT ( 'NONE',  ( 97.31309759000943416, -38.96071495204963497, 166.5054468050763603 ) ) ;
#78182=CARTESIAN_POINT ( 'NONE',  ( 152.0368932755772562, -23.42844715993587812, 180.4678068554149775 ) ) ;
#78183=DIRECTION ( 'NONE',  ( 1.000000000000000000, 0.000000000000000000, 0.000000000000000000 ) ) ;
#78184=VERTEX_POINT ( 'NONE', #11212 ) ;
#78185=VECTOR ( 'NONE', #37661, 1000.000000000000000 ) ;
#78186=LINE ( 'NONE', #36828, #31507 ) ;
#78188=CARTESIAN_POINT ( 'NONE',  ( 116.3201495438094923, -32.94088975182634726, 124.1356252759109537 ) ) ;
#78189=ADVANCED_FACE ( 'NONE', ( #6205 ), #87528, .T. ) ;
#78190=AXIS2_PLACEMENT_3D ( 'NONE', #84319, #27979, #76589 ) ;
#78192=CARTESIAN_POINT ( 'NONE',  ( 83.96770390244806492, -18.82844715994099971, 168.9256252759119548 ) ) ;
#78194=ADVANCED_FACE ( 'NONE', ( #5306 ), #87976, .T. ) ;
#78195=VERTEX_POINT ( 'NONE', #81630 ) ;
#78197=CARTESIAN_POINT ( 'NONE',  ( 100.4443968677459935, -27.79860430499269697, 181.5841967044819683 ) ) ;
#78198=VECTOR ( 'NONE', #61238, 1000.000000000000000 ) ;
#78199=DIRECTION ( 'NONE',  ( 1.000000000000000078E-15, 1.000000000000000083E-30, -1.000000000000000000 ) ) ;
#78201=CARTESIAN_POINT ( 'NONE',  ( 105.2810544170623359, -46.37316503544239765, 8.429910990195965681 ) ) ;
#78202=LINE ( 'NONE', #79088, #33866 ) ;
#78204=FACE_OUTER_BOUND ( 'NONE', #8239, .T. ) ;
#78206=CARTESIAN_POINT ( 'NONE',  ( 105.8005514283656225, -26.72389458433680076, 30.17743840264089528 ) ) ;
#78207=CARTESIAN_POINT ( 'NONE',  ( 106.5981863181247462, -46.53222597210214673, 247.5384824187689787 ) ) ;
#78208=ORIENTED_EDGE ( 'NONE', *, *, #27281, .T. ) ;
#78210=VECTOR ( 'NONE', #1444, 1000.000000000000000 ) ;
#78211=CARTESIAN_POINT ( 'NONE',  ( 97.82234778274722942, -32.72736474536957019, 207.4330118773259528 ) ) ;
#78213=CARTESIAN_POINT ( 'NONE',  ( 97.82387236378413320, -38.41783952554947490, 47.91396425827898753 ) ) ;
#78216=EDGE_CURVE ( 'NONE', #56160, #30248, #18025, .T. ) ;
#78217=DIRECTION ( 'NONE',  ( 0.000000000000000000, 0.000000000000000000, -1.000000000000000000 ) ) ;
#78219=VERTEX_POINT ( 'NONE', #32995 ) ;
#78221=EDGE_CURVE ( 'NONE', #38949, #14757, #60693, .T. ) ;
#78222=DIRECTION ( 'NONE',  ( 1.639958061481212836E-42, -4.100000000000000342E-29, -1.000000000000000000 ) ) ;
#78223=CARTESIAN_POINT ( 'NONE',  ( 115.0380569359702463, -30.04493676975920380, 269.3813395616251682 ) ) ;
#78226=VERTEX_POINT ( 'NONE', #19379 ) ;
#78227=VECTOR ( 'NONE', #19601, 1000.000000000000000 ) ;
#78228=EDGE_CURVE ( 'NONE', #87676, #37352, #61153, .T. ) ;
#78231=CARTESIAN_POINT ( 'NONE',  ( 163.0664832912739826, 19.62155284005901024, 333.4006252759110112 ) ) ;
#78233=CARTESIAN_POINT ( 'NONE',  ( 97.69287098190334007, -33.93680905855630670, 27.09562527591097236 ) ) ;
#78234=VECTOR ( 'NONE', #26330, 1000.000000000000000 ) ;
#78235=CARTESIAN_POINT ( 'NONE',  ( 61.67078992371376245, -0.9290567490904538817, 542.9756252759101471 ) ) ;
#78237=EDGE_CURVE ( 'NONE', #47917, #1770, #70158, .T. ) ;
#78238=ORIENTED_EDGE ( 'NONE', *, *, #14013, .T. ) ;
#78239=CARTESIAN_POINT ( 'NONE',  ( 96.13205292066136565, -38.63620640773733328, 42.45181575210199298 ) ) ;
#78240=CARTESIAN_POINT ( 'NONE',  ( 72.06648329127256147, -9.729447159940422196, -4.970821333494543026 ) ) ;
#78241=CARTESIAN_POINT ( 'NONE',  ( 118.5953454549360231, -33.89261193510051839, 14.01848241876796308 ) ) ;
#78243=EDGE_CURVE ( 'NONE', #85401, #6767, #59949, .T. ) ;
#78244=AXIS2_PLACEMENT_3D ( 'NONE', #68717, #40997, #34636 ) ;
#78246=CARTESIAN_POINT ( 'NONE',  ( 82.81648329127399677, -18.72944715994105636, -5.074374724089055100 ) ) ;
#78248=LINE ( 'NONE', #23288, #39334 ) ;
#78249=CARTESIAN_POINT ( 'NONE',  ( 100.2308834438963174, -41.19087078291441628, 99.60523322673398638 ) ) ;
#78250=CARTESIAN_POINT ( 'NONE',  ( 96.16865940696823145, -32.01143006853777706, 207.0013395616249738 ) ) ;
#78253=AXIS2_PLACEMENT_3D ( 'NONE', #39263, #12915, #89668 ) ;
#78257=PLANE ( 'NONE',  #79296 ) ;
#78258=VERTEX_POINT ( 'NONE', #276 ) ;
#78259=ORIENTED_EDGE ( 'NONE', *, *, #85969, .T. ) ;
#78260=DIRECTION ( 'NONE',  ( 0.7071067811865535679, -0.7071067811865415775, 7.071067811865230786E-16 ) ) ;
#78261=CARTESIAN_POINT ( 'NONE',  ( 114.7326334688429483, -30.28293645095888209, 40.38281810511883663 ) ) ;
#78262=AXIS2_PLACEMENT_3D ( 'NONE', #27291, #75896, #13664 ) ;
#78263=CARTESIAN_POINT ( 'NONE',  ( 115.3871705984363984, -41.73312485046139386, 127.8181341137909470 ) ) ;
#78264=CARTESIAN_POINT ( 'NONE',  ( 96.89273651078235616, -34.20293982824353662, 276.1327681330536734 ) ) ;
#78269=FACE_OUTER_BOUND ( 'NONE', #52918, .T. ) ;
#78273=CARTESIAN_POINT ( 'NONE',  ( 113.8852007176727028, -44.67373811025045427, 108.1413395616249744 ) ) ;
#78275=VERTEX_POINT ( 'NONE', #28885 ) ;
#78276=CARTESIAN_POINT ( 'NONE',  ( 100.8483124575627414, -45.14135884264823773, 257.0699109901967745 ) ) ;
#78277=CARTESIAN_POINT ( 'NONE',  ( 61.68306511546570903, -72.55869591834560595, 542.9756252759101471 ) ) ;
#78281=DIRECTION ( 'NONE',  ( 1.175184669632759901E-16, -1.000000000000000000, -2.000000000000003705E-15 ) ) ;
#78282=FACE_OUTER_BOUND ( 'NONE', #8063, .T. ) ;
#78283=CARTESIAN_POINT ( 'NONE',  ( 131.4622572338342934, -37.61690131753618971, 6.952852217895568288 ) ) ;
#78284=VECTOR ( 'NONE', #2570, 1000.000000000000114 ) ;
#78285=DIRECTION ( 'NONE',  ( 1.000000000000000078E-15, 0.000000000000000000, -1.000000000000000000 ) ) ;
#78286=PLANE ( 'NONE',  #73530 ) ;
#78290=CARTESIAN_POINT ( 'NONE',  ( 63.56670390244828184, -47.82844715994016127, 249.9678068554150343 ) ) ;
#78291=CARTESIAN_POINT ( 'NONE',  ( 116.8111099997371554, -31.41389126640522989, 24.21181575210196257 ) ) ;
#78292=CARTESIAN_POINT ( 'NONE',  ( 96.05396905170981370, -35.78154916559406473, 182.2461014663869889 ) ) ;
#78293=CARTESIAN_POINT ( 'NONE',  ( 117.5626006132557535, -36.54510529939036445, 284.8413395616253752 ) ) ;
#78295=DIRECTION ( 'NONE',  ( 0.000000000000000000, 0.000000000000000000, -1.000000000000000000 ) ) ;
#78296=CARTESIAN_POINT ( 'NONE',  ( 101.9935118427002152, -45.44600903161029493, 138.1564489287590334 ) ) ;
#78297=VECTOR ( 'NONE', #56208, 1000.000000000000000 ) ;
#78299=EDGE_CURVE ( 'NONE', #73456, #39861, #69322, .T. ) ;
#78302=ORIENTED_EDGE ( 'NONE', *, *, #88661, .F. ) ;
#78303=CARTESIAN_POINT ( 'NONE',  ( 118.1148702536303290, -35.48641528967803538, 79.91562527591095488 ) ) ;
#78306=ORIENTED_EDGE ( 'NONE', *, *, #6008, .T. ) ;
#78308=CARTESIAN_POINT ( 'NONE',  ( 101.2129617469313132, -45.32973500739954886, 193.1013395616249682 ) ) ;
#78309=LINE ( 'NONE', #71489, #88998 ) ;
#78311=FACE_OUTER_BOUND ( 'NONE', #41962, .T. ) ;
#78312=CARTESIAN_POINT ( 'NONE',  ( 110.8029255159877806, -27.45356875239903971, 85.77192066089217803 ) ) ;
#78313=PLANE ( 'NONE',  #43350 ) ;
#78315=CARTESIAN_POINT ( 'NONE',  ( 99.54941199951403519, -42.98700854487248080, 116.8784824187689679 ) ) ;
#78316=ORIENTED_EDGE ( 'NONE', *, *, #40174, .F. ) ;
#78317=ORIENTED_EDGE ( 'NONE', *, *, #47000, .F. ) ;
#78318=CARTESIAN_POINT ( 'NONE',  ( 99.53176374547611260, -42.34233651421938305, 108.2796785439919773 ) ) ;
#78321=CARTESIAN_POINT ( 'NONE',  ( 117.3624379696766198, -35.49166588079122420, 234.9337205140059552 ) ) ;
#78322=CARTESIAN_POINT ( 'NONE',  ( 73.06670390244801183, -58.72944715994110254, 250.9178068554160461 ) ) ;
#78324=CARTESIAN_POINT ( 'NONE',  ( 97.07206919424615421, -35.37846131109193948, 112.2194697797737462 ) ) ;
#78326=AXIS2_PLACEMENT_3D ( 'NONE', #34782, #82957, #62487 ) ;
#78330=CARTESIAN_POINT ( 'NONE',  ( 97.81219835445369881, -40.51719899421586746, 151.6362400511890769 ) ) ;
#78331=CARTESIAN_POINT ( 'NONE',  ( 108.7397100058831541, -25.82697924850565840, 144.9432443235299672 ) ) ;
#78333=EDGE_CURVE ( 'NONE', #29833, #23923, #21177, .T. ) ;
#78335=VERTEX_POINT ( 'NONE', #48846 ) ;
#78338=CARTESIAN_POINT ( 'NONE',  ( 51.03742451361318189, -23.42844715994068849, 117.4678068554150485 ) ) ;
#78339=CARTESIAN_POINT ( 'NONE',  ( 105.7980258636739279, -26.72423388751797546, 130.1774127513859867 ) ) ;
#78340=CARTESIAN_POINT ( 'NONE',  ( 99.50448107662171537, -43.30550302426849640, 102.8959900338089994 ) ) ;
#78341=CARTESIAN_POINT ( 'NONE',  ( 105.5353399150147737, -28.71163411781831698, 233.0452332267339841 ) ) ;
#78342=VECTOR ( 'NONE', #20557, 1000.000000000000114 ) ;
#78343=CYLINDRICAL_SURFACE ( 'NONE', #88633, 2.500000000000002220 ) ;
#78344=CARTESIAN_POINT ( 'NONE',  ( 108.2778356434855027, -47.71639565607667066, 157.6518157521019532 ) ) ;
#78345=DIRECTION ( 'NONE',  ( 0.000000000000000000, 0.000000000000000000, -1.000000000000000000 ) ) ;
#78346=ORIENTED_EDGE ( 'NONE', *, *, #51122, .T. ) ;
#78349=EDGE_CURVE ( 'NONE', #67882, #88995, #57051, .T. ) ;
#78350=CIRCLE ( 'NONE', #68140, 2.030000000001311644 ) ;
#78351=DIRECTION ( 'NONE',  ( 1.000000000000000000, 4.299999999999999979E-14, 1.000000000000000078E-15 ) ) ;
#78352=VERTEX_POINT ( 'NONE', #27530 ) ;
#78354=CARTESIAN_POINT ( 'NONE',  ( 116.3263622980238097, -32.93962144782776846, 195.1356252759109680 ) ) ;
#78355=DIRECTION ( 'NONE',  ( 0.7071067811862279395, -0.7071067811868672059, 7.071067811862286363E-16 ) ) ;
#78356=CARTESIAN_POINT ( 'NONE',  ( 115.1162204959661466, -41.57488383322457537, 274.8149166392303755 ) ) ;
#78360=CARTESIAN_POINT ( 'NONE',  ( 114.9151178457587577, -41.28570029556458820, 9.635625275910941312 ) ) ;
#78361=DIRECTION ( 'NONE',  ( 0.000000000000000000, 0.000000000000000000, -1.000000000000000000 ) ) ;
#78363=VECTOR ( 'NONE', #86181, 1000.000000000000000 ) ;
#78364=ORIENTED_EDGE ( 'NONE', *, *, #18313, .F. ) ;
#78365=CARTESIAN_POINT ( 'NONE',  ( 105.7155658375387333, -46.72387182276721518, 112.4690335037959557 ) ) ;
#78366=ORIENTED_EDGE ( 'NONE', *, *, #44750, .F. ) ;
#78368=CARTESIAN_POINT ( 'NONE',  ( 99.98530978427844218, -41.10337153935440568, 11.19051506617196878 ) ) ;
#78370=CARTESIAN_POINT ( 'NONE',  ( 108.2803926554762626, -47.73958771823362213, 157.6518157521019532 ) ) ;
#78371=CARTESIAN_POINT ( 'NONE',  ( 96.72090476913461998, -37.82382852467500811, 126.4099109901969626 ) ) ;
#78372=DIRECTION ( 'NONE',  ( 0.000000000000000000, 0.000000000000000000, 1.000000000000000000 ) ) ;
#78374=CARTESIAN_POINT ( 'NONE',  ( 117.7763469108053869, -31.65663365956905650, 210.1784824187679703 ) ) ;
#78375=FACE_OUTER_BOUND ( 'NONE', #8480, .T. ) ;
#78377=ORIENTED_EDGE ( 'NONE', *, *, #53976, .F. ) ;
#78383=CARTESIAN_POINT ( 'NONE',  ( 117.3348906646497909, -34.51323323996641079, 183.9956252759109532 ) ) ;
#78385=CARTESIAN_POINT ( 'NONE',  ( 101.9719236373881444, -46.53885842731235556, 167.1832443235299763 ) ) ;
#78388=DIRECTION ( 'NONE',  ( 1.000000000000000000, 4.299999999999999979E-14, 9.351236661543306751E-17 ) ) ;
#78389=CARTESIAN_POINT ( 'NONE',  ( 172.5667039024480687, -36.32844715993499563, 129.9678068554150059 ) ) ;
#78391=CARTESIAN_POINT ( 'NONE',  ( 98.46045456725896372, -41.84421156295625366, 56.75289356703274990 ) ) ;
#78392=CARTESIAN_POINT ( 'NONE',  ( 109.9831304889622743, -26.74336511273928707, 255.8499109901966051 ) ) ;
#78393=CARTESIAN_POINT ( 'NONE',  ( 51.06648329127400388, 19.62155284005901024, 333.4006252759110112 ) ) ;
#78396=CARTESIAN_POINT ( 'NONE',  ( 25.56670390244797275, -48.82844715994099971, 290.4678068554150627 ) ) ;
#78398=DIRECTION ( 'NONE',  ( -0.9999999853157766072, -0.0001713722456127401463, 9.999999853157767620E-16 ) ) ;
#78399=DIRECTION ( 'NONE',  ( 0.7071067811865614505, -0.7071067811865336949, 0.000000000000000000 ) ) ;
#78400=CARTESIAN_POINT ( 'NONE',  ( 98.90717908043868078, -38.42765120644578047, 195.5838068554173788 ) ) ;
#78402=DIRECTION ( 'NONE',  ( 0.000000000000000000, 0.000000000000000000, -1.000000000000000000 ) ) ;
#78403=CARTESIAN_POINT ( 'NONE',  ( 112.7922847239315161, -45.46795744031502551, 178.0384824187679556 ) ) ;
#78404=CARTESIAN_POINT ( 'NONE',  ( 96.92116189526866776, -32.34237133930066221, 57.01372051400599616 ) ) ;
#78405=CARTESIAN_POINT ( 'NONE',  ( 99.97865438147567829, -27.17048309217152990, 181.5841967044829630 ) ) ;
#78407=LINE ( 'NONE', #86550, #61965 ) ;
#78410=DIRECTION ( 'NONE',  ( 0.000000000000000000, 0.000000000000000000, -1.000000000000000000 ) ) ;
#78411=PLANE ( 'NONE',  #85841 ) ;
#78412=DIRECTION ( 'NONE',  ( 0.000000000000000000, 0.000000000000000000, 1.000000000000000000 ) ) ;
#78414=DIRECTION ( 'NONE',  ( 1.000000000000000078E-15, 1.000000000000000083E-30, -1.000000000000000000 ) ) ;
#78418=CARTESIAN_POINT ( 'NONE',  ( 108.6382307137633205, -45.64809506003439310, 122.1257531614099747 ) ) ;
#78419=CIRCLE ( 'NONE', #56596, 2.029999999999997140 ) ;
#78421=VERTEX_POINT ( 'NONE', #7985 ) ;
#78422=CARTESIAN_POINT ( 'NONE',  ( 98.22092589535434115, -43.31882777834836418, 107.8480062282919647 ) ) ;
#78423=CARTESIAN_POINT ( 'NONE',  ( 107.0664832912739968, -0.2185775633790978945, 333.4006252759120343 ) ) ;
#78425=CARTESIAN_POINT ( 'NONE',  ( 20.03715912545824906, -46.82818131006190043, 249.9678068554150059 ) ) ;
#78426=EDGE_CURVE ( 'NONE', #40553, #6056, #9215, .T. ) ;
#78427=CARTESIAN_POINT ( 'NONE',  ( 105.7995185030575982, -26.72403496415040891, 176.1772919413423040 ) ) ;
#78428=CARTESIAN_POINT ( 'NONE',  ( 95.98894198207682393, -35.78073158428679790, 36.25848241876794731 ) ) ;
#78429=ORIENTED_EDGE ( 'NONE', *, *, #22105, .T. ) ;
#78431=CIRCLE ( 'NONE', #31961, 2.030000000001807248 ) ;
#78434=PLANE ( 'NONE',  #49211 ) ;
#78437=CYLINDRICAL_SURFACE ( 'NONE', #62083, 1.000000000000000888 ) ;
#78438=CARTESIAN_POINT ( 'NONE',  ( 97.60783471073349915, -39.98226673208375104, 52.58976314850144718 ) ) ;
#78442=CARTESIAN_POINT ( 'NONE',  ( 118.7081646409642133, -34.65111545711807395, 48.96705384733895983 ) ) ;
#78443=EDGE_CURVE ( 'NONE', #81124, #14889, #42932, .T. ) ;
#78444=ORIENTED_EDGE ( 'NONE', *, *, #31412, .F. ) ;
#78445=CARTESIAN_POINT ( 'NONE',  ( 99.09570968012857861, -30.55043098681969838, 270.8022918655054241 ) ) ;
#78448=CARTESIAN_POINT ( 'NONE',  ( 102.8475555715194361, -29.17288882023929730, 103.3118998934009767 ) ) ;
#78449=DIRECTION ( 'NONE',  ( 0.000000000000000000, 1.000000000000000000, 0.000000000000000000 ) ) ;
#78450=VECTOR ( 'NONE', #63360, 1000.000000000000000 ) ;
#78452=ORIENTED_EDGE ( 'NONE', *, *, #46305, .T. ) ;
#78453=EDGE_LOOP ( 'NONE', ( #86833, #45040, #23455, #30802 ) ) ;
#78454=ADVANCED_FACE ( 'NONE', ( #70669 ), #28061, .F. ) ;
#78456=VECTOR ( 'NONE', #60034, 1000.000000000000000 ) ;
#78458=VERTEX_POINT ( 'NONE', #29338 ) ;
#78459=EDGE_CURVE ( 'NONE', #34522, #36080, #52920, .T. ) ;
#78460=CARTESIAN_POINT ( 'NONE',  ( 97.69936372639945432, -35.99897019620807725, 187.7082499725639764 ) ) ;
#78463=CARTESIAN_POINT ( 'NONE',  ( 117.8789659794968543, -39.13265831612300616, 99.64038718067195077 ) ) ;
#78465=CARTESIAN_POINT ( 'NONE',  ( 97.81168921572486852, -40.51740600946125426, 16.63579259794490284 ) ) ;
#78467=ORIENTED_EDGE ( 'NONE', *, *, #33692, .F. ) ;
#78468=VERTEX_POINT ( 'NONE', #71572 ) ;
#78469=CARTESIAN_POINT ( 'NONE',  ( 108.0840670587429599, -45.32394831497818899, 160.5004713219719861 ) ) ;
#78470=CARTESIAN_POINT ( 'NONE',  ( 99.27722696178533113, -43.74484797918319856, 56.90991099019593236 ) ) ;
#78471=VERTEX_POINT ( 'NONE', #78396 ) ;
#78472=CARTESIAN_POINT ( 'NONE',  ( 107.6057229598026339, -48.54288983744056907, 42.61276813305398292 ) ) ;
#78473=CARTESIAN_POINT ( 'NONE',  ( 103.0413726597163446, -26.41035368485499646, 166.3603871806729444 ) ) ;
#78476=CARTESIAN_POINT ( 'NONE',  ( 99.68461964852595258, -45.99997598619422234, 118.0413395616259606 ) ) ;
#78477=AXIS2_PLACEMENT_3D ( 'NONE', #73823, #60173, #87907 ) ;
#78478=PLANE ( 'NONE',  #37885 ) ;
#78479=VERTEX_POINT ( 'NONE', #16596 ) ;
#78483=CARTESIAN_POINT ( 'NONE',  ( 115.7836371542223901, -41.80142107029080734, 134.4074412807795795 ) ) ;
#78486=AXIS2_PLACEMENT_3D ( 'NONE', #29445, #22643, #50314 ) ;
#78488=LINE ( 'NONE', #43474, #84186 ) ;
#78489=CARTESIAN_POINT ( 'NONE',  ( 113.5062182464826748, -28.53085922249196216, 79.54705384733995288 ) ) ;
#78491=B_SPLINE_CURVE_WITH_KNOTS ( 'NONE', 3,
 ( #46311, #67676, #74040, #81769, #11822, #67219, #5002, #83554, #28112, #14054, #47661, #69021, #41736, #34935, #42190, #82670, #14513, #422, #19979, #6786, #872, #20869, #7687, #75394, #48991, #54461, #14962, #69922, #62648, #28569, #13165, #13606, #34030, #89469, #40849, #34485, #62196, #68579, #48099, #61735, #1330, #20429, #6342, #55798, #89930, #27228, #27681, #75832, #63089, #35377 ),
 .UNSPECIFIED., .F., .F.,
 ( 4, 2, 1, 1, 1, 1, 1, 2, 2, 2, 2, 2, 2, 2, 1, 1, 1, 1, 1, 1, 1, 2, 2, 2, 2, 2, 2, 2, 2, 2, 4 ),
 ( 0.5000148422006782667, 0.5002589755784957459, 0.5005031089563133362, 0.5009913757119484057, 0.5019679092232189888, 0.5039209762457607100, 0.5078271102908441526, 0.5156393783810113707, 0.5312639145613456959, 0.5625129869220144574, 0.6250111316433523134, 0.6875092763646900584, 0.7500074210860279145, 0.7500684544304828671, 0.7501294877749378198, 0.7502515544638449496, 0.7504956878416844113, 0.7509839545973868713, 0.7519604881087729176, 0.7539135551315454542, 0.7578196891770798693, 0.7656319572681415941, 0.7812564934502654879, 0.8125055658145132753, 0.8437546381787610628, 0.8750037105430088502, 0.9062527829072566377, 0.9375018552715044251, 0.9687509276357521015, 0.9843754638178759953, 1.000000000000000000 ),
 .UNSPECIFIED. ) ;
#78494=DIRECTION ( 'NONE',  ( -1.000000000000000000, 1.122464679914735423E-15, 0.000000000000000000 ) ) ;
#78495=CARTESIAN_POINT ( 'NONE',  ( 106.6352542858682284, -26.36832623700835398, 40.09753003781596448 ) ) ;
#78496=CARTESIAN_POINT ( 'NONE',  ( 41.56648329127499153, -36.32844715994070839, 78.92562527591199739 ) ) ;
#78497=CARTESIAN_POINT ( 'NONE',  ( 96.62907006607247240, -36.88702529232762828, 132.3384824187679669 ) ) ;
#78498=DIRECTION ( 'NONE',  ( -1.000000000000000000, 0.000000000000000000, -7.723290606088049820E-15 ) ) ;
#78499=CARTESIAN_POINT ( 'NONE',  ( 164.9190312289447888, -35.91149509760580116, 237.4678068554150059 ) ) ;
#78502=DIRECTION ( 'NONE',  ( -4.299999999999999979E-14, 1.000000000000000000, -4.400000000000000367E-29 ) ) ;
#78504=VERTEX_POINT ( 'NONE', #66060 ) ;
#78505=AXIS2_PLACEMENT_3D ( 'NONE', #64512, #13332, #21843 ) ;
#78506=FACE_OUTER_BOUND ( 'NONE', #4595, .T. ) ;
#78507=CARTESIAN_POINT ( 'NONE',  ( 117.8217860357262481, -31.63511105064214490, 214.1784824187679419 ) ) ;
#78508=EDGE_LOOP ( 'NONE', ( #88737, #27161, #29908 ) ) ;
#78509=FACE_OUTER_BOUND ( 'NONE', #81787, .T. ) ;
#78510=CARTESIAN_POINT ( 'NONE',  ( 106.5662934289835988, -47.19983425457502335, 243.5384824187679556 ) ) ;
#78511=CARTESIAN_POINT ( 'NONE',  ( 97.18453276023305420, -31.67528530451021851, 91.96229194257693962 ) ) ;
#78513=DIRECTION ( 'NONE',  ( -0.9254794337955620787, -0.3787978585227822492, 0.000000000000000000 ) ) ;
#78514=CARTESIAN_POINT ( 'NONE',  ( 115.0372575094445295, -42.90846256270808823, 78.30229194297042739 ) ) ;
#78515=EDGE_LOOP ( 'NONE', ( #26157, #32578, #59924, #24241 ) ) ;
#78519=EDGE_CURVE ( 'NONE', #60004, #67149, #85212, .T. ) ;
#78520=AXIS2_PLACEMENT_3D ( 'NONE', #64541, #85006, #22773 ) ;
#78521=ORIENTED_EDGE ( 'NONE', *, *, #54565, .T. ) ;
#78523=CARTESIAN_POINT ( 'NONE',  ( 111.8640475646460857, -46.02486053542493494, 268.9556252759110180 ) ) ;
#78524=CARTESIAN_POINT ( 'NONE',  ( 194.0371591254575492, -24.42818131005417115, 129.9678068554150343 ) ) ;
#78526=EDGE_CURVE ( 'NONE', #35491, #39283, #37035, .T. ) ;
#78528=PLANE ( 'NONE',  #350 ) ;
#78530=DIRECTION ( 'NONE',  ( 0.000000000000000000, 0.000000000000000000, -1.000000000000000000 ) ) ;
#78532=CARTESIAN_POINT ( 'NONE',  ( 111.9487353400944158, -44.35678517904902662, 217.4400388756959615 ) ) ;
#78533=ORIENTED_EDGE ( 'NONE', *, *, #49361, .T. ) ;
#78535=EDGE_LOOP ( 'NONE', ( #82545, #12098 ) ) ;
#78537=AXIS2_PLACEMENT_3D ( 'NONE', #5502, #73176, #10516 ) ;
#78538=DIRECTION ( 'NONE',  ( -4.237773401492740281E-14, 1.000000000000000000, 0.000000000000000000 ) ) ;
#78539=CARTESIAN_POINT ( 'NONE',  ( 109.6427193709274519, -46.48016071713966113, 182.7814590059388138 ) ) ;
#78540=ADVANCED_FACE ( 'NONE', ( #23862 ), #51970, .T. ) ;
#78541=CARTESIAN_POINT ( 'NONE',  ( 98.14754276252335785, -43.36755551587071977, 257.8356252759109566 ) ) ;
#78543=CARTESIAN_POINT ( 'NONE',  ( 97.25364341294459791, -36.87759583893578963, 132.3384824187679669 ) ) ;
#78544=ADVANCED_FACE ( 'NONE', ( #86539 ), #24304, .F. ) ;
#78545=DIRECTION ( 'NONE',  ( -0.9254794337955620787, -0.3787978585227822492, 0.000000000000000000 ) ) ;
#78547=ORIENTED_EDGE ( 'NONE', *, *, #62008, .F. ) ;
#78549=CYLINDRICAL_SURFACE ( 'NONE', #7100, 11.57110091390434903 ) ;
#78550=VERTEX_POINT ( 'NONE', #17483 ) ;
#78552=CARTESIAN_POINT ( 'NONE',  ( 97.82153671710952381, -35.93768077729445309, 34.07666179816293095 ) ) ;
#78554=CARTESIAN_POINT ( 'NONE',  ( 123.6837132603318423, -17.59493780205705704, 239.5838068554170377 ) ) ;
#78555=LINE ( 'NONE', #79442, #4109 ) ;
#78557=CARTESIAN_POINT ( 'NONE',  ( 115.7830320273964304, -41.80243732865377382, 194.4064425540411776 ) ) ;
#78559=DIRECTION ( 'NONE',  ( -0.7071067811865475727, 0.7071067811865475727, 0.000000000000000000 ) ) ;
#78561=DIRECTION ( 'NONE',  ( 1.000000000000000078E-15, -1.000000000000000083E-30, -1.000000000000000000 ) ) ;
#78563=CARTESIAN_POINT ( 'NONE',  ( 113.4596546395850680, -46.70781606211470205, 68.02991099019695298 ) ) ;
#78566=CARTESIAN_POINT ( 'NONE',  ( 116.0925701722734686, -37.46594287791281630, 38.19622935188693447 ) ) ;
#78570=CARTESIAN_POINT ( 'NONE',  ( 114.8570798905637673, -32.50631050113013742, 65.65301187732598009 ) ) ;
#78571=DIRECTION ( 'NONE',  ( 0.000000000000000000, 1.000000000000000000, 0.000000000000000000 ) ) ;
#78573=EDGE_CURVE ( 'NONE', #23208, #43944, #32427, .T. ) ;
#78575=CARTESIAN_POINT ( 'NONE',  ( 110.9086127847465377, -26.95314644129561543, 265.7784824187680783 ) ) ;
#78577=ORIENTED_EDGE ( 'NONE', *, *, #971, .T. ) ;
#78578=DIRECTION ( 'NONE',  ( 0.000000000000000000, 0.000000000000000000, 1.000000000000000000 ) ) ;
#78579=ORIENTED_EDGE ( 'NONE', *, *, #2118, .T. ) ;
#78580=CARTESIAN_POINT ( 'NONE',  ( 102.8960693947464051, -27.08911147246314499, 151.4013395616249511 ) ) ;
#78583=ORIENTED_EDGE ( 'NONE', *, *, #1527, .F. ) ;
#78584=ORIENTED_EDGE ( 'NONE', *, *, #8262, .F. ) ;
#78587=PLANE ( 'NONE',  #15925 ) ;
#78588=CARTESIAN_POINT ( 'NONE',  ( 118.0655259830059265, -38.35211242607485360, 223.7099109901979546 ) ) ;
#78589=CARTESIAN_POINT ( 'NONE',  ( 94.86917197795301604, -31.06128196069623471, 9.425625275910958223 ) ) ;
#78590=CARTESIAN_POINT ( 'NONE',  ( 107.0664832912739968, 0.2215528400590083269, 333.4006252759110112 ) ) ;
#78592=CARTESIAN_POINT ( 'NONE',  ( 116.1583077856502086, -43.02023234939740348, 9.356577656862985037 ) ) ;
#78594=VERTEX_POINT ( 'NONE', #11567 ) ;
#78595=CARTESIAN_POINT ( 'NONE',  ( 105.9988973700097574, -26.77423969884217669, 171.1614530458196271 ) ) ;
#78597=AXIS2_PLACEMENT_3D ( 'NONE', #35912, #22757, #9560 ) ;
#78598=ORIENTED_EDGE ( 'NONE', *, *, #1624, .F. ) ;
#78599=AXIS2_PLACEMENT_3D ( 'NONE', #33085, #74427, #66707 ) ;
#78600=CARTESIAN_POINT ( 'NONE',  ( 82.72805595269750256, -19.42731094490102706, 2.974216770161542289 ) ) ;
#78602=CARTESIAN_POINT ( 'NONE',  ( 117.3910620576583312, -35.19077923515891371, 218.9441967044829482 ) ) ;
#78604=FACE_BOUND ( 'NONE', #7159, .T. ) ;
#78606=CARTESIAN_POINT ( 'NONE',  ( 109.5125757112413822, -28.00996883845181173, 219.2933722090289734 ) ) ;
#78608=CARTESIAN_POINT ( 'NONE',  ( 99.99555918775628527, -44.36035129061379934, 42.98133956162492098 ) ) ;
#78609=DIRECTION ( 'NONE',  ( -8.252657816380299978E-16, -2.773339119917620066E-31, -1.000000000000000000 ) ) ;
#78610=CARTESIAN_POINT ( 'NONE',  ( 109.2642598482130154, -47.00181652296804913, 107.7441967044829880 ) ) ;
#78612=CARTESIAN_POINT ( 'NONE',  ( 131.7606268095719031, -20.22815166919999896, 7.286367513304471188 ) ) ;
#78614=DIRECTION ( 'NONE',  ( 1.000000000000000078E-15, -1.000000000000000000, 0.000000000000000000 ) ) ;
#78615=CARTESIAN_POINT ( 'NONE',  ( 116.3185006702053244, -32.93849971620830530, 275.1356252759109680 ) ) ;
#78617=VECTOR ( 'NONE', #73487, 1000.000000000000000 ) ;
#78618=DIRECTION ( 'NONE',  ( 0.000000000000000000, 0.000000000000000000, 1.000000000000000000 ) ) ;
#78619=ORIENTED_EDGE ( 'NONE', *, *, #27446, .F. ) ;
#78621=DIRECTION ( 'NONE',  ( 0.000000000000000000, 0.000000000000000000, -1.000000000000000000 ) ) ;
#78623=CARTESIAN_POINT ( 'NONE',  ( 29.56670390244743629, -48.82844715994161078, 180.4678068554150911 ) ) ;
#78625=VECTOR ( 'NONE', #4189, 1000.000000000000000 ) ;
#78626=CARTESIAN_POINT ( 'NONE',  ( 109.6894323871380976, -47.49121184687970754, 87.75467289495897205 ) ) ;
#78630=CYLINDRICAL_SURFACE ( 'NONE', #225, 2.750000000000002665 ) ;
#78631=EDGE_CURVE ( 'NONE', #57079, #85514, #75126, .T. ) ;
#78633=ORIENTED_EDGE ( 'NONE', *, *, #20083, .T. ) ;
#78634=VECTOR ( 'NONE', #76234, 1000.000000000000000 ) ;
#78635=EDGE_CURVE ( 'NONE', #83511, #397, #45596, .T. ) ;
#78637=CARTESIAN_POINT ( 'NONE',  ( 85.58420390244802434, -43.72944715994107412, 207.5838068554169809 ) ) ;
#78638=AXIS2_PLACEMENT_3D ( 'NONE', #66510, #31989, #72885 ) ;
#78640=EDGE_CURVE ( 'NONE', #49287, #88413, #59685, .T. ) ;
#78641=EDGE_CURVE ( 'NONE', #2091, #70138, #54199, .T. ) ;
#78642=CARTESIAN_POINT ( 'NONE',  ( 142.0664832912739826, -9.729447159940995959, 14.67562527591100441 ) ) ;
#78643=LINE ( 'NONE', #46297, #29725 ) ;
#78644=CARTESIAN_POINT ( 'NONE',  ( 194.0667039024479834, -40.32844715993407902, 300.4678068554149490 ) ) ;
#78646=EDGE_LOOP ( 'NONE', ( #76235, #62227, #58509, #8610 ) ) ;
#78647=( BOUNDED_CURVE ( )  B_SPLINE_CURVE ( 3, ( #63108, #89485, #84020, #71290 ),
 .UNSPECIFIED., .F., .T. ) 
 B_SPLINE_CURVE_WITH_KNOTS ( ( 4, 4 ),
 ( 3.141592653599576401, 4.712388980396665872 ),
 .UNSPECIFIED. ) 
 CURVE ( )  GEOMETRIC_REPRESENTATION_ITEM ( )  RATIONAL_B_SPLINE_CURVE ( ( 1.000000000000000000, 0.8047378541238481287, 0.8047378541238481287, 1.000000000000000000 ) ) 
 REPRESENTATION_ITEM ( '' )  );
#78649=EDGE_CURVE ( 'NONE', #8827, #58352, #74677, .T. ) ;
#78650=CARTESIAN_POINT ( 'NONE',  ( 103.1049807579881588, -45.67203811392940338, 173.2441967044819648 ) ) ;
#78652=ORIENTED_EDGE ( 'NONE', *, *, #55199, .F. ) ;
#78653=CARTESIAN_POINT ( 'NONE',  ( 100.9534786964906345, -28.35269599622561643, 26.56610146638693948 ) ) ;
#78654=DIRECTION ( 'NONE',  ( 0.000000000000000000, 0.000000000000000000, 1.000000000000000000 ) ) ;
#78655=CARTESIAN_POINT ( 'NONE',  ( 97.81556188947165253, -40.52687520453045522, 51.63643775176898032 ) ) ;
#78656=DIRECTION ( 'NONE',  ( 0.000000000000000000, 0.000000000000000000, -1.000000000000000000 ) ) ;
#78657=EDGE_CURVE ( 'NONE', #30791, #84622, #25178, .T. ) ;
#78659=CARTESIAN_POINT ( 'NONE',  ( 101.0349934672010903, -27.38958028709080139, 220.5327681330539633 ) ) ;
#78663=EDGE_CURVE ( 'NONE', #35463, #2140, #80171, .T. ) ;
#78664=CARTESIAN_POINT ( 'NONE',  ( 98.29135092237498839, -35.49440443996801520, 177.6472975916109647 ) ) ;
#78666=B_SPLINE_CURVE_WITH_KNOTS ( 'NONE', 3,
 ( #36581, #43813, #23410, #37462, #86515, #71553, #72433, #29761, #64284, #72868, #86072, #9315, #58775, #80148, #59227, #65608, #24284, #24721 ),
 .UNSPECIFIED., .F., .F.,
 ( 4, 2, 2, 2, 2, 2, 2, 2, 4 ),
 ( 0.000000000000000000, 0.06249238452393977850, 0.1249847690478795570, 0.1874771535718193216, 0.2499695380957591140, 0.3124619226196989064, 0.3749543071436386432, 0.4374466916675784356, 0.4999390761915182280 ),
 .UNSPECIFIED. ) ;
#78668=CARTESIAN_POINT ( 'NONE',  ( 116.4309197881342612, -37.49355097060504249, 35.20539282970796791 ) ) ;
#78670=DIRECTION ( 'NONE',  ( 1.000000000000000078E-15, -1.000000000000000083E-30, -1.000000000000000000 ) ) ;
#78671=CARTESIAN_POINT ( 'NONE',  ( 61.56670390244639890, -23.42844715994043270, 129.9678068554150911 ) ) ;
#78673=LINE ( 'NONE', #15535, #33374 ) ;
#78675=CARTESIAN_POINT ( 'NONE',  ( 97.57986484199619781, -43.79006170206860560, 261.8356252759109566 ) ) ;
#78677=EDGE_LOOP ( 'NONE', ( #9467, #38327, #70440, #7219 ) ) ;
#78679=EDGE_CURVE ( 'NONE', #22201, #64265, #53753, .T. ) ;
#78680=CARTESIAN_POINT ( 'NONE',  ( 97.81169409577289287, -40.51741657705139232, 81.63570706759205109 ) ) ;
#78681=LINE ( 'NONE', #31828, #57787 ) ;
#78683=CARTESIAN_POINT ( 'NONE',  ( 179.1667039024460166, -26.71338133339251542, 117.4678068554150627 ) ) ;
#78686=CARTESIAN_POINT ( 'NONE',  ( 106.3024736416176950, -26.94527301088420046, 21.13848241876792144 ) ) ;
#78688=ORIENTED_EDGE ( 'NONE', *, *, #73563, .T. ) ;
#78689=AXIS2_PLACEMENT_3D ( 'NONE', #32517, #75221, #47033 ) ;
#78690=CARTESIAN_POINT ( 'NONE',  ( 96.67145939589113368, -37.96898657530446997, 37.42133956162496844 ) ) ;
#78691=CARTESIAN_POINT ( 'NONE',  ( 85.58420390244803855, -51.22944715994107412, 231.5838068554169524 ) ) ;
#78692=CARTESIAN_POINT ( 'NONE',  ( 100.0239399080498544, -28.99471651683304785, 285.6641967044823787 ) ) ;
#78693=EDGE_LOOP ( 'NONE', ( #6391, #21175, #47713, #24171 ) ) ;
#78694=CARTESIAN_POINT ( 'NONE',  ( 97.81168895331838087, -40.51742574516882200, 287.6356252759109680 ) ) ;
#78695=CARTESIAN_POINT ( 'NONE',  ( 97.86658600797379393, -40.64924548183623898, 17.64667790301706063 ) ) ;
#78697=CARTESIAN_POINT ( 'NONE',  ( 99.02147155855831784, -38.11057432192225747, 89.27951894101998676 ) ) ;
#78698=CARTESIAN_POINT ( 'NONE',  ( 103.5350399278988078, -26.85989278392735002, 186.3499109901969746 ) ) ;
#78699=DIRECTION ( 'NONE',  ( 0.000000000000000000, 1.000000000000000000, 0.000000000000000000 ) ) ;
#78700=ORIENTED_EDGE ( 'NONE', *, *, #67919, .T. ) ;
#78701=DIRECTION ( 'NONE',  ( 0.000000000000000000, 0.000000000000000000, 1.000000000000000000 ) ) ;
#78702=ORIENTED_EDGE ( 'NONE', *, *, #4149, .F. ) ;
#78705=FACE_BOUND ( 'NONE', #57378, .T. ) ;
#78706=ORIENTED_EDGE ( 'NONE', *, *, #66281, .T. ) ;
#78707=VERTEX_POINT ( 'NONE', #39696 ) ;
#78709=CARTESIAN_POINT ( 'NONE',  ( 115.1037186944613921, -30.74792710411506391, 40.33566342910106783 ) ) ;
#78710=CARTESIAN_POINT ( 'NONE',  ( 99.62716111080935377, -40.92618603589043147, 136.1581341137909646 ) ) ;
#78711=CARTESIAN_POINT ( 'NONE',  ( 116.2381414160656874, -41.80576965393662903, 263.4241967044824833 ) ) ;
#78714=ORIENTED_EDGE ( 'NONE', *, *, #21605, .F. ) ;
#78715=CARTESIAN_POINT ( 'NONE',  ( 105.9338276561856560, -26.78157160042634644, 136.1666567892166881 ) ) ;
#78716=ORIENTED_EDGE ( 'NONE', *, *, #14198, .F. ) ;
#78717=CARTESIAN_POINT ( 'NONE',  ( 83.06670390244796920, -58.35344715994099829, 204.3338068554149913 ) ) ;
#78718=DIRECTION ( 'NONE',  ( -0.000000000000000000, 1.000000000000000000, 0.000000000000000000 ) ) ;
#78719=PLANE ( 'NONE',  #64989 ) ;
#78720=EDGE_CURVE ( 'NONE', #75399, #60225, #67401, .T. ) ;
#78721=CARTESIAN_POINT ( 'NONE',  ( 116.1780915764957740, -31.53023347274874055, 289.2384824187680579 ) ) ;
#78723=CARTESIAN_POINT ( 'NONE',  ( 97.01631923850186467, -33.95794342121210718, 251.1127681330538337 ) ) ;
#78724=CARTESIAN_POINT ( 'NONE',  ( 97.44667640776515327, -32.59970075057101724, 12.00419670448293985 ) ) ;
#78725=CARTESIAN_POINT ( 'NONE',  ( 115.7831076684064300, -41.80230951324009681, 119.4064586089808699 ) ) ;
#78727=CARTESIAN_POINT ( 'NONE',  ( 165.6738106836030227, -28.98061976758901892, -5.074374724088000832 ) ) ;
#78730=ADVANCED_FACE ( 'NONE', ( #81520 ), #19273, .T. ) ;
#78732=DIRECTION ( 'NONE',  ( 1.000000000000000000, 0.000000000000000000, 0.000000000000000000 ) ) ;
#78734=DIRECTION ( 'NONE',  ( -4.237773401492740281E-14, 1.000000000000000000, 0.000000000000000000 ) ) ;
#78736=AXIS2_PLACEMENT_3D ( 'NONE', #85599, #23378, #78783 ) ;
#78738=CARTESIAN_POINT ( 'NONE',  ( 172.5664832912740110, -9.303447159940999356, 76.80862527591200717 ) ) ;
#78739=CARTESIAN_POINT ( 'NONE',  ( 117.5411534933602837, -36.54545762053501079, 288.8413395616251478 ) ) ;
#78740=CARTESIAN_POINT ( 'NONE',  ( 103.0497676667862947, -26.43187579209836002, 166.3603871806729444 ) ) ;
#78741=CARTESIAN_POINT ( 'NONE',  ( 110.2908372810403819, -46.66631795110420455, 8.827053847339950465 ) ) ;
#78742=DIRECTION ( 'NONE',  ( 1.000000000000000000, 4.299999999999999979E-14, 1.000000000000000078E-15 ) ) ;
#78744=DIRECTION ( 'NONE',  ( 1.000000000000000000, 0.000000000000000000, 9.462128050782575008E-16 ) ) ;
#78745=EDGE_CURVE ( 'NONE', #18287, #71147, #65860, .T. ) ;
#78746=VECTOR ( 'NONE', #26067, 1000.000000000000000 ) ;
#78747=ORIENTED_EDGE ( 'NONE', *, *, #55286, .T. ) ;
#78748=DIRECTION ( 'NONE',  ( 1.000000000000000000, 0.000000000000000000, 0.000000000000000000 ) ) ;
#78749=ORIENTED_EDGE ( 'NONE', *, *, #31010, .T. ) ;
#78750=EDGE_CURVE ( 'NONE', #70047, #76240, #27413, .T. ) ;
#78752=CARTESIAN_POINT ( 'NONE',  ( 110.5640613610537883, -45.86347053068958246, 58.86705384733897972 ) ) ;
#78754=ORIENTED_EDGE ( 'NONE', *, *, #63125, .T. ) ;
#78755=DIRECTION ( 'NONE',  ( -4.194175870806139918E-14, 1.000000000000000000, 0.000000000000000000 ) ) ;
#78756=CARTESIAN_POINT ( 'NONE',  ( 113.0097079652340000, -45.31096836313445664, 199.0584824187679374 ) ) ;
#78757=DIRECTION ( 'NONE',  ( 1.000000000000000078E-15, -1.000000000000000083E-30, -1.000000000000000000 ) ) ;
#78758=CARTESIAN_POINT ( 'NONE',  ( 193.0371591254585155, -47.82818131005411999, 180.4678068554150343 ) ) ;
#78759=CARTESIAN_POINT ( 'NONE',  ( 193.0371591254586576, -47.82818131005411999, 129.9678068554150343 ) ) ;
#78763=CARTESIAN_POINT ( 'NONE',  ( 115.1877794388830836, -42.61991029308448020, 98.32696653269469778 ) ) ;
#78764=CARTESIAN_POINT ( 'NONE',  ( 116.6093774848466325, -38.87601340171674025, 148.6499109901969859 ) ) ;
#78765=ORIENTED_EDGE ( 'NONE', *, *, #57996, .F. ) ;
#78766=EDGE_LOOP ( 'NONE', ( #63092, #31371, #89400, #28825 ) ) ;
#78767=CARTESIAN_POINT ( 'NONE',  ( 111.9416332874190090, -45.54441269975540507, 99.41015473446796591 ) ) ;
#78768=PLANE ( 'NONE',  #57395 ) ;
#78769=CARTESIAN_POINT ( 'NONE',  ( 107.4826147187165333, -46.50135945624614209, 233.6099109901959707 ) ) ;
#78770=CARTESIAN_POINT ( 'NONE',  ( 31.90335556477799628, -33.89581943344391135, -5.074374724088000832 ) ) ;
#78773=CARTESIAN_POINT ( 'NONE',  ( 37.03715912545425937, -48.62818131006122258, 313.9678068554150059 ) ) ;
#78777=CARTESIAN_POINT ( 'NONE',  ( 117.2886123466743271, -34.79635738071011986, 158.9756252759109714 ) ) ;
#78779=ORIENTED_EDGE ( 'NONE', *, *, #25487, .T. ) ;
#78780=CARTESIAN_POINT ( 'NONE',  ( 181.9790560690336463, -31.62489322947673642, 237.4678068554150059 ) ) ;
#78781=DIRECTION ( 'NONE',  ( 0.000000000000000000, 1.000000000000000000, 0.000000000000000000 ) ) ;
#78782=CARTESIAN_POINT ( 'NONE',  ( 19.56670390244796920, -67.87844715994100397, 20.91780685541479912 ) ) ;
#78783=DIRECTION ( 'NONE',  ( 0.0001713722455994998422, -0.9999999853157766072, 0.000000000000000000 ) ) ;
#78784=EDGE_CURVE ( 'NONE', #914, #34504, #13354, .T. ) ;
#78785=CARTESIAN_POINT ( 'NONE',  ( 107.4137727038933150, -44.88475929872373626, 235.4280903695919562 ) ) ;
#78786=AXIS2_PLACEMENT_3D ( 'NONE', #85943, #16887, #23713 ) ;
#78787=FACE_OUTER_BOUND ( 'NONE', #53011, .T. ) ;
#78788=CARTESIAN_POINT ( 'NONE',  ( 101.2005795642084820, -45.34792753215401007, 197.1013395616249966 ) ) ;
#78789=DIRECTION ( 'NONE',  ( 3.999999999999999995E-14, -1.000000000000000000, 4.100000000000000342E-29 ) ) ;
#78792=EDGE_LOOP ( 'NONE', ( #63339, #45585, #76677, #68197 ) ) ;
#78793=CARTESIAN_POINT ( 'NONE',  ( 98.27464689803356634, -41.50197325149740379, 62.72272253483316007 ) ) ;
#78794=ORIENTED_EDGE ( 'NONE', *, *, #7846, .F. ) ;
#78795=LINE ( 'NONE', #85612, #20245 ) ;
#78796=DIRECTION ( 'NONE',  ( 0.000000000000000000, 0.000000000000000000, -1.000000000000000000 ) ) ;
#78797=CARTESIAN_POINT ( 'NONE',  ( 116.4516747918435300, -36.28819209217700603, 265.2834880678017839 ) ) ;
#78799=EDGE_LOOP ( 'NONE', ( #74938, #62890, #30185, #928 ) ) ;
#78800=EDGE_CURVE ( 'NONE', #71390, #58180, #42372, .T. ) ;
#78801=CARTESIAN_POINT ( 'NONE',  ( 103.7043515502224551, -44.10458127404638873, 9.635625275910941312 ) ) ;
#78803=VERTEX_POINT ( 'NONE', #28303 ) ;
#78804=ORIENTED_EDGE ( 'NONE', *, *, #34231, .F. ) ;
#78805=AXIS2_PLACEMENT_3D ( 'NONE', #54867, #89430, #67632 ) ;
#78806=ADVANCED_FACE ( 'NONE', ( #76469 ), #13795, .T. ) ;
#78807=CARTESIAN_POINT ( 'NONE',  ( 110.8545879224105306, -45.98418990642309012, 112.8856352535895837 ) ) ;
#78808=EDGE_LOOP ( 'NONE', ( #25653, #25150, #13517, #56621 ) ) ;
#78809=ORIENTED_EDGE ( 'NONE', *, *, #75845, .F. ) ;
#78810=AXIS2_PLACEMENT_3D ( 'NONE', #10092, #86395, #80037 ) ;
#78811=VECTOR ( 'NONE', #46392, 1000.000000000000000 ) ;
#78812=CARTESIAN_POINT ( 'NONE',  ( 99.21763626795888058, -33.35996782468227195, 15.42670554236297242 ) ) ;
#78813=CARTESIAN_POINT ( 'NONE',  ( 111.4265353497823128, -47.77589283047310431, 172.8756252759109771 ) ) ;
#78814=CARTESIAN_POINT ( 'NONE',  ( 113.9025887763448566, -28.07314977735658701, 124.5565776568629559 ) ) ;
#78815=CARTESIAN_POINT ( 'NONE',  ( 34.33598329127472937, -36.32844715994134788, 313.9678068554150059 ) ) ;
#78816=CARTESIAN_POINT ( 'NONE',  ( 96.51815522165868799, -31.32876289826797134, 241.9499109901969689 ) ) ;
#78817=LINE ( 'NONE', #16577, #69020 ) ;
#78818=CARTESIAN_POINT ( 'NONE',  ( 99.09513708517808084, -30.55119466390278049, 126.8023670118761714 ) ) ;
#78820=ORIENTED_EDGE ( 'NONE', *, *, #48847, .T. ) ;
#78822=CARTESIAN_POINT ( 'NONE',  ( 101.3249093792229871, -46.22930045566884871, 202.1318157521019430 ) ) ;
#78824=CARTESIAN_POINT ( 'NONE',  ( 116.6609997163256764, -40.80771701747383418, 168.5070538473399608 ) ) ;
#78825=CARTESIAN_POINT ( 'NONE',  ( 32.56670390244700997, -18.82844715994111340, -5.074374724088000832 ) ) ;
#78826=VECTOR ( 'NONE', #3642, 1000.000000000000000 ) ;
#78827=CARTESIAN_POINT ( 'NONE',  ( 135.3633572498488888, -34.30134337669387889, 7.962481652684965105 ) ) ;
#78829=CARTESIAN_POINT ( 'NONE',  ( 116.3212776292299253, -32.94146857471393730, 145.1356252759109680 ) ) ;
#78831=CARTESIAN_POINT ( 'NONE',  ( 115.9412561796927577, -30.17946786548973748, 255.3203871806729524 ) ) ;
#78832=DIRECTION ( 'NONE',  ( 0.7071067811868035902, 0.7071067811862914443, 7.071067811868029270E-16 ) ) ;
#78834=LINE ( 'NONE', #73327, #80170 ) ;
#78836=CIRCLE ( 'NONE', #49815, 0.5000000000000004441 ) ;
#78837=EDGE_CURVE ( 'NONE', #81882, #71705, #49842, .T. ) ;
#78839=CARTESIAN_POINT ( 'NONE',  ( 104.4081006870482184, -46.45808914696898739, 258.3647919446885339 ) ) ;
#78840=DIRECTION ( 'NONE',  ( 0.000000000000000000, 0.000000000000000000, -1.000000000000000000 ) ) ;
#78841=CARTESIAN_POINT ( 'NONE',  ( 113.8796460939257287, -30.53604272315569546, 195.5838068554168103 ) ) ;
#78842=ORIENTED_EDGE ( 'NONE', *, *, #40170, .T. ) ;
#78844=CARTESIAN_POINT ( 'NONE',  ( 188.5667039024479834, -48.82844715994099971, 175.9678068554150059 ) ) ;
#78845=CARTESIAN_POINT ( 'NONE',  ( 104.4481554933880716, -26.61555950438322427, 200.2784824187679362 ) ) ;
#78846=CARTESIAN_POINT ( 'NONE',  ( 107.8683515708180636, -26.33524229811608919, 66.01562527591097762 ) ) ;
#78847=CARTESIAN_POINT ( 'NONE',  ( 97.38492667529318680, -42.15761073986299579, 177.7451490854349743 ) ) ;
#78850=PLANE ( 'NONE',  #13048 ) ;
#78851=CARTESIAN_POINT ( 'NONE',  ( 101.6336199742765984, -45.20051650499360107, 38.12198527528386194 ) ) ;
#78852=CARTESIAN_POINT ( 'NONE',  ( 46.03715912545427358, -48.62818131006086020, 300.4678068554150059 ) ) ;
#78853=CARTESIAN_POINT ( 'NONE',  ( 71.25416588882602298, -72.55705569728901594, 396.9756252759102040 ) ) ;
#78854=EDGE_LOOP ( 'NONE', ( #9247, #45523 ) ) ;
#78855=AXIS2_PLACEMENT_3D ( 'NONE', #7903, #84233, #13385 ) ;
#78856=DIRECTION ( 'NONE',  ( 0.000000000000000000, 0.000000000000000000, -1.000000000000000000 ) ) ;
#78857=ADVANCED_FACE ( 'NONE', ( #33788 ), #20616, .F. ) ;
#78858=ORIENTED_EDGE ( 'NONE', *, *, #10406, .T. ) ;
#78860=EDGE_CURVE ( 'NONE', #15500, #5714, #72347, .T. ) ;
#78861=CARTESIAN_POINT ( 'NONE',  ( 113.2121186763659040, -42.70299450126940144, 97.63527697093398672 ) ) ;
#78864=CARTESIAN_POINT ( 'NONE',  ( 113.8422018911646774, -44.62364141802220985, 104.1413395616249744 ) ) ;
#78865=CARTESIAN_POINT ( 'NONE',  ( 57.56670390244744340, -48.82844715994040286, 173.2178068554150911 ) ) ;
#78866=LINE ( 'NONE', #32018, #26854 ) ;
#78868=B_SPLINE_CURVE_WITH_KNOTS ( 'NONE', 3,
 ( #51481, #43784, #66008, #64690, #71522, #9281, #79677, #31488, #37879, #85601, #3361, #24688, #80118, #31050, #66457, #4245, #50601, #85154 ),
 .UNSPECIFIED., .F., .F.,
 ( 4, 2, 2, 2, 2, 2, 2, 2, 4 ),
 ( 0.000000000000000000, 0.06250004591115866648, 0.1250000918223173330, 0.1875001377334760133, 0.2500001836446346659, 0.3125002295557933185, 0.3750002754669520266, 0.4375003213781106792, 0.5000003672892693318 ),
 .UNSPECIFIED. ) ;
#78869=CARTESIAN_POINT ( 'NONE',  ( 100.4186822966649828, -43.90371905523902996, 46.98133956162492098 ) ) ;
#78873=AXIS2_PLACEMENT_3D ( 'NONE', #8444, #36141, #63856 ) ;
#78874=LINE ( 'NONE', #40180, #63099 ) ;
#78877=VECTOR ( 'NONE', #42685, 999.9999999999998863 ) ;
#78878=CARTESIAN_POINT ( 'NONE',  ( 177.0664832912740110, 12.92155284005802685, 349.2756252759111248 ) ) ;
#78879=CARTESIAN_POINT ( 'NONE',  ( 34.33598329127499227, -36.32844715994100682, -5.074374724088000832 ) ) ;
#78883=CARTESIAN_POINT ( 'NONE',  ( 111.9186950350130303, -27.52701776748434170, 59.68991099019693536 ) ) ;
#78887=EDGE_CURVE ( 'NONE', #60920, #45127, #57809, .T. ) ;
#78888=CARTESIAN_POINT ( 'NONE',  ( 115.5296723907996039, -38.53924143319417794, 106.4890427505429642 ) ) ;
#78892=DIRECTION ( 'NONE',  ( -0.7071067811865773267, 0.7071067811865178188, -7.071067811865781017E-16 ) ) ;
#78893=FACE_OUTER_BOUND ( 'NONE', #12312, .T. ) ;
#78896=CARTESIAN_POINT ( 'NONE',  ( 116.8169691553371763, -34.15232147661988193, 139.0309223820618740 ) ) ;
#78897=AXIS2_PLACEMENT_3D ( 'NONE', #75727, #39842, #33038 ) ;
#78899=ORIENTED_EDGE ( 'NONE', *, *, #43782, .T. ) ;
#78900=CARTESIAN_POINT ( 'NONE',  ( 113.2524973562852608, -30.34232264463288686, 170.8958690201829711 ) ) ;
#78902=CARTESIAN_POINT ( 'NONE',  ( 97.59729452806701033, -30.98317272244041121, 121.8803871806729546 ) ) ;
#78904=AXIS2_PLACEMENT_3D ( 'NONE', #68279, #6060, #54157 ) ;
#78906=ORIENTED_EDGE ( 'NONE', *, *, #26281, .T. ) ;
#78907=ADVANCED_FACE ( 'NONE', ( #36488 ), #58688, .F. ) ;
#78908=ORIENTED_EDGE ( 'NONE', *, *, #79778, .T. ) ;
#78910=CARTESIAN_POINT ( 'NONE',  ( 102.4736563324128440, -43.47745920372498318, 194.9195189410199589 ) ) ;
#78911=CARTESIAN_POINT ( 'NONE',  ( 107.2325596213128875, -25.65389481303129315, 80.07657765686299456 ) ) ;
#78912=ORIENTED_EDGE ( 'NONE', *, *, #87326, .F. ) ;
#78913=CARTESIAN_POINT ( 'NONE',  ( 100.4929927897290014, -27.87207479535954135, 35.59657765686397113 ) ) ;
#78914=CARTESIAN_POINT ( 'NONE',  ( 112.3219919889560288, -28.66302566169128596, 249.5838068554155882 ) ) ;
#78915=LINE ( 'NONE', #29415, #88701 ) ;
#78916=DIRECTION ( 'NONE',  ( -8.252657816380299978E-16, -2.773339119917620066E-31, -1.000000000000000000 ) ) ;
#78917=CARTESIAN_POINT ( 'NONE',  ( 114.2399097434533246, -45.14383888093294672, 149.1508633711489722 ) ) ;
#78918=CARTESIAN_POINT ( 'NONE',  ( 36.74138383868169910, -48.33240602328862678, 249.9678068554150343 ) ) ;
#78919=EDGE_LOOP ( 'NONE', ( #5016, #69898, #4488, #4576 ) ) ;
#78922=PLANE ( 'NONE',  #72348 ) ;
#78926=LINE ( 'NONE', #45692, #80908 ) ;
#78928=CARTESIAN_POINT ( 'NONE',  ( 118.7327907441706571, -34.64671908090114272, 48.96705384733895983 ) ) ;
#78929=DIRECTION ( 'NONE',  ( 0.000000000000000000, 0.000000000000000000, 1.000000000000000000 ) ) ;
#78930=CYLINDRICAL_SURFACE ( 'NONE', #69557, 3.249999999999975131 ) ;
#78931=CARTESIAN_POINT ( 'NONE',  ( 80.06648329127398256, -9.029447159941060619, 8.225625275910942946 ) ) ;
#78932=CARTESIAN_POINT ( 'NONE',  ( 103.6990349130722251, -26.13358598113143216, 55.32133956162594046 ) ) ;
#78933=CARTESIAN_POINT ( 'NONE',  ( 107.0664832912739968, -36.72944715994100306, 287.6356252759109680 ) ) ;
#78934=CARTESIAN_POINT ( 'NONE',  ( 114.2383551682309815, -44.26553795382356071, 154.1813395616249807 ) ) ;
#78936=EDGE_CURVE ( 'NONE', #52592, #65495, #35384, .T. ) ;
#78937=CARTESIAN_POINT ( 'NONE',  ( 25.56670390244805446, -42.82844715994167473, 290.7178068554150059 ) ) ;
#78938=ORIENTED_EDGE ( 'NONE', *, *, #8900, .F. ) ;
#78942=CARTESIAN_POINT ( 'NONE',  ( 82.81648329127402519, -36.72944715994107412, -5.074374724089055100 ) ) ;
#78943=DIRECTION ( 'NONE',  ( 0.000000000000000000, 0.000000000000000000, 1.000000000000000000 ) ) ;
#78944=CARTESIAN_POINT ( 'NONE',  ( 101.3249093792229871, -46.22930045566884871, 202.1318157521019430 ) ) ;
#78945=ORIENTED_EDGE ( 'NONE', *, *, #57384, .T. ) ;
#78946=ADVANCED_FACE ( 'NONE', ( #44612 ), #29662, .F. ) ;
#78947=CARTESIAN_POINT ( 'NONE',  ( 97.53194275716850825, -39.74926679241858096, 146.5705568277559223 ) ) ;
#78948=CARTESIAN_POINT ( 'NONE',  ( 100.2339645716073164, -28.82666620644582522, 256.6441967044821695 ) ) ;
#78949=CARTESIAN_POINT ( 'NONE',  ( 118.8919219083537797, -35.39899076563189340, 79.91562527591095488 ) ) ;
#78950=LINE ( 'NONE', #85774, #65048 ) ;
#78952=CARTESIAN_POINT ( 'NONE',  ( 97.80969226196111777, -40.51824922604903634, 262.6357212258262166 ) ) ;
#78957=VERTEX_POINT ( 'NONE', #71904 ) ;
#78961=VECTOR ( 'NONE', #60688, 1000.000000000000000 ) ;
#78963=DIRECTION ( 'NONE',  ( -0.7071067811865475727, 0.000000000000000000, -0.7071067811865475727 ) ) ;
#78964=CARTESIAN_POINT ( 'NONE',  ( 117.4913186190917855, -36.80221964929349809, 259.8213395616249386 ) ) ;
#78965=LINE ( 'NONE', #9460, #64987 ) ;
#78966=EDGE_CURVE ( 'NONE', #19262, #62172, #22865, .T. ) ;
#78968=CARTESIAN_POINT ( 'NONE',  ( 34.27258461953873336, -35.55794170701842916, 313.9678068554150059 ) ) ;
#78970=DIRECTION ( 'NONE',  ( 0.000000000000000000, 0.000000000000000000, 1.000000000000000000 ) ) ;
#78971=CARTESIAN_POINT ( 'NONE',  ( 98.15635076299318484, -32.87196533591951919, 210.4238483995049762 ) ) ;
#78972=ORIENTED_EDGE ( 'NONE', *, *, #61291, .F. ) ;
#78973=ORIENTED_EDGE ( 'NONE', *, *, #33000, .F. ) ;
#78975=CARTESIAN_POINT ( 'NONE',  ( 160.7738106836348777, -48.62134037874901082, 249.9678068554149490 ) ) ;
#78976=CARTESIAN_POINT ( 'NONE',  ( 111.2449163426335303, -45.81617768730462359, 182.9194528165492954 ) ) ;
#78977=CARTESIAN_POINT ( 'NONE',  ( 115.9511604134431195, -42.07746527072326614, 274.3832443235294249 ) ) ;
#78978=CYLINDRICAL_SURFACE ( 'NONE', #16840, 9.999999999999998224 ) ;
#78979=CARTESIAN_POINT ( 'NONE',  ( 156.5667039024483529, -42.82844715993568485, 137.2178068554149775 ) ) ;
#78980=CARTESIAN_POINT ( 'NONE',  ( 162.5667039024470171, -32.29483332968611364, 237.4678068554150059 ) ) ;
#78981=ORIENTED_EDGE ( 'NONE', *, *, #54255, .T. ) ;
#78982=CARTESIAN_POINT ( 'NONE',  ( 78.76417807488600431, -34.30680158339610841, 1.893168945966681838 ) ) ;
#78983=EDGE_LOOP ( 'NONE', ( #49389, #84024, #12290, #85519, #38512 ) ) ;
#78985=CARTESIAN_POINT ( 'NONE',  ( 109.0595394021483742, -27.66723669546327358, 27.72237608387795404 ) ) ;
#78986=VECTOR ( 'NONE', #14140, 1000.000000000000000 ) ;
#78987=DIRECTION ( 'NONE',  ( 5.512527431108029424E-15, -1.000000000000000000, 0.000000000000000000 ) ) ;
#78988=AXIS2_PLACEMENT_3D ( 'NONE', #71343, #9553, #86302 ) ;
#78989=EDGE_CURVE ( 'NONE', #30803, #17437, #35591, .T. ) ;
#78990=DIRECTION ( 'NONE',  ( 0.000000000000000000, 0.000000000000000000, 1.000000000000000000 ) ) ;
#78991=FACE_OUTER_BOUND ( 'NONE', #30531, .T. ) ;
#78996=CARTESIAN_POINT ( 'NONE',  ( 104.2140152791992875, -25.22710339543701963, 90.26991099019693365 ) ) ;
#78997=ORIENTED_EDGE ( 'NONE', *, *, #37087, .T. ) ;
#78998=CARTESIAN_POINT ( 'NONE',  ( 104.2253390597007581, -44.78450961640034222, 56.72956268521994616 ) ) ;
#78999=DIRECTION ( 'NONE',  ( 0.9834602067019598826, 0.1811243270069988198, 0.000000000000000000 ) ) ;
#79000=CARTESIAN_POINT ( 'NONE',  ( 98.26727195740441800, -38.00851302551287603, 62.87301187732596475 ) ) ;
#79001=CARTESIAN_POINT ( 'NONE',  ( 101.9932406875673081, -45.44583697117432308, 13.15642348592802691 ) ) ;
#79004=CARTESIAN_POINT ( 'NONE',  ( 112.9754938005188478, -28.11429459860147873, 40.59848241876795782 ) ) ;
#79006=VERTEX_POINT ( 'NONE', #65955 ) ;
#79007=CARTESIAN_POINT ( 'NONE',  ( 172.5664832912740110, -9.303447159940999356, 316.8086252759120498 ) ) ;
#79008=CIRCLE ( 'NONE', #87745, 0.2999999999999943823 ) ;
#79009=ORIENTED_EDGE ( 'NONE', *, *, #58033, .T. ) ;
#79010=CARTESIAN_POINT ( 'NONE',  ( 114.5587124134895731, -28.54364023664675187, 150.4746728949579619 ) ) ;
#79011=ADVANCED_FACE ( 'NONE', ( #19165 ), #45058, .F. ) ;
#79013=AXIS2_PLACEMENT_3D ( 'NONE', #82316, #40050, #66867 ) ;
#79015=ORIENTED_EDGE ( 'NONE', *, *, #51778, .T. ) ;
#79016=ORIENTED_EDGE ( 'NONE', *, *, #55706, .F. ) ;
#79017=VECTOR ( 'NONE', #12452, 1000.000000000000000 ) ;
#79020=DIRECTION ( 'NONE',  ( -0.0001713722455994998422, 0.9999999853157766072, 0.000000000000000000 ) ) ;
#79021=CARTESIAN_POINT ( 'NONE',  ( 103.9298229712113653, -26.84510867568817716, 205.3089586092449679 ) ) ;
#79022=LINE ( 'NONE', #64932, #73349 ) ;
#79023=CARTESIAN_POINT ( 'NONE',  ( 51.56670390244671154, -32.29483332968566600, 193.9678068554150911 ) ) ;
#79024=CARTESIAN_POINT ( 'NONE',  ( 36.23715912545422668, -47.82818131006125384, 313.9678068554150059 ) ) ;
#79025=CARTESIAN_POINT ( 'NONE',  ( 117.3845446746782386, -38.21944606407609513, 24.71276813305395237 ) ) ;
#79026=EDGE_CURVE ( 'NONE', #66874, #15321, #66400, .T. ) ;
#79027=CARTESIAN_POINT ( 'NONE',  ( 51.42025729304100423, -33.70561438051981185, -5.074374724088000832 ) ) ;
#79028=EDGE_LOOP ( 'NONE', ( #18912, #51132, #80403, #25144 ) ) ;
#79029=CARTESIAN_POINT ( 'NONE',  ( 97.75828382342812972, -40.38462848611586509, 172.6242326989190872 ) ) ;
#79030=EDGE_CURVE ( 'NONE', #55083, #22615, #68729, .T. ) ;
#79034=DIRECTION ( 'NONE',  ( 1.000000000000000000, 1.261617073437676668E-15, 9.462128050782575008E-16 ) ) ;
#79035=CARTESIAN_POINT ( 'NONE',  ( 106.8520627977276831, -47.75749532952668375, 227.5489586092439538 ) ) ;
#79037=EDGE_CURVE ( 'NONE', #15093, #26765, #4190, .T. ) ;
#79038=FACE_BOUND ( 'NONE', #76574, .T. ) ;
#79040=CARTESIAN_POINT ( 'NONE',  ( 98.42407572851979580, -32.30458340910843162, 245.3724198280769428 ) ) ;
#79041=CARTESIAN_POINT ( 'NONE',  ( 179.8608231853560255, -35.55794170701751256, 342.9256252759119548 ) ) ;
#79042=CARTESIAN_POINT ( 'NONE',  ( 99.14404768239424470, -44.40400490628089614, 37.95086337114900488 ) ) ;
#79044=CARTESIAN_POINT ( 'NONE',  ( 107.3350830925955961, -26.26357308316309869, 120.0556252759109555 ) ) ;
#79047=EDGE_LOOP ( 'NONE', ( #86517, #87996, #10911, #64807 ) ) ;
#79048=CARTESIAN_POINT ( 'NONE',  ( 97.06107110448571973, -37.99641202366499471, 67.42729194735355236 ) ) ;
#79049=CARTESIAN_POINT ( 'NONE',  ( 134.0664832912739826, -18.72944715994100306, -5.074374724089001809 ) ) ;
#79051=EDGE_LOOP ( 'NONE', ( #6223, #56174, #8715, #41542 ) ) ;
#79052=CARTESIAN_POINT ( 'NONE',  ( 115.8254254363784810, -31.73000183497265425, 49.23979340379111136 ) ) ;
#79053=ORIENTED_EDGE ( 'NONE', *, *, #48976, .F. ) ;
#79054=LINE ( 'NONE', #71349, #56663 ) ;
#79055=PLANE ( 'NONE',  #75166 ) ;
#79056=AXIS2_PLACEMENT_3D ( 'NONE', #52426, #23882, #78856 ) ;
#79057=LINE ( 'NONE', #45829, #55331 ) ;
#79058=ORIENTED_EDGE ( 'NONE', *, *, #13447, .F. ) ;
#79059=CARTESIAN_POINT ( 'NONE',  ( 102.9623509218069302, -46.33686416246144546, 92.25562527591097250 ) ) ;
#79060=FILL_AREA_STYLE ('',( #10012 ) ) ;
#79062=CARTESIAN_POINT ( 'NONE',  ( 141.9629299006807628, -45.68655394112754919, -5.074374724088960953 ) ) ;
#79066=EDGE_CURVE ( 'NONE', #15987, #39978, #17817, .T. ) ;
#79067=CARTESIAN_POINT ( 'NONE',  ( 46.03715912545343514, -48.62818131006090283, 180.4678068554150911 ) ) ;
#79070=ADVANCED_FACE ( 'NONE', ( #45939, #5546, #86869, #39592, #66857, #67298, #31433 ), #5084, .T. ) ;
#79072=ADVANCED_FACE ( 'NONE', ( #39150 ), #32784, .F. ) ;
#79079=CIRCLE ( 'NONE', #44219, 3.250000000000002665 ) ;
#79080=AXIS2_PLACEMENT_3D ( 'NONE', #46797, #17777, #47249 ) ;
#79081=CYLINDRICAL_SURFACE ( 'NONE', #7083, 0.5000000000000104361 ) ;
#79082=CARTESIAN_POINT ( 'NONE',  ( 114.0056865186721922, -29.02320718445401226, 155.5051490854339704 ) ) ;
#79083=CARTESIAN_POINT ( 'NONE',  ( 151.0371591254572934, -24.42818131005592974, 313.9678068554149490 ) ) ;
#79084=VERTEX_POINT ( 'NONE', #54096 ) ;
#79085=AXIS2_PLACEMENT_3D ( 'NONE', #39812, #62059, #20736 ) ;
#79087=CARTESIAN_POINT ( 'NONE',  ( 116.1206117333611019, -31.56300607074032882, 285.2384824187680579 ) ) ;
#79088=CARTESIAN_POINT ( 'NONE',  ( 51.42025729304100423, -33.70561438051981185, 342.9256252759119548 ) ) ;
#79091=ORIENTED_EDGE ( 'NONE', *, *, #40841, .T. ) ;
#79092=CARTESIAN_POINT ( 'NONE',  ( 97.07210237969420064, -35.37814555816738959, 31.21915939149969077 ) ) ;
#79093=CARTESIAN_POINT ( 'NONE',  ( 96.80143343076635176, -35.25719154489700458, 226.2251490854349640 ) ) ;
#79097=CARTESIAN_POINT ( 'NONE',  ( 112.2422220273998477, -28.08754728269216372, 201.0787261630399598 ) ) ;
#79099=CARTESIAN_POINT ( 'NONE',  ( 115.8966032383871436, -37.77400989437322210, 50.16444044875395747 ) ) ;
#79101=AXIS2_PLACEMENT_3D ( 'NONE', #38261, #9665, #29667 ) ;
#79102=ADVANCED_FACE ( 'NONE', ( #53646 ), #86178, .T. ) ;
#79103=DIRECTION ( 'NONE',  ( 0.000000000000000000, 1.000000000000000000, 0.000000000000000000 ) ) ;
#79104=CARTESIAN_POINT ( 'NONE',  ( 107.0664832912739541, -21.02944715994095759, 311.6356252759109680 ) ) ;
#79106=DIRECTION ( 'NONE',  ( -1.000000000000000000, -8.843517682682131024E-16, -1.000000000000000078E-15 ) ) ;
#79107=DIRECTION ( 'NONE',  ( -4.237773401492740281E-14, 1.000000000000000000, 0.000000000000000000 ) ) ;
#79108=VERTEX_POINT ( 'NONE', #25523 ) ;
#79109=CARTESIAN_POINT ( 'NONE',  ( 105.7790678824445081, -26.40611305247077567, 270.1756252759109884 ) ) ;
#79111=VERTEX_POINT ( 'NONE', #74569 ) ;
#79112=DIRECTION ( 'NONE',  ( -0.7071067811865476838, -0.7071067811865473507, 0.000000000000000000 ) ) ;
#79113=FACE_OUTER_BOUND ( 'NONE', #50290, .T. ) ;
#79114=DIRECTION ( 'NONE',  ( 1.000000000000000000, 6.508581945447490214E-14, 1.000000000000000078E-15 ) ) ;
#79116=CARTESIAN_POINT ( 'NONE',  ( 116.7468388360763925, -38.12735696270775065, 24.71276813305395237 ) ) ;
#79119=CARTESIAN_POINT ( 'NONE',  ( 110.5697598356958764, -46.63222799359486714, 33.84705384733993583 ) ) ;
#79120=ADVANCED_FACE ( 'NONE', ( #12351 ), #38258, .F. ) ;
#79121=LINE ( 'NONE', #78691, #83120 ) ;
#79122=CIRCLE ( 'NONE', #64641, 2.517500000000005844 ) ;
#79123=CARTESIAN_POINT ( 'NONE',  ( 116.3173282457959345, -41.53670860177669510, 288.4441967044823514 ) ) ;
#79124=EDGE_CURVE ( 'NONE', #17571, #42544, #12252, .T. ) ;
#79125=ORIENTED_EDGE ( 'NONE', *, *, #10212, .T. ) ;
#79126=EDGE_CURVE ( 'NONE', #14315, #72641, #20494, .T. ) ;
#79127=CARTESIAN_POINT ( 'NONE',  ( 82.81648329127398256, -18.72944715994105636, 3.101481641215461327 ) ) ;
#79128=CARTESIAN_POINT ( 'NONE',  ( 117.0611971830093410, -38.07833408437429767, 19.71924984274187054 ) ) ;
#79130=CARTESIAN_POINT ( 'NONE',  ( 115.1291642039608547, -38.00337907228554712, 111.5195189410199674 ) ) ;
#79131=CARTESIAN_POINT ( 'NONE',  ( 98.41694670496758590, -29.81058001376278099, 191.7775300378159784 ) ) ;
#79133=EDGE_CURVE ( 'NONE', #18507, #7678, #63010, .T. ) ;
#79137=CARTESIAN_POINT ( 'NONE',  ( 57.56670390244722313, -42.82844715994040996, 137.2178068554150911 ) ) ;
#79138=ORIENTED_EDGE ( 'NONE', *, *, #5615, .T. ) ;
#79140=ADVANCED_FACE ( 'NONE', ( #62278 ), #68659, .F. ) ;
#79141=VECTOR ( 'NONE', #192, 1000.000000000000000 ) ;
#79142=FACE_BOUND ( 'NONE', #63707, .T. ) ;
#79143=VECTOR ( 'NONE', #13281, 1000.000000000000000 ) ;
#79144=ORIENTED_EDGE ( 'NONE', *, *, #86305, .T. ) ;
#79145=ORIENTED_EDGE ( 'NONE', *, *, #84269, .F. ) ;
#79148=EDGE_CURVE ( 'NONE', #51120, #57891, #55890, .T. ) ;
#79149=CARTESIAN_POINT ( 'NONE',  ( 103.2786526221089645, -27.47459228116735375, 41.38561342082059724 ) ) ;
#79150=CARTESIAN_POINT ( 'NONE',  ( 100.0140161817732860, -31.91085406740108610, 120.2724198280769912 ) ) ;
#79151=VECTOR ( 'NONE', #18268, 1000.000000000000000 ) ;
#79152=CARTESIAN_POINT ( 'NONE',  ( 115.6474790210939290, -28.48352029850561706, 39.43562527591099354 ) ) ;
#79153=EDGE_CURVE ( 'NONE', #3395, #18115, #61380, .T. ) ;
#79155=ADVANCED_FACE ( 'NONE', ( #69555 ), #62729, .F. ) ;
#79158=CARTESIAN_POINT ( 'NONE',  ( 115.1113848037478391, -30.75858365065169764, 135.3346201298422216 ) ) ;
#79159=VERTEX_POINT ( 'NONE', #40496 ) ;
#79160=DIRECTION ( 'NONE',  ( 0.000000000000000000, 1.000000000000000000, 0.000000000000000000 ) ) ;
#79161=LINE ( 'NONE', #73657, #29926 ) ;
#79162=CARTESIAN_POINT ( 'NONE',  ( 84.06648329127399677, -18.82844715994099971, 17.92562527591199739 ) ) ;
#79163=AXIS2_PLACEMENT_3D ( 'NONE', #16846, #44524, #77738 ) ;
#79164=CARTESIAN_POINT ( 'NONE',  ( 112.3606361654194075, -28.17110760307337713, 289.6356252759109680 ) ) ;
#79166=CARTESIAN_POINT ( 'NONE',  ( 115.9069864544413662, -30.09434420101750973, 264.3508633711492735 ) ) ;
#79167=CARTESIAN_POINT ( 'NONE',  ( 97.03360904796217312, -33.74039811955494628, 27.09562527591097236 ) ) ;
#79168=CARTESIAN_POINT ( 'NONE',  ( 101.9936209330291064, -45.44607153419508450, 118.1564586085293627 ) ) ;
#79169=VECTOR ( 'NONE', #2320, 1000.000000000000000 ) ;
#79170=CARTESIAN_POINT ( 'NONE',  ( 123.6837132603318707, -20.11243780205705534, 219.5838068554170093 ) ) ;
#79172=CARTESIAN_POINT ( 'NONE',  ( 105.8602753772252498, -25.33367152814009771, 323.3526086649692957 ) ) ;
#79173=CARTESIAN_POINT ( 'NONE',  ( 163.0959832912774914, -23.42844715993537719, 117.4678068554150485 ) ) ;
#79174=CARTESIAN_POINT ( 'NONE',  ( 131.5555141844853040, -37.85480617634013356, 7.067502061095533250 ) ) ;
#79175=LINE ( 'NONE', #65522, #60488 ) ;
#79180=LINE ( 'NONE', #78738, #19129 ) ;
#79181=CARTESIAN_POINT ( 'NONE',  ( 111.0631195717115673, -47.08511319755631774, 17.85753003781598380 ) ) ;
#79182=CARTESIAN_POINT ( 'NONE',  ( 97.38209261381841486, -42.05735084626116560, 172.7146728949589942 ) ) ;
#79183=CARTESIAN_POINT ( 'NONE',  ( 105.4175444341163939, -47.04536977979798706, 33.44991099019695469 ) ) ;
#79186=CARTESIAN_POINT ( 'NONE',  ( 72.26648329127297643, -71.52944715994141234, 361.9756252759109998 ) ) ;
#79187=CARTESIAN_POINT ( 'NONE',  ( 172.5664832912740110, -36.32844715994070839, 14.17562527591199917 ) ) ;
#79188=VECTOR ( 'NONE', #20455, 1000.000000000000000 ) ;
#79189=VECTOR ( 'NONE', #70885, 1000.000000000000000 ) ;
#79192=CARTESIAN_POINT ( 'NONE',  ( 109.7248659590922273, -27.00080519083036990, 185.8647919394705070 ) ) ;
#79193=ORIENTED_EDGE ( 'NONE', *, *, #89740, .F. ) ;
#79194=CARTESIAN_POINT ( 'NONE',  ( 113.0644005321300227, -46.09090919705343481, 64.02991099019594401 ) ) ;
#79196=ORIENTED_EDGE ( 'NONE', *, *, #6008, .F. ) ;
#79197=DIRECTION ( 'NONE',  ( 3.999999999999999995E-14, -1.000000000000000000, 4.100000000000000342E-29 ) ) ;
#79198=CARTESIAN_POINT ( 'NONE',  ( 104.4591861284130232, -26.65816784528765382, 196.2784824187679362 ) ) ;
#79199=DIRECTION ( 'NONE',  ( 1.000000000000000078E-15, -1.000000000000000083E-30, -1.000000000000000000 ) ) ;
#79200=CARTESIAN_POINT ( 'NONE',  ( 97.83900604915858423, -40.58358724573557197, 146.6413223322464603 ) ) ;
#79201=FACE_OUTER_BOUND ( 'NONE', #83996, .T. ) ;
#79204=FACE_OUTER_BOUND ( 'NONE', #33526, .T. ) ;
#79205=CARTESIAN_POINT ( 'NONE',  ( 98.54774150848822956, -41.53511815344526070, 136.7356252759109623 ) ) ;
#79208=CARTESIAN_POINT ( 'NONE',  ( 108.3172770934737628, -27.95654607328577868, 101.3958690201829711 ) ) ;
#79209=AXIS2_PLACEMENT_3D ( 'NONE', #59941, #75831, #74940 ) ;
#79210=CARTESIAN_POINT ( 'NONE',  ( 191.6375511031394865, 22.69262065192448219, 323.8756252759109202 ) ) ;
#79211=VECTOR ( 'NONE', #46319, 1000.000000000000000 ) ;
#79212=CARTESIAN_POINT ( 'NONE',  ( 103.5361331145923032, -27.60804031003073788, 211.3699109901959616 ) ) ;
#79213=DIRECTION ( 'NONE',  ( 0.000000000000000000, 0.000000000000000000, -1.000000000000000000 ) ) ;
#79214=AXIS2_PLACEMENT_3D ( 'NONE', #48224, #84584, #8724 ) ;
#79221=CARTESIAN_POINT ( 'NONE',  ( 96.64068249873260186, -36.21262657180042766, 171.2870538473399620 ) ) ;
#79227=CARTESIAN_POINT ( 'NONE',  ( 41.56648329127398966, -27.57844715994070484, 318.9256252759120116 ) ) ;
#79229=DIRECTION ( 'NONE',  ( 0.7071067811865614505, -0.7071067811865336949, 0.000000000000000000 ) ) ;
#79231=EDGE_CURVE ( 'NONE', #12340, #35953, #37272, .T. ) ;
#79232=CARTESIAN_POINT ( 'NONE',  ( 97.38189020833135601, -42.05746220039552696, 176.7146728949589658 ) ) ;
#79233=EDGE_CURVE ( 'NONE', #14667, #76506, #61516, .T. ) ;
#79236=VERTEX_POINT ( 'NONE', #44511 ) ;
#79238=ADVANCED_FACE ( 'NONE', ( #84993 ), #70280, .T. ) ;
#79241=CARTESIAN_POINT ( 'NONE',  ( 133.0522658620028835, -34.17316201338590531, 8.065992442480034441 ) ) ;
#79242=CARTESIAN_POINT ( 'NONE',  ( 98.30854254679421445, -35.37787306724802505, 262.6358690201826676 ) ) ;
#79244=DIRECTION ( 'NONE',  ( 0.7071067811868056996, 0.7071067811862893349, 7.071067811868050964E-16 ) ) ;
#79246=CARTESIAN_POINT ( 'NONE',  ( 115.1222891817772620, -41.02565380217686908, 9.635625275910943088 ) ) ;
#79247=DIRECTION ( 'NONE',  ( 1.000000000000000078E-15, -1.000000000000000083E-30, -1.000000000000000000 ) ) ;
#79250=EDGE_CURVE ( 'NONE', #49393, #13709, #64534, .T. ) ;
#79252=ORIENTED_EDGE ( 'NONE', *, *, #15565, .F. ) ;
#79253=EDGE_LOOP ( 'NONE', ( #36034, #1083, #81592, #31778 ) ) ;
#79255=CARTESIAN_POINT ( 'NONE',  ( 114.5155466417691912, -41.88356374938643256, 12.77908649474396263 ) ) ;
#79256=CARTESIAN_POINT ( 'NONE',  ( 109.3633609874958523, -25.89340572475189006, 184.9222919425779708 ) ) ;
#79257=CARTESIAN_POINT ( 'NONE',  ( 102.4028819069269218, -26.73371583578772004, 135.4118157521009493 ) ) ;
#79258=CARTESIAN_POINT ( 'NONE',  ( 51.34673845256495639, -36.02818131005847135, 117.4678068554150485 ) ) ;
#79259=CARTESIAN_POINT ( 'NONE',  ( 109.9892391005685255, -26.72245031140752758, 255.8499109901966051 ) ) ;
#79263=VERTEX_POINT ( 'NONE', #77268 ) ;
#79264=EDGE_CURVE ( 'NONE', #52443, #59735, #55028, .T. ) ;
#79265=ORIENTED_EDGE ( 'NONE', *, *, #58271, .F. ) ;
#79266=CIRCLE ( 'NONE', #40066, 3.249999999999975131 ) ;
#79268=AXIS2_PLACEMENT_3D ( 'NONE', #2637, #16708, #51199 ) ;
#79269=CARTESIAN_POINT ( 'NONE',  ( 116.3896376309502045, -44.12590514183388990, 198.2927681330539542 ) ) ;
#79272=CARTESIAN_POINT ( 'NONE',  ( 96.01388918828124019, -36.58377270012555726, 156.3280062282919687 ) ) ;
#79273=FACE_OUTER_BOUND ( 'NONE', #61787, .T. ) ;
#79274=AXIS2_PLACEMENT_3D ( 'NONE', #34614, #29153, #14636 ) ;
#79276=LINE ( 'NONE', #73773, #71126 ) ;
#79278=DIRECTION ( 'NONE',  ( -0.8571673007021084478, -0.5150380749100604838, -8.571673007021083688E-16 ) ) ;
#79279=DIRECTION ( 'NONE',  ( -0.9254794337955620787, -0.3787978585227822492, 0.000000000000000000 ) ) ;
#79280=CARTESIAN_POINT ( 'NONE',  ( 98.95751068421678553, -41.73716824282166016, 7.768006228290936122 ) ) ;
#79282=DIRECTION ( 'NONE',  ( 0.9963424814100680926, -0.08544974978095691565, 0.000000000000000000 ) ) ;
#79285=DIRECTION ( 'NONE',  ( -0.8571673007021110013, 1.917331853055865018E-16, 0.5150380749100563760 ) ) ;
#79287=CARTESIAN_POINT ( 'NONE',  ( 99.35013961165397234, -39.68856579947961194, 195.5838068554172651 ) ) ;
#79289=CARTESIAN_POINT ( 'NONE',  ( 135.9139897988289079, -20.77444411305278749, 7.664507283848439378 ) ) ;
#79290=CARTESIAN_POINT ( 'NONE',  ( 96.62214413241265731, -36.48016117738031738, 196.3070538473399438 ) ) ;
#79291=CARTESIAN_POINT ( 'NONE',  ( 117.2667774650794428, -38.88269731149204489, 59.66133956162595098 ) ) ;
#79292=CARTESIAN_POINT ( 'NONE',  ( 98.90868739403623522, -30.16870437830188934, 236.7870538473399336 ) ) ;
#79293=CARTESIAN_POINT ( 'NONE',  ( 120.1849926298398685, -37.85453553205689303, 293.6356252759106837 ) ) ;
#79294=EDGE_CURVE ( 'NONE', #34565, #36668, #31783, .T. ) ;
#79295=CARTESIAN_POINT ( 'NONE',  ( 172.5664832912729878, -27.82844715994070484, 318.9256252759120116 ) ) ;
#79296=AXIS2_PLACEMENT_3D ( 'NONE', #1033, #37343, #85959 ) ;
#79297=CARTESIAN_POINT ( 'NONE',  ( 50.97905606905900555, -31.62489322948711035, 237.4678068554150059 ) ) ;
#79298=CARTESIAN_POINT ( 'NONE',  ( 112.9469377066634905, -44.85846281290874771, 39.07437081555113423 ) ) ;
#79299=DIRECTION ( 'NONE',  ( 0.000000000000000000, 0.000000000000000000, -1.000000000000000000 ) ) ;
#79300=CARTESIAN_POINT ( 'NONE',  ( 20.03715912545735023, -46.82818131006192175, 180.4678068554150911 ) ) ;
#79301=ORIENTED_EDGE ( 'NONE', *, *, #27908, .T. ) ;
#79302=CARTESIAN_POINT ( 'NONE',  ( 97.31306429104051858, -38.96057676328502595, 66.50610887445193953 ) ) ;
#79303=VECTOR ( 'NONE', #33136, 1000.000000000000000 ) ;
#79304=EDGE_LOOP ( 'NONE', ( #12102, #67280, #25295, #63162 ) ) ;
#79305=ORIENTED_EDGE ( 'NONE', *, *, #66090, .T. ) ;
#79306=CARTESIAN_POINT ( 'NONE',  ( 113.3268105416314171, -43.27322076882862945, 112.5943245899819516 ) ) ;
#79308=VERTEX_POINT ( 'NONE', #11799 ) ;
#79309=CARTESIAN_POINT ( 'NONE',  ( 114.5517459224756038, -44.00510994954048982, 94.21276813305395592 ) ) ;
#79310=DIRECTION ( 'NONE',  ( 0.000000000000000000, 1.000000000000000000, 0.000000000000000000 ) ) ;
#79311=CARTESIAN_POINT ( 'NONE',  ( 80.06648329127398256, -15.97944715994105813, 8.225625275910942946 ) ) ;
#79312=EDGE_CURVE ( 'NONE', #10387, #67090, #79964, .T. ) ;
#79314=CARTESIAN_POINT ( 'NONE',  ( 116.1702204290647984, -31.76348745297265808, 24.21181575210196257 ) ) ;
#79315=VERTEX_POINT ( 'NONE', #88113 ) ;
#79319=CARTESIAN_POINT ( 'NONE',  ( 62.56670390244663338, -48.82844715994099971, 180.4678068554151196 ) ) ;
#79320=DIRECTION ( 'NONE',  ( -3.999999999999999995E-14, 1.000000000000000000, -4.100000000000000342E-29 ) ) ;
#79321=CARTESIAN_POINT ( 'NONE',  ( 97.81170255947417047, -40.51743869465033754, 117.6354096206635518 ) ) ;
#79322=PLANE ( 'NONE',  #16508 ) ;
#79327=CARTESIAN_POINT ( 'NONE',  ( 97.37192905580960200, -32.85904099757679830, 41.02419670448193045 ) ) ;
#79328=ORIENTED_EDGE ( 'NONE', *, *, #31436, .T. ) ;
#79329=ORIENTED_EDGE ( 'NONE', *, *, #41535, .T. ) ;
#79330=CARTESIAN_POINT ( 'NONE',  ( 116.3221839001005264, -32.94216875276463696, 149.1356252759109680 ) ) ;
#79331=CARTESIAN_POINT ( 'NONE',  ( 41.56648329127398966, -27.82844715994070484, 255.9256252759120116 ) ) ;
#79334=CARTESIAN_POINT ( 'NONE',  ( 100.3267271402381624, -32.12451360540737255, 118.6680903695919653 ) ) ;
#79335=AXIS2_PLACEMENT_3D ( 'NONE', #61485, #88329, #12914 ) ;
#79337=VECTOR ( 'NONE', #57974, 1000.000000000000000 ) ;
#79338=EDGE_CURVE ( 'NONE', #88268, #41446, #47040, .T. ) ;
#79341=DIRECTION ( 'NONE',  ( -0.9825752044165969590, -0.1858654558159821002, 0.000000000000000000 ) ) ;
#79342=ORIENTED_EDGE ( 'NONE', *, *, #62188, .F. ) ;
#79344=DIRECTION ( 'NONE',  ( 4.299999999999999979E-14, -1.000000000000000000, 4.400000000000000367E-29 ) ) ;
#79345=ADVANCED_FACE ( 'NONE', ( #59478 ), #32678, .F. ) ;
#79347=VERTEX_POINT ( 'NONE', #10893 ) ;
#79348=CARTESIAN_POINT ( 'NONE',  ( 111.6733053606431412, -27.77132819582071122, 166.1301547344679932 ) ) ;
#79351=AXIS2_PLACEMENT_3D ( 'NONE', #66719, #73531, #39462 ) ;
#79352=CARTESIAN_POINT ( 'NONE',  ( 102.3028228262999164, -26.72980997527264790, 136.4422919425779526 ) ) ;
#79353=CARTESIAN_POINT ( 'NONE',  ( 132.3254539024480039, -42.97311385573998876, 231.5838068554170093 ) ) ;
#79354=CARTESIAN_POINT ( 'NONE',  ( 110.8543047535783330, -45.98430580984275906, 17.88561088277840838 ) ) ;
#79355=ORIENTED_EDGE ( 'NONE', *, *, #58478, .F. ) ;
#79358=ORIENTED_EDGE ( 'NONE', *, *, #66622, .F. ) ;
#79359=EDGE_LOOP ( 'NONE', ( #9151, #2331, #42211, #54962 ) ) ;
#79362=CARTESIAN_POINT ( 'NONE',  ( 100.9764986820135420, -31.29420903488464845, 188.5652332267349607 ) ) ;
#79363=CARTESIAN_POINT ( 'NONE',  ( 110.3610989901968651, -25.31982300743893077, 64.85276813305395649 ) ) ;
#79364=ORIENTED_EDGE ( 'NONE', *, *, #33753, .F. ) ;
#79365=CARTESIAN_POINT ( 'NONE',  ( 96.85498737197825392, -38.89503640450125488, 31.49276813305495892 ) ) ;
#79366=DIRECTION ( 'NONE',  ( -0.7071067708032359178, -0.0001211784769794170747, 0.7071067811865451302 ) ) ;
#79368=CARTESIAN_POINT ( 'NONE',  ( 112.4860951546057919, -26.19083136796355404, 165.6984824187679521 ) ) ;
#79369=CARTESIAN_POINT ( 'NONE',  ( 116.3259679314843282, -32.93868236591013243, 264.1356252759109680 ) ) ;
#79371=DIRECTION ( 'NONE',  ( 1.000000000000000000, 6.831565154159360295E-14, 0.000000000000000000 ) ) ;
#79372=ORIENTED_EDGE ( 'NONE', *, *, #40964, .F. ) ;
#79375=VERTEX_POINT ( 'NONE', #59919 ) ;
#79376=VECTOR ( 'NONE', #842, 1000.000000000000000 ) ;
#79378=CARTESIAN_POINT ( 'NONE',  ( 194.5667039024479834, -67.87844715994100397, 310.9178068554150514 ) ) ;
#79379=CARTESIAN_POINT ( 'NONE',  ( 98.58988425959138624, -43.82355431373886034, 71.86895860924397539 ) ) ;
#79381=DIRECTION ( 'NONE',  ( 6.745093096447288888E-17, 1.000000000000000000, 0.000000000000000000 ) ) ;
#79382=CARTESIAN_POINT ( 'NONE',  ( 182.5667039024480118, -32.29483332968450782, -5.074374724088000832 ) ) ;
#79383=CARTESIAN_POINT ( 'NONE',  ( 100.8224265971272615, -29.20115443902020047, 40.62705384733994407 ) ) ;
#79384=LINE ( 'NONE', #51640, #56472 ) ;
#79385=CARTESIAN_POINT ( 'NONE',  ( 99.30484619187392070, -29.80227926343066613, 186.7470538473389752 ) ) ;
#79387=DIRECTION ( 'NONE',  ( 0.000000000000000000, -1.000000000000000000, 0.000000000000000000 ) ) ;
#79389=CARTESIAN_POINT ( 'NONE',  ( 41.56648329127398966, -27.82844715994070484, 138.9256252759119832 ) ) ;
#79392=DIRECTION ( 'NONE',  ( 0.7071067812123270624, 0.7071067811607679721, 0.000000000000000000 ) ) ;
#79393=CARTESIAN_POINT ( 'NONE',  ( 107.6569944592711607, -47.81385874506208467, 197.6308633711489620 ) ) ;
#79396=CARTESIAN_POINT ( 'NONE',  ( 115.8254250420262252, -31.73000087149041448, 144.2397934866363016 ) ) ;
#79397=CARTESIAN_POINT ( 'NONE',  ( 109.9953477121747767, -26.70153551007575388, 255.8499109901966051 ) ) ;
#79398=CARTESIAN_POINT ( 'NONE',  ( 101.6884573362309823, -27.70642928270265060, 81.50419670448295051 ) ) ;
#79405=ORIENTED_EDGE ( 'NONE', *, *, #72041, .F. ) ;
#79406=AXIS2_PLACEMENT_3D ( 'NONE', #26868, #68217, #74130 ) ;
#79407=VECTOR ( 'NONE', #81689, 1000.000000000000000 ) ;
#79408=VECTOR ( 'NONE', #76530, 999.9999999999998863 ) ;
#79410=ORIENTED_EDGE ( 'NONE', *, *, #17976, .T. ) ;
#79411=ORIENTED_EDGE ( 'NONE', *, *, #86926, .T. ) ;
#79413=CARTESIAN_POINT ( 'NONE',  ( 97.22385571422852024, -40.27120027895552568, 262.6013395616254797 ) ) ;
#79414=CARTESIAN_POINT ( 'NONE',  ( 193.0374249753376432, -23.42844715993431848, 180.4678068554150343 ) ) ;
#79415=CARTESIAN_POINT ( 'NONE',  ( 138.0667039024479266, -14.72944715994091069, 239.5838068554170377 ) ) ;
#79416=AXIS2_PLACEMENT_3D ( 'NONE', #43027, #8540, #29429 ) ;
#79417=AXIS2_PLACEMENT_3D ( 'NONE', #81565, #48783, #75629 ) ;
#79418=CARTESIAN_POINT ( 'NONE',  ( 134.0664832912740110, -46.72944715994100306, 8.225625275910998013 ) ) ;
#79421=CIRCLE ( 'NONE', #5428, 13.49999999999999822 ) ;
#79422=CARTESIAN_POINT ( 'NONE',  ( 106.4400806841681231, -45.24788313703638210, 221.9409912566479477 ) ) ;
#79423=ORIENTED_EDGE ( 'NONE', *, *, #41478, .F. ) ;
#79425=ORIENTED_EDGE ( 'NONE', *, *, #7364, .F. ) ;
#79426=AXIS2_PLACEMENT_3D ( 'NONE', #68703, #53241, #68262 ) ;
#79427=EDGE_CURVE ( 'NONE', #34489, #1069, #76053, .T. ) ;
#79428=DIRECTION ( 'NONE',  ( -0.9999999853157766072, -0.0001713722456143218888, 0.000000000000000000 ) ) ;
#79430=CARTESIAN_POINT ( 'NONE',  ( 100.6687104580203567, -44.89077600156390702, 273.0594347997199520 ) ) ;
#79431=FACE_OUTER_BOUND ( 'NONE', #79028, .T. ) ;
#79432=CARTESIAN_POINT ( 'NONE',  ( 116.3149231129805941, -32.94053081170188335, 174.1356252759109680 ) ) ;
#79433=CARTESIAN_POINT ( 'NONE',  ( 98.30750624414157812, -41.72880715729390744, 26.73978606779152756 ) ) ;
#79435=CARTESIAN_POINT ( 'NONE',  ( 103.2943085291411478, -27.46819606563682470, 56.38426792498484730 ) ) ;
#79436=ORIENTED_EDGE ( 'NONE', *, *, #65994, .F. ) ;
#79437=CIRCLE ( 'NONE', #19967, 13.16666666666670160 ) ;
#79439=CARTESIAN_POINT ( 'NONE',  ( 115.1548909598205057, -41.51005587062507374, 279.8453928297065545 ) ) ;
#79440=AXIS2_PLACEMENT_3D ( 'NONE', #4316, #66526, #32003 ) ;
#79441=LINE ( 'NONE', #58953, #53647 ) ;
#79442=CARTESIAN_POINT ( 'NONE',  ( 192.5667039024474434, -23.42844715993433624, 180.4678068554150343 ) ) ;
#79443=EDGE_CURVE ( 'NONE', #8508, #85887, #79516, .T. ) ;
#79447=FACE_OUTER_BOUND ( 'NONE', #61342, .T. ) ;
#79450=CARTESIAN_POINT ( 'NONE',  ( 113.4154522487949919, -27.68126056648907252, 84.57753003781698453 ) ) ;
#79451=ORIENTED_EDGE ( 'NONE', *, *, #16283, .F. ) ;
#79452=EDGE_CURVE ( 'NONE', #23895, #12725, #20944, .T. ) ;
#79453=CARTESIAN_POINT ( 'NONE',  ( 106.1832117796525807, -28.23380338452170335, 49.58099125664799800 ) ) ;
#79454=CARTESIAN_POINT ( 'NONE',  ( 116.7800429006774436, -34.22024395345221137, 90.02721173792870957 ) ) ;
#79455=CARTESIAN_POINT ( 'NONE',  ( 117.0765951205083439, -35.60322954364740156, 80.34729759161096752 ) ) ;
#79456=PLANE ( 'NONE',  #31714 ) ;
#79459=VECTOR ( 'NONE', #58440, 1000.000000000000000 ) ;
#79461=CARTESIAN_POINT ( 'NONE',  ( 96.66758392153232649, -32.91525239269808623, 17.03467289495896964 ) ) ;
#79463=ORIENTED_EDGE ( 'NONE', *, *, #9282, .T. ) ;
#79465=AXIS2_PLACEMENT_3D ( 'NONE', #23661, #86769, #37274 ) ;
#79467=VECTOR ( 'NONE', #3293, 1000.000000000000000 ) ;
#79468=CARTESIAN_POINT ( 'NONE',  ( 78.35735255114366282, -20.88611802719123389, 2.101554303218999831 ) ) ;
#79469=ORIENTED_EDGE ( 'NONE', *, *, #28591, .F. ) ;
#79472=DIRECTION ( 'NONE',  ( 0.000000000000000000, 1.000000000000000000, 0.000000000000000000 ) ) ;
#79474=CARTESIAN_POINT ( 'NONE',  ( 63.03715912545737865, -24.89890238295017966, 249.9678068554150343 ) ) ;
#79475=CARTESIAN_POINT ( 'NONE',  ( 97.32398421004032230, -35.86507053846867166, 231.2556252759109725 ) ) ;
#79478=CARTESIAN_POINT ( 'NONE',  ( 106.9273518165185948, -26.26990724610170247, 56.08705384733997334 ) ) ;
#79479=CARTESIAN_POINT ( 'NONE',  ( 116.8171323280760276, -34.15294143710698904, 45.03145662157326967 ) ) ;
#79481=CARTESIAN_POINT ( 'NONE',  ( 97.81170986510684884, -40.51745644794008427, 172.6354259520616097 ) ) ;
#79482=CARTESIAN_POINT ( 'NONE',  ( 51.34673845256558167, -29.62846900982264842, 237.4678068554150059 ) ) ;
#79483=EDGE_LOOP ( 'NONE', ( #44442, #26559 ) ) ;
#79486=CARTESIAN_POINT ( 'NONE',  ( 101.9927635143278621, -45.44554184246400297, 113.1570561696343447 ) ) ;
#79487=CARTESIAN_POINT ( 'NONE',  ( 100.8363305107023251, -45.83159080358284854, 242.1108633711489517 ) ) ;
#79490=CARTESIAN_POINT ( 'NONE',  ( 127.0667039024477560, -15.72944715994076681, 239.5838068554164408 ) ) ;
#79491=CARTESIAN_POINT ( 'NONE',  ( 101.7992505034292350, -28.57304559719056058, 219.9552769709339657 ) ) ;
#79493=CARTESIAN_POINT ( 'NONE',  ( 96.05879824974444148, -41.05137697672054742, 92.62419670448296927 ) ) ;
#79495=CARTESIAN_POINT ( 'NONE',  ( 98.41978056949241704, -42.69487473605161654, 126.8070538473389490 ) ) ;
#79496=VERTEX_POINT ( 'NONE', #14836 ) ;
#79497=DIRECTION ( 'NONE',  ( 0.000000000000000000, 1.000000000000000000, 0.000000000000000000 ) ) ;
#79499=CARTESIAN_POINT ( 'NONE',  ( 51.34673845256575930, -36.02818131005845004, 313.9678068554150059 ) ) ;
#79500=FACE_OUTER_BOUND ( 'NONE', #42324, .T. ) ;
#79501=CARTESIAN_POINT ( 'NONE',  ( 135.1485260852069530, -34.20116861175128520, 1.807989644435019416 ) ) ;
#79503=DIRECTION ( 'NONE',  ( 0.7071067811865774377, -0.7071067811865175967, 7.071067811865782003E-16 ) ) ;
#79504=VERTEX_POINT ( 'NONE', #48867 ) ;
#79506=DIRECTION ( 'NONE',  ( 0.7071067811575828532, -0.7071067812155121812, 0.000000000000000000 ) ) ;
#79510=LINE ( 'NONE', #25866, #69887 ) ;
#79511=ORIENTED_EDGE ( 'NONE', *, *, #63136, .T. ) ;
#79512=CARTESIAN_POINT ( 'NONE',  ( 96.06419827846988824, -38.01208726283962847, 86.43086337114897333 ) ) ;
#79513=CARTESIAN_POINT ( 'NONE',  ( 131.0667039024480118, -64.87844715994098976, 237.1838068554150141 ) ) ;
#79514=ADVANCED_FACE ( 'NONE', ( #56126, #36161 ), #81749, .T. ) ;
#79516=LINE ( 'NONE', #12242, #65923 ) ;
#79518=VERTEX_POINT ( 'NONE', #8006 ) ;
#79519=DIRECTION ( 'NONE',  ( 0.000000000000000000, 0.000000000000000000, -1.000000000000000000 ) ) ;
#79523=DIRECTION ( 'NONE',  ( 1.000000000000000078E-15, 0.000000000000000000, -1.000000000000000000 ) ) ;
#79525=DIRECTION ( 'NONE',  ( 0.000000000000000000, 1.000000000000000000, 0.000000000000000000 ) ) ;
#79526=VECTOR ( 'NONE', #9243, 1000.000000000000000 ) ;
#79527=ORIENTED_EDGE ( 'NONE', *, *, #24465, .T. ) ;
#79528=AXIS2_PLACEMENT_3D ( 'NONE', #3969, #52969, #74799 ) ;
#79529=ADVANCED_FACE ( 'NONE', ( #29357 ), #77957, .F. ) ;
#79531=CARTESIAN_POINT ( 'NONE',  ( 117.1170091337236414, -34.17489915221372598, 165.0365776568629315 ) ) ;
#79535=CARTESIAN_POINT ( 'NONE',  ( 114.3402351757609097, -43.26825200597433962, 34.24419670448197905 ) ) ;
#79536=CARTESIAN_POINT ( 'NONE',  ( 160.5667039024483529, -48.82844715993552143, 300.4678068554149490 ) ) ;
#79538=DIRECTION ( 'NONE',  ( -4.237773401492740281E-14, 1.000000000000000000, 0.000000000000000000 ) ) ;
#79539=AXIS2_PLACEMENT_3D ( 'NONE', #61082, #18860, #74279 ) ;
#79540=VERTEX_POINT ( 'NONE', #22106 ) ;
#79542=AXIS2_PLACEMENT_3D ( 'NONE', #55815, #6797, #888 ) ;
#79544=VERTEX_POINT ( 'NONE', #15277 ) ;
#79545=ORIENTED_EDGE ( 'NONE', *, *, #66302, .F. ) ;
#79546=CARTESIAN_POINT ( 'NONE',  ( 113.7804517773139708, -30.94577135814159519, 180.8244404487539612 ) ) ;
#79548=CARTESIAN_POINT ( 'NONE',  ( 105.0852382675896024, -45.91373775275845759, 28.85110711542093753 ) ) ;
#79550=CARTESIAN_POINT ( 'NONE',  ( 99.09570908192057459, -30.55043174579301635, 80.80229194183452535 ) ) ;
#79551=AXIS2_PLACEMENT_3D ( 'NONE', #79137, #71428, #8295 ) ;
#79553=ORIENTED_EDGE ( 'NONE', *, *, #70395, .T. ) ;
#79555=CARTESIAN_POINT ( 'NONE',  ( 50.88849390559467878, -32.11662333284566273, 237.4678068554150059 ) ) ;
#79556=ORIENTED_EDGE ( 'NONE', *, *, #7078, .F. ) ;
#79557=CARTESIAN_POINT ( 'NONE',  ( 100.1532602078032568, -44.50350736857021161, 266.9984824187679919 ) ) ;
#79562=DIRECTION ( 'NONE',  ( -1.000000000000000000, 6.036837696399408848E-13, 0.000000000000000000 ) ) ;
#79563=DIRECTION ( 'NONE',  ( 0.000000000000000000, 0.000000000000000000, 1.000000000000000000 ) ) ;
#79564=CARTESIAN_POINT ( 'NONE',  ( 69.67078994678415427, -0.9293259921821603875, 540.9756252759101471 ) ) ;
#79566=VECTOR ( 'NONE', #68348, 1000.000000000000000 ) ;
#79567=CARTESIAN_POINT ( 'NONE',  ( 113.2457357650714727, -45.17988020286173878, 224.0784824187679476 ) ) ;
#79568=CARTESIAN_POINT ( 'NONE',  ( 182.2420472961728137, -31.76306994223154589, 313.9678068554149490 ) ) ;
#79570=CARTESIAN_POINT ( 'NONE',  ( 116.7853252867327996, -32.83880582269000570, 50.12991099019698282 ) ) ;
#79572=CARTESIAN_POINT ( 'NONE',  ( 97.77253489752784787, -40.53345146323919579, 11.63562527591094309 ) ) ;
#79573=VERTEX_POINT ( 'NONE', #53988 ) ;
#79575=CARTESIAN_POINT ( 'NONE',  ( 80.25489464535442607, -15.97944715994106524, 1.625625275910945078 ) ) ;
#79577=EDGE_CURVE ( 'NONE', #59850, #41003, #80411, .T. ) ;
#79578=DIRECTION ( 'NONE',  ( -1.000000000000000078E-15, 1.000000000000000083E-30, 1.000000000000000000 ) ) ;
#79579=CARTESIAN_POINT ( 'NONE',  ( 104.7498880507309451, -44.55652276380406818, 105.1652332267339602 ) ) ;
#79580=CARTESIAN_POINT ( 'NONE',  ( 96.78746529907793672, -40.85582509469530521, 247.6422919425769749 ) ) ;
#79584=CARTESIAN_POINT ( 'NONE',  ( 136.3243469132048062, -38.30306751046402525, 2.518077574340959579 ) ) ;
#79585=VERTEX_POINT ( 'NONE', #7566 ) ;
#79586=ORIENTED_EDGE ( 'NONE', *, *, #4246, .F. ) ;
#79587=VECTOR ( 'NONE', #72363, 1000.000000000000000 ) ;
#79590=ORIENTED_EDGE ( 'NONE', *, *, #60236, .F. ) ;
#79591=EDGE_LOOP ( 'NONE', ( #88978, #70810, #49928, #69923 ) ) ;
#79592=CARTESIAN_POINT ( 'NONE',  ( 99.04438571895173027, -42.84170729117609255, 167.8444702960626387 ) ) ;
#79593=CARTESIAN_POINT ( 'NONE',  ( 107.0664832912739968, 0.2215528400590083269, 333.4006252759110112 ) ) ;
#79594=CARTESIAN_POINT ( 'NONE',  ( 100.9546606413581458, -28.70703445851304991, 41.59391690566671684 ) ) ;
#79595=CARTESIAN_POINT ( 'NONE',  ( 103.2107857629706018, -44.35110894017614669, 126.6267055423619610 ) ) ;
#79596=CARTESIAN_POINT ( 'NONE',  ( 99.73113825573250324, -44.24905506706784308, 21.96133956162593748 ) ) ;
#79597=VECTOR ( 'NONE', #69727, 1000.000000000000000 ) ;
#79601=CARTESIAN_POINT ( 'NONE',  ( 176.7669697523291461, -48.62818131005361977, 249.9678068554149775 ) ) ;
#79602=ORIENTED_EDGE ( 'NONE', *, *, #36074, .T. ) ;
#79603=DIRECTION ( 'NONE',  ( 2.900000000000000265E-14, -2.000000000000000155E-15, 1.000000000000000000 ) ) ;
#79604=AXIS2_PLACEMENT_3D ( 'NONE', #15263, #57476, #56577 ) ;
#79605=CARTESIAN_POINT ( 'NONE',  ( 116.7945501114407278, -39.38987908835133567, 33.61483829906352838 ) ) ;
#79607=DIRECTION ( 'NONE',  ( 0.7071067811865779928, -0.7071067811865171526, 7.071067811865785947E-16 ) ) ;
#79609=CARTESIAN_POINT ( 'NONE',  ( 117.4915365000037042, -36.80222117025145678, 263.8213395616251660 ) ) ;
#79610=CARTESIAN_POINT ( 'NONE',  ( 110.2975601020867202, -46.68703778808450267, 8.827053847339950465 ) ) ;
#79615=CARTESIAN_POINT ( 'NONE',  ( 105.6195873783703831, -25.36179723890650450, 323.1871736463168645 ) ) ;
#79616=CARTESIAN_POINT ( 'NONE',  ( 49.21213752016101495, -29.73316016639650172, -5.074374724088000832 ) ) ;
#79617=CARTESIAN_POINT ( 'NONE',  ( 131.6545875264125129, -38.05177997655169264, 7.178113714837632386 ) ) ;
#79618=VECTOR ( 'NONE', #79927, 1000.000000000000000 ) ;
#79621=CARTESIAN_POINT ( 'NONE',  ( 34.33598329127499227, -36.32844715994100682, -5.074374724088000832 ) ) ;
#79622=CARTESIAN_POINT ( 'NONE',  ( 112.2192032947272509, -26.89661630634724432, 14.68038718067299442 ) ) ;
#79623=CARTESIAN_POINT ( 'NONE',  ( 114.3439067968150624, -29.21543093042305728, 170.4641967044829585 ) ) ;
#79624=CARTESIAN_POINT ( 'NONE',  ( 115.7467025339723250, -43.60978142820201242, 44.30514908543492680 ) ) ;
#79625=CARTESIAN_POINT ( 'NONE',  ( 167.2371591254545535, -47.82818131005522133, 129.9678068554149775 ) ) ;
#79626=DIRECTION ( 'NONE',  ( 1.000000000000000000, 3.999999999999999995E-14, 1.000000000000000078E-15 ) ) ;
#79627=CYLINDRICAL_SURFACE ( 'NONE', #45016, 3.250000000000002665 ) ;
#79628=VECTOR ( 'NONE', #17194, 1000.000000000000000 ) ;
#79629=EDGE_CURVE ( 'NONE', #89037, #28914, #71145, .T. ) ;
#79632=CARTESIAN_POINT ( 'NONE',  ( 108.4174892967461403, -26.73503593441724391, 185.9689586056932740 ) ) ;
#79633=EDGE_LOOP ( 'NONE', ( #55818, #41168, #44890, #2675 ) ) ;
#79634=CARTESIAN_POINT ( 'NONE',  ( 97.30000116515917341, -37.25789978020652171, 72.36991099019596163 ) ) ;
#79637=VERTEX_POINT ( 'NONE', #69790 ) ;
#79638=CARTESIAN_POINT ( 'NONE',  ( 105.7151186495713944, -46.72380402441561387, 48.46893004826933549 ) ) ;
#79639=CARTESIAN_POINT ( 'NONE',  ( 103.3114313307234085, -27.02747569519259230, 211.3699109901969848 ) ) ;
#79640=DIRECTION ( 'NONE',  ( 0.000000000000000000, 0.000000000000000000, 1.000000000000000000 ) ) ;
#79641=CARTESIAN_POINT ( 'NONE',  ( 108.3332376935612871, -46.73488331510854010, 147.6773181741651513 ) ) ;
#79643=CARTESIAN_POINT ( 'NONE',  ( 151.0371591254575492, -24.95799193692592155, 180.4678068554149775 ) ) ;
#79646=ADVANCED_FACE ( 'NONE', ( #77058, #15726 ), #33130, .F. ) ;
#79648=CARTESIAN_POINT ( 'NONE',  ( 107.0664832912739968, -36.72944715994100306, 287.6356252759109680 ) ) ;
#79649=CARTESIAN_POINT ( 'NONE',  ( 113.6473777113568531, -44.00994186338857617, 133.1613395616259936 ) ) ;
#79651=ORIENTED_EDGE ( 'NONE', *, *, #48026, .F. ) ;
#79654=CARTESIAN_POINT ( 'NONE',  ( 104.3250142303409831, -45.18796221723782480, 78.75872616303996665 ) ) ;
#79655=AXIS2_PLACEMENT_3D ( 'NONE', #48126, #83140, #902 ) ;
#79656=CARTESIAN_POINT ( 'NONE',  ( 107.0664832912739541, -23.22944715994095688, 315.6356252759111953 ) ) ;
#79657=CARTESIAN_POINT ( 'NONE',  ( 114.7458293810856418, -30.61868467657538062, 240.3613395616249875 ) ) ;
#79658=DIRECTION ( 'NONE',  ( 0.000000000000000000, 0.000000000000000000, -1.000000000000000000 ) ) ;
#79660=EDGE_CURVE ( 'NONE', #22927, #31607, #34021, .T. ) ;
#79661=DIRECTION ( 'NONE',  ( 1.000000000000000000, 0.000000000000000000, 0.000000000000000000 ) ) ;
#79663=AXIS2_PLACEMENT_3D ( 'NONE', #559, #36882, #70060 ) ;
#79664=DIRECTION ( 'NONE',  ( 0.000000000000000000, 0.000000000000000000, -1.000000000000000000 ) ) ;
#79665=DIRECTION ( 'NONE',  ( -1.000000000000000000, -6.514610998690690188E-14, -1.000000000000000078E-15 ) ) ;
#79667=CARTESIAN_POINT ( 'NONE',  ( 117.1049515565469221, -33.87427183379790563, 149.0470538473389581 ) ) ;
#79669=ADVANCED_FACE ( 'NONE', ( #85671 ), #86556, .T. ) ;
#79671=CIRCLE ( 'NONE', #1329, 2.030000000001310312 ) ;
#79673=CARTESIAN_POINT ( 'NONE',  ( 115.8254323941762891, -31.73001883427092196, 150.2397919421048300 ) ) ;
#79674=AXIS2_PLACEMENT_3D ( 'NONE', #70219, #7991, #78399 ) ;
#79675=CARTESIAN_POINT ( 'NONE',  ( 194.0371591254572934, -24.89890238294407965, 300.4678068554149490 ) ) ;
#79676=DIRECTION ( 'NONE',  ( 9.351236661543306751E-17, -3.725950533538267725E-29, -1.000000000000000000 ) ) ;
#79677=CARTESIAN_POINT ( 'NONE',  ( 115.0372528418681242, -42.90846878759241179, 269.3022913304283747 ) ) ;
#79678=CARTESIAN_POINT ( 'NONE',  ( 117.4575111195971857, -40.49848259682686802, 173.5375300378159693 ) ) ;
#79679=CARTESIAN_POINT ( 'NONE',  ( 136.1600792929918953, -38.51483178663133344, 7.477467810854448338 ) ) ;
#79682=ORIENTED_EDGE ( 'NONE', *, *, #21315, .T. ) ;
#79683=CIRCLE ( 'NONE', #21657, 11.45913725231036118 ) ;
#79684=EDGE_CURVE ( 'NONE', #43506, #56405, #50673, .T. ) ;
#79685=CARTESIAN_POINT ( 'NONE',  ( 100.1576839525979352, -44.03386264563039987, 62.97446275362836587 ) ) ;
#79686=DIRECTION ( 'NONE',  ( 1.000000000000000078E-15, -1.000000000000000083E-30, -1.000000000000000000 ) ) ;
#79687=EDGE_CURVE ( 'NONE', #9211, #82640, #39856, .T. ) ;
#79688=CARTESIAN_POINT ( 'NONE',  ( 132.9844404253386472, -34.20116865955331065, 8.043260881866558520 ) ) ;
#79689=EDGE_CURVE ( 'NONE', #1932, #59530, #10239, .T. ) ;
#79690=CARTESIAN_POINT ( 'NONE',  ( 100.5340721669357009, -30.74146890971161739, 272.1672975916113160 ) ) ;
#79691=DIRECTION ( 'NONE',  ( 0.000000000000000000, 1.000000000000000000, 0.000000000000000000 ) ) ;
#79693=ADVANCED_FACE ( 'NONE', ( #57938 ), #18073, .F. ) ;
#79694=CARTESIAN_POINT ( 'NONE',  ( 114.6673900882561554, -41.57871802750004520, 9.635625275910941312 ) ) ;
#79695=VECTOR ( 'NONE', #77528, 1000.000000000000000 ) ;
#79698=ORIENTED_EDGE ( 'NONE', *, *, #84700, .F. ) ;
#79699=CARTESIAN_POINT ( 'NONE',  ( 116.3212776292296127, -32.94146857471318413, 287.6356252759109680 ) ) ;
#79702=CARTESIAN_POINT ( 'NONE',  ( 109.7226905202563501, -27.00022865876924172, 155.8647339722907645 ) ) ;
#79703=CARTESIAN_POINT ( 'NONE',  ( 98.56427472769081533, -33.61093641167653345, 20.45718173283900398 ) ) ;
#79704=CARTESIAN_POINT ( 'NONE',  ( 113.0348518357461955, -45.34727401701223926, 203.0584824187679374 ) ) ;
#79705=CARTESIAN_POINT ( 'NONE',  ( 117.2167691715783064, -39.01263929987995027, 148.6499109901969859 ) ) ;
#79706=PLANE ( 'NONE',  #32189 ) ;
#79707=CARTESIAN_POINT ( 'NONE',  ( 99.38154727845876835, -29.68499927947409489, 271.7356252759109907 ) ) ;
#79708=DIRECTION ( 'NONE',  ( -4.163336342344333240E-14, -1.000000000000000000, 0.000000000000000000 ) ) ;
#79709=FACE_OUTER_BOUND ( 'NONE', #45092, .T. ) ;
#79711=VECTOR ( 'NONE', #34803, 1000.000000000000000 ) ;
#79713=VECTOR ( 'NONE', #229, 1000.000000000000000 ) ;
#79714=CARTESIAN_POINT ( 'NONE',  ( 97.72299786849482928, -41.53060059208619492, 196.7041967044819728 ) ) ;
#79716=CARTESIAN_POINT ( 'NONE',  ( 102.6834449319766378, -27.27027144519976787, 180.4213395616249898 ) ) ;
#79717=CARTESIAN_POINT ( 'NONE',  ( 102.0662944402908749, -27.97094399341936821, 265.4898263988108624 ) ) ;
#79718=DIRECTION ( 'NONE',  ( 0.000000000000000000, 0.000000000000000000, -1.000000000000000000 ) ) ;
#79719=CARTESIAN_POINT ( 'NONE',  ( 100.1253875378072848, -39.57043109886186727, 9.635625275910941312 ) ) ;
#79723=CARTESIAN_POINT ( 'NONE',  ( 113.7419942178972576, -29.10023054337259296, 285.5032443235299979 ) ) ;
#79724=CARTESIAN_POINT ( 'NONE',  ( 41.56648329127399677, 0.2215528400590013880, 16.80862527591200006 ) ) ;
#79726=CARTESIAN_POINT ( 'NONE',  ( 25.56670390244797275, -65.37844715994100397, 293.2178068554150627 ) ) ;
#79727=CIRCLE ( 'NONE', #40534, 3.000000000000002665 ) ;
#79731=CARTESIAN_POINT ( 'NONE',  ( 127.0664832912740394, -46.72944715994101017, -4.824374724089008915 ) ) ;
#79732=CARTESIAN_POINT ( 'NONE',  ( 101.7839708215018106, -42.86206951696545531, 195.5838068554171798 ) ) ;
#79734=CARTESIAN_POINT ( 'NONE',  ( 136.5146477271300682, -19.98222059078257473, 7.138441653512620277 ) ) ;
#79735=CARTESIAN_POINT ( 'NONE',  ( 117.4357963365922615, -35.45519799489562729, 193.9241967044829664 ) ) ;
#79736=CARTESIAN_POINT ( 'NONE',  ( 116.2315886754559386, -31.76121500512346074, 65.22133956162595325 ) ) ;
#79737=CARTESIAN_POINT ( 'NONE',  ( 103.8062037941931095, -48.17417041148343060, 213.3556252759109668 ) ) ;
#79738=DIRECTION ( 'NONE',  ( 1.000000000000000078E-15, -1.000000000000000083E-30, -1.000000000000000000 ) ) ;
#79740=CARTESIAN_POINT ( 'NONE',  ( 83.06670390244804025, -42.97311385574013798, 207.5838068554169809 ) ) ;
#79741=DIRECTION ( 'NONE',  ( 0.000000000000000000, 0.000000000000000000, 1.000000000000000000 ) ) ;
#79742=CARTESIAN_POINT ( 'NONE',  ( 109.7368013281214445, -46.41511743547308555, 38.79047438361208577 ) ) ;
#79745=CARTESIAN_POINT ( 'NONE',  ( 104.4917770246300535, -26.97830201417560403, 65.28281118898505042 ) ) ;
#79747=EDGE_CURVE ( 'NONE', #61299, #37060, #71591, .T. ) ;
#79748=EDGE_LOOP ( 'NONE', ( #34452, #18533, #34987, #18561, #42227 ) ) ;
#79750=CARTESIAN_POINT ( 'NONE',  ( 112.1857315011839802, -29.85591823435125747, 103.9895626852199655 ) ) ;
#79753=ORIENTED_EDGE ( 'NONE', *, *, #47618, .T. ) ;
#79754=CARTESIAN_POINT ( 'NONE',  ( 98.35456548258461851, -42.41549619454038123, 97.78705384733993355 ) ) ;
#79755=LINE ( 'NONE', #51996, #22340 ) ;
#79758=EDGE_CURVE ( 'NONE', #44882, #2509, #13877, .T. ) ;
#79759=CARTESIAN_POINT ( 'NONE',  ( 107.0667039024479834, -36.72944715994100306, 239.5838068554170093 ) ) ;
#79760=CARTESIAN_POINT ( 'NONE',  ( 110.3395589168170972, -45.98151452052003663, 37.84705384733994293 ) ) ;
#79763=EDGE_LOOP ( 'NONE', ( #86709, #65925, #22361, #47662 ) ) ;
#79767=CARTESIAN_POINT ( 'NONE',  ( 73.10937651008742932, -46.62589376934775487, -5.074374724089109279 ) ) ;
#79768=DIRECTION ( 'NONE',  ( 0.000000000000000000, -1.000000000000000000, 0.000000000000000000 ) ) ;
#79770=CARTESIAN_POINT ( 'NONE',  ( 50.96943157743499597, -34.03355364505720360, -5.074374724088000832 ) ) ;
#79771=EDGE_CURVE ( 'NONE', #61198, #11064, #60146, .T. ) ;
#79772=CARTESIAN_POINT ( 'NONE',  ( 116.3181333158508295, -32.94392590426259204, 50.13562527591097506 ) ) ;
#79773=DIRECTION ( 'NONE',  ( 1.000000000000000000, 4.163336342344333240E-14, 0.000000000000000000 ) ) ;
#79774=CIRCLE ( 'NONE', #34744, 2.500000000000002220 ) ;
#79776=CARTESIAN_POINT ( 'NONE',  ( 103.4847015977353379, -25.45917443855071838, 55.32133956162594046 ) ) ;
#79778=EDGE_CURVE ( 'NONE', #28741, #24002, #87881, .T. ) ;
#79780=CIRCLE ( 'NONE', #2865, 4.875000000000017764 ) ;
#79781=DIRECTION ( 'NONE',  ( 1.000000000000000000, 4.163336342344333240E-14, 0.000000000000000000 ) ) ;
#79782=CARTESIAN_POINT ( 'NONE',  ( 163.0667039024466760, -32.29483332967941323, 237.4678068554150059 ) ) ;
#79784=CARTESIAN_POINT ( 'NONE',  ( 103.9214495108435017, -28.66658863671924706, 168.1785665600669688 ) ) ;
#79786=AXIS2_PLACEMENT_3D ( 'NONE', #51528, #44718, #86973 ) ;
#79790=VERTEX_POINT ( 'NONE', #18837 ) ;
#79791=AXIS2_PLACEMENT_3D ( 'NONE', #42335, #22827, #50955 ) ;
#79792=CARTESIAN_POINT ( 'NONE',  ( 127.0664832912740394, -54.72944906728950798, -5.074374724089008915 ) ) ;
#79793=EDGE_LOOP ( 'NONE', ( #56735, #70507, #50575, #57735 ) ) ;
#79796=ADVANCED_FACE ( 'NONE', ( #12029 ), #5208, .F. ) ;
#79797=CARTESIAN_POINT ( 'NONE',  ( 109.0147404159584568, -27.53810233378435157, 181.3539642582779550 ) ) ;
#79800=EDGE_CURVE ( 'NONE', #89348, #14315, #42014, .T. ) ;
#79801=CARTESIAN_POINT ( 'NONE',  ( 164.7812970173289955, -35.65087443492610930, -5.074374724088000832 ) ) ;
#79802=CARTESIAN_POINT ( 'NONE',  ( 100.8872678004313457, -44.70005588500947624, 17.05233985846918898 ) ) ;
#79803=ORIENTED_EDGE ( 'NONE', *, *, #22516, .F. ) ;
#79804=ORIENTED_EDGE ( 'NONE', *, *, #62778, .T. ) ;
#79807=CARTESIAN_POINT ( 'NONE',  ( 104.1201707603140107, -29.11702517433068138, 213.1880903695919756 ) ) ;
#79808=CARTESIAN_POINT ( 'NONE',  ( 117.3753987692272602, -38.63066374137464720, 88.68133956162493803 ) ) ;
#79809=CARTESIAN_POINT ( 'NONE',  ( 117.4328057974123567, -37.95573561897359838, 53.73276813305394484 ) ) ;
#79810=CARTESIAN_POINT ( 'NONE',  ( 101.9926078131534979, -45.44544624334183425, 252.1566658911062007 ) ) ;
#79811=CARTESIAN_POINT ( 'NONE',  ( 134.5667039024480118, -50.82844715994100682, 104.9178068554150087 ) ) ;
#79812=DIRECTION ( 'NONE',  ( 0.000000000000000000, 0.000000000000000000, -1.000000000000000000 ) ) ;
#79813=CARTESIAN_POINT ( 'NONE',  ( 96.61884675261427446, -36.21154414529181764, 167.2870538473399620 ) ) ;
#79814=DIRECTION ( 'NONE',  ( 1.000000000000000078E-15, -1.000000000000000083E-30, -1.000000000000000000 ) ) ;
#79815=EDGE_LOOP ( 'NONE', ( #32393, #57049, #72237, #51054 ) ) ;
#79817=ORIENTED_EDGE ( 'NONE', *, *, #38592, .T. ) ;
#79818=ORIENTED_EDGE ( 'NONE', *, *, #52082, .T. ) ;
#79819=LINE ( 'NONE', #17574, #1285 ) ;
#79825=ORIENTED_EDGE ( 'NONE', *, *, #48335, .T. ) ;
#79826=CARTESIAN_POINT ( 'NONE',  ( 100.8874678597574785, -44.70022135617958980, 177.0522919403976232 ) ) ;
#79827=CARTESIAN_POINT ( 'NONE',  ( 96.19295485998075890, -38.71576710077270889, 51.48229194257797303 ) ) ;
#79828=FACE_BOUND ( 'NONE', #51158, .T. ) ;
#79830=CARTESIAN_POINT ( 'NONE',  ( 80.06648329127399677, 0.2215528400590013880, 306.1181252759120071 ) ) ;
#79831=CARTESIAN_POINT ( 'NONE',  ( 104.3903674582245742, -25.93822912171379969, 90.26991099019693365 ) ) ;
#79832=DIRECTION ( 'NONE',  ( -4.237773401492740281E-14, 1.000000000000000000, 0.000000000000000000 ) ) ;
#79833=CARTESIAN_POINT ( 'NONE',  ( 103.0581626738562306, -26.45339789934171293, 166.3603871806729444 ) ) ;
#79834=DIRECTION ( 'NONE',  ( 0.000000000000000000, -1.000000000000000000, 0.000000000000000000 ) ) ;
#79838=AXIS2_PLACEMENT_3D ( 'NONE', #72616, #22687, #50359 ) ;
#79839=DIRECTION ( 'NONE',  ( 0.000000000000000000, 1.000000000000000000, 0.000000000000000000 ) ) ;
#79840=CARTESIAN_POINT ( 'NONE',  ( 97.80867505543230322, -40.51006205963207663, 136.6353762839628985 ) ) ;
#79842=DIRECTION ( 'NONE',  ( 0.000000000000000000, 0.000000000000000000, -1.000000000000000000 ) ) ;
#79843=CARTESIAN_POINT ( 'NONE',  ( 106.8507020815961397, -47.82747951245497831, 227.5489586092439538 ) ) ;
#79844=ORIENTED_EDGE ( 'NONE', *, *, #32316, .F. ) ;
#79846=CARTESIAN_POINT ( 'NONE',  ( 115.2688234373398046, -30.20251741173218818, 240.3613395616249875 ) ) ;
#79847=CARTESIAN_POINT ( 'NONE',  ( 97.53157056845665807, -31.04763954905634193, 126.9108633711489915 ) ) ;
#79848=CARTESIAN_POINT ( 'NONE',  ( 109.7287935134955035, -27.00184743278844124, 250.8695244108087365 ) ) ;
#79849=CARTESIAN_POINT ( 'NONE',  ( 82.26793483429604237, -38.38027623202342653, 7.385026757020076715 ) ) ;
#79851=DIRECTION ( 'NONE',  ( 0.000000000000000000, 1.000000000000000000, 0.000000000000000000 ) ) ;
#79852=CARTESIAN_POINT ( 'NONE',  ( 177.3246001664174969, -48.34074026909178912, 180.4678068554150059 ) ) ;
#79854=VECTOR ( 'NONE', #4073, 1000.000000000000000 ) ;
#79855=ADVANCED_FACE ( 'NONE', ( #76033 ), #6998, .T. ) ;
#79856=VERTEX_POINT ( 'NONE', #34244 ) ;
#79857=ADVANCED_FACE ( 'NONE', ( #21076 ), #75602, .F. ) ;
#79858=EDGE_LOOP ( 'NONE', ( #26763, #9210, #49154, #5338, #452 ) ) ;
#79861=EDGE_LOOP ( 'NONE', ( #9982, #71706, #57195, #40331 ) ) ;
#79863=CARTESIAN_POINT ( 'NONE',  ( 105.1090458072749527, -25.85091697680629608, 271.2061014663872243 ) ) ;
#79864=CARTESIAN_POINT ( 'NONE',  ( 167.6524903400755875, -49.32844715993520879, 180.4678068554150059 ) ) ;
#79865=CARTESIAN_POINT ( 'NONE',  ( 132.6481957738560311, -34.37139167075012125, 1.944749297857192083 ) ) ;
#79867=AXIS2_PLACEMENT_3D ( 'NONE', #6303, #89431, #79718 ) ;
#79868=CARTESIAN_POINT ( 'NONE',  ( 134.0664832912740110, -33.97944715994100306, 1.625625275910997480 ) ) ;
#79869=CARTESIAN_POINT ( 'NONE',  ( 172.5664832912740110, -36.32844715994070839, 134.1756252759119832 ) ) ;
#79870=CARTESIAN_POINT ( 'NONE',  ( 115.3626348109362425, -40.36077478062563983, 207.9086103042679667 ) ) ;
#79873=EDGE_LOOP ( 'NONE', ( #8769, #9287, #66501, #2097 ) ) ;
#79874=EDGE_CURVE ( 'NONE', #55592, #60004, #47109, .T. ) ;
#79876=CARTESIAN_POINT ( 'NONE',  ( 110.8542377207676992, -45.98433324150028767, 182.8856051340782471 ) ) ;
#79878=CARTESIAN_POINT ( 'NONE',  ( 98.26720277155988015, -37.77870449121756025, 37.85301187732598294 ) ) ;
#79879=EDGE_CURVE ( 'NONE', #51322, #3721, #7972, .T. ) ;
#79880=VECTOR ( 'NONE', #83821, 1000.000000000000000 ) ;
#79882=AXIS2_PLACEMENT_3D ( 'NONE', #4319, #11585, #39276 ) ;
#79883=PLANE ( 'NONE',  #5636 ) ;
#79884=FACE_OUTER_BOUND ( 'NONE', #76532, .T. ) ;
#79885=ORIENTED_EDGE ( 'NONE', *, *, #64246, .T. ) ;
#79886=CARTESIAN_POINT ( 'NONE',  ( 115.8361900164103275, -31.75800120241248337, 55.23740761269547761 ) ) ;
#79889=CARTESIAN_POINT ( 'NONE',  ( 107.6943352634791182, -28.59092592337147209, 67.83380465530596837 ) ) ;
#79890=LINE ( 'NONE', #24906, #20359 ) ;
#79892=FACE_OUTER_BOUND ( 'NONE', #33267, .T. ) ;
#79894=DIRECTION ( 'NONE',  ( 0.000000000000000000, 0.000000000000000000, -1.000000000000000000 ) ) ;
#79896=ORIENTED_EDGE ( 'NONE', *, *, #38171, .F. ) ;
#79897=CARTESIAN_POINT ( 'NONE',  ( 113.8565348333340665, -44.64034031543166492, 108.1413395616249744 ) ) ;
#79898=ORIENTED_EDGE ( 'NONE', *, *, #77592, .T. ) ;
#79899=CARTESIAN_POINT ( 'NONE',  ( 101.2610328325635010, -42.99465878394229179, 46.40384839950495177 ) ) ;
#79900=AXIS2_PLACEMENT_3D ( 'NONE', #33830, #26128, #53796 ) ;
#79901=VECTOR ( 'NONE', #43629, 1000.000000000000114 ) ;
#79903=CARTESIAN_POINT ( 'NONE',  ( 98.21780894689015895, -37.20823830323941905, 72.80158330589698323 ) ) ;
#79904=FACE_OUTER_BOUND ( 'NONE', #71177, .T. ) ;
#79905=DIRECTION ( 'NONE',  ( 9.351236661543306751E-17, -3.725950533538267725E-29, -1.000000000000000000 ) ) ;
#79906=EDGE_CURVE ( 'NONE', #11120, #74275, #34690, .T. ) ;
#79908=CARTESIAN_POINT ( 'NONE',  ( 114.1052656684236979, -46.29384956339717405, 29.08133956162595268 ) ) ;
#79909=AXIS2_PLACEMENT_3D ( 'NONE', #29552, #49523, #77258 ) ;
#79910=CARTESIAN_POINT ( 'NONE',  ( 37.35959712144378386, -48.62134037893557803, 129.9678068554150911 ) ) ;
#79911=ORIENTED_EDGE ( 'NONE', *, *, #80952, .F. ) ;
#79913=ORIENTED_EDGE ( 'NONE', *, *, #68671, .F. ) ;
#79914=FACE_OUTER_BOUND ( 'NONE', #78508, .T. ) ;
#79915=VERTEX_POINT ( 'NONE', #62401 ) ;
#79917=AXIS2_PLACEMENT_3D ( 'NONE', #6621, #12545, #61568 ) ;
#79920=CARTESIAN_POINT ( 'NONE',  ( 99.57924082623969753, -30.38476633542323313, 215.7670538473399517 ) ) ;
#79921=CARTESIAN_POINT ( 'NONE',  ( 30.48091746481826192, -48.32844715994148999, 300.4678068554150059 ) ) ;
#79922=CARTESIAN_POINT ( 'NONE',  ( 94.58945128933383728, -41.88441296220994303, 289.6356252759106837 ) ) ;
#79923=CARTESIAN_POINT ( 'NONE',  ( 117.0915230934440103, -32.07406775014006683, 55.16038718067301261 ) ) ;
#79924=CARTESIAN_POINT ( 'NONE',  ( 97.81200933032994271, -40.51820848727025037, 42.63569297931775282 ) ) ;
#79926=CARTESIAN_POINT ( 'NONE',  ( 102.0659925822678531, -27.97112074188683550, 171.4898645953594212 ) ) ;
#79927=DIRECTION ( 'NONE',  ( 0.7071067811873671394, 0.7071067811857280061, 6.612322855862553737E-17 ) ) ;
#79930=CARTESIAN_POINT ( 'NONE',  ( 31.78666935232895341, -36.02818131005931690, 117.4678068554150485 ) ) ;
#79931=CARTESIAN_POINT ( 'NONE',  ( 117.0603190384279912, -38.08450654926203072, 114.7195913024953313 ) ) ;
#79932=CARTESIAN_POINT ( 'NONE',  ( 99.55514648348071205, -29.48070623161989801, 250.7156252759109520 ) ) ;
#79933=LINE ( 'NONE', #72658, #83517 ) ;
#79935=CARTESIAN_POINT ( 'NONE',  ( 77.53592152231081513, -37.80596063775247728, 2.807537029279840279 ) ) ;
#79937=CARTESIAN_POINT ( 'NONE',  ( 114.1034101198941215, -31.83723292758831747, 278.7324198280767860 ) ) ;
#79939=CARTESIAN_POINT ( 'NONE',  ( 101.7670726180548542, -27.05576796868586698, 96.46324432352997746 ) ) ;
#79941=CARTESIAN_POINT ( 'NONE',  ( 102.3732866125132688, -26.67028275327534814, 135.4118157521009493 ) ) ;
#79942=VERTEX_POINT ( 'NONE', #12313 ) ;
#79944=ORIENTED_EDGE ( 'NONE', *, *, #72951, .T. ) ;
#79946=VECTOR ( 'NONE', #37279, 1000.000000000000000 ) ;
#79948=DIRECTION ( 'NONE',  ( -1.000000000000000078E-15, 1.000000000000000083E-30, 1.000000000000000000 ) ) ;
#79950=ORIENTED_EDGE ( 'NONE', *, *, #87090, .T. ) ;
#79951=CARTESIAN_POINT ( 'NONE',  ( 97.75843041625837770, -40.38500185162371992, 51.62426656411139447 ) ) ;
#79952=CARTESIAN_POINT ( 'NONE',  ( 117.9021936627155895, -39.13782096276514721, 103.6403871806729455 ) ) ;
#79954=DIRECTION ( 'NONE',  ( 0.000000000000000000, 0.000000000000000000, -1.000000000000000000 ) ) ;
#79955=LINE ( 'NONE', #50883, #73731 ) ;
#79956=CARTESIAN_POINT ( 'NONE',  ( 83.06670390244804025, -43.72944715994108122, 207.5838068554169809 ) ) ;
#79957=VERTEX_POINT ( 'NONE', #33650 ) ;
#79958=AXIS2_PLACEMENT_3D ( 'NONE', #69516, #13208, #34977 ) ;
#79959=CARTESIAN_POINT ( 'NONE',  ( 106.0743573402139930, -48.56370683269541644, 112.5099109901969712 ) ) ;
#79961=DIRECTION ( 'NONE',  ( 0.7071067811865279218, -0.7071067811865670016, 6.612322855859973915E-17 ) ) ;
#79964=LINE ( 'NONE', #18604, #35454 ) ;
#79967=EDGE_CURVE ( 'NONE', #62846, #33523, #57239, .T. ) ;
#79968=ORIENTED_EDGE ( 'NONE', *, *, #48683, .T. ) ;
#79973=CIRCLE ( 'NONE', #14733, 2.116999999999980009 ) ;
#79974=ADVANCED_FACE ( 'NONE', ( #1378 ), #70876, .F. ) ;
#79975=CARTESIAN_POINT ( 'NONE',  ( 41.56648329127399677, -9.303447159940999356, 316.8086252759120498 ) ) ;
#79976=CARTESIAN_POINT ( 'NONE',  ( 107.0664832912739399, -36.72944715994095333, 293.1356252759106837 ) ) ;
#79979=DIRECTION ( 'NONE',  ( 1.000000000000000078E-15, -1.000000000000000083E-30, -1.000000000000000000 ) ) ;
#79980=CARTESIAN_POINT ( 'NONE',  ( 103.5361331145923032, -27.60804031003073788, 211.3699109901959616 ) ) ;
#79982=VECTOR ( 'NONE', #69088, 1000.000000000000114 ) ;
#79985=CARTESIAN_POINT ( 'NONE',  ( 110.1509004715571507, -26.04776408289600909, 60.85276813305296173 ) ) ;
#79986=CARTESIAN_POINT ( 'NONE',  ( 98.04154294162555061, -41.04190759109129516, 51.68120649424626123 ) ) ;
#79988=AXIS2_PLACEMENT_3D ( 'NONE', #31202, #30770, #23532 ) ;
#79990=EDGE_LOOP ( 'NONE', ( #21444, #22603, #52579, #71306 ) ) ;
#79993=ORIENTED_EDGE ( 'NONE', *, *, #53995, .T. ) ;
#79994=CARTESIAN_POINT ( 'NONE',  ( 115.7580415341064111, -34.85356206270782309, 180.4272975916109374 ) ) ;
#79995=DIRECTION ( 'NONE',  ( -0.1858654557293118459, 0.9825752044329915114, 0.000000000000000000 ) ) ;
#79997=PLANE ( 'NONE',  #31597 ) ;
#79999=CIRCLE ( 'NONE', #59662, 2.500000000000002220 ) ;
#80002=CARTESIAN_POINT ( 'NONE',  ( 116.8180460095236981, -34.15649538984454381, 185.0317730482575769 ) ) ;
#80003=ORIENTED_EDGE ( 'NONE', *, *, #24759, .F. ) ;
#80004=CARTESIAN_POINT ( 'NONE',  ( 96.68578154376476164, -42.44622222083611263, 26.72705384733997747 ) ) ;
#80008=CARTESIAN_POINT ( 'NONE',  ( 41.56648329127398966, -27.82844715994070484, 258.9256252759120116 ) ) ;
#80010=CARTESIAN_POINT ( 'NONE',  ( 131.0667039024480118, -61.87844715994100397, 213.1838068554149856 ) ) ;
#80011=AXIS2_PLACEMENT_3D ( 'NONE', #33231, #89548, #23219 ) ;
#80013=CARTESIAN_POINT ( 'NONE',  ( 107.2439061797007156, -47.23213900083308658, 208.5899109901969837 ) ) ;
#80014=FACE_OUTER_BOUND ( 'NONE', #35667, .T. ) ;
#80015=ORIENTED_EDGE ( 'NONE', *, *, #41981, .T. ) ;
#80016=AXIS2_PLACEMENT_3D ( 'NONE', #70751, #71648, #16675 ) ;
#80017=CARTESIAN_POINT ( 'NONE',  ( 100.5235407922616133, -27.76354498484767674, 26.56610146638793779 ) ) ;
#80018=CARTESIAN_POINT ( 'NONE',  ( 150.5667039024485803, -47.82844715993594065, 129.9678068554149775 ) ) ;
#80019=EDGE_CURVE ( 'NONE', #25675, #71030, #21861, .T. ) ;
#80022=CARTESIAN_POINT ( 'NONE',  ( 81.97596355239433308, -16.74831825238168648, 2.232988539019116647 ) ) ;
#80024=DIRECTION ( 'NONE',  ( 0.000000000000000000, 0.000000000000000000, -1.000000000000000000 ) ) ;
#80025=CARTESIAN_POINT ( 'NONE',  ( 115.2991214174112002, -34.06025354975611918, 131.9061856076869788 ) ) ;
#80026=CARTESIAN_POINT ( 'NONE',  ( 99.52368306943544951, -29.45034277662237443, 246.7156252759109520 ) ) ;
#80027=AXIS2_PLACEMENT_3D ( 'NONE', #6348, #86907, #45983 ) ;
#80030=CARTESIAN_POINT ( 'NONE',  ( 136.1031425115661193, -38.57949487819416134, 2.327894807233447327 ) ) ;
#80031=EDGE_LOOP ( 'NONE', ( #82502, #78908, #81700 ) ) ;
#80032=VERTEX_POINT ( 'NONE', #83604 ) ;
#80034=DIRECTION ( 'NONE',  ( 0.000000000000000000, 0.000000000000000000, -1.000000000000000000 ) ) ;
#80035=ORIENTED_EDGE ( 'NONE', *, *, #35366, .F. ) ;
#80036=ORIENTED_EDGE ( 'NONE', *, *, #5807, .F. ) ;
#80037=DIRECTION ( 'NONE',  ( 9.912705577010326536E-16, 1.000000000000000000, 0.000000000000000000 ) ) ;
#80040=CARTESIAN_POINT ( 'NONE',  ( 105.3429517235655766, -27.17434032488695550, 124.6409912566479647 ) ) ;
#80042=CARTESIAN_POINT ( 'NONE',  ( 96.29878009220107060, -39.42515072222565209, 16.53372051400597798 ) ) ;
#80043=VERTEX_POINT ( 'NONE', #27730 ) ;
#80045=VECTOR ( 'NONE', #78832, 1000.000000000000000 ) ;
#80046=EDGE_LOOP ( 'NONE', ( #85473, #77418, #62777, #19686 ) ) ;
#80047=CARTESIAN_POINT ( 'NONE',  ( 41.56648329127399677, -9.303447159940999356, 321.0426252759119734 ) ) ;
#80048=ORIENTED_EDGE ( 'NONE', *, *, #32770, .F. ) ;
#80049=CARTESIAN_POINT ( 'NONE',  ( 97.54864246082097168, -39.81029565519295943, 167.5757964592916096 ) ) ;
#80050=CARTESIAN_POINT ( 'NONE',  ( 115.0361479189475205, -42.90987010871590712, 33.30236611295504190 ) ) ;
#80051=LINE ( 'NONE', #51409, #79467 ) ;
#80052=CYLINDRICAL_SURFACE ( 'NONE', #49502, 2.750000000000002665 ) ;
#80054=CARTESIAN_POINT ( 'NONE',  ( 97.46629803964546568, -32.60812463323921406, 16.00419670448194154 ) ) ;
#80055=CARTESIAN_POINT ( 'NONE',  ( 112.2188834189205409, -26.89723471487287654, 10.68038718067299087 ) ) ;
#80059=DIRECTION ( 'NONE',  ( 0.9242245927363031965, 0.3818493186865917766, 0.000000000000000000 ) ) ;
#80060=CARTESIAN_POINT ( 'NONE',  ( 134.0664828118826506, -39.47944715903992829, 8.225259175038003079 ) ) ;
#80062=CIRCLE ( 'NONE', #1739, 2.116999999999980009 ) ;
#80064=EDGE_CURVE ( 'NONE', #19911, #71480, #34562, .T. ) ;
#80065=CARTESIAN_POINT ( 'NONE',  ( 113.1786937796897092, -44.75156961497670238, 163.0938295933654842 ) ) ;
#80067=CARTESIAN_POINT ( 'NONE',  ( 105.0173152498862947, -25.84384494483574102, 280.2365776568630622 ) ) ;
#80068=CARTESIAN_POINT ( 'NONE',  ( 116.3773924821832111, -41.41873894932305689, 199.4556252759109611 ) ) ;
#80069=CARTESIAN_POINT ( 'NONE',  ( 118.1061288724552725, -37.63024191249119355, 34.77372051400695341 ) ) ;
#80070=VECTOR ( 'NONE', #88990, 1000.000000000000000 ) ;
#80072=DIRECTION ( 'NONE',  ( -0.000000000000000000, -0.000000000000000000, -1.000000000000000000 ) ) ;
#80073=CARTESIAN_POINT ( 'NONE',  ( 80.81118397279048793, -34.08035908359610033, 1.709393751551411045 ) ) ;
#80074=COLOUR_RGB ( '', 0.09019608, 0.27058824, 0.51372549) ;
#80075=EDGE_LOOP ( 'NONE', ( #79015, #9846 ) ) ;
#80076=CARTESIAN_POINT ( 'NONE',  ( 83.73314995793998605, 12.92155284005730387, 361.9756252759109998 ) ) ;
#80078=CARTESIAN_POINT ( 'NONE',  ( 104.1495640007033501, -46.68084741754449851, 58.33753003781600199 ) ) ;
#80079=EDGE_CURVE ( 'NONE', #70797, #52812, #80471, .T. ) ;
#80080=PLANE ( 'NONE',  #51495 ) ;
#80082=LINE ( 'NONE', #37845, #56200 ) ;
#80083=CARTESIAN_POINT ( 'NONE',  ( 100.8363305107023820, -45.83159080358277748, 238.1108633711489517 ) ) ;
#80084=CARTESIAN_POINT ( 'NONE',  ( 49.21437657595017612, -35.91149509761089575, 342.9256252759109884 ) ) ;
#80086=CARTESIAN_POINT ( 'NONE',  ( 104.4079568779007730, -46.45804709415482847, 147.3648544342418347 ) ) ;
#80087=ADVANCED_FACE ( 'NONE', ( #4044 ), #87174, .F. ) ;
#80089=DIRECTION ( 'NONE',  ( 0.000000000000000000, 0.000000000000000000, 1.000000000000000000 ) ) ;
#80091=CARTESIAN_POINT ( 'NONE',  ( 132.3573525511384048, -38.88611802718990873, 2.101554303222315845 ) ) ;
#80093=CARTESIAN_POINT ( 'NONE',  ( 99.18511857479137461, -30.88155312011791409, 180.8184824187689799 ) ) ;
#80096=CIRCLE ( 'NONE', #52479, 1.000000000000000888 ) ;
#80097=CARTESIAN_POINT ( 'NONE',  ( 107.5226574059108202, -27.84946772507149504, 91.46729759161098627 ) ) ;
#80100=CARTESIAN_POINT ( 'NONE',  ( 106.3491918589965763, -46.48387837312645132, 218.5184824187679453 ) ) ;
#80101=CARTESIAN_POINT ( 'NONE',  ( 116.3188053082936051, -32.94429434937755019, 19.13562527591095019 ) ) ;
#80102=CARTESIAN_POINT ( 'NONE',  ( 141.0667039024479834, -48.82844715994099971, 10.91780685541499807 ) ) ;
#80105=VECTOR ( 'NONE', #52952, 1000.000000000000000 ) ;
#80109=CYLINDRICAL_SURFACE ( 'NONE', #45888, 9.999999999999998224 ) ;
#80110=CARTESIAN_POINT ( 'NONE',  ( 117.0123300003821640, -30.33189756676010163, 144.2813395616249750 ) ) ;
#80112=CIRCLE ( 'NONE', #4622, 2.517500000000005844 ) ;
#80113=EDGE_LOOP ( 'NONE', ( #51687, #44752 ) ) ;
#80115=CARTESIAN_POINT ( 'NONE',  ( 77.40501520703328708, -18.03131342367423073, 2.974074870387416691 ) ) ;
#80117=CARTESIAN_POINT ( 'NONE',  ( 172.5664832912729878, -18.82844715994071194, 18.92562527591200094 ) ) ;
#80118=CARTESIAN_POINT ( 'NONE',  ( 104.4080847095425639, -46.45808491063921508, 268.3647906417609761 ) ) ;
#80120=CARTESIAN_POINT ( 'NONE',  ( 116.6609997163256764, -40.80771701747383418, 168.5070538473399608 ) ) ;
#80121=CARTESIAN_POINT ( 'NONE',  ( 31.90335556477799628, -33.89581943344391135, -5.074374724088000832 ) ) ;
#80122=EDGE_LOOP ( 'NONE', ( #67143, #3116, #65921, #46771 ) ) ;
#80123=EDGE_LOOP ( 'NONE', ( #68533, #73889, #14326, #88615 ) ) ;
#80125=AXIS2_PLACEMENT_3D ( 'NONE', #26659, #19854, #68002 ) ;
#80127=DIRECTION ( 'NONE',  ( 0.000000000000000000, 0.000000000000000000, -1.000000000000000000 ) ) ;
#80129=CARTESIAN_POINT ( 'NONE',  ( 105.0496896133374918, -44.66766052993097702, 45.19666179816294971 ) ) ;
#80131=EDGE_LOOP ( 'NONE', ( #72677, #48317, #42853, #50169 ) ) ;
#80132=AXIS2_PLACEMENT_3D ( 'NONE', #68889, #62061, #89796 ) ;
#80134=CARTESIAN_POINT ( 'NONE',  ( 82.57621891717900553, -17.60488046387944294, 7.068409955839225489 ) ) ;
#80135=ORIENTED_EDGE ( 'NONE', *, *, #87426, .F. ) ;
#80136=ORIENTED_EDGE ( 'NONE', *, *, #29121, .F. ) ;
#80137=VECTOR ( 'NONE', #71628, 1000.000000000000000 ) ;
#80142=DIRECTION ( 'NONE',  ( 2.900000000000000265E-14, -2.000000000000000155E-15, 1.000000000000000000 ) ) ;
#80143=CARTESIAN_POINT ( 'NONE',  ( 107.1721053552439713, -28.18866407513752392, 34.48956268521896362 ) ) ;
#80144=CARTESIAN_POINT ( 'NONE',  ( 110.5061846383585475, -26.86461981176654845, 209.8099109901969541 ) ) ;
#80145=CARTESIAN_POINT ( 'NONE',  ( 111.4081670832169237, -47.72935575799012753, 172.8756252759109771 ) ) ;
#80146=CARTESIAN_POINT ( 'NONE',  ( 151.0371591254576060, -24.95799193692592155, 129.9678068554149775 ) ) ;
#80147=CARTESIAN_POINT ( 'NONE',  ( 105.6320745483020147, -47.05538338894268691, 253.4670538473393719 ) ) ;
#80148=CARTESIAN_POINT ( 'NONE',  ( 101.9936794628098369, -45.44610784961911065, 98.15771542624335666 ) ) ;
#80150=ADVANCED_FACE ( 'NONE', ( #46132 ), #72537, .F. ) ;
#80151=ORIENTED_EDGE ( 'NONE', *, *, #49489, .F. ) ;
#80153=EDGE_CURVE ( 'NONE', #22550, #35335, #67061, .T. ) ;
#80155=CIRCLE ( 'NONE', #43888, 17.00000000000090239 ) ;
#80156=DIRECTION ( 'NONE',  ( 1.907762142705490052E-15, 7.167082501179359715E-16, -1.000000000000000000 ) ) ;
#80157=CARTESIAN_POINT ( 'NONE',  ( 106.9399074540173871, -47.82885535071048366, 232.5794347997199907 ) ) ;
#80158=ORIENTED_EDGE ( 'NONE', *, *, #39245, .T. ) ;
#80159=CARTESIAN_POINT ( 'NONE',  ( 118.9178230750475649, -36.92810663041961305, 153.8127681330539644 ) ) ;
#80160=CARTESIAN_POINT ( 'NONE',  ( 97.07203916561205403, -35.37876108150283017, 266.2190116188336901 ) ) ;
#80161=DIRECTION ( 'NONE',  ( 1.000000000000000000, 0.000000000000000000, -0.000000000000000000 ) ) ;
#80162=EDGE_CURVE ( 'NONE', #4014, #28273, #59769, .T. ) ;
#80166=CARTESIAN_POINT ( 'NONE',  ( 21.03689327557705369, -23.42844715994187155, 237.4678068554150059 ) ) ;
#80167=CARTESIAN_POINT ( 'NONE',  ( 118.0799254396264786, -36.12288750354066735, 269.8822919425776945 ) ) ;
#80168=DIRECTION ( 'NONE',  ( -0.1811243269279065315, 0.9834602067165264527, 0.000000000000000000 ) ) ;
#80170=VECTOR ( 'NONE', #24303, 1000.000000000000000 ) ;
#80171=LINE ( 'NONE', #87864, #15109 ) ;
#80174=EDGE_CURVE ( 'NONE', #18741, #75087, #63150, .T. ) ;
#80176=CARTESIAN_POINT ( 'NONE',  ( 106.7204202803107904, -44.74667865324451554, 195.5838068554169809 ) ) ;
#80178=DIRECTION ( 'NONE',  ( 0.000000000000000000, 0.000000000000000000, 1.000000000000000000 ) ) ;
#80179=CARTESIAN_POINT ( 'NONE',  ( 110.7040309646834970, -48.03441345040916843, 207.8241967044819489 ) ) ;
#80180=CARTESIAN_POINT ( 'NONE',  ( 102.3023240427231570, -27.41686860022338124, 116.4527681330539650 ) ) ;
#80181=CARTESIAN_POINT ( 'NONE',  ( 110.0644950372451945, -26.04256623378434554, 215.8708633711489711 ) ) ;
#80184=DIRECTION ( 'NONE',  ( 0.000000000000000000, 1.000000000000000000, 0.000000000000000000 ) ) ;
#80185=CARTESIAN_POINT ( 'NONE',  ( 116.6468703464407355, -39.65304199921658324, 39.59041423949068417 ) ) ;
#80188=CARTESIAN_POINT ( 'NONE',  ( 77.31648329127402519, -36.72944715994107412, -5.074374724089059541 ) ) ;
#80191=CARTESIAN_POINT ( 'NONE',  ( 98.02237212078092909, -37.19498283172546849, 120.8019436376009708 ) ) ;
#80192=EDGE_CURVE ( 'NONE', #74330, #18892, #58438, .T. ) ;
#80193=CARTESIAN_POINT ( 'NONE',  ( 45.77381068356938698, -48.62134037881676818, 249.9678068554150343 ) ) ;
#80195=VECTOR ( 'NONE', #28330, 1000.000000000000000 ) ;
#80196=CARTESIAN_POINT ( 'NONE',  ( 97.95167206076199307, -31.64175201202211341, 106.9213395616259703 ) ) ;
#80197=LINE ( 'NONE', #17944, #4771 ) ;
#80199=EDGE_CURVE ( 'NONE', #10583, #5137, #22582, .T. ) ;
#80200=DIRECTION ( 'NONE',  ( 0.000000000000000000, 0.000000000000000000, 1.000000000000000000 ) ) ;
#80202=CARTESIAN_POINT ( 'NONE',  ( 34.27258461953881152, -35.55794170701842916, 237.4678068554150059 ) ) ;
#80203=EDGE_CURVE ( 'NONE', #4730, #15894, #1155, .T. ) ;
#80204=CARTESIAN_POINT ( 'NONE',  ( 114.3402351757609665, -43.26825200597438226, 38.24419670448392594 ) ) ;
#80206=VERTEX_POINT ( 'NONE', #56084 ) ;
#80207=EDGE_LOOP ( 'NONE', ( #87385, #38111 ) ) ;
#80210=CARTESIAN_POINT ( 'NONE',  ( 111.8077268321493278, -46.78591733285061594, 133.9270538473389536 ) ) ;
#80211=CARTESIAN_POINT ( 'NONE',  ( 73.17003668186733023, -46.47944715994106701, -5.074374724089063982 ) ) ;
#80212=DIRECTION ( 'NONE',  ( 0.000000000000000000, 0.000000000000000000, 1.000000000000000000 ) ) ;
#80214=DIRECTION ( 'NONE',  ( 0.000000000000000000, -1.000000000000000000, 0.000000000000000000 ) ) ;
#80216=LINE ( 'NONE', #43981, #37111 ) ;
#80217=CARTESIAN_POINT ( 'NONE',  ( 110.3472192523918380, -25.36789009815977636, 64.85276813305395649 ) ) ;
#80218=ORIENTED_EDGE ( 'NONE', *, *, #65498, .T. ) ;
#80222=DIRECTION ( 'NONE',  ( -4.237773401492740281E-14, 1.000000000000000000, 0.000000000000000000 ) ) ;
#80223=CARTESIAN_POINT ( 'NONE',  ( 103.3443811052163568, -28.91619688769685936, 138.2604713219729717 ) ) ;
#80224=B_SPLINE_CURVE_WITH_KNOTS ( 'NONE', 3,
 ( #84679, #30587, #77854, #36951, #57387, #1553, #44644, #51889, #72377, #58286, #10145, #29694, #9256, #2888, #37853, #64659, #2445, #45088, #16079, #71929, #17406, #30143, #15630, #50573, #57839, #64223, #85130, #50118, #85576, #23790, #8823, #9696, #22896, #23353, #3333, #43304, #10580, #37403, #86018, #51023, #36521, #78763, #1993, #65550, #16517, #31027, #44194, #58717, #86458 ),
 .UNSPECIFIED., .F., .F.,
 ( 4, 2, 1, 1, 1, 1, 1, 1, 2, 2, 2, 2, 2, 2, 2, 1, 1, 1, 1, 1, 1, 1, 2, 2, 2, 2, 2, 2, 2, 2, 4 ),
 ( 0.5000144601850410320, 0.5001365269672251035, 0.5002585937494091750, 0.5005027273137773181, 0.5009909944425138262, 0.5019675286999867314, 0.5039205972149323198, 0.5078267342448233856, 0.5156390083046059614, 0.5312635564241712238, 0.5625126526633018598, 0.6250108451415630206, 0.6875090376198240705, 0.7500072300980851203, 0.7500682634891768785, 0.7501292968802688588, 0.7502513636624523752, 0.7504954972268100821, 0.7509837643555183906, 0.7519602986129432232, 0.7539133671277988835, 0.7578195041575164215, 0.7656317782169517194, 0.7812563263358216492, 0.8125054225735615088, 0.8437545188113011463, 0.8750036150490410058, 0.9062527112867807544, 0.9375018075245205029, 0.9687509037622602515, 1.000000000000000000 ),
 .UNSPECIFIED. ) ;
#80228=ORIENTED_EDGE ( 'NONE', *, *, #79030, .F. ) ;
#80229=ORIENTED_EDGE ( 'NONE', *, *, #18603, .T. ) ;
#80230=CARTESIAN_POINT ( 'NONE',  ( 63.06670390244641311, -24.92844715994017335, 180.4678068554151196 ) ) ;
#80232=ORIENTED_EDGE ( 'NONE', *, *, #28736, .F. ) ;
#80234=CARTESIAN_POINT ( 'NONE',  ( 98.20738808897236538, -36.51799785534514342, 192.7387261630399564 ) ) ;
#80235=DIRECTION ( 'NONE',  ( 0.000000000000000000, 0.000000000000000000, 1.000000000000000000 ) ) ;
#80240=ADVANCED_FACE ( 'NONE', ( #43360 ), #64281, .T. ) ;
#80241=VECTOR ( 'NONE', #59483, 1000.000000000000000 ) ;
#80243=ORIENTED_EDGE ( 'NONE', *, *, #16458, .T. ) ;
#80244=EDGE_CURVE ( 'NONE', #51011, #2099, #42460, .T. ) ;
#80245=B_SPLINE_CURVE_WITH_KNOTS ( 'NONE', 3,
 ( #11584, #25193, #65202, #45179, #51110, #3868, #51984, #51547, #72903, #2979, #30679, #80185, #10668, #38373, #66979, #46061, #9791, #79298, #72025, #45609, #79742, #31559, #24753, #86993, #4760, #78851, #32444, #66073, #3423, #52421, #39275, #18377, #17933, #17499, #17056, #58377, #73341, #11115, #44737, #72469 ),
 .UNSPECIFIED., .F., .F.,
 ( 4, 2, 2, 2, 2, 2, 2, 2, 2, 2, 2, 2, 2, 2, 2, 2, 1, 1, 1, 1, 2, 4 ),
 ( 0.000000000000000000, 0.06250740735585620655, 0.1250148147117124131, 0.1562685183896407870, 0.1875222220675691609, 0.2187759257454975625, 0.2500296294234259364, 0.2812833331013543381, 0.3125370367792826842, 0.3437907404572110859, 0.3750444441351394320, 0.4062981478130678337, 0.4375518514909962353, 0.4688055551689245815, 0.4844324070078888655, 0.4922458329273708966, 0.4961525458871118288, 0.4981059023669823782, 0.4990825806069176251, 0.4995709197268851653, 0.4998150892868689077, 0.5000592588468526500 ),
 .UNSPECIFIED. ) ;
#80247=CARTESIAN_POINT ( 'NONE',  ( 114.7326537306653762, -39.53293727251440970, 216.3652332267339773 ) ) ;
#80248=EDGE_CURVE ( 'NONE', #73072, #44803, #70646, .T. ) ;
#80249=CIRCLE ( 'NONE', #29477, 2.117000000000000881 ) ;
#80250=CARTESIAN_POINT ( 'NONE',  ( 116.6186327310674500, -29.67321183330947321, 109.3327681330539605 ) ) ;
#80251=CARTESIAN_POINT ( 'NONE',  ( 96.94826409162251935, -39.14818769109204055, 56.51276813305394597 ) ) ;
#80252=DIRECTION ( 'NONE',  ( 0.000000000000000000, 1.000000000000000000, 0.000000000000000000 ) ) ;
#80253=FACE_OUTER_BOUND ( 'NONE', #20903, .T. ) ;
#80254=CARTESIAN_POINT ( 'NONE',  ( 106.8112376695022192, -25.27147963872677039, 323.5310614826137794 ) ) ;
#80255=CARTESIAN_POINT ( 'NONE',  ( 108.3661019610163123, -47.70601195518164417, 158.6822919425779617 ) ) ;
#80258=PLANE ( 'NONE',  #78689 ) ;
#80261=EDGE_CURVE ( 'NONE', #20221, #88467, #73312, .T. ) ;
#80262=ORIENTED_EDGE ( 'NONE', *, *, #5272, .T. ) ;
#80264=CARTESIAN_POINT ( 'NONE',  ( 176.7669697523293735, -48.62818131005361266, 129.9678068554150059 ) ) ;
#80268=DIRECTION ( 'NONE',  ( -6.524622321627019585E-16, -4.013151879589939944E-16, -1.000000000000000000 ) ) ;
#80270=CARTESIAN_POINT ( 'NONE',  ( 101.9270123149900513, -28.12399952947236059, 131.5047745096841254 ) ) ;
#80271=CARTESIAN_POINT ( 'NONE',  ( 106.8411850752606966, -48.57806423327891565, 77.56133956162491927 ) ) ;
#80273=EDGE_CURVE ( 'NONE', #49695, #68284, #10530, .T. ) ;
#80274=CARTESIAN_POINT ( 'NONE',  ( 20.03715912545644784, -24.42818131006202975, 117.4678068554150485 ) ) ;
#80275=DIRECTION ( 'NONE',  ( 1.000000000000000000, 0.000000000000000000, 0.000000000000000000 ) ) ;
#80276=CARTESIAN_POINT ( 'NONE',  ( 112.4079628628857677, -28.49644221148687251, 69.61848241876894861 ) ) ;
#80277=DIRECTION ( 'NONE',  ( 0.000000000000000000, -1.000000000000000000, 0.000000000000000000 ) ) ;
#80278=CARTESIAN_POINT ( 'NONE',  ( 109.3536845750984128, -25.93905639472658819, 180.9222919425779708 ) ) ;
#80280=LINE ( 'NONE', #87526, #68483 ) ;
#80282=DIRECTION ( 'NONE',  ( 0.000000000000000000, 0.000000000000000000, 1.000000000000000000 ) ) ;
#80283=CARTESIAN_POINT ( 'NONE',  ( 29.77381068363397887, -48.62134037875510018, 129.9678068554150627 ) ) ;
#80284=CARTESIAN_POINT ( 'NONE',  ( 176.5667039024392579, -48.82844715994099971, 129.9678068554150343 ) ) ;
#80285=EDGE_CURVE ( 'NONE', #21324, #48511, #44261, .T. ) ;
#80286=CARTESIAN_POINT ( 'NONE',  ( 188.5667039024479834, -65.37844715994100397, 293.2178068554150627 ) ) ;
#80287=CARTESIAN_POINT ( 'NONE',  ( 116.3896376309502045, -44.12590514183388990, 198.2927681330539542 ) ) ;
#80289=CARTESIAN_POINT ( 'NONE',  ( 97.81169536214920868, -40.51742132101362870, 146.6356105553879274 ) ) ;
#80290=CARTESIAN_POINT ( 'NONE',  ( 109.2164500608077873, -48.40848361911378817, 273.7213395616253706 ) ) ;
#80291=CARTESIAN_POINT ( 'NONE',  ( 117.4068710881028323, -38.36326476267787200, 109.7013395616249767 ) ) ;
#80292=CARTESIAN_POINT ( 'NONE',  ( 48.85858412958051389, -30.08671355700274574, 313.9678068554150059 ) ) ;
#80293=CARTESIAN_POINT ( 'NONE',  ( 82.72821098189017164, -37.44060378568480019, 6.877169033942653442 ) ) ;
#80294=DIRECTION ( 'NONE',  ( 0.7071067811865449082, 0.7071067811865501263, 7.071067811865448709E-16 ) ) ;
#80297=VECTOR ( 'NONE', #83857, 1000.000000000000000 ) ;
#80300=VERTEX_POINT ( 'NONE', #35205 ) ;
#80301=ORIENTED_EDGE ( 'NONE', *, *, #31624, .T. ) ;
#80302=LINE ( 'NONE', #65746, #23373 ) ;
#80303=CARTESIAN_POINT ( 'NONE',  ( 105.1675567143510364, -46.98732170830142962, 8.429910990196965770 ) ) ;
#80306=EDGE_CURVE ( 'NONE', #1830, #66807, #66829, .T. ) ;
#80310=CARTESIAN_POINT ( 'NONE',  ( 99.99456525420680464, -31.07253584695887483, 195.2000388756959808 ) ) ;
#80311=ORIENTED_EDGE ( 'NONE', *, *, #32428, .F. ) ;
#80314=DIRECTION ( 'NONE',  ( 1.000000000000000000, 1.261617073437676668E-15, 9.462128050782575008E-16 ) ) ;
#80315=VECTOR ( 'NONE', #74817, 1000.000000000000000 ) ;
#80316=CARTESIAN_POINT ( 'NONE',  ( 110.8973285702773950, -45.96660512525729558, 182.8893129469914811 ) ) ;
#80318=CARTESIAN_POINT ( 'NONE',  ( 105.6677623720644306, -45.47998190943052066, 33.88158330589596545 ) ) ;
#80320=CIRCLE ( 'NONE', #13520, 4.749999999999976907 ) ;
#80321=CARTESIAN_POINT ( 'NONE',  ( 115.0870674648954690, -30.61525487349474872, 174.3441961381653016 ) ) ;
#80322=LINE ( 'NONE', #18067, #13837 ) ;
#80323=ORIENTED_EDGE ( 'NONE', *, *, #73220, .T. ) ;
#80324=CARTESIAN_POINT ( 'NONE',  ( 103.2767410102387231, -27.47537489543444877, 56.38577783829719436 ) ) ;
#80327=CARTESIAN_POINT ( 'NONE',  ( 111.5243040195562401, -29.85845577577017806, 67.43666179816293038 ) ) ;
#80331=CARTESIAN_POINT ( 'NONE',  ( 109.6429171241200038, -46.48011071818258699, 193.7814046315215251 ) ) ;
#80332=ORIENTED_EDGE ( 'NONE', *, *, #18313, .T. ) ;
#80333=FACE_OUTER_BOUND ( 'NONE', #2747, .T. ) ;
#80336=CARTESIAN_POINT ( 'NONE',  ( 97.61684652917979577, -30.99503764212949264, 125.8803871806719599 ) ) ;
#80337=ORIENTED_EDGE ( 'NONE', *, *, #15852, .T. ) ;
#80338=CARTESIAN_POINT ( 'NONE',  ( 112.3043975166656736, -44.90470753876829235, 67.45241982807698378 ) ) ;
#80339=DIRECTION ( 'NONE',  ( -0.7071067811864980568, -0.7071067811865969777, 0.000000000000000000 ) ) ;
#80340=CARTESIAN_POINT ( 'NONE',  ( 108.6974651445452764, -45.43968118700122005, 79.15586902018296200 ) ) ;
#80341=CARTESIAN_POINT ( 'NONE',  ( 86.06670390244796920, -58.72944715994110254, 310.9178068554150514 ) ) ;
#80344=CARTESIAN_POINT ( 'NONE',  ( 96.66430309996448500, -42.45805065352005414, 22.72705384733997391 ) ) ;
#80347=DIRECTION ( 'NONE',  ( -2.900000000000000265E-14, 2.000000000000000155E-15, -1.000000000000000000 ) ) ;
#80348=EDGE_LOOP ( 'NONE', ( #31731, #2279, #45117, #47296 ) ) ;
#80350=AXIS2_PLACEMENT_3D ( 'NONE', #61244, #76223, #89875 ) ;
#80351=VERTEX_POINT ( 'NONE', #45915 ) ;
#80353=ADVANCED_FACE ( 'NONE', ( #39125 ), #81388, .T. ) ;
#80355=B_SPLINE_CURVE_WITH_KNOTS ( 'NONE', 3,
 ( #61427, #89154, #26918, #20115, #75526, #77314, #1910, #550, #29164, #6923, #21915, #34625, #21460, #70502, #29608, #70051, #28250, #56400, #57297, #84143, #112, #69607, #22810, #7819, #1468, #62331, #27810, #35509 ),
 .UNSPECIFIED., .F., .F.,
 ( 4, 2, 2, 2, 2, 2, 2, 2, 2, 2, 1, 1, 1, 1, 2, 4 ),
 ( 0.000000000000000000, 0.06251150331641630586, 0.1250230066328326117, 0.1875345099492489176, 0.2500460132656652235, 0.3125575165820815848, 0.3750690198984978352, 0.4375805232149141411, 0.4688362748731219609, 0.4844641507022258153, 0.4922780886167778536, 0.4961850575740540670, 0.4981385420526921459, 0.4991152842920111299, 0.4996036554116704553, 0.5000920265313297808 ),
 .UNSPECIFIED. ) ;
#80356=EDGE_CURVE ( 'NONE', #72283, #34034, #60453, .T. ) ;
#80358=CARTESIAN_POINT ( 'NONE',  ( 98.06605190618643064, -40.64173669134676459, 231.6527681330539679 ) ) ;
#80359=CARTESIAN_POINT ( 'NONE',  ( 97.81286927418427979, -40.51761286958078756, 126.6352223400343746 ) ) ;
#80360=CYLINDRICAL_SURFACE ( 'NONE', #31689, 0.4999999999999989453 ) ;
#80361=CARTESIAN_POINT ( 'NONE',  ( 112.7598396812348369, -27.95408244994987967, 65.61848241876793963 ) ) ;
#80362=DIRECTION ( 'NONE',  ( 4.299999999999999979E-14, -1.000000000000000000, 4.100000000000000342E-29 ) ) ;
#80364=LINE ( 'NONE', #40347, #40906 ) ;
#80365=EDGE_CURVE ( 'NONE', #56941, #84744, #59108, .T. ) ;
#80367=ORIENTED_EDGE ( 'NONE', *, *, #2329, .T. ) ;
#80368=EDGE_CURVE ( 'NONE', #65464, #27479, #32298, .T. ) ;
#80370=FACE_OUTER_BOUND ( 'NONE', #48153, .T. ) ;
#80371=CIRCLE ( 'NONE', #20908, 0.5000000000000004441 ) ;
#80373=CARTESIAN_POINT ( 'NONE',  ( 110.7254274611716056, -26.32387412717027786, 254.8194347997205682 ) ) ;
#80376=CARTESIAN_POINT ( 'NONE',  ( 77.55659459556547120, -37.85370728022186171, 2.783021134850681477 ) ) ;
#80378=CARTESIAN_POINT ( 'NONE',  ( 99.32305605351064060, -40.33436967443800825, 256.0952769709339236 ) ) ;
#80380=CARTESIAN_POINT ( 'NONE',  ( 106.8416606513710008, -48.55305329746386178, 73.56133956162497611 ) ) ;
#80382=CARTESIAN_POINT ( 'NONE',  ( 95.98102948456921979, -37.30005869795228080, 121.3794347997209684 ) ) ;
#80383=ORIENTED_EDGE ( 'NONE', *, *, #79030, .T. ) ;
#80384=CARTESIAN_POINT ( 'NONE',  ( 83.56670559755357885, -36.73837296219067383, 249.5838068554176630 ) ) ;
#80385=EDGE_LOOP ( 'NONE', ( #84638, #56143, #63925, #57708 ) ) ;
#80386=CARTESIAN_POINT ( 'NONE',  ( 72.26648329127297643, -1.929447159941394263, 361.9756252759109998 ) ) ;
#80387=CIRCLE ( 'NONE', #70186, 2.117000000000007987 ) ;
#80389=CARTESIAN_POINT ( 'NONE',  ( 135.3321452824027631, -34.28157797493338421, 1.873071231924423374 ) ) ;
#80393=CARTESIAN_POINT ( 'NONE',  ( 117.6400240572639575, -42.19104337252187520, 93.44705384733897802 ) ) ;
#80394=ORIENTED_EDGE ( 'NONE', *, *, #48678, .F. ) ;
#80396=DIRECTION ( 'NONE',  ( 1.000000000000000000, 0.000000000000000000, 0.000000000000000000 ) ) ;
#80398=VERTEX_POINT ( 'NONE', #66373 ) ;
#80399=CARTESIAN_POINT ( 'NONE',  ( 117.3857798876165788, -38.35993227889734669, 113.7013395616249767 ) ) ;
#80400=CARTESIAN_POINT ( 'NONE',  ( 61.56670390244727287, -23.42844715994024085, 300.4678068554150627 ) ) ;
#80403=ORIENTED_EDGE ( 'NONE', *, *, #70336, .F. ) ;
#80404=FACE_OUTER_BOUND ( 'NONE', #26488, .T. ) ;
#80405=CARTESIAN_POINT ( 'NONE',  ( 194.0371591254575208, -24.42818131005417115, 180.4678068554150343 ) ) ;
#80406=DIRECTION ( 'NONE',  ( 0.000000000000000000, 0.000000000000000000, 1.000000000000000000 ) ) ;
#80407=PLANE ( 'NONE',  #8841 ) ;
#80410=CARTESIAN_POINT ( 'NONE',  ( 108.4173540871620389, -26.73501544328009416, 179.9689693287395755 ) ) ;
#80411=CIRCLE ( 'NONE', #41212, 2.500000000000002220 ) ;
#80412=ORIENTED_EDGE ( 'NONE', *, *, #28415, .F. ) ;
#80414=CARTESIAN_POINT ( 'NONE',  ( 105.7154775075611752, -46.72385841472092949, 33.46895862334973515 ) ) ;
#80415=CARTESIAN_POINT ( 'NONE',  ( 99.76930146980372172, -30.21680002102814555, 186.7470538473389752 ) ) ;
#80416=FACE_OUTER_BOUND ( 'NONE', #73423, .T. ) ;
#80417=ORIENTED_EDGE ( 'NONE', *, *, #80669, .F. ) ;
#80418=CARTESIAN_POINT ( 'NONE',  ( 102.2761128416349692, -28.20209198692217356, 56.48419670448195973 ) ) ;
#80419=CARTESIAN_POINT ( 'NONE',  ( 110.8542252850209309, -45.98433833104029844, 52.88560406628666044 ) ) ;
#80422=ORIENTED_EDGE ( 'NONE', *, *, #32765, .T. ) ;
#80423=ADVANCED_FACE ( 'NONE', ( #73645 ), #12324, .T. ) ;
#80425=ORIENTED_EDGE ( 'NONE', *, *, #533, .T. ) ;
#80427=CARTESIAN_POINT ( 'NONE',  ( 114.5371455856629694, -43.48665885088448135, 229.6730118773259619 ) ) ;
#80430=AXIS2_PLACEMENT_3D ( 'NONE', #19178, #8695, #41829 ) ;
#80434=LINE ( 'NONE', #10928, #25764 ) ;
#80435=CARTESIAN_POINT ( 'NONE',  ( 80.81785596310795938, -39.40256188477532362, 1.690787648074149496 ) ) ;
#80437=LINE ( 'NONE', #33169, #8754 ) ;
#80439=CARTESIAN_POINT ( 'NONE',  ( 98.34811578340129756, -31.65970814803674571, 36.90641431777298465 ) ) ;
#80440=ORIENTED_EDGE ( 'NONE', *, *, #21315, .F. ) ;
#80441=CARTESIAN_POINT ( 'NONE',  ( 96.91023542590092177, -30.67149048741783091, 280.8984824187682534 ) ) ;
#80444=CARTESIAN_POINT ( 'NONE',  ( 104.1201707603140107, -29.11702517433068138, 213.1880903695919756 ) ) ;
#80445=CARTESIAN_POINT ( 'NONE',  ( 21.03715912545829170, -47.82818131006186491, 249.9678068554150059 ) ) ;
#80447=DIRECTION ( 'NONE',  ( 0.000000000000000000, 0.000000000000000000, -1.000000000000000000 ) ) ;
#80449=CARTESIAN_POINT ( 'NONE',  ( 97.05457585776278506, -41.52102392564493272, 212.6937205140059461 ) ) ;
#80450=CARTESIAN_POINT ( 'NONE',  ( 194.5667039024483529, -47.82844715993405771, 249.9678068554149775 ) ) ;
#80451=VERTEX_POINT ( 'NONE', #11880 ) ;
#80452=CARTESIAN_POINT ( 'NONE',  ( 107.6053842629478794, -26.23908965751013156, 91.03562527591097364 ) ) ;
#80453=CARTESIAN_POINT ( 'NONE',  ( 194.5664832912729878, -18.82844715994100326, 342.9256252759109884 ) ) ;
#80455=ORIENTED_EDGE ( 'NONE', *, *, #43340, .F. ) ;
#80458=EDGE_LOOP ( 'NONE', ( #25135, #86003, #17671, #87193 ) ) ;
#80459=EDGE_CURVE ( 'NONE', #3107, #14741, #8040, .T. ) ;
#80460=CARTESIAN_POINT ( 'NONE',  ( 81.08070086926866793, -16.17316201338597992, 1.785258157649182165 ) ) ;
#80461=CARTESIAN_POINT ( 'NONE',  ( 71.06648329127399677, -18.82844715994099971, 284.9256252759119548 ) ) ;
#80462=DIRECTION ( 'NONE',  ( 0.000000000000000000, 1.000000000000000000, 0.000000000000000000 ) ) ;
#80463=CARTESIAN_POINT ( 'NONE',  ( 104.0192455041231767, -29.15686055524244935, 128.1995189410199600 ) ) ;
#80464=CARTESIAN_POINT ( 'NONE',  ( 118.8146046005060015, -38.46262239392275717, 219.7099109901969882 ) ) ;
#80465=CARTESIAN_POINT ( 'NONE',  ( 116.8180029026503206, -34.15632288917988291, 60.03118074130109960 ) ) ;
#80466=ORIENTED_EDGE ( 'NONE', *, *, #16391, .F. ) ;
#80467=EDGE_CURVE ( 'NONE', #10437, #16028, #38, .T. ) ;
#80469=ORIENTED_EDGE ( 'NONE', *, *, #22683, .T. ) ;
#80470=ORIENTED_EDGE ( 'NONE', *, *, #74928, .T. ) ;
#80471=CIRCLE ( 'NONE', #81977, 0.5000000000000004441 ) ;
#80472=DIRECTION ( 'NONE',  ( 0.000000000000000000, -1.000000000000000000, 0.000000000000000000 ) ) ;
#80473=ORIENTED_EDGE ( 'NONE', *, *, #86809, .T. ) ;
#80474=ORIENTED_EDGE ( 'NONE', *, *, #2635, .T. ) ;
#80478=FACE_OUTER_BOUND ( 'NONE', #7495, .T. ) ;
#80480=B_SPLINE_CURVE_WITH_KNOTS ( 'NONE', 3,
 ( #72790, #30115, #3307, #65081, #43730, #86872, #30562, #51866, #16490, #24198, #80065, #24633, #2863, #44169, #71467, #10118, #58260, #45063 ),
 .UNSPECIFIED., .F., .F.,
 ( 4, 2, 2, 2, 2, 2, 2, 2, 4 ),
 ( 0.4999681725817722855, 0.5624721510090507914, 0.6249761294363291864, 0.6874801078636076923, 0.7499840862908861983, 0.8124880647181645932, 0.8749920431454430991, 0.9374960215727214941, 1.000000000000000000 ),
 .UNSPECIFIED. ) ;
#80481=CARTESIAN_POINT ( 'NONE',  ( 99.77605516222793369, -32.27907757783855658, 170.3124198280769974 ) ) ;
#80482=CARTESIAN_POINT ( 'NONE',  ( 118.2557925370599179, -40.78261322564650015, 23.54991099019593292 ) ) ;
#80483=ORIENTED_EDGE ( 'NONE', *, *, #19957, .F. ) ;
#80484=PLANE ( 'NONE',  #55669 ) ;
#80485=ORIENTED_EDGE ( 'NONE', *, *, #46600, .T. ) ;
#80486=CYLINDRICAL_SURFACE ( 'NONE', #89648, 0.9999999999991942001 ) ;
#80487=VERTEX_POINT ( 'NONE', #83614 ) ;
#80488=CARTESIAN_POINT ( 'NONE',  ( 97.45633071946963355, -39.50260968302539055, 167.5502217315908808 ) ) ;
#80490=CARTESIAN_POINT ( 'NONE',  ( 123.6837132603318992, -53.34645651782490461, 239.5838068554164693 ) ) ;
#80491=CARTESIAN_POINT ( 'NONE',  ( 25.56670390244805091, -42.82844715994167473, 293.2178068554150059 ) ) ;
#80493=CARTESIAN_POINT ( 'NONE',  ( 116.4944971008961261, -32.22846566477972630, 19.18133956162493092 ) ) ;
#80494=VECTOR ( 'NONE', #67205, 1000.000000000000000 ) ;
#80495=CARTESIAN_POINT ( 'NONE',  ( 96.64260770218685082, -42.46999856532355011, 22.72705384733997391 ) ) ;
#80499=CARTESIAN_POINT ( 'NONE',  ( 150.5667039024476139, -25.42844715993593852, 129.9678068554149775 ) ) ;
#80501=CARTESIAN_POINT ( 'NONE',  ( 172.5664832912729878, -27.82844715994070484, 138.9256252759119832 ) ) ;
#80503=DIRECTION ( 'NONE',  ( 0.000000000000000000, 0.000000000000000000, 1.000000000000000000 ) ) ;
#80504=AXIS2_PLACEMENT_3D ( 'NONE', #26977, #68312, #47842 ) ;
#80505=AXIS2_PLACEMENT_3D ( 'NONE', #52662, #87234, #5905 ) ;
#80506=DIRECTION ( 'NONE',  ( 0.000000000000000000, 1.000000000000000000, 0.000000000000000000 ) ) ;
#80508=CARTESIAN_POINT ( 'NONE',  ( 95.20909952976953150, -35.71394341709248721, 36.25848241876794731 ) ) ;
#80509=CARTESIAN_POINT ( 'NONE',  ( 103.8197751496740011, -48.12653019911325458, 213.3556252759109668 ) ) ;
#80510=CARTESIAN_POINT ( 'NONE',  ( 107.8700274897790479, -26.31351822515222949, 66.01562527591097762 ) ) ;
#80511=DIRECTION ( 'NONE',  ( 0.000000000000000000, 0.000000000000000000, -1.000000000000000000 ) ) ;
#80513=EDGE_CURVE ( 'NONE', #73956, #52482, #66044, .T. ) ;
#80514=CARTESIAN_POINT ( 'NONE',  ( 81.01407827912798609, -34.14703303315388183, 1.764000745016844007 ) ) ;
#80515=EDGE_CURVE ( 'NONE', #65403, #33963, #36666, .T. ) ;
#80516=VECTOR ( 'NONE', #10211, 1000.000000000000000 ) ;
#80518=CARTESIAN_POINT ( 'NONE',  ( 32.09598329128129279, -23.42844715994118587, 313.9678068554150059 ) ) ;
#80519=ORIENTED_EDGE ( 'NONE', *, *, #64697, .F. ) ;
#80520=CARTESIAN_POINT ( 'NONE',  ( 116.7274023843878581, -38.25590632018514725, 109.7013395616249767 ) ) ;
#80521=DIRECTION ( 'NONE',  ( 0.9999999853157766072, 0.0001713722456126751754, 0.000000000000000000 ) ) ;
#80524=CARTESIAN_POINT ( 'NONE',  ( 109.9541224118590321, -48.19721710984605068, 238.7727681330539724 ) ) ;
#80525=LINE ( 'NONE', #4213, #61418 ) ;
#80526=CARTESIAN_POINT ( 'NONE',  ( 31.56670390244800828, -33.35206098992711077, -5.074374724088000832 ) ) ;
#80529=CARTESIAN_POINT ( 'NONE',  ( 194.5664832912739826, 0.2215528400590083269, 323.8756252759109202 ) ) ;
#80531=CARTESIAN_POINT ( 'NONE',  ( 98.51953950620406886, -30.85675296092858844, 165.8594347997209582 ) ) ;
#80533=ORIENTED_EDGE ( 'NONE', *, *, #78679, .F. ) ;
#80535=CARTESIAN_POINT ( 'NONE',  ( 116.0874278420761527, -39.35605806303598797, 135.0206309249449532 ) ) ;
#80536=ADVANCED_FACE ( 'NONE', ( #34992 ), #7305, .F. ) ;
#80537=FACE_OUTER_BOUND ( 'NONE', #73654, .T. ) ;
#80538=CARTESIAN_POINT ( 'NONE',  ( 110.6561457788924230, -27.59554888373227755, 265.7784824187677941 ) ) ;
#80540=CIRCLE ( 'NONE', #37027, 13.31747058675099815 ) ;
#80541=DIRECTION ( 'NONE',  ( 3.999999999999999995E-14, -1.000000000000000000, 4.100000000000000342E-29 ) ) ;
#80542=CARTESIAN_POINT ( 'NONE',  ( 188.5667039024486087, -48.82844715993430640, 134.7178068554150059 ) ) ;
#80546=FACE_OUTER_BOUND ( 'NONE', #49082, .T. ) ;
#80547=CYLINDRICAL_SURFACE ( 'NONE', #18346, 4.874999999999990230 ) ;
#80548=CARTESIAN_POINT ( 'NONE',  ( 114.7977927517518566, -29.71579763117545880, 209.4127681330539872 ) ) ;
#80556=AXIS2_PLACEMENT_3D ( 'NONE', #35260, #21662, #84346 ) ;
#80557=ORIENTED_EDGE ( 'NONE', *, *, #18030, .T. ) ;
#80559=CARTESIAN_POINT ( 'NONE',  ( 109.6412877908718713, -46.48052073322395472, 62.78131853186246047 ) ) ;
#80561=VECTOR ( 'NONE', #20474, 1000.000000000000114 ) ;
#80562=CARTESIAN_POINT ( 'NONE',  ( 98.03659727384791722, -44.40418782976336587, 226.8870538473399563 ) ) ;
#80563=CARTESIAN_POINT ( 'NONE',  ( 136.2679348342933281, -38.38027623202234651, 7.385026757022528088 ) ) ;
#80566=ORIENTED_EDGE ( 'NONE', *, *, #58631, .T. ) ;
#80567=VECTOR ( 'NONE', #72128, 1000.000000000000000 ) ;
#80569=CARTESIAN_POINT ( 'NONE',  ( 116.9574880481188899, -38.55991405319311127, 64.68174541508243180 ) ) ;
#80572=CARTESIAN_POINT ( 'NONE',  ( 97.83899624421785290, -40.58356376421257750, 166.6413203159688976 ) ) ;
#80573=CARTESIAN_POINT ( 'NONE',  ( 102.2704046875766579, -44.67259270758150080, 49.96237608387698970 ) ) ;
#80574=AXIS2_PLACEMENT_3D ( 'NONE', #2665, #78970, #2211 ) ;
#80575=CYLINDRICAL_SURFACE ( 'NONE', #68169, 0.2500000000000002220 ) ;
#80576=ORIENTED_EDGE ( 'NONE', *, *, #89275, .F. ) ;
#80577=EDGE_CURVE ( 'NONE', #38949, #52724, #16797, .T. ) ;
#80578=AXIS2_PLACEMENT_3D ( 'NONE', #38275, #2879, #45511 ) ;
#80579=CARTESIAN_POINT ( 'NONE',  ( 172.5667039024478129, -36.32844715993500273, 300.4678068554149490 ) ) ;
#80580=CARTESIAN_POINT ( 'NONE',  ( 82.18073802037548603, -16.97076862298585453, 7.459445689451158934 ) ) ;
#80581=VERTEX_POINT ( 'NONE', #43590 ) ;
#80582=ORIENTED_EDGE ( 'NONE', *, *, #1203, .F. ) ;
#80585=VERTEX_POINT ( 'NONE', #15473 ) ;
#80586=CARTESIAN_POINT ( 'NONE',  ( 108.4153923495623104, -26.73476988454542536, 155.9688923574878743 ) ) ;
#80587=AXIS2_PLACEMENT_3D ( 'NONE', #21525, #8335, #15150 ) ;
#80589=CARTESIAN_POINT ( 'NONE',  ( 99.48186602960301173, -30.66774701162068695, 45.21241982807700310 ) ) ;
#80590=CARTESIAN_POINT ( 'NONE',  ( 101.1881973814857076, -45.36612005690837890, 197.1013395616249966 ) ) ;
#80591=CARTESIAN_POINT ( 'NONE',  ( 116.7861719071672866, -43.46560779248406448, 163.3441967044829823 ) ) ;
#80593=CARTESIAN_POINT ( 'NONE',  ( 99.18578730576537339, -42.92413673961824117, 21.85661952785993378 ) ) ;
#80594=CARTESIAN_POINT ( 'NONE',  ( 96.76336351750784104, -35.13941245127819002, 262.2041967044821149 ) ) ;
#80596=CARTESIAN_POINT ( 'NONE',  ( 31.71315051186898870, -31.94127993907790852, -5.074374724088000832 ) ) ;
#80597=EDGE_LOOP ( 'NONE', ( #67425, #59828, #33415, #50164 ) ) ;
#80598=ORIENTED_EDGE ( 'NONE', *, *, #79066, .F. ) ;
#80599=CIRCLE ( 'NONE', #53286, 0.5000000000000004441 ) ;
#80601=CARTESIAN_POINT ( 'NONE',  ( 109.9724474192709351, -48.26999177473817326, 242.7727681330539724 ) ) ;
#80602=ORIENTED_EDGE ( 'NONE', *, *, #58424, .T. ) ;
#80603=CARTESIAN_POINT ( 'NONE',  ( 103.5423316596719445, -26.88027146080960961, 190.3499109901969746 ) ) ;
#80604=LINE ( 'NONE', #25621, #80516 ) ;
#80605=CIRCLE ( 'NONE', #73318, 0.5000000000000129896 ) ;
#80607=DIRECTION ( 'NONE',  ( -1.000000000000000078E-15, -1.000000000000000083E-30, 1.000000000000000000 ) ) ;
#80609=CARTESIAN_POINT ( 'NONE',  ( 109.2954090318264377, -45.76736768674248168, 277.6356252759110816 ) ) ;
#80611=CARTESIAN_POINT ( 'NONE',  ( 114.3996560367811099, -27.45190519937929707, 270.5441967044823741 ) ) ;
#80612=CARTESIAN_POINT ( 'NONE',  ( 182.4202572930257134, -31.94127993907681073, 342.9256252759109884 ) ) ;
#80614=DIRECTION ( 'NONE',  ( 0.000000000000000000, 0.000000000000000000, 1.000000000000000000 ) ) ;
#80615=CARTESIAN_POINT ( 'NONE',  ( 123.6837132603319560, -53.34645651782485487, 219.5838068554170093 ) ) ;
#80619=ORIENTED_EDGE ( 'NONE', *, *, #7549, .F. ) ;
#80620=CARTESIAN_POINT ( 'NONE',  ( 136.5939002653058196, -19.81452881268075572, 7.047625865513104770 ) ) ;
#80621=CARTESIAN_POINT ( 'NONE',  ( 96.10188529952328906, -35.15685947849579662, 226.2251490854349640 ) ) ;
#80622=CARTESIAN_POINT ( 'NONE',  ( 101.7559735582952953, -27.03550746236556890, 96.46324432352997746 ) ) ;
#80623=CARTESIAN_POINT ( 'NONE',  ( 98.86476787746175887, -29.25085353348518424, 226.7261014663869503 ) ) ;
#80624=DIRECTION ( 'NONE',  ( 0.000000000000000000, 0.000000000000000000, 1.000000000000000000 ) ) ;
#80625=CYLINDRICAL_SURFACE ( 'NONE', #33324, 3.250000000000002665 ) ;
#80626=DIRECTION ( 'NONE',  ( 0.000000000000000000, -1.000000000000000000, 0.000000000000000000 ) ) ;
#80627=EDGE_CURVE ( 'NONE', #82808, #12675, #77243, .T. ) ;
#80628=DIRECTION ( 'NONE',  ( 0.000000000000000000, -1.000000000000000000, 0.000000000000000000 ) ) ;
#80630=VECTOR ( 'NONE', #61737, 1000.000000000000000 ) ;
#80632=VECTOR ( 'NONE', #64125, 1000.000000000000000 ) ;
#80633=EDGE_CURVE ( 'NONE', #13721, #33634, #2280, .T. ) ;
#80634=ORIENTED_EDGE ( 'NONE', *, *, #80952, .T. ) ;
#80635=EDGE_LOOP ( 'NONE', ( #17119, #75451, #32280, #16465 ) ) ;
#80636=CARTESIAN_POINT ( 'NONE',  ( 110.9399543235443559, -27.82625392046294266, 134.1724198280769826 ) ) ;
#80640=CARTESIAN_POINT ( 'NONE',  ( 117.6812658759004222, -39.72780374360937827, 139.6194347997199827 ) ) ;
#80641=LINE ( 'NONE', #18849, #67132 ) ;
#80642=CIRCLE ( 'NONE', #42672, 4.875000000000017764 ) ;
#80643=DIRECTION ( 'NONE',  ( -4.299999999999999979E-14, 1.000000000000000000, -4.400000000000000367E-29 ) ) ;
#80646=VECTOR ( 'NONE', #14958, 1000.000000000000000 ) ;
#80647=CARTESIAN_POINT ( 'NONE',  ( 97.35459460924916186, -38.14118110200430323, 66.44133956162595211 ) ) ;
#80648=ORIENTED_EDGE ( 'NONE', *, *, #39630, .T. ) ;
#80650=ORIENTED_EDGE ( 'NONE', *, *, #29622, .T. ) ;
#80653=CARTESIAN_POINT ( 'NONE',  ( 113.7357275853186280, -44.67049210939290305, 144.1203871806719690 ) ) ;
#80658=CARTESIAN_POINT ( 'NONE',  ( 141.8164832912739826, -8.729447159940995959, 14.67562527591100441 ) ) ;
#80661=CARTESIAN_POINT ( 'NONE',  ( 100.9560042165379059, -28.30978499293925310, 75.57562527591093726 ) ) ;
#80662=EDGE_LOOP ( 'NONE', ( #32014, #81299, #25982 ) ) ;
#80664=EDGE_CURVE ( 'NONE', #3721, #51322, #87851, .T. ) ;
#80668=CARTESIAN_POINT ( 'NONE',  ( 103.1394548971403680, -44.44173430692483606, 170.0318998934009755 ) ) ;
#80669=EDGE_CURVE ( 'NONE', #75722, #10086, #85422, .T. ) ;
#80670=CARTESIAN_POINT ( 'NONE',  ( 180.1667039024460166, -26.71338133339240528, -5.074374724088000832 ) ) ;
#80671=ORIENTED_EDGE ( 'NONE', *, *, #11132, .F. ) ;
#80672=ORIENTED_EDGE ( 'NONE', *, *, #28772, .F. ) ;
#80675=ORIENTED_EDGE ( 'NONE', *, *, #27463, .F. ) ;
#80676=CARTESIAN_POINT ( 'NONE',  ( 77.40528906089566874, -19.42303004212691775, 6.877070700249886315 ) ) ;
#80678=CARTESIAN_POINT ( 'NONE',  ( 104.8455658278054017, -28.15064746346142144, 196.7101547344689720 ) ) ;
#80679=CARTESIAN_POINT ( 'NONE',  ( 160.5667039024428391, -48.82844715994099971, 180.4678068554150059 ) ) ;
#80680=AXIS2_PLACEMENT_3D ( 'NONE', #70399, #36326, #12407 ) ;
#80681=PLANE ( 'NONE',  #61769 ) ;
#80683=VECTOR ( 'NONE', #18302, 1000.000000000000000 ) ;
#80685=ORIENTED_EDGE ( 'NONE', *, *, #14985, .T. ) ;
#80686=AXIS2_PLACEMENT_3D ( 'NONE', #30775, #69545, #63168 ) ;
#80690=ORIENTED_EDGE ( 'NONE', *, *, #23157, .F. ) ;
#80691=EDGE_CURVE ( 'NONE', #45550, #89277, #51737, .T. ) ;
#80692=CARTESIAN_POINT ( 'NONE',  ( 114.1044565855118265, -40.86425766668616433, 236.2223760838769806 ) ) ;
#80693=CARTESIAN_POINT ( 'NONE',  ( 102.5485826229696329, -27.30952478670668881, 95.43276813305395478 ) ) ;
#80694=CARTESIAN_POINT ( 'NONE',  ( 113.4461594614341777, -46.68675298423774223, 68.02991099019695298 ) ) ;
#80695=EDGE_CURVE ( 'NONE', #71968, #69308, #60280, .T. ) ;
#80697=CARTESIAN_POINT ( 'NONE',  ( 114.3200451278417518, -29.78195214854387629, 195.4345394874663384 ) ) ;
#80698=CARTESIAN_POINT ( 'NONE',  ( 113.5650955083461326, -44.92635950737134465, 164.1099109901969655 ) ) ;
#80699=CARTESIAN_POINT ( 'NONE',  ( 106.7711676359460000, -46.77985028430433800, 277.5523465834128274 ) ) ;
#80700=ORIENTED_EDGE ( 'NONE', *, *, #45505, .F. ) ;
#80702=EDGE_LOOP ( 'NONE', ( #18327, #16656, #13005, #25798 ) ) ;
#80704=FACE_BOUND ( 'NONE', #32288, .T. ) ;
#80707=ORIENTED_EDGE ( 'NONE', *, *, #83393, .T. ) ;
#80709=EDGE_LOOP ( 'NONE', ( #54465, #35673, #3364, #43618, #30495 ) ) ;
#80710=CARTESIAN_POINT ( 'NONE',  ( 103.8017946383473031, -27.25047886087329729, 131.3403327703989021 ) ) ;
#80711=CARTESIAN_POINT ( 'NONE',  ( 115.2672674329477900, -44.14067019768319966, 83.25372051400698581 ) ) ;
#80715=DIRECTION ( 'NONE',  ( 1.907762142705490052E-15, 7.167082501179359715E-16, -1.000000000000000000 ) ) ;
#80716=CARTESIAN_POINT ( 'NONE',  ( 113.1080853710608238, -29.03773216254911915, 79.54705384733995288 ) ) ;
#80718=CARTESIAN_POINT ( 'NONE',  ( 107.9164806882189254, -47.13338536194948603, 173.6413395616249886 ) ) ;
#80719=CARTESIAN_POINT ( 'NONE',  ( 51.06648329127400388, 22.62155284005901024, 339.0006252759110339 ) ) ;
#80720=CARTESIAN_POINT ( 'NONE',  ( 172.5667039024480687, -36.32844715993499563, 129.9678068554150059 ) ) ;
#80722=CARTESIAN_POINT ( 'NONE',  ( 188.5667039024483529, -48.82844715993431350, 293.2178068554150059 ) ) ;
#80724=CARTESIAN_POINT ( 'NONE',  ( 21.03715912545738220, -47.82818131006197149, 193.9678068554150627 ) ) ;
#80725=PLANE ( 'NONE',  #18697 ) ;
#80726=CARTESIAN_POINT ( 'NONE',  ( 118.0872578842352993, -35.40452791748241879, 238.9337205140059552 ) ) ;
#80729=CARTESIAN_POINT ( 'NONE',  ( 116.3364580279229301, -41.54664843801584340, 284.4441967044824082 ) ) ;
#80730=CARTESIAN_POINT ( 'NONE',  ( 97.70743813507087339, -42.69650533217181021, 137.7661014663869992 ) ) ;
#80732=CARTESIAN_POINT ( 'NONE',  ( 81.19091742811399115, -39.23916151080219095, 8.028235474616696621 ) ) ;
#80734=CARTESIAN_POINT ( 'NONE',  ( 142.8821648370248170, -72.54478064608022692, 540.9756252759101471 ) ) ;
#80740=CARTESIAN_POINT ( 'NONE',  ( 126.0667039024479550, -14.72944715994094977, 199.5838068554170093 ) ) ;
#80741=CARTESIAN_POINT ( 'NONE',  ( 107.6057229598026197, -48.54288983744045538, 38.61276813305397582 ) ) ;
#80742=CARTESIAN_POINT ( 'NONE',  ( 31.71315051186898870, -31.94127993907790852, -5.074374724088000832 ) ) ;
#80744=CARTESIAN_POINT ( 'NONE',  ( 63.03715912545639100, -24.42818131006026761, 180.4678068554151196 ) ) ;
#80746=CIRCLE ( 'NONE', #15520, 4.749999999999976907 ) ;
#80747=CARTESIAN_POINT ( 'NONE',  ( 109.6796103444932129, -28.56711482602328900, 234.2524198280769951 ) ) ;
#80750=VECTOR ( 'NONE', #64127, 1000.000000000000000 ) ;
#80752=VECTOR ( 'NONE', #50090, 1000.000000000000000 ) ;
#80753=AXIS2_PLACEMENT_3D ( 'NONE', #75638, #55147, #13849 ) ;
#80754=ADVANCED_FACE ( 'NONE', ( #17249 ), #87181, .T. ) ;
#80756=AXIS2_PLACEMENT_3D ( 'NONE', #2135, #23485, #57073 ) ;
#80758=CARTESIAN_POINT ( 'NONE',  ( 188.5667039024479834, -48.82844715994099971, 295.9678068554150059 ) ) ;
#80760=CARTESIAN_POINT ( 'NONE',  ( 103.4018642804673789, -27.34641595622759169, 16.80444044875395448 ) ) ;
#80763=CARTESIAN_POINT ( 'NONE',  ( 100.9535969414460794, -28.70786762247625035, 175.5940665755088048 ) ) ;
#80764=CARTESIAN_POINT ( 'NONE',  ( 104.3638673426610666, -27.29495504168057707, 225.2984824187689981 ) ) ;
#80766=EDGE_CURVE ( 'NONE', #12989, #55881, #79933, .T. ) ;
#80768=EDGE_CURVE ( 'NONE', #85840, #3395, #5178, .T. ) ;
#80769=LINE ( 'NONE', #18520, #50454 ) ;
#80771=CARTESIAN_POINT ( 'NONE',  ( 156.5667039024483813, -48.82844715993569196, 259.7178068554149490 ) ) ;
#80772=CARTESIAN_POINT ( 'NONE',  ( 111.6835086010359532, -29.99796862204811987, 42.41666179816294857 ) ) ;
#80773=EDGE_CURVE ( 'NONE', #18895, #59994, #38129, .T. ) ;
#80774=EDGE_CURVE ( 'NONE', #7579, #23174, #65822, .T. ) ;
#80775=VECTOR ( 'NONE', #54293, 1000.000000000000000 ) ;
#80776=CARTESIAN_POINT ( 'NONE',  ( 136.1807380203812272, -16.97076862299123334, 7.459445689446392969 ) ) ;
#80783=EDGE_CURVE ( 'NONE', #25445, #60868, #24063, .T. ) ;
#80785=CARTESIAN_POINT ( 'NONE',  ( 98.20221454234541625, -43.33276655250838871, 111.8480062282919647 ) ) ;
#80786=VERTEX_POINT ( 'NONE', #80823 ) ;
#80787=CARTESIAN_POINT ( 'NONE',  ( 114.4871815801477624, -30.46814820527590228, 73.80670554236196779 ) ) ;
#80788=EDGE_CURVE ( 'NONE', #7841, #41944, #57370, .T. ) ;
#80789=DIRECTION ( 'NONE',  ( -0.7071067811874389708, 0.7071067811856560636, 0.000000000000000000 ) ) ;
#80790=CARTESIAN_POINT ( 'NONE',  ( 110.4802244392091950, -27.25226000720831721, 96.23301187732596418 ) ) ;
#80791=DIRECTION ( 'NONE',  ( 1.000000000000000000, 4.299999999999999979E-14, 9.351236661543306751E-17 ) ) ;
#80792=DIRECTION ( 'NONE',  ( 0.9963424814100680926, -0.08544974978095698503, 0.000000000000000000 ) ) ;
#80793=CARTESIAN_POINT ( 'NONE',  ( 97.08395347075709481, -39.80944164022105980, 17.56419670448195092 ) ) ;
#80795=CARTESIAN_POINT ( 'NONE',  ( 113.2459685721311047, -28.75903239629483465, 180.5526760553944996 ) ) ;
#80796=EDGE_LOOP ( 'NONE', ( #10376, #10347 ) ) ;
#80797=CARTESIAN_POINT ( 'NONE',  ( 117.0608477614241707, -38.08078333794142623, 258.7188941364966581 ) ) ;
#80799=DIRECTION ( 'NONE',  ( 1.000000000000000000, 6.145690160522480771E-16, 0.000000000000000000 ) ) ;
#80800=VERTEX_POINT ( 'NONE', #31753 ) ;
#80802=EDGE_CURVE ( 'NONE', #35086, #1484, #60341, .T. ) ;
#80804=ORIENTED_EDGE ( 'NONE', *, *, #75020, .F. ) ;
#80805=CARTESIAN_POINT ( 'NONE',  ( 111.3277751695583078, -45.53312973143663811, 247.9356252759109509 ) ) ;
#80806=EDGE_CURVE ( 'NONE', #66670, #38273, #80599, .T. ) ;
#80807=CARTESIAN_POINT ( 'NONE',  ( 110.9910846855449478, -27.45570243918006170, 124.7564986738925796 ) ) ;
#80808=DIRECTION ( 'NONE',  ( 1.000000000000000078E-15, -1.000000000000000083E-30, -1.000000000000000000 ) ) ;
#80809=CARTESIAN_POINT ( 'NONE',  ( 118.7325469213664633, -34.64676260937859098, 44.96705384733895272 ) ) ;
#80810=CARTESIAN_POINT ( 'NONE',  ( 97.86649994386787910, -40.64904342295498907, 42.64697140597041880 ) ) ;
#80811=ADVANCED_FACE ( 'NONE', ( #45808 ), #25386, .T. ) ;
#80813=CARTESIAN_POINT ( 'NONE',  ( 104.4897322876167323, -26.97885769723445648, 115.2836109755910030 ) ) ;
#80814=VECTOR ( 'NONE', #84327, 1000.000000000000000 ) ;
#80816=VECTOR ( 'NONE', #10918, 1000.000000000000000 ) ;
#80817=DIRECTION ( 'NONE',  ( -2.900000000000000265E-14, 2.000000000000000155E-15, -1.000000000000000000 ) ) ;
#80818=EDGE_LOOP ( 'NONE', ( #76552, #11046 ) ) ;
#80819=VECTOR ( 'NONE', #20173, 1000.000000000000000 ) ;
#80822=CARTESIAN_POINT ( 'NONE',  ( 118.0844448206164827, -36.21142561920247971, 268.8518157521015723 ) ) ;
#80823=CARTESIAN_POINT ( 'NONE',  ( 32.56670390244700997, -18.82844715994112050, 342.9256252759109884 ) ) ;
#80824=AXIS2_PLACEMENT_3D ( 'NONE', #34395, #62106, #89838 ) ;
#80827=CARTESIAN_POINT ( 'NONE',  ( 115.1439687268531600, -40.82418761129420659, 247.8876579233149755 ) ) ;
#80829=CARTESIAN_POINT ( 'NONE',  ( 109.7644292386349889, -47.42453529627113085, 88.78514908543493789 ) ) ;
#80831=CARTESIAN_POINT ( 'NONE',  ( 116.8367917427482467, -32.96809911012589112, 139.1184824187679396 ) ) ;
#80834=ORIENTED_EDGE ( 'NONE', *, *, #55799, .F. ) ;
#80835=CARTESIAN_POINT ( 'NONE',  ( 32.15435173583699680, -31.62489322948790971, -5.074374724088000832 ) ) ;
#80836=CARTESIAN_POINT ( 'NONE',  ( 107.0664832912748068, -36.72944715993923381, -4.074374724089028454 ) ) ;
#80838=CARTESIAN_POINT ( 'NONE',  ( 25.56670390244820368, -48.82844715994168183, 259.7178068554150059 ) ) ;
#80839=ORIENTED_EDGE ( 'NONE', *, *, #52464, .T. ) ;
#80840=CARTESIAN_POINT ( 'NONE',  ( 100.9544648868430414, -28.70718114071191351, 50.59397893232809906 ) ) ;
#80841=CARTESIAN_POINT ( 'NONE',  ( 114.0157635323931515, -28.07379075743241259, 119.5261014663869474 ) ) ;
#80842=ORIENTED_EDGE ( 'NONE', *, *, #567, .T. ) ;
#80845=PLANE ( 'NONE',  #20057 ) ;
#80847=CARTESIAN_POINT ( 'NONE',  ( 107.0664832912739399, -36.72944715994095333, 290.1356252759106837 ) ) ;
#80848=DIRECTION ( 'NONE',  ( 0.000000000000000000, 0.000000000000000000, -1.000000000000000000 ) ) ;
#80849=ORIENTED_EDGE ( 'NONE', *, *, #22016, .T. ) ;
#80851=CARTESIAN_POINT ( 'NONE',  ( 107.9474950258210413, -25.68774170017952940, 115.0251490854349612 ) ) ;
#80853=CARTESIAN_POINT ( 'NONE',  ( 107.0664832912739968, -0.2185775633790978945, 333.4006252759120343 ) ) ;
#80855=EDGE_LOOP ( 'NONE', ( #64605, #55159, #82599, #8243 ) ) ;
#80859=FACE_OUTER_BOUND ( 'NONE', #59183, .T. ) ;
#80861=CARTESIAN_POINT ( 'NONE',  ( 20.03715912545729338, -24.42818131006189830, 313.9678068554150059 ) ) ;
#80862=FACE_OUTER_BOUND ( 'NONE', #27360, .T. ) ;
#80866=CARTESIAN_POINT ( 'NONE',  ( 109.6430122704383763, -46.48008669675207472, 33.78145862070494587 ) ) ;
#80868=CARTESIAN_POINT ( 'NONE',  ( 97.28849942844340148, -36.49606577720026479, 192.3070538473389490 ) ) ;
#80869=DIRECTION ( 'NONE',  ( 1.000000000000000078E-15, 1.000000000000000083E-30, -1.000000000000000000 ) ) ;
#80870=ORIENTED_EDGE ( 'NONE', *, *, #37294, .F. ) ;
#80872=CARTESIAN_POINT ( 'NONE',  ( 109.7352083718000131, -46.17358189742679286, 68.79562527591099297 ) ) ;
#80873=CARTESIAN_POINT ( 'NONE',  ( 21.03715912545830591, -47.82818131006186491, 237.4678068554150059 ) ) ;
#80874=CARTESIAN_POINT ( 'NONE',  ( 138.8167039024479834, -67.87844715994100397, 35.51780685541480409 ) ) ;
#80875=PLANE ( 'NONE',  #34368 ) ;
#80876=EDGE_CURVE ( 'NONE', #58384, #18192, #6736, .T. ) ;
#80880=AXIS2_PLACEMENT_3D ( 'NONE', #17791, #74546, #5060 ) ;
#80881=EDGE_LOOP ( 'NONE', ( #60463, #53826, #72379, #45023 ) ) ;
#80883=CARTESIAN_POINT ( 'NONE',  ( 112.7895289397446561, -28.43984804668171051, 236.0272975916119549 ) ) ;
#80884=ADVANCED_FACE ( 'NONE', ( #83065 ), #13552, .T. ) ;
#80886=LINE ( 'NONE', #18639, #79211 ) ;
#80891=DIRECTION ( 'NONE',  ( 0.000000000000000000, 1.000000000000000000, 0.000000000000000000 ) ) ;
#80892=CARTESIAN_POINT ( 'NONE',  ( 194.0371591254573218, -24.42818131005417825, 249.9678068554149775 ) ) ;
#80895=CARTESIAN_POINT ( 'NONE',  ( 97.06391965937397970, -37.34326081457973601, 37.37502593264307649 ) ) ;
#80896=ORIENTED_EDGE ( 'NONE', *, *, #19678, .F. ) ;
#80897=CARTESIAN_POINT ( 'NONE',  ( 100.5506404981706510, -27.80068015945615656, 30.56610146638794134 ) ) ;
#80898=ORIENTED_EDGE ( 'NONE', *, *, #54892, .T. ) ;
#80900=CARTESIAN_POINT ( 'NONE',  ( 99.31750181266291122, -39.29518527230509051, 239.3995189410199487 ) ) ;
#80901=EDGE_CURVE ( 'NONE', #9938, #3093, #33544, .T. ) ;
#80902=AXIS2_PLACEMENT_3D ( 'NONE', #57909, #15249, #57461 ) ;
#80905=CARTESIAN_POINT ( 'NONE',  ( 177.8371591254543489, -47.82818131005477369, 249.9678068554149775 ) ) ;
#80906=CIRCLE ( 'NONE', #14170, 1.000000000000000888 ) ;
#80907=CARTESIAN_POINT ( 'NONE',  ( 172.5664832912729878, -27.82844715994070484, 78.92562527591199739 ) ) ;
#80908=VECTOR ( 'NONE', #80268, 1000.000000000000000 ) ;
#80910=CARTESIAN_POINT ( 'NONE',  ( 117.2345208925008109, -41.18012235578145663, 204.4861014663869696 ) ) ;
#80912=AXIS2_PLACEMENT_3D ( 'NONE', #70935, #65759, #3547 ) ;
#80914=CARTESIAN_POINT ( 'NONE',  ( 104.2021517265174992, -25.17926459036136322, 86.26991099019699050 ) ) ;
#80915=FACE_OUTER_BOUND ( 'NONE', #70514, .T. ) ;
#80916=EDGE_LOOP ( 'NONE', ( #56000, #7482, #36553, #89683 ) ) ;
#80917=VERTEX_POINT ( 'NONE', #75787 ) ;
#80918=ORIENTED_EDGE ( 'NONE', *, *, #24943, .T. ) ;
#80919=CARTESIAN_POINT ( 'NONE',  ( 97.81136857603131318, -40.51756142711754194, 161.6353372277744143 ) ) ;
#80920=DIRECTION ( 'NONE',  ( 0.000000000000000000, 0.000000000000000000, 1.000000000000000000 ) ) ;
#80921=FACE_OUTER_BOUND ( 'NONE', #30757, .T. ) ;
#80922=CARTESIAN_POINT ( 'NONE',  ( 103.3817498881349906, -44.01315952142851984, 125.0223760838769778 ) ) ;
#80923=CARTESIAN_POINT ( 'NONE',  ( 96.75463230179867935, -40.77307608890721013, 242.6118157521009664 ) ) ;
#80924=DIRECTION ( 'NONE',  ( 0.000000000000000000, 1.000000000000000000, 0.000000000000000000 ) ) ;
#80930=EDGE_LOOP ( 'NONE', ( #6999, #18936, #84297, #16036 ) ) ;
#80931=AXIS2_PLACEMENT_3D ( 'NONE', #8642, #9527, #2720 ) ;
#80932=VERTEX_POINT ( 'NONE', #62144 ) ;
#80934=ORIENTED_EDGE ( 'NONE', *, *, #20404, .F. ) ;
#80935=EDGE_LOOP ( 'NONE', ( #25872, #78067, #57578, #1936 ) ) ;
#80936=DIRECTION ( 'NONE',  ( 0.000000000000000000, 0.000000000000000000, 1.000000000000000000 ) ) ;
#80939=CARTESIAN_POINT ( 'NONE',  ( 113.0289883941274525, -30.57309799635150682, 173.8867055423629608 ) ) ;
#80940=CARTESIAN_POINT ( 'NONE',  ( 112.1386966202503430, -26.85596833298010111, 19.71086337114896736 ) ) ;
#80941=CARTESIAN_POINT ( 'NONE',  ( 113.2436075868320984, -28.75722666126760529, 125.5524796337008979 ) ) ;
#80943=DIRECTION ( 'NONE',  ( 0.000000000000000000, 0.000000000000000000, -1.000000000000000000 ) ) ;
#80945=EDGE_CURVE ( 'NONE', #73072, #13477, #89877, .T. ) ;
#80947=ORIENTED_EDGE ( 'NONE', *, *, #22130, .T. ) ;
#80948=CARTESIAN_POINT ( 'NONE',  ( 101.2924984490993836, -28.53423124992686155, 166.5645102773719373 ) ) ;
#80949=CIRCLE ( 'NONE', #69332, 2.116999999999980009 ) ;
#80951=CARTESIAN_POINT ( 'NONE',  ( 111.2955958668267584, -45.79294333952354634, 132.9238878757940938 ) ) ;
#80952=EDGE_CURVE ( 'NONE', #54341, #15887, #40357, .T. ) ;
#80953=AXIS2_PLACEMENT_3D ( 'NONE', #79864, #17618, #30795 ) ;
#80954=DIRECTION ( 'NONE',  ( -1.000000000000000078E-15, 1.000000000000000083E-30, 1.000000000000000000 ) ) ;
#80955=ORIENTED_EDGE ( 'NONE', *, *, #87405, .F. ) ;
#80957=CARTESIAN_POINT ( 'NONE',  ( 98.40533970481327231, -42.07952101345657780, 11.76800622829193799 ) ) ;
#80958=CARTESIAN_POINT ( 'NONE',  ( 104.0301208637212369, -47.40549519127628031, 63.36800622829197494 ) ) ;
#80959=DIRECTION ( 'NONE',  ( -1.000000000000000000, 1.011922027653136551E-15, 0.000000000000000000 ) ) ;
#80962=DIRECTION ( 'NONE',  ( 1.000000000000000078E-15, -1.000000000000000000, 0.000000000000000000 ) ) ;
#80964=DIRECTION ( 'NONE',  ( -1.000000000000000000, -4.299999999999999979E-14, -1.000000000000000078E-15 ) ) ;
#80965=CIRCLE ( 'NONE', #41757, 2.999999999999947153 ) ;
#80967=ORIENTED_EDGE ( 'NONE', *, *, #51616, .F. ) ;
#80968=CARTESIAN_POINT ( 'NONE',  ( 107.6091449839925929, -48.61785814739364042, 42.61276813305398292 ) ) ;
#80969=CARTESIAN_POINT ( 'NONE',  ( 99.08600912489498569, -29.96680234772274787, 211.7670538473399517 ) ) ;
#80970=CARTESIAN_POINT ( 'NONE',  ( 101.1293421793351968, -28.09060746778665418, 46.55562527591094835 ) ) ;
#80971=AXIS2_PLACEMENT_3D ( 'NONE', #45765, #19427, #87581 ) ;
#80972=CARTESIAN_POINT ( 'NONE',  ( 109.6444706913881930, -46.47971972121219864, 172.7775026101618039 ) ) ;
#80973=DIRECTION ( 'NONE',  ( -0.9254794337955620787, -0.3787978585227823602, 0.000000000000000000 ) ) ;
#80974=CARTESIAN_POINT ( 'NONE',  ( 172.5664832912740110, 0.2215528400590013880, 16.80862527591200006 ) ) ;
#80976=EDGE_CURVE ( 'NONE', #9481, #88962, #5859, .T. ) ;
#80977=DIRECTION ( 'NONE',  ( 1.000000000000000000, 4.163336342344347755E-14, 0.000000000000000000 ) ) ;
#80979=EDGE_CURVE ( 'NONE', #78000, #27916, #9832, .T. ) ;
#80980=CARTESIAN_POINT ( 'NONE',  ( 99.54941199951412045, -42.98700854487240974, 112.8784824187679732 ) ) ;
#80982=CARTESIAN_POINT ( 'NONE',  ( 142.8690268918515471, 4.118420757222291506, 542.9756252759101471 ) ) ;
#80984=EDGE_CURVE ( 'NONE', #18119, #27695, #75049, .T. ) ;
#80985=CARTESIAN_POINT ( 'NONE',  ( 105.1150531980676561, -26.51080800785444680, 231.2270538473399597 ) ) ;
#80986=CARTESIAN_POINT ( 'NONE',  ( 37.56670390244801183, -48.82844715994119866, 300.4678068554150059 ) ) ;
#80987=DIRECTION ( 'NONE',  ( 0.000000000000000000, 1.000000000000000000, 0.000000000000000000 ) ) ;
#80988=CARTESIAN_POINT ( 'NONE',  ( 142.8698897858160706, -0.9167816978817300289, 542.9756252759101471 ) ) ;
#80990=CARTESIAN_POINT ( 'NONE',  ( 131.4524275574069350, -37.60567372263788144, 2.908038864009826252 ) ) ;
#80993=CARTESIAN_POINT ( 'NONE',  ( 108.7386892141029477, -46.36620816325537930, 167.7127681330539701 ) ) ;
#80994=AXIS2_PLACEMENT_3D ( 'NONE', #4129, #58634, #2359 ) ;
#80995=ORIENTED_EDGE ( 'NONE', *, *, #28378, .F. ) ;
#80996=EDGE_LOOP ( 'NONE', ( #2265, #84618 ) ) ;
#80997=CARTESIAN_POINT ( 'NONE',  ( 99.03419491772403660, -31.85514013008181777, 122.3120594963729673 ) ) ;
#80999=DIRECTION ( 'NONE',  ( 1.000000000000000078E-15, -1.000000000000000000, 0.000000000000000000 ) ) ;
#81000=CARTESIAN_POINT ( 'NONE',  ( 112.0813997088635432, -45.80630777137064058, 248.9661014663869878 ) ) ;
#81004=EDGE_CURVE ( 'NONE', #56941, #22696, #86665, .T. ) ;
#81007=LINE ( 'NONE', #11949, #47809 ) ;
#81009=CARTESIAN_POINT ( 'NONE',  ( 102.6926969729869938, -27.29023857175969781, 180.4213395616249898 ) ) ;
#81010=DIRECTION ( 'NONE',  ( 8.673617379884035472E-16, 1.000000000000000000, 0.000000000000000000 ) ) ;
#81011=ORIENTED_EDGE ( 'NONE', *, *, #17537, .T. ) ;
#81012=ORIENTED_EDGE ( 'NONE', *, *, #31518, .F. ) ;
#81014=CARTESIAN_POINT ( 'NONE',  ( 82.53070037945653326, -19.95069274174520402, 7.120636252911432429 ) ) ;
#81015=DIRECTION ( 'NONE',  ( 0.000000000000000000, 0.000000000000000000, -1.000000000000000000 ) ) ;
#81017=AXIS2_PLACEMENT_3D ( 'NONE', #21991, #49659, #43744 ) ;
#81019=ORIENTED_EDGE ( 'NONE', *, *, #37073, .F. ) ;
#81022=( BOUNDED_CURVE ( )  B_SPLINE_CURVE ( 3, ( #72987, #66164, #3950, #87080 ),
 .UNSPECIFIED., .F., .T. ) 
 B_SPLINE_CURVE_WITH_KNOTS ( ( 4, 4 ),
 ( 7.227822158068946767E-12, 1.570796326804053678 ),
 .UNSPECIFIED. ) 
 CURVE ( )  GEOMETRIC_REPRESENTATION_ITEM ( )  RATIONAL_B_SPLINE_CURVE ( ( 1.000000000000000000, 0.8047378541239101901, 0.8047378541239101901, 1.000000000000000000 ) ) 
 REPRESENTATION_ITEM ( '' )  );
#81023=CARTESIAN_POINT ( 'NONE',  ( 114.6056301357651819, -29.52887111919123697, 234.4327681330539690 ) ) ;
#81027=CIRCLE ( 'NONE', #11362, 1.000000000000000888 ) ;
#81029=LINE ( 'NONE', #82364, #66657 ) ;
#81030=CARTESIAN_POINT ( 'NONE',  ( 99.50478645252971432, -43.30584932723667890, 166.8960762454959195 ) ) ;
#81031=CARTESIAN_POINT ( 'NONE',  ( 97.82153671710952381, -35.93768077729445309, 34.07666179816293095 ) ) ;
#81032=VECTOR ( 'NONE', #37078, 1000.000000000000000 ) ;
#81033=CARTESIAN_POINT ( 'NONE',  ( 102.6884963789050289, -46.90384819475383438, 133.2651490854349561 ) ) ;
#81036=VECTOR ( 'NONE', #37260, 1000.000000000000000 ) ;
#81044=EDGE_LOOP ( 'NONE', ( #78090, #21361, #3775, #41979 ) ) ;
#81045=CARTESIAN_POINT ( 'NONE',  ( 183.6524903400785718, -49.32844715993451956, 180.4678068554150343 ) ) ;
#81046=CIRCLE ( 'NONE', #59290, 11.45913725231036118 ) ;
#81047=CARTESIAN_POINT ( 'NONE',  ( 100.6982016950751699, -42.46504578929962292, 56.33241982807696502 ) ) ;
#81048=CARTESIAN_POINT ( 'NONE',  ( 106.4823715260129688, -24.86804634255730662, 195.1156252759109861 ) ) ;
#81049=CARTESIAN_POINT ( 'NONE',  ( 117.2886123466743271, -34.79635738071011986, 158.9756252759109714 ) ) ;
#81051=CARTESIAN_POINT ( 'NONE',  ( 96.70769389551976758, -42.43415482991306220, 22.72705384733997391 ) ) ;
#81052=DIRECTION ( 'NONE',  ( -1.000000000000000000, -4.163336342344275811E-14, 0.000000000000000000 ) ) ;
#81053=DIRECTION ( 'NONE',  ( -0.3818493186865920541, 0.9242245927363033076, 0.000000000000000000 ) ) ;
#81054=EDGE_LOOP ( 'NONE', ( #24805, #47358, #79145, #69788 ) ) ;
#81057=EDGE_CURVE ( 'NONE', #11825, #53364, #22621, .T. ) ;
#81058=DIRECTION ( 'NONE',  ( 0.000000000000000000, 0.000000000000000000, -1.000000000000000000 ) ) ;
#81059=CARTESIAN_POINT ( 'NONE',  ( 106.2986956077118208, -47.17057584017531724, 222.5184824187679453 ) ) ;
#81061=CARTESIAN_POINT ( 'NONE',  ( 113.0222799004901333, -45.32912119007338703, 203.0584824187679374 ) ) ;
#81062=CYLINDRICAL_SURFACE ( 'NONE', #73228, 9.999999999999998224 ) ;
#81064=CARTESIAN_POINT ( 'NONE',  ( 53.56670390244749314, -48.82844715994058049, 129.9678068554150911 ) ) ;
#81065=CARTESIAN_POINT ( 'NONE',  ( 34.33598329127499227, -36.32844715994100682, 237.4678068554150059 ) ) ;
#81066=CARTESIAN_POINT ( 'NONE',  ( 112.5738672296349705, -43.44503014251905171, 277.6356252759110248 ) ) ;
#81068=CARTESIAN_POINT ( 'NONE',  ( 113.1781702599491979, -44.75196522829472912, 174.0939462851112580 ) ) ;
#81077=DIRECTION ( 'NONE',  ( 0.000000000000000000, 1.000000000000000000, 0.000000000000000000 ) ) ;
#81078=CARTESIAN_POINT ( 'NONE',  ( 97.07499705966343129, -41.51125058752681696, 216.6937205140059461 ) ) ;
#81079=CARTESIAN_POINT ( 'NONE',  ( 108.5379568639253449, -26.40872756427751611, 100.9641967044829727 ) ) ;
#81080=CARTESIAN_POINT ( 'NONE',  ( 104.3129624051631907, -25.97697669550431243, 241.2880062282919482 ) ) ;
#81081=LINE ( 'NONE', #74249, #16439 ) ;
#81083=CARTESIAN_POINT ( 'NONE',  ( 116.3212776292296127, -32.94146857471318413, 287.6356252759109680 ) ) ;
#81084=CARTESIAN_POINT ( 'NONE',  ( 69.68306499799194853, -72.55732494037970071, 540.9756252759101471 ) ) ;
#81088=CIRCLE ( 'NONE', #8517, 3.600000000000000089 ) ;
#81093=CARTESIAN_POINT ( 'NONE',  ( 115.3083805796901373, -34.38525866856544866, 148.4695626852189605 ) ) ;
#81096=VERTEX_POINT ( 'NONE', #2173 ) ;
#81097=DIRECTION ( 'NONE',  ( -1.000000000000000078E-15, 1.000000000000000083E-30, 1.000000000000000000 ) ) ;
#81099=CARTESIAN_POINT ( 'NONE',  ( 114.0662423116485229, -44.47333502991302367, 129.1613395616249704 ) ) ;
#81100=CARTESIAN_POINT ( 'NONE',  ( 142.0664832912739826, -9.729447159940995959, 14.92562527591100618 ) ) ;
#81101=EDGE_CURVE ( 'NONE', #32858, #61827, #50399, .T. ) ;
#81105=ADVANCED_FACE ( 'NONE', ( #1276 ), #46030, .T. ) ;
#81106=CARTESIAN_POINT ( 'NONE',  ( 115.7831076713507343, -41.80230950795940714, 109.4064586094590652 ) ) ;
#81107=VECTOR ( 'NONE', #26637, 1000.000000000000000 ) ;
#81108=CARTESIAN_POINT ( 'NONE',  ( 115.5638989210038119, -29.55965564860105843, 74.38419670448293175 ) ) ;
#81110=ORIENTED_EDGE ( 'NONE', *, *, #52130, .T. ) ;
#81113=CARTESIAN_POINT ( 'NONE',  ( 98.36735121233628831, -42.37464764417345719, 142.7965776568629508 ) ) ;
#81118=CIRCLE ( 'NONE', #31799, 0.5000000000000004441 ) ;
#81119=FACE_OUTER_BOUND ( 'NONE', #64240, .T. ) ;
#81122=CARTESIAN_POINT ( 'NONE',  ( 106.6611865629619018, -26.33404432545455265, 85.10705384733896040 ) ) ;
#81123=ORIENTED_EDGE ( 'NONE', *, *, #73892, .T. ) ;
#81124=VERTEX_POINT ( 'NONE', #87517 ) ;
#81128=CARTESIAN_POINT ( 'NONE',  ( 114.8623915286450199, -39.24071799505598079, 156.3966617981629668 ) ) ;
#81129=AXIS2_PLACEMENT_3D ( 'NONE', #60289, #47554, #75285 ) ;
#81130=DIRECTION ( 'NONE',  ( 0.7071067811575898476, -0.7071067812155052978, 0.000000000000000000 ) ) ;
#81131=ORIENTED_EDGE ( 'NONE', *, *, #6962, .T. ) ;
#81132=ORIENTED_EDGE ( 'NONE', *, *, #40241, .F. ) ;
#81134=ORIENTED_EDGE ( 'NONE', *, *, #80945, .F. ) ;
#81137=CARTESIAN_POINT ( 'NONE',  ( 109.6768956016245227, -27.70380185851407973, 211.2720594963729752 ) ) ;
#81139=LINE ( 'NONE', #32956, #44324 ) ;
#81140=EDGE_CURVE ( 'NONE', #76300, #8047, #66159, .T. ) ;
#81141=PLANE ( 'NONE',  #47244 ) ;
#81145=AXIS2_PLACEMENT_3D ( 'NONE', #5938, #35402, #55831 ) ;
#81146=ORIENTED_EDGE ( 'NONE', *, *, #70927, .T. ) ;
#81148=ORIENTED_EDGE ( 'NONE', *, *, #16815, .F. ) ;
#81149=ADVANCED_FACE ( 'NONE', ( #18917 ), #65717, .F. ) ;
#81150=CARTESIAN_POINT ( 'NONE',  ( 109.9373871219287082, -28.56496087843131448, 252.6376141791152747 ) ) ;
#81151=VECTOR ( 'NONE', #58218, 1000.000000000000000 ) ;
#81152=CARTESIAN_POINT ( 'NONE',  ( 104.2079940790944477, -25.20282339889105927, 90.26991099019693365 ) ) ;
#81153=CARTESIAN_POINT ( 'NONE',  ( 101.7220374796296909, -27.76276858577399409, 85.50419670448295051 ) ) ;
#81154=CARTESIAN_POINT ( 'NONE',  ( 108.0208457958009234, -27.96381440099374416, 249.5838068554170377 ) ) ;
#81155=DIRECTION ( 'NONE',  ( -0.4214249218767880945, -0.9068632946707806397, -4.214249218767889924E-16 ) ) ;
#81156=CARTESIAN_POINT ( 'NONE',  ( 72.31648329127402519, -45.62589376934781882, -5.074374724089063982 ) ) ;
#81157=CARTESIAN_POINT ( 'NONE',  ( 103.5424053135282634, -26.88047730603072694, 186.3499109901969746 ) ) ;
#81158=CARTESIAN_POINT ( 'NONE',  ( 100.9173739041163174, -44.68471384580785610, 277.0520784369447824 ) ) ;
#81159=ORIENTED_EDGE ( 'NONE', *, *, #18517, .F. ) ;
#81160=LINE ( 'NONE', #67494, #3200 ) ;
#81161=ORIENTED_EDGE ( 'NONE', *, *, #31686, .F. ) ;
#81164=CARTESIAN_POINT ( 'NONE',  ( 51.42025729302698522, -31.94127993907710206, -5.074374724088000832 ) ) ;
#81165=CYLINDRICAL_SURFACE ( 'NONE', #41577, 0.5000000000000031086 ) ;
#81167=CARTESIAN_POINT ( 'NONE',  ( 107.0664832912739399, -36.72944715994095333, 302.6356252759109680 ) ) ;
#81169=CARTESIAN_POINT ( 'NONE',  ( 97.07199446366847440, -35.37919910817579705, 92.21901894701355218 ) ) ;
#81170=CARTESIAN_POINT ( 'NONE',  ( 117.5955728976552166, -42.16808282502534411, 93.44705384733897802 ) ) ;
#81171=CARTESIAN_POINT ( 'NONE',  ( 116.3212776292296127, -32.94146857471318413, 287.6356252759109680 ) ) ;
#81172=DIRECTION ( 'NONE',  ( 1.000000000000000078E-15, -1.000000000000000083E-30, -1.000000000000000000 ) ) ;
#81173=CARTESIAN_POINT ( 'NONE',  ( 116.3191775144681515, -32.94222376661483764, 89.13562527591095375 ) ) ;
#81174=CARTESIAN_POINT ( 'NONE',  ( 32.24491389930059881, -32.11662333284641591, 313.9678068554150059 ) ) ;
#81175=DIRECTION ( 'NONE',  ( 1.000000000000000000, 0.000000000000000000, 9.462128050782575008E-16 ) ) ;
#81176=CARTESIAN_POINT ( 'NONE',  ( 107.6532706963292441, -47.74396045468172645, 193.6308633711489620 ) ) ;
#81177=CARTESIAN_POINT ( 'NONE',  ( 83.06670390244796920, -58.35344715994099829, 231.5838068554150198 ) ) ;
#81178=DIRECTION ( 'NONE',  ( 1.000000000000000000, 0.000000000000000000, 0.000000000000000000 ) ) ;
#81179=VERTEX_POINT ( 'NONE', #3946 ) ;
#81183=CARTESIAN_POINT ( 'NONE',  ( 98.34988348865829266, -31.65649366854221469, 135.9064676967609842 ) ) ;
#81184=EDGE_CURVE ( 'NONE', #14045, #18758, #17142, .T. ) ;
#81186=CARTESIAN_POINT ( 'NONE',  ( 115.8130859178907599, -30.97587361506452197, 254.2899109901966028 ) ) ;
#81187=ORIENTED_EDGE ( 'NONE', *, *, #85707, .F. ) ;
#81189=CARTESIAN_POINT ( 'NONE',  ( 105.7736751693905148, -26.36287077168075754, 266.1756252759109884 ) ) ;
#81190=CARTESIAN_POINT ( 'NONE',  ( 97.75552660847078812, -42.77168409777202385, 142.7965776568629508 ) ) ;
#81192=CARTESIAN_POINT ( 'NONE',  ( 82.77032304066686663, -37.23127003359135756, 6.817519769820709286 ) ) ;
#81193=CIRCLE ( 'NONE', #18783, 0.5000000000000004441 ) ;
#81195=CARTESIAN_POINT ( 'NONE',  ( 188.5667039024479834, -58.35344715994099829, 137.2178068554150059 ) ) ;
#81196=LINE ( 'NONE', #12131, #33695 ) ;
#81198=ORIENTED_EDGE ( 'NONE', *, *, #16812, .T. ) ;
#81200=CIRCLE ( 'NONE', #41994, 1.000000000000000888 ) ;
#81201=ORIENTED_EDGE ( 'NONE', *, *, #87574, .F. ) ;
#81202=CARTESIAN_POINT ( 'NONE',  ( 20.03715912545824906, -46.82818131006190043, 249.9678068554150059 ) ) ;
#81203=CARTESIAN_POINT ( 'NONE',  ( 118.0525141433397636, -37.71481444994962118, 29.74324432352998215 ) ) ;
#81208=DIRECTION ( 'NONE',  ( -1.000000000000000078E-15, 1.000000000000000083E-30, 1.000000000000000000 ) ) ;
#81209=CARTESIAN_POINT ( 'NONE',  ( 172.5664832912740110, -27.82844715994070484, 203.6756252759119832 ) ) ;
#81210=CARTESIAN_POINT ( 'NONE',  ( 104.5043403851385904, -28.58134581971437882, 249.7409912566480727 ) ) ;
#81212=ORIENTED_EDGE ( 'NONE', *, *, #20741, .F. ) ;
#81213=AXIS2_PLACEMENT_3D ( 'NONE', #39908, #62148, #75343 ) ;
#81215=VERTEX_POINT ( 'NONE', #73428 ) ;
#81216=DIRECTION ( 'NONE',  ( 0.9999999853157766072, 0.0001713722456127291416, -9.999999853157765648E-16 ) ) ;
#81217=CARTESIAN_POINT ( 'NONE',  ( 111.4712670676476307, -45.71312987848808973, 182.9392243914140295 ) ) ;
#81218=DIRECTION ( 'NONE',  ( 0.000000000000000000, 0.000000000000000000, -1.000000000000000000 ) ) ;
#81219=DIRECTION ( 'NONE',  ( 0.000000000000000000, 0.000000000000000000, -1.000000000000000000 ) ) ;
#81221=CARTESIAN_POINT ( 'NONE',  ( 101.5279499456468528, -29.13990343739101974, 26.99777378208800727 ) ) ;
#81223=ADVANCED_FACE ( 'NONE', ( #38903 ), #8334, .T. ) ;
#81224=CIRCLE ( 'NONE', #2878, 4.874999999999990230 ) ;
#81226=ADVANCED_FACE ( 'NONE', ( #53403 ), #25729, .T. ) ;
#81227=CARTESIAN_POINT ( 'NONE',  ( 113.9608400058234849, -28.00707201207230668, 274.5441967044828857 ) ) ;
#81230=CARTESIAN_POINT ( 'NONE',  ( 103.5010607639055706, -27.38617375340112403, 56.36656921207620741 ) ) ;
#81231=VECTOR ( 'NONE', #77673, 1000.000000000000000 ) ;
#81232=DIRECTION ( 'NONE',  ( -0.8758084860610321210, -0.03696114963002913867, -0.4812414873652411940 ) ) ;
#81233=CARTESIAN_POINT ( 'NONE',  ( 98.96126485936372319, -37.90763323093077020, 64.25951894101994810 ) ) ;
#81234=DIRECTION ( 'NONE',  ( -2.999999999999999839E-15, 1.000000000000000000, -2.999999999999999900E-30 ) ) ;
#81235=CARTESIAN_POINT ( 'NONE',  ( 130.0664832912740110, -18.82844715994099971, 239.5838068554170377 ) ) ;
#81236=VECTOR ( 'NONE', #45589, 1000.000000000000000 ) ;
#81238=ORIENTED_EDGE ( 'NONE', *, *, #81762, .F. ) ;
#81239=LINE ( 'NONE', #53012, #88570 ) ;
#81241=ORIENTED_EDGE ( 'NONE', *, *, #81919, .T. ) ;
#81242=CARTESIAN_POINT ( 'NONE',  ( 113.9170494572507266, -28.05483877344520849, 124.5565776568629559 ) ) ;
#81243=ORIENTED_EDGE ( 'NONE', *, *, #21100, .F. ) ;
#81244=CARTESIAN_POINT ( 'NONE',  ( 101.5215670198552544, -44.69967496328137457, 86.51527697093396796 ) ) ;
#81245=PLANE ( 'NONE',  #76458 ) ;
#81246=CARTESIAN_POINT ( 'NONE',  ( 109.6943014565619450, -45.19247559555673632, 94.24729759161093057 ) ) ;
#81247=CARTESIAN_POINT ( 'NONE',  ( 97.81168895331838087, -40.51742574516882200, 287.6356252759109680 ) ) ;
#81248=CARTESIAN_POINT ( 'NONE',  ( 107.0664832912739399, -36.72944715994095333, 293.9356252759109793 ) ) ;
#81249=AXIS2_PLACEMENT_3D ( 'NONE', #14067, #21335, #62212 ) ;
#81250=CARTESIAN_POINT ( 'NONE',  ( 103.4696982656617479, -25.41196563057017244, 51.32133956162493149 ) ) ;
#81252=ORIENTED_EDGE ( 'NONE', *, *, #67526, .F. ) ;
#81253=CARTESIAN_POINT ( 'NONE',  ( 116.3214902495786873, -32.94210931476069248, 180.1356252759109680 ) ) ;
#81254=ORIENTED_EDGE ( 'NONE', *, *, #7986, .T. ) ;
#81255=CARTESIAN_POINT ( 'NONE',  ( 77.53258422225754032, -19.79809288067777118, 2.811527366592890154 ) ) ;
#81258=ADVANCED_FACE ( 'NONE', ( #79828, #10750 ), #10320, .T. ) ;
#81259=AXIS2_PLACEMENT_3D ( 'NONE', #7698, #13615, #35387 ) ;
#81260=LINE ( 'NONE', #53943, #33929 ) ;
#81261=ORIENTED_EDGE ( 'NONE', *, *, #89798, .T. ) ;
#81262=CARTESIAN_POINT ( 'NONE',  ( 98.14754276252327259, -43.36755551587079083, 261.8356252759109566 ) ) ;
#81264=CARTESIAN_POINT ( 'NONE',  ( 154.4409905298078058, -0.9147987323338667709, 396.9756252759102040 ) ) ;
#81265=CARTESIAN_POINT ( 'NONE',  ( 117.9246037767874498, -41.47663949653230020, 54.49848241876792088 ) ) ;
#81266=CYLINDRICAL_SURFACE ( 'NONE', #88667, 1.000000000000000888 ) ;
#81267=ORIENTED_EDGE ( 'NONE', *, *, #40200, .F. ) ;
#81270=DIRECTION ( 'NONE',  ( 0.000000000000000000, 0.000000000000000000, 1.000000000000000000 ) ) ;
#81271=ORIENTED_EDGE ( 'NONE', *, *, #7946, .T. ) ;
#81275=CARTESIAN_POINT ( 'NONE',  ( 80.54920390244805617, -58.72944715994108833, 231.5838068554169524 ) ) ;
#81276=CARTESIAN_POINT ( 'NONE',  ( 112.3272512417296980, -28.22507648531173530, 289.6356252759109680 ) ) ;
#81277=DIRECTION ( 'NONE',  ( 1.000000000000000000, 4.163336342344333240E-14, 0.000000000000000000 ) ) ;
#81278=CARTESIAN_POINT ( 'NONE',  ( 107.0664832912739541, -36.72944715994095333, 309.2406250056037038 ) ) ;
#81279=CARTESIAN_POINT ( 'NONE',  ( 99.04430456227140667, -42.84162139839268235, 91.84393114961771687 ) ) ;
#81280=CARTESIAN_POINT ( 'NONE',  ( 98.21912858861395534, -34.79631884261151242, 255.5657531614102709 ) ) ;
#81281=DIRECTION ( 'NONE',  ( 0.000000000000000000, -1.000000000000000000, 0.000000000000000000 ) ) ;
#81282=CARTESIAN_POINT ( 'NONE',  ( 117.3319688044106925, -38.62265419183309945, 84.68133956162593279 ) ) ;
#81283=FACE_OUTER_BOUND ( 'NONE', #55546, .T. ) ;
#81284=CARTESIAN_POINT ( 'NONE',  ( 103.7935660395325073, -26.78486678718983072, 165.3299109901969643 ) ) ;
#81288=AXIS2_PLACEMENT_3D ( 'NONE', #14207, #62347, #128 ) ;
#81289=EDGE_CURVE ( 'NONE', #17437, #47694, #72983, .T. ) ;
#81291=CARTESIAN_POINT ( 'NONE',  ( 57.56670390244832447, -48.82844715994039575, 257.2178068554150627 ) ) ;
#81293=DIRECTION ( 'NONE',  ( -4.237773401492740281E-14, 1.000000000000000000, 0.000000000000000000 ) ) ;
#81297=CARTESIAN_POINT ( 'NONE',  ( 97.81066791858781073, -40.51493114651297134, 51.63541036076257740 ) ) ;
#81298=CARTESIAN_POINT ( 'NONE',  ( 98.41978056949241704, -42.69487473605161654, 126.8070538473389490 ) ) ;
#81299=ORIENTED_EDGE ( 'NONE', *, *, #11010, .T. ) ;
#81303=FACE_OUTER_BOUND ( 'NONE', #58183, .T. ) ;
#81304=EDGE_CURVE ( 'NONE', #35335, #75906, #23482, .T. ) ;
#81305=CARTESIAN_POINT ( 'NONE',  ( 142.0664832912740394, -46.47944715994099596, 14.67562527591100441 ) ) ;
#81306=ORIENTED_EDGE ( 'NONE', *, *, #41872, .F. ) ;
#81308=EDGE_CURVE ( 'NONE', #4456, #26477, #30116, .T. ) ;
#81309=DIRECTION ( 'NONE',  ( 0.7071067811989784069, -0.7071067811741166276, 7.071067811989791923E-16 ) ) ;
#81312=AXIS2_PLACEMENT_3D ( 'NONE', #27051, #7058, #77442 ) ;
#81314=DIRECTION ( 'NONE',  ( -0.1811243269278930978, 0.9834602067165288952, 0.000000000000000000 ) ) ;
#81316=DIRECTION ( 'NONE',  ( -0.000000000000000000, -0.000000000000000000, 1.000000000000000000 ) ) ;
#81317=EDGE_CURVE ( 'NONE', #13444, #50715, #43824, .T. ) ;
#81318=FACE_OUTER_BOUND ( 'NONE', #66835, .T. ) ;
#81319=CARTESIAN_POINT ( 'NONE',  ( 97.31584970183817518, -39.30599062596471072, 106.5314598669042425 ) ) ;
#81321=CARTESIAN_POINT ( 'NONE',  ( 97.12557807017356026, -37.99703648465538208, 181.4273212068781902 ) ) ;
#81322=VECTOR ( 'NONE', #17210, 1000.000000000000000 ) ;
#81323=VERTEX_POINT ( 'NONE', #29329 ) ;
#81325=CARTESIAN_POINT ( 'NONE',  ( 113.6884830475838442, -29.53135334845051574, 195.4841967044819739 ) ) ;
#81329=ADVANCED_FACE ( 'NONE', ( #42474 ), #14808, .T. ) ;
#81330=CARTESIAN_POINT ( 'NONE',  ( 104.6499073705539473, -46.24122592705968771, 43.37848241876795896 ) ) ;
#81331=DIRECTION ( 'NONE',  ( 0.000000000000000000, 0.000000000000000000, -1.000000000000000000 ) ) ;
#81332=EDGE_CURVE ( 'NONE', #51305, #33391, #57009, .T. ) ;
#81334=EDGE_CURVE ( 'NONE', #28440, #43956, #7976, .T. ) ;
#81335=DIRECTION ( 'NONE',  ( 1.639958061481212836E-42, -4.100000000000000342E-29, -1.000000000000000000 ) ) ;
#81337=ORIENTED_EDGE ( 'NONE', *, *, #32838, .T. ) ;
#81338=CARTESIAN_POINT ( 'NONE',  ( 97.81413651554109379, -40.51640884438177181, 97.63607350422876152 ) ) ;
#81342=CARTESIAN_POINT ( 'NONE',  ( 106.8838381269920745, -46.12323054477403161, 223.9806309249449612 ) ) ;
#81343=AXIS2_PLACEMENT_3D ( 'NONE', #9557, #37262, #22297 ) ;
#81345=DIRECTION ( 'NONE',  ( 1.907762142705490052E-15, 7.167082501179359715E-16, -1.000000000000000000 ) ) ;
#81348=DIRECTION ( 'NONE',  ( 1.000000000000000000, 0.000000000000000000, 0.000000000000000000 ) ) ;
#81349=ORIENTED_EDGE ( 'NONE', *, *, #43205, .F. ) ;
#81350=DIRECTION ( 'NONE',  ( 0.9963424814100680926, -0.08544974978095712381, 0.000000000000000000 ) ) ;
#81352=VERTEX_POINT ( 'NONE', #8435 ) ;
#81353=CARTESIAN_POINT ( 'NONE',  ( 104.5933598291445463, -26.62426044571792616, 285.2670538473396391 ) ) ;
#81355=ORIENTED_EDGE ( 'NONE', *, *, #70057, .T. ) ;
#81356=CARTESIAN_POINT ( 'NONE',  ( 101.6421866332951396, -42.82917926744636361, 264.8166617981626700 ) ) ;
#81358=CARTESIAN_POINT ( 'NONE',  ( 116.2045471004838078, -43.06251688283441581, 163.3441967044829823 ) ) ;
#81360=CARTESIAN_POINT ( 'NONE',  ( 130.1657039024480014, -18.82844715994099971, 239.5838068554170377 ) ) ;
#81361=DIRECTION ( 'NONE',  ( 0.000000000000000000, 0.000000000000000000, 1.000000000000000000 ) ) ;
#81362=CARTESIAN_POINT ( 'NONE',  ( 115.4227270478554317, -30.42340481720227885, 215.3413395616249773 ) ) ;
#81364=VERTEX_POINT ( 'NONE', #707 ) ;
#81365=CARTESIAN_POINT ( 'NONE',  ( 109.6947933286257353, -47.51320739032397000, 83.75467289495897205 ) ) ;
#81366=DIRECTION ( 'NONE',  ( 1.000000000000000078E-15, 0.000000000000000000, 1.000000000000000000 ) ) ;
#81368=VERTEX_POINT ( 'NONE', #85203 ) ;
#81369=ORIENTED_EDGE ( 'NONE', *, *, #12050, .F. ) ;
#81371=CARTESIAN_POINT ( 'NONE',  ( 45.77381068350460680, -48.62134037888156968, 300.4678068554150059 ) ) ;
#81372=DIRECTION ( 'NONE',  ( 0.000000000000000000, -1.000000000000000000, 0.000000000000000000 ) ) ;
#81373=DIRECTION ( 'NONE',  ( -0.9254794337955620787, -0.3787978585227822492, 0.000000000000000000 ) ) ;
#81374=CARTESIAN_POINT ( 'NONE',  ( 103.4072989863811074, -28.88653346237834185, 133.2299951314959685 ) ) ;
#81375=CARTESIAN_POINT ( 'NONE',  ( 98.01791376823749147, -44.42006743888428133, 222.8870538473399563 ) ) ;
#81379=CARTESIAN_POINT ( 'NONE',  ( 136.8005346357622614, -37.07423037058595838, 3.076719480830206077 ) ) ;
#81380=AXIS2_PLACEMENT_3D ( 'NONE', #16475, #30548, #84189 ) ;
#81382=EDGE_LOOP ( 'NONE', ( #9717, #35343 ) ) ;
#81383=CARTESIAN_POINT ( 'NONE',  ( 31.56670390244700641, -19.82844715994111340, -5.074374724088000832 ) ) ;
#81386=ORIENTED_EDGE ( 'NONE', *, *, #61861, .T. ) ;
#81387=DIRECTION ( 'NONE',  ( -1.000200923085726652E-15, -1.000000000000000000, 0.000000000000000000 ) ) ;
#81388=CYLINDRICAL_SURFACE ( 'NONE', #84961, 10.00000000000000711 ) ;
#81390=CARTESIAN_POINT ( 'NONE',  ( 97.31589562384981207, -39.30610287545482606, 26.53146951830015610 ) ) ;
#81391=CARTESIAN_POINT ( 'NONE',  ( 102.8925193805077498, -44.76628084087394654, 166.6057531614099503 ) ) ;
#81392=CARTESIAN_POINT ( 'NONE',  ( 96.14704956656235879, -38.72415284237285960, 51.48229194257797303 ) ) ;
#81394=ORIENTED_EDGE ( 'NONE', *, *, #82021, .F. ) ;
#81395=EDGE_CURVE ( 'NONE', #14785, #11421, #71563, .T. ) ;
#81398=EDGE_LOOP ( 'NONE', ( #1258, #41773, #8209, #6027 ) ) ;
#81399=EDGE_CURVE ( 'NONE', #1134, #24776, #22079, .T. ) ;
#81400=AXIS2_PLACEMENT_3D ( 'NONE', #22129, #70713, #42973 ) ;
#81402=CARTESIAN_POINT ( 'NONE',  ( 97.80969226196111777, -40.51824922604903634, 262.6357212258262166 ) ) ;
#81403=ORIENTED_EDGE ( 'NONE', *, *, #76967, .T. ) ;
#81405=CARTESIAN_POINT ( 'NONE',  ( 152.4532656103850172, -72.54314042502360849, 542.9756252759101471 ) ) ;
#81407=DIRECTION ( 'NONE',  ( -0.9254794337955621897, -0.3787978585227819717, 0.000000000000000000 ) ) ;
#81408=AXIS2_PLACEMENT_3D ( 'NONE', #14479, #50774, #71681 ) ;
#81410=CARTESIAN_POINT ( 'NONE',  ( 25.56670390244797275, -58.35344715994099829, 173.2178068554149775 ) ) ;
#81411=ORIENTED_EDGE ( 'NONE', *, *, #72352, .T. ) ;
#81412=CARTESIAN_POINT ( 'NONE',  ( 117.5344697633125577, -37.28603910398157240, 18.78419670448294809 ) ) ;
#81413=CARTESIAN_POINT ( 'NONE',  ( 96.91449086013869874, -32.24229349230230923, 51.98324432352996638 ) ) ;
#81414=ADVANCED_FACE ( 'NONE', ( #15701 ), #43375, .T. ) ;
#81417=CARTESIAN_POINT ( 'NONE',  ( 31.71315051185421297, -33.70561438052095582, 193.9678068554150911 ) ) ;
#81418=CARTESIAN_POINT ( 'NONE',  ( 133.3151861768211006, -39.40257939794550879, 8.160477455076955877 ) ) ;
#81421=EDGE_CURVE ( 'NONE', #78184, #76706, #22970, .T. ) ;
#81424=CARTESIAN_POINT ( 'NONE',  ( 109.6539202653692087, -46.87399426414072678, 47.77562527591094721 ) ) ;
#81425=CARTESIAN_POINT ( 'NONE',  ( 104.4537254180046375, -26.63707460721619213, 196.2784824187679362 ) ) ;
#81426=CARTESIAN_POINT ( 'NONE',  ( 98.62975546523678361, -43.90627301359564427, 72.89943479972099283 ) ) ;
#81428=DIRECTION ( 'NONE',  ( 0.000000000000000000, 1.000000000000000000, 0.000000000000000000 ) ) ;
#81430=ORIENTED_EDGE ( 'NONE', *, *, #43012, .F. ) ;
#81431=CARTESIAN_POINT ( 'NONE',  ( 109.1197153606379828, -46.32621810461552059, 103.7441967044819791 ) ) ;
#81433=ORIENTED_EDGE ( 'NONE', *, *, #39314, .T. ) ;
#81434=VECTOR ( 'NONE', #30906, 1000.000000000000000 ) ;
#81435=CARTESIAN_POINT ( 'NONE',  ( 97.03753386688410387, -33.96379371595042329, 247.1127681330539758 ) ) ;
#81436=CARTESIAN_POINT ( 'NONE',  ( 113.1776502951240388, -44.75236549504541728, 254.0960424504467596 ) ) ;
#81437=FACE_OUTER_BOUND ( 'NONE', #75411, .T. ) ;
#81438=CARTESIAN_POINT ( 'NONE',  ( 179.1667039024460166, -28.27351298637280408, -5.074374724088000832 ) ) ;
#81439=DIRECTION ( 'NONE',  ( -0.000000000000000000, -0.000000000000000000, 1.000000000000000000 ) ) ;
#81440=EDGE_CURVE ( 'NONE', #14322, #26947, #64732, .T. ) ;
#81442=DIRECTION ( 'NONE',  ( 0.000000000000000000, 0.000000000000000000, -1.000000000000000000 ) ) ;
#81444=CARTESIAN_POINT ( 'NONE',  ( 113.8941270090217444, -29.67983328691845557, 174.4641967044829585 ) ) ;
#81445=ORIENTED_EDGE ( 'NONE', *, *, #89926, .F. ) ;
#81446=CIRCLE ( 'NONE', #37912, 0.9999999999999800160 ) ;
#81447=ORIENTED_EDGE ( 'NONE', *, *, #74991, .T. ) ;
#81448=CARTESIAN_POINT ( 'NONE',  ( 116.1082436049511415, -39.28347229878176705, 140.0511071154209617 ) ) ;
#81449=CIRCLE ( 'NONE', #23417, 2.116999999999993776 ) ;
#81450=CARTESIAN_POINT ( 'NONE',  ( 113.5448393278429364, -34.07786215028152554, -2.364374724089013391 ) ) ;
#81451=CARTESIAN_POINT ( 'NONE',  ( 100.6687104580203567, -44.89077600156390702, 273.0594347997199520 ) ) ;
#81452=CARTESIAN_POINT ( 'NONE',  ( 172.5664832912740110, -36.32844715994070839, 74.17562527591199739 ) ) ;
#81453=LINE ( 'NONE', #5582, #87020 ) ;
#81456=DIRECTION ( 'NONE',  ( 0.000000000000000000, 0.000000000000000000, -1.000000000000000000 ) ) ;
#81458=CARTESIAN_POINT ( 'NONE',  ( 113.7366723824214887, -44.71300795807898965, 193.1299109901969757 ) ) ;
#81459=DIRECTION ( 'NONE',  ( -4.012088370409549976E-14, 1.000000000000000000, 0.000000000000000000 ) ) ;
#81461=ORIENTED_EDGE ( 'NONE', *, *, #9230, .T. ) ;
#81462=AXIS2_PLACEMENT_3D ( 'NONE', #43425, #23022, #15752 ) ;
#81465=CARTESIAN_POINT ( 'NONE',  ( 156.5667039024485803, -48.82844715993568485, 134.7178068554149775 ) ) ;
#81467=AXIS2_PLACEMENT_3D ( 'NONE', #10228, #31552, #23437 ) ;
#81469=EDGE_LOOP ( 'NONE', ( #70897, #81146, #78109, #45818, #31222, #52802, #27269, #63065, #8865, #49856, #61806, #56216, #6134, #39351, #28020, #84466, #39991, #71873, #73014, #89630, #6271, #38092, #73355, #82241, #85957, #49428, #31124, #52095, #27061, #43113, #23014, #44869, #12043, #82964, #69806, #61558, #70685, #38180, #53028, #28077, #39368, #59654, #50576, #65205, #54880, #15797, #82723, #54153 ) ) ;
#81471=CARTESIAN_POINT ( 'NONE',  ( 97.91908366271991326, -41.73065806300744640, 221.7241967044819546 ) ) ;
#81476=CARTESIAN_POINT ( 'NONE',  ( 184.5664832912729878, -71.37844715994266664, 342.9256252759109884 ) ) ;
#81479=CARTESIAN_POINT ( 'NONE',  ( 101.9647735066782843, -29.73848997801458083, 28.38428084578198352 ) ) ;
#81480=CARTESIAN_POINT ( 'NONE',  ( 102.6068629045982021, -46.86833229348674479, 128.2346728949589760 ) ) ;
#81481=CARTESIAN_POINT ( 'NONE',  ( 33.96670390244647564, -26.71338133339342136, 193.9678068554150911 ) ) ;
#81482=ORIENTED_EDGE ( 'NONE', *, *, #62438, .F. ) ;
#81484=EDGE_CURVE ( 'NONE', #50121, #75621, #2201, .T. ) ;
#81485=CARTESIAN_POINT ( 'NONE',  ( 82.77273044669111357, -18.23917853419690971, 6.814128304791288393 ) ) ;
#81490=VERTEX_POINT ( 'NONE', #17472 ) ;
#81491=CARTESIAN_POINT ( 'NONE',  ( 75.31670390244798341, -50.82844715994100682, 60.91780685541480267 ) ) ;
#81492=EDGE_CURVE ( 'NONE', #61827, #75223, #83439, .T. ) ;
#81493=CARTESIAN_POINT ( 'NONE',  ( 99.45175552060571533, -32.86007347668476086, 50.37527697093396739 ) ) ;
#81494=CARTESIAN_POINT ( 'NONE',  ( 96.02321403599634664, -35.86825885766610611, 191.2765776568629690 ) ) ;
#81495=AXIS2_PLACEMENT_3D ( 'NONE', #63180, #84549, #49534 ) ;
#81497=CARTESIAN_POINT ( 'NONE',  ( 117.7782040715257921, -34.09831434418944696, 164.0061014663869798 ) ) ;
#81498=CARTESIAN_POINT ( 'NONE',  ( 113.5781282841511484, -44.42724326460464823, 23.13510136712798371 ) ) ;
#81499=CARTESIAN_POINT ( 'NONE',  ( 96.88896422860915436, -30.65880273170215276, 276.8984824187680829 ) ) ;
#81500=CARTESIAN_POINT ( 'NONE',  ( 188.5667039024486087, -48.82844715993430640, 134.7178068554150059 ) ) ;
#81503=EDGE_CURVE ( 'NONE', #30378, #67525, #80604, .T. ) ;
#81505=VECTOR ( 'NONE', #63171, 1000.000000000000000 ) ;
#81506=ADVANCED_FACE ( 'NONE', ( #86969 ), #3840, .T. ) ;
#81508=DIRECTION ( 'NONE',  ( 1.000000000000000000, 0.000000000000000000, 0.000000000000000000 ) ) ;
#81509=CARTESIAN_POINT ( 'NONE',  ( 114.6374585114582771, -29.49847210400304576, 234.4327681330539690 ) ) ;
#81510=VERTEX_POINT ( 'NONE', #24730 ) ;
#81511=CARTESIAN_POINT ( 'NONE',  ( 117.1924066864372520, -41.16168844948898453, 208.4861014663869696 ) ) ;
#81513=CARTESIAN_POINT ( 'NONE',  ( 99.08956014417853453, -42.79550325639331732, 22.84392096656654658 ) ) ;
#81514=DIRECTION ( 'NONE',  ( 4.299999999999999979E-14, -1.000000000000000000, 4.400000000000000367E-29 ) ) ;
#81515=CARTESIAN_POINT ( 'NONE',  ( 99.29589592323129921, -33.18472740410275179, 277.6356252759111953 ) ) ;
#81516=DIRECTION ( 'NONE',  ( -0.7071067811567173234, 0.7071067812163779331, 0.000000000000000000 ) ) ;
#81517=CARTESIAN_POINT ( 'NONE',  ( 97.81399931465544739, -40.51646775427786196, 252.6355816051047896 ) ) ;
#81519=EDGE_CURVE ( 'NONE', #48806, #51052, #31982, .T. ) ;
#81520=FACE_OUTER_BOUND ( 'NONE', #83923, .T. ) ;
#81522=CARTESIAN_POINT ( 'NONE',  ( 62.03715912545754207, -47.82818131006020934, 129.9678068554150911 ) ) ;
#81523=CYLINDRICAL_SURFACE ( 'NONE', #8601, 2.517500000000005844 ) ;
#81524=VECTOR ( 'NONE', #23140, 1000.000000000000000 ) ;
#81525=EDGE_CURVE ( 'NONE', #86596, #5327, #19102, .T. ) ;
#81527=ORIENTED_EDGE ( 'NONE', *, *, #38935, .T. ) ;
#81528=PLANE ( 'NONE',  #23448 ) ;
#81529=CARTESIAN_POINT ( 'NONE',  ( 96.16820482414080118, -32.01123326506838396, 211.0013395616249738 ) ) ;
#81530=CARTESIAN_POINT ( 'NONE',  ( 102.5581934769535906, -27.32956362888499768, 91.43276813305395478 ) ) ;
#81531=CARTESIAN_POINT ( 'NONE',  ( 115.6911734784272170, -30.73338764459478867, 275.3099109901965562 ) ) ;
#81532=CARTESIAN_POINT ( 'NONE',  ( 97.81168895331838087, -40.51742574516882200, 287.6356252759109680 ) ) ;
#81533=CARTESIAN_POINT ( 'NONE',  ( 48.16670390244654953, -26.71338133339281029, 117.4678068554150485 ) ) ;
#81534=FACE_OUTER_BOUND ( 'NONE', #85271, .T. ) ;
#81537=CIRCLE ( 'NONE', #49584, 2.116999999999980009 ) ;
#81538=CARTESIAN_POINT ( 'NONE',  ( 133.1188885517742619, -21.31186128672819535, 1.764000668899316837 ) ) ;
#81540=ORIENTED_EDGE ( 'NONE', *, *, #45663, .T. ) ;
#81541=VERTEX_POINT ( 'NONE', #37473 ) ;
#81543=CARTESIAN_POINT ( 'NONE',  ( 113.1668408875787435, -30.74627054922163438, 148.8667055423629790 ) ) ;
#81546=DIRECTION ( 'NONE',  ( -1.000000000000000000, 1.011922027653136551E-15, 0.000000000000000000 ) ) ;
#81547=CARTESIAN_POINT ( 'NONE',  ( 111.7842945758856246, -25.88553347519915349, 130.7499109901969518 ) ) ;
#81548=DIRECTION ( 'NONE',  ( 0.000000000000000000, 0.000000000000000000, -1.000000000000000000 ) ) ;
#81549=VECTOR ( 'NONE', #12350, 1000.000000000000000 ) ;
#81550=CARTESIAN_POINT ( 'NONE',  ( 74.38348329127296665, -1.929447159941392931, 352.4506252759079530 ) ) ;
#81552=CIRCLE ( 'NONE', #65573, 2.999999999999919176 ) ;
#81553=CARTESIAN_POINT ( 'NONE',  ( 162.8913605087219878, -31.76306994223740432, -5.074374724088000832 ) ) ;
#81555=CARTESIAN_POINT ( 'NONE',  ( 96.75683229781650141, -37.84742820979680289, 81.40038718067398804 ) ) ;
#81557=ORIENTED_EDGE ( 'NONE', *, *, #63878, .F. ) ;
#81559=DIRECTION ( 'NONE',  ( 0.000000000000000000, 1.000000000000000000, 0.000000000000000000 ) ) ;
#81560=( BOUNDED_CURVE ( )  B_SPLINE_CURVE ( 3, ( #71359, #79062, #43167, #44508 ),
 .UNSPECIFIED., .F., .T. ) 
 B_SPLINE_CURVE_WITH_KNOTS ( ( 4, 4 ),
 ( 1.570796326805116383, 3.141592653598081153 ),
 .UNSPECIFIED. ) 
 CURVE ( )  GEOMETRIC_REPRESENTATION_ITEM ( )  RATIONAL_B_SPLINE_CURVE ( ( 1.000000000000000000, 0.8047378541248202399, 0.8047378541248202399, 1.000000000000000000 ) ) 
 REPRESENTATION_ITEM ( '' )  );
#81561=CARTESIAN_POINT ( 'NONE',  ( 113.1634500054121872, -44.41975088505036240, 164.1099109901959707 ) ) ;
#81562=DIRECTION ( 'NONE',  ( 0.000000000000000000, 0.000000000000000000, 1.000000000000000000 ) ) ;
#81565=CARTESIAN_POINT ( 'NONE',  ( 107.0664832912739968, -36.72944715994100306, 287.6356252759109680 ) ) ;
#81568=CARTESIAN_POINT ( 'NONE',  ( 107.6020193903983824, -26.30459096080988246, 95.03562527591097364 ) ) ;
#81569=ORIENTED_EDGE ( 'NONE', *, *, #34202, .F. ) ;
#81570=ORIENTED_EDGE ( 'NONE', *, *, #31708, .T. ) ;
#81571=EDGE_CURVE ( 'NONE', #3896, #25804, #65964, .T. ) ;
#81573=FACE_OUTER_BOUND ( 'NONE', #10184, .T. ) ;
#81574=CONICAL_SURFACE ( 'NONE', #59740, 1.258750000000002922, 1.029744258676650093 ) ;
#81576=CARTESIAN_POINT ( 'NONE',  ( 112.6937225954192172, -42.64246220573352275, 155.9995189410199714 ) ) ;
#81580=VERTEX_POINT ( 'NONE', #38797 ) ;
#81582=LINE ( 'NONE', #56407, #17749 ) ;
#81583=CARTESIAN_POINT ( 'NONE',  ( 135.3687878533466176, -21.15209318184243514, 1.893168666208430162 ) ) ;
#81584=VERTEX_POINT ( 'NONE', #23853 ) ;
#81585=ORIENTED_EDGE ( 'NONE', *, *, #37643, .T. ) ;
#81586=CARTESIAN_POINT ( 'NONE',  ( 77.72936414032787411, -20.17925173418399964, 7.255518600576354338 ) ) ;
#81587=AXIS2_PLACEMENT_3D ( 'NONE', #14417, #7598, #41639 ) ;
#81588=CARTESIAN_POINT ( 'NONE',  ( 97.77711562652216060, -35.32084007268648662, 217.6263452106589682 ) ) ;
#81590=DIRECTION ( 'NONE',  ( -0.7071067811864980568, -0.7071067811865969777, 0.000000000000000000 ) ) ;
#81592=ORIENTED_EDGE ( 'NONE', *, *, #69895, .T. ) ;
#81593=ORIENTED_EDGE ( 'NONE', *, *, #71148, .F. ) ;
#81595=LINE ( 'NONE', #72195, #88482 ) ;
#81598=EDGE_CURVE ( 'NONE', #62770, #69306, #65175, .T. ) ;
#81599=ADVANCED_FACE ( 'NONE', ( #79273 ), #74668, .T. ) ;
#81600=VECTOR ( 'NONE', #20720, 1000.000000000000000 ) ;
#81601=CARTESIAN_POINT ( 'NONE',  ( 112.9694095044039841, -31.09161174735247002, 232.2509475124489597 ) ) ;
#81602=CARTESIAN_POINT ( 'NONE',  ( 109.6894323871380976, -47.49121184687970754, 87.75467289495897205 ) ) ;
#81603=EDGE_CURVE ( 'NONE', #66915, #63598, #44180, .T. ) ;
#81604=CARTESIAN_POINT ( 'NONE',  ( 112.7479404651554376, -27.97242311821432992, 69.61848241876793963 ) ) ;
#81605=CARTESIAN_POINT ( 'NONE',  ( 99.23474689667037296, -34.85485995268171422, 249.5838068554169809 ) ) ;
#81606=CARTESIAN_POINT ( 'NONE',  ( 131.5867845949885009, -17.53883969337127979, 7.103318745424658687 ) ) ;
#81607=CARTESIAN_POINT ( 'NONE',  ( 126.8164832912740110, -46.72944715994101017, 14.67562527591099020 ) ) ;
#81608=CARTESIAN_POINT ( 'NONE',  ( 117.4137378716304738, -35.45790868367866722, 189.9241967044829664 ) ) ;
#81609=CARTESIAN_POINT ( 'NONE',  ( 105.7140747251564079, -46.69282035222812510, 277.4689685590014960 ) ) ;
#81610=ORIENTED_EDGE ( 'NONE', *, *, #66454, .F. ) ;
#81612=ORIENTED_EDGE ( 'NONE', *, *, #14885, .T. ) ;
#81614=EDGE_LOOP ( 'NONE', ( #27381, #5477, #22161, #65571 ) ) ;
#81615=CARTESIAN_POINT ( 'NONE',  ( 71.24189083761808661, -0.9290567490904538817, 542.9756252759101471 ) ) ;
#81617=CARTESIAN_POINT ( 'NONE',  ( 97.78478039248422249, -40.45110315034128234, 137.6299286654718230 ) ) ;
#81619=CARTESIAN_POINT ( 'NONE',  ( 117.1066318038510303, -39.53701698219273908, 98.60991099019594230 ) ) ;
#81621=FACE_OUTER_BOUND ( 'NONE', #55616, .T. ) ;
#81622=DIRECTION ( 'NONE',  ( -1.000000000000000078E-15, 0.000000000000000000, 1.000000000000000000 ) ) ;
#81623=CARTESIAN_POINT ( 'NONE',  ( 117.0608945233090878, -38.08045312323447007, 144.7189586090517253 ) ) ;
#81624=CARTESIAN_POINT ( 'NONE',  ( 107.0664832912739968, -36.72944715994100306, 287.6356252759109680 ) ) ;
#81625=CARTESIAN_POINT ( 'NONE',  ( 113.0874441278155160, -45.97130050132138024, 219.0480062282919960 ) ) ;
#81626=LINE ( 'NONE', #33446, #75695 ) ;
#81628=EDGE_CURVE ( 'NONE', #29668, #11890, #40591, .T. ) ;
#81630=CARTESIAN_POINT ( 'NONE',  ( 131.0667039024480118, -61.87844715994100397, 210.8338068554149913 ) ) ;
#81631=AXIS2_PLACEMENT_3D ( 'NONE', #78968, #58927, #3538 ) ;
#81633=CARTESIAN_POINT ( 'NONE',  ( 97.53214211805510558, -39.74989731879190202, 136.5709469236470284 ) ) ;
#81634=CARTESIAN_POINT ( 'NONE',  ( 20.03715912545741418, -46.82818131006202123, 117.4678068554150485 ) ) ;
#81635=CARTESIAN_POINT ( 'NONE',  ( 112.4344423749254531, -46.44530527459760805, 252.9661014663871015 ) ) ;
#81636=ORIENTED_EDGE ( 'NONE', *, *, #80577, .T. ) ;
#81637=DIRECTION ( 'NONE',  ( -1.000000000000000078E-15, 1.000000000000000083E-30, 1.000000000000000000 ) ) ;
#81638=CARTESIAN_POINT ( 'NONE',  ( 111.0462345608747796, -47.04136251952688497, 13.85753003781498016 ) ) ;
#81639=CARTESIAN_POINT ( 'NONE',  ( 114.5587124134895731, -28.54364023664675187, 150.4746728949579619 ) ) ;
#81641=CARTESIAN_POINT ( 'NONE',  ( 151.5667039024486087, -48.82844715993590512, 129.9678068554149775 ) ) ;
#81642=DIRECTION ( 'NONE',  ( 0.7071067811865475727, -0.7071067811865475727, 0.000000000000000000 ) ) ;
#81643=CARTESIAN_POINT ( 'NONE',  ( 188.5667039024481255, -42.82844715993431350, 257.2178068554150059 ) ) ;
#81645=ORIENTED_EDGE ( 'NONE', *, *, #54163, .T. ) ;
#81646=AXIS2_PLACEMENT_3D ( 'NONE', #39993, #61327, #67251 ) ;
#81648=ORIENTED_EDGE ( 'NONE', *, *, #30413, .T. ) ;
#81649=EDGE_LOOP ( 'NONE', ( #81569, #69382, #10884, #29099 ) ) ;
#81651=CARTESIAN_POINT ( 'NONE',  ( 96.68076663292312389, -33.01451620012166899, 22.06514908543494258 ) ) ;
#81657=CARTESIAN_POINT ( 'NONE',  ( 103.8089036935402021, -45.87596577953674881, 251.7267055423626516 ) ) ;
#81659=ORIENTED_EDGE ( 'NONE', *, *, #24366, .T. ) ;
#81660=EDGE_LOOP ( 'NONE', ( #21309, #63028, #73454, #19970 ) ) ;
#81662=LINE ( 'NONE', #89363, #10066 ) ;
#81663=ADVANCED_FACE ( 'NONE', ( #47837 ), #5641, .T. ) ;
#81664=CARTESIAN_POINT ( 'NONE',  ( 123.6837132603319702, -55.86395651782485317, 229.5838068554170093 ) ) ;
#81665=LINE ( 'NONE', #46653, #89649 ) ;
#81666=CARTESIAN_POINT ( 'NONE',  ( 98.36824592180721538, -38.57411413555575308, 27.92444044875497156 ) ) ;
#81667=CIRCLE ( 'NONE', #29393, 5.599999999999994316 ) ;
#81670=CARTESIAN_POINT ( 'NONE',  ( 111.2075918398242038, -27.22220237496667394, 284.7375300378162706 ) ) ;
#81673=CARTESIAN_POINT ( 'NONE',  ( 164.7830935719630361, -29.99615139349950965, -5.074374724088000832 ) ) ;
#81674=LINE ( 'NONE', #82577, #32144 ) ;
#81675=CARTESIAN_POINT ( 'NONE',  ( 115.0531750927473951, -38.41541278395968817, 61.47951894101993986 ) ) ;
#81676=ADVANCED_FACE ( 'NONE', ( #67854 ), #69201, .F. ) ;
#81677=CARTESIAN_POINT ( 'NONE',  ( 136.2652213604061160, -17.07517613921647026, 7.387586420629034478 ) ) ;
#81679=CARTESIAN_POINT ( 'NONE',  ( 116.3212776292296127, -32.94146857471318413, 287.6356252759109680 ) ) ;
#81681=CARTESIAN_POINT ( 'NONE',  ( 83.06670390244796920, -61.87844715994100397, 210.8338068554149913 ) ) ;
#81683=AXIS2_PLACEMENT_3D ( 'NONE', #36630, #29811, #50683 ) ;
#81685=CARTESIAN_POINT ( 'NONE',  ( 107.9456392385311005, -25.71100025151098478, 115.0251490854349612 ) ) ;
#81687=CARTESIAN_POINT ( 'NONE',  ( 107.2022627278996652, -27.67438038655213006, 79.49908649474396327 ) ) ;
#81688=ORIENTED_CLOSED_SHELL ( 'NONE', *, #89461, .F. );
#81689=DIRECTION ( 'NONE',  ( -4.237773401492740281E-14, 1.000000000000000000, 0.000000000000000000 ) ) ;
#81690=CARTESIAN_POINT ( 'NONE',  ( 107.5226574059108202, -27.84946772507149504, 91.46729759161098627 ) ) ;
#81692=CARTESIAN_POINT ( 'NONE',  ( 107.0664832912739399, -36.72944715994095333, 302.6356252759109680 ) ) ;
#81693=CARTESIAN_POINT ( 'NONE',  ( 115.2842354651272814, -44.15600456922878436, 79.25372051400697160 ) ) ;
#81694=CARTESIAN_POINT ( 'NONE',  ( 102.0673354423506396, -27.97033358461368735, 181.4902337030571289 ) ) ;
#81695=AXIS2_PLACEMENT_3D ( 'NONE', #54228, #75158, #66544 ) ;
#81697=ORIENTED_EDGE ( 'NONE', *, *, #66795, .T. ) ;
#81698=DIRECTION ( 'NONE',  ( 0.000000000000000000, -1.000000000000000000, 0.000000000000000000 ) ) ;
#81700=ORIENTED_EDGE ( 'NONE', *, *, #86908, .F. ) ;
#81701=ADVANCED_FACE ( 'NONE', ( #33333 ), #12005, .F. ) ;
#81704=CARTESIAN_POINT ( 'NONE',  ( 109.8085987287837497, -27.34093086507531112, 259.8499109901970314 ) ) ;
#81705=CARTESIAN_POINT ( 'NONE',  ( 109.2058805625337925, -26.50397703278076733, 135.9127681330539872 ) ) ;
#81706=CARTESIAN_POINT ( 'NONE',  ( 168.0371591254543091, -48.62818131005519717, 313.9678068554149490 ) ) ;
#81707=CARTESIAN_POINT ( 'NONE',  ( 97.06107109563198776, -37.99641195030216068, 142.4272919415186323 ) ) ;
#81708=EDGE_CURVE ( 'NONE', #82549, #20374, #48274, .T. ) ;
#81709=CARTESIAN_POINT ( 'NONE',  ( 98.09687384527185827, -31.41638835794072193, 81.90133956162493689 ) ) ;
#81710=DIRECTION ( 'NONE',  ( -0.7071067812162686872, -0.7071067811568263473, -7.071067812162680651E-16 ) ) ;
#81712=DIRECTION ( 'NONE',  ( -1.000000000000000078E-15, 1.000000000000000083E-30, 1.000000000000000000 ) ) ;
#81713=EDGE_CURVE ( 'NONE', #61107, #20086, #70339, .T. ) ;
#81714=CARTESIAN_POINT ( 'NONE',  ( 101.9937552062217776, -45.44615440094798942, 158.1562831739205990 ) ) ;
#81716=CIRCLE ( 'NONE', #19325, 1.000000000000000888 ) ;
#81717=CARTESIAN_POINT ( 'NONE',  ( 162.5667039024478981, -32.29483332968042220, 117.4678068554150485 ) ) ;
#81719=CARTESIAN_POINT ( 'NONE',  ( 115.8883252675857847, -30.10835006627621269, 264.3508633711492735 ) ) ;
#81720=CARTESIAN_POINT ( 'NONE',  ( 168.3664380525675881, -48.62818131005417399, 180.4678068554150059 ) ) ;
#81721=AXIS2_PLACEMENT_3D ( 'NONE', #41450, #69181, #26499 ) ;
#81722=DIRECTION ( 'NONE',  ( 9.073094938289460781E-13, 1.000000000000000000, 0.000000000000000000 ) ) ;
#81723=FACE_OUTER_BOUND ( 'NONE', #6236, .T. ) ;
#81724=CARTESIAN_POINT ( 'NONE',  ( 116.1088647163993386, -36.23144265813309772, 273.3048007804578674 ) ) ;
#81725=LINE ( 'NONE', #53965, #21685 ) ;
#81726=CARTESIAN_POINT ( 'NONE',  ( 98.22092589535434115, -43.31882777834836418, 107.8480062282919647 ) ) ;
#81728=CARTESIAN_POINT ( 'NONE',  ( 108.6554276816787734, -25.75039326353942926, 149.9737205140059473 ) ) ;
#81730=DIRECTION ( 'NONE',  ( -1.000000000000000000, -4.510281037539694659E-14, 0.000000000000000000 ) ) ;
#81731=ADVANCED_FACE ( 'NONE', ( #34218 ), #40133, .T. ) ;
#81732=ORIENTED_EDGE ( 'NONE', *, *, #53865, .T. ) ;
#81735=ADVANCED_FACE ( 'NONE', ( #68306 ), #81062, .T. ) ;
#81736=CARTESIAN_POINT ( 'NONE',  ( 51.06648329127400388, 0.2215528400590083269, 336.6506252759110112 ) ) ;
#81737=EDGE_LOOP ( 'NONE', ( #47637, #73514, #88911, #67852 ) ) ;
#81738=CARTESIAN_POINT ( 'NONE',  ( 141.0235900724605358, -46.62589376934771224, 14.92562527591103105 ) ) ;
#81739=CARTESIAN_POINT ( 'NONE',  ( 103.1581569894456294, -27.01699888143334860, 130.3813395616259925 ) ) ;
#81740=EDGE_LOOP ( 'NONE', ( #85792, #10889, #69294, #9025 ) ) ;
#81744=FACE_OUTER_BOUND ( 'NONE', #84504, .T. ) ;
#81746=ORIENTED_EDGE ( 'NONE', *, *, #63750, .F. ) ;
#81748=AXIS2_PLACEMENT_3D ( 'NONE', #37731, #16835, #65426 ) ;
#81749=PLANE ( 'NONE',  #33956 ) ;
#81750=ORIENTED_EDGE ( 'NONE', *, *, #69003, .F. ) ;
#81752=CYLINDRICAL_SURFACE ( 'NONE', #61202, 0.2500000000000002220 ) ;
#81754=CARTESIAN_POINT ( 'NONE',  ( 100.8874677930869552, -44.70022130517887149, 157.0522919335028007 ) ) ;
#81758=CARTESIAN_POINT ( 'NONE',  ( 181.9694315774057713, -34.03355364505798519, 313.9678068554149490 ) ) ;
#81761=CARTESIAN_POINT ( 'NONE',  ( 177.0664832912740110, 12.92155284005802685, 334.6228282640715292 ) ) ;
#81762=EDGE_CURVE ( 'NONE', #9949, #58653, #73311, .T. ) ;
#81763=CARTESIAN_POINT ( 'NONE',  ( 101.7545977962314652, -44.98157700518526525, 218.1213395616249784 ) ) ;
#81764=CARTESIAN_POINT ( 'NONE',  ( 162.7131505118679797, -31.94127993907790852, -5.074374724088000832 ) ) ;
#81765=EDGE_LOOP ( 'NONE', ( #47901, #23549, #77669, #68490 ) ) ;
#81766=CARTESIAN_POINT ( 'NONE',  ( 116.4719273984280790, -32.36179259691363796, 55.16038718067301261 ) ) ;
#81767=CARTESIAN_POINT ( 'NONE',  ( 116.5686728426965857, -33.54608030872165614, 54.08363974141789754 ) ) ;
#81768=CARTESIAN_POINT ( 'NONE',  ( 88.24325903289653183, -55.55267141831875222, -5.074374724089048883 ) ) ;
#81769=CARTESIAN_POINT ( 'NONE',  ( 97.80396990294123327, -40.49851493234764632, 22.63399986120327867 ) ) ;
#81770=ORIENTED_EDGE ( 'NONE', *, *, #30409, .F. ) ;
#81771=CARTESIAN_POINT ( 'NONE',  ( 41.56648329127499153, -32.07844715994070839, 138.9256252759119832 ) ) ;
#81773=ORIENTED_EDGE ( 'NONE', *, *, #5088, .F. ) ;
#81774=CARTESIAN_POINT ( 'NONE',  ( 104.6178464025351218, -28.18156397322882967, 221.7301547344689823 ) ) ;
#81776=LINE ( 'NONE', #39968, #9565 ) ;
#81777=ADVANCED_FACE ( 'NONE', ( #69650, #27855 ), #83733, .T. ) ;
#81779=AXIS2_PLACEMENT_3D ( 'NONE', #30430, #10864, #24945 ) ;
#81780=CARTESIAN_POINT ( 'NONE',  ( 107.0664832912739399, -36.72944715994095333, 311.6356252759109680 ) ) ;
#81781=CARTESIAN_POINT ( 'NONE',  ( 156.5667039024483529, -42.82844715993568485, 137.2178068554149775 ) ) ;
#81782=ORIENTED_EDGE ( 'NONE', *, *, #71557, .T. ) ;
#81785=VERTEX_POINT ( 'NONE', #42364 ) ;
#81786=CARTESIAN_POINT ( 'NONE',  ( 101.0991643652557173, -45.25116564454923207, 282.0899109901967563 ) ) ;
#81787=EDGE_LOOP ( 'NONE', ( #5654, #13294, #34102 ) ) ;
#81788=CARTESIAN_POINT ( 'NONE',  ( 111.3125147634731462, -44.27080922411229835, 255.8147570362582712 ) ) ;
#81789=EDGE_CURVE ( 'NONE', #60401, #7119, #61629, .T. ) ;
#81790=FACE_BOUND ( 'NONE', #45227, .T. ) ;
#81791=CARTESIAN_POINT ( 'NONE',  ( 97.25364341294451265, -36.87759583893578252, 136.3384824187689333 ) ) ;
#81796=CARTESIAN_POINT ( 'NONE',  ( 117.3777842326014706, -34.92111847156615312, 239.9641967044819637 ) ) ;
#81798=ORIENTED_EDGE ( 'NONE', *, *, #31355, .F. ) ;
#81799=AXIS2_PLACEMENT_3D ( 'NONE', #9060, #49914, #36759 ) ;
#81800=CARTESIAN_POINT ( 'NONE',  ( 96.74875621672018156, -38.50074266403909462, 87.46133956162493917 ) ) ;
#81801=CARTESIAN_POINT ( 'NONE',  ( 63.03715912545729338, -24.42818131006027826, 313.9678068554150059 ) ) ;
#81802=VECTOR ( 'NONE', #62526, 1000.000000000000000 ) ;
#81804=ORIENTED_EDGE ( 'NONE', *, *, #63054, .T. ) ;
#81805=ORIENTED_EDGE ( 'NONE', *, *, #21789, .F. ) ;
#81806=ORIENTED_EDGE ( 'NONE', *, *, #48565, .F. ) ;
#81807=AXIS2_PLACEMENT_3D ( 'NONE', #23468, #85256, #51137 ) ;
#81808=CARTESIAN_POINT ( 'NONE',  ( 188.5667039024479834, -58.35344715994099829, 293.2178068554150627 ) ) ;
#81810=CYLINDRICAL_SURFACE ( 'NONE', #21922, 9.999999999999998224 ) ;
#81813=CARTESIAN_POINT ( 'NONE',  ( 111.0233670443594463, -45.12224181339347240, 135.7452332267339443 ) ) ;
#81814=CARTESIAN_POINT ( 'NONE',  ( 97.20328444759655895, -40.27860260594448505, 262.6013395616254797 ) ) ;
#81815=DIRECTION ( 'NONE',  ( 1.000000000000000000, 4.299999999999999979E-14, 1.000000000000000078E-15 ) ) ;
#81819=VERTEX_POINT ( 'NONE', #57346 ) ;
#81820=CARTESIAN_POINT ( 'NONE',  ( 30.48091746481741637, -48.32844715994156815, 180.4678068554150911 ) ) ;
#81821=ORIENTED_EDGE ( 'NONE', *, *, #74580, .F. ) ;
#81822=EDGE_LOOP ( 'NONE', ( #74201, #46856 ) ) ;
#81823=DIRECTION ( 'NONE',  ( -0.7071067812162665778, -0.7071067811568285677, -6.612322856132800227E-17 ) ) ;
#81825=B_SPLINE_CURVE_WITH_KNOTS ( 'NONE', 3,
 ( #10318, #38023, #52066, #79826, #40243, #60232, #87964, #76448, #67961, #67064, #39787, #73878, #4844, #74334, #32526, #41908, #12105, #7410 ),
 .UNSPECIFIED., .F., .F.,
 ( 4, 2, 2, 2, 2, 2, 2, 2, 4 ),
 ( 0.4999740858641279484, 0.5624773251311119271, 0.6249805643980959058, 0.6874838036650799955, 0.7499870429320639742, 0.8124902821990479529, 0.8749935214660320426, 0.9374967607330160213, 1.000000000000000000 ),
 .UNSPECIFIED. ) ;
#81826=PLANE ( 'NONE',  #42303 ) ;
#81828=CARTESIAN_POINT ( 'NONE',  ( 111.5068547175069824, -28.09499701576110198, 169.1209912566479545 ) ) ;
#81829=CARTESIAN_POINT ( 'NONE',  ( 98.68712911129445331, -43.00583860492766064, 66.83848241876793850 ) ) ;
#81830=ORIENTED_EDGE ( 'NONE', *, *, #22016, .F. ) ;
#81831=CARTESIAN_POINT ( 'NONE',  ( 162.8913605087224710, -31.76306994223275382, 193.9678068554149775 ) ) ;
#81832=ADVANCED_FACE ( 'NONE', ( #28764 ), #85087, .F. ) ;
#81835=CARTESIAN_POINT ( 'NONE',  ( 48.79742451361987321, -36.32844715994078655, 193.9678068554150911 ) ) ;
#81837=EDGE_CURVE ( 'NONE', #50690, #62285, #50534, .T. ) ;
#81839=ORIENTED_EDGE ( 'NONE', *, *, #3231, .T. ) ;
#81841=EDGE_CURVE ( 'NONE', #52939, #82504, #41327, .T. ) ;
#81843=CARTESIAN_POINT ( 'NONE',  ( 101.9931123694998973, -45.44575822371417928, 132.1564871734879318 ) ) ;
#81845=DIRECTION ( 'NONE',  ( -1.000000000000000000, 6.036837696399451257E-13, 0.000000000000000000 ) ) ;
#81846=ORIENTED_EDGE ( 'NONE', *, *, #53322, .F. ) ;
#81847=CARTESIAN_POINT ( 'NONE',  ( 114.1055592783800137, -46.29424852498188869, 33.08133956162495792 ) ) ;
#81848=CARTESIAN_POINT ( 'NONE',  ( 117.9699911065184637, -41.49648292930365301, 54.49848241876792088 ) ) ;
#81849=VECTOR ( 'NONE', #12331, 1000.000000000000000 ) ;
#81850=CARTESIAN_POINT ( 'NONE',  ( 182.2738106836200132, -23.19206098993950604, -5.074374724088000832 ) ) ;
#81853=CARTESIAN_POINT ( 'NONE',  ( 71.24189083761808661, -0.9290567490904538817, 396.9756252759102040 ) ) ;
#81855=FACE_OUTER_BOUND ( 'NONE', #45658, .T. ) ;
#81856=CYLINDRICAL_SURFACE ( 'NONE', #77520, 9.999999999999998224 ) ;
#81857=ORIENTED_EDGE ( 'NONE', *, *, #49043, .T. ) ;
#81858=CARTESIAN_POINT ( 'NONE',  ( 103.4619715496438630, -25.38765309446003116, 55.32133956162594046 ) ) ;
#81859=CARTESIAN_POINT ( 'NONE',  ( 104.2081133107797228, -25.20330419090194951, 86.26991099019699050 ) ) ;
#81860=CARTESIAN_POINT ( 'NONE',  ( 97.83900064082345693, -40.58357432020694233, 171.6415561560118590 ) ) ;
#81861=LINE ( 'NONE', #19614, #25305 ) ;
#81863=AXIS2_PLACEMENT_3D ( 'NONE', #32836, #60530, #68712 ) ;
#81864=AXIS2_PLACEMENT_3D ( 'NONE', #52856, #80626, #37940 ) ;
#81865=CIRCLE ( 'NONE', #68753, 11.57110091390449469 ) ;
#81867=B_SPLINE_CURVE_WITH_KNOTS ( 'NONE', 3,
 ( #12641, #25356, #19002, #38988, #32171, #53937, #46686, #74417, #40776, #19897, #73513, #53029, #45785, #19446, #80797, #74865, #26260, #87599 ),
 .UNSPECIFIED., .F., .F.,
 ( 4, 2, 2, 2, 2, 2, 2, 2, 4 ),
 ( 0.4999998914591470833, 0.5624999050267537326, 0.6249999185943603264, 0.6874999321619669201, 0.7499999457295736249, 0.8124999592971802187, 0.8749999728647868125, 0.9374999864323934062, 1.000000000000000000 ),
 .UNSPECIFIED. ) ;
#81868=CARTESIAN_POINT ( 'NONE',  ( 179.8585841295805210, -30.08671355699668837, 313.9678068554149490 ) ) ;
#81869=ORIENTED_EDGE ( 'NONE', *, *, #74185, .F. ) ;
#81870=CARTESIAN_POINT ( 'NONE',  ( 98.87588542518402335, -42.07524381596787322, 97.78705384733893879 ) ) ;
#81872=ORIENTED_EDGE ( 'NONE', *, *, #89490, .T. ) ;
#81874=CARTESIAN_POINT ( 'NONE',  ( 97.93839266929580845, -41.72010113774604889, 217.7241967044829494 ) ) ;
#81875=CARTESIAN_POINT ( 'NONE',  ( 121.3042370176062548, -43.34581843340460239, 9.125625275910984158 ) ) ;
#81878=CARTESIAN_POINT ( 'NONE',  ( 98.34985892484459669, -31.65658478873675108, 81.90645860733756933 ) ) ;
#81879=CARTESIAN_POINT ( 'NONE',  ( 167.7413838386817702, -48.33240602328261559, 249.9678068554149775 ) ) ;
#81880=DIRECTION ( 'NONE',  ( 0.000000000000000000, 0.000000000000000000, -1.000000000000000000 ) ) ;
#81881=CARTESIAN_POINT ( 'NONE',  ( 112.1511370651177231, -26.84216853020813076, 169.6984824187689469 ) ) ;
#81882=VERTEX_POINT ( 'NONE', #70092 ) ;
#81884=CARTESIAN_POINT ( 'NONE',  ( 111.0851542815211985, -27.49251106464650007, 131.1815833058969645 ) ) ;
#81885=DIRECTION ( 'NONE',  ( -0.7071067811865253683, 0.7071067811865696662, -7.071067811865261355E-16 ) ) ;
#81886=EDGE_CURVE ( 'NONE', #76826, #67926, #7864, .T. ) ;
#81887=CARTESIAN_POINT ( 'NONE',  ( 111.3277751695582651, -45.53312973143654574, 243.9356252759109509 ) ) ;
#81888=DIRECTION ( 'NONE',  ( 1.000000000000000000, 2.106816776397999944E-14, 9.351236661543306751E-17 ) ) ;
#81889=CARTESIAN_POINT ( 'NONE',  ( 182.3467384525660862, -36.02818131005237490, 117.4678068554150627 ) ) ;
#81890=ADVANCED_FACE ( 'NONE', ( #35562 ), #54407, .T. ) ;
#81892=ADVANCED_FACE ( 'NONE', ( #36917 ), #55903, .T. ) ;
#81893=CARTESIAN_POINT ( 'NONE',  ( 46.03715912545342093, -48.62818131006090283, 193.9678068554150911 ) ) ;
#81896=CARTESIAN_POINT ( 'NONE',  ( 107.6532706963292725, -47.74396045468181882, 197.6308633711489620 ) ) ;
#81898=ORIENTED_EDGE ( 'NONE', *, *, #9128, .F. ) ;
#81899=VERTEX_POINT ( 'NONE', #21965 ) ;
#81904=DIRECTION ( 'NONE',  ( 1.000000000000000000, 0.000000000000000000, 0.000000000000000000 ) ) ;
#81906=ADVANCED_FACE ( 'NONE', ( #63733 ), #15305, .F. ) ;
#81908=LINE ( 'NONE', #19658, #77516 ) ;
#81909=ORIENTED_EDGE ( 'NONE', *, *, #58705, .F. ) ;
#81912=ADVANCED_FACE ( 'NONE', ( #84640 ), #82203, .F. ) ;
#81913=CARTESIAN_POINT ( 'NONE',  ( 99.75298236265237506, -29.29979477046331127, 225.6956252759109702 ) ) ;
#81914=ORIENTED_EDGE ( 'NONE', *, *, #28481, .T. ) ;
#81916=EDGE_CURVE ( 'NONE', #62559, #82107, #6591, .T. ) ;
#81917=DIRECTION ( 'NONE',  ( 0.000000000000000000, 0.000000000000000000, -1.000000000000000000 ) ) ;
#81919=EDGE_CURVE ( 'NONE', #26048, #11858, #57350, .T. ) ;
#81920=CARTESIAN_POINT ( 'NONE',  ( 115.1453852183930593, -37.89609606526670404, 26.53094751244894312 ) ) ;
#81921=CARTESIAN_POINT ( 'NONE',  ( 102.0714078572591319, -27.55412165564507632, 141.4727681330539895 ) ) ;
#81922=CARTESIAN_POINT ( 'NONE',  ( 50.87649884952384127, -33.54226604284969682, 117.4678068554150485 ) ) ;
#81923=VERTEX_POINT ( 'NONE', #21640 ) ;
#81925=CARTESIAN_POINT ( 'NONE',  ( 99.02771868422573220, -42.71062859073643381, 66.83645039813700350 ) ) ;
#81927=ORIENTED_EDGE ( 'NONE', *, *, #45753, .T. ) ;
#81930=AXIS2_PLACEMENT_3D ( 'NONE', #43972, #70812, #1773 ) ;
#81931=ORIENTED_EDGE ( 'NONE', *, *, #21279, .T. ) ;
#81932=EDGE_LOOP ( 'NONE', ( #49915, #16723, #4183, #12042 ) ) ;
#81933=FACE_BOUND ( 'NONE', #46788, .T. ) ;
#81934=AXIS2_PLACEMENT_3D ( 'NONE', #42926, #70663, #7535 ) ;
#81935=CARTESIAN_POINT ( 'NONE',  ( 114.7034172354883168, -32.83980166744527196, 43.62384839950495063 ) ) ;
#81937=CARTESIAN_POINT ( 'NONE',  ( 112.4231589263966526, -46.42488254349225940, 252.9661014663871015 ) ) ;
#81938=EDGE_CURVE ( 'NONE', #42224, #69089, #9468, .T. ) ;
#81940=CARTESIAN_POINT ( 'NONE',  ( 116.9962961068553966, -33.62662860631126449, 174.0670538473389399 ) ) ;
#81941=CARTESIAN_POINT ( 'NONE',  ( 98.42165055296780451, -41.76806737957761584, 21.74622857282093591 ) ) ;
#81942=CARTESIAN_POINT ( 'NONE',  ( 112.1867106929447573, -26.95862322015898016, 10.68038718067299087 ) ) ;
#81945=DIRECTION ( 'NONE',  ( 0.7071067811571405404, 0.7071067812159546051, 0.000000000000000000 ) ) ;
#81946=ADVANCED_FACE ( 'NONE', ( #33793 ), #47401, .T. ) ;
#81947=ORIENTED_EDGE ( 'NONE', *, *, #86959, .F. ) ;
#81948=ADVANCED_FACE ( 'NONE', ( #66970 ), #32434, .F. ) ;
#81949=FACE_OUTER_BOUND ( 'NONE', #22168, .T. ) ;
#81950=CARTESIAN_POINT ( 'NONE',  ( 116.5766284862631466, -42.45395780223795157, 278.3832443235297660 ) ) ;
#81952=CARTESIAN_POINT ( 'NONE',  ( 117.9328099866778246, -34.70409988052399086, 203.9851490854349549 ) ) ;
#81953=CARTESIAN_POINT ( 'NONE',  ( 112.1393456185932251, -28.01282276695584983, 34.65645861137475947 ) ) ;
#81956=FACE_BOUND ( 'NONE', #76736, .T. ) ;
#81958=CARTESIAN_POINT ( 'NONE',  ( 115.1744752910655620, -38.35034237767378329, 277.6356252759110248 ) ) ;
#81959=CARTESIAN_POINT ( 'NONE',  ( 179.4595971212905852, -28.98061976758350511, 313.9678068554149490 ) ) ;
#81960=DIRECTION ( 'NONE',  ( 0.000000000000000000, 0.000000000000000000, 1.000000000000000000 ) ) ;
#81964=CARTESIAN_POINT ( 'NONE',  ( 97.31602727650306406, -39.30641804829839714, 41.53089032425290839 ) ) ;
#81967=VERTEX_POINT ( 'NONE', #31996 ) ;
#81969=CARTESIAN_POINT ( 'NONE',  ( 106.3003094972131208, -47.14862859053906874, 222.5184824187679453 ) ) ;
#81970=CARTESIAN_POINT ( 'NONE',  ( 96.64197643737422538, -36.61924597882073584, 107.3184824187679567 ) ) ;
#81971=CARTESIAN_POINT ( 'NONE',  ( 115.9970180223098311, -30.13831313182449989, 255.3203871806730660 ) ) ;
#81973=FACE_OUTER_BOUND ( 'NONE', #47769, .T. ) ;
#81975=CARTESIAN_POINT ( 'NONE',  ( 89.17003477451885374, -56.47944715994104570, -5.074374724089047106 ) ) ;
#81977=AXIS2_PLACEMENT_3D ( 'NONE', #43583, #58120, #52162 ) ;
#81978=CARTESIAN_POINT ( 'NONE',  ( 131.6146038194058292, -19.97617057400509566, 2.716753174561010287 ) ) ;
#81979=AXIS2_PLACEMENT_3D ( 'NONE', #77937, #15260, #71128 ) ;
#81980=ORIENTED_EDGE ( 'NONE', *, *, #43746, .T. ) ;
#81981=EDGE_LOOP ( 'NONE', ( #49112, #10204, #74044, #44947 ) ) ;
#81982=CARTESIAN_POINT ( 'NONE',  ( 108.0589421777836492, -45.73103505524393597, 157.0743245899819556 ) ) ;
#81984=ORIENTED_EDGE ( 'NONE', *, *, #7488, .T. ) ;
#81985=DIRECTION ( 'NONE',  ( -0.7071067811865779928, 0.7071067811865171526, -7.071067811865785947E-16 ) ) ;
#81986=CARTESIAN_POINT ( 'NONE',  ( 98.47430666977648173, -42.65725675464086919, 122.8070538473389490 ) ) ;
#81987=CARTESIAN_POINT ( 'NONE',  ( 168.3664380525669912, -48.62818131005517586, 180.4678068554150059 ) ) ;
#81990=DIRECTION ( 'NONE',  ( 0.000000000000000000, -1.000000000000000000, 0.000000000000000000 ) ) ;
#81991=CARTESIAN_POINT ( 'NONE',  ( 97.00151786184777336, -41.45262973156714992, 61.67562527591097421 ) ) ;
#81995=AXIS2_PLACEMENT_3D ( 'NONE', #79648, #29255, #56939 ) ;
#81997=CARTESIAN_POINT ( 'NONE',  ( 97.81168895331838087, -40.51742574516882200, 287.6356252759109680 ) ) ;
#81998=AXIS2_PLACEMENT_3D ( 'NONE', #19412, #61186, #46649 ) ;
#81999=CARTESIAN_POINT ( 'NONE',  ( 108.7386892141029335, -46.36620816325528693, 163.7127681330539701 ) ) ;
#82000=LINE ( 'NONE', #40640, #34577 ) ;
#82001=CIRCLE ( 'NONE', #42791, 10.00000000000000355 ) ;
#82005=EDGE_CURVE ( 'NONE', #64140, #41877, #46052, .T. ) ;
#82006=DIRECTION ( 'NONE',  ( -1.000000000000000000, 0.000000000000000000, 0.000000000000000000 ) ) ;
#82009=CARTESIAN_POINT ( 'NONE',  ( 115.0369792144555134, -42.90881563258641052, 179.3022564342772114 ) ) ;
#82010=CARTESIAN_POINT ( 'NONE',  ( 117.8338636819851644, -39.12263375953642708, 103.6403871806729455 ) ) ;
#82012=EDGE_LOOP ( 'NONE', ( #81482, #59096, #82030, #4011 ) ) ;
#82013=EDGE_LOOP ( 'NONE', ( #14317, #23897, #32315, #15370 ) ) ;
#82018=DIRECTION ( 'NONE',  ( 0.000000000000000000, -1.000000000000000000, 0.000000000000000000 ) ) ;
#82019=VECTOR ( 'NONE', #8242, 1000.000000000000000 ) ;
#82020=CARTESIAN_POINT ( 'NONE',  ( 115.5744916924636954, -35.14366089088881751, 201.8033284648299457 ) ) ;
#82021=EDGE_CURVE ( 'NONE', #70182, #73152, #55842, .T. ) ;
#82023=EDGE_CURVE ( 'NONE', #1995, #41277, #776, .T. ) ;
#82024=CARTESIAN_POINT ( 'NONE',  ( 115.8261224330695569, -31.73121246411632512, 25.23977400646692715 ) ) ;
#82025=ORIENTED_EDGE ( 'NONE', *, *, #19232, .T. ) ;
#82026=ORIENTED_EDGE ( 'NONE', *, *, #48526, .F. ) ;
#82028=DIRECTION ( 'NONE',  ( 0.000000000000000000, 0.000000000000000000, -1.000000000000000000 ) ) ;
#82030=ORIENTED_EDGE ( 'NONE', *, *, #77754, .T. ) ;
#82032=CARTESIAN_POINT ( 'NONE',  ( 77.65458752641551143, -20.05177997656060995, 7.178113714840788973 ) ) ;
#82033=EDGE_CURVE ( 'NONE', #23851, #78707, #27870, .T. ) ;
#82034=CARTESIAN_POINT ( 'NONE',  ( 116.1701677112242237, -32.41741342456931818, 210.6101547344689777 ) ) ;
#82036=EDGE_CURVE ( 'NONE', #48953, #78000, #20176, .T. ) ;
#82037=VECTOR ( 'NONE', #50174, 1000.000000000000000 ) ;
#82041=DIRECTION ( 'NONE',  ( 0.000000000000000000, 1.000000000000000000, 0.000000000000000000 ) ) ;
#82042=CIRCLE ( 'NONE', #15317, 2.749999999999974687 ) ;
#82043=EDGE_LOOP ( 'NONE', ( #35433, #23237, #63069, #57825 ) ) ;
#82044=VERTEX_POINT ( 'NONE', #14256 ) ;
#82045=CARTESIAN_POINT ( 'NONE',  ( 115.6911714722407396, -33.30735935496929301, 246.9452332267339614 ) ) ;
#82046=CARTESIAN_POINT ( 'NONE',  ( 114.5280328947845732, -29.41122550446140949, 149.4441967044819819 ) ) ;
#82047=CARTESIAN_POINT ( 'NONE',  ( 106.9276426037745011, -26.29176787048580266, 60.08705384733897858 ) ) ;
#82048=CARTESIAN_POINT ( 'NONE',  ( 99.79500342874349883, -40.09713400422746332, 249.5838068554171514 ) ) ;
#82050=CARTESIAN_POINT ( 'NONE',  ( 107.8711561831457857, -25.29845801491854473, 321.2571935114572739 ) ) ;
#82051=CARTESIAN_POINT ( 'NONE',  ( 117.4872506282070503, -40.41476785070875621, 174.5680062282919778 ) ) ;
#82052=DIRECTION ( 'NONE',  ( 1.000000000000000000, 4.299999999999999979E-14, 1.000000000000000078E-15 ) ) ;
#82054=DIRECTION ( 'NONE',  ( 0.000000000000000000, 1.000000000000000000, 1.914177628664063178E-15 ) ) ;
#82056=EDGE_LOOP ( 'NONE', ( #22334, #1846, #16721, #43640, #12777, #63145, #10949, #11081, #88138, #18012, #44971, #34164, #80417, #81267, #25237, #80383, #15659, #78057, #80533, #1874, #21797, #48651, #69991, #83360, #17297, #55063, #4441, #61182, #39519, #43006, #79590, #30513, #82253, #59067, #84007, #44853, #81187, #80842, #68796, #39529, #46928, #75076, #72715, #15970, #65266, #45222, #88191, #69882 ) ) ;
#82058=EDGE_CURVE ( 'NONE', #3590, #52727, #36033, .T. ) ;
#82059=ORIENTED_EDGE ( 'NONE', *, *, #42745, .T. ) ;
#82060=CIRCLE ( 'NONE', #73345, 3.250000000000002665 ) ;
#82061=CARTESIAN_POINT ( 'NONE',  ( 97.80395965993845664, -40.49850016457129698, 137.6339984679455313 ) ) ;
#82064=CARTESIAN_POINT ( 'NONE',  ( 105.7968630617233288, -26.72439637550503377, 91.17750313677824181 ) ) ;
#82065=CARTESIAN_POINT ( 'NONE',  ( 116.5985118214053813, -29.68807528100325044, 109.3327681330539605 ) ) ;
#82066=CARTESIAN_POINT ( 'NONE',  ( 104.4929461018149937, -26.97798581942615215, 255.2813983111578011 ) ) ;
#82067=CIRCLE ( 'NONE', #61726, 0.5000000000000004441 ) ;
#82068=CARTESIAN_POINT ( 'NONE',  ( 136.7302760451810286, -36.02416100034015756, 6.874390491355895527 ) ) ;
#82070=CARTESIAN_POINT ( 'NONE',  ( 116.7951252707073024, -39.38782979302678910, 144.6147919423369785 ) ) ;
#82072=CARTESIAN_POINT ( 'NONE',  ( 117.9098725419244005, -34.70837513311213485, 199.9851490854349549 ) ) ;
#82073=LINE ( 'NONE', #20282, #82907 ) ;
#82075=ORIENTED_EDGE ( 'NONE', *, *, #1302, .F. ) ;
#82076=DIRECTION ( 'NONE',  ( 0.000000000000000000, 0.000000000000000000, 1.000000000000000000 ) ) ;
#82077=CIRCLE ( 'NONE', #81864, 5.599999999999994316 ) ;
#82078=CARTESIAN_POINT ( 'NONE',  ( 75.31670390244798341, -57.40094715994099772, 33.40080685541480676 ) ) ;
#82079=CARTESIAN_POINT ( 'NONE',  ( 125.9611475301391721, -14.72944715994100484, 239.5838068554164977 ) ) ;
#82080=CIRCLE ( 'NONE', #41250, 0.5000000000000004441 ) ;
#82082=ADVANCED_FACE ( 'NONE', ( #89669 ), #41930, .F. ) ;
#82083=CARTESIAN_POINT ( 'NONE',  ( 115.9975756407361018, -30.13790158448777845, 259.3203871806730945 ) ) ;
#82084=ORIENTED_EDGE ( 'NONE', *, *, #51222, .F. ) ;
#82085=CYLINDRICAL_SURFACE ( 'NONE', #74181, 16.00000000000090239 ) ;
#82086=CARTESIAN_POINT ( 'NONE',  ( 104.5830001944168259, -26.58193179050359589, 281.2670538473395823 ) ) ;
#82087=CARTESIAN_POINT ( 'NONE',  ( 97.63545021146504155, -41.27351965004424983, 167.6841967044829573 ) ) ;
#82089=CARTESIAN_POINT ( 'NONE',  ( 109.7248315322984524, -27.00080197363539725, 100.8648701262310823 ) ) ;
#82090=VECTOR ( 'NONE', #29476, 1000.000000000000000 ) ;
#82093=DIRECTION ( 'NONE',  ( 1.000000000000000000, 0.000000000000000000, 0.000000000000000000 ) ) ;
#82098=ORIENTED_EDGE ( 'NONE', *, *, #26914, .F. ) ;
#82099=ORIENTED_EDGE ( 'NONE', *, *, #87436, .T. ) ;
#82102=CARTESIAN_POINT ( 'NONE',  ( 95.28387218206130171, -35.72034718286344912, 32.25848241876794020 ) ) ;
#82104=DIRECTION ( 'NONE',  ( -0.0001713722456129692653, 0.9999999853157764962, 0.000000000000000000 ) ) ;
#82105=CARTESIAN_POINT ( 'NONE',  ( 131.3164832912740110, -36.72944715994100306, -5.074374724089004474 ) ) ;
#82106=CARTESIAN_POINT ( 'NONE',  ( 99.20650695390740736, -40.14600596985821568, 231.0752769709339418 ) ) ;
#82107=VERTEX_POINT ( 'NONE', #27420 ) ;
#82108=EDGE_LOOP ( 'NONE', ( #32131, #86366, #27621, #24350 ) ) ;
#82112=CARTESIAN_POINT ( 'NONE',  ( 99.50492789300037089, -43.30601609924293172, 101.8962887008209464 ) ) ;
#82113=DIRECTION ( 'NONE',  ( 1.387778780781444492E-15, 0.000000000000000000, -1.000000000000000000 ) ) ;
#82114=CARTESIAN_POINT ( 'NONE',  ( 102.0649443859605299, -27.97173592226543093, 275.4895552553568905 ) ) ;
#82115=EDGE_CURVE ( 'NONE', #7119, #8522, #1528, .T. ) ;
#82118=EDGE_CURVE ( 'NONE', #9110, #73852, #60264, .T. ) ;
#82119=CARTESIAN_POINT ( 'NONE',  ( 109.7226150969135716, -27.00020866801084196, 174.8649754870583308 ) ) ;
#82120=CARTESIAN_POINT ( 'NONE',  ( 106.1957191385480570, -47.06291487533376028, 262.4975300378164320 ) ) ;
#82122=ORIENTED_EDGE ( 'NONE', *, *, #36293, .T. ) ;
#82124=DIRECTION ( 'NONE',  ( 1.000000000000000000, 4.272717921125132861E-14, 0.000000000000000000 ) ) ;
#82126=CARTESIAN_POINT ( 'NONE',  ( 98.90209562501077301, -37.38172185807169967, 99.20809036959194316 ) ) ;
#82128=EDGE_CURVE ( 'NONE', #11434, #14889, #16720, .T. ) ;
#82131=FACE_OUTER_BOUND ( 'NONE', #45784, .T. ) ;
#82132=AXIS2_PLACEMENT_3D ( 'NONE', #88262, #27354, #26022 ) ;
#82133=CARTESIAN_POINT ( 'NONE',  ( 97.81170508561586985, -40.51744524251693491, 57.63550115181184452 ) ) ;
#82135=DIRECTION ( 'NONE',  ( 1.000000000000000078E-15, -1.000000000000000083E-30, -1.000000000000000000 ) ) ;
#82137=CYLINDRICAL_SURFACE ( 'NONE', #65817, 3.000000000000002665 ) ;
#82138=ORIENTED_EDGE ( 'NONE', *, *, #89002, .F. ) ;
#82139=CARTESIAN_POINT ( 'NONE',  ( 116.8067323440835565, -43.47985705614018315, 163.3441967044829823 ) ) ;
#82140=ORIENTED_EDGE ( 'NONE', *, *, #69912, .T. ) ;
#82142=CARTESIAN_POINT ( 'NONE',  ( 108.1315353547809224, -45.52682987947058280, 114.1044404487549571 ) ) ;
#82143=DIRECTION ( 'NONE',  ( 4.299999999999999979E-14, -1.000000000000000000, 4.400000000000000367E-29 ) ) ;
#82146=CARTESIAN_POINT ( 'NONE',  ( 112.7717388973142647, -27.93574178168534061, 65.61848241876793963 ) ) ;
#82148=DIRECTION ( 'NONE',  ( 1.000000000000000000, 4.299999999999999979E-14, 1.000000000000000078E-15 ) ) ;
#82149=VERTEX_POINT ( 'NONE', #63291 ) ;
#82153=VERTEX_POINT ( 'NONE', #84207 ) ;
#82156=CARTESIAN_POINT ( 'NONE',  ( 115.2378349030890945, -31.35427756934436871, 254.2899109901970292 ) ) ;
#82157=CARTESIAN_POINT ( 'NONE',  ( 113.3444227873369243, -45.07958072982976461, 139.0899109901969553 ) ) ;
#82159=CARTESIAN_POINT ( 'NONE',  ( 163.0664832912739826, 22.62155284005901024, 339.0006252759110339 ) ) ;
#82160=CARTESIAN_POINT ( 'NONE',  ( 96.07767081433036083, -37.92107664550148627, 77.40038718067299328 ) ) ;
#82161=CARTESIAN_POINT ( 'NONE',  ( 36.23715912545424089, -47.82818131006125384, 300.4678068554150059 ) ) ;
#82162=ORIENTED_EDGE ( 'NONE', *, *, #79879, .T. ) ;
#82163=CARTESIAN_POINT ( 'NONE',  ( 37.03715912545433753, -48.62818131006121547, 237.4678068554150059 ) ) ;
#82165=EDGE_CURVE ( 'NONE', #86561, #55881, #28779, .T. ) ;
#82169=CARTESIAN_POINT ( 'NONE',  ( 97.23737678141878860, -33.32131919061083636, 286.0613395616252888 ) ) ;
#82170=CARTESIAN_POINT ( 'NONE',  ( 85.24325998657074877, -58.55267046464445002, -4.824374724089051547 ) ) ;
#82171=DIRECTION ( 'NONE',  ( -1.000000000000000078E-15, -1.000000000000000083E-30, 1.000000000000000000 ) ) ;
#82173=CARTESIAN_POINT ( 'NONE',  ( 115.3461623907574563, -31.52268719801062957, 34.27276813305396530 ) ) ;
#82174=CARTESIAN_POINT ( 'NONE',  ( 100.9654861239525161, -28.69876604995092961, 100.5949546195926132 ) ) ;
#82175=CARTESIAN_POINT ( 'NONE',  ( 108.9808406375926779, -47.59218431635552093, 118.7032443235299723 ) ) ;
#82176=FACE_OUTER_BOUND ( 'NONE', #82492, .T. ) ;
#82177=CARTESIAN_POINT ( 'NONE',  ( 108.7503283313270543, -25.75779200005056779, 144.9432443235299672 ) ) ;
#82178=ORIENTED_EDGE ( 'NONE', *, *, #16145, .F. ) ;
#82183=CARTESIAN_POINT ( 'NONE',  ( 136.8164832912740110, -36.72944715994100306, 3.101481641215515950 ) ) ;
#82185=CARTESIAN_POINT ( 'NONE',  ( 115.0909704615979763, -30.62031916169713597, 60.34404414507040570 ) ) ;
#82186=CARTESIAN_POINT ( 'NONE',  ( 102.8958089960464690, -27.08850953439599962, 155.4013395616249795 ) ) ;
#82188=CARTESIAN_POINT ( 'NONE',  ( 182.4202572930400095, -33.70561438051981185, -5.074374724088000832 ) ) ;
#82192=CARTESIAN_POINT ( 'NONE',  ( 105.7154773402737789, -46.72385839347782621, 77.46895861002991523 ) ) ;
#82193=VECTOR ( 'NONE', #66789, 1000.000000000000000 ) ;
#82195=ADVANCED_FACE ( 'NONE', ( #2416 ), #65957, .F. ) ;
#82196=AXIS2_PLACEMENT_3D ( 'NONE', #47282, #82295, #54977 ) ;
#82200=ORIENTED_EDGE ( 'NONE', *, *, #75755, .F. ) ;
#82201=ORIENTED_EDGE ( 'NONE', *, *, #84057, .T. ) ;
#82202=FACE_OUTER_BOUND ( 'NONE', #10679, .T. ) ;
#82203=B_SPLINE_SURFACE_WITH_KNOTS ( 'NONE', 3, 3, ( 
 ( #15593, #36480, #73209, #65513, #79610, #65948, #58678, #80055, #44604, #23317, #78724, #58251, #50983, #24625, #4185, #57802, #37364, #85539, #31427, #38251, #44156, #51416, #3298, #3735, #10989, #24189, #25070, #59127, #10109, #16478, #80495, #30990, #17811, #23749, #52293, #11448, #18254, #37817, #79167, #86422, #17369, #39145, #45051, #85980, #51858, #31881, #59571, #16928, #72341, #86864, #72781, #10548, #30105, #71896, #30552, #45487, #9655, #45932, #2406, #65071, #73665, #38689, #2853, #66394, #87306, #52734, #46834, #56224, #60014, #35346, #4632, #87749, #53639, #21748, #48960, #14929, #69885, #7658, #33234, #63060, #60933, #83975, #19598, #74562, #12804, #81413, #32779, #840, #28529, #76701, #81848, #39586, #5076, #40492, #66852, #68208, #49417, #32318, #77153, #19160, #11901, #89099, #55768, #12344, #25517, #60471, #53187, #80958, #18703, #46387, #14481, #88217, #40035, #25974, #67753, #74121, #5541, #26858, #42157, #83514, #61375, #88660, #67292, #26422, #54092, #21286, #5991, #47289, #75014, #33679, #8108, #23980, #43498, #50776, #51654, #49866, #71244, #8560, #78949, #36260, #77598, #79398, #58040, #1748, #37606, #23543, #63971, #29447, #70789, #57128, #72124, #50316, #2645, #16714, #85773, #37157, #84875, #42597, #35795, #15381, #30345, #78511, #29900, #51206, #65307, #63509, #70333, #9015, #16270, #1296, #43048, #36714, #22645, #44393, #78060, #15823, #29002, #9898, #64413, #2194, #56687, #71683, #43948, #84430, #57586, #85329, #9447, #3085, #23104, #30781, #64858, #58471, #22197, #86202, #80291, #4862, #38475, #67085, #26201, #5316, #24861, #66178, #18036, #4423, #53875, #59804, #10768, #73447, #46623, #74354, #31667, #73003, #52967, #3967, #11221, #44844, #3516, #45284, #32551, #72574, #60703, #17162, #24422, #33006, #52528, #65734, #39379, #79847, #45717, #87095, #88440, #10341, #12125, #38045, #31216, #59365, #58912, #87987, #86648, #18940, #39807, #38926, #67529, #66633, #52087, #87538, #32110, #80730, #25298, #18479, #17605, #46171, #25746, #73902, #11686, #60256, #53422, #81190, #55222, #35242, #19387, #62950, #6214, #26642, #13919, #69331, #27099, #42054, #19834, #28433, #81639, #47063, #33458, #13470, #5767, #54767, #7557, #54317, #62509, #82537, #68883, #82979, #47965, #7108, #33904, #12579, #67985, #47518, #40265, #41598, #83410, #74798, #41155, #13031, #75255, #20297, #6653, #40715, #75702, #61162, #76135, #88890, #61598, #82087, #68439, #34347, #34800, #89337, #27985, #726, #62054, #89788, #27542, #287, #55659, #20732, #48402, #21186, #48858, #76595, #14377, #69781, #78847, #77489, #70224, #22989, #1648, #84768, #37045, #78405, #7997, #50664, #43395, #57929, #22534, #65197, #49762, #36614, #49315, #85662, #16605, #22097, #70678, #29348, #23440, #8453, #35694, #57027, #72020, #64750, #30236, #51106, #36152, #64314, #2974, #56117, #29789, #44283, #2537, #50212, #84326, #83869, #9787, #15718, #37495, #77947, #71136, #8915, #2084, #21645, #57483, #77048, #14828, #85222, #16167, #43846, #71582, #9341, #42496, #63407, #63868, #1189, #28899, #56583, #15269, #42944, #31555, #66524, #17495, #79737, #44733, #32001, #74248, #87430, #80181, #24748, #51980, #59695, #18830, #32440, #73793, #45175, #46057, #59258, #4313, #72899, #10664, #72464, #25189, #12023, #52851, #17929, #52417, #38369, #80623, #46512, #60140, #10231, #45605, #37936, #66069, #39705, #3419, #11579, #3863, #73337, #18372, #86988, #39270, #11110, #51543, #17052, #86548, #79292, #66975, #87875, #86100, #38819, #4756, #24313, #25638, #53314, #81080, #67413, #30675, #58373, #23873, #65635, #31108, #58805, #40610, #55107, #26538, #41489, #21070, #68327, #54210, #61050, #76028, #82869, #48745, #6107, #48294, #47857, #6991, #34685, #13364, #27875, #81971, #19283, #61941, #33799, #61493, #13806, #27427, #46956, #89674, #82421, #62394, #89225, #14261, #88781, #75594, #88337, #173, #55550, #19719, #47407, #26989, #83303, #75136, #74686, #54655, #76479, #69219, #41936, #5203, #12922, #41051, #32897, #60594, #68776, #26096, #53765, #20182, #33351, #81531, #12467, #6542, #40151, #34237, #20626, #67872, #5659, #50998, #15155, #43736, #36934, #77833, #15610, #70567, #1975, #56921, #50098, #78293, #49650, #71024, #29672 ),
 ( #69667, #43283, #23332, #7439, #78741, #84212, #14711, #57366, #85106, #42831, #30121, #7886, #16496, #35128, #62839, #64635, #50551, #35579, #56466, #63296, #1073, #9235, #77376, #22876, #71474, #16056, #64203, #28785, #615, #28312, #42385, #2421, #8801, #84656, #57819, #85554, #56004, #83754, #8340, #36499, #21530, #76933, #36038, #21983, #49199, #63754, #70112, #1533, #29235, #22424, #79183, #37381, #73223, #80069, #85995, #3312, #17383, #45498, #25081, #65960, #66865, #11001, #51871, #9669, #32331, #45067, #31893, #65528, #4199, #53200, #60030, #79624, #31003, #72794, #31440, #80970, #86876, #37833, #10559, #73683, #11463, #58697, #10123, #17824, #86437, #38264, #71911, #30566, #72356, #59583, #65086, #87765, #44175, #51435, #25529, #3752, #2869, #66408, #16941, #59144, #24203, #58265, #23767, #39160, #44620, #24638, #52305, #38703, #52746, #87319, #45944, #4644, #80510, #18266, #12819, #6877, #61387, #88676, #54549, #5553, #74575, #20526, #41385, #27322, #33694, #81426, #46845, #82313, #18719, #20073, #62286, #46402, #71, #33246, #53655, #40942, #6433, #54105, #69115, #12357, #55450, #74138, #11912, #13695, #89561, #40047, #60944, #67763, #26434, #48193, #81859, #68667, #82765, #34128, #13257, #19612, #27771, #39598, #19174, #61828, #47750, #6004, #54996, #34581, #67305, #5093, #47302, #26873, #32791, #25985, #75027, #40503, #75924, #68223, #89113, #60481, #88230, #75485, #62737, #48638, #8234, #42720, #69562, #49091, #35467, #35923, #22313, #56359, #36394, #63642, #70011, #76374, #1869, #63189, #56808, #21417, #29126, #85002, #29567, #7780, #76821, #964, #21871, #22770, #77274, #83647, #28666, #70917, #8691, #14605, #55897, #70463, #42280, #84100, #20959, #41826, #28206, #84556, #14149, #57253, #83202, #49541, #7338, #15048, #1425, #43176, #49990, #77729, #15503, #35026, #64098, #512, #12200, #5385, #61231, #28051, #55293, #21253, #76210, #13986, #40786, #39888, #55730, #74426, #81705, #354, #19906, #33084, #6721, #47141, #82157, #54392, #62577, #67606, #41666, #60781, #88516, #88953, #83479, #83051, #26270, #69405, #7180, #68509, #34869, #6276, #53946, #27165, #47588, #20364, #26706, #40340, #19457, #74874, #20802, #89407, #12649, #68058, #48037, #5842, #75771, #33531, #75323, #13103, #33967, #61670, #34419, #62128, #54840, #82605, #13539, #41223, #68953, #89861, #27611, #48467, #14895, #35760, #77118, #42559, #78473, #56648, #8979, #23064, #64380, #43462, #70292, #30306, #14448, #21711, #36678, #84835, #36222, #2155, #43912, #42124, #58001, #49830, #57092, #85734, #56188, #77557, #8069, #85290, #63473, #83941, #48923, #29864, #1260, #49383, #69851, #78018, #22605, #803, #28966, #22163, #50277, #57548, #70749, #71647, #15786, #84396, #7622, #37122, #15342, #50737, #43011, #16236, #76665, #64823, #8524, #63932, #1711, #29414, #35308, #71203, #9410, #2605, #63021, #28497, #9092, #42596, #56223, #389, #21747, #49865, #21285, #70332, #1295, #8107, #27648, #41705, #77597, #7657, #68988, #55329, #69438, #56686, #6756, #84874, #78059, #48504, #57127, #76700, #89897, #63508, #14019, #48959, #14480, #29446, #34454, #8559, #62162, #83085, #28083, #22644, #22196, #41260, #43047, #70788, #35345, #36259, #63059, #50315, #83974, #42156, #77152, #55767, #7214, #63970, #1747, #15380, #49416, #34902, #62614, #14928, #20837, #35794, #76247, #83513, #69884, #839, #28528, #29001, #84429, #51205, #66177, #43947, #52527, #15822, #71243, #10767, #86647, #71682, #2644, #9446, #37156, #45283, #23542, #65733, #79846, #31215, #10340, #64857, #87094, #9014, #78510, #3515, #51653, #3084, #58911, #38474, #36713, #24860, #16713, #23979, #43497, #23103, #44392, #30344, #52086, #58039, #50775, #64412, #24421, #85772, #16269, #2193, #44843, #79397, #57585, #78948, #72123, #17161, #17604, #37605, #3966, #72573, #9897, #29899, #31666, #65306, #73002, #30780, #59364, #85328, #58470, #86201, #38044, #81189, #67528, #27098, #33005, #73901, #46622, #19833, #47517, #18035, #66632, #18478, #5766, #45716, #33903, #80290, #87537, #6213, #25745, #38925, #12578, #52966, #87986, #88439, #39806, #74353, #11685, #19386, #68438, #82086, #32109, #12124, #4422, #53421, #61597, #80729, #61161, #18939, #5315, #53874 ),
 ( #46170, #60702, #73446, #74797, #11220, #32550, #39378, #67084, #26200, #40264, #4861, #26641, #89336, #81638, #60255, #47062, #88889, #67984, #59803, #33457, #54316, #75254, #13030, #40714, #25297, #77488, #76134, #68882, #21644, #286, #83409, #35693, #77047, #6652, #49314, #42053, #56582, #21185, #63867, #48401, #35241, #47964, #84325, #15268, #20731, #69330, #27984, #22096, #7107, #34346, #55658, #70677, #63406, #28898, #49761, #34799, #62949, #1647, #54766, #28432, #42943, #1188, #48857, #82978, #82536, #8452, #14376, #36151, #76594, #69780, #7556, #725, #20296, #56116, #75701, #13469, #83868, #41154, #14827, #42495, #13918, #70223, #62053, #7996, #89787, #27541, #55221, #41597, #62508, #3418, #86547, #37494, #72898, #30674, #44282, #78404, #9786, #37935, #9340, #58372, #79291, #72463, #43845, #44732, #30235, #65196, #16166, #71581, #64313, #2083, #79736, #2973, #78846, #23439, #50663, #86099, #17494, #31107, #71135, #51105, #43394, #64749, #45174, #29788, #10230, #2536, #16604, #23872, #85661, #17051, #37044, #50211, #15717, #85221, #77946, #51542, #58804, #84767, #72019, #57928, #22988, #65634, #24312, #51979, #10663, #66068, #38368, #22533, #29347, #57482, #57026, #8914, #36613, #25188, #40150, #19718, #66974, #52850, #59694, #74685, #81530, #47406, #4755, #46955, #46511, #5658, #33350, #12022, #26537, #80622, #17928, #60593, #39269, #32439, #12466, #26095, #45604, #88336, #81079, #61049, #60139, #12921, #87429, #74247, #86987, #88780, #54209, #18371, #46056, #87874, #81970, #73792, #73336, #25637, #75135, #67871, #40609, #3862, #11578, #39704, #31554, #59257, #67412, #24747, #52416, #53313, #32000, #80180, #11109, #38818, #66523, #18829, #5202, #32896, #53764, #4312, #19282, #61940, #34684, #7885, #35578, #7438, #54654, #68775, #76932, #62393, #6106, #82420, #6541, #83753, #33798, #21982, #15154, #75593, #84211, #13805, #26988, #63295, #20625, #49198, #20181, #56465, #61492, #1072, #89224, #47856, #55106, #49649, #14710, #68326, #70111, #28784, #172, #77375, #27874, #13363, #21069, #48293, #14260, #82868, #34236, #41050, #89673, #42384, #83302, #27426, #76027, #41935, #41488, #69666, #69218, #6990, #55549, #48744, #76478, #614, #56003, #35127, #62838, #28311, #21529, #42830, #8339, #37832, #23766, #8800, #29671, #71023, #36498, #72355, #50550, #2868, #16940, #58264, #37380, #64202, #24202, #36037, #15609, #30565, #78740, #30120, #85994, #65527, #63753, #51870, #43735, #50997, #79623, #50097, #71473, #1974, #79182, #57365, #77832, #70566, #51434, #85105, #43282, #1532, #71910, #16495, #84655, #22875, #16055, #44174, #44619, #64634, #3311, #9668, #78292, #29234, #31002, #9234, #10122, #36933, #58696, #86436, #2420, #57818, #65085, #56920, #85553, #22423, #23331, #55341, #17382, #72793, #13584, #88229, #73222, #4198, #45497, #11000, #46844, #25080, #67304, #81425, #32790, #11911, #38702, #89911, #10558, #80068, #5092, #53199, #4643, #60480, #41271, #38263, #27663, #18265, #25528, #45066, #24637, #45943, #66407, #53654, #31892, #52304, #65959, #25984, #59582, #17823, #3751, #46401, #80969, #59143, #87318, #80509, #18718, #19173, #39159, #69001, #74137, #52745, #31439, #6769, #73682, #74574, #11462, #34469, #86875, #62174, #66864, #32330, #60029, #87764, #39597, #35810, #76711, #49430, #22657, #50330, #22208, #69451, #83529, #1759, #77166, #20850, #7227, #21299, #8572, #48516, #36727, #29912, #403, #9027, #28546, #41718, #78073, #35360, #63983, #34917, #71256, #76258, #15833, #14036, #62627, #69900, #64428, #29461, #83097, #84888, #43511, #14943, #2206, #42612, #28096, #63525, #63072, #29015, #7670, #48974, #55779, #14495, #57142, #8119, #42170, #851, #56699, #56237, #84443, #83987, #21760, #70344, #36272, #1307, #49882, #77611, #15392, #43061, #70800, #18052, #65747, #17176, #51665, #78964, #86662, #45730, #59376, #9459, #79413, #71696, #3097, #73458, #30356, #38488, #30794, #44859, #31228, #23993, #45296, #9914, #78523, #43961, #23554, #16280, #79863, #87108, #23115, #72588, #16725, #51219, #86216, #10352, #44403, #58486, #4435, #52098, #50787, #37619, #58053, #85783, #38058, #17617, #72139, #3982, #11235, #3533, #65318, #58923, #66188, #73016, #38939, #24436, #10785, #31680 ),
 ( #24876, #66646, #52542, #80303, #37167, #57600, #85343, #64875, #2659, #5329, #61616, #74368, #46182, #33023, #47980, #13046, #6228, #27113, #12141, #40282, #68901, #32122, #5782, #82552, #68453, #88455, #60269, #59819, #33919, #81651, #89352, #60718, #53889, #74816, #19401, #13485, #67545, #54787, #20311, #67999, #75715, #33473, #47082, #81203, #12593, #40729, #39828, #61176, #82102, #75269, #26212, #41170, #25760, #88904, #25313, #87552, #52980, #88000, #46636, #26656, #80741, #54336, #73916, #19850, #18494, #11698, #39391, #67097, #47536, #4878, #32569, #53436, #18955, #57042, #42959, #62967, #34816, #34361, #70693, #56132, #8471, #35257, #28448, #49330, #83887, #77962, #42068, #36169, #63885, #14844, #50228, #8015, #21660, #55674, #77064, #15287, #76611, #35710, #56599, #49779, #21200, #22111, #7571, #42512, #83425, #48872, #41612, #69348, #84786, #70240, #63422, #746, #27999, #1207, #22554, #1663, #48417, #28915, #20746, #69798, #15735, #7123, #77507, #84342, #29363, #43410, #6667, #62071, #14392, #27558, #82992, #62525, #55237, #89806, #76154, #13934, #300, #2554, #37065, #9805, #58389, #64769, #72035, #17943, #65650, #64329, #23456, #43864, #71597, #16621, #31126, #30254, #17510, #87002, #44302, #57945, #85679, #51995, #58825, #24765, #37515, #24327, #23890, #72912, #10680, #79309, #3878, #51123, #85237, #37950, #65214, #2990, #79754, #3434, #23006, #86562, #86117, #38385, #45191, #51562, #66088, #31569, #17067, #59274, #78864, #50682, #52434, #30691, #44753, #80196, #71153, #78422, #8931, #72480, #36629, #10246, #2100, #29810, #57500, #16184, #9358, #68343, #11595, #60155, #18848, #75152, #87892, #59712, #46529, #61506, #26552, #19741, #40627, #25655, #53782, #82438, #45622, #19298, #6125, #81986, #12036, #73810, #73356, #47425, #5220, #12938, #74264, #67430, #88354, #32912, #27006, #81099, #33816, #89241, #81547, #54674, #46969, #60611, #4773, #26113, #54224, #53329, #74704, #5677, #88799, #39721, #61067, #12486, #40167, #32457, #67887, #80640, #18388, #11127, #33367, #38834, #66540, #66990, #4329, #32015, #87446, #25204, #52866, #46073, #39285, #36054, #82884, #1090, #83317, #7455, #83772, #76495, #7898, #62410, #41067, #6557, #76043, #68790, #42401, #21997, #75611, #69685, #41506, #13822, #48765, #35144, #69238, #21087, #56934, #14728, #13380, #189, #20645, #48310, #55567, #70128, #7006, #56483, #63770, #14277, #34704, #27891, #28801, #35597, #1548, #41952, #62854, #630, #84228, #28329, #21543, #63314, #49667, #56023, #77392, #49215, #76947, #15168, #42845, #55122, #70584, #8357, #29249, #20199, #47872, #34256, #61957, #89692, #27444, #36513, #16510, #8816, #30136, #10574, #57380, #65543, #57832, #71923, #58279, #51014, #72369, #36945, #15625, #71041, #50566, #43297, #16955, #86451, #50112, #44188, #16072, #78308, #23347, #9688, #43751, #85569, #31455, #79198, #77849, #64651, #85123, #22890, #78756, #44636, #71488, #31020, #38279, #37396, #9250, #2438, #3326, #10137, #65975, #65099, #37846, #2882, #24218, #51883, #30581, #17398, #86011, #64217, #51447, #23783, #58710, #79639, #45080, #1987, #72807, #3766, #84672, #22436, #29686, #52760, #39611, #52319, #60960, #81874, #25097, #73699, #32343, #88688, #11475, #73236, #60046, #75043, #40058, #33257, #54117, #39173, #67317, #6018, #59160, #32801, #19624, #5565, #25539, #87334, #86888, #26444, #18731, #47311, #87777, #80985, #11923, #46414, #40514, #4658, #12830, #68235, #5106, #24653, #60496, #74149, #46857, #53214, #80083, #80524, #17837, #45515, #11016, #38720, #67776, #18277, #45962, #66876, #88243, #66423, #25999, #19186, #4212, #74589, #53668, #81435, #31906, #59598, #12368, #83658, #69573, #20978, #21430, #28682, #89129, #15061, #34593, #41837, #42735, #40957, #62297, #89574, #70023, #27334, #68679, #70475, #49103, #82776, #6447, #26886, #62746, #7347, #75497, #20537, #6890, #35037, #14618, #55461, #56371, #522, #41396, #54559, #21883, #84, #76832, #55009, #42290, #33707, #49552, #69125, #48204, #27781, #48652, #61398, #76383, #75939, #83214, #63201, #978, #28221, #20087, #34140, #7791, #14162, #82325, #47760, #61838, #35483, #13268, #77285, #13712, #55911, #84111, #43641, #56818, #3222, #50455, #79087, #84567, #86340 ),
 ( #71817, #64553, #85905, #78201, #29138, #22325, #64109, #50006, #30476, #10037, #63655, #57725, #29577, #1879, #36842, #85466, #57269, #9145, #44978, #2780, #30032, #30916, #9585, #15961, #1437, #24115, #71379, #23677, #85014, #58175, #17298, #51782, #2332, #22780, #23243, #50909, #8244, #78653, #16405, #44082, #37742, #65440, #37288, #77740, #8705, #16848, #64996, #35941, #15514, #36406, #51339, #43189, #79535, #70933, #44526, #72263, #58605, #31356, #67673, #24999, #53562, #59046, #60845, #65871, #39956, #10475, #3661, #59496, #26336, #81330, #19518, #74488, #12260, #39063, #5452, #66770, #88578, #25437, #52660, #18627, #87230, #38618, #33149, #54008, #19072, #87670, #45414, #10914, #46306, #72710, #74037, #81766, #38177, #86785, #80418, #17738, #4999, #60393, #18173, #24556, #66314, #52219, #79985, #73133, #4102, #46756, #31802, #45856, #73587, #11363, #4556, #32242, #32699, #59940, #88131, #67214, #53105, #80872, #11818, #39515, #25892, #83110, #34483, #34933, #42186, #12717, #28566, #48097, #55357, #56253, #54457, #75830, #13162, #83550, #40846, #82220, #84003, #62645, #6338, #19976, #40409, #76277, #20867, #89015, #34028, #20426, #48535, #28110, #47205, #14052, #7685, #21316, #13602, #75391, #74939, #48989, #6784, #76729, #41286, #69018, #89928, #62191, #68122, #82668, #14511, #69920, #41734, #870, #69469, #27678, #61732, #7244, #55796, #27224, #420, #35375, #63087, #89467, #5903, #33597, #61293, #54905, #26773, #47657, #68575, #73368, #29934, #71274, #15853, #43078, #50806, #11140, #24781, #63543, #43532, #35827, #57158, #38845, #84461, #3887, #84907, #9045, #85360, #78088, #9477, #64001, #42626, #8137, #77627, #70362, #43978, #52447, #77183, #36745, #70818, #15412, #50349, #64444, #8594, #22676, #59726, #16300, #14960, #1779, #22223, #49897, #2223, #71711, #36291, #59286, #66552, #57618, #29478, #23132, #31582, #37187, #4342, #78543, #66101, #87013, #80210, #17954, #45636, #32028, #21778, #1325, #49446, #29031, #56716, #68356, #19756, #39300, #54236, #74719, #89255, #53794, #6570, #81113, #67900, #80653, #27017, #20212, #53343, #12047, #60625, #54688, #39735, #11607, #88366, #13391, #6138, #61518, #82451, #67445, #5690, #34268, #47436, #75169, #32923, #47882, #25667, #87459, #25218, #52878, #75624, #33828, #18859, #74278, #46543, #5234, #41080, #26126, #12950, #68802, #40639, #81999, #81561, #18399, #46088, #60171, #73821, #33378, #12498, #67002, #4787, #32470, #87904, #19310, #61081, #46980, #40181, #88811, #26564, #8370, #55582, #69250, #8830, #77406, #21104, #7019, #55134, #1105, #7912, #13835, #48778, #35157, #63327, #42860, #83785, #84688, #28816, #69701, #27456, #50127, #62868, #49683, #83329, #22011, #71057, #77863, #7470, #76509, #644, #49228, #61968, #14745, #14293, #28344, #1561, #29262, #56498, #48321, #62424, #70598, #56038, #89707, #76056, #204, #15182, #82896, #15638, #20657, #34720, #43312, #21558, #41518, #56945, #41965, #36070, #27904, #76960, #42414, #22449, #70142, #35612, #84241, #63784, #17413, #73250, #38291, #65990, #2896, #3782, #30596, #24669, #79212, #16525, #72384, #23360, #2452, #31470, #59174, #45096, #51462, #9263, #64669, #10152, #36529, #37861, #80100, #64229, #17850, #51031, #71502, #9706, #24232, #57848, #86468, #45528, #52335, #44200, #85584, #37409, #23796, #2000, #16969, #30150, #58294, #86904, #29703, #65559, #22904, #36958, #72821, #86025, #57396, #50581, #78769, #51898, #85138, #78321, #16086, #43767, #71939, #65113, #44653, #3339, #31034, #10587, #58724, #79657, #4226, #68249, #38736, #31919, #87790, #54575, #81887, #47776, #12845, #40530, #67330, #6033, #5119, #89141, #53683, #81000, #46870, #25555, #66891, #33723, #61412, #19639, #26016, #73713, #39186, #74604, #11034, #12382, #82340, #66439, #20101, #53230, #45980, #33272, #88703, #46430, #26900, #4676, #59614, #87350, #25110, #52773, #47328, #32356, #18746, #60059, #74163, #80538, #11940, #60975, #75059, #26460, #5580, #39626, #18292, #11491, #32817, #54129, #40075, #88257, #60513, #81451, #19201, #67792, #76400, #83675, #56833, #82789, #14178, #41411, #21896, #69140, #20552, #22339, #995, #34609, #48218, #68693, #14631, #21448, #27349, #62313, #48668, #76848, #56387, #7360, #8258 ),
 ( #84127, #63215, #29150, #41851, #28700, #28233, #77299, #15074, #49116, #35958, #6906, #89592, #42305, #20991, #69590, #49567, #7804, #55025, #70038, #62761, #42748, #35051, #84580, #98, #55928, #6461, #70489, #63670, #27796, #55476, #536, #1453, #83226, #75953, #35496, #75511, #13282, #40973, #34153, #61855, #13726, #79548, #50017, #65009, #58617, #72278, #23255, #50471, #77752, #10048, #16418, #37755, #85479, #78668, #71829, #44092, #15529, #57740, #65453, #30929, #2793, #43203, #85920, #37303, #36854, #30491, #3235, #30046, #58188, #16861, #86355, #2344, #44541, #50922, #23690, #64565, #9596, #78213, #15975, #51797, #51354, #79099, #24125, #9156, #70947, #8720, #36421, #43655, #64122, #71394, #1892, #29590, #57282, #85025, #22795, #38098, #30839, #86702, #37659, #16768, #52582, #73505, #59419, #65789, #23598, #79000, #24479, #50832, #52141, #4476, #78570, #32165, #65357, #85828, #73054, #38535, #3574, #31271, #59859, #86253, #24918, #18089, #58965, #87591, #79903, #17658, #9955, #45334, #87152, #58528, #10830, #66230, #4019, #3139, #31722, #51705, #80340, #24035, #79455, #51257, #44448, #11277, #45778, #10393, #44898, #72179, #38982, #66690, #16322, #2697, #72628, #64912, #17219, #43999, #71735, #9504, #37211, #30394, #58092, #81690, #13084, #67590, #46224, #11737, #81246, #73959, #47572, #27152, #80790, #74858, #46680, #18997, #53932, #12633, #74410, #26254, #62113, #19891, #18538, #5368, #88045, #25808, #60765, #75306, #12185, #61651, #41208, #88500, #39869, #33064, #6262, #40771, #68935, #19439, #68495, #68040, #54824, #82590, #33515, #48019, #47123, #39435, #82142, #40320, #5827, #33952, #89390, #67138, #20348, #61216, #75757, #88938, #34404, #26691, #54372, #4918, #13526, #6704, #25349, #53021, #32608, #60309, #53480, #13972, #63005, #15772, #70737, #63920, #84822, #69837, #8053, #36663, #89846, #63462, #50263, #36207, #56175, #28037, #27597, #1697, #49370, #29401, #28486, #21697, #8965, #78003, #7610, #48910, #788, #77106, #55277, #42549, #83463, #83925, #57081, #22590, #28953, #76193, #338, #8510, #14883, #83035, #41652, #55716, #15325, #20789, #43449, #48454, #7167, #71190, #35293, #69389, #34857, #42111, #62563, #21239, #76648, #14434, #70276, #35748, #1246, #56635, #84382, #22152, #49818, #77544, #42996, #30730, #86152, #10284, #17983, #51600, #44342, #37989, #51159, #30287, #66126, #87046, #72950, #79348, #37106, #2592, #65686, #64366, #3473, #45664, #2142, #73396, #78900, #9396, #86598, #52037, #9848, #24810, #57984, #11167, #29848, #57536, #59312, #45229, #85718, #16658, #23494, #72076, #3915, #37552, #24369, #38425, #79797, #58862, #65253, #85276, #23045, #64809, #17552, #31164, #17110, #10721, #52476, #50722, #78460, #3029, #72523, #16220, #71632, #58425, #23927, #31611, #44794, #80234, #43898, #54269, #87929, #73846, #32060, #67930, #74748, #80678, #25696, #12078, #40209, #19784, #60651, #61551, #5717, #46569, #4371, #27049, #39763, #26592, #60196, #88840, #18431, #88391, #52907, #74306, #54719, #11633, #18886, #89286, #53373, #5258, #32953, #82034, #81137, #59755, #25244, #4814, #87487, #61110, #40668, #46117, #26151, #67475, #32500, #53820, #81588, #19339, #47015, #75653, #33411, #39325, #12525, #67034, #47468, #75199, #12980, #68389, #6166, #82484, #33855, #20238, #47911, #38873, #66577, #56981, #14324, #56528, #56067, #15216, #42892, #21590, #36101, #34750, #27487, #70170, #48804, #42000, #84274, #35644, #55162, #7945, #677, #70627, #69732, #22485, #7055, #83815, #6601, #8405, #63815, #69281, #27934, #76539, #1594, #55611, #82924, #7502, #29297, #22046, #77439, #84723, #83364, #49261, #50159, #13423, #76996, #41107, #49716, #35187, #41545, #68834, #34296, #62897, #62003, #28381, #14778, #42445, #63356, #89738, #1136, #20685, #48353, #28845, #76088, #13865, #62456, #230, #21133, #86495, #57881, #79242, #37890, #31060, #2484, #3371, #78797, #23823, #64705, #36998, #22937, #50614, #38322, #86053, #37442, #71974, #9295, #17002, #66020, #79690, #31497, #15669, #59205, #30182, #78356, #10181, #65588, #23394, #3811, #16118, #24701, #77892, #43346, #72849, #58754, #43795, #85615, #71533, #51059, #17443, #16554, #24260, #51930, #45125, #72417, #44235, #86939, #71088 ),
 ( #9738, #85166, #8863, #10617, #65143, #2926, #36560, #44686, #51492, #29744, #30628, #58326, #64262, #2036, #57430, #75084, #53712, #60089, #17879, #40560, #25589, #40103, #73739, #12413, #61438, #68280, #87825, #11522, #53262, #39659, #89168, #5150, #46006, #18777, #81920, #19673, #6061, #81479, #67359, #39217, #32847, #61001, #32387, #19230, #67819, #5610, #66929, #33303, #81031, #88289, #4709, #46460, #87380, #25139, #12874, #60542, #11975, #74197, #26045, #46906, #33749, #54158, #4258, #74636, #66467, #88730, #52367, #52799, #26485, #80129, #47355, #45556, #73286, #11062, #38764, #31954, #59648, #18325, #80573, #49145, #28728, #82366, #76425, #48248, #82817, #20130, #69168, #89622, #27377, #62345, #76882, #75980, #63250, #42777, #125, #13753, #20581, #7831, #14663, #70520, #27825, #70063, #69620, #56414, #84158, #35079, #49601, #41438, #41000, #83701, #55503, #83256, #35526, #42333, #68720, #21472, #14204, #21932, #21017, #35987, #6939, #7388, #47804, #77327, #15102, #34641, #48695, #41884, #8291, #62786, #6486, #563, #63700, #1025, #26938, #54606, #28262, #55957, #75541, #13314, #34184, #61890, #55056, #57770, #29623, #29181, #37784, #50952, #3269, #30076, #23289, #44123, #78697, #72748, #65483, #16896, #56869, #30960, #45020, #2822, #16446, #50503, #71862, #10080, #71424, #30519, #51381, #44575, #16006, #72307, #2376, #37333, #78249, #43687, #36449, #64154, #51828, #9627, #65038, #85511, #22825, #58221, #79579, #58647, #43234, #85950, #15561, #36886, #17340, #1927, #9189, #24158, #64595, #23721, #79130, #86382, #10517, #22369, #77783, #57311, #50046, #38222, #1481, #84611, #70976, #8749, #85058, #4601, #53153, #31847, #66816, #12765, #60438, #87274, #25938, #74981, #54054, #73633, #25040, #32285, #80922, #65915, #18670, #45457, #73177, #19119, #80463, #5044, #52260, #66360, #74533, #59983, #3702, #80025, #4147, #81374, #31395, #19564, #59092, #10955, #81813, #11409, #24597, #60898, #18222, #46800, #17779, #47252, #86828, #33197, #38660, #59540, #52703, #45902, #12309, #39107, #67717, #5503, #87713, #25482, #11865, #46351, #74082, #39557, #67260, #32742, #88182, #88627, #26381, #40002, #53608, #13211, #68621, #76322, #40454, #14101, #85285, #68174, #23059, #54949, #75440, #62692, #28163, #75880, #2151, #6385, #78469, #5956, #33645, #36672, #21367, #34074, #27274, #61779, #89518, #71199, #48145, #469, #14563, #55850, #34979, #82716, #50733, #61336, #40894, #83600, #41782, #27726, #49041, #64376, #89063, #26822, #41334, #48589, #54503, #47700, #69063, #20477, #76775, #13652, #6833, #82266, #42237, #34536, #62239, #20024, #69518, #7294, #26, #55405, #83160, #8975, #29860, #20918, #57544, #17561, #23937, #71642, #4383, #79362, #3926, #10296, #37563, #45241, #32070, #17994, #57997, #38003, #30300, #51613, #59766, #78910, #86163, #38884, #30741, #72533, #65695, #31622, #58433, #37118, #2601, #72085, #64819, #38433, #45675, #9406, #3480, #65263, #9858, #44805, #31174, #3043, #17120, #52921, #10729, #85730, #58873, #16669, #44356, #86608, #66139, #24382, #52486, #87496, #52045, #79807, #72961, #87055, #59326, #25254, #24821, #80247, #73408, #11180, #66588, #16232, #43907, #23505, #51169, #47479, #26164, #19351, #61561, #12992, #32508, #75211, #67942, #82495, #47024, #89750, #74319, #61122, #73858, #20252, #13434, #46580, #5271, #53832, #47923, #32968, #4824, #81601, #6614, #89298, #54732, #75664, #60663, #88851, #27499, #80692, #54281, #41119, #27062, #74759, #18897, #18442, #68844, #40223, #34311, #12537, #5729, #33421, #26603, #62016, #46129, #6178, #11644, #39338, #67045, #82045, #19798, #39772, #40678, #60208, #88401, #68399, #33865, #87944, #25709, #53383, #81150, #12087, #67485, #14337, #243, #27947, #15685, #63370, #14790, #21147, #69744, #28393, #84737, #7513, #69296, #56081, #71102, #36114, #29311, #50170, #35201, #1152, #2050, #55175, #28857, #43357, #1607, #21603, #83374, #82937, #56994, #42457, #22496, #83830, #77008, #7958, #70184, #36574, #77908, #70643, #20697, #8876, #64278, #56543, #35656, #42015, #84287, #63828, #62911, #22059, #15229, #8419, #689, #48364, #49277, #49729, #77451, #42906, #55623, #48819, #76099, #13878, #41560, #7067, #76555, #34763, #62467, #31516 ),
 ( #85628, #78368, #51945, #59222, #85182, #79255, #51072, #23404, #58338, #17017, #78812, #30640, #66485, #24279, #22954, #71984, #2500, #30198, #65155, #79703, #16570, #66035, #45572, #2938, #44250, #9754, #10632, #17457, #73300, #86067, #72863, #72428, #86951, #24715, #37901, #52379, #37457, #43809, #86509, #23838, #51507, #38335, #45137, #71548, #3824, #44700, #80143, #10194, #38779, #65602, #3384, #50627, #17893, #11074, #9310, #31076, #29756, #57893, #58770, #57441, #16131, #37011, #64716, #81935, #46476, #25152, #80589, #60105, #52815, #26502, #6074, #59660, #53728, #25603, #87841, #32860, #81493, #53278, #5166, #41014, #88744, #87392, #74213, #66940, #4723, #39674, #54175, #81047, #40575, #20146, #67376, #18792, #11988, #75099, #19689, #47818, #60558, #47369, #46920, #33763, #61455, #12428, #26953, #88303, #18336, #61016, #26060, #19247, #12888, #68294, #46022, #89188, #74653, #54621, #40117, #13326, #67835, #5627, #73756, #82381, #75558, #33316, #4273, #31967, #11537, #39233, #32402, #41898, #84625, #49615, #42794, #63716, #48710, #76895, #15577, #68736, #42347, #29200, #15118, #35093, #6953, #6505, #70536, #28278, #8304, #7402, #579, #21489, #55972, #50063, #36002, #84174, #34203, #1496, #22385, #70077, #83714, #27838, #49164, #77341, #76439, #7847, #28745, #21945, #83269, #56881, #69632, #14678, #55517, #21034, #13769, #41454, #77798, #35544, #63263, #62800, #139, #1037, #61904, #89637, #20594, #56431, #69183, #27391, #55069, #14222, #82832, #34655, #48260, #75994, #62357, #38236, #24175, #9206, #30090, #71439, #36899, #72763, #50967, #3282, #17355, #58663, #37799, #64608, #24612, #8763, #16021, #30975, #79150, #30536, #86401, #65931, #36464, #52276, #44140, #51398, #80040, #50520, #71878, #2392, #79595, #57785, #78263, #43248, #51841, #85528, #43702, #64170, #72324, #16911, #85073, #23302, #16461, #44588, #45035, #65055, #3718, #10095, #78710, #1940, #31409, #9642, #10533, #37349, #59111, #70991, #86844, #2838, #58236, #85964, #23735, #29637, #65499, #22839, #57328, #60917, #32301, #46814, #4167, #18239, #26401, #74102, #45473, #31863, #45917, #33216, #73193, #61353, #54522, #25054, #33663, #53170, #66376, #12783, #59999, #88644, #59554, #5974, #10972, #74999, #38674, #87290, #4616, #89082, #54074, #17793, #19581, #47273, #11882, #39570, #53624, #26839, #5061, #87730, #81391, #25502, #73647, #40475, #68192, #81828, #32761, #80481, #11427, #19141, #52718, #74547, #39129, #66831, #80939, #18686, #46368, #67277, #60456, #88198, #25957, #12327, #40020, #67735, #5523, #48605, #14120, #28177, #35898, #69533, #62256, #55867, #69086, #48164, #84069, #15017, #939, #7310, #54967, #20498, #83618, #82286, #21385, #63610, #20042, #1391, #6850, #27293, #14578, #69981, #27741, #42691, #75898, #29095, #47719, #75459, #77247, #63157, #13666, #34551, #41352, #42, #21841, #55424, #42253, #56322, #7750, #76791, #83175, #13228, #40914, #82734, #35441, #49059, #34995, #28636, #70432, #68637, #6402, #20933, #486, #34095, #89536, #76342, #41796, #49511, #62707, #8205, #61799, #72219, #15917, #1841, #49960, #85863, #2736, #8658, #43594, #29993, #58131, #37699, #78606, #79491, #23633, #64509, #22285, #44933, #57683, #44487, #78157, #16805, #65825, #72663, #2289, #71333, #85426, #44038, #3610, #9544, #36356, #64066, #9990, #9104, #51293, #43147, #57224, #65398, #23201, #84527, #70888, #84969, #3178, #77694, #10430, #56779, #29539, #38132, #50868, #15478, #51741, #36801, #30876, #22739, #50414, #16360, #71773, #58561, #37249, #64952, #30436, #79040, #86291, #24071, #17253, #86739, #80827, #52616, #87186, #59894, #18576, #24950, #32198, #68075, #25846, #24510, #73540, #4057, #31756, #66725, #81280, #80378, #67624, #47159, #4510, #18127, #45811, #12219, #19026, #74892, #87627, #74443, #73992, #33103, #60800, #39468, #53964, #11314, #45372, #88083, #25391, #53057, #39907, #53512, #73092, #46713, #46256, #88533, #11771, #40361, #39015, #67170, #52174, #26287, #81724, #4953, #32649, #60345, #19476, #5408, #10870, #12670, #31305, #59001, #79937, #17693, #38568, #66266, #59452, #42580, #69422, #56207, #42141, #62147, #33986, #33547, #69869, #55312, #7641, #34438, #27631, #48487, #83068, #77137, #35330, #21269 ),
 ( #41687, #82624, #54859, #40805, #68527, #83958, #14003, #20822, #89880, #27184, #34887, #21729, #63042, #47609, #76229, #19928, #41241, #49401, #6295, #75790, #28514, #20385, #7197, #28068, #83498, #68972, #14914, #61688, #5862, #61249, #88971, #824, #76684, #89423, #48055, #13556, #6739, #26727, #62597, #55751, #54410, #48942, #373, #14464, #82173, #75342, #13121, #30329, #16255, #57569, #58021, #65290, #35780, #51639, #71225, #78495, #79383, #77580, #8997, #36242, #16697, #63952, #15365, #17145, #85757, #29432, #43030, #63494, #9431, #43930, #22182, #57112, #43480, #71668, #51191, #2177, #3066, #37142, #78040, #1279, #58457, #36698, #23529, #1731, #78932, #70315, #86187, #15808, #84858, #64399, #85313, #8090, #23086, #49851, #70772, #44379, #22627, #64843, #56670, #8544, #72108, #29886, #28984, #84414, #50300, #9882, #50760, #23962, #2627, #37589, #30767, #80276, #3502, #41025, #87079, #26966, #31199, #34213, #38028, #13340, #72557, #65720, #31650, #89650, #54631, #82843, #47832, #75570, #11206, #66616, #80716, #27400, #32094, #24845, #18465, #59350, #10754, #68746, #6517, #82395, #59790, #17587, #72986, #46154, #44829, #73883, #55080, #10324, #58895, #52511, #79831, #4407, #38906, #66163, #11670, #61917, #86633, #24407, #87522, #52071, #18019, #45270, #38459, #45702, #3949, #73433, #25283, #52948, #33771, #39363, #67069, #6084, #61466, #89200, #20157, #70545, #48268, #21505, #48720, #21047, #589, #49175, #76453, #28291, #50076, #1048, #13779, #69645, #27850, #55526, #35105, #56443, #14237, #15128, #29212, #62812, #41913, #7413, #49626, #84187, #84634, #55982, #21960, #76909, #8316, #36015, #42358, #63728, #83726, #6969, #63273, #14688, #70086, #77350, #28758, #34663, #42807, #7857, #1510, #35557, #22394, #56896, #20603, #41465, #76002, #69194, #62368, #150, #83278, #41314, #54032, #25921, #74960, #27704, #82693, #75857, #6808, #81791, #20002, #48567, #11845, #75417, #62219, #48123, #68151, #39983, #39539, #13629, #61318, #69043, #40433, #33625, #54483, #89040, #83137, #34511, #27254, #67242, #4, #55381, #13191, #26802, #60876, #82246, #20453, #19544, #40874, #61758, #54929, #26363, #20895, #12744, #47682, #88607, #47233, #46782, #74513, #5026, #68602, #32724, #60417, #88162, #67698, #5935, #6363, #53589, #34054, #81358, #89493, #19097, #12293, #5481, #33178, #56282, #84489, #23159, #76303, #49920, #36766, #22699, #42650, #14536, #14074, #50370, #35854, #78117, #14981, #8164, #29056, #63572, #57639, #15880, #1804, #41760, #43558, #29955, #77655, #1353, #35399, #56745, #84932, #84027, #15436, #36317, #29502, #899, #57185, #77210, #22250, #63117, #28593, #21342, #49016, #64468, #43104, #70849, #70389, #7709, #8621, #2251, #71298, #28137, #64027, #444, #21804, #85384, #76752, #49473, #9066, #69494, #7271, #34957, #62668, #55828, #83578, #42215, #69942, #85844, #37226, #2717, #10411, #64491, #38114, #18109, #2268, #45793, #79021, #9523, #86720, #52156, #9973, #24933, #30415, #11294, #29970, #57661, #59436, #45353, #58112, #51274, #23616, #16785, #4038, #72198, #24494, #38551, #79920, #58980, #44466, #73519, #85406, #64931, #17674, #65805, #51721, #73073, #87167, #23181, #50849, #65378, #72645, #78588, #71756, #3158, #37678, #10851, #16340, #44018, #52597, #66246, #30855, #58545, #86274, #24053, #31739, #79475, #80358, #17235, #44914, #3594, #31287, #20363, #4493, #11753, #88952, #74873, #26269, #26705, #33966, #32178, #48036, #39887, #47140, #75770, #46239, #67605, #4934, #75322, #32629, #73974, #38997, #54391, #88062, #39450, #59874, #68057, #12648, #80805, #25826, #12199, #40339, #19905, #60780, #61669, #5841, #46694, #87607, #27164, #5384, #82156, #60327, #47587, #66706, #54839, #74425, #53496, #33083, #53945, #25371, #81704, #18556, #67152, #13102, #81262, #33530, #53039, #19011, #40785, #88515, #19456, #61230, #68508, #6275, #89406, #82604, #50276, #20801, #29413, #48922, #62127, #8523, #55729, #84395, #89860, #1710, #6720, #70748, #41222, #34418, #353, #57091, #22162, #13538, #15341, #43010, #69850, #35307, #49382, #84834, #802, #83478, #77117, #28050, #69404, #21252, #63020, #8068, #34868, #76209, #41665, #14894, #68952, #42558, #22604, #27610, #55292, #76664, #48466 ),
 ( #14447, #7179, #62576, #36221, #42123, #63472, #77556, #28965, #35759, #7621, #83050, #13985, #28496, #1259, #70291, #56187, #56647, #63931, #83940, #21710, #49829, #86166, #59329, #85289, #16673, #43911, #24385, #71646, #23063, #24823, #3482, #37121, #50736, #71202, #17123, #23940, #29863, #64822, #51172, #79365, #58875, #9861, #10731, #44809, #85733, #43461, #66141, #78913, #65699, #9409, #38006, #87057, #3928, #23508, #2604, #44359, #65267, #78017, #30744, #57547, #78472, #31176, #30305, #72536, #64379, #16235, #86611, #72088, #15785, #2154, #58000, #52048, #8978, #31625, #36677, #37567, #3046, #58437, #51617, #72964, #10300, #79809, #17563, #45244, #38435, #19800, #80251, #73410, #39340, #6180, #33423, #89300, #54283, #82047, #18899, #74321, #88404, #33868, #39774, #32510, #26166, #67047, #18444, #60211, #12090, #47026, #73861, #25257, #80694, #53834, #52488, #81604, #61564, #17996, #45677, #4827, #87499, #74761, #40226, #87946, #47481, #25711, #12539, #26607, #67944, #5732, #11647, #11182, #38886, #52923, #61124, #19354, #67487, #88853, #75214, #66592, #4385, #53385, #60665, #32072, #59768, #81153, #46131, #12995, #46583, #5274, #32970, #40681, #68401, #62018, #20256, #56083, #62914, #68846, #76101, #246, #28395, #7960, #48821, #49731, #83832, #34766, #82497, #15232, #27949, #14792, #48367, #77011, #36116, #42908, #62470, #13880, #55626, #14339, #63831, #69746, #6617, #34313, #70188, #41563, #21606, #13436, #27502, #35658, #83376, #54734, #41122, #55179, #42459, #47926, #70645, #27064, #89752, #8421, #21149, #75666, #22061, #69298, #63372, #82939, #20699, #7069, #84290, #76558, #42018, #7515, #35204, #1154, #691, #28859, #56547, #49280, #77454, #37459, #45140, #78814, #71551, #65158, #78371, #57443, #9313, #51074, #86069, #22956, #64280, #29758, #2941, #1611, #30643, #72865, #29313, #10634, #16134, #36577, #23841, #79257, #37013, #51947, #85185, #38339, #56996, #84739, #86512, #72430, #50629, #43811, #64718, #2502, #30201, #15687, #57895, #17460, #10198, #65604, #24281, #85631, #9756, #22498, #50173, #58340, #79705, #37904, #23407, #16574, #77910, #3386, #44252, #31079, #71986, #51510, #17019, #44702, #43359, #58772, #71105, #8879, #2053, #19691, #67379, #81049, #25154, #46479, #74657, #46024, #5168, #26063, #19249, #80591, #81497, #66943, #11990, #52819, #18338, #11076, #38781, #26505, #74216, #25605, #60109, #87394, #32862, #54177, #67838, #17895, #87843, #80145, #11541, #81940, #66488, #73758, #88747, #39236, #32404, #53280, #53731, #4725, #86953, #47371, #18795, #39676, #75102, #5629, #31519, #60561, #88305, #31969, #46922, #12430, #59663, #40119, #12890, #33319, #59224, #61019, #4276, #66037, #3826, #24718, #52382, #45575, #73302, #13773, #89640, #6508, #21493, #28282, #85421, #41457, #83716, #83271, #42349, #70079, #48712, #64505, #61907, #54623, #7404, #75996, #69185, #49166, #62802, #82384, #35095, #27840, #7849, #6957, #50864, #34205, #21038, #33765, #35547, #2283, #27393, #55072, #34657, #29988, #57677, #23198, #41901, #55519, #82835, #76442, #76898, #20596, #69635, #581, #14681, #48262, #55974, #62360, #14225, #142, #78602, #75561, #13329, #40578, #68296, #6076, #61458, #89192, #26956, #20148, #47821, #41016, #68738, #30431, #51736, #32193, #79035, #86286, #39010, #30872, #72657, #10425, #4052, #58558, #37243, #87620, #38128, #52169, #4505, #18122, #71769, #65821, #37693, #72215, #44929, #3605, #9986, #17248, #53053, #10865, #9539, #24066, #16800, #44482, #79487, #66261, #65392, #52609, #59888, #31299, #3174, #58995, #87180, #31752, #25385, #86735, #59448, #24506, #45807, #73534, #79932, #66721, #17687, #58126, #73087, #45367, #38562, #24946, #80373, #85860, #11310, #16355, #44033, #64948, #2730, #23629, #51288, #73988, #82618, #13551, #46709, #5402, #53959, #20379, #33099, #4948, #81719, #6735, #61683, #54855, #75786, #60796, #88966, #27625, #80822, #54405, #41237, #27179, #47155, #19022, #18571, #48051, #40356, #68967, #19471, #12664, #33543, #68071, #62143, #34433, #6290, #46252, #5858, #74888, #12214, #19923, #89876, #11767, #32642, #61245, #60340, #26283, #39464, #53508, #88529, #67165, #26722, #82169, #47603, #68522, #75338, #88078, #25842, #13117, #40801, #81276 ),
 ( #33981, #89419, #39903, #74438, #67618, #28509, #14460, #21265, #36238, #43026, #8994, #56203, #8539, #8085, #57107, #84853, #63489, #78036, #76680, #69418, #22178, #819, #83954, #63948, #77573, #7193, #49846, #42573, #22620, #21725, #64394, #48938, #35776, #48482, #50295, #15804, #42137, #69865, #49397, #43475, #7635, #34883, #77133, #71221, #1727, #29428, #36694, #35324, #1275, #2172, #55307, #28980, #83064, #20817, #14910, #83492, #76224, #13999, #70309, #41682, #56666, #84410, #15359, #70768, #62591, #368, #28064, #55747, #63037, #73427, #31194, #44825, #78928, #10319, #38453, #9878, #58890, #79827, #72982, #44374, #45265, #30763, #65716, #16692, #72104, #64839, #2621, #58017, #58452, #38024, #11202, #37137, #86182, #85753, #66158, #23524, #30324, #66612, #10749, #37583, #51187, #23082, #86629, #3496, #71663, #65285, #3062, #24403, #3945, #51634, #52505, #52067, #23957, #85308, #18014, #79379, #17581, #17141, #31646, #38902, #45697, #72551, #59346, #87075, #24841, #29881, #80271, #9426, #57563, #50756, #78489, #16251, #43926, #4845, #13009, #60683, #32090, #80711, #32527, #19816, #59786, #47940, #41136, #11666, #20274, #39788, #52943, #12106, #40244, #82512, #60233, #75681, #87516, #61578, #25277, #18460, #81170, #13449, #75233, #4402, #6195, #33882, #88420, #26182, #67962, #46150, #81619, #74335, #5748, #18916, #87965, #67503, #53850, #88867, #25728, #67065, #53402, #33438, #73879, #61142, #39359, #46602, #5294, #32985, #19369, #26623, #82065, #47043, #54748, #74778, #12556, #54298, #47496, #89315, #40696, #68418, #27079, #7086, #34780, #8434, #76575, #28875, #42922, #84307, #63388, #264, #50191, #34328, #41578, #56564, #14807, #56098, #22078, #63845, #62034, #77926, #42034, #70205, #49743, #706, #1628, #7975, #14356, #89768, #57008, #69761, #77467, #27962, #15248, #15700, #84750, #7532, #55640, #35221, #83846, #68859, #21623, #48381, #76115, #70660, #83389, #35675, #55197, #69312, #36132, #62928, #6631, #82955, #62485, #29328, #27518, #22511, #20712, #13895, #21165, #28412, #48835, #49296, #42473, #77029, #1170, #31535, #36593, #10644, #71117, #64294, #30216, #86968, #24294, #80159, #45153, #72877, #9769, #65174, #79272, #24729, #30656, #23420, #17034, #57908, #9323, #51087, #2954, #37916, #64731, #16148, #71562, #44714, #43374, #72442, #52393, #8892, #2066, #85643, #78385, #65615, #31089, #78824, #3839, #37025, #29770, #57460, #85202, #38349, #51960, #2515, #16586, #44264, #72001, #66048, #37472, #3396, #17471, #58782, #86527, #58353, #22969, #50644, #43823, #79716, #10210, #86080, #59238, #23852, #51523, #89204, #18808, #26076, #26970, #25166, #46490, #73770, #54189, #11557, #52830, #54637, #33332, #66957, #80603, #11091, #46936, #53741, #59675, #4737, #61471, #32416, #18352, #40132, #5640, #53295, #68305, #46038, #17906, #45586, #73316, #12901, #88758, #39249, #60121, #87855, #25620, #47384, #81061, #67853, #81952, #61029, #12444, #74229, #38796, #66502, #12004, #26517, #81511, #5182, #19700, #40590, #4291, #31981, #39687, #19263, #87406, #67390, #32876, #60576, #75116, #88317, #74667, #6089, #33776, #41469, #27405, #75574, #21510, #28295, #34217, #69200, #55531, #83732, #63278, #14241, #15134, #49179, #154, #47836, #70550, #83283, #70091, #13783, #42363, #1514, #8322, #27854, #6973, #21052, #69649, #29216, #35110, #61922, #89654, #35561, #34667, #76913, #68751, #82847, #1055, #48724, #20161, #6521, #20607, #7862, #13344, #36020, #82400, #55084, #63732, #76459, #41031, #41917, #55987, #48273, #76008, #62373, #7418, #49631, #62817, #595, #14692, #28763, #56447, #84192, #21964, #77356, #42811, #78723, #2852, #10547, #44154, #36915, #30551, #43716, #22856, #64619, #16477, #51414, #78276, #29650, #85086, #58250, #56902, #85979, #38250, #84639, #16038, #30104, #23748, #37816, #71895, #79609, #79166, #2405, #22400, #45050, #57801, #44603, #71456, #16927, #65946, #72780, #85538, #9219, #23316, #9654, #3734, #37363, #36479, #64184, #10108, #50982, #72340, #43265, #57345, #65512, #65070, #50080, #71005, #50533, #3297, #77814, #15592, #8779, #1956, #30989, #58676, #86421, #24188, #51857, #17368, #59570, #19596, #24624, #88659, #59126, #52292, #18253, #75013, #12342, #68207, #33233 ),
 ( #86863, #80957, #52733, #87305, #60013, #18702, #25069, #32317, #31426, #25973, #80054, #73664, #4184, #31880, #66851, #81412, #80493, #67752, #47288, #4631, #45931, #11447, #40034, #19159, #12803, #87747, #74561, #74120, #60932, #26421, #39585, #54091, #39144, #45486, #88216, #25516, #53186, #5540, #53638, #73207, #46833, #46386, #81847, #11900, #40491, #67291, #5074, #17810, #10988, #38688, #32778, #60470, #66393, #35457, #48180, #20058, #69101, #49077, #20514, #35011, #82301, #6420, #14593, #62273, #33678, #47738, #34111, #21404, #61374, #49529, #42709, #13244, #21860, #41369, #54536, #13680, #41814, #84088, #61817, #77264, #89098, #63174, #26856, #75473, #82752, #15035, #76809, #5990, #7769, #955, #56, #27759, #69549, #40930, #83191, #75913, #7326, #6867, #89550, #34567, #55439, #502, #27309, #68653, #54981, #62725, #20948, #28193, #48619, #76360, #14136, #55882, #83633, #42270, #69997, #28653, #56344, #8677, #17275, #70448, #35914, #65419, #51316, #36379, #57243, #64085, #1860, #10011, #78179, #30456, #44507, #85882, #64971, #29558, #51763, #63627, #43165, #58153, #16383, #57703, #23650, #3201, #1413, #79512, #71356, #78626, #8223, #77713, #9123, #84987, #16825, #22760, #15495, #29113, #79059, #50433, #70907, #56797, #9563, #44058, #22303, #15937, #43613, #71792, #72239, #2309, #30895, #37269, #36822, #84544, #58580, #64529, #37723, #30011, #86314, #49977, #24091, #85446, #23221, #50887, #2759, #82977, #87651, #24532, #52197, #72688, #31329, #73114, #60368, #10453, #89786, #44953, #79959, #62052, #80399, #3630, #52639, #80851, #34345, #10890, #27540, #38154, #13468, #65846, #59023, #31780, #55220, #27097, #86762, #47963, #75700, #11340, #66748, #18599, #17718, #32221, #24972, #46283, #59474, #38589, #18149, #4532, #39493, #66293, #45393, #4078, #74015, #87209, #11796, #45832, #73562, #39038, #59915, #25413, #67192, #32674, #53080, #6651, #4974, #89335, #54765, #82535, #41153, #20295, #68881, #7555, #48856, #76593, #50210, #28431, #70676, #84766, #36150, #15267, #42052, #2082, #76133, #83408, #8451, #56581, #7995, #63866, #15716, #13917, #29787, #21643, #28897, #57481, #27983, #49313, #14375, #57025, #69779, #55657, #20730, #1646, #35240, #21184, #41596, #49760, #84324, #62507, #62948, #83867, #22095, #29346, #42494, #43393, #77487, #56115, #69329, #8913, #77046, #22532, #724, #77945, #48400, #36612, #14826, #70222, #35692, #63405, #7106, #1187, #285, #42942, #71134, #64312, #34798, #71580, #85660, #3861, #51541, #44281, #30234, #78403, #24311, #31106, #37043, #72018, #58371, #86546, #66067, #17050, #17927, #51978, #2972, #50662, #73335, #86098, #72897, #16603, #45173, #4311, #11108, #30673, #9785, #23871, #72462, #31999, #37934, #64748, #2535, #38367, #37493, #79735, #9339, #23438, #31553, #79290, #22987, #57927, #51104, #10662, #16165, #38817, #85220, #78845, #66522, #44731, #43844, #10229, #58803, #65195, #65633, #3417, #17493, #52415, #59256, #86986, #24746, #80179, #45603, #6540, #61491, #89223, #26094, #81529, #5657, #13362, #46954, #39703, #33349, #46510, #25636, #67411, #19281, #54208, #81078, #32438, #87873, #61048, #59693, #88779, #41049, #87428, #68774, #74246, #4754, #81969, #47405, #5201, #20180, #53312, #25187, #52849, #80621, #54653, #40608, #18828, #12021, #32895, #60592, #26987, #88335, #19717, #33797, #75134, #12920, #53763, #18370, #46055, #60138, #68325, #26536, #74684, #6105, #82419, #73791, #11577, #12465, #67870, #39268, #66973, #40149, #47855, #75592, #27873, #41487, #71022, #49648, #7437, #50096, #15153, #8338, #29233, #14259, #42383, #34235, #61939, #7884, #84654, #70565, #613, #62392, #89672, #36036, #83752, #63752, #62837, #56002, #76931, #21528, #15608, #1531, #77374, #27425, #56919, #77831, #35577, #49197, #83301, #14709, #42829, #41934, #63294, #84210, #22422, #48743, #43281, #35126, #70110, #21068, #76477, #55105, #69665, #82867, #34683, #1071, #28310, #55548, #28783, #20624, #48292, #76026, #56464, #13804, #21981, #69217, #6989, #171, #31438, #23330, #65084, #2867, #86435, #50996, #29670, #80067, #30564, #44618, #86874, #10557, #64201, #58263, #30119, #64633, #37379, #85993, #2419, #9667, #45496, #3310, #1973, #78739, #71472, #9233, #44173 ),
 ( #16939, #59142, #57817, #22874, #65526, #71909, #23765, #79622, #31001, #50549, #58695, #51433, #38262, #79181, #17822, #85552, #72354, #57364, #65958, #24636, #16494, #10121, #37831, #3750, #24201, #78291, #51869, #17381, #52303, #36932, #8799, #36497, #85104, #16054, #45065, #72792, #43734, #45942, #73681, #60943, #60028, #19172, #5552, #46843, #53653, #11461, #75026, #10999, #80508, #74573, #32789, #11910, #12356, #88675, #38701, #12818, #53198, #5091, #47301, #52744, #80968, #39158, #67762, #66863, #18264, #73221, #33245, #32329, #4642, #31891, #81424, #25983, #87763, #25527, #18717, #40046, #26433, #39596, #19611, #54104, #46400, #59581, #66406, #74136, #81858, #67303, #4197, #87317, #25079, #60479, #88228, #41466, #34214, #14689, #89651, #42359, #83727, #33773, #7858, #21961, #69646, #83279, #27401, #48721, #76910, #48270, #7414, #28292, #21506, #82844, #49176, #69195, #14238, #55081, #20604, #56444, #76004, #61467, #68747, #27851, #62369, #13780, #35106, #84188, #70088, #20158, #151, #82396, #6970, #49627, #41028, #34664, #1050, #55528, #21049, #76454, #55984, #41914, #89201, #77352, #62814, #590, #15129, #35558, #26967, #63274, #28759, #61918, #68302, #6086, #54632, #47833, #75571, #13341, #6518, #8775, #80393, #64180, #18141, #59466, #8317, #73554, #87643, #45387, #59016, #1953, #24523, #52632, #22851, #73107, #4071, #87200, #57340, #24964, #43713, #79952, #29646, #85082, #32212, #50530, #36017, #43261, #3623, #38147, #78273, #10883, #59909, #45824, #84636, #65840, #56898, #16034, #25405, #15587, #71452, #66741, #10445, #31321, #86754, #31772, #52189, #63729, #53071, #17709, #38581, #80841, #11331, #1511, #66283, #39030, #36476, #4524, #42808, #70546, #29213, #22395, #50077, #77810, #71002, #81298, #19041, #53979, #68540, #39920, #54872, #34451, #81739, #67639, #74457, #89435, #6309, #62159, #19489, #61702, #61264, #20399, #48069, #26744, #41257, #5423, #32664, #75356, #47172, #74905, #27196, #40818, #60359, #13135, #5876, #75803, #12686, #27645, #12233, #88985, #11787, #13568, #68985, #33118, #60814, #40376, #6753, #88547, #88099, #68090, #89893, #82639, #55326, #18590, #26304, #54423, #46273, #74007, #82186, #39483, #67184, #33561, #46729, #4967, #25860, #19942, #53526, #47624, #34001, #28998, #69881, #48956, #836, #42593, #77594, #14477, #55764, #21282, #56683, #83082, #84426, #36710, #20834, #64409, #7654, #28080, #15377, #70785, #28525, #43494, #76697, #29896, #48501, #76244, #78056, #63967, #42153, #35342, #63056, #56220, #22640, #83971, #43044, #57124, #8556, #36256, #21744, #2190, #14016, #83510, #1744, #22193, #70329, #29443, #15819, #41702, #69435, #49413, #1292, #7211, #386, #77149, #14925, #84871, #8104, #35791, #34899, #50312, #63505, #49862, #62610, #71240, #9010, #9443, #16710, #30777, #58907, #38471, #79393, #80287, #86644, #65303, #23100, #45713, #58467, #45280, #78944, #17601, #66629, #73443, #3081, #44389, #50772, #65730, #37602, #66174, #37153, #64853, #10764, #72119, #24418, #43943, #58036, #3962, #23975, #85325, #71679, #85769, #72999, #78507, #11217, #4419, #2641, #38921, #86198, #16266, #51650, #3512, #57581, #23539, #30341, #51202, #24857, #9894, #17158, #44840, #72570, #31663, #10337, #59361, #87091, #38041, #31212, #52083, #79843, #52524, #18032, #11682, #39375, #75251, #46619, #61158, #18475, #32546, #40711, #88436, #59800, #46167, #60252, #47513, #87534, #75697, #68877, #67081, #47960, #67524, #80726, #39803, #67981, #20292, #87983, #13465, #25294, #89332, #52963, #73897, #18935, #41150, #13027, #32106, #33899, #61594, #26197, #53870, #5763, #4858, #19383, #12121, #33454, #74350, #25742, #5312, #81635, #26638, #53418, #81186, #33002, #88885, #60699, #54313, #47059, #74794, #12574, #40261, #82083, #19830, #68435, #6210, #82531, #27094, #54762, #6648, #62049, #1643, #77483, #62503, #83405, #34795, #282, #36147, #14372, #56578, #70673, #22092, #1184, #27980, #77942, #89783, #69326, #84321, #42490, #83863, #49757, #29343, #27536, #15713, #7551, #14822, #43390, #13913, #35237, #55654, #42939, #21181, #41593, #34342, #15264, #48852, #7103, #55217, #35689, #70220, #48397, #76590, #69776, #7992, #8448, #28428, #57022, #63402, #42049, #82974, #84763, #62945 ) ),
 .UNSPECIFIED., .F., .F., .F.,
 ( 4, 3, 1, 1, 1, 3, 4 ),
 ( 4, 1, 1, 1, 1, 1, 1, 1, 1, 1, 1, 1, 1, 1, 1, 1, 1, 1, 1, 1, 1, 1, 1, 1, 1, 1, 1, 1, 1, 1, 1, 1, 1, 1, 1, 1, 1, 1, 1, 1, 1, 1, 1, 1, 1, 1, 1, 1, 1, 1, 1, 1, 1, 1, 1, 1, 1, 1, 1, 1, 1, 1, 1, 1, 1, 1, 1, 1, 1, 1, 1, 1, 1, 1, 1, 1, 1, 1, 1, 1, 1, 1, 1, 1, 1, 1, 1, 1, 1, 1, 1, 1, 1, 1, 1, 1, 1, 1, 1, 1, 1, 1, 1, 1, 1, 1, 1, 1, 1, 1, 1, 1, 1, 1, 1, 1, 1, 1, 1, 1, 1, 1, 1, 1, 1, 1, 1, 1, 1, 1, 1, 1, 1, 1, 1, 1, 1, 1, 1, 1, 1, 1, 1, 1, 1, 1, 1, 1, 1, 1, 1, 1, 1, 1, 1, 1, 1, 1, 1, 1, 1, 1, 1, 1, 1, 1, 1, 1, 1, 1, 1, 1, 1, 1, 1, 1, 1, 1, 1, 1, 1, 1, 1, 1, 1, 1, 1, 1, 1, 1, 1, 1, 1, 1, 1, 1, 1, 1, 1, 1, 1, 1, 1, 1, 1, 1, 1, 1, 1, 1, 1, 1, 1, 1, 1, 1, 1, 1, 1, 1, 1, 1, 1, 1, 1, 1, 1, 1, 1, 1, 1, 1, 1, 1, 1, 1, 1, 1, 1, 1, 1, 1, 1, 1, 1, 1, 1, 1, 1, 1, 1, 1, 1, 1, 1, 1, 1, 1, 1, 1, 1, 1, 1, 1, 1, 1, 1, 1, 1, 1, 1, 1, 1, 1, 1, 1, 1, 1, 1, 1, 1, 1, 1, 1, 1, 1, 1, 1, 1, 1, 1, 1, 1, 1, 1, 1, 1, 1, 1, 1, 1, 1, 1, 1, 1, 1, 1, 1, 1, 1, 1, 1, 1, 1, 1, 1, 1, 1, 1, 1, 1, 1, 1, 1, 1, 1, 1, 1, 1, 1, 1, 1, 1, 1, 1, 1, 1, 1, 1, 1, 1, 1, 1, 1, 1, 1, 1, 1, 1, 1, 1, 1, 1, 1, 1, 1, 1, 1, 1, 1, 1, 1, 1, 1, 1, 1, 1, 1, 1, 1, 1, 1, 1, 1, 1, 1, 1, 1, 1, 1, 1, 1, 1, 1, 1, 1, 1, 1, 1, 1, 1, 1, 1, 1, 1, 1, 1, 1, 1, 1, 1, 1, 1, 1, 1, 1, 1, 1, 1, 1, 1, 1, 1, 1, 1, 1, 1, 1, 1, 1, 1, 1, 1, 1, 1, 1, 1, 1, 1, 1, 1, 1, 1, 1, 1, 1, 1, 1, 1, 1, 1, 1, 1, 1, 1, 1, 1, 1, 1, 1, 1, 1, 1, 1, 1, 1, 1, 1, 1, 1, 1, 1, 1, 1, 1, 1, 1, 1, 1, 1, 1, 1, 1, 1, 1, 1, 1, 1, 1, 1, 1, 1, 1, 1, 1, 1, 1, 1, 1, 1, 1, 1, 1, 1, 1, 1, 1, 1, 1, 1, 1, 1, 1, 1, 1, 1, 1, 1, 1, 1, 1, 1, 1, 1, 1, 1, 1, 1, 1, 1, 1, 1, 1, 1, 1, 4 ),
 ( -1.602212253331664948, -1.570796326795749875, -0.6731984257695950991, -0.2243994752565149908, 0.6731984257696440599, 1.570796326795800057, 1.602526412597075067 ),
 ( 0.000000000000000000, 0.4990644329702639825, 0.9981288659405289643, 1.497193298910790116, 1.996257731881059927, 2.994386597821590001, 3.992515463762110084, 4.491579896732379673, 4.990644329702639936, 5.489708762672909970, 5.988773195643170233, 6.986902061583700529, 7.985030927524229938, 8.484095360494489313, 8.983159793464759346, 9.482224226435020498, 9.981288659405290531, 10.97941752534580040, 11.97754639128630139, 12.47661082425659984, 12.97567525722690007, 13.47473969019709905, 13.97380412316740106, 14.97193298910790027, 15.97006185504850073, 16.46912628801869971, 16.96819072098899994, 17.46725515395930017, 17.96631958692950093, 18.96444845286999836, 19.96257731881059883, 20.46164175178079958, 20.96070618475109981, 21.45977061772140004, 21.95883505069160080, 22.95696391663220126, 23.95509278257270225, 24.45415721554289945, 24.95322164851319968, 25.45228608148349991, 25.95135051445370067, 26.94947938039430113, 27.94760824633480212, 28.44667267930509880, 28.94573711227529955, 29.44480154524559978, 29.94386597821590001, 30.94199484415640100, 31.94012371009690199, 32.43918814306720577, 32.93825257603739942, 33.43731700900769965, 33.93638144197799988, 34.93451030791850087, 35.93263917385900186, 36.43170360682930209, 36.93076803979960232, 37.42983247276980308, 37.92889690574009620, 38.92702577168060429, 39.92515463762109817, 40.42421907059139841, 40.92328350356169864, 41.42234793653189939, 41.92141236950219962, 42.91954123544270061, 43.91767010138330107, 44.41673453435349472, 44.91579896732380206, 45.41486340029400282, 45.91392783326430305, 46.91205669920479693, 47.91018556514539739, 48.40924999811559815, 48.90831443108589838, 49.40737886405619861, 49.90644329702639936, 50.90457216296699983, 51.90270102890750081, 52.40176546187770157, 52.90082989484799469, 53.39989432781830203, 53.89895876078850279, 54.89708762672909614, 55.89521649266960424, 56.39428092563989736, 56.89334535861009812, 57.39240979158039835, 57.89147422455069858, 58.88960309049119957, 59.88773195643170055, 60.38679638940200078, 60.88586082237220154, 61.38492525534249467, 61.88398968831280200, 62.88211855425329588, 63.88024742019380398, 64.37931185316409710, 64.87837628613441154, 65.37744071910459809, 65.87650515207489832, 66.87463401801539931, 67.87276288395590029, 68.37182731692620052, 68.87089174989650076, 69.36995618286670151, 69.86902061583700174, 70.86714948177750273, 71.86527834771810319, 72.36434278068828974, 72.86340721365860418, 73.36247164662880493, 73.86153607959910516, 74.85966494553959194, 75.85779381148019240, 76.35685824445040737, 76.85592267742069339, 77.35498711039100783, 77.85405154336119438, 78.85218040930179484, 79.85030927524229583, 80.34937370821249658, 80.84843814118279681, 81.34750257415311125, 81.84656700712329780, 82.84469587306389826, 83.84282473900439925, 84.34188917197469948, 84.84095360494490023, 85.34001803791520047, 85.83908247088550070, 86.83721133682600168, 87.83534020276650267, 88.33440463573680290, 88.83346906870698945, 89.33253350167728968, 89.83159793464760412, 90.82972680058810511, 91.82785566652860609, 92.32692009949890632, 92.82598453246910708, 93.32504896543939310, 93.82411339840969333, 94.82224226435020853, 95.82037113029070952, 96.31943556326099554, 96.81849999623130998, 97.31756442920149652, 97.81662886217179675, 98.81475772811229774, 99.81288659405289820, 100.3119510270229995, 100.8110154599930013, 101.3100798929639978, 101.8091443259339997, 102.8072731918740033, 103.8054020578150016, 104.3044664907849892, 104.8035309237550052, 105.3025953567259876, 105.8016597896960036, 106.7997886556370020, 107.7979175215769914, 108.2969819545470074, 108.7960463875180039, 109.2951108204880057, 109.7941752534579933, 110.7923041193989917, 111.7904329853389953, 112.2894974183089971, 112.7885618512799937, 113.2876262842500097, 113.7866907172199973, 114.7848195831609956, 115.7829484491009993, 116.2820128820720100, 116.7810773150420118, 117.2801417480119994, 117.7792061809820012, 118.7773350469229996, 119.7754639128630032, 120.2745283458339998, 120.7735927788040016, 121.2726572117740034, 121.7717216447440052, 122.7698505106850035, 123.7679793766259877, 124.2670438095959895, 124.7661082425660055, 125.2651726755359931, 125.7642371085070039, 126.7623659744470075, 127.7604948403880059, 128.2595592733580077, 128.7586237063279953, 129.2576881392979828, 129.7567525722689936, 130.7548814382089972, 131.7530103041499956, 132.2520747371200116, 132.7511391700899992, 133.2502036030609815, 133.7492680360309976, 134.7473969019710012, 135.7455257679119995, 136.2445902008820156, 136.7436546338520031, 137.2427190668229855, 137.7417834997930015, 138.7399123657329767, 139.7380412316740035, 140.2371056646440195, 140.7361700976149734, 141.2352345305849894, 141.7342989635550055, 142.7324278294960038, 143.7305566954360074, 144.2296211284059950, 144.7286855613770058, 145.2277499943469934, 145.7268144273169810, 146.7249432932580078, 147.7230721591979830, 148.2221365921679990, 148.7212010251390097, 149.2202654581089973, 149.7193298910789849, 150.7174587570200117, 151.7155876229599869, 152.2146520559309977, 152.7137164889010137, 153.2127809218710013, 153.7118453548409889, 154.7099742207820157, 155.7081030867219908, 156.2071675196930016, 156.7062319526630176, 157.2052963856329768, 157.7043608186039876, 158.7024896845440196, 159.7006185504849896, 160.1996829834550056, 160.6987474164249932, 161.1978118493950092, 161.6968762823659915, 162.6950051483059951, 163.6931340142469935, 164.1921984472169811, 164.6912628801869971, 165.1903273131570131, 165.6893917461279955, 166.6875206120679991, 167.6856494780089974, 168.1847139109789850, 168.6837783439490011, 169.1828427769200118, 169.6819072098899994, 170.6800360758300030, 171.6781649417710014, 172.1772293747409890, 172.6762938077110050, 173.1753582406820158, 173.6744226736520034, 174.6725515395920070, 175.6706804055330053, 176.6688092714740037, 177.1678737044439913, 177.6669381374140073, 178.6650670033550057, 179.6631958692950093, 180.1622603022650253, 180.6613247352360077, 181.1603891682059952, 181.6594536011760113, 182.6575824671170096, 183.6557113330570132, 184.1547757660279956, 184.6538401989979832, 185.1529046319679992, 185.6519690649380152, 186.6500979308789852, 187.6482267968190172, 188.1472912297899995, 188.6463556627599871, 189.1454200957300031, 189.6444845286999907, 190.6426133946409891, 191.6407422605809927, 192.1398066935519751, 192.6388711265219911, 193.1379355594920071, 193.6369999924630179, 194.6351288584029930, 195.6332577243439914, 196.1323221573140074, 196.6313865902839950, 197.1304510232539826, 197.6295154562249934, 198.6276443221649970, 199.6257731881059954, 200.1248376210760114, 200.6239020540459990, 201.1229664870159866, 201.6220309199869973, 202.6201597859270009, 203.6182886518679993, 204.1173530848380153, 204.6164175178080029, 205.1154819507789853, 205.6145463837490013, 206.6126752496890049, 207.6108041156300033, 208.1098685485999908, 208.6089329815700069, 209.1079974145409892, 209.6070618475110052, 210.6051907134520036, 211.6033195793920072, 212.1023840123619948, 212.6014484453330056, 213.1005128783029932, 213.5995773112729808, 214.5977061772140075, 215.5958350431539827, 216.0948994761239987, 216.5939639090950095, 217.0930283420649971, 217.5920927750350131, 218.5902216409760115, 219.5883505069159867, 220.0874149398869974, 220.5864793728569850, 221.0855438058270011, 221.5846082387970171, 222.5827371047380154, 223.5808659706779906, 224.0799304036490014, 224.5789948366189890, 225.0780592695890050, 225.5771237025589926, 226.5752525685000194, 227.5733814344410177, 228.0724458674109769, 228.5715103003809929, 229.0705747333509805, 229.5696391663219913, 230.5677680322619949, 231.5658968982030217, 232.0649613311730093, 232.5640257641429969, 233.0630901971129845, 233.5621546300839952, 234.5602834960239989, 235.5584123619649972, 236.0574767949350132, 236.5565412279050008, 237.0556056608760116, 237.5546700938459992, 238.5527989597860028, 239.5509278257270012, 240.0499922586970172, 240.5490566916670048, 241.0481211246380155, 241.5471855576080031, 242.5453144235479783, 243.5434432894890051, 244.0425077224589927, 244.5415721554290087, 245.0406365884000195, 245.5397010213700071, 246.5378298873109770, 247.5359587532509806, 248.0350231862209966, 248.5340876191920074, 249.0331520521619950, 249.5322164851320110, 250.5303453510730094, 251.5284742170129846, 252.0275386499830006, 252.5266030829539829, 253.0256675159239990, 253.5247319488940150, 254.5228608148350133, 255.5209896807749885, 256.0200541137460277, 256.5191185467160153, 257.0181829796860029, 257.5172474126559905, 258.5153762785969889, 259.5135051445370209, 260.0125695775079748, 260.5116340104780193, 261.0106984434480069, 261.5097628764180513, 262.5078917423589928, 263.5060206082999912, 264.0050850412700356, 264.5041494742399664, 265.0032139072100108, 265.5022783401809647, 266.5004072061209968, 267.4985360720619951, 267.9976005050319827, 268.4966649380020272, 268.9957293709719579, 269.4947938039430255, 270.4929226698830007, 271.4910515358239991, 271.9901159687939867, 272.4891804017639743, 272.9882448347349850, 273.4873092677049726, 274.4854381336450047, 275.4835669995860030, 275.9826314325560475, 276.4816958655259782, 276.9807602984969890, 277.4798247314670334, 278.4779535974070086, 279.4760824633480070, 279.9751468963179946, 280.4742113292880390, 280.9732757622589929, 281.4723401952289805, 282.4704690611699789, 283.4685979271100109, 283.9676623600799985, 284.4667267930510093, 284.9657912260209969, 285.4648556589909845, 286.4629845249319828, 287.4611133908720149, 287.9601778238429688, 288.4592422568130132, 288.9583066897830008, 289.4573711227530453, 290.4554999886939868, 291.4536288546339620, 291.9526932876050296, 292.4517577205749603, 292.9508221535450048, 293.4498865865149924, 294.4480154524559907, 295.4461443183960228, 295.9452087513669767, 296.4442731843370211, 296.9433376173070087, 297.4424020502780195, 298.4405309162180515, 299.4386597821589930, 299.9377242151289806, 300.4367886480989682, 300.9358530810690127, 301.4349175140399666, 302.4330463799799986, 303.4311752459209970, 303.9302396788909846, 304.4293041118610290, 304.9283685448309598, 305.4274329778020274, 306.4255618437420026, 307.4236907096830009, 307.9227551426529885, 308.4218195756230330, 308.9208840085939869, 309.4199484415639745, 310.4180773075040065, 311.4162061734450049, 311.9152706064150493, 312.4143350393849801, 312.9133994723560477, 313.4124639053259784, 314.4105927712660105, 315.4087216372070088, 315.9077860701769964, 316.4068505031480072, 316.9059149361179948, 317.4049793690880392, 318.4031082350289807, 319.4012371009689559, 319.9003015339390004, 320.3993659669100111, 320.8984303998799987, 321.3974948328499863, 322.3956236987909847, 323.3937525647310167, 323.8928169977019706, 324.3918814306720151, 324.8909458636420027, 325.3900102966119903, 326.3881391625530455, 327.3862680284929638, 327.8853324614640314, 328.3843968944339622, 328.8834613274040066, 329.3825257603739942, 330.3806546263149926, 331.3787834922550246, 331.8778479252259785, 332.3769123581960230, 332.8759767911659537, 333.3750412241370213, 334.3731700900769965, 335.3712989560180517, 335.8703633889879825, 336.3694278219579701, 336.8684922549280145, 337.3675566878989684, 338.3656855538390005, 339.3638144197799988, 339.8628788527500433, 340.3619432857199740, 340.8610077186899616, 341.3600721516610292, 342.3582010176010044, 343.3563298835420028, 343.8553943165119904, 344.3544587494820348, 344.8535231824529887, 345.3525876154230332, 346.3507164813629515, 347.3488453473040067, 347.8479097802739943, 348.3469742132439819, 348.8460386462150495, 349.3451030791849803 ),
 .UNSPECIFIED. ) ;
#82208=PLANE ( 'NONE',  #33452 ) ;
#82209=DIRECTION ( 'NONE',  ( 0.000000000000000000, -1.000000000000000000, 0.000000000000000000 ) ) ;
#82210=CARTESIAN_POINT ( 'NONE',  ( 102.0668616197963985, -27.97060589024009047, 180.4898093164620718 ) ) ;
#82211=CIRCLE ( 'NONE', #25641, 2.117000000000007987 ) ;
#82212=ORIENTED_EDGE ( 'NONE', *, *, #61673, .F. ) ;
#82213=ORIENTED_EDGE ( 'NONE', *, *, #60762, .F. ) ;
#82214=CARTESIAN_POINT ( 'NONE',  ( 194.0371591254572650, -24.42818131005417825, 313.9678068554149490 ) ) ;
#82215=PLANE ( 'NONE',  #88394 ) ;
#82216=CARTESIAN_POINT ( 'NONE',  ( 96.80143343076643703, -35.25719154489702589, 222.2251490854339693 ) ) ;
#82217=EDGE_CURVE ( 'NONE', #76316, #65852, #57815, .T. ) ;
#82219=ORIENTED_EDGE ( 'NONE', *, *, #70246, .F. ) ;
#82220=CARTESIAN_POINT ( 'NONE',  ( 104.0406618471960627, -46.06530165129700549, 78.32705384733895926 ) ) ;
#82221=EDGE_CURVE ( 'NONE', #23005, #46468, #50546, .T. ) ;
#82222=CARTESIAN_POINT ( 'NONE',  ( 110.8742435910063051, -45.97612887520801195, 52.88732575667828684 ) ) ;
#82228=ADVANCED_FACE ( 'NONE', ( #10556 ), #37081, .T. ) ;
#82229=ORIENTED_EDGE ( 'NONE', *, *, #29104, .F. ) ;
#82230=ORIENTED_EDGE ( 'NONE', *, *, #24163, .T. ) ;
#82232=CARTESIAN_POINT ( 'NONE',  ( 99.29109958770327182, -40.98052783126505005, 218.1558690201829620 ) ) ;
#82234=CARTESIAN_POINT ( 'NONE',  ( 141.8164832912739826, -9.729447159940995959, 14.92562527591100618 ) ) ;
#82235=LINE ( 'NONE', #19085, #22877 ) ;
#82236=EDGE_CURVE ( 'NONE', #55559, #70423, #58769, .T. ) ;
#82237=CARTESIAN_POINT ( 'NONE',  ( 81.55985452234320121, -39.04079274305795622, 1.981704437692578313 ) ) ;
#82238=VERTEX_POINT ( 'NONE', #79621 ) ;
#82239=CARTESIAN_POINT ( 'NONE',  ( 25.56670390244808289, -42.82844715994167473, 257.2178068554150059 ) ) ;
#82241=ORIENTED_EDGE ( 'NONE', *, *, #62088, .F. ) ;
#82242=CARTESIAN_POINT ( 'NONE',  ( 115.8917813183058740, -31.17956921574393903, 34.27276813305396530 ) ) ;
#82243=ORIENTED_EDGE ( 'NONE', *, *, #86119, .F. ) ;
#82244=CARTESIAN_POINT ( 'NONE',  ( 104.9194883499490061, -28.34545421100826346, 243.1061856076869958 ) ) ;
#82246=CARTESIAN_POINT ( 'NONE',  ( 108.5509251780138271, -26.47246927008487205, 149.9737205140069420 ) ) ;
#82248=DIRECTION ( 'NONE',  ( 0.000000000000000000, 0.000000000000000000, -1.000000000000000000 ) ) ;
#82251=CARTESIAN_POINT ( 'NONE',  ( 110.8324567285566076, -26.28842506301429083, 245.7889586092439629 ) ) ;
#82252=CARTESIAN_POINT ( 'NONE',  ( 107.0664832912739399, -36.72944715994095333, 294.6356252759106837 ) ) ;
#82253=ORIENTED_EDGE ( 'NONE', *, *, #6503, .F. ) ;
#82255=CARTESIAN_POINT ( 'NONE',  ( 99.47006920962783738, -43.93274313109116491, 77.92991099019597812 ) ) ;
#82257=DIRECTION ( 'NONE',  ( 0.000000000000000000, 0.000000000000000000, 1.000000000000000000 ) ) ;
#82258=CIRCLE ( 'NONE', #80824, 2.500000000000002220 ) ;
#82260=VERTEX_POINT ( 'NONE', #23328 ) ;
#82262=DIRECTION ( 'NONE',  ( 0.000000000000000000, 0.000000000000000000, -1.000000000000000000 ) ) ;
#82263=LINE ( 'NONE', #63139, #63101 ) ;
#82264=LINE ( 'NONE', #27272, #62483 ) ;
#82266=CARTESIAN_POINT ( 'NONE',  ( 98.98344471881878803, -35.59181213353920725, 179.0338046553059712 ) ) ;
#82267=CARTESIAN_POINT ( 'NONE',  ( 96.22678813199759418, -34.45212096497557042, 257.1737205140064475 ) ) ;
#82268=CARTESIAN_POINT ( 'NONE',  ( 115.0357021915621090, -42.91043845286343128, 59.30209018972115587 ) ) ;
#82269=ORIENTED_EDGE ( 'NONE', *, *, #73918, .T. ) ;
#82272=AXIS2_PLACEMENT_3D ( 'NONE', #78152, #15912, #17685 ) ;
#82274=ADVANCED_FACE ( 'NONE', ( #31000 ), #9231, .T. ) ;
#82278=CARTESIAN_POINT ( 'NONE',  ( 123.6837132603318992, -56.64645651782490177, 239.5838068554164693 ) ) ;
#82280=EDGE_LOOP ( 'NONE', ( #34, #16857, #58289, #8714 ) ) ;
#82282=CARTESIAN_POINT ( 'NONE',  ( 116.3265979651016409, -32.94445627519164077, 14.13562527591094664 ) ) ;
#82283=ADVANCED_FACE ( 'NONE', ( #36930 ), #24200, .T. ) ;
#82284=DIRECTION ( 'NONE',  ( 0.000000000000000000, 0.000000000000000000, -1.000000000000000000 ) ) ;
#82285=CARTESIAN_POINT ( 'NONE',  ( 72.31648329127402519, -36.72944715994106701, -5.074374724089063982 ) ) ;
#82286=CARTESIAN_POINT ( 'NONE',  ( 116.7432888474544370, -37.52321155953265475, 188.1838483995059619 ) ) ;
#82287=CARTESIAN_POINT ( 'NONE',  ( 117.3100546213214699, -38.89183298362549834, 63.66133956162494911 ) ) ;
#82288=CARTESIAN_POINT ( 'NONE',  ( 141.0664832912740394, -46.72944715994099596, -4.824374724088994704 ) ) ;
#82290=CARTESIAN_POINT ( 'NONE',  ( 73.06670390244801183, -58.72944715994112386, 198.9178068554149945 ) ) ;
#82292=CARTESIAN_POINT ( 'NONE',  ( 113.2442291481427361, -28.75770190614504429, 260.5523025446513543 ) ) ;
#82293=VERTEX_POINT ( 'NONE', #71907 ) ;
#82295=DIRECTION ( 'NONE',  ( -4.237773401492740281E-14, 1.000000000000000000, 0.000000000000000000 ) ) ;
#82296=DIRECTION ( 'NONE',  ( 1.907762142705490052E-15, 7.167082501179359715E-16, -1.000000000000000000 ) ) ;
#82300=EDGE_CURVE ( 'NONE', #33618, #11998, #67467, .T. ) ;
#82301=CARTESIAN_POINT ( 'NONE',  ( 107.6080043092626113, -48.59286871074260006, 42.61276813305398292 ) ) ;
#82304=CARTESIAN_POINT ( 'NONE',  ( 172.5664832912740110, 0.2215528400590013880, 258.9256252759120116 ) ) ;
#82305=CARTESIAN_POINT ( 'NONE',  ( 36.23715912545339535, -47.82818131006131779, 180.4678068554150911 ) ) ;
#82306=CARTESIAN_POINT ( 'NONE',  ( 131.8086190314096484, -17.15582774929994869, 2.518078172612508769 ) ) ;
#82307=VERTEX_POINT ( 'NONE', #37376 ) ;
#82308=CARTESIAN_POINT ( 'NONE',  ( 97.01457192517754891, -36.67423255113659764, 122.3204556863920232 ) ) ;
#82309=DIRECTION ( 'NONE',  ( 0.000000000000000000, 0.000000000000000000, -1.000000000000000000 ) ) ;
#82312=VERTEX_POINT ( 'NONE', #84651 ) ;
#82313=CARTESIAN_POINT ( 'NONE',  ( 115.2242804385497976, -44.22181337150698255, 74.22324432352993995 ) ) ;
#82315=DIRECTION ( 'NONE',  ( 0.7071067811865779928, -0.7071067811865171526, 7.071067811865785947E-16 ) ) ;
#82316=CARTESIAN_POINT ( 'NONE',  ( 51.06648329127400388, 0.2215528400590083269, 333.4006252759110112 ) ) ;
#82317=DIRECTION ( 'NONE',  ( -1.000000000000000000, -4.163336342344333240E-14, 0.000000000000000000 ) ) ;
#82319=AXIS2_PLACEMENT_3D ( 'NONE', #86591, #52898, #18877 ) ;
#82320=DIRECTION ( 'NONE',  ( 0.7071067811865443531, 6.205111755629953205E-16, 0.7071067811865506814 ) ) ;
#82321=EDGE_LOOP ( 'NONE', ( #31980, #71116, #82915, #17545 ) ) ;
#82322=CARTESIAN_POINT ( 'NONE',  ( 102.0112516875887678, -27.67497761899955933, 101.4937205140059575 ) ) ;
#82325=CARTESIAN_POINT ( 'NONE',  ( 105.8960369669305948, -47.10223136823062617, 278.4870538473395527 ) ) ;
#82327=LINE ( 'NONE', #63657, #67849 ) ;
#82328=CARTESIAN_POINT ( 'NONE',  ( 33.78129701732328982, -35.65087443489905183, 193.9678068554150911 ) ) ;
#82329=EDGE_CURVE ( 'NONE', #18476, #75636, #45064, .T. ) ;
#82331=VECTOR ( 'NONE', #52068, 1000.000000000000000 ) ;
#82332=LINE ( 'NONE', #21437, #63666 ) ;
#82335=CARTESIAN_POINT ( 'NONE',  ( 96.72778144249456034, -35.92320320382069099, 191.2765776568639922 ) ) ;
#82336=ORIENTED_EDGE ( 'NONE', *, *, #80766, .F. ) ;
#82338=CARTESIAN_POINT ( 'NONE',  ( 115.6492561437540445, -34.52393389210755004, 120.4587261630399837 ) ) ;
#82339=CARTESIAN_POINT ( 'NONE',  ( 107.0664832912739257, -52.72944715994095333, 357.5272416190308604 ) ) ;
#82340=CARTESIAN_POINT ( 'NONE',  ( 109.8085987287837213, -27.34093086507540704, 255.8499109901960367 ) ) ;
#82341=CARTESIAN_POINT ( 'NONE',  ( 80.06648329127398256, -8.729447159941058132, 1.325625275910934597 ) ) ;
#82342=DIRECTION ( 'NONE',  ( 9.351236661543306751E-17, -3.725950533538267725E-29, -1.000000000000000000 ) ) ;
#82346=CARTESIAN_POINT ( 'NONE',  ( 105.7995184837401155, -26.72403496634397868, 106.1772919428844091 ) ) ;
#82348=ADVANCED_FACE ( 'NONE', ( #8795 ), #36494, .T. ) ;
#82349=CARTESIAN_POINT ( 'NONE',  ( 109.4403364888817123, -25.95778788316468422, 179.8918157521019339 ) ) ;
#82354=CYLINDRICAL_SURFACE ( 'NONE', #67906, 2.030000000001807248 ) ;
#82355=CARTESIAN_POINT ( 'NONE',  ( 100.9550373873344569, -28.70674047333049117, 185.5943939165742336 ) ) ;
#82357=AXIS2_PLACEMENT_3D ( 'NONE', #84770, #15271, #56585 ) ;
#82358=DIRECTION ( 'NONE',  ( 0.000000000000000000, 0.000000000000000000, -1.000000000000000000 ) ) ;
#82361=CARTESIAN_POINT ( 'NONE',  ( 115.4600223225059494, -29.53725764737424342, 229.4022919425779605 ) ) ;
#82362=ORIENTED_EDGE ( 'NONE', *, *, #11974, .F. ) ;
#82364=CARTESIAN_POINT ( 'NONE',  ( 107.0664832912739257, -49.72944715994095333, 311.6343304127839815 ) ) ;
#82366=CARTESIAN_POINT ( 'NONE',  ( 115.2001725772484662, -37.69162533786680314, 51.55094751244793372 ) ) ;
#82367=CARTESIAN_POINT ( 'NONE',  ( 102.6743760996991597, -27.25069970728465307, 176.4213395616249898 ) ) ;
#82369=EDGE_LOOP ( 'NONE', ( #79753, #54731, #65236, #40868 ) ) ;
#82370=AXIS2_PLACEMENT_3D ( 'NONE', #25260, #51175, #31628 ) ;
#82372=CARTESIAN_POINT ( 'NONE',  ( 116.8390257611673917, -34.20685525486396728, 69.02717489141187457 ) ) ;
#82373=ORIENTED_EDGE ( 'NONE', *, *, #3631, .F. ) ;
#82375=AXIS2_PLACEMENT_3D ( 'NONE', #58487, #86217, #23555 ) ;
#82376=VECTOR ( 'NONE', #21542, 999.9999999999998863 ) ;
#82378=EDGE_LOOP ( 'NONE', ( #5700, #55120, #44536, #69486 ) ) ;
#82379=ORIENTED_EDGE ( 'NONE', *, *, #87326, .T. ) ;
#82380=CARTESIAN_POINT ( 'NONE',  ( 30.48091746481831166, -48.32844715994148999, 249.9678068554150059 ) ) ;
#82381=CARTESIAN_POINT ( 'NONE',  ( 116.0261628859374383, -38.04732875056770780, 73.14480078045792766 ) ) ;
#82382=CARTESIAN_POINT ( 'NONE',  ( 118.0640922190486890, -35.40731289736847032, 238.9337205140059552 ) ) ;
#82384=CARTESIAN_POINT ( 'NONE',  ( 108.1794352217186344, -47.07304438381573419, 202.6613395616249704 ) ) ;
#82385=DIRECTION ( 'NONE',  ( -7.723290606088049820E-15, 0.000000000000000000, 1.000000000000000000 ) ) ;
#82386=CARTESIAN_POINT ( 'NONE',  ( 116.7068942081671423, -31.36975501082244477, 25.24229194257798881 ) ) ;
#82387=DIRECTION ( 'NONE',  ( 0.000000000000000000, 1.000000000000000000, 0.000000000000000000 ) ) ;
#82388=CARTESIAN_POINT ( 'NONE',  ( 117.0602913923447090, -38.08470216738429315, 94.71862027038207543 ) ) ;
#82389=AXIS2_PLACEMENT_3D ( 'NONE', #41017, #34206, #29994 ) ;
#82390=VERTEX_POINT ( 'NONE', #85101 ) ;
#82394=AXIS2_PLACEMENT_3D ( 'NONE', #36408, #56820, #46196 ) ;
#82395=CARTESIAN_POINT ( 'NONE',  ( 113.0229309284916752, -28.24065945027244595, 84.57753003781698453 ) ) ;
#82396=CARTESIAN_POINT ( 'NONE',  ( 115.2418052506917832, -44.23790868596334747, 78.22324432352995416 ) ) ;
#82397=CARTESIAN_POINT ( 'NONE',  ( 105.0129988258793645, -25.82091521352475283, 280.2365776568630622 ) ) ;
#82400=CARTESIAN_POINT ( 'NONE',  ( 104.4105186412307944, -25.99981812482467092, 240.2575300378159682 ) ) ;
#82401=DIRECTION ( 'NONE',  ( 3.999999999999999995E-14, -1.000000000000000000, 4.100000000000000342E-29 ) ) ;
#82403=DIRECTION ( 'NONE',  ( 1.000000000000000000, 1.000000000000000078E-15, 1.000000000000000078E-15 ) ) ;
#82404=DIRECTION ( 'NONE',  ( 1.000000000000000000, 1.261617073437676668E-15, 9.462128050782575008E-16 ) ) ;
#82405=CARTESIAN_POINT ( 'NONE',  ( 112.9946529305922667, -31.31372160417125627, 277.6356252759109680 ) ) ;
#82407=CARTESIAN_POINT ( 'NONE',  ( 98.38041226088876101, -41.69525672787395365, 172.7397638099760684 ) ) ;
#82408=CARTESIAN_POINT ( 'NONE',  ( 19.56670390244643443, -25.42844715994203852, 180.4678068554150911 ) ) ;
#82410=EDGE_CURVE ( 'NONE', #58062, #69308, #58839, .T. ) ;
#82411=DIRECTION ( 'NONE',  ( 0.000000000000000000, 0.000000000000000000, -1.000000000000000000 ) ) ;
#82412=DIRECTION ( 'NONE',  ( -4.237773401492740281E-14, 1.000000000000000000, 0.000000000000000000 ) ) ;
#82415=CARTESIAN_POINT ( 'NONE',  ( 101.1598124200938571, -28.84337187651578915, 195.5838068554168672 ) ) ;
#82416=ORIENTED_EDGE ( 'NONE', *, *, #67904, .T. ) ;
#82417=ADVANCED_FACE ( 'NONE', ( #81855 ), #67601, .T. ) ;
#82418=DIRECTION ( 'NONE',  ( -0.7071067811855900054, -0.7071067811875051401, 0.000000000000000000 ) ) ;
#82419=CARTESIAN_POINT ( 'NONE',  ( 107.5109734667377239, -47.16730098390026882, 237.6099109901969655 ) ) ;
#82420=CARTESIAN_POINT ( 'NONE',  ( 97.57126093554219892, -31.07129084365559279, 126.9108633711489915 ) ) ;
#82421=CARTESIAN_POINT ( 'NONE',  ( 117.5348948014565593, -36.80252384088669260, 259.8213395616249386 ) ) ;
#82422=CARTESIAN_POINT ( 'NONE',  ( 97.31584368291662202, -39.30597587107634894, 156.5314585988082285 ) ) ;
#82425=DIRECTION ( 'NONE',  ( -1.000000000000000078E-15, 1.000000000000000083E-30, 1.000000000000000000 ) ) ;
#82426=LINE ( 'NONE', #41054, #32698 ) ;
#82428=CIRCLE ( 'NONE', #43221, 2.999999999999919176 ) ;
#82430=CARTESIAN_POINT ( 'NONE',  ( 131.3164832912739826, -18.72944715994100662, 3.101481641215524832 ) ) ;
#82432=EDGE_LOOP ( 'NONE', ( #74714, #7521, #47130, #3924 ) ) ;
#82433=EDGE_LOOP ( 'NONE', ( #71781, #8117 ) ) ;
#82434=CARTESIAN_POINT ( 'NONE',  ( 98.57243884988349691, -37.62796858414048273, 125.8324198280769650 ) ) ;
#82436=VERTEX_POINT ( 'NONE', #31889 ) ;
#82437=DIRECTION ( 'NONE',  ( -1.000000000000000078E-15, 1.000000000000000083E-30, 1.000000000000000000 ) ) ;
#82438=CARTESIAN_POINT ( 'NONE',  ( 113.9025887763447997, -28.07314977735667938, 120.5565776568639507 ) ) ;
#82439=CARTESIAN_POINT ( 'NONE',  ( 98.30745143774481676, -41.72867539435345208, 147.7403404978439880 ) ) ;
#82443=DIRECTION ( 'NONE',  ( 0.1811243268507065352, -0.9834602067307444129, 0.000000000000000000 ) ) ;
#82444=CARTESIAN_POINT ( 'NONE',  ( 109.7352083718000415, -46.17358189742688523, 72.79562527591099297 ) ) ;
#82446=EDGE_LOOP ( 'NONE', ( #40387, #69584, #27277, #76645 ) ) ;
#82449=VECTOR ( 'NONE', #21399, 1000.000000000000114 ) ;
#82450=CARTESIAN_POINT ( 'NONE',  ( 70.14948329127297200, -1.929447159941395817, 352.4506252759079530 ) ) ;
#82451=CARTESIAN_POINT ( 'NONE',  ( 103.1701080265564912, -27.72257962874998327, 151.4013395616249511 ) ) ;
#82452=CARTESIAN_POINT ( 'NONE',  ( 107.0664832912739683, -24.97944715994095333, 307.1356252759109680 ) ) ;
#82453=LINE ( 'NONE', #75626, #27482 ) ;
#82456=DIRECTION ( 'NONE',  ( 0.000000000000000000, 0.000000000000000000, 1.000000000000000000 ) ) ;
#82459=CARTESIAN_POINT ( 'NONE',  ( 57.56670390244808289, -42.82844715994040286, 257.2178068554150627 ) ) ;
#82462=CARTESIAN_POINT ( 'NONE',  ( 97.24623519876071498, -31.70684325556592853, 95.96229194257799122 ) ) ;
#82464=ORIENTED_EDGE ( 'NONE', *, *, #18573, .F. ) ;
#82469=CIRCLE ( 'NONE', #54792, 2.750000000000002665 ) ;
#82472=DIRECTION ( 'NONE',  ( 0.000000000000000000, 0.000000000000000000, 1.000000000000000000 ) ) ;
#82473=CARTESIAN_POINT ( 'NONE',  ( 115.5869623526398016, -35.21209367091628906, 196.7728522743529425 ) ) ;
#82475=ORIENTED_EDGE ( 'NONE', *, *, #86857, .F. ) ;
#82478=VECTOR ( 'NONE', #83606, 1000.000000000000000 ) ;
#82479=DIRECTION ( 'NONE',  ( 1.000000000000000000, 3.999999999999999995E-14, 1.000000000000000078E-15 ) ) ;
#82480=CARTESIAN_POINT ( 'NONE',  ( 136.4640758026638991, -20.08864647350496924, 2.654395117688020278 ) ) ;
#82482=ORIENTED_EDGE ( 'NONE', *, *, #21486, .T. ) ;
#82484=CARTESIAN_POINT ( 'NONE',  ( 112.2971567814265512, -43.88265157833087926, 224.5101547344679886 ) ) ;
#82487=AXIS2_PLACEMENT_3D ( 'NONE', #24331, #2558, #30259 ) ;
#82489=EDGE_LOOP ( 'NONE', ( #34087, #84682 ) ) ;
#82490=EDGE_LOOP ( 'NONE', ( #25398, #45294, #83090, #82558 ) ) ;
#82491=DIRECTION ( 'NONE',  ( 0.9068632946707807507, -0.4214249218767881500, 1.031805784967618114E-15 ) ) ;
#82492=EDGE_LOOP ( 'NONE', ( #62453, #21708, #64791, #47363 ) ) ;
#82493=B_SPLINE_CURVE_WITH_KNOTS ( 'NONE', 3,
 ( #7559, #13921, #20299, #47065, #6216, #83412, #7111, #76598, #75257, #67988, #14381, #5769, #42056, #35244, #41157, #88892, #54320, #34802, #19836, #13472, #33460, #34350, #20734, #26644, #82089, #41600, #69783, #62953, #48404, #68885 ),
 .UNSPECIFIED., .F., .F.,
 ( 4, 2, 1, 1, 1, 1, 1, 1, 2, 2, 2, 2, 2, 2, 2, 2, 2, 4 ),
 ( 0.5000144061015490138, 0.5001364728969340812, 0.5002585396923192596, 0.5005026732830898384, 0.5009909404646311071, 0.5019674748277139775, 0.5039205435538794964, 0.5078266810062112002, 0.5156389559108744969, 0.5312635057202012012, 0.5625126053388546099, 0.6250108045761610942, 0.6875090038134675785, 0.7500072030507740628, 0.8125054022880805471, 0.8750036015253870314, 0.9375018007626936267, 1.000000000000000000 ),
 .UNSPECIFIED. ) ;
#82495=CARTESIAN_POINT ( 'NONE',  ( 99.99635294717694478, -42.73853927783394369, 224.7052332267339807 ) ) ;
#82496=CARTESIAN_POINT ( 'NONE',  ( 109.0765542020472907, -47.62233732142709641, 127.7337205140059382 ) ) ;
#82497=CARTESIAN_POINT ( 'NONE',  ( 96.05879824974435621, -41.05137697672059716, 96.62419670448197451 ) ) ;
#82498=CARTESIAN_POINT ( 'NONE',  ( 106.1381103904814012, -44.89503369465886351, 249.5838068554170377 ) ) ;
#82499=CARTESIAN_POINT ( 'NONE',  ( 32.16397622746005425, -34.03355364505773650, 342.9256252759109884 ) ) ;
#82500=CARTESIAN_POINT ( 'NONE',  ( 104.4537254180046375, -26.63707460721619213, 196.2784824187679362 ) ) ;
#82502=ORIENTED_EDGE ( 'NONE', *, *, #2639, .F. ) ;
#82504=VERTEX_POINT ( 'NONE', #963 ) ;
#82506=VERTEX_POINT ( 'NONE', #21869 ) ;
#82508=VERTEX_POINT ( 'NONE', #14603 ) ;
#82509=TOROIDAL_SURFACE ( 'NONE', #75230, 13.50000000000000000, 0.5000000000000000000 ) ;
#82510=CARTESIAN_POINT ( 'NONE',  ( 87.31648329127403940, -46.47944715994105280, -5.074374724089048883 ) ) ;
#82512=CARTESIAN_POINT ( 'NONE',  ( 113.3425240358415778, -27.63052414531908596, 89.60800622829195561 ) ) ;
#82514=CARTESIAN_POINT ( 'NONE',  ( 136.7838203269360520, -36.30343833342887905, 6.798133076502122840 ) ) ;
#82515=LINE ( 'NONE', #48385, #20909 ) ;
#82519=CARTESIAN_POINT ( 'NONE',  ( 116.8369567342159456, -40.30247308064090817, 214.5470538473389581 ) ) ;
#82520=FACE_OUTER_BOUND ( 'NONE', #50432, .T. ) ;
#82523=CARTESIAN_POINT ( 'NONE',  ( 97.81252181392954981, -40.51708140501057187, 272.6353344860016819 ) ) ;
#82527=CARTESIAN_POINT ( 'NONE',  ( 41.56648329127398966, -27.57844715994070484, 315.9256252759120116 ) ) ;
#82529=EDGE_CURVE ( 'NONE', #13668, #71916, #76371, .T. ) ;
#82531=CARTESIAN_POINT ( 'NONE',  ( 96.20350199017366322, -34.44722874799195722, 261.1737205140063338 ) ) ;
#82532=ORIENTED_EDGE ( 'NONE', *, *, #3466, .T. ) ;
#82535=CARTESIAN_POINT ( 'NONE',  ( 117.7016330746719035, -39.82606306527180351, 138.5889586092439743 ) ) ;
#82536=CARTESIAN_POINT ( 'NONE',  ( 112.9631696212496905, -28.13226286662721165, 40.59848241876795782 ) ) ;
#82537=CARTESIAN_POINT ( 'NONE',  ( 117.3528398777633299, -34.78421141941176842, 154.9756252759109714 ) ) ;
#82538=LINE ( 'NONE', #7109, #80814 ) ;
#82539=VECTOR ( 'NONE', #67980, 1000.000000000000000 ) ;
#82542=CYLINDRICAL_SURFACE ( 'NONE', #18172, 3.000000000000002665 ) ;
#82543=CARTESIAN_POINT ( 'NONE',  ( 97.06107108305931774, -37.99641184612347189, 191.4272919332322545 ) ) ;
#82545=ORIENTED_EDGE ( 'NONE', *, *, #8262, .T. ) ;
#82549=VERTEX_POINT ( 'NONE', #77273 ) ;
#82550=ORIENTED_EDGE ( 'NONE', *, *, #84700, .T. ) ;
#82551=DIRECTION ( 'NONE',  ( 0.000000000000000000, 0.000000000000000000, -1.000000000000000000 ) ) ;
#82552=CARTESIAN_POINT ( 'NONE',  ( 111.1204619107249556, -46.98756979654999810, 18.88800622829195319 ) ) ;
#82555=CARTESIAN_POINT ( 'NONE',  ( 116.4921925463200552, -40.17707423577839876, 118.5492147079741585 ) ) ;
#82557=CARTESIAN_POINT ( 'NONE',  ( 107.4298862253102698, -45.26314917194000742, 237.0324198280769679 ) ) ;
#82558=ORIENTED_EDGE ( 'NONE', *, *, #46986, .T. ) ;
#82559=AXIS2_PLACEMENT_3D ( 'NONE', #9695, #45087, #72812 ) ;
#82560=ADVANCED_FACE ( 'NONE', ( #49540 ), #6430, .T. ) ;
#82563=CARTESIAN_POINT ( 'NONE',  ( 125.9611475301394847, -14.72944715994102616, 249.5838068554164693 ) ) ;
#82564=DIRECTION ( 'NONE',  ( 1.907762142705490052E-15, 7.167082501179359715E-16, -1.000000000000000000 ) ) ;
#82565=CARTESIAN_POINT ( 'NONE',  ( 37.36643805256732520, -48.62818131006020650, 300.4678068554150059 ) ) ;
#82568=DIRECTION ( 'NONE',  ( 0.000000000000000000, 0.000000000000000000, 1.000000000000000000 ) ) ;
#82569=DIRECTION ( 'NONE',  ( 0.04216478779797398074, -0.9991106698809455455, 0.000000000000000000 ) ) ;
#82570=CARTESIAN_POINT ( 'NONE',  ( 99.85651329992167291, -30.12038005267077878, 275.7356252759109907 ) ) ;
#82572=ORIENTED_EDGE ( 'NONE', *, *, #65994, .T. ) ;
#82575=DIRECTION ( 'NONE',  ( 0.7071067811869263808, -0.7071067811861687646, 7.071067811869270740E-16 ) ) ;
#82576=EDGE_CURVE ( 'NONE', #89264, #9747, #20956, .T. ) ;
#82577=CARTESIAN_POINT ( 'NONE',  ( 36.65249034007441509, -48.32844715994130524, 180.4678068554150911 ) ) ;
#82578=CARTESIAN_POINT ( 'NONE',  ( 102.8730905416367278, -29.69395531543277400, 83.32237608387698913 ) ) ;
#82579=AXIS2_PLACEMENT_3D ( 'NONE', #47198, #75385, #11812 ) ;
#82580=CIRCLE ( 'NONE', #2811, 1.000000000000000888 ) ;
#82581=DIRECTION ( 'NONE',  ( 0.000000000000000000, 0.000000000000000000, -1.000000000000000000 ) ) ;
#82582=CARTESIAN_POINT ( 'NONE',  ( 97.06107109773994068, -37.99641196776861563, 46.42729194290728856 ) ) ;
#82583=ORIENTED_EDGE ( 'NONE', *, *, #45449, .T. ) ;
#82584=CIRCLE ( 'NONE', #15851, 0.5000000000000004441 ) ;
#82585=DIRECTION ( 'NONE',  ( 0.000000000000000000, 1.000000000000000000, 0.000000000000000000 ) ) ;
#82586=VERTEX_POINT ( 'NONE', #49089 ) ;
#82587=CARTESIAN_POINT ( 'NONE',  ( 95.56927879810542947, -39.60255952144336078, 166.5213395616259788 ) ) ;
#82590=CARTESIAN_POINT ( 'NONE',  ( 107.8137748826309377, -27.36365403737595159, 111.4568214011349738 ) ) ;
#82593=DIRECTION ( 'NONE',  ( 1.000000000000000078E-15, -1.000000000000000000, 0.000000000000000000 ) ) ;
#82594=CARTESIAN_POINT ( 'NONE',  ( 109.9169591795599388, -46.81676508990216234, 68.79562527591099297 ) ) ;
#82599=ORIENTED_EDGE ( 'NONE', *, *, #71364, .T. ) ;
#82601=VECTOR ( 'NONE', #87624, 1000.000000000000000 ) ;
#82604=CARTESIAN_POINT ( 'NONE',  ( 106.2788006184939888, -47.06957971430152554, 267.5280062282925542 ) ) ;
#82605=CARTESIAN_POINT ( 'NONE',  ( 113.6281748933624556, -28.60039662530314430, 160.5356252759109736 ) ) ;
#82606=CARTESIAN_POINT ( 'NONE',  ( 163.2449138992999735, -32.11662333284611748, 342.9256252759119548 ) ) ;
#82608=CARTESIAN_POINT ( 'NONE',  ( 106.8411897839350786, -48.57781660025092663, 73.56133956162497611 ) ) ;
#82610=VERTEX_POINT ( 'NONE', #54546 ) ;
#82611=CARTESIAN_POINT ( 'NONE',  ( 97.80792351950141494, -40.51905676813210988, 116.6359120812046939 ) ) ;
#82613=AXIS2_PLACEMENT_3D ( 'NONE', #1680, #64348, #48891 ) ;
#82614=EDGE_CURVE ( 'NONE', #68568, #38559, #54993, .T. ) ;
#82615=ORIENTED_EDGE ( 'NONE', *, *, #47744, .F. ) ;
#82617=CARTESIAN_POINT ( 'NONE',  ( 51.24204729617327558, -31.76306994223702418, 342.9256252759109884 ) ) ;
#82618=CARTESIAN_POINT ( 'NONE',  ( 104.8459308146384643, -26.52976224399699134, 260.2470538473397710 ) ) ;
#82620=EDGE_CURVE ( 'NONE', #89126, #52429, #73370, .T. ) ;
#82624=CARTESIAN_POINT ( 'NONE',  ( 98.95807093800334542, -41.73853705562144967, 11.76800622829293808 ) ) ;
#82625=CARTESIAN_POINT ( 'NONE',  ( 97.44822407315507462, -39.47994946543299477, 101.5486323904540029 ) ) ;
#82626=CARTESIAN_POINT ( 'NONE',  ( 116.5135284680787322, -32.37261310794437463, 100.1699109901969535 ) ) ;
#82628=CARTESIAN_POINT ( 'NONE',  ( 114.2703446987665643, -45.17953892438131192, 153.1508633711489722 ) ) ;
#82629=DIRECTION ( 'NONE',  ( 1.000000000000000000, 4.163336342344333240E-14, 0.000000000000000000 ) ) ;
#82632=EDGE_CURVE ( 'NONE', #38380, #37957, #76292, .T. ) ;
#82633=FACE_BOUND ( 'NONE', #30792, .T. ) ;
#82636=VECTOR ( 'NONE', #69336, 1000.000000000000000 ) ;
#82639=CARTESIAN_POINT ( 'NONE',  ( 95.26177648276406273, -38.28579333248966776, 151.4299109901969871 ) ) ;
#82640=VERTEX_POINT ( 'NONE', #50441 ) ;
#82645=CARTESIAN_POINT ( 'NONE',  ( 194.0667039024479834, -40.32844715993407902, 300.4678068554149490 ) ) ;
#82646=EDGE_LOOP ( 'NONE', ( #51675, #14415, #65768, #49951 ) ) ;
#82651=ORIENTED_EDGE ( 'NONE', *, *, #31190, .F. ) ;
#82652=ORIENTED_EDGE ( 'NONE', *, *, #32316, .T. ) ;
#82653=DIRECTION ( 'NONE',  ( 0.000000000000000000, 0.000000000000000000, -1.000000000000000000 ) ) ;
#82655=CARTESIAN_POINT ( 'NONE',  ( 51.03742451361634380, -23.42844715994068849, 180.4678068554151196 ) ) ;
#82656=EDGE_CURVE ( 'NONE', #78195, #17392, #67539, .T. ) ;
#82657=AXIS2_PLACEMENT_3D ( 'NONE', #64044, #28158, #55845 ) ;
#82660=FACE_OUTER_BOUND ( 'NONE', #3652, .T. ) ;
#82661=ORIENTED_EDGE ( 'NONE', *, *, #32450, .T. ) ;
#82663=CIRCLE ( 'NONE', #75383, 10.00000000000000711 ) ;
#82664=CARTESIAN_POINT ( 'NONE',  ( 107.0664832912739399, -36.72944715994095333, 292.6356252759106837 ) ) ;
#82666=CARTESIAN_POINT ( 'NONE',  ( 115.9419818307743668, -40.91744192719421847, 224.4756252759109714 ) ) ;
#82668=CARTESIAN_POINT ( 'NONE',  ( 103.5129713284350146, -46.47169217660395191, 93.28610146638693834 ) ) ;
#82669=DIRECTION ( 'NONE',  ( 0.000000000000000000, 0.000000000000000000, -1.000000000000000000 ) ) ;
#82670=CARTESIAN_POINT ( 'NONE',  ( 97.33772894284302879, -34.07151874822147875, 22.11475355860416769 ) ) ;
#82671=ORIENTED_EDGE ( 'NONE', *, *, #46285, .F. ) ;
#82674=ORIENTED_EDGE ( 'NONE', *, *, #59704, .T. ) ;
#82675=EDGE_CURVE ( 'NONE', #52659, #83508, #31117, .T. ) ;
#82676=AXIS2_PLACEMENT_3D ( 'NONE', #35963, #13289, #15080 ) ;
#82677=CARTESIAN_POINT ( 'NONE',  ( 21.03689327557705369, -23.42844715994186089, 313.9678068554150059 ) ) ;
#82678=CARTESIAN_POINT ( 'NONE',  ( 101.2699428795238106, -44.12381293138377458, 273.4911071154209594 ) ) ;
#82679=FACE_OUTER_BOUND ( 'NONE', #62964, .T. ) ;
#82681=CARTESIAN_POINT ( 'NONE',  ( 180.3521107875676250, -35.65087443490890706, 342.9256252759109884 ) ) ;
#82683=ORIENTED_EDGE ( 'NONE', *, *, #57215, .T. ) ;
#82684=VECTOR ( 'NONE', #37411, 1000.000000000000000 ) ;
#82686=DIRECTION ( 'NONE',  ( -4.237773401492740281E-14, 1.000000000000000000, 0.000000000000000000 ) ) ;
#82687=ORIENTED_EDGE ( 'NONE', *, *, #38305, .F. ) ;
#82688=CARTESIAN_POINT ( 'NONE',  ( 110.5552498863747246, -46.59121243395724576, 37.84705384733994293 ) ) ;
#82690=CARTESIAN_POINT ( 'NONE',  ( 115.2503885696571047, -36.58558574821132936, 286.6595189410200533 ) ) ;
#82692=CARTESIAN_POINT ( 'NONE',  ( 101.9944482998265158, -45.44656310684662515, 127.1564288467080530 ) ) ;
#82693=CARTESIAN_POINT ( 'NONE',  ( 111.5019814087853831, -26.53443175268781218, 134.7499109901969518 ) ) ;
#82694=EDGE_CURVE ( 'NONE', #68161, #73068, #10024, .T. ) ;
#82696=DIRECTION ( 'NONE',  ( 4.299999999999999979E-14, -1.000000000000000000, 4.400000000000000367E-29 ) ) ;
#82699=CARTESIAN_POINT ( 'NONE',  ( 104.8319786719434603, -26.46567573359534364, 256.2470538473397710 ) ) ;
#82701=CIRCLE ( 'NONE', #63822, 2.517500000000005844 ) ;
#82702=ORIENTED_EDGE ( 'NONE', *, *, #67092, .F. ) ;
#82704=EDGE_LOOP ( 'NONE', ( #30102, #31088, #22156, #53050, #89014 ) ) ;
#82705=CARTESIAN_POINT ( 'NONE',  ( 101.7337754387761635, -26.99498644972499051, 96.46324432352997746 ) ) ;
#82706=CARTESIAN_POINT ( 'NONE',  ( 172.5664832912729878, -27.57844715994070484, 201.9256252759119832 ) ) ;
#82707=ORIENTED_EDGE ( 'NONE', *, *, #30260, .F. ) ;
#82709=ORIENTED_EDGE ( 'NONE', *, *, #55324, .T. ) ;
#82710=AXIS2_PLACEMENT_3D ( 'NONE', #81922, #47357, #62788 ) ;
#82711=CARTESIAN_POINT ( 'NONE',  ( 109.7226905202519873, -27.00022865876807643, 159.8647339765212791 ) ) ;
#82715=DIRECTION ( 'NONE',  ( 0.7071067811868696484, 0.7071067811862253860, 7.071067811868689941E-16 ) ) ;
#82716=CARTESIAN_POINT ( 'NONE',  ( 100.0993174663912697, -32.47640984694866262, 168.7080903695919858 ) ) ;
#82717=CARTESIAN_POINT ( 'NONE',  ( 115.9252781128442535, -30.08061567962537453, 260.3508633711493871 ) ) ;
#82718=CARTESIAN_POINT ( 'NONE',  ( 100.8868427626595690, -44.69971354075113368, 58.05222648633483118 ) ) ;
#82722=PLANE ( 'NONE',  #4118 ) ;
#82723=ORIENTED_EDGE ( 'NONE', *, *, #26955, .T. ) ;
#82725=FACE_BOUND ( 'NONE', #36585, .T. ) ;
#82727=ORIENTED_EDGE ( 'NONE', *, *, #67681, .T. ) ;
#82728=CARTESIAN_POINT ( 'NONE',  ( 162.7866693523280048, -29.62846900982320264, -5.074374724088000832 ) ) ;
#82729=DIRECTION ( 'NONE',  ( -4.237773401492740281E-14, 1.000000000000000000, 0.000000000000000000 ) ) ;
#82730=FACE_OUTER_BOUND ( 'NONE', #26497, .T. ) ;
#82731=LINE ( 'NONE', #20496, #33067 ) ;
#82734=CARTESIAN_POINT ( 'NONE',  ( 112.0552156641497703, -28.39979068407086515, 204.0695626852199496 ) ) ;
#82735=CARTESIAN_POINT ( 'NONE',  ( 110.3859512856231788, -47.32161482583386913, 52.80610146638697699 ) ) ;
#82736=CARTESIAN_POINT ( 'NONE',  ( 123.6837132603319418, -50.82895651782485658, 219.5838068554170093 ) ) ;
#82740=EDGE_CURVE ( 'NONE', #66312, #21358, #60320, .T. ) ;
#82741=VERTEX_POINT ( 'NONE', #58161 ) ;
#82742=CARTESIAN_POINT ( 'NONE',  ( 87.31648329127402519, -54.62589567669624557, 14.92562527591095112 ) ) ;
#82745=DIRECTION ( 'NONE',  ( 9.351236661543306751E-17, -3.725950533538267725E-29, -1.000000000000000000 ) ) ;
#82747=CARTESIAN_POINT ( 'NONE',  ( 112.1253770014904205, -45.36205269762271541, 132.9982990853162903 ) ) ;
#82750=VERTEX_POINT ( 'NONE', #3211 ) ;
#82752=CARTESIAN_POINT ( 'NONE',  ( 103.4695482323410118, -25.41149354249025549, 55.32133956162594046 ) ) ;
#82753=CARTESIAN_POINT ( 'NONE',  ( 113.2448793187668059, -28.75819631133450116, 164.5523540477198026 ) ) ;
#82755=DIRECTION ( 'NONE',  ( 0.000000000000000000, 0.000000000000000000, 1.000000000000000000 ) ) ;
#82756=CARTESIAN_POINT ( 'NONE',  ( 132.2189018279154595, -16.68450975841260941, 2.186797062529802105 ) ) ;
#82760=CARTESIAN_POINT ( 'NONE',  ( 97.56637869462663559, -33.41331154858068686, 122.0570635727724209 ) ) ;
#82761=CARTESIAN_POINT ( 'NONE',  ( 128.2504969244201618, -12.91928723231331588, 394.9756252759100903 ) ) ;
#82763=DIRECTION ( 'NONE',  ( -1.907762142705490052E-15, -7.167082501179359715E-16, 1.000000000000000000 ) ) ;
#82764=VERTEX_POINT ( 'NONE', #58590 ) ;
#82765=CARTESIAN_POINT ( 'NONE',  ( 96.77023068570494502, -38.49705603518268049, 87.46133956162493917 ) ) ;
#82766=CARTESIAN_POINT ( 'NONE',  ( 112.0674640741628707, -45.48753058403565319, 172.9858083296317375 ) ) ;
#82769=VECTOR ( 'NONE', #31323, 999.9999999999998863 ) ;
#82772=CARTESIAN_POINT ( 'NONE',  ( 113.7357275853186280, -44.67049210939290305, 144.1203871806719690 ) ) ;
#82775=ORIENTED_EDGE ( 'NONE', *, *, #31923, .T. ) ;
#82776=CARTESIAN_POINT ( 'NONE',  ( 112.6519946835718144, -45.50616226388157770, 259.0270538473393458 ) ) ;
#82780=CARTESIAN_POINT ( 'NONE',  ( 99.09570909016483142, -30.55043173533305989, 81.80229194078304999 ) ) ;
#82783=CARTESIAN_POINT ( 'NONE',  ( 109.9476544338203325, -26.76763818355050262, 214.8403871806739289 ) ) ;
#82784=VERTEX_POINT ( 'NONE', #78188 ) ;
#82785=ORIENTED_EDGE ( 'NONE', *, *, #61906, .F. ) ;
#82786=EDGE_CURVE ( 'NONE', #25323, #41091, #821, .T. ) ;
#82787=CARTESIAN_POINT ( 'NONE',  ( 105.9222987080832752, -26.72137021301569959, 156.5987261630399701 ) ) ;
#82789=CARTESIAN_POINT ( 'NONE',  ( 105.1480534186857483, -26.53835308478808130, 276.2365776568628917 ) ) ;
#82790=CARTESIAN_POINT ( 'NONE',  ( 79.31510987520702827, -34.05633243510678199, 1.690787911858491421 ) ) ;
#82791=CARTESIAN_POINT ( 'NONE',  ( 46.03715912545348488, -48.62818131006090283, 129.9678068554150911 ) ) ;
#82792=EDGE_CURVE ( 'NONE', #40647, #55396, #22312, .T. ) ;
#82793=VECTOR ( 'NONE', #84194, 1000.000000000000000 ) ;
#82797=DIRECTION ( 'NONE',  ( 0.000000000000000000, 0.000000000000000000, 1.000000000000000000 ) ) ;
#82799=CARTESIAN_POINT ( 'NONE',  ( 107.2427983594548948, -47.16656068249886857, 212.5899109901969837 ) ) ;
#82800=LINE ( 'NONE', #26027, #31530 ) ;
#82802=EDGE_LOOP ( 'NONE', ( #40215, #75096, #87237, #80036 ) ) ;
#82804=CARTESIAN_POINT ( 'NONE',  ( 78.57311110805129317, -16.41810224486967584, 1.981704920694429495 ) ) ;
#82808=VERTEX_POINT ( 'NONE', #8689 ) ;
#82810=CARTESIAN_POINT ( 'NONE',  ( 97.44667640776515327, -32.59970075057101724, 12.00419670448293985 ) ) ;
#82811=CARTESIAN_POINT ( 'NONE',  ( 97.55979742750555772, -43.80499729575070234, 261.8356252759109566 ) ) ;
#82814=CARTESIAN_POINT ( 'NONE',  ( 36.65249034007526063, -48.32844715994123419, 300.4678068554150059 ) ) ;
#82815=CARTESIAN_POINT ( 'NONE',  ( 111.4977754997606780, -45.70022213410786094, 167.9415684329345879 ) ) ;
#82817=CARTESIAN_POINT ( 'NONE',  ( 104.2561231690431782, -27.88649476002280636, 53.13951894101997908 ) ) ;
#82818=CARTESIAN_POINT ( 'NONE',  ( 117.3128790654603080, -34.51798396817098080, 179.9956252759109532 ) ) ;
#82819=VECTOR ( 'NONE', #40395, 1000.000000000000000 ) ;
#82820=AXIS2_PLACEMENT_3D ( 'NONE', #83904, #48889, #63901 ) ;
#82822=ORIENTED_EDGE ( 'NONE', *, *, #11365, .T. ) ;
#82823=CARTESIAN_POINT ( 'NONE',  ( 182.0667039024469886, -33.35206098992630075, -5.074374724088000832 ) ) ;
#82825=VECTOR ( 'NONE', #70331, 1000.000000000000000 ) ;
#82826=VERTEX_POINT ( 'NONE', #25423 ) ;
#82830=DIRECTION ( 'NONE',  ( 0.000000000000000000, 1.000000000000000000, 0.000000000000000000 ) ) ;
#82831=EDGE_CURVE ( 'NONE', #14469, #51166, #45842, .T. ) ;
#82832=CARTESIAN_POINT ( 'NONE',  ( 114.8760577754623569, -30.96046336120327069, 108.7552769709339771 ) ) ;
#82834=CARTESIAN_POINT ( 'NONE',  ( 113.2331319966886412, -45.16264392691098806, 228.0784824187679760 ) ) ;
#82835=CARTESIAN_POINT ( 'NONE',  ( 107.2427983594548948, -47.16656068249886857, 212.5899109901969837 ) ) ;
#82836=CARTESIAN_POINT ( 'NONE',  ( 105.0216744116726630, -25.86700170375123520, 276.2365776568634033 ) ) ;
#82837=PLANE ( 'NONE',  #84778 ) ;
#82838=EDGE_CURVE ( 'NONE', #38868, #51146, #24985, .T. ) ;
#82843=CARTESIAN_POINT ( 'NONE',  ( 99.16769444712198833, -43.44866735504071187, 76.89943479972100704 ) ) ;
#82844=CARTESIAN_POINT ( 'NONE',  ( 118.0351107906133876, -38.43300062509310067, 68.69181575210198787 ) ) ;
#82845=CARTESIAN_POINT ( 'NONE',  ( 118.1498169324930529, -36.11903826555217023, 273.8822919425775808 ) ) ;
#82846=ORIENTED_EDGE ( 'NONE', *, *, #79231, .T. ) ;
#82847=CARTESIAN_POINT ( 'NONE',  ( 105.1109252617814604, -26.48919212138316581, 235.2270538473399313 ) ) ;
#82850=CARTESIAN_POINT ( 'NONE',  ( 115.0365814371429991, -42.90932526432983707, 24.30220417310802716 ) ) ;
#82851=CARTESIAN_POINT ( 'NONE',  ( 194.0667039024480118, -40.32844715993407902, 249.9678068554149775 ) ) ;
#82852=DIRECTION ( 'NONE',  ( 0.000000000000000000, 0.000000000000000000, 1.000000000000000000 ) ) ;
#82853=CARTESIAN_POINT ( 'NONE',  ( 165.9667039024474491, -26.71338133338628751, 237.4678068554150059 ) ) ;
#82854=FACE_OUTER_BOUND ( 'NONE', #52204, .T. ) ;
#82855=LINE ( 'NONE', #63741, #70040 ) ;
#82860=CARTESIAN_POINT ( 'NONE',  ( 41.56648329127398966, -27.57844715994070484, 75.92562527591199739 ) ) ;
#82861=ADVANCED_FACE ( 'NONE', ( #81318 ), #19505, .T. ) ;
#82866=PLANE ( 'NONE',  #46664 ) ;
#82867=CARTESIAN_POINT ( 'NONE',  ( 118.1310582692406257, -36.20923403681121044, 268.8518157521014587 ) ) ;
#82868=CARTESIAN_POINT ( 'NONE',  ( 114.1750726078950890, -45.19361863149571690, 144.1203871806729637 ) ) ;
#82869=CARTESIAN_POINT ( 'NONE',  ( 115.8125398181975783, -30.97623284308500757, 250.2899109901966028 ) ) ;
#82870=CARTESIAN_POINT ( 'NONE',  ( 21.56670390244634561, -23.42844715994195326, 180.4678068554150911 ) ) ;
#82871=DIRECTION ( 'NONE',  ( -0.9825752044165969590, -0.1858654558159821002, 0.000000000000000000 ) ) ;
#82875=CIRCLE ( 'NONE', #4531, 10.00000000000000888 ) ;
#82877=ORIENTED_EDGE ( 'NONE', *, *, #30359, .T. ) ;
#82880=CARTESIAN_POINT ( 'NONE',  ( 103.7755263489600281, -28.29248842296361133, 169.7828960185539415 ) ) ;
#82882=ORIENTED_EDGE ( 'NONE', *, *, #73310, .F. ) ;
#82883=LINE ( 'NONE', #49214, #63433 ) ;
#82884=CARTESIAN_POINT ( 'NONE',  ( 100.8994224252809033, -45.87202276647009569, 148.0918157521009562 ) ) ;
#82885=DIRECTION ( 'NONE',  ( 0.7071067811874264253, -0.7071067811856686092, 7.071067811874271132E-16 ) ) ;
#82886=CARTESIAN_POINT ( 'NONE',  ( 20.56670390244743984, -48.82844715994200158, 180.4678068554150911 ) ) ;
#82888=DIRECTION ( 'NONE',  ( 0.000000000000000000, 0.000000000000000000, 1.000000000000000000 ) ) ;
#82889=DIRECTION ( 'NONE',  ( 0.000000000000000000, 0.000000000000000000, -1.000000000000000000 ) ) ;
#82890=CARTESIAN_POINT ( 'NONE',  ( 98.49710108934563380, -31.94619897774420636, 110.9213395616259703 ) ) ;
#82891=EDGE_LOOP ( 'NONE', ( #53337, #9298, #32466, #75983, #15828 ) ) ;
#82896=CARTESIAN_POINT ( 'NONE',  ( 96.12852455334832769, -38.72269610271986551, 197.4699109901959844 ) ) ;
#82897=LINE ( 'NONE', #46089, #83947 ) ;
#82898=DIRECTION ( 'NONE',  ( 0.7071067811865753283, -0.7071067811865197061, 7.071067811865760309E-16 ) ) ;
#82900=EDGE_CURVE ( 'NONE', #4612, #42888, #25518, .T. ) ;
#82901=CARTESIAN_POINT ( 'NONE',  ( 152.0371591254582881, -47.82818131005588214, 300.4678068554149490 ) ) ;
#82902=FACE_OUTER_BOUND ( 'NONE', #283, .T. ) ;
#82904=CARTESIAN_POINT ( 'NONE',  ( 114.0662423116486082, -44.47333502991310183, 133.1613395616249989 ) ) ;
#82906=VERTEX_POINT ( 'NONE', #26323 ) ;
#82907=VECTOR ( 'NONE', #41143, 1000.000000000000000 ) ;
#82908=ORIENTED_EDGE ( 'NONE', *, *, #74819, .F. ) ;
#82910=DIRECTION ( 'NONE',  ( 1.000000000000000000, 4.163336342344333240E-14, 0.000000000000000000 ) ) ;
#82911=CARTESIAN_POINT ( 'NONE',  ( 92.82872956494375671, -30.11307588647346023, 9.125625275910955736 ) ) ;
#82912=CARTESIAN_POINT ( 'NONE',  ( 112.2491357751623582, -43.66061143999345262, 185.9176141791149917 ) ) ;
#82913=EDGE_CURVE ( 'NONE', #53871, #6226, #10898, .T. ) ;
#82914=CARTESIAN_POINT ( 'NONE',  ( 97.31582012341550580, -39.30591678905398112, 27.53171479399969712 ) ) ;
#82915=ORIENTED_EDGE ( 'NONE', *, *, #67742, .F. ) ;
#82917=EDGE_LOOP ( 'NONE', ( #11082, #78317, #22257, #18394, #56074, #66549 ) ) ;
#82919=PLANE ( 'NONE',  #53414 ) ;
#82920=ORIENTED_EDGE ( 'NONE', *, *, #68658, .T. ) ;
#82921=EDGE_LOOP ( 'NONE', ( #3185, #669, #56796, #44512 ) ) ;
#82922=FACE_OUTER_BOUND ( 'NONE', #39622, .T. ) ;
#82924=CARTESIAN_POINT ( 'NONE',  ( 106.6421946519922983, -45.61100719954815474, 243.9701547344679682 ) ) ;
#82927=VECTOR ( 'NONE', #50885, 1000.000000000000000 ) ;
#82928=CARTESIAN_POINT ( 'NONE',  ( 51.56670390244799762, -33.35206098992650681, -5.074374724088000832 ) ) ;
#82931=ORIENTED_EDGE ( 'NONE', *, *, #53008, .F. ) ;
#82932=AXIS2_PLACEMENT_3D ( 'NONE', #58003, #43013, #1712 ) ;
#82933=DIRECTION ( 'NONE',  ( -1.000000000000000078E-15, 1.000000000000000083E-30, 1.000000000000000000 ) ) ;
#82936=EDGE_CURVE ( 'NONE', #52812, #20444, #38166, .T. ) ;
#82937=CARTESIAN_POINT ( 'NONE',  ( 106.0563433008199752, -28.62948770221197137, 267.9938046553056665 ) ) ;
#82938=CARTESIAN_POINT ( 'NONE',  ( 108.2792694979413568, -26.31707411447196421, 129.9841967044819739 ) ) ;
#82939=CARTESIAN_POINT ( 'NONE',  ( 96.04673288144547882, -37.20790665022158805, 116.3489586092439652 ) ) ;
#82940=CARTESIAN_POINT ( 'NONE',  ( 103.4004682572699920, -43.97339471306070635, 249.5838068554171514 ) ) ;
#82941=CARTESIAN_POINT ( 'NONE',  ( 131.6729728819767047, -17.37149612621589156, 7.198162082950363860 ) ) ;
#82942=CARTESIAN_POINT ( 'NONE',  ( 98.66592356458792779, -30.49631559909255074, 176.8184824187679567 ) ) ;
#82944=EDGE_CURVE ( 'NONE', #35045, #56594, #65856, .T. ) ;
#82945=FACE_OUTER_BOUND ( 'NONE', #83261, .T. ) ;
#82948=ORIENTED_EDGE ( 'NONE', *, *, #36462, .F. ) ;
#82949=VECTOR ( 'NONE', #12621, 1000.000000000000000 ) ;
#82950=ORIENTED_EDGE ( 'NONE', *, *, #9625, .F. ) ;
#82951=LINE ( 'NONE', #35216, #69228 ) ;
#82952=AXIS2_PLACEMENT_3D ( 'NONE', #5438, #60828, #14035 ) ;
#82953=LINE ( 'NONE', #4842, #37447 ) ;
#82955=CARTESIAN_POINT ( 'NONE',  ( 97.74620163809125017, -42.67179083687646823, 141.7661014663869707 ) ) ;
#82957=DIRECTION ( 'NONE',  ( 9.351236661543306751E-17, -3.725950533538267725E-29, -1.000000000000000000 ) ) ;
#82958=DIRECTION ( 'NONE',  ( 0.000000000000000000, -1.000000000000000000, 0.000000000000000000 ) ) ;
#82960=CYLINDRICAL_SURFACE ( 'NONE', #61545, 9.999999999999998224 ) ;
#82961=CARTESIAN_POINT ( 'NONE',  ( 96.21411768969888101, -32.03111041547180804, 207.0013395616249738 ) ) ;
#82962=CARTESIAN_POINT ( 'NONE',  ( 151.0371591254573787, -24.95799193692592866, 249.9678068554149490 ) ) ;
#82964=ORIENTED_EDGE ( 'NONE', *, *, #62995, .F. ) ;
#82965=VECTOR ( 'NONE', #50764, 999.9999999999998863 ) ;
#82966=CARTESIAN_POINT ( 'NONE',  ( 123.0079629938350223, -38.09664315643626509, 247.7440089327910755 ) ) ;
#82970=DIRECTION ( 'NONE',  ( 1.175184669632759901E-16, -1.000000000000000000, -2.000000000000003705E-15 ) ) ;
#82972=EDGE_CURVE ( 'NONE', #79496, #49561, #74477, .T. ) ;
#82973=CARTESIAN_POINT ( 'NONE',  ( 51.56670390244678970, -32.29483332968566600, 117.4678068554150485 ) ) ;
#82974=CARTESIAN_POINT ( 'NONE',  ( 116.1780915764957740, -31.53023347274874055, 289.2384824187680579 ) ) ;
#82977=CARTESIAN_POINT ( 'NONE',  ( 98.13060510664840308, -43.27509626496242134, 106.8175300378159704 ) ) ;
#82978=CARTESIAN_POINT ( 'NONE',  ( 116.3875994391314634, -31.98201348113981268, 40.20133956162496958 ) ) ;
#82979=CARTESIAN_POINT ( 'NONE',  ( 105.7148016331714757, -24.90641244965552659, 156.1670538473399574 ) ) ;
#82980=ADVANCED_FACE ( 'NONE', ( #59035 ), #11806, .T. ) ;
#82984=CARTESIAN_POINT ( 'NONE',  ( 107.0667039024480260, -36.72944715994100306, 199.5838068554169809 ) ) ;
#82985=CARTESIAN_POINT ( 'NONE',  ( 112.1393456646557212, -28.01282279536882669, 189.6564586071203564 ) ) ;
#82987=ORIENTED_EDGE ( 'NONE', *, *, #38990, .F. ) ;
#82990=ORIENTED_EDGE ( 'NONE', *, *, #17970, .F. ) ;
#82992=CARTESIAN_POINT ( 'NONE',  ( 113.4926247784320452, -28.54816540729044405, 75.54705384733995288 ) ) ;
#82993=CARTESIAN_POINT ( 'NONE',  ( 63.03715912545637678, -24.42818131006026761, 193.9678068554150911 ) ) ;
#82995=CARTESIAN_POINT ( 'NONE',  ( 115.0109179074633374, -28.97809521412381883, 190.4537205140059655 ) ) ;
#82996=DIRECTION ( 'NONE',  ( 0.9068632946707805287, -0.4214249218767882055, 9.081056412856297650E-16 ) ) ;
#82998=CARTESIAN_POINT ( 'NONE',  ( 108.8243102715920685, -46.27830423087877421, 277.1438483995053161 ) ) ;
#83001=ORIENTED_EDGE ( 'NONE', *, *, #16064, .F. ) ;
#83002=( GEOMETRIC_REPRESENTATION_CONTEXT ( 3 ) GLOBAL_UNCERTAINTY_ASSIGNED_CONTEXT ( ( #16037 ) ) GLOBAL_UNIT_ASSIGNED_CONTEXT ( ( #48823, #16135, #77013 ) ) REPRESENTATION_CONTEXT ( 'NONE', 'WORKASPACE' ) );
#83003=DIRECTION ( 'NONE',  ( 0.000000000000000000, 0.000000000000000000, -1.000000000000000000 ) ) ;
#83004=CARTESIAN_POINT ( 'NONE',  ( 98.34974946644537397, -31.65678111301215836, 161.9064763829012463 ) ) ;
#83006=CARTESIAN_POINT ( 'NONE',  ( 113.2419700359208434, -28.75597482910771419, 274.5522191157403995 ) ) ;
#83007=CARTESIAN_POINT ( 'NONE',  ( 57.56670390244832447, -48.82844715994039575, 254.7178068554150627 ) ) ;
#83010=DIRECTION ( 'NONE',  ( 1.346944695195362088E-15, -1.000000000000000000, 3.469446951953620425E-31 ) ) ;
#83011=CARTESIAN_POINT ( 'NONE',  ( 97.60228370312334789, -39.19771807597653179, 276.5299109901972088 ) ) ;
#83012=FACE_BOUND ( 'NONE', #3677, .T. ) ;
#83013=CONICAL_SURFACE ( 'NONE', #16284, 11.57110091390439699, 0.7853981633974452814 ) ;
#83015=CARTESIAN_POINT ( 'NONE',  ( 107.0664832912739257, -49.72944715994096043, 312.6356252759112522 ) ) ;
#83016=CARTESIAN_POINT ( 'NONE',  ( 142.8821648370248170, -72.54478064608022692, 396.9756252759102040 ) ) ;
#83017=CARTESIAN_POINT ( 'NONE',  ( 102.2720406957515991, -30.12315877573194101, 73.39380465530592801 ) ) ;
#83020=EDGE_CURVE ( 'NONE', #87481, #8418, #34270, .T. ) ;
#83021=EDGE_CURVE ( 'NONE', #54444, #58766, #66160, .T. ) ;
#83022=CARTESIAN_POINT ( 'NONE',  ( 193.5667039024483529, -48.82844715993410034, 300.4678068554149490 ) ) ;
#83024=CARTESIAN_POINT ( 'NONE',  ( 113.2454986974503015, -28.75867294428107002, 44.55229194263754522 ) ) ;
#83025=ORIENTED_EDGE ( 'NONE', *, *, #26512, .F. ) ;
#83028=CYLINDRICAL_SURFACE ( 'NONE', #67249, 3.000000000000002665 ) ;
#83029=ORIENTED_EDGE ( 'NONE', *, *, #61069, .T. ) ;
#83030=CARTESIAN_POINT ( 'NONE',  ( 116.9043533071046568, -40.17956947857189220, 133.5584824187679658 ) ) ;
#83032=VECTOR ( 'NONE', #25073, 1000.000000000000000 ) ;
#83034=CARTESIAN_POINT ( 'NONE',  ( 104.4081007064180824, -46.45808915210482581, 68.36479194626816991 ) ) ;
#83035=CARTESIAN_POINT ( 'NONE',  ( 115.6173342623064713, -34.29738501013303420, 145.4787261630399371 ) ) ;
#83036=EDGE_CURVE ( 'NONE', #46741, #48304, #71150, .T. ) ;
#83039=CARTESIAN_POINT ( 'NONE',  ( 96.63486483157898022, -37.29388950852173679, 72.36991099019596163 ) ) ;
#83040=ADVANCED_FACE ( 'NONE', ( #77062 ), #15285, .F. ) ;
#83042=VERTEX_POINT ( 'NONE', #75375 ) ;
#83044=ORIENTED_EDGE ( 'NONE', *, *, #79026, .T. ) ;
#83045=ORIENTED_EDGE ( 'NONE', *, *, #80788, .T. ) ;
#83048=CARTESIAN_POINT ( 'NONE',  ( 71.23990787207000608, 10.64204399490126463, 540.9756252759101471 ) ) ;
#83049=ORIENTED_EDGE ( 'NONE', *, *, #54264, .F. ) ;
#83050=CARTESIAN_POINT ( 'NONE',  ( 97.50674219252212538, -32.62548708300529654, 16.00419670448194154 ) ) ;
#83051=CARTESIAN_POINT ( 'NONE',  ( 114.1899296859532171, -45.21130890035909999, 144.1203871806729637 ) ) ;
#83053=LINE ( 'NONE', #48039, #5394 ) ;
#83054=CARTESIAN_POINT ( 'NONE',  ( 101.6782318212999314, -27.07850282373152950, 101.4937205140059575 ) ) ;
#83055=ADVANCED_FACE ( 'NONE', ( #8469 ), #42957, .T. ) ;
#83056=CARTESIAN_POINT ( 'NONE',  ( 97.33810157587271306, -34.07000700935488169, 97.11433392722962310 ) ) ;
#83057=EDGE_LOOP ( 'NONE', ( #53790, #73062 ) ) ;
#83058=CARTESIAN_POINT ( 'NONE',  ( 97.79857776613020803, -40.48525735399483949, 116.6331486142001808 ) ) ;
#83059=CARTESIAN_POINT ( 'NONE',  ( 104.4083119130582702, -46.45815109594069980, 158.3646258352321752 ) ) ;
#83060=ORIENTED_EDGE ( 'NONE', *, *, #15228, .T. ) ;
#83062=DIRECTION ( 'NONE',  ( 0.000000000000000000, 1.000000000000000000, 0.000000000000000000 ) ) ;
#83064=CARTESIAN_POINT ( 'NONE',  ( 114.8195649486642225, -43.69914982757761379, 38.24419670448192221 ) ) ;
#83065=FACE_OUTER_BOUND ( 'NONE', #48375, .T. ) ;
#83068=CARTESIAN_POINT ( 'NONE',  ( 115.6302422591030137, -36.57899571384957937, 288.2638483995053775 ) ) ;
#83070=CARTESIAN_POINT ( 'NONE',  ( 114.7552509866191599, -44.63809267644810319, 114.2022919425779719 ) ) ;
#83071=DIRECTION ( 'NONE',  ( 0.7071067811864666375, 0.7071067811866283970, 7.071067811864659848E-16 ) ) ;
#83072=CARTESIAN_POINT ( 'NONE',  ( 114.2052324763531743, -45.22952987728847063, 148.1203871806719405 ) ) ;
#83073=DIRECTION ( 'NONE',  ( 1.000000000000000000, 4.299999999999999979E-14, 1.000000000000000078E-15 ) ) ;
#83074=VERTEX_POINT ( 'NONE', #35708 ) ;
#83075=CARTESIAN_POINT ( 'NONE',  ( 105.7995771162975416, -24.27178701759104840, 322.4846826458744431 ) ) ;
#83076=FACE_OUTER_BOUND ( 'NONE', #30316, .T. ) ;
#83077=PLANE ( 'NONE',  #20949 ) ;
#83078=ORIENTED_EDGE ( 'NONE', *, *, #33941, .T. ) ;
#83079=AXIS2_PLACEMENT_3D ( 'NONE', #82911, #49701, #21576 ) ;
#83081=DIRECTION ( 'NONE',  ( 0.7071067811873675835, 0.7071067811857274510, 7.071067811873668640E-16 ) ) ;
#83082=CARTESIAN_POINT ( 'NONE',  ( 95.52074050172029729, -39.61468907688732344, 166.5213395616259788 ) ) ;
#83083=ORIENTED_EDGE ( 'NONE', *, *, #42362, .T. ) ;
#83085=CARTESIAN_POINT ( 'NONE',  ( 115.4053350490088548, -30.43652969535880359, 215.3413395616249773 ) ) ;
#83088=DIRECTION ( 'NONE',  ( 0.000000000000000000, 1.000000000000000000, 0.000000000000000000 ) ) ;
#83089=LINE ( 'NONE', #48507, #46704 ) ;
#83090=ORIENTED_EDGE ( 'NONE', *, *, #9001, .T. ) ;
#83092=ORIENTED_EDGE ( 'NONE', *, *, #14837, .T. ) ;
#83093=ORIENTED_EDGE ( 'NONE', *, *, #28078, .F. ) ;
#83095=EDGE_LOOP ( 'NONE', ( #85355, #20306, #81610, #85839 ) ) ;
#83097=CARTESIAN_POINT ( 'NONE',  ( 104.3244243092125032, -26.02173531178284804, 241.2880062282919482 ) ) ;
#83098=DIRECTION ( 'NONE',  ( -0.000000000000000000, 0.000000000000000000, -1.000000000000000000 ) ) ;
#83099=CARTESIAN_POINT ( 'NONE',  ( 135.0807008692694922, -16.17316201338588399, 1.785258157649496136 ) ) ;
#83102=CARTESIAN_POINT ( 'NONE',  ( 107.0664832912739968, -36.72944715994100306, 287.6356252759109680 ) ) ;
#83105=DIRECTION ( 'NONE',  ( 0.000000000000000000, 1.000000000000000000, 0.000000000000000000 ) ) ;
#83107=CARTESIAN_POINT ( 'NONE',  ( 116.7002268312855051, -35.03994406823841246, 239.9641967044819637 ) ) ;
#83108=FACE_OUTER_BOUND ( 'NONE', #12567, .T. ) ;
#83110=CARTESIAN_POINT ( 'NONE',  ( 107.3052971647831697, -26.36210646096938959, 71.04610146638695767 ) ) ;
#83111=CARTESIAN_POINT ( 'NONE',  ( 41.56648329127399677, 0.2215528400590013880, 321.0426252759119734 ) ) ;
#83113=ORIENTED_EDGE ( 'NONE', *, *, #69895, .F. ) ;
#83115=ORIENTED_EDGE ( 'NONE', *, *, #69032, .F. ) ;
#83116=ORIENTED_EDGE ( 'NONE', *, *, #8900, .T. ) ;
#83117=ADVANCED_FACE ( 'NONE', ( #63883 ), #49328, .F. ) ;
#83118=CARTESIAN_POINT ( 'NONE',  ( 84.06648329127399677, -18.82844715994099971, 239.5838068554169809 ) ) ;
#83119=CARTESIAN_POINT ( 'NONE',  ( 101.9834712436270507, -43.98831800240917289, 278.5215833058970247 ) ) ;
#83120=VECTOR ( 'NONE', #45011, 1000.000000000000000 ) ;
#83121=LINE ( 'NONE', #41744, #44351 ) ;
#83122=DIRECTION ( 'NONE',  ( 1.000000000000000000, 4.443626637970152463E-14, 0.000000000000000000 ) ) ;
#83124=ADVANCED_FACE ( 'NONE', ( #62965 ), #33580, .F. ) ;
#83125=CARTESIAN_POINT ( 'NONE',  ( 113.2454987016537302, -28.75867294776266903, 84.55229194220528655 ) ) ;
#83128=CARTESIAN_POINT ( 'NONE',  ( 45.76696975232854925, -48.62818131006087441, 300.4678068554150059 ) ) ;
#83129=EDGE_CURVE ( 'NONE', #72194, #13679, #27019, .T. ) ;
#83130=DIRECTION ( 'NONE',  ( 1.000000000000000000, 4.443626637970137948E-14, 0.000000000000000000 ) ) ;
#83131=VERTEX_POINT ( 'NONE', #1661 ) ;
#83132=CARTESIAN_POINT ( 'NONE',  ( 96.71451373887593661, -37.96385262316839260, 41.42133956162496844 ) ) ;
#83134=CARTESIAN_POINT ( 'NONE',  ( 103.5342718762226895, -27.68543744656516026, 19.79527697093397265 ) ) ;
#83135=ADVANCED_FACE ( 'NONE', ( #28446 ), #1205, .T. ) ;
#83136=CARTESIAN_POINT ( 'NONE',  ( 90.44969454456405344, -20.11243780205715481, 218.0711402470150801 ) ) ;
#83137=CARTESIAN_POINT ( 'NONE',  ( 102.3899016914588458, -28.13915478247111679, 145.4727681330539610 ) ) ;
#83138=DIRECTION ( 'NONE',  ( 9.351236661543306751E-17, -3.725950533538267725E-29, -1.000000000000000000 ) ) ;
#83139=CARTESIAN_POINT ( 'NONE',  ( 32.56670390244700997, -18.82844715994111340, -5.074374724088000832 ) ) ;
#83140=DIRECTION ( 'NONE',  ( 1.000000000000000078E-15, -1.000000000000000083E-30, -1.000000000000000000 ) ) ;
#83142=CARTESIAN_POINT ( 'NONE',  ( 106.1344768297789329, -47.78968505587090476, 258.4975300378158636 ) ) ;
#83143=CARTESIAN_POINT ( 'NONE',  ( 99.97047271725682549, -43.84442383188222436, 116.9535692024431057 ) ) ;
#83145=EDGE_LOOP ( 'NONE', ( #40763, #18343, #38138, #38042, #16429, #477 ) ) ;
#83147=CARTESIAN_POINT ( 'NONE',  ( 180.1667039024476651, -26.71338133338667120, 117.4678068554150627 ) ) ;
#83148=ORIENTED_EDGE ( 'NONE', *, *, #24870, .F. ) ;
#83149=CARTESIAN_POINT ( 'NONE',  ( 114.5987772146603731, -44.05082428708011832, 94.21276813305395592 ) ) ;
#83151=AXIS2_PLACEMENT_3D ( 'NONE', #64167, #1938, #1492 ) ;
#83153=ORIENTED_EDGE ( 'NONE', *, *, #67338, .F. ) ;
#83158=DIRECTION ( 'NONE',  ( 1.000000000000000000, 0.000000000000000000, 0.000000000000000000 ) ) ;
#83160=CARTESIAN_POINT ( 'NONE',  ( 98.44383420958352815, -35.98725590436672661, 184.0642808457819797 ) ) ;
#83161=CARTESIAN_POINT ( 'NONE',  ( 104.5830001944168259, -26.58193179050359589, 281.2670538473395823 ) ) ;
#83162=EDGE_CURVE ( 'NONE', #27981, #58550, #11124, .T. ) ;
#83163=CARTESIAN_POINT ( 'NONE',  ( 97.81311576760518278, -40.52091172574487388, 57.63592544568884790 ) ) ;
#83166=DIRECTION ( 'NONE',  ( 1.000000000000000000, 4.299999999999999979E-14, 1.000000000000000078E-15 ) ) ;
#83167=ORIENTED_EDGE ( 'NONE', *, *, #41193, .T. ) ;
#83169=LINE ( 'NONE', #27735, #1011 ) ;
#83171=DIRECTION ( 'NONE',  ( 0.1811243268507098381, -0.9834602067307437467, 0.000000000000000000 ) ) ;
#83172=CARTESIAN_POINT ( 'NONE',  ( 97.70652731244065592, -40.25122769212212859, 16.61284818632429250 ) ) ;
#83173=DIRECTION ( 'NONE',  ( 1.000000000000000000, 1.000000000000000078E-15, 1.000000000000000078E-15 ) ) ;
#83174=DIRECTION ( 'NONE',  ( -1.000000000000000078E-15, 1.000000000000000000, 0.000000000000000000 ) ) ;
#83175=CARTESIAN_POINT ( 'NONE',  ( 111.9460571495898620, -43.77514521526708080, 202.4809912566479397 ) ) ;
#83176=CARTESIAN_POINT ( 'NONE',  ( 101.1158648436187235, -27.35912039304959009, 65.51467289495799662 ) ) ;
#83177=DIRECTION ( 'NONE',  ( 0.7071067811865789920, -0.7071067811865159314, 0.000000000000000000 ) ) ;
#83178=EDGE_LOOP ( 'NONE', ( #63895, #62611, #37345, #75180 ) ) ;
#83180=LINE ( 'NONE', #20937, #6421 ) ;
#83181=ORIENTED_EDGE ( 'NONE', *, *, #79124, .T. ) ;
#83182=CARTESIAN_POINT ( 'NONE',  ( 116.3259296754763028, -32.93870509136930025, 260.1356252759109680 ) ) ;
#83183=ORIENTED_EDGE ( 'NONE', *, *, #83036, .F. ) ;
#83184=CARTESIAN_POINT ( 'NONE',  ( 113.5222875812157071, -29.01406153566750845, 165.5214312225362789 ) ) ;
#83186=EDGE_CURVE ( 'NONE', #8752, #34742, #43861, .T. ) ;
#83187=CARTESIAN_POINT ( 'NONE',  ( 117.0613444152393754, -38.07727497758394009, 274.7187601539478692 ) ) ;
#83188=AXIS2_PLACEMENT_3D ( 'NONE', #58976, #40330, #74419 ) ;
#83189=CARTESIAN_POINT ( 'NONE',  ( 177.3246001664173264, -48.34074026909179622, 249.9678068554149775 ) ) ;
#83190=ORIENTED_EDGE ( 'NONE', *, *, #49696, .T. ) ;
#83191=CARTESIAN_POINT ( 'NONE',  ( 101.9496561033292039, -27.62096520655628851, 60.48419670448296159 ) ) ;
#83193=CARTESIAN_POINT ( 'NONE',  ( 194.0667039024480118, -40.32844715993407902, 249.9678068554149775 ) ) ;
#83194=LINE ( 'NONE', #48184, #4688 ) ;
#83195=DIRECTION ( 'NONE',  ( 0.000000000000000000, 0.000000000000000000, 1.000000000000000000 ) ) ;
#83200=ORIENTED_EDGE ( 'NONE', *, *, #49092, .T. ) ;
#83202=CARTESIAN_POINT ( 'NONE',  ( 102.3506485400807975, -46.05136549539959390, 123.2041967044829818 ) ) ;
#83204=CARTESIAN_POINT ( 'NONE',  ( 52.65249034007835149, -49.32844715994059470, 249.9678068554150343 ) ) ;
#83207=EDGE_CURVE ( 'NONE', #19003, #62636, #3802, .T. ) ;
#83210=VERTEX_POINT ( 'NONE', #58386 ) ;
#83211=CARTESIAN_POINT ( 'NONE',  ( 108.8662857618680846, -46.94215964495589333, 118.7032443235299723 ) ) ;
#83212=CARTESIAN_POINT ( 'NONE',  ( 141.0667039024479834, -58.72944715994110254, 198.9178068554149945 ) ) ;
#83213=ORIENTED_EDGE ( 'NONE', *, *, #68041, .F. ) ;
#83214=CARTESIAN_POINT ( 'NONE',  ( 116.5166575185068467, -42.41785904284974862, 274.3832443235299365 ) ) ;
#83220=CARTESIAN_POINT ( 'NONE',  ( 109.2168187703261282, -26.58475186820026792, 184.9222919425779708 ) ) ;
#83223=CARTESIAN_POINT ( 'NONE',  ( 116.1908163682739712, -34.48822628859398520, 160.4377737820879588 ) ) ;
#83224=CIRCLE ( 'NONE', #59971, 14.00000000000000888 ) ;
#83226=CARTESIAN_POINT ( 'NONE',  ( 110.7632188227358512, -44.78316835090528514, 24.35015473446894418 ) ) ;
#83228=LINE ( 'NONE', #55930, #17375 ) ;
#83231=CARTESIAN_POINT ( 'NONE',  ( 105.7149878756584798, -46.72378413123163199, 267.4690543908536711 ) ) ;
#83233=CIRCLE ( 'NONE', #44046, 2.750000000000002665 ) ;
#83234=CARTESIAN_POINT ( 'NONE',  ( 115.8254323917787332, -31.73001882841382937, 105.2397919426083206 ) ) ;
#83236=CARTESIAN_POINT ( 'NONE',  ( 188.5667039024479834, -48.82844715994099971, 170.4678068554149775 ) ) ;
#83237=CARTESIAN_POINT ( 'NONE',  ( 102.2473430764596714, -45.94923854148477460, 212.1927681330539599 ) ) ;
#83238=CARTESIAN_POINT ( 'NONE',  ( 97.80895962946385680, -40.51075741989382095, 171.6353300661548928 ) ) ;
#83239=VERTEX_POINT ( 'NONE', #80193 ) ;
#83241=EDGE_CURVE ( 'NONE', #27698, #76097, #11053, .T. ) ;
#83249=CARTESIAN_POINT ( 'NONE',  ( 104.2291421067619694, -46.80627582718438617, 18.35848241876792031 ) ) ;
#83250=CARTESIAN_POINT ( 'NONE',  ( 116.2188219837490522, -41.79507674895632618, 263.4241967044824833 ) ) ;
#83251=ORIENTED_EDGE ( 'NONE', *, *, #32927, .T. ) ;
#83253=CARTESIAN_POINT ( 'NONE',  ( 107.0664832912739968, 19.62155284005901024, 333.4006252759110112 ) ) ;
#83254=DIRECTION ( 'NONE',  ( 0.000000000000000000, 1.000000000000000000, 0.000000000000000000 ) ) ;
#83256=CARTESIAN_POINT ( 'NONE',  ( 111.5243040195562401, -29.85845577577017806, 67.43666179816293038 ) ) ;
#83257=CARTESIAN_POINT ( 'NONE',  ( 117.0378900095125942, -33.61363155034663208, 170.0670538473399631 ) ) ;
#83259=ORIENTED_EDGE ( 'NONE', *, *, #72769, .F. ) ;
#83260=DIRECTION ( 'NONE',  ( 0.000000000000000000, 0.000000000000000000, 1.000000000000000000 ) ) ;
#83261=EDGE_LOOP ( 'NONE', ( #6186, #71798, #85488, #42940 ) ) ;
#83262=ORIENTED_EDGE ( 'NONE', *, *, #34931, .T. ) ;
#83263=VECTOR ( 'NONE', #12014, 1000.000000000000000 ) ;
#83267=CARTESIAN_POINT ( 'NONE',  ( 163.0664832912739826, 19.62155284005901024, 333.4006252759110112 ) ) ;
#83268=AXIS2_PLACEMENT_3D ( 'NONE', #30539, #37351, #77801 ) ;
#83269=CARTESIAN_POINT ( 'NONE',  ( 109.5993548714604060, -44.88669505861042808, 97.23813411379100557 ) ) ;
#83270=CARTESIAN_POINT ( 'NONE',  ( 117.3567523603254159, -34.92480690411444044, 243.9641967044819637 ) ) ;
#83271=CARTESIAN_POINT ( 'NONE',  ( 96.66614461754329568, -36.48121138304695421, 196.3070538473399438 ) ) ;
#83272=CARTESIAN_POINT ( 'NONE',  ( 110.5478855402367913, -46.57039549162846015, 33.84705384733993583 ) ) ;
#83275=ORIENTED_EDGE ( 'NONE', *, *, #64143, .F. ) ;
#83276=ADVANCED_FACE ( 'NONE', ( #3432 ), #17508, .T. ) ;
#83278=CARTESIAN_POINT ( 'NONE',  ( 96.47668441219802560, -40.11591174724604514, 131.5727681330539554 ) ) ;
#83279=CARTESIAN_POINT ( 'NONE',  ( 117.0961560025638306, -31.97355093185684538, 64.19086337114899266 ) ) ;
#83280=CARTESIAN_POINT ( 'NONE',  ( 115.3585040474263508, -45.26590950091470233, 268.1899109901965517 ) ) ;
#83282=ORIENTED_EDGE ( 'NONE', *, *, #36377, .T. ) ;
#83283=CARTESIAN_POINT ( 'NONE',  ( 99.75298236265237506, -29.29979477046331127, 225.6956252759109702 ) ) ;
#83288=CARTESIAN_POINT ( 'NONE',  ( 97.92323840168593563, -40.78071684388427087, 22.65838076743288454 ) ) ;
#83289=CARTESIAN_POINT ( 'NONE',  ( 97.82830680173087501, -40.55783747296570851, 27.63952666306597195 ) ) ;
#83292=CARTESIAN_POINT ( 'NONE',  ( 105.8903942048936386, -25.33046657390624290, 320.7024103198550051 ) ) ;
#83293=CARTESIAN_POINT ( 'NONE',  ( 180.3503142329376487, -29.99615139351623583, 237.4678068554150059 ) ) ;
#83295=DIRECTION ( 'NONE',  ( -0.1858654557293118459, 0.9825752044329915114, 0.000000000000000000 ) ) ;
#83296=FACE_OUTER_BOUND ( 'NONE', #40165, .T. ) ;
#83298=DIRECTION ( 'NONE',  ( 0.000000000000000000, 0.000000000000000000, 1.000000000000000000 ) ) ;
#83299=ORIENTED_EDGE ( 'NONE', *, *, #14198, .T. ) ;
#83301=CARTESIAN_POINT ( 'NONE',  ( 100.2336795655629089, -28.82633655636628589, 260.6441967044821695 ) ) ;
#83302=CARTESIAN_POINT ( 'NONE',  ( 99.42212199502026237, -27.67378918447352731, 146.6356252759109395 ) ) ;
#83303=CARTESIAN_POINT ( 'NONE',  ( 105.7709788128635182, -26.34124963128569163, 266.1756252759109884 ) ) ;
#83304=CARTESIAN_POINT ( 'NONE',  ( 184.5664832912729878, -71.37844715994266664, 361.9756252759109998 ) ) ;
#83306=LINE ( 'NONE', #42388, #44298 ) ;
#83307=CARTESIAN_POINT ( 'NONE',  ( 105.7153723085520056, -46.72384505539759658, 138.4689504240039071 ) ) ;
#83310=ORIENTED_EDGE ( 'NONE', *, *, #68142, .F. ) ;
#83311=DIRECTION ( 'NONE',  ( 0.0001713722456127401463, -0.9999999853157766072, -1.713722456137401502E-19 ) ) ;
#83312=ORIENTED_EDGE ( 'NONE', *, *, #54370, .T. ) ;
#83313=CARTESIAN_POINT ( 'NONE',  ( 100.0898434420045788, -43.48201142159524579, 191.3609912566489584 ) ) ;
#83314=CARTESIAN_POINT ( 'NONE',  ( 115.0340621167422626, -42.91251456256151897, 188.3024629498006846 ) ) ;
#83316=FACE_OUTER_BOUND ( 'NONE', #6674, .T. ) ;
#83317=CARTESIAN_POINT ( 'NONE',  ( 114.2249171546290967, -45.12625265263328345, 149.1508633711489722 ) ) ;
#83320=CARTESIAN_POINT ( 'NONE',  ( 110.1700060600548312, -27.22182654212957331, 85.82575214445022027 ) ) ;
#83323=CARTESIAN_POINT ( 'NONE',  ( 117.2073019650709256, -38.89799087863980276, 108.6708633711499772 ) ) ;
#83324=ORIENTED_EDGE ( 'NONE', *, *, #39995, .F. ) ;
#83325=ORIENTED_EDGE ( 'NONE', *, *, #6716, .F. ) ;
#83326=ORIENTED_EDGE ( 'NONE', *, *, #15782, .T. ) ;
#83327=CARTESIAN_POINT ( 'NONE',  ( 104.8770057419572908, -45.34735396192071732, 43.81015473446897346 ) ) ;
#83329=CARTESIAN_POINT ( 'NONE',  ( 114.5468542906242391, -29.54732804739400365, 185.4232443235299570 ) ) ;
#83331=VECTOR ( 'NONE', #38143, 1000.000000000000000 ) ;
#83333=DIRECTION ( 'NONE',  ( 0.000000000000000000, 1.000000000000000000, 0.000000000000000000 ) ) ;
#83335=CARTESIAN_POINT ( 'NONE',  ( 20.03715912545639100, -24.42818131006202265, 180.4678068554150911 ) ) ;
#83336=CARTESIAN_POINT ( 'NONE',  ( 22.49541547940750519, -78.44951497180814215, 361.9756252759109998 ) ) ;
#83339=CARTESIAN_POINT ( 'NONE',  ( 113.0643619202157879, -28.22920495858469891, 129.5870538473399449 ) ) ;
#83345=DIRECTION ( 'NONE',  ( 2.900000000000000265E-14, -2.000000000000000155E-15, 1.000000000000000000 ) ) ;
#83348=CARTESIAN_POINT ( 'NONE',  ( 100.3081386793954408, -31.32336695771306623, 193.5957094172099744 ) ) ;
#83350=DIRECTION ( 'NONE',  ( 0.000000000000000000, 0.000000000000000000, 1.000000000000000000 ) ) ;
#83351=VECTOR ( 'NONE', #83105, 1000.000000000000000 ) ;
#83354=ORIENTED_EDGE ( 'NONE', *, *, #60023, .T. ) ;
#83355=EDGE_LOOP ( 'NONE', ( #65907, #27208 ) ) ;
#83358=VECTOR ( 'NONE', #69817, 1000.000000000000000 ) ;
#83359=DIRECTION ( 'NONE',  ( 1.000000000000000000, 0.000000000000000000, 0.000000000000000000 ) ) ;
#83360=ORIENTED_EDGE ( 'NONE', *, *, #60188, .T. ) ;
#83361=ORIENTED_EDGE ( 'NONE', *, *, #31128, .F. ) ;
#83363=CARTESIAN_POINT ( 'NONE',  ( 78.92327517541272641, -21.23064218986597851, 8.021355262920510043 ) ) ;
#83364=CARTESIAN_POINT ( 'NONE',  ( 100.6682639674293114, -30.55490919580550013, 247.1472975916109647 ) ) ;
#83366=PLANE ( 'NONE',  #30514 ) ;
#83368=ORIENTED_EDGE ( 'NONE', *, *, #55726, .T. ) ;
#83370=FACE_OUTER_BOUND ( 'NONE', #64273, .T. ) ;
#83371=ORIENTED_EDGE ( 'NONE', *, *, #34709, .T. ) ;
#83372=ORIENTED_EDGE ( 'NONE', *, *, #13761, .T. ) ;
#83374=CARTESIAN_POINT ( 'NONE',  ( 110.0622958990556839, -29.10660024649327227, 267.5966617981628701 ) ) ;
#83375=CARTESIAN_POINT ( 'NONE',  ( 114.7424063621565722, -43.81651770963347303, 123.2327681330539519 ) ) ;
#83376=CARTESIAN_POINT ( 'NONE',  ( 113.8422018911647484, -44.62364141802228090, 108.1413395616249744 ) ) ;
#83377=CARTESIAN_POINT ( 'NONE',  ( 131.5441285970350691, -17.63380991825878397, 7.053480412781381048 ) ) ;
#83378=CARTESIAN_POINT ( 'NONE',  ( 98.89890862997502552, -29.28198419350761483, 226.7261014663869503 ) ) ;
#83379=CYLINDRICAL_SURFACE ( 'NONE', #67521, 27.99999999999999645 ) ;
#83381=EDGE_LOOP ( 'NONE', ( #56382, #6700, #11376, #63691 ) ) ;
#83384=ORIENTED_EDGE ( 'NONE', *, *, #5734, .T. ) ;
#83385=DIRECTION ( 'NONE',  ( 1.000000000000000000, 0.000000000000000000, 9.868649107779159826E-16 ) ) ;
#83387=VECTOR ( 'NONE', #66531, 1000.000000000000000 ) ;
#83389=CARTESIAN_POINT ( 'NONE',  ( 112.1201679527454047, -47.44862423305024635, 137.9270538473389820 ) ) ;
#83393=EDGE_CURVE ( 'NONE', #26931, #30738, #25578, .T. ) ;
#83394=LINE ( 'NONE', #21168, #62340 ) ;
#83397=CARTESIAN_POINT ( 'NONE',  ( 96.69582475441080760, -35.54038568221479011, 202.2356252759109623 ) ) ;
#83398=PLANE ( 'NONE',  #52437 ) ;
#83405=CARTESIAN_POINT ( 'NONE',  ( 99.36439196449877898, -28.73628302914087840, 265.6746728949588032 ) ) ;
#83407=CARTESIAN_POINT ( 'NONE',  ( 114.0075790447407087, -33.88846322102013175, 9.635625275910941312 ) ) ;
#83408=CARTESIAN_POINT ( 'NONE',  ( 97.77451808712464754, -42.75935979880518545, 146.7965776568629508 ) ) ;
#83409=CARTESIAN_POINT ( 'NONE',  ( 96.68599849774213340, -42.44610274171655817, 22.72705384733997391 ) ) ;
#83410=CARTESIAN_POINT ( 'NONE',  ( 108.9530382828359052, -26.39605832486118331, 160.9327681330539690 ) ) ;
#83411=CARTESIAN_POINT ( 'NONE',  ( 113.2454986637468011, -28.75867291636540912, 30.55229194610398480 ) ) ;
#83412=CARTESIAN_POINT ( 'NONE',  ( 97.79820142046531828, -40.48432854127982239, 102.6327809001923157 ) ) ;
#83415=CARTESIAN_POINT ( 'NONE',  ( 102.0670549713190667, -27.97049805303531045, 70.48979194156258643 ) ) ;
#83417=VERTEX_POINT ( 'NONE', #52863 ) ;
#83418=DIRECTION ( 'NONE',  ( 1.000000000000000000, 0.000000000000000000, 0.000000000000000000 ) ) ;
#83420=ORIENTED_EDGE ( 'NONE', *, *, #80945, .T. ) ;
#83421=VERTEX_POINT ( 'NONE', #74261 ) ;
#83423=AXIS2_PLACEMENT_3D ( 'NONE', #72052, #22131, #29829 ) ;
#83424=EDGE_LOOP ( 'NONE', ( #4429, #85064 ) ) ;
#83425=CARTESIAN_POINT ( 'NONE',  ( 97.30890135812539654, -33.12136451854836849, 62.04419670448196911 ) ) ;
#83426=DIRECTION ( 'NONE',  ( -1.000000000000000000, -4.299999999999999979E-14, -1.000000000000000078E-15 ) ) ;
#83427=CARTESIAN_POINT ( 'NONE',  ( 116.9216359643101839, -34.79311186879120044, 118.9822785838860710 ) ) ;
#83429=CARTESIAN_POINT ( 'NONE',  ( 102.0300696065151982, -46.62045497284175610, 168.2137205140059564 ) ) ;
#83431=CARTESIAN_POINT ( 'NONE',  ( 115.6302422591030137, -36.57899571384957937, 288.2638483995053775 ) ) ;
#83432=VERTEX_POINT ( 'NONE', #75149 ) ;
#83433=ORIENTED_EDGE ( 'NONE', *, *, #23070, .F. ) ;
#83434=ORIENTED_EDGE ( 'NONE', *, *, #46905, .F. ) ;
#83436=CARTESIAN_POINT ( 'NONE',  ( 151.5667039024483245, -48.82844715993591223, 300.4678068554149490 ) ) ;
#83437=DIRECTION ( 'NONE',  ( 0.000000000000000000, 0.000000000000000000, -1.000000000000000000 ) ) ;
#83439=CIRCLE ( 'NONE', #35498, 2.030000000002086580 ) ;
#83441=CARTESIAN_POINT ( 'NONE',  ( 72.06648329127401098, -46.72944715994106701, 14.67562527591093513 ) ) ;
#83442=CARTESIAN_POINT ( 'NONE',  ( 51.56670390244699576, -19.82844715994031048, 342.9256252759109884 ) ) ;
#83443=CARTESIAN_POINT ( 'NONE',  ( 128.0667039024480118, -58.35344715994099829, 310.9178068554150514 ) ) ;
#83444=CARTESIAN_POINT ( 'NONE',  ( 118.5467753794659842, -33.90456151647278205, 14.01848241876796308 ) ) ;
#83445=EDGE_CURVE ( 'NONE', #13645, #66334, #40624, .T. ) ;
#83449=DIRECTION ( 'NONE',  ( 0.000000000000000000, 0.000000000000000000, -1.000000000000000000 ) ) ;
#83450=CARTESIAN_POINT ( 'NONE',  ( 109.4870457054322941, -44.52499740455228761, 95.63380465530596553 ) ) ;
#83452=AXIS2_PLACEMENT_3D ( 'NONE', #67863, #33343, #89216 ) ;
#83453=DIRECTION ( 'NONE',  ( 1.000000000000000000, 4.299999999999999979E-14, 1.000000000000000078E-15 ) ) ;
#83454=DIRECTION ( 'NONE',  ( 0.7071067811862279395, -0.7071067811868672059, 7.071067811862286363E-16 ) ) ;
#83455=ORIENTED_EDGE ( 'NONE', *, *, #51616, .T. ) ;
#83456=ORIENTED_EDGE ( 'NONE', *, *, #76897, .F. ) ;
#83458=CARTESIAN_POINT ( 'NONE',  ( 141.8545562996767444, -1.932463243632623229, 361.9756252759100335 ) ) ;
#83459=VERTEX_POINT ( 'NONE', #11592 ) ;
#83463=CARTESIAN_POINT ( 'NONE',  ( 115.5384384484689804, -31.27996107247446744, 140.7130118773259539 ) ) ;
#83464=CARTESIAN_POINT ( 'NONE',  ( 41.56670390244783420, -36.32844715994104234, 249.9678068554150343 ) ) ;
#83465=CARTESIAN_POINT ( 'NONE',  ( 98.84076182955313072, -43.22688528923472262, 87.85848241876792031 ) ) ;
#83466=LINE ( 'NONE', #6709, #986 ) ;
#83467=CIRCLE ( 'NONE', #32689, 0.5000000000000004441 ) ;
#83468=ORIENTED_EDGE ( 'NONE', *, *, #78047, .T. ) ;
#83471=AXIS2_PLACEMENT_3D ( 'NONE', #54573, #46429, #20100 ) ;
#83472=AXIS2_PLACEMENT_3D ( 'NONE', #17636, #3552, #11258 ) ;
#83473=ORIENTED_EDGE ( 'NONE', *, *, #78966, .T. ) ;
#83474=EDGE_LOOP ( 'NONE', ( #78016, #87505, #15334, #22147 ) ) ;
#83476=CARTESIAN_POINT ( 'NONE',  ( 107.0667039024479834, -36.72944715994099596, 239.5838068554170093 ) ) ;
#83477=ORIENTED_EDGE ( 'NONE', *, *, #27423, .F. ) ;
#83478=CARTESIAN_POINT ( 'NONE',  ( 97.18779033502694631, -39.88384928074078317, 281.5603871806734446 ) ) ;
#83479=CARTESIAN_POINT ( 'NONE',  ( 105.3125989252256147, -48.47411034989094958, 143.4584824187689662 ) ) ;
#83482=CARTESIAN_POINT ( 'NONE',  ( 117.8753414029365842, -39.04084647772175032, 104.6708633711489824 ) ) ;
#83483=CARTESIAN_POINT ( 'NONE',  ( 115.0372575151875054, -42.90846255504887097, 263.3022919437246401 ) ) ;
#83484=VERTEX_POINT ( 'NONE', #62850 ) ;
#83486=CARTESIAN_POINT ( 'NONE',  ( 97.81072293460368883, -40.51506560680811475, 116.6357015805674706 ) ) ;
#83487=DIRECTION ( 'NONE',  ( 0.000000000000000000, 1.000000000000000000, 0.000000000000000000 ) ) ;
#83491=CARTESIAN_POINT ( 'NONE',  ( 194.5664832912729878, -81.37844715994266664, 342.9256252759109884 ) ) ;
#83492=CARTESIAN_POINT ( 'NONE',  ( 106.6068369155051698, -25.68554329116653534, 40.09753003781596448 ) ) ;
#83494=AXIS2_PLACEMENT_3D ( 'NONE', #76130, #56112, #63862 ) ;
#83495=ADVANCED_FACE ( 'NONE', ( #56480, #7452 ), #15622, .T. ) ;
#83497=CYLINDRICAL_SURFACE ( 'NONE', #60616, 9.999999999999998224 ) ;
#83498=CARTESIAN_POINT ( 'NONE',  ( 117.5198883494731632, -40.51604253578042858, 23.54991099019792955 ) ) ;
#83499=CARTESIAN_POINT ( 'NONE',  ( 179.7974245136207685, -36.32844715993469720, 313.9678068554149490 ) ) ;
#83500=CARTESIAN_POINT ( 'NONE',  ( 97.63679352021421209, -31.00714225716596673, 121.8803871806729546 ) ) ;
#83501=CARTESIAN_POINT ( 'NONE',  ( 97.81170008160388818, -40.51743097690945916, 72.63551179937353197 ) ) ;
#83502=PLANE ( 'NONE',  #20575 ) ;
#83503=VERTEX_POINT ( 'NONE', #49212 ) ;
#83504=CARTESIAN_POINT ( 'NONE',  ( 53.56670390244749314, -48.82844715994058049, 129.9678068554150911 ) ) ;
#83506=DIRECTION ( 'NONE',  ( 1.000000000000000078E-15, 1.000000000000000083E-30, -1.000000000000000000 ) ) ;
#83507=AXIS2_PLACEMENT_3D ( 'NONE', #59162, #10576, #71490 ) ;
#83508=VERTEX_POINT ( 'NONE', #56019 ) ;
#83510=CARTESIAN_POINT ( 'NONE',  ( 104.5519768891453651, -48.36156025571956718, 182.4070538473399665 ) ) ;
#83511=VERTEX_POINT ( 'NONE', #43294 ) ;
#83513=CARTESIAN_POINT ( 'NONE',  ( 115.8735763837842256, -44.69546008661756531, 229.2413395616249545 ) ) ;
#83514=CARTESIAN_POINT ( 'NONE',  ( 118.0477628396966310, -38.34468641101997122, 69.72229194257801055 ) ) ;
#83517=VECTOR ( 'NONE', #10426, 1000.000000000000000 ) ;
#83518=DIRECTION ( 'NONE',  ( 1.639958061481212836E-42, -4.100000000000000342E-29, -1.000000000000000000 ) ) ;
#83520=EDGE_CURVE ( 'NONE', #75367, #39978, #8354, .T. ) ;
#83527=ORIENTED_EDGE ( 'NONE', *, *, #32941, .F. ) ;
#83528=DIRECTION ( 'NONE',  ( 1.000000000000000078E-15, -1.000000000000000083E-30, -1.000000000000000000 ) ) ;
#83529=CARTESIAN_POINT ( 'NONE',  ( 97.47313694375068849, -40.89946378256092174, 227.6527681330539679 ) ) ;
#83530=LINE ( 'NONE', #55342, #44598 ) ;
#83536=DIRECTION ( 'NONE',  ( 0.000000000000000000, 0.000000000000000000, -1.000000000000000000 ) ) ;
#83537=CARTESIAN_POINT ( 'NONE',  ( 115.6294417704117734, -28.50085323451786579, 39.43562527591099354 ) ) ;
#83538=ORIENTED_EDGE ( 'NONE', *, *, #44176, .F. ) ;
#83540=EDGE_CURVE ( 'NONE', #25056, #49045, #37001, .T. ) ;
#83542=CIRCLE ( 'NONE', #67576, 0.5000000000000004441 ) ;
#83543=VECTOR ( 'NONE', #28578, 1000.000000000000000 ) ;
#83544=LINE ( 'NONE', #82214, #87683 ) ;
#83546=DIRECTION ( 'NONE',  ( -0.7071067811567310901, 0.7071067812163639443, 0.000000000000000000 ) ) ;
#83548=CARTESIAN_POINT ( 'NONE',  ( 116.0161715043949471, -40.67488961668902192, 249.4956252759109532 ) ) ;
#83549=DIRECTION ( 'NONE',  ( 0.000000000000000000, 0.000000000000000000, 1.000000000000000000 ) ) ;
#83550=CARTESIAN_POINT ( 'NONE',  ( 96.75683229781660089, -37.84742820979678868, 77.40038718067299328 ) ) ;
#83551=ADVANCED_FACE ( 'NONE', ( #36050 ), #70124, .F. ) ;
#83553=EDGE_CURVE ( 'NONE', #28392, #8532, #70581, .T. ) ;
#83554=CARTESIAN_POINT ( 'NONE',  ( 97.70650013186612171, -40.25115521776017857, 22.61283738089579742 ) ) ;
#83555=ORIENTED_EDGE ( 'NONE', *, *, #20008, .T. ) ;
#83561=CARTESIAN_POINT ( 'NONE',  ( 116.4296429186904049, -33.01435002197194279, 245.5587261630399780 ) ) ;
#83562=CARTESIAN_POINT ( 'NONE',  ( 115.7831076517189928, -41.80230954316925818, 193.4064586062707463 ) ) ;
#83565=CARTESIAN_POINT ( 'NONE',  ( 71.25502878279074537, -77.59225815239315693, 542.9756252759101471 ) ) ;
#83567=ORIENTED_EDGE ( 'NONE', *, *, #56884, .T. ) ;
#83569=EDGE_CURVE ( 'NONE', #85174, #64215, #5916, .T. ) ;
#83572=CARTESIAN_POINT ( 'NONE',  ( 116.3877942521162936, -31.98191425893181261, 44.20133956162491984 ) ) ;
#83574=ADVANCED_FACE ( 'NONE', ( #24650 ), #57377, .F. ) ;
#83575=CARTESIAN_POINT ( 'NONE',  ( 116.4921678451845111, -34.41013889705870099, 13.44099125664899219 ) ) ;
#83576=EDGE_CURVE ( 'NONE', #56843, #70, #38478, .T. ) ;
#83577=DIRECTION ( 'NONE',  ( -1.000000000000000000, -4.299999999999999979E-14, -1.000000000000000078E-15 ) ) ;
#83578=CARTESIAN_POINT ( 'NONE',  ( 117.2759483237920080, -34.91131378075001379, 198.9546728949589749 ) ) ;
#83579=CARTESIAN_POINT ( 'NONE',  ( 20.03715912545729338, -24.42818131006189830, 313.9678068554150059 ) ) ;
#83580=CARTESIAN_POINT ( 'NONE',  ( 172.5664832912729878, -18.82844715994071194, 78.92562527591199739 ) ) ;
#83581=CARTESIAN_POINT ( 'NONE',  ( 183.6524903400785433, -48.32844715993451956, 180.4678068554150343 ) ) ;
#83584=CARTESIAN_POINT ( 'NONE',  ( 103.0738860297313266, -47.93972279484852095, 248.3041967044829619 ) ) ;
#83586=ORIENTED_EDGE ( 'NONE', *, *, #53939, .T. ) ;
#83587=LINE ( 'NONE', #76761, #41490 ) ;
#83589=CARTESIAN_POINT ( 'NONE',  ( 95.73188602939242742, -40.35408750269280631, 127.5727681330539554 ) ) ;
#83594=VERTEX_POINT ( 'NONE', #2435 ) ;
#83595=CARTESIAN_POINT ( 'NONE',  ( 100.8874677604249115, -44.70022128019346752, 122.0522919302606795 ) ) ;
#83596=CARTESIAN_POINT ( 'NONE',  ( 172.5664832912740110, -9.303447159940999356, 198.9256252759119832 ) ) ;
#83597=LINE ( 'NONE', #35423, #80561 ) ;
#83598=CARTESIAN_POINT ( 'NONE',  ( 57.56670390244819657, -42.82844715994040286, 259.7178068554150627 ) ) ;
#83600=CARTESIAN_POINT ( 'NONE',  ( 110.4730825863185260, -45.36026475776040456, 170.6938046553059678 ) ) ;
#83601=CARTESIAN_POINT ( 'NONE',  ( 100.8354465997397540, -45.15876371340904427, 253.0699109901969450 ) ) ;
#83604=CARTESIAN_POINT ( 'NONE',  ( 123.6837132603319560, -53.34645651782485487, 218.0711402470151370 ) ) ;
#83605=CONICAL_SURFACE ( 'NONE', #28471, 1.624999999999987566, 1.029744258676650093 ) ;
#83606=DIRECTION ( 'NONE',  ( 1.907762142705490052E-15, 7.167082501179359715E-16, -1.000000000000000000 ) ) ;
#83607=ORIENTED_EDGE ( 'NONE', *, *, #28485, .T. ) ;
#83611=LINE ( 'NONE', #62251, #53223 ) ;
#83613=FACE_OUTER_BOUND ( 'NONE', #30352, .T. ) ;
#83614=CARTESIAN_POINT ( 'NONE',  ( 80.06648329127399677, -8.729447159940999512, 2.408125275911999097 ) ) ;
#83615=VECTOR ( 'NONE', #60863, 1000.000000000000000 ) ;
#83616=CARTESIAN_POINT ( 'NONE',  ( 29.56670390244828184, -48.82844715994152551, 300.4678068554150059 ) ) ;
#83617=CARTESIAN_POINT ( 'NONE',  ( 141.8545562996768012, -1.932463243632623229, 394.9756252759100903 ) ) ;
#83618=CARTESIAN_POINT ( 'NONE',  ( 112.4896002948435410, -43.98220334580144453, 187.5219436376009696 ) ) ;
#83619=CARTESIAN_POINT ( 'NONE',  ( 117.6400240572639575, -42.19104337252187520, 93.44705384733897802 ) ) ;
#83621=CYLINDRICAL_SURFACE ( 'NONE', #43703, 11.45913725231036118 ) ;
#83622=ORIENTED_EDGE ( 'NONE', *, *, #72338, .F. ) ;
#83628=CARTESIAN_POINT ( 'NONE',  ( 37.06648329127298780, 12.92155284005730387, 358.9756252759109998 ) ) ;
#83630=CIRCLE ( 'NONE', #6775, 13.44999999999999396 ) ;
#83631=DIRECTION ( 'NONE',  ( 0.000000000000000000, 0.000000000000000000, 1.000000000000000000 ) ) ;
#83632=ORIENTED_EDGE ( 'NONE', *, *, #65061, .T. ) ;
#83633=CARTESIAN_POINT ( 'NONE',  ( 107.8700610081582738, -26.31308374369285730, 70.01562527591099183 ) ) ;
#83634=VECTOR ( 'NONE', #80406, 1000.000000000000000 ) ;
#83635=EDGE_CURVE ( 'NONE', #31632, #11502, #23983, .T. ) ;
#83638=DIRECTION ( 'NONE',  ( 0.7071067811865279218, -0.7071067811865670016, 6.612322855859973915E-17 ) ) ;
#83640=CARTESIAN_POINT ( 'NONE',  ( 132.9233478419694165, -16.22821065591804768, 1.829869330583287157 ) ) ;
#83641=ORIENTED_EDGE ( 'NONE', *, *, #21898, .T. ) ;
#83642=ADVANCED_FACE ( 'NONE', ( #31015 ), #23779, .F. ) ;
#83643=CARTESIAN_POINT ( 'NONE',  ( 192.5667039024472444, -23.42844715993434335, 300.4678068554149490 ) ) ;
#83645=DIRECTION ( 'NONE',  ( -0.1811243269279065315, 0.9834602067165264527, 0.000000000000000000 ) ) ;
#83646=ADVANCED_FACE ( 'NONE', ( #51010 ), #51444, .T. ) ;
#83647=CARTESIAN_POINT ( 'NONE',  ( 114.0008668920709738, -28.09234522576677762, 115.5261014663869474 ) ) ;
#83648=ADVANCED_FACE ( 'NONE', ( #30577 ), #80080, .T. ) ;
#83650=DIRECTION ( 'NONE',  ( 1.000000000000000078E-15, -1.000000000000000083E-30, -1.000000000000000000 ) ) ;
#83655=CARTESIAN_POINT ( 'NONE',  ( 116.2961327041337825, -39.96626766897446714, 129.5584824187679658 ) ) ;
#83656=DIRECTION ( 'NONE',  ( 1.000000000000000078E-15, 0.000000000000000000, -1.000000000000000000 ) ) ;
#83657=EDGE_LOOP ( 'NONE', ( #782, #41204, #10036, #1218 ) ) ;
#83658=CARTESIAN_POINT ( 'NONE',  ( 116.5858064714420976, -40.92601143571967270, 249.4956252759109532 ) ) ;
#83659=DIRECTION ( 'NONE',  ( 0.000000000000000000, 0.000000000000000000, -1.000000000000000000 ) ) ;
#83660=CARTESIAN_POINT ( 'NONE',  ( 130.0664832912740110, -14.47844715994100007, 284.9256252759119548 ) ) ;
#83661=DIRECTION ( 'NONE',  ( 0.000000000000000000, -1.000000000000000000, 0.000000000000000000 ) ) ;
#83664=CARTESIAN_POINT ( 'NONE',  ( 142.8698897858160706, -0.9167816978817300289, 540.9756252759101471 ) ) ;
#83665=LINE ( 'NONE', #27341, #39876 ) ;
#83666=AXIS2_PLACEMENT_3D ( 'NONE', #8868, #79247, #57434 ) ;
#83667=CARTESIAN_POINT ( 'NONE',  ( 113.2764755850018048, -45.03455287549805774, 188.0994347997209672 ) ) ;
#83669=VERTEX_POINT ( 'NONE', #18275 ) ;
#83670=EDGE_CURVE ( 'NONE', #28502, #36969, #40056, .T. ) ;
#83671=CARTESIAN_POINT ( 'NONE',  ( 109.4376220470258119, -28.19094731436911871, 171.2930118773249717 ) ) ;
#83672=VECTOR ( 'NONE', #79285, 1000.000000000000000 ) ;
#83675=CARTESIAN_POINT ( 'NONE',  ( 115.1244435615320612, -31.12738976831575144, 275.3099109901961015 ) ) ;
#83676=CARTESIAN_POINT ( 'NONE',  ( 75.31670390244798341, -67.87844715994100397, 35.51780685541480409 ) ) ;
#83677=CARTESIAN_POINT ( 'NONE',  ( 115.0366439558389544, -42.90924087293481648, 268.3024198942891871 ) ) ;
#83678=CARTESIAN_POINT ( 'NONE',  ( 165.6738106836030227, -28.98061976758901892, 193.9678068554150059 ) ) ;
#83679=CARTESIAN_POINT ( 'NONE',  ( 98.34985890914866502, -31.65658481524367929, 106.9064586097658207 ) ) ;
#83681=CARTESIAN_POINT ( 'NONE',  ( 97.49318720818078532, -40.89074837367932957, 231.6527681330539679 ) ) ;
#83683=ORIENTED_EDGE ( 'NONE', *, *, #25200, .F. ) ;
#83689=FACE_OUTER_BOUND ( 'NONE', #7261, .T. ) ;
#83691=VECTOR ( 'NONE', #62701, 1000.000000000000000 ) ;
#83692=CARTESIAN_POINT ( 'NONE',  ( 80.06648329127399677, -8.350947159940998787, 296.1531252759119752 ) ) ;
#83693=CLOSED_SHELL ( 'NONE', ( #47605, #46929, #58758, #48332 ) ) ;
#83695=CARTESIAN_POINT ( 'NONE',  ( 181.5667039024459939, -18.82844715994031048, -5.074374724088000832 ) ) ;
#83696=CARTESIAN_POINT ( 'NONE',  ( 110.7331673686684610, -26.30186281216086996, 254.8194347997205682 ) ) ;
#83698=CARTESIAN_POINT ( 'NONE',  ( 77.38816033347453072, -37.35482103167625212, 6.853567712192049299 ) ) ;
#83700=CARTESIAN_POINT ( 'NONE',  ( 110.9691608666757219, -45.93657765348226718, 167.8955081847088309 ) ) ;
#83701=CARTESIAN_POINT ( 'NONE',  ( 115.6184857618795121, -38.05767108254817543, 66.50999513149596964 ) ) ;
#83702=CARTESIAN_POINT ( 'NONE',  ( 112.4974222397575545, -26.16880547358812947, 165.6984824187679521 ) ) ;
#83703=DIRECTION ( 'NONE',  ( 1.000000000000000078E-15, -1.000000000000000083E-30, -1.000000000000000000 ) ) ;
#83704=EDGE_LOOP ( 'NONE', ( #71252, #52874, #89105, #71109 ) ) ;
#83705=CARTESIAN_POINT ( 'NONE',  ( 107.0664832912739399, -36.72944715994095333, 293.6369201390379544 ) ) ;
#83709=DIRECTION ( 'NONE',  ( 0.7071067811868657627, 0.7071067811862293828, 7.071067811868650498E-16 ) ) ;
#83714=CARTESIAN_POINT ( 'NONE',  ( 115.6929481903037100, -41.18531195142565338, 92.86956268521994673 ) ) ;
#83715=CARTESIAN_POINT ( 'NONE',  ( 109.9663390834669912, -48.24573355310754152, 242.7727681330539724 ) ) ;
#83716=CARTESIAN_POINT ( 'NONE',  ( 98.45302666770167832, -29.83944080489365902, 195.7775300378159784 ) ) ;
#83717=PLANE ( 'NONE',  #58599 ) ;
#83720=ORIENTED_EDGE ( 'NONE', *, *, #16535, .F. ) ;
#83725=EDGE_CURVE ( 'NONE', #81584, #18119, #33255, .T. ) ;
#83726=CARTESIAN_POINT ( 'NONE',  ( 98.99072789581755671, -31.21169308021397981, 120.8499109901969604 ) ) ;
#83727=CARTESIAN_POINT ( 'NONE',  ( 96.29295924727914269, -41.78513476824832651, 61.67562527591097421 ) ) ;
#83729=CARTESIAN_POINT ( 'NONE',  ( 105.1007409166104054, -25.80476224416663200, 275.2061014663870537 ) ) ;
#83730=VERTEX_POINT ( 'NONE', #63199 ) ;
#83732=CARTESIAN_POINT ( 'NONE',  ( 97.91908366271991326, -41.73065806300744640, 221.7241967044819546 ) ) ;
#83733=PLANE ( 'NONE',  #13788 ) ;
#83734=VECTOR ( 'NONE', #64802, 1000.000000000000000 ) ;
#83736=ADVANCED_FACE ( 'NONE', ( #29136 ), #27332, .F. ) ;
#83737=CARTESIAN_POINT ( 'NONE',  ( 107.9576737208367518, -46.48113836195031467, 277.6356252759107974 ) ) ;
#83738=DIRECTION ( 'NONE',  ( 1.000000000000000000, 4.163336342344333240E-14, 0.000000000000000000 ) ) ;
#83739=CARTESIAN_POINT ( 'NONE',  ( 105.5702964725068114, -25.36820327604221248, 320.9276179173060086 ) ) ;
#83740=EDGE_CURVE ( 'NONE', #49393, #16580, #31219, .T. ) ;
#83741=CARTESIAN_POINT ( 'NONE',  ( 97.81168895331838087, -40.51742574516882200, 9.635625275910941312 ) ) ;
#83743=EDGE_CURVE ( 'NONE', #74068, #67267, #15059, .T. ) ;
#83744=CARTESIAN_POINT ( 'NONE',  ( 130.0664832912740110, -18.72922654876698090, 199.5838068554170093 ) ) ;
#83745=DIRECTION ( 'NONE',  ( 2.050609665440986486E-14, 0.7071067811865465735, 0.7071067811865484609 ) ) ;
#83748=DIRECTION ( 'NONE',  ( 0.000000000000000000, 1.000000000000000000, 0.000000000000000000 ) ) ;
#83749=ORIENTED_EDGE ( 'NONE', *, *, #34291, .T. ) ;
#83750=ADVANCED_FACE ( 'NONE', ( #41835 ), #82, .T. ) ;
#83752=CARTESIAN_POINT ( 'NONE',  ( 116.6260796636124155, -40.94376574832517690, 253.4956252759109532 ) ) ;
#83753=CARTESIAN_POINT ( 'NONE',  ( 102.6161641507259219, -46.84718603934155823, 128.2346728949589760 ) ) ;
#83754=CARTESIAN_POINT ( 'NONE',  ( 100.5371587349295055, -27.78220587661078156, 26.56610146638793779 ) ) ;
#83755=AXIS2_PLACEMENT_3D ( 'NONE', #18863, #39304, #52451 ) ;
#83757=VECTOR ( 'NONE', #44823, 1000.000000000000000 ) ;
#83758=DIRECTION ( 'NONE',  ( 2.279500465453769633E-16, -3.481761372429950061E-31, -1.000000000000000000 ) ) ;
#83760=CARTESIAN_POINT ( 'NONE',  ( 97.83894798970808893, -40.58344824236100834, 137.6413097730125230 ) ) ;
#83763=EDGE_CURVE ( 'NONE', #18132, #1382, #27778, .T. ) ;
#83764=EDGE_LOOP ( 'NONE', ( #72362, #58274 ) ) ;
#83765=CARTESIAN_POINT ( 'NONE',  ( 34.67381068360400320, -28.98061976758901892, 313.9678068554150059 ) ) ;
#83767=EDGE_CURVE ( 'NONE', #85398, #62066, #55459, .T. ) ;
#83768=CARTESIAN_POINT ( 'NONE',  ( 103.7078221352084881, -28.31921139840152435, 174.8133722090289552 ) ) ;
#83770=VERTEX_POINT ( 'NONE', #42731 ) ;
#83772=CARTESIAN_POINT ( 'NONE',  ( 114.5119312840559473, -28.59475203354334027, 150.4746728949579619 ) ) ;
#83773=CARTESIAN_POINT ( 'NONE',  ( 107.0664832912750057, -36.72944715993903486, 4.925625275910970657 ) ) ;
#83774=CARTESIAN_POINT ( 'NONE',  ( 80.06648329127399677, -33.97944715994105991, 8.225625275910942946 ) ) ;
#83777=PLANE ( 'NONE',  #45408 ) ;
#83778=CARTESIAN_POINT ( 'NONE',  ( 112.9285164932676224, -28.85859325239445994, 104.5670538473399347 ) ) ;
#83779=AXIS2_PLACEMENT_3D ( 'NONE', #4919, #26255, #19441 ) ;
#83780=ORIENTED_EDGE ( 'NONE', *, *, #39315, .T. ) ;
#83781=EDGE_LOOP ( 'NONE', ( #74770, #58233, #35004, #74362, #40457, #87007, #12177, #71976 ) ) ;
#83782=ORIENTED_EDGE ( 'NONE', *, *, #33575, .F. ) ;
#83783=CARTESIAN_POINT ( 'NONE',  ( 116.9829645355111154, -34.95910688594825189, 45.39872616303996722 ) ) ;
#83785=CARTESIAN_POINT ( 'NONE',  ( 109.2168187703260998, -26.58475186820039582, 180.9222919425769760 ) ) ;
#83786=CARTESIAN_POINT ( 'NONE',  ( 97.81168731305311326, -40.51740136754563082, 36.63591984386916067 ) ) ;
#83787=CARTESIAN_POINT ( 'NONE',  ( 97.31577621049066806, -39.30573770266337164, 56.53083703567445895 ) ) ;
#83788=DIRECTION ( 'NONE',  ( 1.387778780781444492E-15, 0.000000000000000000, -1.000000000000000000 ) ) ;
#83792=CARTESIAN_POINT ( 'NONE',  ( 98.00553567079148820, -41.84099229931894115, 136.7356252759109623 ) ) ;
#83793=ORIENTED_EDGE ( 'NONE', *, *, #71238, .T. ) ;
#83795=VERTEX_POINT ( 'NONE', #6444 ) ;
#83799=DIRECTION ( 'NONE',  ( 0.000000000000000000, -1.000000000000000000, 0.000000000000000000 ) ) ;
#83802=CARTESIAN_POINT ( 'NONE',  ( 113.2609745038455742, -30.68550774403005121, 192.2718998934009562 ) ) ;
#83803=VECTOR ( 'NONE', #20851, 1000.000000000000000 ) ;
#83805=CYLINDRICAL_SURFACE ( 'NONE', #69695, 13.16666666666669627 ) ;
#83806=CARTESIAN_POINT ( 'NONE',  ( 107.0620278373210255, -36.73691869758540207, 361.9756252759100903 ) ) ;
#83807=VERTEX_POINT ( 'NONE', #20973 ) ;
#83809=ORIENTED_EDGE ( 'NONE', *, *, #56546, .T. ) ;
#83811=CARTESIAN_POINT ( 'NONE',  ( 116.3201542697790529, -32.94256427661516540, 65.13562527591099638 ) ) ;
#83813=ORIENTED_EDGE ( 'NONE', *, *, #35315, .F. ) ;
#83814=CARTESIAN_POINT ( 'NONE',  ( 163.5667039024460223, -18.82844715994111340, 342.9256252759109884 ) ) ;
#83815=CARTESIAN_POINT ( 'NONE',  ( 109.5261983718769585, -46.49778922373468504, 239.2044404487539566 ) ) ;
#83816=CIRCLE ( 'NONE', #35946, 5.599999999999994316 ) ;
#83817=CARTESIAN_POINT ( 'NONE',  ( 108.4179576672466396, -26.73509541248044030, 180.9693683432445823 ) ) ;
#83818=ORIENTED_EDGE ( 'NONE', *, *, #76774, .F. ) ;
#83819=VECTOR ( 'NONE', #84583, 1000.000000000000000 ) ;
#83821=DIRECTION ( 'NONE',  ( -0.7071067812163264188, 0.7071067811567686157, -7.071067812163272297E-16 ) ) ;
#83824=VERTEX_POINT ( 'NONE', #13708 ) ;
#83826=EDGE_CURVE ( 'NONE', #82610, #2655, #84938, .T. ) ;
#83827=DIRECTION ( 'NONE',  ( 0.000000000000000000, 1.000000000000000000, 1.914177628664063178E-15 ) ) ;
#83830=CARTESIAN_POINT ( 'NONE',  ( 106.8863607564096725, -44.89016293055450291, 270.3766617981627860 ) ) ;
#83831=CARTESIAN_POINT ( 'NONE',  ( 96.64877318785802629, -35.94450158219160585, 146.2670538473399517 ) ) ;
#83832=CARTESIAN_POINT ( 'NONE',  ( 102.5676158828201352, -27.34920955258903419, 95.43276813305395478 ) ) ;
#83833=FACE_OUTER_BOUND ( 'NONE', #89071, .T. ) ;
#83834=CARTESIAN_POINT ( 'NONE',  ( 100.6563598938200812, -44.95093154396422364, 228.0499109901969348 ) ) ;
#83836=CARTESIAN_POINT ( 'NONE',  ( 51.23005224011598102, -33.89581943344511217, -5.074374724088000832 ) ) ;
#83837=ORIENTED_EDGE ( 'NONE', *, *, #58202, .T. ) ;
#83839=ORIENTED_EDGE ( 'NONE', *, *, #52344, .T. ) ;
#83840=ORIENTED_EDGE ( 'NONE', *, *, #27657, .F. ) ;
#83841=CARTESIAN_POINT ( 'NONE',  ( 107.0664832912739968, -36.72944715994100306, 294.6356252759106837 ) ) ;
#83843=VECTOR ( 'NONE', #14712, 1000.000000000000000 ) ;
#83844=CARTESIAN_POINT ( 'NONE',  ( 103.2806894308011891, -27.47375879996335613, 136.3854383369816503 ) ) ;
#83846=CARTESIAN_POINT ( 'NONE',  ( 111.7942743463426609, -25.86259492108981206, 134.7499109901969518 ) ) ;
#83847=DIRECTION ( 'NONE',  ( -0.7071067811865774377, 0.7071067811865175967, -7.071067811865470403E-16 ) ) ;
#83851=CARTESIAN_POINT ( 'NONE',  ( 98.03901516409368355, -41.03442269213341120, 56.68020503552938294 ) ) ;
#83852=CARTESIAN_POINT ( 'NONE',  ( 107.5091008941355994, -47.12332782054429714, 233.6099109901969655 ) ) ;
#83856=ORIENTED_EDGE ( 'NONE', *, *, #29622, .F. ) ;
#83857=DIRECTION ( 'NONE',  ( 0.000000000000000000, 0.000000000000000000, 1.000000000000000000 ) ) ;
#83859=CARTESIAN_POINT ( 'NONE',  ( 176.7669697523293735, -48.62818131005481348, 129.9678068554150059 ) ) ;
#83861=CARTESIAN_POINT ( 'NONE',  ( 41.56648329127499153, -27.82844715994070484, 263.6756252759120116 ) ) ;
#83863=CARTESIAN_POINT ( 'NONE',  ( 115.7319096639420906, -42.60456859047142331, 273.3527681330537575 ) ) ;
#83864=ORIENTED_EDGE ( 'NONE', *, *, #51827, .F. ) ;
#83866=CARTESIAN_POINT ( 'NONE',  ( 116.3212776292296127, -32.94146857471318413, 287.6356252759109680 ) ) ;
#83867=CARTESIAN_POINT ( 'NONE',  ( 96.62784866533952766, -37.15519789137512419, 161.3584824187679487 ) ) ;
#83868=CARTESIAN_POINT ( 'NONE',  ( 97.77247047105220190, -32.00675585678803969, 46.95276813305393659 ) ) ;
#83869=CARTESIAN_POINT ( 'NONE',  ( 108.1864281049355867, -47.13803512191609713, 198.6613395616249989 ) ) ;
#83870=AXIS2_PLACEMENT_3D ( 'NONE', #68074, #62595, #20821 ) ;
#83872=CARTESIAN_POINT ( 'NONE',  ( 163.0664832912739826, -8.350947159940998787, 335.9181252759120184 ) ) ;
#83873=DIRECTION ( 'NONE',  ( -4.299999999999999979E-14, 1.000000000000000000, -4.128053709984630540E-29 ) ) ;
#83874=CARTESIAN_POINT ( 'NONE',  ( 29.77381068363597194, -48.62134037875381409, 300.4678068554150059 ) ) ;
#83875=DIRECTION ( 'NONE',  ( -0.7071067811865475727, 0.000000000000000000, -0.7071067811865475727 ) ) ;
#83877=VERTEX_POINT ( 'NONE', #83212 ) ;
#83879=AXIS2_PLACEMENT_3D ( 'NONE', #36046, #29243, #86882 ) ;
#83880=AXIS2_PLACEMENT_3D ( 'NONE', #4424, #87989, #53423 ) ;
#83882=ORIENTED_EDGE ( 'NONE', *, *, #4031, .T. ) ;
#83883=ADVANCED_FACE ( 'NONE', ( #20534 ), #76829, .T. ) ;
#83884=CIRCLE ( 'NONE', #75174, 2.030000000001872529 ) ;
#83887=CARTESIAN_POINT ( 'NONE',  ( 103.4847015977353379, -25.45917443855082496, 51.32133956162493149 ) ) ;
#83888=CARTESIAN_POINT ( 'NONE',  ( 167.6524903400755306, -48.32844715993520879, 180.4678068554150059 ) ) ;
#83889=VECTOR ( 'NONE', #67380, 1000.000000000000000 ) ;
#83890=DIRECTION ( 'NONE',  ( -1.000000000000000000, 0.000000000000000000, 0.000000000000000000 ) ) ;
#83891=CARTESIAN_POINT ( 'NONE',  ( 117.4696809092536256, -30.95150704042223211, 175.2299109901969700 ) ) ;
#83894=CARTESIAN_POINT ( 'NONE',  ( 110.2012955024488718, -28.75291567525416170, 269.2009912566482512 ) ) ;
#83897=ORIENTED_EDGE ( 'NONE', *, *, #87559, .F. ) ;
#83898=ORIENTED_EDGE ( 'NONE', *, *, #36113, .F. ) ;
#83899=CARTESIAN_POINT ( 'NONE',  ( 107.0664832912739541, -36.72944715994095333, 307.1356252759109680 ) ) ;
#83900=DIRECTION ( 'NONE',  ( 0.000000000000000000, 0.000000000000000000, -1.000000000000000000 ) ) ;
#83901=CARTESIAN_POINT ( 'NONE',  ( 105.7990713734985917, -26.72409577044663465, 161.1773275022462144 ) ) ;
#83902=CARTESIAN_POINT ( 'NONE',  ( 97.81477617152367543, -40.51601309134415629, 21.63528831556280707 ) ) ;
#83904=CARTESIAN_POINT ( 'NONE',  ( 179.8608231853569919, -35.55794170701178558, 193.9678068554150059 ) ) ;
#83908=CARTESIAN_POINT ( 'NONE',  ( 97.50674219252212538, -32.62548708300529654, 16.00419670448194154 ) ) ;
#83910=EDGE_LOOP ( 'NONE', ( #84946, #78820, #84576, #63003, #22278, #33972 ) ) ;
#83912=CIRCLE ( 'NONE', #66496, 10.00000000000002487 ) ;
#83913=CARTESIAN_POINT ( 'NONE',  ( 71.24189083761808661, -0.9290567490904538817, 394.9756252759102040 ) ) ;
#83914=EDGE_CURVE ( 'NONE', #62031, #27163, #9451, .T. ) ;
#83915=CARTESIAN_POINT ( 'NONE',  ( 104.1008407059626251, -44.85999997644839254, 95.10428084578198593 ) ) ;
#83916=B_SPLINE_CURVE_WITH_KNOTS ( 'NONE', 3,
 ( #70083, #61141, #25727, #81169, #67502, #5747, #53849, #74777, #19815, #11665, #82064, #28286, #5293, #33437, #88866, #32984, #55979, #53401 ),
 .UNSPECIFIED., .F., .F.,
 ( 4, 2, 2, 2, 2, 2, 2, 2, 4 ),
 ( 0.4999956047813029492, 0.5624961541836400736, 0.6249967035859771425, 0.6874972529883143224, 0.7499978023906515023, 0.8124983517929885712, 0.8749989011953256401, 0.9374994505976628201, 1.000000000000000000 ),
 .UNSPECIFIED. ) ;
#83919=CARTESIAN_POINT ( 'NONE',  ( 102.0670549579451460, -27.97049806049410137, 45.48979194277244886 ) ) ;
#83921=ORIENTED_EDGE ( 'NONE', *, *, #11367, .F. ) ;
#83923=EDGE_LOOP ( 'NONE', ( #75872, #89333, #67384, #18637 ) ) ;
#83924=ORIENTED_EDGE ( 'NONE', *, *, #20860, .F. ) ;
#83925=CARTESIAN_POINT ( 'NONE',  ( 108.4917517584632236, -27.44263408611272936, 141.3749166392299514 ) ) ;
#83926=AXIS2_PLACEMENT_3D ( 'NONE', #66617, #58896, #58458 ) ;
#83927=LINE ( 'NONE', #27598, #28649 ) ;
#83928=CARTESIAN_POINT ( 'NONE',  ( 103.1973475860487639, -46.47157139977531415, 113.2756252759109827 ) ) ;
#83929=LINE ( 'NONE', #43002, #58988 ) ;
#83931=ORIENTED_EDGE ( 'NONE', *, *, #70183, .T. ) ;
#83932=AXIS2_PLACEMENT_3D ( 'NONE', #60420, #81361, #59524 ) ;
#83934=( BOUNDED_CURVE ( )  B_SPLINE_CURVE ( 3, ( #999, #102, #28703, #56838 ),
 .UNSPECIFIED., .F., .T. ) 
 B_SPLINE_CURVE_WITH_KNOTS ( ( 4, 4 ),
 ( 4.777055387349745885, 4.778685762418977134 ),
 .UNSPECIFIED. ) 
 CURVE ( )  GEOMETRIC_REPRESENTATION_ITEM ( )  RATIONAL_B_SPLINE_CURVE ( ( 1.000000000000000000, 0.9999997784897733943, 0.9999997784897733943, 1.000000000000000000 ) ) 
 REPRESENTATION_ITEM ( '' )  );
#83936=ORIENTED_EDGE ( 'NONE', *, *, #42183, .T. ) ;
#83937=VECTOR ( 'NONE', #44231, 1000.000000000000000 ) ;
#83939=ORIENTED_EDGE ( 'NONE', *, *, #68360, .F. ) ;
#83940=CARTESIAN_POINT ( 'NONE',  ( 102.7643194828038276, -25.71402177940525746, 20.37276813305294354 ) ) ;
#83941=CARTESIAN_POINT ( 'NONE',  ( 117.0891209002388678, -39.67630891660421355, 179.5984824187679294 ) ) ;
#83942=CARTESIAN_POINT ( 'NONE',  ( 41.56648329127399677, -18.82844715994099971, 21.04262527591200183 ) ) ;
#83944=CARTESIAN_POINT ( 'NONE',  ( 96.69923704014651378, -37.82612059164544860, 122.4099109901969626 ) ) ;
#83945=CARTESIAN_POINT ( 'NONE',  ( 63.03715912545818156, -46.82818131006018092, 313.9678068554150059 ) ) ;
#83947=VECTOR ( 'NONE', #25668, 1000.000000000000000 ) ;
#83948=CARTESIAN_POINT ( 'NONE',  ( 138.8167039024479834, -67.87844715994100397, 63.03480685541479289 ) ) ;
#83950=CARTESIAN_POINT ( 'NONE',  ( 117.0717238224210917, -35.46104157321313011, 134.9276073507514013 ) ) ;
#83951=VERTEX_POINT ( 'NONE', #15512 ) ;
#83952=CYLINDRICAL_SURFACE ( 'NONE', #59077, 0.2500000000000039968 ) ;
#83954=CARTESIAN_POINT ( 'NONE',  ( 104.2408938701987040, -46.76453939261368475, 22.35848241876792031 ) ) ;
#83956=DIRECTION ( 'NONE',  ( -1.000000000000000078E-15, 0.000000000000000000, 1.000000000000000000 ) ) ;
#83957=CARTESIAN_POINT ( 'NONE',  ( 180.3503142329310265, -29.99615139349890569, -5.074374724088000832 ) ) ;
#83958=CARTESIAN_POINT ( 'NONE',  ( 115.5964019700117973, -42.63146254436634308, 13.35657765686398868 ) ) ;
#83959=CARTESIAN_POINT ( 'NONE',  ( 97.75853391132390868, -40.38526537496221636, 111.6242890961639773 ) ) ;
#83960=CARTESIAN_POINT ( 'NONE',  ( 113.3182355088850386, -45.04474967211692160, 139.0899109901969553 ) ) ;
#83962=FACE_BOUND ( 'NONE', #57406, .T. ) ;
#83964=AXIS2_PLACEMENT_3D ( 'NONE', #38122, #31747, #51730 ) ;
#83966=DIRECTION ( 'NONE',  ( 0.000000000000000000, 1.000000000000000000, 0.000000000000000000 ) ) ;
#83971=CARTESIAN_POINT ( 'NONE',  ( 112.8043457091679471, -45.48636447812791062, 178.0384824187679556 ) ) ;
#83972=ORIENTED_EDGE ( 'NONE', *, *, #48843, .F. ) ;
#83974=CARTESIAN_POINT ( 'NONE',  ( 104.1798084317939725, -26.65242854998196265, 221.2984824187679465 ) ) ;
#83975=CARTESIAN_POINT ( 'NONE',  ( 117.4979393226723516, -37.96344061660173708, 49.73276813305393773 ) ) ;
#83977=CARTESIAN_POINT ( 'NONE',  ( 181.9694315774339941, -34.03355364505720360, 193.9678068554150059 ) ) ;
#83978=CIRCLE ( 'NONE', #46191, 3.250000000000002665 ) ;
#83979=DIRECTION ( 'NONE',  ( 1.000000000000000000, 0.000000000000000000, 0.000000000000000000 ) ) ;
#83980=ORIENTED_EDGE ( 'NONE', *, *, #24535, .T. ) ;
#83982=EDGE_LOOP ( 'NONE', ( #60569, #56221, #50398, #53285 ) ) ;
#83983=ORIENTED_EDGE ( 'NONE', *, *, #9133, .T. ) ;
#83986=DIRECTION ( 'NONE',  ( 1.000000000000000000, 4.163336342344333240E-14, 0.000000000000000000 ) ) ;
#83987=CARTESIAN_POINT ( 'NONE',  ( 97.61538875609650745, -41.12936756086440226, 252.6727681330536655 ) ) ;
#83988=CARTESIAN_POINT ( 'NONE',  ( 97.15942515429802029, -38.46280294437263336, 251.4648788724661586 ) ) ;
#83990=CARTESIAN_POINT ( 'NONE',  ( 136.2777084067364797, -17.08426318378579012, 2.472582314395108671 ) ) ;
#83992=FACE_OUTER_BOUND ( 'NONE', #13749, .T. ) ;
#83993=CARTESIAN_POINT ( 'NONE',  ( 163.1639762274895702, -34.03355364505878811, 313.9678068554149490 ) ) ;
#83994=FACE_OUTER_BOUND ( 'NONE', #85978, .T. ) ;
#83995=CARTESIAN_POINT ( 'NONE',  ( 97.75265732597522117, -31.99668793782200993, 50.95276813305294183 ) ) ;
#83996=EDGE_LOOP ( 'NONE', ( #16376, #41441, #25462, #79651 ) ) ;
#83998=EDGE_LOOP ( 'NONE', ( #50270, #6872 ) ) ;
#83999=DIRECTION ( 'NONE',  ( -4.299999999999999979E-14, 1.000000000000000000, 0.000000000000000000 ) ) ;
#84000=CARTESIAN_POINT ( 'NONE',  ( 97.12550670785735463, -37.99649542378719502, 17.42805171007513820 ) ) ;
#84001=CARTESIAN_POINT ( 'NONE',  ( 98.59486473514179750, -43.92970144294050527, 222.8870538473389615 ) ) ;
#84003=CARTESIAN_POINT ( 'NONE',  ( 108.8666348730871078, -46.34312957481623840, 78.72419670448194040 ) ) ;
#84004=LINE ( 'NONE', #55797, #861 ) ;
#84005=VECTOR ( 'NONE', #60060, 1000.000000000000000 ) ;
#84007=ORIENTED_EDGE ( 'NONE', *, *, #83763, .F. ) ;
#84008=CARTESIAN_POINT ( 'NONE',  ( 172.5664832912729878, -27.57844715994070484, 258.9256252759120116 ) ) ;
#84009=ORIENTED_EDGE ( 'NONE', *, *, #22548, .F. ) ;
#84012=CARTESIAN_POINT ( 'NONE',  ( 115.9278856700424143, -36.79130581669468825, 260.2530118773256049 ) ) ;
#84013=CARTESIAN_POINT ( 'NONE',  ( 181.9790560690580037, -31.62489322948711035, -5.074374724088000832 ) ) ;
#84014=CARTESIAN_POINT ( 'NONE',  ( 36.23715912545345930, -47.82818131006131779, 117.4678068554150485 ) ) ;
#84015=EDGE_CURVE ( 'NONE', #73817, #74757, #30473, .T. ) ;
#84018=CARTESIAN_POINT ( 'NONE',  ( 177.0664832912740110, 12.92155284005802685, 335.5992267699913327 ) ) ;
#84019=ORIENTED_EDGE ( 'NONE', *, *, #18727, .T. ) ;
#84020=CARTESIAN_POINT ( 'NONE',  ( 141.9629299006806491, -9.772340378754520884, 14.92562527591104349 ) ) ;
#84021=LINE ( 'NONE', #20888, #10708 ) ;
#84023=CARTESIAN_POINT ( 'NONE',  ( 111.9289591080100053, -27.50755150920414849, 59.68991099019693536 ) ) ;
#84024=ORIENTED_EDGE ( 'NONE', *, *, #57005, .F. ) ;
#84025=CARTESIAN_POINT ( 'NONE',  ( 99.35431583021956214, -34.05534528112548287, 283.8795189410199100 ) ) ;
#84026=CARTESIAN_POINT ( 'NONE',  ( 100.8881676017241489, -44.70077481762183425, 127.0522015394391673 ) ) ;
#84027=CARTESIAN_POINT ( 'NONE',  ( 97.38117110781242047, -35.36630255995240191, 181.2156252759109805 ) ) ;
#84029=DIRECTION ( 'NONE',  ( 2.900000000000000265E-14, -2.000000000000000155E-15, 1.000000000000000000 ) ) ;
#84030=FACE_OUTER_BOUND ( 'NONE', #3221, .T. ) ;
#84031=CARTESIAN_POINT ( 'NONE',  ( 46.48091746482051434, -49.32844715994088602, 129.9678068554150911 ) ) ;
#84032=VECTOR ( 'NONE', #28465, 1000.000000000000000 ) ;
#84033=CARTESIAN_POINT ( 'NONE',  ( 97.77292256144662019, -40.53329279276322694, 7.635625275910939536 ) ) ;
#84037=ORIENTED_EDGE ( 'NONE', *, *, #73173, .T. ) ;
#84038=CARTESIAN_POINT ( 'NONE',  ( 107.3350663223963153, -26.26422652666180468, 116.0556252759109555 ) ) ;
#84039=EDGE_CURVE ( 'NONE', #42888, #4612, #89270, .T. ) ;
#84043=VERTEX_POINT ( 'NONE', #16402 ) ;
#84045=EDGE_CURVE ( 'NONE', #31761, #50719, #44080, .T. ) ;
#84047=CARTESIAN_POINT ( 'NONE',  ( 97.07207478302663617, -35.37842197911977138, 267.2189570788717674 ) ) ;
#84049=CARTESIAN_POINT ( 'NONE',  ( 51.56670390244671154, -32.29483332968566600, 193.9678068554150911 ) ) ;
#84050=FACE_OUTER_BOUND ( 'NONE', #33325, .T. ) ;
#84051=CARTESIAN_POINT ( 'NONE',  ( 105.3204089162997263, -26.45171782723944176, 11.20991099019697046 ) ) ;
#84052=ADVANCED_FACE ( 'NONE', ( #1877 ), #59044, .F. ) ;
#84054=EDGE_LOOP ( 'NONE', ( #60871, #80634, #42361, #7048 ) ) ;
#84057=EDGE_CURVE ( 'NONE', #61299, #73246, #67532, .T. ) ;
#84058=LINE ( 'NONE', #43585, #49034 ) ;
#84059=ORIENTED_EDGE ( 'NONE', *, *, #5227, .F. ) ;
#84061=VECTOR ( 'NONE', #64342, 1000.000000000000114 ) ;
#84063=CARTESIAN_POINT ( 'NONE',  ( 123.6837132603318992, -20.11243780205710507, 239.5838068554165545 ) ) ;
#84066=EDGE_CURVE ( 'NONE', #47474, #10820, #70930, .T. ) ;
#84067=CARTESIAN_POINT ( 'NONE',  ( 116.3254862984629909, -32.93730789470958342, 129.1356252759109680 ) ) ;
#84068=PLANE ( 'NONE',  #44595 ) ;
#84069=CARTESIAN_POINT ( 'NONE',  ( 108.9443472801882393, -27.87019791606706320, 184.3448007804579447 ) ) ;
#84070=CARTESIAN_POINT ( 'NONE',  ( 41.56648329127398966, -27.82844715994070484, 314.1756252759120116 ) ) ;
#84072=CARTESIAN_POINT ( 'NONE',  ( 98.26918992425659383, -28.71468409831775404, 80.73848241876795839 ) ) ;
#84074=DIRECTION ( 'NONE',  ( 0.000000000000000000, 0.000000000000000000, 1.000000000000000000 ) ) ;
#84075=EDGE_LOOP ( 'NONE', ( #73483, #80469, #11877, #73857 ) ) ;
#84076=VECTOR ( 'NONE', #5153, 1000.000000000000000 ) ;
#84077=DIRECTION ( 'NONE',  ( -1.000000000000000000, -4.299999999999999979E-14, -1.000000000000000078E-15 ) ) ;
#84078=EDGE_CURVE ( 'NONE', #29859, #48706, #16772, .T. ) ;
#84079=ORIENTED_EDGE ( 'NONE', *, *, #55176, .T. ) ;
#84080=CARTESIAN_POINT ( 'NONE',  ( 109.7247418026906729, -27.00076879412921826, 49.86480213811073980 ) ) ;
#84081=EDGE_LOOP ( 'NONE', ( #10497, #35381, #38472, #62560 ) ) ;
#84084=CARTESIAN_POINT ( 'NONE',  ( 80.06648329127402519, -46.72944715994105991, -0.5743747240890559880 ) ) ;
#84085=CARTESIAN_POINT ( 'NONE',  ( 105.7167510403503741, -46.72405128237544858, 273.4686170738095825 ) ) ;
#84086=LINE ( 'NONE', #84542, #81505 ) ;
#84088=CARTESIAN_POINT ( 'NONE',  ( 96.17000221327154463, -38.71995997157278424, 51.48229194257797303 ) ) ;
#84089=LINE ( 'NONE', #77265, #36193 ) ;
#84091=CARTESIAN_POINT ( 'NONE',  ( 138.8167039024479834, -50.82844715994100682, 63.03480685541479289 ) ) ;
#84092=CARTESIAN_POINT ( 'NONE',  ( 112.0659116084588049, -45.48839626879258446, 142.9897919413060094 ) ) ;
#84094=EDGE_CURVE ( 'NONE', #59559, #36906, #86336, .T. ) ;
#84095=CARTESIAN_POINT ( 'NONE',  ( 112.8075328016465022, -28.50283045258476378, 120.5906983358263460 ) ) ;
#84098=ADVANCED_FACE ( 'NONE', ( #2778 ), #76219, .F. ) ;
#84100=CARTESIAN_POINT ( 'NONE',  ( 117.2306693829537210, -39.29235896168534481, 119.6299109901969615 ) ) ;
#84101=EDGE_CURVE ( 'NONE', #57694, #50013, #72260, .T. ) ;
#84104=DIRECTION ( 'NONE',  ( 0.000000000000000000, -1.000000000000000000, 0.000000000000000000 ) ) ;
#84105=AXIS2_PLACEMENT_3D ( 'NONE', #10595, #36535, #57402 ) ;
#84106=VERTEX_POINT ( 'NONE', #57265 ) ;
#84108=CARTESIAN_POINT ( 'NONE',  ( 98.40655050692429029, -32.18313002855528993, 131.9413395616250000 ) ) ;
#84109=DIRECTION ( 'NONE',  ( 0.000000000000000000, 0.000000000000000000, -1.000000000000000000 ) ) ;
#84111=CARTESIAN_POINT ( 'NONE',  ( 96.58568816239609589, -40.17018292043292860, 282.5908633711490552 ) ) ;
#84113=CARTESIAN_POINT ( 'NONE',  ( 193.0371591254574639, -23.42818131005411786, 180.4678068554150343 ) ) ;
#84115=LINE ( 'NONE', #89, #76151 ) ;
#84118=DIRECTION ( 'NONE',  ( -0.9254794337955620787, -0.3787978585227822492, 0.000000000000000000 ) ) ;
#84119=B_SPLINE_CURVE_WITH_KNOTS ( 'NONE', 3,
 ( #40988, #33736, #11958, #32832, #61426, #60073, #89153, #20565, #87805, #48234, #26917, #46888, #54592, #89606, #6473, #68707, #61872, #27364, #25571, #53246, #81014, #46444, #12397, #77764, #41423, #35508, #7375, #41866, #14647, #63231, #69605, #1008, #28712, #549, #49128 ),
 .UNSPECIFIED., .F., .F.,
 ( 4, 2, 2, 1, 1, 2, 2, 2, 2, 2, 2, 1, 1, 2, 2, 2, 1, 1, 1, 2, 4 ),
 ( 0.3333434881890883217, 0.4166701562233613432, 0.4218780729755014502, 0.4270859897276415573, 0.4375018232319191069, 0.4583334902404722633, 0.4999968242575802968, 0.5208284912661340638, 0.5416601582746880528, 0.5624918252832418197, 0.5650957836593112349, 0.5676997420353806501, 0.5729076587875210347, 0.5833234922918014709, 0.6249868263089239928, 0.6275907846849948513, 0.6301947430610657097, 0.6354026598132067605, 0.6458184933174879738, 0.6562343268217694092, 0.6666501603260506226 ),
 .UNSPECIFIED. ) ;
#84120=CARTESIAN_POINT ( 'NONE',  ( 116.7742277529940225, -35.53649587948895316, 193.9241967044829664 ) ) ;
#84121=VERTEX_POINT ( 'NONE', #3220 ) ;
#84122=ORIENTED_EDGE ( 'NONE', *, *, #69334, .T. ) ;
#84123=VECTOR ( 'NONE', #79278, 1000.000000000000114 ) ;
#84124=CARTESIAN_POINT ( 'NONE',  ( 103.6521623672117158, -27.97622271609356659, 166.7920594963739802 ) ) ;
#84125=VECTOR ( 'NONE', #51057, 1000.000000000000000 ) ;
#84126=CARTESIAN_POINT ( 'NONE',  ( 30.48091746481751230, -49.32844715994156815, 129.9678068554150627 ) ) ;
#84127=CARTESIAN_POINT ( 'NONE',  ( 99.18317230595245348, -39.95607890373031523, 8.067297591610955720 ) ) ;
#84129=B_SPLINE_CURVE_WITH_KNOTS ( 'NONE', 3,
 ( #48027, #55281, #27602, #54829, #20352, #13531, #42115, #41213, #69842, #35297, #63011, #44800, #17116, #8969, #72081, #86157, #71637, #63924 ),
 .UNSPECIFIED., .F., .F.,
 ( 4, 2, 2, 2, 2, 2, 2, 2, 4 ),
 ( 0.000000000000000000, 0.06250000006729680702, 0.1250000001345936140, 0.1875000002018904210, 0.2500000002691872281, 0.3125000003364840628, 0.3750000004037808421, 0.4375000004710776214, 0.5000000005383744561 ),
 .UNSPECIFIED. ) ;
#84130=DIRECTION ( 'NONE',  ( 0.9999999853157766072, 0.0001713722456134502174, 0.000000000000000000 ) ) ;
#84132=CARTESIAN_POINT ( 'NONE',  ( 51.03742451361402743, -23.42844715994066362, 313.9678068554150059 ) ) ;
#84133=DIRECTION ( 'NONE',  ( -1.000000000000000078E-15, 1.000000000000000083E-30, 1.000000000000000000 ) ) ;
#84134=LINE ( 'NONE', #34160, #37238 ) ;
#84135=PRODUCT_DEFINITION_FORMATION_WITH_SPECIFIED_SOURCE ( 'ANY', '', #87948, .NOT_KNOWN. ) ;
#84136=CARTESIAN_POINT ( 'NONE',  ( 97.93839266929572318, -41.72010113774609152, 221.7241967044819546 ) ) ;
#84137=CARTESIAN_POINT ( 'NONE',  ( 83.06670390244796920, -61.87844715994100397, 207.5838068554149913 ) ) ;
#84139=ORIENTED_EDGE ( 'NONE', *, *, #51920, .F. ) ;
#84140=CARTESIAN_POINT ( 'NONE',  ( 105.7154773117002264, -46.72385838984938289, 87.46895860775489950 ) ) ;
#84142=AXIS2_PLACEMENT_3D ( 'NONE', #56538, #62463, #89747 ) ;
#84143=CARTESIAN_POINT ( 'NONE',  ( 98.15071166569833849, -41.26109095279260686, 122.7000959776797799 ) ) ;
#84144=DIRECTION ( 'NONE',  ( 1.000000000000000000, 8.673617379883546378E-16, 9.757819552368989676E-16 ) ) ;
#84145=CARTESIAN_POINT ( 'NONE',  ( 99.56037394151449860, -43.88466257697679396, 32.92038718067297509 ) ) ;
#84146=CARTESIAN_POINT ( 'NONE',  ( 50.87649884952499946, -33.54226604284930602, -5.074374724088000832 ) ) ;
#84148=CARTESIAN_POINT ( 'NONE',  ( 118.2550939253582811, -40.78236016348033388, 19.54991099019698453 ) ) ;
#84150=DIRECTION ( 'NONE',  ( 1.000000000000000078E-15, -1.000000000000000083E-30, -1.000000000000000000 ) ) ;
#84151=CARTESIAN_POINT ( 'NONE',  ( 96.51793475972648650, -31.32865002300666646, 245.9499109901969689 ) ) ;
#84153=EDGE_LOOP ( 'NONE', ( #29585, #13405, #35339, #25947, #1800, #73808, #73140, #9845, #3818, #78700, #70074, #63471, #72435, #55649, #64551, #25953, #58521, #75226, #9634, #64359, #3624, #20134, #22933, #82229, #73419, #65154, #29412, #86958, #35198, #79817, #79329, #8637, #27013, #35745, #85134, #25526, #58333, #67655, #27764, #16109, #48155, #23884, #35167, #81648, #3940, #46620, #83044, #30441 ) ) ;
#84154=EDGE_CURVE ( 'NONE', #47812, #75087, #17735, .T. ) ;
#84156=DIRECTION ( 'NONE',  ( 0.000000000000000000, 0.000000000000000000, 1.000000000000000000 ) ) ;
#84157=CARTESIAN_POINT ( 'NONE',  ( 110.8537976423054374, -45.98451334053003592, 167.8855672870433295 ) ) ;
#84158=CARTESIAN_POINT ( 'NONE',  ( 99.41042786952979782, -33.89845062227509231, 63.86237608387695985 ) ) ;
#84159=CARTESIAN_POINT ( 'NONE',  ( 114.2683966348991760, -44.29710505712337465, 154.1813395616249807 ) ) ;
#84160=EDGE_CURVE ( 'NONE', #30939, #31976, #69026, .T. ) ;
#84161=DIRECTION ( 'NONE',  ( 0.000000000000000000, 0.000000000000000000, 1.000000000000000000 ) ) ;
#84163=ADVANCED_FACE ( 'NONE', ( #54005, #10910, #39512, #18624, #33146, #80416 ), #74035, .T. ) ;
#84164=LINE ( 'NONE', #70067, #43658 ) ;
#84167=EDGE_CURVE ( 'NONE', #58422, #1886, #11816, .T. ) ;
#84170=ORIENTED_EDGE ( 'NONE', *, *, #33789, .T. ) ;
#84171=DIRECTION ( 'NONE',  ( 0.000000000000000000, 0.000000000000000000, 1.000000000000000000 ) ) ;
#84174=CARTESIAN_POINT ( 'NONE',  ( 99.03715563995052662, -32.54106229299839725, 90.35432458998199934 ) ) ;
#84175=CARTESIAN_POINT ( 'NONE',  ( 115.3410742220599872, -45.24796585940374882, 268.1899109901965517 ) ) ;
#84176=AXIS2_PLACEMENT_3D ( 'NONE', #37646, #70834, #36304 ) ;
#84179=EDGE_CURVE ( 'NONE', #11502, #31632, #26943, .T. ) ;
#84181=VECTOR ( 'NONE', #72796, 1000.000000000000000 ) ;
#84186=VECTOR ( 'NONE', #8084, 1000.000000000000000 ) ;
#84187=CARTESIAN_POINT ( 'NONE',  ( 96.70615320395830850, -37.17927570127479697, 116.3489586092449599 ) ) ;
#84188=CARTESIAN_POINT ( 'NONE',  ( 97.58231912995226764, -32.21254287871169453, 75.97276813305397525 ) ) ;
#84189=DIRECTION ( 'NONE',  ( -1.000000000000000000, -2.756263715554006823E-15, 0.000000000000000000 ) ) ;
#84190=ORIENTED_EDGE ( 'NONE', *, *, #88997, .T. ) ;
#84192=CARTESIAN_POINT ( 'NONE',  ( 118.0818320075808856, -32.35879749485835788, 249.1270538473389706 ) ) ;
#84193=DIRECTION ( 'NONE',  ( 0.000000000000000000, 1.000000000000000000, 0.000000000000000000 ) ) ;
#84194=DIRECTION ( 'NONE',  ( 0.000000000000000000, 0.000000000000000000, -1.000000000000000000 ) ) ;
#84198=DIRECTION ( 'NONE',  ( 3.999999999999999995E-14, -1.000000000000000000, 4.100000000000000342E-29 ) ) ;
#84200=B_SPLINE_CURVE_WITH_KNOTS ( 'NONE', 3,
 ( #27548, #47524, #33909, #55227, #82985, #40720, #74360, #33013, #88446, #292, #33463, #68444, #26206, #61603, #27104, #82543, #61167, #53880 ),
 .UNSPECIFIED., .F., .F.,
 ( 4, 2, 2, 2, 2, 2, 2, 2, 4 ),
 ( 0.000000000000000000, 0.06249999974512615575, 0.1249999994902523115, 0.1874999992353784672, 0.2499999989805046230, 0.3124999987256307787, 0.3749999984707569345, 0.4374999982158830902, 0.4999999979610092460 ),
 .UNSPECIFIED. ) ;
#84201=CARTESIAN_POINT ( 'NONE',  ( 184.5667039024480118, -67.87844715994100397, 310.9178068554150514 ) ) ;
#84203=CARTESIAN_POINT ( 'NONE',  ( 163.0664832912739826, 19.62155284005901024, 336.6506252759110112 ) ) ;
#84204=DIRECTION ( 'NONE',  ( -0.7071067811855830110, -0.7071067811875120235, 0.000000000000000000 ) ) ;
#84206=ADVANCED_FACE ( 'NONE', ( #26333 ), #18170, .T. ) ;
#84207=CARTESIAN_POINT ( 'NONE',  ( 188.5667039024479834, -48.82844715994099971, 134.4678068554150059 ) ) ;
#84208=ORIENTED_EDGE ( 'NONE', *, *, #36542, .T. ) ;
#84210=CARTESIAN_POINT ( 'NONE',  ( 116.2381414160656874, -41.80576965393662903, 263.4241967044824833 ) ) ;
#84211=CARTESIAN_POINT ( 'NONE',  ( 111.7941755367341443, -25.86282203548705283, 130.7499109901969518 ) ) ;
#84212=CARTESIAN_POINT ( 'NONE',  ( 116.1773114014176969, -43.03338396708490166, 9.356577656862985037 ) ) ;
#84213=AXIS2_PLACEMENT_3D ( 'NONE', #86301, #65836, #36811 ) ;
#84215=CARTESIAN_POINT ( 'NONE',  ( 80.06648329127402519, -46.72944715994105991, -0.8743747240890559214 ) ) ;
#84216=CYLINDRICAL_SURFACE ( 'NONE', #88523, 2.500000000000002220 ) ;
#84217=CARTESIAN_POINT ( 'NONE',  ( 82.54568444101083458, -35.53793914064088000, 7.103892432648359012 ) ) ;
#84218=DIRECTION ( 'NONE',  ( 0.000000000000000000, 1.000000000000000000, 0.000000000000000000 ) ) ;
#84219=EDGE_LOOP ( 'NONE', ( #8939, #14186, #78467, #11628 ) ) ;
#84221=ORIENTED_EDGE ( 'NONE', *, *, #45349, .T. ) ;
#84223=CARTESIAN_POINT ( 'NONE',  ( 99.71244791179715605, -41.13061414147755812, 161.1781341137909465 ) ) ;
#84224=CARTESIAN_POINT ( 'NONE',  ( 101.9922426440110428, -45.44522117600308775, 187.1568647513990697 ) ) ;
#84226=VECTOR ( 'NONE', #27431, 1000.000000000000114 ) ;
#84227=CARTESIAN_POINT ( 'NONE',  ( 142.8687636814962616, 5.654319119531167281, 361.9756252759100335 ) ) ;
#84228=CARTESIAN_POINT ( 'NONE',  ( 114.3286968523003253, -29.23113535793739359, 170.4641967044829585 ) ) ;
#84229=CARTESIAN_POINT ( 'NONE',  ( 112.0634988668466576, -45.48974152076988986, 148.9902647339903581 ) ) ;
#84230=FACE_OUTER_BOUND ( 'NONE', #5977, .T. ) ;
#84231=FACE_OUTER_BOUND ( 'NONE', #29399, .T. ) ;
#84232=FACE_OUTER_BOUND ( 'NONE', #84081, .T. ) ;
#84233=DIRECTION ( 'NONE',  ( -2.900000000000000265E-14, 2.000000000000000155E-15, -1.000000000000000000 ) ) ;
#84234=CARTESIAN_POINT ( 'NONE',  ( 96.20363159075253634, -34.36081134307595164, 106.1556252759109640 ) ) ;
#84235=VERTEX_POINT ( 'NONE', #68120 ) ;
#84236=VECTOR ( 'NONE', #35175, 1000.000000000000000 ) ;
#84237=ORIENTED_EDGE ( 'NONE', *, *, #85702, .T. ) ;
#84239=CARTESIAN_POINT ( 'NONE',  ( 99.86128698970316009, -42.75951115570669714, 68.30063092494498278 ) ) ;
#84241=CARTESIAN_POINT ( 'NONE',  ( 110.2867295656602380, -27.49400189596552835, 205.8099109901959594 ) ) ;
#84245=PLANE ( 'NONE',  #89523 ) ;
#84247=DIRECTION ( 'NONE',  ( 0.000000000000000000, 0.000000000000000000, 1.000000000000000000 ) ) ;
#84248=CARTESIAN_POINT ( 'NONE',  ( 117.1424269838423839, -34.14023410701941685, 124.0270538473399426 ) ) ;
#84249=ORIENTED_EDGE ( 'NONE', *, *, #60042, .T. ) ;
#84251=VECTOR ( 'NONE', #24344, 1000.000000000000000 ) ;
#84252=ORIENTED_EDGE ( 'NONE', *, *, #68252, .F. ) ;
#84253=CIRCLE ( 'NONE', #36392, 0.5000000000000007772 ) ;
#84256=CARTESIAN_POINT ( 'NONE',  ( 151.0371591254575776, -24.42818131005592264, 129.9678068554149775 ) ) ;
#84257=CARTESIAN_POINT ( 'NONE',  ( 131.0667039024480118, -58.72944715994098885, 234.8338068554150198 ) ) ;
#84258=CARTESIAN_POINT ( 'NONE',  ( 106.8982433325019059, -45.38234380569505788, 225.3671379886389730 ) ) ;
#84260=CIRCLE ( 'NONE', #13114, 2.500000000000002220 ) ;
#84263=EDGE_CURVE ( 'NONE', #2705, #83951, #49682, .T. ) ;
#84265=ORIENTED_EDGE ( 'NONE', *, *, #65874, .T. ) ;
#84268=AXIS2_PLACEMENT_3D ( 'NONE', #3933, #30310, #58007 ) ;
#84269=EDGE_CURVE ( 'NONE', #75328, #3377, #12715, .T. ) ;
#84273=LINE ( 'NONE', #22044, #84125 ) ;
#84274=CARTESIAN_POINT ( 'NONE',  ( 111.6463204169710082, -44.35094448583814852, 234.4387261630399450 ) ) ;
#84275=EDGE_CURVE ( 'NONE', #45317, #22746, #38616, .T. ) ;
#84276=DIRECTION ( 'NONE',  ( 1.000000000000000078E-15, -1.000000000000000083E-30, -1.000000000000000000 ) ) ;
#84277=VERTEX_POINT ( 'NONE', #74937 ) ;
#84278=LINE ( 'NONE', #21137, #78450 ) ;
#84283=CARTESIAN_POINT ( 'NONE',  ( 110.8548543103858322, -45.98408086708722919, 112.8856581590341932 ) ) ;
#84284=EDGE_LOOP ( 'NONE', ( #741, #50604, #61914, #12224 ) ) ;
#84287=CARTESIAN_POINT ( 'NONE',  ( 113.7913882254195101, -32.05415687329151098, 277.1280903695913480 ) ) ;
#84288=CARTESIAN_POINT ( 'NONE',  ( 114.5434305778746733, -28.56033675696621899, 154.4746728949589851 ) ) ;
#84289=AXIS2_PLACEMENT_3D ( 'NONE', #34132, #81428, #33698 ) ;
#84290=CARTESIAN_POINT ( 'NONE',  ( 108.3168256696638281, -47.05733704442519638, 117.6727681330539639 ) ) ;
#84291=DIRECTION ( 'NONE',  ( 1.000000000000000078E-15, -1.000000000000000083E-30, -1.000000000000000000 ) ) ;
#84292=CARTESIAN_POINT ( 'NONE',  ( 77.31648329127402519, -36.72944715994107412, -5.074374724089059541 ) ) ;
#84293=CARTESIAN_POINT ( 'NONE',  ( 100.8232821092315845, -45.85065428865130599, 238.1108633711489517 ) ) ;
#84296=DIRECTION ( 'NONE',  ( -0.7071067811865175967, -0.7071067811865774377, -7.071067811865168663E-16 ) ) ;
#84297=ORIENTED_EDGE ( 'NONE', *, *, #27845, .F. ) ;
#84300=ADVANCED_FACE ( 'NONE', ( #48096 ), #77182, .F. ) ;
#84301=ORIENTED_EDGE ( 'NONE', *, *, #74131, .T. ) ;
#84302=DIRECTION ( 'NONE',  ( 0.000000000000000000, 0.000000000000000000, 1.000000000000000000 ) ) ;
#84303=CIRCLE ( 'NONE', #1623, 2.116999999999993776 ) ;
#84304=CARTESIAN_POINT ( 'NONE',  ( 97.60784930588656039, -39.98230802730879674, 137.5900448901282971 ) ) ;
#84305=AXIS2_PLACEMENT_3D ( 'NONE', #58220, #84609, #9626 ) ;
#84306=ORIENTED_EDGE ( 'NONE', *, *, #69083, .T. ) ;
#84307=CARTESIAN_POINT ( 'NONE',  ( 114.7715153371978687, -44.65482214316887877, 118.2022919425779719 ) ) ;
#84308=DIRECTION ( 'NONE',  ( 0.000000000000000000, 0.000000000000000000, -1.000000000000000000 ) ) ;
#84309=DIRECTION ( 'NONE',  ( 0.000000000000000000, 0.000000000000000000, -1.000000000000000000 ) ) ;
#84312=CARTESIAN_POINT ( 'NONE',  ( 105.6178435110047644, -46.65043233106474929, 57.46071414996635696 ) ) ;
#84313=CARTESIAN_POINT ( 'NONE',  ( 118.6297112294782892, -39.20734283244433982, 254.6584824187681022 ) ) ;
#84314=DIRECTION ( 'NONE',  ( 0.000000000000000000, -1.000000000000000000, 0.000000000000000000 ) ) ;
#84316=CARTESIAN_POINT ( 'NONE',  ( 69.68306499799194853, -72.55732494038082336, 540.9756252759101471 ) ) ;
#84318=CARTESIAN_POINT ( 'NONE',  ( 194.5664832912739826, -18.82844715994099971, 342.9256252759119548 ) ) ;
#84319=CARTESIAN_POINT ( 'NONE',  ( 51.34673845256598668, -29.62846900982231446, -5.074374724088000832 ) ) ;
#84321=CARTESIAN_POINT ( 'NONE',  ( 106.8354617269136497, -47.19621815579884583, 272.5584824187680510 ) ) ;
#84322=ORIENTED_EDGE ( 'NONE', *, *, #25648, .T. ) ;
#84323=DIRECTION ( 'NONE',  ( 0.000000000000000000, 0.000000000000000000, 1.000000000000000000 ) ) ;
#84324=CARTESIAN_POINT ( 'NONE',  ( 114.4785830672529130, -28.49803820358978612, 159.5051490854349652 ) ) ;
#84325=CARTESIAN_POINT ( 'NONE',  ( 114.0905851706116181, -46.27390148416495208, 29.08133956162595268 ) ) ;
#84326=CARTESIAN_POINT ( 'NONE',  ( 101.3252678580387709, -46.22870732629148449, 198.1318157521009482 ) ) ;
#84327=DIRECTION ( 'NONE',  ( 0.000000000000000000, 0.000000000000000000, 1.000000000000000000 ) ) ;
#84329=LINE ( 'NONE', #37047, #15634 ) ;
#84331=CYLINDRICAL_SURFACE ( 'NONE', #26719, 3.000000000000002665 ) ;
#84332=CARTESIAN_POINT ( 'NONE',  ( 105.7995184974070213, -26.72403496479216756, 70.17729194179682395 ) ) ;
#84333=LINE ( 'NONE', #21192, #29160 ) ;
#84336=CARTESIAN_POINT ( 'NONE',  ( 156.5667039024483813, -48.82844715993569196, 257.2178068554149490 ) ) ;
#84338=ORIENTED_EDGE ( 'NONE', *, *, #74276, .T. ) ;
#84339=VECTOR ( 'NONE', #8663, 999.9999999999998863 ) ;
#84342=CARTESIAN_POINT ( 'NONE',  ( 97.64212626138838402, -32.24102647341089778, 71.97276813305397525 ) ) ;
#84344=B_SPLINE_CURVE_WITH_KNOTS ( 'NONE', 3,
 ( #63697, #64591, #27821, #7828, #83698, #1478, #35522, #56864, #55499, #14201, #55953, #48692, #76422, #41879, #69616, #35075, #7385, #1022, #62783, #28259, #28725, #84606, #22366, #50043, #37781, #30957, #73174, #24593, #4144, #17337, #16892, #51824, #58644, #11406, #85947, #72745, #85508, #31843 ),
 .UNSPECIFIED., .F., .F.,
 ( 4, 2, 2, 1, 2, 2, 2, 2, 1, 1, 2, 2, 2, 1, 2, 2, 1, 2, 1, 2, 2, 4 ),
 ( 0.000000000000000000, 0.04166793602364177868, 0.05208492002955201344, 0.05729341203250709613, 0.05989765803398427318, 0.06250190403546145024, 0.08333587204728039322, 0.1041698400590993639, 0.1145868240650088354, 0.1197953160679635781, 0.1223995620694415670, 0.1250038080709195421, 0.1666717440945562900, 0.1770887281004662195, 0.1822972201034212258, 0.1875057121063762045, 0.2083396801181911784, 0.2291736481300061246, 0.2395906321359124735, 0.2447991241388655925, 0.2500076161418187115, 0.3333434881890895429 ),
 .UNSPECIFIED. ) ;
#84345=VECTOR ( 'NONE', #75345, 1000.000000000000000 ) ;
#84346=DIRECTION ( 'NONE',  ( 1.000000000000000000, 4.163336342344333240E-14, 0.000000000000000000 ) ) ;
#84347=EDGE_CURVE ( 'NONE', #1345, #8193, #13601, .T. ) ;
#84348=CARTESIAN_POINT ( 'NONE',  ( 99.25607838769128932, -29.75875458388292571, 186.7470538473389752 ) ) ;
#84349=CARTESIAN_POINT ( 'NONE',  ( 98.62497865991430501, -35.42670724699001283, 265.6267055423624583 ) ) ;
#84350=VERTEX_POINT ( 'NONE', #868 ) ;
#84354=EDGE_LOOP ( 'NONE', ( #51615, #58145, #44427, #71454, #73970, #36313 ) ) ;
#84355=CARTESIAN_POINT ( 'NONE',  ( 104.4081006654926114, -46.45808914125378664, 107.3647919429337492 ) ) ;
#84356=FACE_BOUND ( 'NONE', #87133, .T. ) ;
#84357=CYLINDRICAL_SURFACE ( 'NONE', #72381, 2.500000000000002220 ) ;
#84359=CARTESIAN_POINT ( 'NONE',  ( 90.44969454456422397, -23.41243780205710578, 239.5838068554175209 ) ) ;
#84360=FACE_OUTER_BOUND ( 'NONE', #28131, .T. ) ;
#84362=LINE ( 'NONE', #1229, #41912 ) ;
#84363=CARTESIAN_POINT ( 'NONE',  ( 97.21286698537356585, -39.96429565625729907, 286.5908633711495668 ) ) ;
#84365=VERTEX_POINT ( 'NONE', #28565 ) ;
#84367=VECTOR ( 'NONE', #65417, 1000.000000000000000 ) ;
#84368=DIRECTION ( 'NONE',  ( 1.000000000000000000, 0.000000000000000000, 0.000000000000000000 ) ) ;
#84369=CARTESIAN_POINT ( 'NONE',  ( 100.6253115865833365, -30.05058211904245624, 113.5052332267339779 ) ) ;
#84370=AXIS2_PLACEMENT_3D ( 'NONE', #66594, #79366, #53387 ) ;
#84372=LINE ( 'NONE', #89837, #60097 ) ;
#84375=ORIENTED_EDGE ( 'NONE', *, *, #58705, .T. ) ;
#84376=VERTEX_POINT ( 'NONE', #20865 ) ;
#84377=CYLINDRICAL_SURFACE ( 'NONE', #14855, 9.999999999999998224 ) ;
#84378=EDGE_CURVE ( 'NONE', #78030, #46083, #39965, .T. ) ;
#84379=ORIENTED_EDGE ( 'NONE', *, *, #15565, .T. ) ;
#84382=CARTESIAN_POINT ( 'NONE',  ( 99.36575536895223593, -31.34657530650553880, 157.2606309249449623 ) ) ;
#84383=EDGE_CURVE ( 'NONE', #20396, #36063, #5155, .T. ) ;
#84385=CARTESIAN_POINT ( 'NONE',  ( 101.7448744985357223, -27.01524695604527082, 96.46324432352997746 ) ) ;
#84386=VECTOR ( 'NONE', #81077, 1000.000000000000000 ) ;
#84387=DIRECTION ( 'NONE',  ( 0.000000000000000000, 0.000000000000000000, 1.000000000000000000 ) ) ;
#84390=ORIENTED_EDGE ( 'NONE', *, *, #12588, .T. ) ;
#84391=ADVANCED_FACE ( 'NONE', ( #83108 ), #70361, .T. ) ;
#84395=CARTESIAN_POINT ( 'NONE',  ( 100.6033219294167793, -44.83909144599476804, 272.0289586092449667 ) ) ;
#84396=CARTESIAN_POINT ( 'NONE',  ( 98.53347975398118308, -44.98838784992466344, 187.9384824187679612 ) ) ;
#84398=FACE_OUTER_BOUND ( 'NONE', #21963, .T. ) ;
#84399=CARTESIAN_POINT ( 'NONE',  ( 96.60720999893194971, -36.88735532319633847, 132.3384824187679669 ) ) ;
#84401=DIRECTION ( 'NONE',  ( -0.9254794337955620787, -0.3787978585227822492, 0.000000000000000000 ) ) ;
#84403=CARTESIAN_POINT ( 'NONE',  ( 97.75865386173192917, -40.38557078241878884, 116.6246290760604438 ) ) ;
#84404=ORIENTED_EDGE ( 'NONE', *, *, #33116, .T. ) ;
#84405=DIRECTION ( 'NONE',  ( -3.999999999999999995E-14, 1.000000000000000000, -4.100000000000000342E-29 ) ) ;
#84406=ORIENTED_EDGE ( 'NONE', *, *, #56184, .F. ) ;
#84409=CARTESIAN_POINT ( 'NONE',  ( 97.02380861106273358, -36.97117146848575686, 132.3454236201547758 ) ) ;
#84410=CARTESIAN_POINT ( 'NONE',  ( 115.6733145644062262, -43.66497474544748059, 43.27467289495795200 ) ) ;
#84412=DIRECTION ( 'NONE',  ( 1.000000000000000078E-15, -1.000000000000000083E-30, -1.000000000000000000 ) ) ;
#84414=CARTESIAN_POINT ( 'NONE',  ( 101.5072281473882043, -27.97539281467247108, 65.51467289495899138 ) ) ;
#84415=CARTESIAN_POINT ( 'NONE',  ( 97.80519586107577368, -40.50152893159460632, 111.6342583986536425 ) ) ;
#84416=CARTESIAN_POINT ( 'NONE',  ( 98.87380182923587313, -30.31772012733814492, 151.7984824187679465 ) ) ;
#84417=CARTESIAN_POINT ( 'NONE',  ( 113.2454986963039261, -28.75867294333132662, 70.55229194275597138 ) ) ;
#84418=DIRECTION ( 'NONE',  ( 0.000000000000000000, 0.000000000000000000, -1.000000000000000000 ) ) ;
#84419=ORIENTED_EDGE ( 'NONE', *, *, #28236, .F. ) ;
#84420=CARTESIAN_POINT ( 'NONE',  ( 29.56648329127298069, -81.37844715994266664, 342.9256252759109884 ) ) ;
#84421=VECTOR ( 'NONE', #82755, 1000.000000000000000 ) ;
#84424=ORIENTED_EDGE ( 'NONE', *, *, #62188, .T. ) ;
#84426=CARTESIAN_POINT ( 'NONE',  ( 101.9504156919933280, -46.58027128656367921, 167.1832443235299763 ) ) ;
#84428=CARTESIAN_POINT ( 'NONE',  ( 162.5667039024470171, -32.29483332968611364, 193.9678068554150059 ) ) ;
#84429=CARTESIAN_POINT ( 'NONE',  ( 98.82211989244140682, -29.33244250316893087, 231.7565776568629587 ) ) ;
#84430=CARTESIAN_POINT ( 'NONE',  ( 109.2641226286370824, -47.00117516105910198, 103.7441967044829880 ) ) ;
#84432=EDGE_CURVE ( 'NONE', #2876, #25445, #89013, .T. ) ;
#84435=VERTEX_POINT ( 'NONE', #76275 ) ;
#84436=AXIS2_PLACEMENT_3D ( 'NONE', #65159, #11077, #2942 ) ;
#84438=ADVANCED_FACE ( 'NONE', ( #63086 ), #14510, .F. ) ;
#84442=CARTESIAN_POINT ( 'NONE',  ( 63.56670390244708813, -40.82844715994014706, 180.4678068554151196 ) ) ;
#84443=CARTESIAN_POINT ( 'NONE',  ( 96.26801084314395496, -34.37000373589627600, 252.1432443235302969 ) ) ;
#84444=LINE ( 'NONE', #62175, #83803 ) ;
#84445=CARTESIAN_POINT ( 'NONE',  ( 134.9467300988947613, -16.12360705087671775, 1.744847597652565030 ) ) ;
#84447=CARTESIAN_POINT ( 'NONE',  ( 90.44969454456408187, -20.11243780205710507, 239.5838068554175209 ) ) ;
#84448=DIRECTION ( 'NONE',  ( 0.000000000000000000, 0.000000000000000000, -1.000000000000000000 ) ) ;
#84449=LINE ( 'NONE', #14042, #52961 ) ;
#84450=CARTESIAN_POINT ( 'NONE',  ( 107.6080043092626113, -48.59286871074260006, 42.61276813305398292 ) ) ;
#84451=ORIENTED_EDGE ( 'NONE', *, *, #9495, .T. ) ;
#84452=VECTOR ( 'NONE', #16938, 1000.000000000000000 ) ;
#84454=AXIS2_PLACEMENT_3D ( 'NONE', #72543, #79371, #45252 ) ;
#84455=EDGE_CURVE ( 'NONE', #59488, #82044, #68573, .T. ) ;
#84456=DIRECTION ( 'NONE',  ( -0.000000000000000000, -0.000000000000000000, 1.000000000000000000 ) ) ;
#84457=CARTESIAN_POINT ( 'NONE',  ( 113.2469266849859650, -28.75976546129976086, 15.55424117046798038 ) ) ;
#84458=CARTESIAN_POINT ( 'NONE',  ( 97.82556271424805061, -33.52526948863204126, 282.0613395616247772 ) ) ;
#84459=CIRCLE ( 'NONE', #27820, 2.117000000000007987 ) ;
#84460=DIRECTION ( 'NONE',  ( -0.9254794337955620787, -0.3787978585227822492, 0.000000000000000000 ) ) ;
#84461=CARTESIAN_POINT ( 'NONE',  ( 99.34849973496659459, -28.72665311504493246, 111.6870538473389587 ) ) ;
#84462=DIRECTION ( 'NONE',  ( 1.639958061481212836E-42, -4.100000000000000342E-29, -1.000000000000000000 ) ) ;
#84463=AXIS2_PLACEMENT_3D ( 'NONE', #41924, #20614, #84198 ) ;
#84464=CARTESIAN_POINT ( 'NONE',  ( 52.65249034007741358, -48.32844715994062312, 180.4678068554151196 ) ) ;
#84466=ORIENTED_EDGE ( 'NONE', *, *, #72063, .T. ) ;
#84467=CARTESIAN_POINT ( 'NONE',  ( 48.16670390244701139, -26.71338133339251542, 313.9678068554150059 ) ) ;
#84468=CARTESIAN_POINT ( 'NONE',  ( 80.06648329127401098, -33.97944715994105991, 1.625625275910943746 ) ) ;
#84469=ORIENTED_EDGE ( 'NONE', *, *, #7673, .F. ) ;
#84472=CARTESIAN_POINT ( 'NONE',  ( 106.8709381294020488, -45.58890767966684621, 268.9901547344683763 ) ) ;
#84474=( BOUNDED_CURVE ( )  B_SPLINE_CURVE ( 3, ( #52029, #38866, #4361, #72941 ),
 .UNSPECIFIED., .F., .T. ) 
 B_SPLINE_CURVE_WITH_KNOTS ( ( 4, 4 ),
 ( -3.022471162239526166E-12, 1.570796326791795705 ),
 .UNSPECIFIED. ) 
 CURVE ( )  GEOMETRIC_REPRESENTATION_ITEM ( )  RATIONAL_B_SPLINE_CURVE ( ( 1.000000000000000000, 0.8047378541243834782, 0.8047378541243834782, 1.000000000000000000 ) ) 
 REPRESENTATION_ITEM ( '' )  );
#84476=DIRECTION ( 'NONE',  ( -0.7071067811865513475, -0.7071067811865436870, -7.071067811865520693E-16 ) ) ;
#84479=ORIENTED_EDGE ( 'NONE', *, *, #56218, .T. ) ;
#84481=DIRECTION ( 'NONE',  ( -0.000000000000000000, 1.000000000000000000, 0.000000000000000000 ) ) ;
#84482=ADVANCED_FACE ( 'NONE', ( #69467 ), #77733, .T. ) ;
#84484=CARTESIAN_POINT ( 'NONE',  ( 101.1408812403245747, -27.39851324166288649, 65.51467289495799662 ) ) ;
#84487=CARTESIAN_POINT ( 'NONE',  ( 110.1408960893143956, -44.29103306967431308, 280.7023760838771409 ) ) ;
#84489=CARTESIAN_POINT ( 'NONE',  ( 102.2868918306627961, -45.93239726994513461, 167.1832443235309995 ) ) ;
#84492=FACE_OUTER_BOUND ( 'NONE', #64034, .T. ) ;
#84493=DIRECTION ( 'NONE',  ( 0.000000000000000000, 0.000000000000000000, -1.000000000000000000 ) ) ;
#84494=VECTOR ( 'NONE', #7563, 1000.000000000000000 ) ;
#84496=CARTESIAN_POINT ( 'NONE',  ( 106.8354761508916226, -47.19556465630029862, 268.5584824187679374 ) ) ;
#84500=CARTESIAN_POINT ( 'NONE',  ( 136.8164763767841521, -36.77596264856137509, 6.749779334551647914 ) ) ;
#84501=VERTEX_POINT ( 'NONE', #51684 ) ;
#84502=CARTESIAN_POINT ( 'NONE',  ( 97.89440201276070752, -31.60978508062128967, 106.9213395616259703 ) ) ;
#84503=CARTESIAN_POINT ( 'NONE',  ( 141.0667039024479834, -48.82844715994099971, 205.9178068554149945 ) ) ;
#84504=EDGE_LOOP ( 'NONE', ( #46674, #13866, #85133, #75506 ) ) ;
#84505=ORIENTED_EDGE ( 'NONE', *, *, #69567, .T. ) ;
#84507=EDGE_CURVE ( 'NONE', #78550, #51823, #57617, .T. ) ;
#84508=CARTESIAN_POINT ( 'NONE',  ( 113.1782937098645192, -44.75186864062681025, 123.0939586030858379 ) ) ;
#84509=LINE ( 'NONE', #22267, #34699 ) ;
#84511=EDGE_CURVE ( 'NONE', #38582, #8395, #50144, .T. ) ;
#84512=LINE ( 'NONE', #15001, #37913 ) ;
#84514=CARTESIAN_POINT ( 'NONE',  ( 118.0755232325510917, -37.71687819837586630, 29.74324432352998215 ) ) ;
#84516=DIRECTION ( 'NONE',  ( -2.999999999999999839E-15, 1.000000000000000000, -2.999999999999999900E-30 ) ) ;
#84519=FACE_OUTER_BOUND ( 'NONE', #46700, .T. ) ;
#84525=DIRECTION ( 'NONE',  ( 1.000000000000000078E-15, 1.000000000000000083E-30, -1.000000000000000000 ) ) ;
#84526=FACE_OUTER_BOUND ( 'NONE', #2711, .T. ) ;
#84527=CARTESIAN_POINT ( 'NONE',  ( 113.2432932581317289, -30.83002766685618923, 233.8552769709339429 ) ) ;
#84528=AXIS2_PLACEMENT_3D ( 'NONE', #17591, #38911, #10758 ) ;
#84529=DIRECTION ( 'NONE',  ( 0.000000000000000000, 1.000000000000000000, 0.000000000000000000 ) ) ;
#84531=CARTESIAN_POINT ( 'NONE',  ( 107.2329094490511068, -25.63056496568808029, 80.07657765686299456 ) ) ;
#84533=CARTESIAN_POINT ( 'NONE',  ( 131.4308125312103641, -19.51428458726955739, 6.911392308671674201 ) ) ;
#84534=ORIENTED_EDGE ( 'NONE', *, *, #67949, .T. ) ;
#84535=CARTESIAN_POINT ( 'NONE',  ( 111.0682029062220266, -27.51397330308390465, 275.7507068285485730 ) ) ;
#84536=ORIENTED_EDGE ( 'NONE', *, *, #82410, .T. ) ;
#84537=CARTESIAN_POINT ( 'NONE',  ( 80.06648329127398256, -8.729447159941058132, 4.925625275910944012 ) ) ;
#84538=ORIENTED_EDGE ( 'NONE', *, *, #72286, .T. ) ;
#84539=DIRECTION ( 'NONE',  ( -0.7071067811865774377, 0.7071067811865175967, -7.071067811865470403E-16 ) ) ;
#84540=CARTESIAN_POINT ( 'NONE',  ( 117.0714725379134364, -35.45898311558699589, 274.9271173339710117 ) ) ;
#84541=ADVANCED_FACE ( 'NONE', ( #79431 ), #78087, .T. ) ;
#84542=CARTESIAN_POINT ( 'NONE',  ( 57.56670390244832447, -48.82844715994039575, 259.7178068554150627 ) ) ;
#84544=CARTESIAN_POINT ( 'NONE',  ( 101.7446525173404979, -27.01484174591878329, 100.4632443235299633 ) ) ;
#84545=( NAMED_UNIT ( * ) PLANE_ANGLE_UNIT ( ) SI_UNIT ( $, .RADIAN. ) );
#84546=CARTESIAN_POINT ( 'NONE',  ( 97.33772238324482373, -34.07151022348116243, 166.1148286285612414 ) ) ;
#84548=EDGE_CURVE ( 'NONE', #5714, #70652, #23130, .T. ) ;
#84549=DIRECTION ( 'NONE',  ( -0.0001713722456143218888, 0.9999999853157766072, 0.000000000000000000 ) ) ;
#84550=CARTESIAN_POINT ( 'NONE',  ( 117.0608945229600408, -38.08045312664489757, 143.7189586087818896 ) ) ;
#84551=EDGE_LOOP ( 'NONE', ( #68195, #82416 ) ) ;
#84553=CARTESIAN_POINT ( 'NONE',  ( 36.23715912545429063, -47.82818131006125384, 249.9678068554150343 ) ) ;
#84554=CARTESIAN_POINT ( 'NONE',  ( 98.34985896237778036, -31.65658472535170276, 155.9064586015307157 ) ) ;
#84555=DIRECTION ( 'NONE',  ( 0.000000000000000000, -1.000000000000000000, 0.000000000000000000 ) ) ;
#84556=CARTESIAN_POINT ( 'NONE',  ( 97.59729452806701033, -30.98317272244041121, 121.8803871806729546 ) ) ;
#84558=CARTESIAN_POINT ( 'NONE',  ( 177.3246001664175537, -48.34074026909178912, 129.9678068554150059 ) ) ;
#84560=AXIS2_PLACEMENT_3D ( 'NONE', #41325, #69054, #20464 ) ;
#84563=CARTESIAN_POINT ( 'NONE',  ( 50.87649884952499946, -33.54226604284930602, -5.074374724088000832 ) ) ;
#84564=CARTESIAN_POINT ( 'NONE',  ( 114.0663967180212950, -29.08153105160607410, 150.4746728949579619 ) ) ;
#84566=EDGE_LOOP ( 'NONE', ( #46180, #40025, #58320, #78164 ) ) ;
#84567=CARTESIAN_POINT ( 'NONE',  ( 113.7419942178972576, -29.10023054337259296, 285.5032443235299979 ) ) ;
#84568=DIRECTION ( 'NONE',  ( -0.7071067811865774377, 0.7071067811865175967, -7.071067811865782003E-16 ) ) ;
#84569=DIRECTION ( 'NONE',  ( 0.000000000000000000, 0.000000000000000000, -1.000000000000000000 ) ) ;
#84570=DIRECTION ( 'NONE',  ( 0.000000000000000000, 0.000000000000000000, 1.000000000000000000 ) ) ;
#84571=DIRECTION ( 'NONE',  ( 9.351236661543306751E-17, -3.725950533538267725E-29, -1.000000000000000000 ) ) ;
#84572=ADVANCED_FACE ( 'NONE', ( #50804 ), #78978, .T. ) ;
#84573=CARTESIAN_POINT ( 'NONE',  ( 51.03742451361402743, -23.42844715994066362, 313.9678068554150059 ) ) ;
#84574=CARTESIAN_POINT ( 'NONE',  ( 105.2318265017783716, -27.12228994480470945, 235.2270538473399313 ) ) ;
#84576=ORIENTED_EDGE ( 'NONE', *, *, #67396, .F. ) ;
#84577=CARTESIAN_POINT ( 'NONE',  ( 108.4114243528872095, -27.43637152299345061, 146.4053928297069547 ) ) ;
#84578=AXIS2_PLACEMENT_3D ( 'NONE', #79389, #85319, #2633 ) ;
#84580=CARTESIAN_POINT ( 'NONE',  ( 104.6647032408819200, -45.25937870008434771, 18.79015473446898810 ) ) ;
#84583=DIRECTION ( 'NONE',  ( 3.999999999999999995E-14, -1.000000000000000000, 4.100000000000000342E-29 ) ) ;
#84584=DIRECTION ( 'NONE',  ( 0.000000000000000000, 0.000000000000000000, 1.000000000000000000 ) ) ;
#84585=CARTESIAN_POINT ( 'NONE',  ( 194.0371591254573502, -24.42818131005417825, 236.4678068554149775 ) ) ;
#84586=CARTESIAN_POINT ( 'NONE',  ( 97.75833061367904975, -40.38474740428294751, 37.62395470578984913 ) ) ;
#84587=CARTESIAN_POINT ( 'NONE',  ( 110.2492204789523242, -26.78788743924345184, 234.8299109901969643 ) ) ;
#84590=EDGE_CURVE ( 'NONE', #43506, #44014, #71272, .T. ) ;
#84594=CYLINDRICAL_SURFACE ( 'NONE', #62099, 9.999999999999998224 ) ;
#84596=CARTESIAN_POINT ( 'NONE',  ( 114.9268010244024225, -42.60560063232393446, 24.31562527591096767 ) ) ;
#84599=CARTESIAN_POINT ( 'NONE',  ( 96.64260770218685082, -42.46999856532355011, 22.72705384733997391 ) ) ;
#84602=CARTESIAN_POINT ( 'NONE',  ( 112.6638099339533028, -45.52472799210174514, 263.0270538473394595 ) ) ;
#84603=ORIENTED_EDGE ( 'NONE', *, *, #82656, .T. ) ;
#84604=EDGE_CURVE ( 'NONE', #88157, #68103, #43077, .T. ) ;
#84605=AXIS2_PLACEMENT_3D ( 'NONE', #2101, #44754, #58390 ) ;
#84606=CARTESIAN_POINT ( 'NONE',  ( 77.97204591016883057, -38.52018918693340055, 7.480061334638488546 ) ) ;
#84607=DIRECTION ( 'NONE',  ( -4.237773401492740281E-14, 1.000000000000000000, 0.000000000000000000 ) ) ;
#84608=ADVANCED_FACE ( 'NONE', ( #70816 ), #1778, .T. ) ;
#84609=DIRECTION ( 'NONE',  ( 3.999999999999999995E-14, -1.000000000000000000, 4.100000000000000342E-29 ) ) ;
#84610=EDGE_CURVE ( 'NONE', #48706, #29859, #12492, .T. ) ;
#84611=CARTESIAN_POINT ( 'NONE',  ( 113.0992926495536182, -42.93477843977468922, 116.0204713219719679 ) ) ;
#84612=CARTESIAN_POINT ( 'NONE',  ( 106.9748050991984059, -47.17592283179411083, 183.5699109901969734 ) ) ;
#84614=EDGE_LOOP ( 'NONE', ( #6715, #45135, #25785, #21694 ) ) ;
#84615=EDGE_CURVE ( 'NONE', #51989, #25435, #16298, .T. ) ;
#84616=DIRECTION ( 'NONE',  ( 1.000000000000000078E-15, -1.000000000000000083E-30, -1.000000000000000000 ) ) ;
#84618=ORIENTED_EDGE ( 'NONE', *, *, #18183, .F. ) ;
#84620=CARTESIAN_POINT ( 'NONE',  ( 140.9629299006807059, -46.47944715994099596, 14.92562527591100618 ) ) ;
#84621=ORIENTED_EDGE ( 'NONE', *, *, #43528, .F. ) ;
#84622=VERTEX_POINT ( 'NONE', #71710 ) ;
#84623=CARTESIAN_POINT ( 'NONE',  ( 117.0715500276773184, -35.45963891618318797, 169.9274906265435732 ) ) ;
#84624=CARTESIAN_POINT ( 'NONE',  ( 103.2832018370665565, -27.47273118576459794, 41.38522229241210226 ) ) ;
#84625=CARTESIAN_POINT ( 'NONE',  ( 115.5717340297064197, -37.51483979961712123, 78.17527697093396455 ) ) ;
#84626=CARTESIAN_POINT ( 'NONE',  ( 117.5411534933602837, -36.54545762053501079, 288.8413395616251478 ) ) ;
#84629=ORIENTED_EDGE ( 'NONE', *, *, #79687, .F. ) ;
#84630=ORIENTED_EDGE ( 'NONE', *, *, #41118, .F. ) ;
#84633=DIRECTION ( 'NONE',  ( 0.000000000000000000, 0.000000000000000000, 1.000000000000000000 ) ) ;
#84634=CARTESIAN_POINT ( 'NONE',  ( 99.54941199951403519, -42.98700854487248080, 116.8784824187689679 ) ) ;
#84635=VECTOR ( 'NONE', #53862, 1000.000000000000000 ) ;
#84636=CARTESIAN_POINT ( 'NONE',  ( 101.4772741282170472, -27.87691040622789274, 110.5241967044819944 ) ) ;
#84638=ORIENTED_EDGE ( 'NONE', *, *, #43205, .T. ) ;
#84639=CARTESIAN_POINT ( 'NONE',  ( 100.2480723708022197, -28.84298388537911606, 260.6441967044822263 ) ) ;
#84640=FACE_OUTER_BOUND ( 'NONE', #18215, .T. ) ;
#84641=AXIS2_PLACEMENT_3D ( 'NONE', #83267, #13767, #14220 ) ;
#84642=CARTESIAN_POINT ( 'NONE',  ( 97.84512178009099159, -40.59816388786018138, 27.64300878097207814 ) ) ;
#84644=DIRECTION ( 'NONE',  ( -4.237773401492740281E-14, 1.000000000000000000, 0.000000000000000000 ) ) ;
#84645=CARTESIAN_POINT ( 'NONE',  ( 105.1754357245111180, -25.42735205269929821, 322.5490683446364528 ) ) ;
#84647=DIRECTION ( 'NONE',  ( 0.7071067811861589947, -0.7071067811869361508, 0.000000000000000000 ) ) ;
#84649=DIRECTION ( 'NONE',  ( 0.000000000000000000, 0.000000000000000000, 1.000000000000000000 ) ) ;
#84650=CARTESIAN_POINT ( 'NONE',  ( 100.3567573962561710, -39.47573163423117393, -2.114374724089040924 ) ) ;
#84651=CARTESIAN_POINT ( 'NONE',  ( 37.36643805256573359, -48.62818131006097389, 129.9678068554150911 ) ) ;
#84652=ORIENTED_EDGE ( 'NONE', *, *, #36573, .T. ) ;
#84654=CARTESIAN_POINT ( 'NONE',  ( 103.9326413674837539, -26.76323430032771000, 250.3184824187677577 ) ) ;
#84655=CARTESIAN_POINT ( 'NONE',  ( 97.42522746746806206, -42.13501527293522742, 177.7451490854349743 ) ) ;
#84656=CARTESIAN_POINT ( 'NONE',  ( 115.4621199703947241, -43.00579008905405232, 24.31562527591096767 ) ) ;
#84657=FACE_OUTER_BOUND ( 'NONE', #71539, .T. ) ;
#84658=CARTESIAN_POINT ( 'NONE',  ( 82.81648124396181743, -36.63640413216758418, 6.749771997051381867 ) ) ;
#84660=EDGE_CURVE ( 'NONE', #18083, #81364, #28436, .T. ) ;
#84661=VECTOR ( 'NONE', #88456, 1000.000000000000000 ) ;
#84663=EDGE_CURVE ( 'NONE', #11696, #55509, #30812, .T. ) ;
#84664=DIRECTION ( 'NONE',  ( 9.351236661543306751E-17, -3.725950533538267725E-29, -1.000000000000000000 ) ) ;
#84666=CARTESIAN_POINT ( 'NONE',  ( 99.85230398470191915, -41.30238370604462261, 186.1981341137909567 ) ) ;
#84668=CARTESIAN_POINT ( 'NONE',  ( 108.3302456646921144, -46.73522246767858945, 187.6775912052179081 ) ) ;
#84669=ORIENTED_EDGE ( 'NONE', *, *, #23869, .T. ) ;
#84670=VECTOR ( 'NONE', #5796, 1000.000000000000000 ) ;
#84672=CARTESIAN_POINT ( 'NONE',  ( 113.0129699484215564, -46.01939436189636012, 214.0175300378159591 ) ) ;
#84673=CARTESIAN_POINT ( 'NONE',  ( 194.5667039024482108, -40.82844715993405060, 180.4678068554150343 ) ) ;
#84674=DIRECTION ( 'NONE',  ( 0.000000000000000000, -1.000000000000000000, 0.000000000000000000 ) ) ;
#84679=CARTESIAN_POINT ( 'NONE',  ( 97.81168883536605563, -40.51740680051663190, 96.63562987897269352 ) ) ;
#84680=CARTESIAN_POINT ( 'NONE',  ( 102.0112516875887252, -27.67497761899947406, 105.4937205140069665 ) ) ;
#84681=VERTEX_POINT ( 'NONE', #25780 ) ;
#84682=ORIENTED_EDGE ( 'NONE', *, *, #67522, .T. ) ;
#84685=CARTESIAN_POINT ( 'NONE',  ( 98.21780894689015895, -37.20823830323941905, 72.80158330589698323 ) ) ;
#84686=EDGE_CURVE ( 'NONE', #83131, #54506, #74862, .T. ) ;
#84688=CARTESIAN_POINT ( 'NONE',  ( 100.4443968677459935, -27.79860430499269697, 181.5841967044819683 ) ) ;
#84689=CARTESIAN_POINT ( 'NONE',  ( 116.8171228645041140, -34.15291831569319214, 39.03145860967040193 ) ) ;
#84690=DIRECTION ( 'NONE',  ( -1.000000000000000078E-15, 1.000000000000000000, 0.000000000000000000 ) ) ;
#84691=ADVANCED_FACE ( 'NONE', ( #318 ), #68014, .F. ) ;
#84693=DIRECTION ( 'NONE',  ( -0.7071067811865779928, 0.7071067811865171526, -7.071067811865475333E-16 ) ) ;
#84694=DIRECTION ( 'NONE',  ( 0.9825752044328148749, 0.1858654557302456822, 0.000000000000000000 ) ) ;
#84695=CARTESIAN_POINT ( 'NONE',  ( 179.8585841295805778, -30.08671355699668837, 237.4678068554150059 ) ) ;
#84696=ADVANCED_FACE ( 'NONE', ( #13060 ), #20329, .T. ) ;
#84697=CARTESIAN_POINT ( 'NONE',  ( 116.9011659702704264, -33.23038410113876040, 114.0984824187679720 ) ) ;
#84698=ORIENTED_EDGE ( 'NONE', *, *, #24812, .F. ) ;
#84700=EDGE_CURVE ( 'NONE', #14757, #28401, #18312, .T. ) ;
#84704=CARTESIAN_POINT ( 'NONE',  ( 109.6430121197684571, -46.48008673816740099, 78.78145860836009717 ) ) ;
#84706=CARTESIAN_POINT ( 'NONE',  ( 98.93571844094823575, -36.00806725600566693, 229.0738046553059633 ) ) ;
#84709=CARTESIAN_POINT ( 'NONE',  ( 113.8435853237685933, -28.76095960330615142, 139.5156252759109634 ) ) ;
#84711=DIRECTION ( 'NONE',  ( 0.000000000000000000, 1.000000000000000000, 0.000000000000000000 ) ) ;
#84715=EDGE_CURVE ( 'NONE', #45258, #4000, #37133, .T. ) ;
#84717=ORIENTED_EDGE ( 'NONE', *, *, #87034, .T. ) ;
#84718=ORIENTED_EDGE ( 'NONE', *, *, #36957, .T. ) ;
#84719=DIRECTION ( 'NONE',  ( -0.9999999853157766072, -0.0001713722456150811827, 0.000000000000000000 ) ) ;
#84721=DIRECTION ( 'NONE',  ( -1.000000000000000078E-15, 1.000000000000000083E-30, 1.000000000000000000 ) ) ;
#84723=CARTESIAN_POINT ( 'NONE',  ( 104.4082965424966147, -28.27590814835049926, 246.7501547344679693 ) ) ;
#84724=DIRECTION ( 'NONE',  ( 1.000000000000000000, 3.552853285012605541E-15, 0.000000000000000000 ) ) ;
#84725=EDGE_LOOP ( 'NONE', ( #43100, #22753, #27609, #43778 ) ) ;
#84727=CARTESIAN_POINT ( 'NONE',  ( 113.6715427071513318, -42.59351399727410126, 9.635625275910943088 ) ) ;
#84729=EDGE_LOOP ( 'NONE', ( #8495, #63515, #74075, #25288 ) ) ;
#84732=CARTESIAN_POINT ( 'NONE',  ( 152.0368932755772562, -23.42844715993587812, 193.9678068554149775 ) ) ;
#84733=AXIS2_PLACEMENT_3D ( 'NONE', #21250, #69402, #68950 ) ;
#84735=ORIENTED_EDGE ( 'NONE', *, *, #40174, .T. ) ;
#84736=AXIS2_PLACEMENT_3D ( 'NONE', #53406, #73882, #80275 ) ;
#84737=CARTESIAN_POINT ( 'NONE',  ( 98.59685088459899305, -34.95005064942726136, 258.9918998934010119 ) ) ;
#84738=CARTESIAN_POINT ( 'NONE',  ( 113.5789493677227711, -44.94383383376451491, 168.1099109901969939 ) ) ;
#84739=CARTESIAN_POINT ( 'NONE',  ( 117.6568287320716877, -39.81301747186228113, 138.5889586092439743 ) ) ;
#84740=CARTESIAN_POINT ( 'NONE',  ( 116.3916404119186154, -39.77162857537385321, 249.5838068554167819 ) ) ;
#84741=CARTESIAN_POINT ( 'NONE',  ( 107.2431676328701684, -47.18842012194354396, 208.5899109901969837 ) ) ;
#84742=DIRECTION ( 'NONE',  ( 0.000000000000000000, 0.000000000000000000, 1.000000000000000000 ) ) ;
#84743=FACE_OUTER_BOUND ( 'NONE', #75398, .T. ) ;
#84744=VERTEX_POINT ( 'NONE', #61191 ) ;
#84748=CARTESIAN_POINT ( 'NONE',  ( 117.9786848761844453, -34.69554937534774552, 203.9851490854349549 ) ) ;
#84749=ORIENTED_EDGE ( 'NONE', *, *, #47846, .F. ) ;
#84750=CARTESIAN_POINT ( 'NONE',  ( 109.5085389712880612, -46.86470218963918200, 132.7641967044819751 ) ) ;
#84754=DIRECTION ( 'NONE',  ( -6.524622321627019585E-16, -4.013151879589939944E-16, -1.000000000000000000 ) ) ;
#84755=CARTESIAN_POINT ( 'NONE',  ( 109.3947377649931383, -46.48697826211399331, 57.76270257490259041 ) ) ;
#84756=CARTESIAN_POINT ( 'NONE',  ( 96.83034234600431489, -40.83861266248838007, 247.6422919425769749 ) ) ;
#84758=CARTESIAN_POINT ( 'NONE',  ( 164.7812970173265512, -35.65087443490954655, 342.9256252759109884 ) ) ;
#84760=DIRECTION ( 'NONE',  ( -1.000000000000000000, 6.745093096447288888E-17, -2.283216351027200160E-14 ) ) ;
#84763=CARTESIAN_POINT ( 'NONE',  ( 113.7843247631140571, -29.05179538500707892, 289.5032443235299979 ) ) ;
#84764=ORIENTED_EDGE ( 'NONE', *, *, #12685, .F. ) ;
#84766=CARTESIAN_POINT ( 'NONE',  ( 117.7261736041901372, -39.74048882516440528, 143.6194347997209775 ) ) ;
#84767=CARTESIAN_POINT ( 'NONE',  ( 115.2670960386832775, -44.14051530504124088, 79.25372051400697160 ) ) ;
#84768=CARTESIAN_POINT ( 'NONE',  ( 114.9980252723336207, -29.89690579156949823, 180.3927681330539770 ) ) ;
#84770=CARTESIAN_POINT ( 'NONE',  ( 182.0374245136174522, -23.42844715993458848, 180.4678068554150343 ) ) ;
#84773=CARTESIAN_POINT ( 'NONE',  ( 116.3201356630459884, -32.94258242523766711, 69.13562527591093954 ) ) ;
#84774=CARTESIAN_POINT ( 'NONE',  ( 134.0664832912740110, -8.350947159940998787, 311.1531252759119752 ) ) ;
#84775=ORIENTED_EDGE ( 'NONE', *, *, #19874, .T. ) ;
#84776=AXIS2_PLACEMENT_3D ( 'NONE', #81853, #60022, #46839 ) ;
#84778=AXIS2_PLACEMENT_3D ( 'NONE', #62362, #15120, #21040 ) ;
#84779=EDGE_CURVE ( 'NONE', #83074, #36953, #29940, .T. ) ;
#84782=VERTEX_POINT ( 'NONE', #83442 ) ;
#84783=ADVANCED_FACE ( 'NONE', ( #47553 ), #61631, .F. ) ;
#84785=EDGE_LOOP ( 'NONE', ( #47568, #86886, #19336, #87026 ) ) ;
#84786=CARTESIAN_POINT ( 'NONE',  ( 113.4461594614341209, -46.68675298423766407, 64.02991099019695298 ) ) ;
#84787=PLANE ( 'NONE',  #84605 ) ;
#84790=CARTESIAN_POINT ( 'NONE',  ( 97.38492667529318680, -42.15761073986299579, 177.7451490854349743 ) ) ;
#84791=CARTESIAN_POINT ( 'NONE',  ( 99.00226700525801959, -39.63126001020209799, 266.0238483995056527 ) ) ;
#84792=VERTEX_POINT ( 'NONE', #13504 ) ;
#84794=ORIENTED_EDGE ( 'NONE', *, *, #33440, .F. ) ;
#84797=CIRCLE ( 'NONE', #80430, 5.499999999999999112 ) ;
#84799=CARTESIAN_POINT ( 'NONE',  ( 141.0667039024479834, -48.82844715994099971, 198.9178068554149945 ) ) ;
#84800=FACE_OUTER_BOUND ( 'NONE', #22641, .T. ) ;
#84801=VECTOR ( 'NONE', #40248, 1000.000000000000000 ) ;
#84802=CARTESIAN_POINT ( 'NONE',  ( 100.9552960800314310, -28.70654040160240328, 20.59290076991167595 ) ) ;
#84805=DIRECTION ( 'NONE',  ( -1.000000000000000078E-15, 0.000000000000000000, -1.000000000000000000 ) ) ;
#84807=DIRECTION ( 'NONE',  ( 0.000000000000000000, 0.000000000000000000, -1.000000000000000000 ) ) ;
#84808=CARTESIAN_POINT ( 'NONE',  ( 104.7405551043178491, -47.51155644559854352, 32.41943479972098174 ) ) ;
#84811=DIRECTION ( 'NONE',  ( 0.000000000000000000, 1.000000000000000000, 0.000000000000000000 ) ) ;
#84812=CARTESIAN_POINT ( 'NONE',  ( 154.4439038579832300, -17.91479848270203945, 396.9756252759102040 ) ) ;
#84813=CARTESIAN_POINT ( 'NONE',  ( 116.3348466390194460, -36.28970630669515174, 116.6823760838769601 ) ) ;
#84815=CARTESIAN_POINT ( 'NONE',  ( 97.81135238452728231, -40.51660343587602142, 96.63555416999651015 ) ) ;
#84816=CARTESIAN_POINT ( 'NONE',  ( 37.56670390244806157, -48.82844715994099971, 300.4678068554150059 ) ) ;
#84817=VERTEX_POINT ( 'NONE', #18347 ) ;
#84818=ORIENTED_EDGE ( 'NONE', *, *, #78989, .T. ) ;
#84819=CARTESIAN_POINT ( 'NONE',  ( 101.9936818365031144, -45.44611147528136286, 137.1550710178724444 ) ) ;
#84820=VERTEX_POINT ( 'NONE', #39683 ) ;
#84821=VERTEX_POINT ( 'NONE', #19697 ) ;
#84822=CARTESIAN_POINT ( 'NONE',  ( 97.47186360698646013, -39.79766782782348855, 128.0044404487539396 ) ) ;
#84824=EDGE_CURVE ( 'NONE', #78010, #58653, #40587, .T. ) ;
#84825=CARTESIAN_POINT ( 'NONE',  ( 101.6996507173639088, -27.72520905039313632, 81.50419670448295051 ) ) ;
#84826=AXIS2_PLACEMENT_3D ( 'NONE', #6548, #69227, #47863 ) ;
#84827=CARTESIAN_POINT ( 'NONE',  ( 110.9020743365320243, -45.96463798019833291, 17.88972164584141566 ) ) ;
#84829=VECTOR ( 'NONE', #40372, 1000.000000000000000 ) ;
#84832=CARTESIAN_POINT ( 'NONE',  ( 113.4731498177359725, -46.72887913999166898, 68.02991099019695298 ) ) ;
#84834=CARTESIAN_POINT ( 'NONE',  ( 105.1480534446306621, -26.53835310083740850, 280.2365776568638580 ) ) ;
#84835=CARTESIAN_POINT ( 'NONE',  ( 95.88671040095643150, -32.72508343906864781, 172.0527681330539735 ) ) ;
#84836=CARTESIAN_POINT ( 'NONE',  ( 99.66264782090949836, -39.75983002812326106, 9.635625275910941312 ) ) ;
#84838=CARTESIAN_POINT ( 'NONE',  ( 117.2094703596446550, -39.28701360234872197, 119.6299109901969615 ) ) ;
#84839=DIRECTION ( 'NONE',  ( 0.000000000000000000, 0.000000000000000000, 1.000000000000000000 ) ) ;
#84845=EDGE_LOOP ( 'NONE', ( #17215, #75822 ) ) ;
#84847=ADVANCED_FACE ( 'NONE', ( #81949 ), #5179, .F. ) ;
#84853=CARTESIAN_POINT ( 'NONE',  ( 117.5124197103495050, -37.28486668576427121, 18.78419670448294809 ) ) ;
#84855=AXIS2_PLACEMENT_3D ( 'NONE', #39215, #66924, #32845 ) ;
#84858=CARTESIAN_POINT ( 'NONE',  ( 103.8130989789263197, -45.95327097697902730, 57.30705384734097407 ) ) ;
#84859=CARTESIAN_POINT ( 'NONE',  ( 172.5664832912740110, -32.07844715994070839, 263.6756252759120116 ) ) ;
#84860=CARTESIAN_POINT ( 'NONE',  ( 108.9412587213990804, -26.46057952311826611, 160.9327681330539690 ) ) ;
#84861=CARTESIAN_POINT ( 'NONE',  ( 98.34985890762048655, -31.65658481782444156, 71.90645861000221828 ) ) ;
#84862=CARTESIAN_POINT ( 'NONE',  ( 194.0371591254574923, -24.42818131005417115, 193.9678068554150343 ) ) ;
#84864=LINE ( 'NONE', #84420, #59884 ) ;
#84865=AXIS2_PLACEMENT_3D ( 'NONE', #58254, #85984, #3302 ) ;
#84866=CIRCLE ( 'NONE', #77587, 2.750000000000002665 ) ;
#84867=CARTESIAN_POINT ( 'NONE',  ( 73.17003668186730181, -46.47944715994106701, 14.92562527591093691 ) ) ;
#84871=CARTESIAN_POINT ( 'NONE',  ( 108.6818361061225602, -26.38549717321916788, 189.9527681330539792 ) ) ;
#84874=CARTESIAN_POINT ( 'NONE',  ( 102.2271567091324158, -45.98785831331388607, 208.1927681330539599 ) ) ;
#84875=CARTESIAN_POINT ( 'NONE',  ( 117.6393638915270827, -42.19070237429166070, 89.44705384733997278 ) ) ;
#84876=CARTESIAN_POINT ( 'NONE',  ( 115.8281814319410046, -31.73477621452418873, 250.2407391550281943 ) ) ;
#84879=VERTEX_POINT ( 'NONE', #46035 ) ;
#84881=EDGE_CURVE ( 'NONE', #62879, #72320, #5637, .T. ) ;
#84882=ORIENTED_EDGE ( 'NONE', *, *, #38599, .T. ) ;
#84884=ORIENTED_EDGE ( 'NONE', *, *, #68252, .T. ) ;
#84886=VERTEX_POINT ( 'NONE', #66954 ) ;
#84887=CARTESIAN_POINT ( 'NONE',  ( 182.5667039024480118, -32.29483332968430886, 342.9256252759109884 ) ) ;
#84888=CARTESIAN_POINT ( 'NONE',  ( 96.51815522165868799, -31.32876289826797134, 241.9499109901969689 ) ) ;
#84889=DIRECTION ( 'NONE',  ( 1.000000000000000000, 1.374769042280159607E-11, 0.000000000000000000 ) ) ;
#84891=EDGE_CURVE ( 'NONE', #41960, #56128, #60312, .T. ) ;
#84892=LINE ( 'NONE', #22661, #3285 ) ;
#84895=CARTESIAN_POINT ( 'NONE',  ( 106.2504075017224210, -26.27849585604564098, 25.13848241876792855 ) ) ;
#84898=VECTOR ( 'NONE', #86167, 1000.000000000000000 ) ;
#84900=EDGE_CURVE ( 'NONE', #13709, #68878, #47284, .T. ) ;
#84901=DIRECTION ( 'NONE',  ( 0.7071067811575898476, -0.7071067812155052978, 0.000000000000000000 ) ) ;
#84904=CARTESIAN_POINT ( 'NONE',  ( 113.9608400058609874, -28.00707201209563024, 270.5441967044819194 ) ) ;
#84906=DIRECTION ( 'NONE',  ( 1.000000000000000078E-15, 1.000000000000000083E-30, -1.000000000000000000 ) ) ;
#84907=CARTESIAN_POINT ( 'NONE',  ( 99.54941199951412045, -42.98700854487240974, 112.8784824187679732 ) ) ;
#84910=CARTESIAN_POINT ( 'NONE',  ( 143.9834832912729894, -71.52944715994142655, 361.9756252759109998 ) ) ;
#84911=DIRECTION ( 'NONE',  ( 0.000000000000000000, 0.000000000000000000, 1.000000000000000000 ) ) ;
#84912=ORIENTED_EDGE ( 'NONE', *, *, #54097, .T. ) ;
#84913=ORIENTED_EDGE ( 'NONE', *, *, #57790, .F. ) ;
#84915=CARTESIAN_POINT ( 'NONE',  ( 114.9297498758896126, -40.81563990160193356, 284.8758690201828472 ) ) ;
#84916=AXIS2_PLACEMENT_3D ( 'NONE', #40521, #33715, #50915 ) ;
#84919=AXIS2_PLACEMENT_3D ( 'NONE', #47697, #49493, #70414 ) ;
#84920=PLANE ( 'NONE',  #72272 ) ;
#84921=DIRECTION ( 'NONE',  ( -0.9254794337955623007, -0.3787978585227819162, 0.000000000000000000 ) ) ;
#84924=DIRECTION ( 'NONE',  ( 0.000000000000000000, 0.000000000000000000, -1.000000000000000000 ) ) ;
#84925=DIRECTION ( 'NONE',  ( -1.000000000000000078E-15, 1.000000000000000083E-30, 1.000000000000000000 ) ) ;
#84926=EDGE_LOOP ( 'NONE', ( #47146, #61952, #83749, #59335 ) ) ;
#84927=CARTESIAN_POINT ( 'NONE',  ( 96.03551326368828711, -41.06051932364815826, 96.62419670448197451 ) ) ;
#84928=VERTEX_POINT ( 'NONE', #18805 ) ;
#84929=CARTESIAN_POINT ( 'NONE',  ( 100.5619151801845419, -43.03049977154007166, 41.37337220902998070 ) ) ;
#84932=CARTESIAN_POINT ( 'NONE',  ( 99.18511857479137461, -30.88155312011791409, 180.8184824187689799 ) ) ;
#84934=LINE ( 'NONE', #57187, #53182 ) ;
#84935=FACE_OUTER_BOUND ( 'NONE', #75312, .T. ) ;
#84938=CIRCLE ( 'NONE', #5098, 2.517499999999998739 ) ;
#84939=CARTESIAN_POINT ( 'NONE',  ( 115.7313686325390876, -42.60420177353093862, 269.3527681330536439 ) ) ;
#84942=LINE ( 'NONE', #907, #18284 ) ;
#84944=CARTESIAN_POINT ( 'NONE',  ( 109.2103426150987104, -26.48265019188898606, 135.9127681330539872 ) ) ;
#84945=FACE_OUTER_BOUND ( 'NONE', #17965, .T. ) ;
#84946=ORIENTED_EDGE ( 'NONE', *, *, #38644, .F. ) ;
#84947=ORIENTED_EDGE ( 'NONE', *, *, #79264, .T. ) ;
#84949=DIRECTION ( 'NONE',  ( 1.000000000000000000, 0.000000000000000000, 0.000000000000000000 ) ) ;
#84950=CARTESIAN_POINT ( 'NONE',  ( 116.3251085584666527, -32.94148239642360210, 265.1356252759109680 ) ) ;
#84953=DIRECTION ( 'NONE',  ( 0.000000000000000000, 0.000000000000000000, 1.000000000000000000 ) ) ;
#84954=CARTESIAN_POINT ( 'NONE',  ( 100.4110913530865332, -28.70521849941338033, 36.62705384733894221 ) ) ;
#84956=ORIENTED_EDGE ( 'NONE', *, *, #42698, .T. ) ;
#84958=CARTESIAN_POINT ( 'NONE',  ( 84.06648329127399677, -18.82844715994099971, 199.5838068554169524 ) ) ;
#84961=AXIS2_PLACEMENT_3D ( 'NONE', #52715, #53621, #4614 ) ;
#84962=ADVANCED_FACE ( 'NONE', ( #12001 ), #46932, .T. ) ;
#84964=CARTESIAN_POINT ( 'NONE',  ( 191.6375511031384633, -78.44951497180814215, 342.9256252759109884 ) ) ;
#84965=VECTOR ( 'NONE', #53306, 1000.000000000000000 ) ;
#84967=PLANE ( 'NONE',  #36165 ) ;
#84968=DIRECTION ( 'NONE',  ( -1.000000000000000078E-15, 1.000000000000000083E-30, 1.000000000000000000 ) ) ;
#84969=CARTESIAN_POINT ( 'NONE',  ( 105.4642979808546670, -28.33962392264099250, 234.6495626852199621 ) ) ;
#84970=CARTESIAN_POINT ( 'NONE',  ( 61.68306511546570903, -72.55869591834559174, 542.9756252759101471 ) ) ;
#84971=CARTESIAN_POINT ( 'NONE',  ( 97.30890135812539654, -33.12136451854836849, 62.04419670448196911 ) ) ;
#84973=CARTESIAN_POINT ( 'NONE',  ( 117.9021936627155895, -39.13782096276514721, 103.6403871806729455 ) ) ;
#84977=DIRECTION ( 'NONE',  ( 1.000000000000000078E-15, -1.000000000000000083E-30, -1.000000000000000000 ) ) ;
#84980=LINE ( 'NONE', #10003, #11374 ) ;
#84982=LINE ( 'NONE', #71788, #40656 ) ;
#84983=CARTESIAN_POINT ( 'NONE',  ( 63.03715912545646205, -24.89890238295017255, 129.9678068554150911 ) ) ;
#84984=CARTESIAN_POINT ( 'NONE',  ( 76.06670390244805446, -58.72944715994109544, 239.5838068554169809 ) ) ;
#84985=AXIS2_PLACEMENT_3D ( 'NONE', #44532, #8250, #10042 ) ;
#84987=CARTESIAN_POINT ( 'NONE',  ( 113.3557719660652339, -27.61131746675945209, 89.60800622829195561 ) ) ;
#84988=VECTOR ( 'NONE', #86891, 1000.000000000000000 ) ;
#84989=VECTOR ( 'NONE', #5689, 1000.000000000000000 ) ;
#84990=AXIS2_PLACEMENT_3D ( 'NONE', #74390, #38509, #18974 ) ;
#84991=CARTESIAN_POINT ( 'NONE',  ( 172.5664832912740110, -36.32844715994070839, 78.92562527591199739 ) ) ;
#84993=FACE_OUTER_BOUND ( 'NONE', #71413, .T. ) ;
#84996=EDGE_CURVE ( 'NONE', #75042, #76300, #46891, .T. ) ;
#84998=CARTESIAN_POINT ( 'NONE',  ( 34.96670390244699433, -28.27351298637401200, -5.074374724088000832 ) ) ;
#85002=CARTESIAN_POINT ( 'NONE',  ( 107.9474582775578568, -25.68820226555254749, 111.0251490854349754 ) ) ;
#85003=ADVANCED_FACE ( 'NONE', ( #64713 ), #2935, .T. ) ;
#85005=PLANE ( 'NONE',  #55744 ) ;
#85006=DIRECTION ( 'NONE',  ( 0.000000000000000000, 0.000000000000000000, 1.000000000000000000 ) ) ;
#85007=VECTOR ( 'NONE', #3659, 1000.000000000000114 ) ;
#85010=CARTESIAN_POINT ( 'NONE',  ( 99.59366209610200826, -44.96145431533973635, 152.9899109901959946 ) ) ;
#85011=EDGE_CURVE ( 'NONE', #21358, #66312, #61814, .T. ) ;
#85014=CARTESIAN_POINT ( 'NONE',  ( 101.7353989658871853, -28.52926574618699362, 21.53562527591096298 ) ) ;
#85015=DIRECTION ( 'NONE',  ( 0.000000000000000000, 0.000000000000000000, -1.000000000000000000 ) ) ;
#85016=FACE_OUTER_BOUND ( 'NONE', #30772, .T. ) ;
#85019=DIRECTION ( 'NONE',  ( -1.000000000000000000, 6.745093096447288888E-17, 2.089354330573420398E-14 ) ) ;
#85020=CARTESIAN_POINT ( 'NONE',  ( 112.7271506738796347, -45.41826929060063378, 223.0480062282919675 ) ) ;
#85021=EDGE_LOOP ( 'NONE', ( #72774, #69035, #55062, #32465 ) ) ;
#85023=CARTESIAN_POINT ( 'NONE',  ( 108.0145050256332979, -45.54020952213421936, 199.0930118773259778 ) ) ;
#85025=CARTESIAN_POINT ( 'NONE',  ( 106.9482176359816634, -27.83854490981203256, 56.51872616303998598 ) ) ;
#85026=CIRCLE ( 'NONE', #15387, 1.000000000000000888 ) ;
#85028=CARTESIAN_POINT ( 'NONE',  ( 100.8872800922797239, -44.70006565411546262, 267.0523716391360267 ) ) ;
#85030=ORIENTED_EDGE ( 'NONE', *, *, #47577, .F. ) ;
#85032=FACE_OUTER_BOUND ( 'NONE', #35396, .T. ) ;
#85033=CARTESIAN_POINT ( 'NONE',  ( 95.25611604350963546, -37.33230102880722967, 271.3670538473393776 ) ) ;
#85034=CARTESIAN_POINT ( 'NONE',  ( 188.5667039024479834, -62.87844715994099687, 173.2178068554149775 ) ) ;
#85035=ORIENTED_EDGE ( 'NONE', *, *, #3428, .T. ) ;
#85036=ORIENTED_EDGE ( 'NONE', *, *, #6167, .F. ) ;
#85040=LINE ( 'NONE', #30062, #7085 ) ;
#85043=CARTESIAN_POINT ( 'NONE',  ( 115.1412022171004281, -43.23618977845870148, 39.27467289495795200 ) ) ;
#85044=VECTOR ( 'NONE', #51907, 999.9999999999997726 ) ;
#85046=ORIENTED_EDGE ( 'NONE', *, *, #50230, .F. ) ;
#85047=VECTOR ( 'NONE', #56821, 1000.000000000000000 ) ;
#85048=CARTESIAN_POINT ( 'NONE',  ( 96.29363189909904008, -41.78481911317979325, 57.67562527591096710 ) ) ;
#85049=VECTOR ( 'NONE', #1890, 1000.000000000000000 ) ;
#85053=CARTESIAN_POINT ( 'NONE',  ( 116.1776873554136813, -43.03363693755514419, 13.35657765686298859 ) ) ;
#85058=CARTESIAN_POINT ( 'NONE',  ( 107.2759047676296120, -28.56943069780466971, 117.8738046553059462 ) ) ;
#85059=CARTESIAN_POINT ( 'NONE',  ( 96.62257978078039855, -36.48017157545621814, 192.3070538473399438 ) ) ;
#85060=CYLINDRICAL_SURFACE ( 'NONE', #79791, 2.117000000000007987 ) ;
#85061=VERTEX_POINT ( 'NONE', #84732 ) ;
#85062=AXIS2_PLACEMENT_3D ( 'NONE', #9932, #84906, #85359 ) ;
#85063=CARTESIAN_POINT ( 'NONE',  ( 107.0664832912739399, -36.72944715994095333, 289.6356252759107406 ) ) ;
#85064=ORIENTED_EDGE ( 'NONE', *, *, #79133, .T. ) ;
#85067=CYLINDRICAL_SURFACE ( 'NONE', #16901, 5.599999999999994316 ) ;
#85068=VERTEX_POINT ( 'NONE', #45565 ) ;
#85069=ORIENTED_EDGE ( 'NONE', *, *, #2035, .T. ) ;
#85072=CARTESIAN_POINT ( 'NONE',  ( 105.8901181204952309, -26.78673948403035610, 41.17015456836836051 ) ) ;
#85073=CARTESIAN_POINT ( 'NONE',  ( 109.0672552851176249, -45.03324407163384535, 132.1867055423619775 ) ) ;
#85074=CARTESIAN_POINT ( 'NONE',  ( 100.8351866834200337, -45.15911532695984931, 257.0699109901966608 ) ) ;
#85075=CARTESIAN_POINT ( 'NONE',  ( 184.5667039024480118, -67.87844715994100397, 10.91780685541479734 ) ) ;
#85077=EDGE_CURVE ( 'NONE', #63620, #18180, #64812, .T. ) ;
#85079=CARTESIAN_POINT ( 'NONE',  ( 32.25690895536977365, -33.54226604285049262, 193.9678068554150911 ) ) ;
#85080=LINE ( 'NONE', #41910, #12985 ) ;
#85081=CYLINDRICAL_SURFACE ( 'NONE', #55624, 2.117000000000000881 ) ;
#85082=CARTESIAN_POINT ( 'NONE',  ( 113.3411949225463502, -28.30449682957925717, 104.5670538473399347 ) ) ;
#85083=CARTESIAN_POINT ( 'NONE',  ( 96.51917584821923413, -40.19201726479878545, 286.5908633711491120 ) ) ;
#85084=EDGE_LOOP ( 'NONE', ( #41699, #59371, #73245, #46159 ) ) ;
#85086=CARTESIAN_POINT ( 'NONE',  ( 112.4894639655092305, -46.36118470102660183, 257.9965776568635647 ) ) ;
#85087=CYLINDRICAL_SURFACE ( 'NONE', #60187, 3.250000000000002665 ) ;
#85090=CARTESIAN_POINT ( 'NONE',  ( 124.0664832912757163, -36.72944715993921960, -5.074374724089012467 ) ) ;
#85091=B_SPLINE_CURVE_WITH_KNOTS ( 'NONE', 3,
 ( #51686, #79433, #64445, #57161, #17195, #71276, #2225, #15414, #30375, #64894, #16744, #57619, #10372, #9047, #85361, #29479, #16303, #49899 ),
 .UNSPECIFIED., .F., .F.,
 ( 4, 2, 2, 2, 2, 2, 2, 2, 4 ),
 ( 0.4999879786943189908, 0.5624894813575290753, 0.6249909840207392708, 0.6874924866839493554, 0.7499939893471594399, 0.8124954920103696354, 0.8749969946735797199, 0.9374984973367899155, 1.000000000000000000 ),
 .UNSPECIFIED. ) ;
#85094=FACE_OUTER_BOUND ( 'NONE', #51893, .T. ) ;
#85095=FACE_OUTER_BOUND ( 'NONE', #25515, .T. ) ;
#85098=LINE ( 'NONE', #30113, #88010 ) ;
#85101=CARTESIAN_POINT ( 'NONE',  ( 48.79742451362098166, -36.32844715994040996, -5.074374724088000832 ) ) ;
#85104=CARTESIAN_POINT ( 'NONE',  ( 111.4338919110110311, -46.24429912893436523, 27.91848241876792969 ) ) ;
#85105=CARTESIAN_POINT ( 'NONE',  ( 117.4263761885577537, -30.97555849962366281, 175.2299109901969700 ) ) ;
#85106=CARTESIAN_POINT ( 'NONE',  ( 105.3167593786310903, -26.43023667424511913, 11.20991099019697046 ) ) ;
#85108=DIRECTION ( 'NONE',  ( 0.000000000000000000, 0.000000000000000000, 1.000000000000000000 ) ) ;
#85109=CARTESIAN_POINT ( 'NONE',  ( 80.06648329127399677, -33.97944715994105991, 8.225625275910942946 ) ) ;
#85110=CARTESIAN_POINT ( 'NONE',  ( 115.7830851429092291, -41.80234991274182477, 139.4064549843119778 ) ) ;
#85111=AXIS2_PLACEMENT_3D ( 'NONE', #16426, #23698, #23265 ) ;
#85113=AXIS2_PLACEMENT_3D ( 'NONE', #23375, #16984, #38748 ) ;
#85114=CONICAL_SURFACE ( 'NONE', #25557, 1.625000000000001332, 1.029744258676650093 ) ;
#85115=VERTEX_POINT ( 'NONE', #25148 ) ;
#85116=DIRECTION ( 'NONE',  ( 4.299999999999999979E-14, -1.000000000000000000, 4.400000000000000367E-29 ) ) ;
#85117=ORIENTED_EDGE ( 'NONE', *, *, #37878, .T. ) ;
#85118=CARTESIAN_POINT ( 'NONE',  ( 111.6283393632454022, -28.07768985461837730, 55.68991099019593349 ) ) ;
#85121=EDGE_LOOP ( 'NONE', ( #8320, #51487, #85035, #73229 ) ) ;
#85122=CARTESIAN_POINT ( 'NONE',  ( 108.3329992365411556, -46.73491031212436297, 48.67725624094877901 ) ) ;
#85123=CARTESIAN_POINT ( 'NONE',  ( 101.3611157396114635, -46.16939438856402944, 198.1318157521009482 ) ) ;
#85125=CARTESIAN_POINT ( 'NONE',  ( 97.81169536214920868, -40.51742132101362870, 146.6356105553879274 ) ) ;
#85127=DIRECTION ( 'NONE',  ( -1.000000000000000000, 9.376883653928684652E-16, 1.500301384628589584E-15 ) ) ;
#85128=CARTESIAN_POINT ( 'NONE',  ( 25.56670390244797275, -58.35344715994099829, 290.4678068554150627 ) ) ;
#85130=CARTESIAN_POINT ( 'NONE',  ( 110.8541803763881859, -45.98435675075571538, 97.88560012996084936 ) ) ;
#85132=CARTESIAN_POINT ( 'NONE',  ( 97.31342953368660176, -35.99458159538090030, 146.2670538473399517 ) ) ;
#85133=ORIENTED_EDGE ( 'NONE', *, *, #59489, .F. ) ;
#85134=ORIENTED_EDGE ( 'NONE', *, *, #77237, .T. ) ;
#85135=CARTESIAN_POINT ( 'NONE',  ( 114.7653520042265143, -30.23343873216411026, 70.81586902018300123 ) ) ;
#85136=CLOSED_SHELL ( 'NONE', ( #79140, #5602, #25170, #5085 ) ) ;
#85137=DIRECTION ( 'NONE',  ( -1.000000000000000078E-15, 1.000000000000000000, 0.000000000000000000 ) ) ;
#85138=CARTESIAN_POINT ( 'NONE',  ( 115.4995704134666141, -41.68388727776409297, 234.4041967044819899 ) ) ;
#85140=LINE ( 'NONE', #50583, #82684 ) ;
#85145=CARTESIAN_POINT ( 'NONE',  ( 114.2249171546291677, -45.12625265263336871, 153.1508633711489722 ) ) ;
#85146=EDGE_LOOP ( 'NONE', ( #75546, #75025, #32042, #62327 ) ) ;
#85150=CARTESIAN_POINT ( 'NONE',  ( 100.9537233733097992, -28.70776136095884468, 130.5940555066760567 ) ) ;
#85151=CARTESIAN_POINT ( 'NONE',  ( 97.83872692038849550, -40.58291890258023926, 102.6412641178015548 ) ) ;
#85152=CARTESIAN_POINT ( 'NONE',  ( 109.5637425988213636, -28.92903792723274847, 232.6480903695909603 ) ) ;
#85154=CARTESIAN_POINT ( 'NONE',  ( 97.81413906161476746, -40.51632882248723888, 267.6361360915977343 ) ) ;
#85156=CARTESIAN_POINT ( 'NONE',  ( 117.6792309033718027, -39.81954026856703877, 138.5889586092439743 ) ) ;
#85159=ORIENTED_EDGE ( 'NONE', *, *, #14533, .F. ) ;
#85160=VERTEX_POINT ( 'NONE', #66478 ) ;
#85161=CARTESIAN_POINT ( 'NONE',  ( 107.0667039024468039, -54.72944715994092491, 196.8538068554169911 ) ) ;
#85162=VERTEX_POINT ( 'NONE', #19242 ) ;
#85166=CARTESIAN_POINT ( 'NONE',  ( 100.2991084500796575, -40.90897653417852098, 9.586185607686982024 ) ) ;
#85168=ORIENTED_EDGE ( 'NONE', *, *, #66949, .F. ) ;
#85169=AXIS2_PLACEMENT_3D ( 'NONE', #87431, #73794, #38370 ) ;
#85170=CIRCLE ( 'NONE', #45946, 2.029999999999997140 ) ;
#85171=CARTESIAN_POINT ( 'NONE',  ( 111.8278880821266767, -43.86989008726008166, 9.635625275910941312 ) ) ;
#85174=VERTEX_POINT ( 'NONE', #46017 ) ;
#85175=VECTOR ( 'NONE', #10116, 1000.000000000000000 ) ;
#85176=AXIS2_PLACEMENT_3D ( 'NONE', #70960, #8732, #49127 ) ;
#85178=CARTESIAN_POINT ( 'NONE',  ( 112.0330966381960991, -45.41505981916921542, 112.9898362350633221 ) ) ;
#85181=ORIENTED_EDGE ( 'NONE', *, *, #73320, .F. ) ;
#85182=CARTESIAN_POINT ( 'NONE',  ( 109.7027494226597071, -44.85393009491053817, 12.24956268521998304 ) ) ;
#85184=CARTESIAN_POINT ( 'NONE',  ( 99.08440026364779385, -45.52245356036965518, 156.9899109901969609 ) ) ;
#85185=CARTESIAN_POINT ( 'NONE',  ( 98.00553567079148820, -41.84099229931894115, 136.7356252759109623 ) ) ;
#85187=CARTESIAN_POINT ( 'NONE',  ( 101.4046705256369734, -45.52519664383009257, 218.1213395616249784 ) ) ;
#85188=CARTESIAN_POINT ( 'NONE',  ( 51.06648329127400388, 25.62155284005901379, 327.8006252759110453 ) ) ;
#85193=EDGE_LOOP ( 'NONE', ( #32921, #33253, #59030, #57202 ) ) ;
#85194=EDGE_CURVE ( 'NONE', #21457, #14514, #52809, .T. ) ;
#85195=EDGE_LOOP ( 'NONE', ( #75478, #31339, #27076, #77044 ) ) ;
#85196=VECTOR ( 'NONE', #53799, 1000.000000000000000 ) ;
#85198=EDGE_CURVE ( 'NONE', #63781, #81490, #11984, .T. ) ;
#85199=VECTOR ( 'NONE', #39637, 1000.000000000000000 ) ;
#85200=CARTESIAN_POINT ( 'NONE',  ( 102.2167607299587928, -46.00774749580600798, 212.1927681330539599 ) ) ;
#85202=CARTESIAN_POINT ( 'NONE',  ( 96.61862839515298162, -36.21153332102672806, 171.2870538473399620 ) ) ;
#85203=CARTESIAN_POINT ( 'NONE',  ( 164.7812970173289955, -35.65087443492610930, -5.074374724088000832 ) ) ;
#85205=DIRECTION ( 'NONE',  ( -0.7071067811865475727, 0.7071067811865475727, 0.000000000000000000 ) ) ;
#85206=DIRECTION ( 'NONE',  ( 0.000000000000000000, -1.000000000000000000, 0.000000000000000000 ) ) ;
#85207=LINE ( 'NONE', #21170, #4152 ) ;
#85208=CARTESIAN_POINT ( 'NONE',  ( 34.27258461953899626, -35.55794170701810941, 342.9256252759119548 ) ) ;
#85209=CARTESIAN_POINT ( 'NONE',  ( 115.2346088729119629, -30.22974330756305505, 240.3613395616249875 ) ) ;
#85212=LINE ( 'NONE', #10221, #35320 ) ;
#85214=CARTESIAN_POINT ( 'NONE',  ( 116.8171228659443557, -34.15291831921626198, 260.0314586093679168 ) ) ;
#85215=EDGE_CURVE ( 'NONE', #69535, #14111, #67369, .T. ) ;
#85217=CARTESIAN_POINT ( 'NONE',  ( 99.18160966223959463, -39.27556854586995883, 195.5838068554172651 ) ) ;
#85218=VERTEX_POINT ( 'NONE', #53724 ) ;
#85220=CARTESIAN_POINT ( 'NONE',  ( 109.6112504147204163, -26.56025234872169349, 199.8813395616249977 ) ) ;
#85221=CARTESIAN_POINT ( 'NONE',  ( 96.07767081433036083, -37.92107664550148627, 77.40038718067299328 ) ) ;
#85222=CARTESIAN_POINT ( 'NONE',  ( 117.2394727393827765, -34.25896837304814113, 205.0156252759109634 ) ) ;
#85223=DIRECTION ( 'NONE',  ( 1.000000000000000000, 0.000000000000000000, 0.000000000000000000 ) ) ;
#85225=DIRECTION ( 'NONE',  ( 0.000000000000000000, 0.000000000000000000, 1.000000000000000000 ) ) ;
#85230=CIRCLE ( 'NONE', #51834, 3.250000000000002665 ) ;
#85231=CARTESIAN_POINT ( 'NONE',  ( 109.7274023519750159, -27.00147441307279550, 64.86589663587605514 ) ) ;
#85235=DIRECTION ( 'NONE',  ( 0.000000000000000000, 0.000000000000000000, -1.000000000000000000 ) ) ;
#85236=ORIENTED_EDGE ( 'NONE', *, *, #52324, .T. ) ;
#85237=CARTESIAN_POINT ( 'NONE',  ( 111.0741232671659020, -25.60348521778456288, 95.80133956162495679 ) ) ;
#85239=EDGE_CURVE ( 'NONE', #75364, #47935, #32856, .T. ) ;
#85240=ADVANCED_FACE ( 'NONE', ( #14217 ), #21028, .T. ) ;
#85241=CARTESIAN_POINT ( 'NONE',  ( 21.03715912545829170, -47.82818131006186491, 249.9678068554150059 ) ) ;
#85242=CARTESIAN_POINT ( 'NONE',  ( 172.5664832912740110, 0.2215528400590013880, 21.04262527591200183 ) ) ;
#85243=ADVANCED_FACE ( 'NONE', ( #89181, #13763 ), #69178, .F. ) ;
#85244=CIRCLE ( 'NONE', #82370, 5.499999999999999112 ) ;
#85245=CARTESIAN_POINT ( 'NONE',  ( 115.0831197249980420, -29.02584261466826021, 39.43562527591099354 ) ) ;
#85247=ORIENTED_EDGE ( 'NONE', *, *, #69379, .T. ) ;
#85249=AXIS2_PLACEMENT_3D ( 'NONE', #51324, #51769, #72696 ) ;
#85252=CARTESIAN_POINT ( 'NONE',  ( 134.0664832912739826, -9.029447159941003775, 8.225625275910998013 ) ) ;
#85253=DIRECTION ( 'NONE',  ( 0.000000000000000000, 0.000000000000000000, 1.000000000000000000 ) ) ;
#85255=DIRECTION ( 'NONE',  ( -4.299999999999999979E-14, 1.000000000000000000, -4.400000000000000367E-29 ) ) ;
#85256=DIRECTION ( 'NONE',  ( 0.000000000000000000, 0.000000000000000000, 1.000000000000000000 ) ) ;
#85257=CARTESIAN_POINT ( 'NONE',  ( 181.9790560690580037, -31.62489322948711035, -5.074374724088000832 ) ) ;
#85258=DIRECTION ( 'NONE',  ( -1.000000000000000000, 0.000000000000000000, 0.000000000000000000 ) ) ;
#85259=DIRECTION ( 'NONE',  ( -0.7071067811865171526, -0.7071067811865779928, -7.071067811865164719E-16 ) ) ;
#85261=CARTESIAN_POINT ( 'NONE',  ( 116.8729656461675148, -36.55725972750698105, 288.8413395616257731 ) ) ;
#85262=VERTEX_POINT ( 'NONE', #20589 ) ;
#85267=CARTESIAN_POINT ( 'NONE',  ( 115.3203086601475320, -34.12650808536288594, 126.8757094172099613 ) ) ;
#85270=DIRECTION ( 'NONE',  ( 1.000000000000000078E-15, 1.000000000000000083E-30, -1.000000000000000000 ) ) ;
#85271=EDGE_LOOP ( 'NONE', ( #84170, #20037, #56629, #31322 ) ) ;
#85272=ORIENTED_EDGE ( 'NONE', *, *, #79879, .F. ) ;
#85274=ORIENTED_EDGE ( 'NONE', *, *, #78837, .F. ) ;
#85275=ORIENTED_EDGE ( 'NONE', *, *, #50702, .F. ) ;
#85276=CARTESIAN_POINT ( 'NONE',  ( 99.58187507909633496, -41.47380365182278439, 183.2072975916109385 ) ) ;
#85278=CARTESIAN_POINT ( 'NONE',  ( 109.2595486427728559, -46.97979643076451595, 103.7441967044829880 ) ) ;
#85280=CARTESIAN_POINT ( 'NONE',  ( 98.04153897299465825, -41.04189894509466541, 16.68120577741022004 ) ) ;
#85282=EDGE_LOOP ( 'NONE', ( #63721, #25718, #43391, #71561 ) ) ;
#85283=EDGE_LOOP ( 'NONE', ( #55787, #51502, #38759, #7120 ) ) ;
#85285=CARTESIAN_POINT ( 'NONE',  ( 108.0149359080884324, -45.33189881898218232, 155.4699951314959776 ) ) ;
#85287=CARTESIAN_POINT ( 'NONE',  ( 97.60225484043094468, -32.22203741027808377, 75.97276813305397525 ) ) ;
#85288=ORIENTED_EDGE ( 'NONE', *, *, #17352, .F. ) ;
#85289=CARTESIAN_POINT ( 'NONE',  ( 111.1204619107249982, -46.98756979655009047, 22.88800622829195675 ) ) ;
#85290=CARTESIAN_POINT ( 'NONE',  ( 104.5573670441197720, -48.33662538491821437, 178.4070538473399665 ) ) ;
#85293=CARTESIAN_POINT ( 'NONE',  ( 114.7260775003150712, -43.80144150384058577, 119.2327681330539804 ) ) ;
#85294=CARTESIAN_POINT ( 'NONE',  ( 100.8874679133985381, -44.70022139721319832, 262.0522919454450630 ) ) ;
#85295=ORIENTED_EDGE ( 'NONE', *, *, #87467, .T. ) ;
#85296=PLANE ( 'NONE',  #84454 ) ;
#85297=EDGE_CURVE ( 'NONE', #34907, #52360, #19684, .T. ) ;
#85299=CIRCLE ( 'NONE', #83870, 10.00000000000002487 ) ;
#85301=CARTESIAN_POINT ( 'NONE',  ( 50.97905606905900555, -31.62489322948711035, -5.074374724088000832 ) ) ;
#85304=ADVANCED_FACE ( 'NONE', ( #89633 ), #76433, .T. ) ;
#85306=AXIS2_PLACEMENT_3D ( 'NONE', #52318, #58278, #36512 ) ;
#85307=DIRECTION ( 'NONE',  ( 0.000000000000000000, 1.000000000000000000, 0.000000000000000000 ) ) ;
#85308=CARTESIAN_POINT ( 'NONE',  ( 101.0660769631361688, -27.44644056990073366, 70.54514908543497143 ) ) ;
#85309=CARTESIAN_POINT ( 'NONE',  ( 107.0664832912739399, -36.72944715994096754, 298.1356252759109680 ) ) ;
#85310=EDGE_CURVE ( 'NONE', #51322, #9402, #7397, .T. ) ;
#85311=FACE_BOUND ( 'NONE', #63128, .T. ) ;
#85313=CARTESIAN_POINT ( 'NONE',  ( 117.2535196871930481, -41.18324016912744412, 58.49848241876892985 ) ) ;
#85314=CARTESIAN_POINT ( 'NONE',  ( 113.2454051795150463, -28.75859548762567641, 109.5523015492156986 ) ) ;
#85315=CARTESIAN_POINT ( 'NONE',  ( 98.10941331148548272, -42.08998169807667722, 157.7556252759109725 ) ) ;
#85317=CYLINDRICAL_SURFACE ( 'NONE', #45240, 27.99999999999999645 ) ;
#85319=DIRECTION ( 'NONE',  ( -4.237773401492740281E-14, 1.000000000000000000, 0.000000000000000000 ) ) ;
#85322=EDGE_CURVE ( 'NONE', #89449, #65816, #27386, .T. ) ;
#85323=VECTOR ( 'NONE', #4058, 1000.000000000000000 ) ;
#85324=CARTESIAN_POINT ( 'NONE',  ( 59.67078992371374113, -0.9290567490904538817, 542.9756252759101471 ) ) ;
#85325=CARTESIAN_POINT ( 'NONE',  ( 102.2167607299587928, -46.00774749580600798, 212.1927681330539599 ) ) ;
#85327=CARTESIAN_POINT ( 'NONE',  ( 80.06648329127402519, -36.72944715994107412, -5.074374724089057764 ) ) ;
#85328=CARTESIAN_POINT ( 'NONE',  ( 115.3407290770031324, -45.24761053976980918, 264.1899109901965517 ) ) ;
#85329=CARTESIAN_POINT ( 'NONE',  ( 117.9205228141932054, -39.05050820906062370, 104.6708633711489824 ) ) ;
#85330=AXIS2_PLACEMENT_3D ( 'NONE', #50820, #30383, #9488 ) ;
#85331=DIRECTION ( 'NONE',  ( 0.000000000000000000, 0.000000000000000000, 1.000000000000000000 ) ) ;
#85335=CARTESIAN_POINT ( 'NONE',  ( 34.96670390244661775, -28.27351298637442056, 117.4678068554150485 ) ) ;
#85337=CIRCLE ( 'NONE', #34520, 1.000000000000000888 ) ;
#85340=AXIS2_PLACEMENT_3D ( 'NONE', #34081, #61785, #27280 ) ;
#85341=ORIENTED_EDGE ( 'NONE', *, *, #50817, .T. ) ;
#85343=CARTESIAN_POINT ( 'NONE',  ( 118.5467753794658705, -33.90456151647279626, 10.01848241876795953 ) ) ;
#85344=DIRECTION ( 'NONE',  ( 0.000000000000000000, 0.000000000000000000, -1.000000000000000000 ) ) ;
#85347=CARTESIAN_POINT ( 'NONE',  ( 194.5664832912739826, 0.2215528400590013880, -5.074374724088000832 ) ) ;
#85349=ADVANCED_FACE ( 'NONE', ( #78705, #15571, #8758, #23297, #9635, #79142, #30530, #57779 ), #78257, .T. ) ;
#85351=VECTOR ( 'NONE', #88717, 999.9999999999998863 ) ;
#85352=CARTESIAN_POINT ( 'NONE',  ( 116.6718245901296171, -38.14650263757180682, 223.1324198280769622 ) ) ;
#85353=ORIENTED_EDGE ( 'NONE', *, *, #66546, .T. ) ;
#85354=ORIENTED_EDGE ( 'NONE', *, *, #7427, .T. ) ;
#85355=ORIENTED_EDGE ( 'NONE', *, *, #17880, .F. ) ;
#85357=CYLINDRICAL_SURFACE ( 'NONE', #41942, 0.5000000000000031086 ) ;
#85358=CARTESIAN_POINT ( 'NONE',  ( 105.9660761217308931, -46.48152529548401901, 278.4870538473389843 ) ) ;
#85359=DIRECTION ( 'NONE',  ( -0.9068632946707807507, 0.4214249218767881500, -9.028300618466658994E-16 ) ) ;
#85360=CARTESIAN_POINT ( 'NONE',  ( 108.2420053567034017, -46.43931755893575541, 113.6727681330529691 ) ) ;
#85361=CARTESIAN_POINT ( 'NONE',  ( 117.0606848385255319, -38.08193180985016113, 28.71884086846101525 ) ) ;
#85362=EDGE_LOOP ( 'NONE', ( #61955, #71304 ) ) ;
#85367=CARTESIAN_POINT ( 'NONE',  ( 114.1852310984691883, -41.65497984893937655, 11.17475703625792072 ) ) ;
#85368=ADVANCED_FACE ( 'NONE', ( #70529 ), #36457, .F. ) ;
#85369=CIRCLE ( 'NONE', #83879, 3.000000000000002665 ) ;
#85370=AXIS2_PLACEMENT_3D ( 'NONE', #50777, #63972, #65735 ) ;
#85371=LINE ( 'NONE', #3559, #26133 ) ;
#85372=LINE ( 'NONE', #58515, #46103 ) ;
#85373=CARTESIAN_POINT ( 'NONE',  ( 117.0719183210286900, -35.46267133667483762, 194.9273074894743729 ) ) ;
#85374=ORIENTED_EDGE ( 'NONE', *, *, #48325, .F. ) ;
#85376=AXIS2_PLACEMENT_3D ( 'NONE', #54702, #6586, #5246 ) ;
#85377=DIRECTION ( 'NONE',  ( -0.9068632946707805287, 0.4214249218767882610, -9.061988307341536250E-16 ) ) ;
#85378=ORIENTED_EDGE ( 'NONE', *, *, #15953, .F. ) ;
#85379=CARTESIAN_POINT ( 'NONE',  ( 116.2317802277880787, -31.76111116818806224, 69.22133956162495849 ) ) ;
#85380=ORIENTED_EDGE ( 'NONE', *, *, #19511, .T. ) ;
#85381=CARTESIAN_POINT ( 'NONE',  ( 109.1520131464112069, -27.24676858702523674, 29.32670554236194249 ) ) ;
#85382=AXIS2_PLACEMENT_3D ( 'NONE', #72922, #30703, #65227 ) ;
#85384=CARTESIAN_POINT ( 'NONE',  ( 116.7742277529940225, -35.53649587948895316, 193.9241967044829664 ) ) ;
#85385=CARTESIAN_POINT ( 'NONE',  ( 128.0667039024480118, -50.82844715994100682, 198.9178068554149945 ) ) ;
#85386=CARTESIAN_POINT ( 'NONE',  ( 180.2121375201600131, -29.73316016639650172, 193.9678068554150059 ) ) ;
#85387=AXIS2_PLACEMENT_3D ( 'NONE', #54422, #26303, #75355 ) ;
#85389=ADVANCED_FACE ( 'NONE', ( #64164 ), #77791, .F. ) ;
#85390=CARTESIAN_POINT ( 'NONE',  ( 105.0131270392176646, -25.82159629633810738, 276.2365776568634033 ) ) ;
#85391=DIRECTION ( 'NONE',  ( 0.000000000000000000, 0.000000000000000000, 1.000000000000000000 ) ) ;
#85392=EDGE_LOOP ( 'NONE', ( #50042, #48066, #87975, #1694, #64962 ) ) ;
#85393=CYLINDRICAL_SURFACE ( 'NONE', #56005, 2.030000000002079918 ) ;
#85395=CARTESIAN_POINT ( 'NONE',  ( 102.2928874563330055, -26.70895414482565045, 136.4422919425779526 ) ) ;
#85396=DIRECTION ( 'NONE',  ( 0.000000000000000000, 0.000000000000000000, 1.000000000000000000 ) ) ;
#85397=EDGE_LOOP ( 'NONE', ( #84956, #55803, #50672, #62202 ) ) ;
#85398=VERTEX_POINT ( 'NONE', #43243 ) ;
#85399=EDGE_CURVE ( 'NONE', #41571, #82149, #38664, .T. ) ;
#85401=VERTEX_POINT ( 'NONE', #16454 ) ;
#85403=CARTESIAN_POINT ( 'NONE',  ( 112.0659115482700088, -45.48839630408555479, 122.9897919358033249 ) ) ;
#85404=ADVANCED_FACE ( 'NONE', ( #29194 ), #23730, .F. ) ;
#85405=CARTESIAN_POINT ( 'NONE',  ( 107.0664832912739968, -36.72944715994100306, 249.5838068554170093 ) ) ;
#85406=CARTESIAN_POINT ( 'NONE',  ( 112.6571330189593141, -45.46348522128867131, 218.0175300378159591 ) ) ;
#85407=LINE ( 'NONE', #2718, #3716 ) ;
#85408=DIRECTION ( 'NONE',  ( 0.000000000000000000, 0.000000000000000000, 1.000000000000000000 ) ) ;
#85409=DIRECTION ( 'NONE',  ( 0.000000000000000000, 1.000000000000000000, 0.000000000000000000 ) ) ;
#85410=CARTESIAN_POINT ( 'NONE',  ( 102.7553090513238487, -25.69095112480093945, 16.37276813305293999 ) ) ;
#85411=DIRECTION ( 'NONE',  ( 1.000000000000000000, -5.337610695313248426E-16, 0.000000000000000000 ) ) ;
#85412=VERTEX_POINT ( 'NONE', #16905 ) ;
#85414=CIRCLE ( 'NONE', #46188, 0.5000000000000004441 ) ;
#85415=DIRECTION ( 'NONE',  ( 0.000000000000000000, 0.000000000000000000, -1.000000000000000000 ) ) ;
#85416=VECTOR ( 'NONE', #25329, 1000.000000000000000 ) ;
#85417=ORIENTED_EDGE ( 'NONE', *, *, #61376, .F. ) ;
#85418=ADVANCED_FACE ( 'NONE', ( #29631 ), #85067, .F. ) ;
#85420=PLANE ( 'NONE',  #15055 ) ;
#85421=CARTESIAN_POINT ( 'NONE',  ( 114.9613132280022683, -29.02649429439048134, 194.4537205140059370 ) ) ;
#85422=LINE ( 'NONE', #16356, #843 ) ;
#85423=DIRECTION ( 'NONE',  ( 0.000000000000000000, 0.000000000000000000, -1.000000000000000000 ) ) ;
#85424=DIRECTION ( 'NONE',  ( 0.000000000000000000, 0.000000000000000000, -1.000000000000000000 ) ) ;
#85425=EDGE_CURVE ( 'NONE', #42008, #68551, #82211, .T. ) ;
#85426=CARTESIAN_POINT ( 'NONE',  ( 106.8904373410712481, -45.78382058659838094, 226.9714674471249509 ) ) ;
#85427=FACE_OUTER_BOUND ( 'NONE', #82369, .T. ) ;
#85428=CARTESIAN_POINT ( 'NONE',  ( 112.8057071037347185, -27.31004523576153886, 45.62895860924398761 ) ) ;
#85430=CARTESIAN_POINT ( 'NONE',  ( 116.6387536407295329, -29.65834838561569242, 109.3327681330539605 ) ) ;
#85431=ORIENTED_EDGE ( 'NONE', *, *, #11010, .F. ) ;
#85432=CARTESIAN_POINT ( 'NONE',  ( 131.5922609085388331, -19.93375462384614494, 7.110117206084406227 ) ) ;
#85434=CARTESIAN_POINT ( 'NONE',  ( 180.2121375201587625, -29.73316016638863957, 117.4678068554150627 ) ) ;
#85435=CARTESIAN_POINT ( 'NONE',  ( 115.1492182743862998, -30.73465633580296341, 275.3339211662992625 ) ) ;
#85436=ORIENTED_EDGE ( 'NONE', *, *, #75931, .F. ) ;
#85438=CARTESIAN_POINT ( 'NONE',  ( 115.0888839854113002, -30.61760552574517646, 49.34396152961115689 ) ) ;
#85439=VERTEX_POINT ( 'NONE', #50514 ) ;
#85442=CIRCLE ( 'NONE', #38966, 0.5000000000000004441 ) ;
#85445=VECTOR ( 'NONE', #46890, 1000.000000000000000 ) ;
#85446=CARTESIAN_POINT ( 'NONE',  ( 113.3280054804099137, -28.32220607287434078, 104.5670538473399347 ) ) ;
#85451=VERTEX_POINT ( 'NONE', #84620 ) ;
#85452=CARTESIAN_POINT ( 'NONE',  ( 25.56670390244797275, -62.87844715994099687, 293.2178068554150627 ) ) ;
#85453=CYLINDRICAL_SURFACE ( 'NONE', #46872, 5.599999999999994316 ) ;
#85454=VECTOR ( 'NONE', #66213, 1000.000000000000000 ) ;
#85456=CARTESIAN_POINT ( 'NONE',  ( 179.4595971212738164, -26.00627455218718254, 237.4678068554150059 ) ) ;
#85458=ADVANCED_FACE ( 'NONE', ( #42786 ), #22377, .T. ) ;
#85461=LINE ( 'NONE', #64104, #50577 ) ;
#85462=CARTESIAN_POINT ( 'NONE',  ( 102.2868918306628387, -45.93239726994502803, 163.1832443235289816 ) ) ;
#85465=ORIENTED_EDGE ( 'NONE', *, *, #57696, .F. ) ;
#85466=CARTESIAN_POINT ( 'NONE',  ( 116.8666056714781973, -37.25052799200011577, 14.78419670448194445 ) ) ;
#85468=LINE ( 'NONE', #86342, #29855 ) ;
#85469=CARTESIAN_POINT ( 'NONE',  ( 115.0352726211783079, -42.91098005955615236, 13.30258960125530798 ) ) ;
#85470=EDGE_CURVE ( 'NONE', #46563, #57647, #83630, .T. ) ;
#85471=CARTESIAN_POINT ( 'NONE',  ( 113.2466805891969415, -28.75957719968114290, 29.55240580932557393 ) ) ;
#85472=CARTESIAN_POINT ( 'NONE',  ( 98.59486473514172644, -43.92970144294059054, 226.8870538473399563 ) ) ;
#85473=ORIENTED_EDGE ( 'NONE', *, *, #70513, .T. ) ;
#85474=ORIENTED_EDGE ( 'NONE', *, *, #54497, .F. ) ;
#85475=CIRCLE ( 'NONE', #81129, 1.000000000000000888 ) ;
#85476=CARTESIAN_POINT ( 'NONE',  ( 99.15781305739687923, -40.79332027783682690, 193.1358690201829518 ) ) ;
#85478=LINE ( 'NONE', #51794, #85049 ) ;
#85479=CARTESIAN_POINT ( 'NONE',  ( 113.6566823882007355, -42.65376606380868196, 34.67586902018199169 ) ) ;
#85481=FACE_OUTER_BOUND ( 'NONE', #15893, .T. ) ;
#85482=LINE ( 'NONE', #78671, #12534 ) ;
#85483=VERTEX_POINT ( 'NONE', #36894 ) ;
#85484=CARTESIAN_POINT ( 'NONE',  ( 165.6738106836199904, -26.00627455219321860, 117.4678068554150485 ) ) ;
#85486=CARTESIAN_POINT ( 'NONE',  ( 96.99990081654250673, -39.35482002063354656, 276.5299109901967540 ) ) ;
#85488=ORIENTED_EDGE ( 'NONE', *, *, #73052, .T. ) ;
#85489=VERTEX_POINT ( 'NONE', #2384 ) ;
#85491=CARTESIAN_POINT ( 'NONE',  ( 41.56670390244783420, -36.32844715994104234, 249.9678068554150343 ) ) ;
#85492=CARTESIAN_POINT ( 'NONE',  ( 49.16670390244701139, -28.27351298637340093, -5.074374724088000832 ) ) ;
#85495=CARTESIAN_POINT ( 'NONE',  ( 104.4155842969358332, -46.14412564300911157, 18.35848241876792031 ) ) ;
#85496=AXIS2_PLACEMENT_3D ( 'NONE', #46751, #54003, #75824 ) ;
#85497=DIRECTION ( 'NONE',  ( 0.1858654558203195195, -0.9825752044157765042, 0.000000000000000000 ) ) ;
#85499=ORIENTED_EDGE ( 'NONE', *, *, #26338, .F. ) ;
#85500=CARTESIAN_POINT ( 'NONE',  ( 109.6537587170975030, -46.87336088289573865, 43.77562527591094721 ) ) ;
#85502=CARTESIAN_POINT ( 'NONE',  ( 96.53679867426635042, -40.09171982297686299, 281.5603871806728762 ) ) ;
#85504=EDGE_LOOP ( 'NONE', ( #63348, #55188, #25241, #43009 ) ) ;
#85505=B_SPLINE_CURVE_WITH_KNOTS ( 'NONE', 3,
 ( #85125, #52321, #30138, #51449, #16074, #16512, #79200, #71925, #9690, #43753, #16957, #65101, #22892, #72809, #72371, #9252, #10139, #80086, #3328, #79641, #64219, #45082, #31022, #29688, #38281, #36515, #65977, #1989, #50568, #64653, #45965, #40516, #52762, #11926, #26888, #39175, #68237, #32803, #54119, #54561, #67319, #5567, #87337, #88245, #12832, #40060, #66425, #19626, #53217, #6020, #73238 ),
 .UNSPECIFIED., .F., .F.,
 ( 4, 2, 1, 1, 1, 1, 1, 1, 2, 2, 2, 2, 2, 2, 2, 1, 1, 1, 1, 1, 1, 1, 2, 2, 2, 2, 2, 2, 2, 2, 2, 4 ),
 ( 0.5000151712595112263, 0.5001372378680968289, 0.5002593044766825425, 0.5005034376938537477, 0.5009917041281959360, 0.5019682369968807567, 0.5039213027342506201, 0.5078274342089901250, 0.5156396971584693567, 0.5312642230574272650, 0.5625132748553431927, 0.6250113784511752701, 0.6875094820470073476, 0.7500075856428394250, 0.7500686189471321708, 0.7501296522514248055, 0.7502517188599931997, 0.7504958520771425334, 0.7509841185114412010, 0.7519606513800297654, 0.7539137171171848006, 0.7578198485915111915, 0.7656321115401695243, 0.7812566374374917411, 0.8125056892321357305, 0.8437547410267797199, 0.8750037928214238203, 0.9062528446160678097, 0.9375018964107117991, 0.9687509482053557885, 0.9843754741026778943, 1.000000000000000000 ),
 .UNSPECIFIED. ) ;
#85507=EDGE_CURVE ( 'NONE', #7119, #60401, #37264, .T. ) ;
#85508=CARTESIAN_POINT ( 'NONE',  ( 79.68962695805252849, -39.47945062089030444, 8.225625248534937484 ) ) ;
#85509=DIRECTION ( 'NONE',  ( 1.000000000000000078E-15, -1.000000000000000083E-30, -1.000000000000000000 ) ) ;
#85510=DIRECTION ( 'NONE',  ( 0.000000000000000000, 1.000000000000000000, 0.000000000000000000 ) ) ;
#85511=CARTESIAN_POINT ( 'NONE',  ( 102.8475555715194361, -29.17288882023929730, 103.3118998934009767 ) ) ;
#85512=CARTESIAN_POINT ( 'NONE',  ( 103.8129894719335624, -48.15035030529833904, 213.3556252759109668 ) ) ;
#85514=VERTEX_POINT ( 'NONE', #65924 ) ;
#85515=EDGE_CURVE ( 'NONE', #231, #87802, #66369, .T. ) ;
#85516=AXIS2_PLACEMENT_3D ( 'NONE', #23433, #37487, #24743 ) ;
#85518=ORIENTED_EDGE ( 'NONE', *, *, #20034, .T. ) ;
#85519=ORIENTED_EDGE ( 'NONE', *, *, #55926, .T. ) ;
#85520=ADVANCED_FACE ( 'NONE', ( #52269 ), #10964, .F. ) ;
#85521=DIRECTION ( 'NONE',  ( 0.000000000000000000, 1.000000000000000000, 0.000000000000000000 ) ) ;
#85524=CYLINDRICAL_SURFACE ( 'NONE', #83151, 2.117000000000007987 ) ;
#85525=CARTESIAN_POINT ( 'NONE',  ( 103.6639831185296288, -27.32465593432968021, 41.35270917185196993 ) ) ;
#85526=EDGE_CURVE ( 'NONE', #11027, #58704, #3866, .T. ) ;
#85527=VECTOR ( 'NONE', #3500, 1000.000000000000000 ) ;
#85528=CARTESIAN_POINT ( 'NONE',  ( 108.0580239150950774, -28.21657753114420331, 129.4067055423629711 ) ) ;
#85529=CARTESIAN_POINT ( 'NONE',  ( 106.2251211966456879, -47.77424462129209815, 267.5280062282920994 ) ) ;
#85531=EDGE_LOOP ( 'NONE', ( #43164, #65149, #39652, #21596 ) ) ;
#85532=EDGE_LOOP ( 'NONE', ( #73455, #84603 ) ) ;
#85534=CARTESIAN_POINT ( 'NONE',  ( 90.44969454456408187, -56.64645651782490177, 239.5838068554174356 ) ) ;
#85536=CARTESIAN_POINT ( 'NONE',  ( 111.7936012040045597, -46.77578388097458628, 287.9146728949587555 ) ) ;
#85538=CARTESIAN_POINT ( 'NONE',  ( 110.8926993666852496, -26.99363814275770679, 269.7784824187681920 ) ) ;
#85539=CARTESIAN_POINT ( 'NONE',  ( 112.1383799374394670, -26.85658479980368440, 15.71086337114896381 ) ) ;
#85540=DIRECTION ( 'NONE',  ( 1.000000000000000078E-15, 0.000000000000000000, -1.000000000000000000 ) ) ;
#85541=DIRECTION ( 'NONE',  ( 0.000000000000000000, 0.000000000000000000, -1.000000000000000000 ) ) ;
#85542=PLANE ( 'NONE',  #84865 ) ;
#85543=CARTESIAN_POINT ( 'NONE',  ( 83.06670390244796920, -64.87844715994098976, 207.5838068554149913 ) ) ;
#85544=CARTESIAN_POINT ( 'NONE',  ( 73.06670390244801183, -58.35344715994099829, 10.91780685541479734 ) ) ;
#85545=CARTESIAN_POINT ( 'NONE',  ( 188.5667039024479834, -58.35344715994099829, 173.2178068554149775 ) ) ;
#85547=CARTESIAN_POINT ( 'NONE',  ( 100.9546727792195639, -28.70702575126005485, 11.59395861232007263 ) ) ;
#85549=CARTESIAN_POINT ( 'NONE',  ( 188.5667039024479834, -58.35344715994099829, 257.2178068554150059 ) ) ;
#85550=VECTOR ( 'NONE', #62058, 1000.000000000000000 ) ;
#85552=CARTESIAN_POINT ( 'NONE',  ( 117.5565198162756104, -37.28721152219886648, 18.78419670448294809 ) ) ;
#85553=CARTESIAN_POINT ( 'NONE',  ( 107.5657681238088941, -47.77139876010166830, 188.6003871806729535 ) ) ;
#85554=CARTESIAN_POINT ( 'NONE',  ( 116.7472758669860013, -31.34730438484761805, 25.24229194257798881 ) ) ;
#85555=DIRECTION ( 'NONE',  ( 0.9068632946707807507, -0.4214249218767880945, 9.080193194566099635E-16 ) ) ;
#85556=CARTESIAN_POINT ( 'NONE',  ( 71.25416588882602298, -72.55705569728901594, 542.9756252759101471 ) ) ;
#85558=CARTESIAN_POINT ( 'NONE',  ( 81.91153210827047815, -34.68812259376856133, 2.188418746634181122 ) ) ;
#85559=AXIS2_PLACEMENT_3D ( 'NONE', #73284, #52364, #2924 ) ;
#85562=CARTESIAN_POINT ( 'NONE',  ( 107.0664832912739968, -18.82844715994099971, 168.9256252759119832 ) ) ;
#85563=ORIENTED_EDGE ( 'NONE', *, *, #73947, .T. ) ;
#85564=CARTESIAN_POINT ( 'NONE',  ( 97.89279369561094768, -33.33727167892453735, 62.04419670448196911 ) ) ;
#85568=CARTESIAN_POINT ( 'NONE',  ( 115.0368097993288785, -42.90903055077831141, 49.30223481898713089 ) ) ;
#85569=CARTESIAN_POINT ( 'NONE',  ( 114.1099639442525699, -29.07320488188167218, 195.4841967044819739 ) ) ;
#85570=DIRECTION ( 'NONE',  ( 1.000000000000000000, 4.163336342344333240E-14, 0.000000000000000000 ) ) ;
#85571=DIRECTION ( 'NONE',  ( 0.000000000000000000, 0.000000000000000000, 1.000000000000000000 ) ) ;
#85573=CARTESIAN_POINT ( 'NONE',  ( 98.35000460789950694, -31.65632374290893480, 150.9069170840674872 ) ) ;
#85576=CARTESIAN_POINT ( 'NONE',  ( 110.8610854611956995, -45.98152856190351656, 97.88619379672280729 ) ) ;
#85577=CIRCLE ( 'NONE', #86990, 0.1499999999999965528 ) ;
#85578=CARTESIAN_POINT ( 'NONE',  ( 102.6065612795739952, -27.36740250608067626, 140.4422919425779526 ) ) ;
#85580=EDGE_LOOP ( 'NONE', ( #78858, #33525, #14334, #76488 ) ) ;
#85581=CARTESIAN_POINT ( 'NONE',  ( 108.6974651445452764, -45.43968118700122005, 79.15586902018296200 ) ) ;
#85584=CARTESIAN_POINT ( 'NONE',  ( 116.8310051202517457, -36.16593252570071115, 224.8727681330539667 ) ) ;
#85587=CARTESIAN_POINT ( 'NONE',  ( 131.0667039024480118, -61.87844715994100397, 207.5838068554149913 ) ) ;
#85588=VECTOR ( 'NONE', #32092, 1000.000000000000000 ) ;
#85589=CARTESIAN_POINT ( 'NONE',  ( 182.2300522401149863, -33.89581943344511217, -5.074374724088000832 ) ) ;
#85592=CARTESIAN_POINT ( 'NONE',  ( 117.7782040715257921, -34.09831434418944696, 164.0061014663869798 ) ) ;
#85594=VERTEX_POINT ( 'NONE', #31855 ) ;
#85595=ORIENTED_EDGE ( 'NONE', *, *, #47527, .F. ) ;
#85597=CARTESIAN_POINT ( 'NONE',  ( 77.33253968407630907, -18.38436945696972202, 3.076560175368437733 ) ) ;
#85599=CARTESIAN_POINT ( 'NONE',  ( 59.67079009362632291, -0.9310397146383332379, 396.9756252759102040 ) ) ;
#85600=CARTESIAN_POINT ( 'NONE',  ( 111.8846140958497273, -43.31847907419767552, 225.8966617981629668 ) ) ;
#85601=CARTESIAN_POINT ( 'NONE',  ( 109.6429999896449914, -46.48009007242004031, 268.7814576145019601 ) ) ;
#85602=CARTESIAN_POINT ( 'NONE',  ( 97.42502596350711030, -42.13512825026991493, 181.7451490854349743 ) ) ;
#85603=DIRECTION ( 'NONE',  ( 0.000000000000000000, 0.000000000000000000, -1.000000000000000000 ) ) ;
#85604=ORIENTED_EDGE ( 'NONE', *, *, #44785, .F. ) ;
#85608=AXIS2_PLACEMENT_3D ( 'NONE', #69481, #62657, #433 ) ;
#85610=ORIENTED_EDGE ( 'NONE', *, *, #57492, .T. ) ;
#85612=CARTESIAN_POINT ( 'NONE',  ( 194.0371591254585439, -46.82818131005407736, 116.4678068554150201 ) ) ;
#85613=EDGE_CURVE ( 'NONE', #53629, #87604, #32752, .T. ) ;
#85614=CARTESIAN_POINT ( 'NONE',  ( 132.8008218761653723, -34.28157759251718772, 7.978179524060857730 ) ) ;
#85615=CARTESIAN_POINT ( 'NONE',  ( 110.8184301750971485, -28.11564833443670608, 281.1692023535160843 ) ) ;
#85618=ADVANCED_FACE ( 'NONE', ( #38668 ), #60386, .F. ) ;
#85619=CARTESIAN_POINT ( 'NONE',  ( 114.1502950862027603, -42.12385254268857437, 9.635625275910941312 ) ) ;
#85622=CIRCLE ( 'NONE', #53659, 13.49999999999999822 ) ;
#85624=DIRECTION ( 'NONE',  ( 0.000000000000000000, 0.000000000000000000, -1.000000000000000000 ) ) ;
#85625=VERTEX_POINT ( 'NONE', #65493 ) ;
#85628=CARTESIAN_POINT ( 'NONE',  ( 99.46800687602927837, -39.83949638310546248, 11.05813411379097388 ) ) ;
#85629=VECTOR ( 'NONE', #54161, 1000.000000000000000 ) ;
#85630=CARTESIAN_POINT ( 'NONE',  ( 117.3133064751534249, -34.51789172102134984, 183.9956252759109532 ) ) ;
#85631=CARTESIAN_POINT ( 'NONE',  ( 98.29923130492881000, -31.06375673945261440, 145.8699109901969848 ) ) ;
#85633=CARTESIAN_POINT ( 'NONE',  ( 57.56670390244808289, -42.82844715994040286, 257.2178068554150627 ) ) ;
#85634=CARTESIAN_POINT ( 'NONE',  ( 117.4906655440605334, -35.85895469176247019, 249.8927681330537780 ) ) ;
#85636=CARTESIAN_POINT ( 'NONE',  ( 48.45959712127302055, -26.00627455219131789, 342.9256252759109884 ) ) ;
#85638=EDGE_LOOP ( 'NONE', ( #69056, #40239, #19114, #13672 ) ) ;
#85640=AXIS2_PLACEMENT_3D ( 'NONE', #40371, #32207, #88543 ) ;
#85641=CARTESIAN_POINT ( 'NONE',  ( 113.6419851944692425, -45.67235822675655754, 183.0689586092439640 ) ) ;
#85642=ORIENTED_EDGE ( 'NONE', *, *, #66090, .F. ) ;
#85643=CARTESIAN_POINT ( 'NONE',  ( 95.56927879810542947, -39.60255952144336078, 166.5213395616259788 ) ) ;
#85644=DIRECTION ( 'NONE',  ( 1.000000000000000078E-15, 1.000000000000000083E-30, -1.000000000000000000 ) ) ;
#85649=CARTESIAN_POINT ( 'NONE',  ( 104.4161250475293485, -26.02246701806305751, 236.2575300378159682 ) ) ;
#85650=FACE_OUTER_BOUND ( 'NONE', #75357, .T. ) ;
#85651=DIRECTION ( 'NONE',  ( 1.000000000000000078E-15, 1.000000000000000083E-30, -1.000000000000000000 ) ) ;
#85653=CARTESIAN_POINT ( 'NONE',  ( 97.31592806723080002, -39.30618353892086958, 272.5310398921420756 ) ) ;
#85654=CARTESIAN_POINT ( 'NONE',  ( 107.0664832912739968, 22.62155284005901024, 333.4006252759110112 ) ) ;
#85655=CARTESIAN_POINT ( 'NONE',  ( 105.7995184719876960, -26.72403496767840281, 256.1772919438192275 ) ) ;
#85657=CARTESIAN_POINT ( 'NONE',  ( 110.6252048999878497, -43.92627768550128309, 195.5838068554168387 ) ) ;
#85658=ORIENTED_EDGE ( 'NONE', *, *, #84604, .F. ) ;
#85659=DIRECTION ( 'NONE',  ( 1.000000000000000000, 4.510281037539819615E-14, 0.000000000000000000 ) ) ;
#85660=CARTESIAN_POINT ( 'NONE',  ( 102.9583934913338652, -26.44260899983745006, 175.3908633711489813 ) ) ;
#85661=CARTESIAN_POINT ( 'NONE',  ( 117.4474071775726287, -37.68804338056689573, 74.75276813305397638 ) ) ;
#85662=CARTESIAN_POINT ( 'NONE',  ( 99.25607838769128932, -29.75875458388292571, 186.7470538473389752 ) ) ;
#85664=DIRECTION ( 'NONE',  ( 1.000000000000000000, 4.163336342344333240E-14, 0.000000000000000000 ) ) ;
#85666=CARTESIAN_POINT ( 'NONE',  ( 168.3595971214442102, -48.62134037892998606, 249.9678068554149775 ) ) ;
#85668=LINE ( 'NONE', #23445, #85714 ) ;
#85669=CYLINDRICAL_SURFACE ( 'NONE', #89120, 2.750000000000002665 ) ;
#85670=EDGE_LOOP ( 'NONE', ( #5634, #62418, #85378, #59273, #26058, #81134 ) ) ;
#85671=FACE_OUTER_BOUND ( 'NONE', #20269, .T. ) ;
#85672=EDGE_CURVE ( 'NONE', #22054, #54909, #64882, .T. ) ;
#85673=ORIENTED_EDGE ( 'NONE', *, *, #51827, .T. ) ;
#85674=ORIENTED_EDGE ( 'NONE', *, *, #15356, .F. ) ;
#85675=CARTESIAN_POINT ( 'NONE',  ( 98.52328466580365784, -37.41198607556916755, 100.8124198280769832 ) ) ;
#85676=AXIS2_PLACEMENT_3D ( 'NONE', #21575, #83799, #49242 ) ;
#85679=CARTESIAN_POINT ( 'NONE',  ( 117.5733473178507467, -42.15660255127702527, 89.44705384733997278 ) ) ;
#85682=CARTESIAN_POINT ( 'NONE',  ( 79.87807227643494912, -15.97944715994105813, 8.225625275910944723 ) ) ;
#85683=CARTESIAN_POINT ( 'NONE',  ( 46.83715912545429205, -47.82818131006082751, 249.9678068554150343 ) ) ;
#85684=CARTESIAN_POINT ( 'NONE',  ( 96.85055626654745708, -38.51091292166576352, 46.45181575210194325 ) ) ;
#85685=ORIENTED_EDGE ( 'NONE', *, *, #81837, .T. ) ;
#85686=ORIENTED_EDGE ( 'NONE', *, *, #31436, .F. ) ;
#85687=CIRCLE ( 'NONE', #81343, 9.571100913904507124 ) ;
#85691=DIRECTION ( 'NONE',  ( 0.000000000000000000, 0.000000000000000000, -1.000000000000000000 ) ) ;
#85692=DIRECTION ( 'NONE',  ( 0.000000000000000000, 0.000000000000000000, -1.000000000000000000 ) ) ;
#85694=CARTESIAN_POINT ( 'NONE',  ( 165.9667039024459996, -26.71338133339301635, -5.074374724088000832 ) ) ;
#85695=CARTESIAN_POINT ( 'NONE',  ( 97.80395968718781319, -40.49850023374117569, 52.63358577967416352 ) ) ;
#85696=VECTOR ( 'NONE', #72203, 1000.000000000000000 ) ;
#85699=CARTESIAN_POINT ( 'NONE',  ( 96.97787942770413849, -32.27031107066116533, 55.98324432352897162 ) ) ;
#85701=ORIENTED_EDGE ( 'NONE', *, *, #86029, .F. ) ;
#85702=EDGE_CURVE ( 'NONE', #83669, #87871, #88192, .T. ) ;
#85703=CARTESIAN_POINT ( 'NONE',  ( 108.4174897361023824, -26.73503600100527677, 269.9689585707081960 ) ) ;
#85705=FACE_OUTER_BOUND ( 'NONE', #74174, .T. ) ;
#85706=CARTESIAN_POINT ( 'NONE',  ( 114.9723337227840005, -34.69788249897437993, 121.8452332267339671 ) ) ;
#85707=EDGE_CURVE ( 'NONE', #27001, #14582, #51836, .T. ) ;
#85708=DIRECTION ( 'NONE',  ( 0.000000000000000000, 0.000000000000000000, -1.000000000000000000 ) ) ;
#85711=ORIENTED_EDGE ( 'NONE', *, *, #70721, .F. ) ;
#85712=EDGE_LOOP ( 'NONE', ( #33672, #81241 ) ) ;
#85713=LINE ( 'NONE', #63458, #80137 ) ;
#85714=VECTOR ( 'NONE', #51111, 1000.000000000000000 ) ;
#85715=ORIENTED_EDGE ( 'NONE', *, *, #82831, .F. ) ;
#85716=ORIENTED_EDGE ( 'NONE', *, *, #71760, .F. ) ;
#85718=CARTESIAN_POINT ( 'NONE',  ( 99.92577194148378794, -31.43111053364522434, 177.2501547344679693 ) ) ;
#85721=CARTESIAN_POINT ( 'NONE',  ( 96.67756931115832231, -37.82841265861588909, 122.4099109901969626 ) ) ;
#85722=DIRECTION ( 'NONE',  ( -1.000000000000000000, -4.163336342344275811E-14, 0.000000000000000000 ) ) ;
#85723=CARTESIAN_POINT ( 'NONE',  ( 116.7474494541973087, -34.15064250361619003, 19.03369576739390823 ) ) ;
#85725=AXIS2_PLACEMENT_3D ( 'NONE', #52259, #11408, #60437 ) ;
#85729=EDGE_CURVE ( 'NONE', #73068, #82750, #83611, .T. ) ;
#85730=CARTESIAN_POINT ( 'NONE',  ( 109.7539934464052465, -29.02185251678796618, 207.6280903695909501 ) ) ;
#85731=CARTESIAN_POINT ( 'NONE',  ( 114.3686432469292527, -44.20104832357726110, 73.19276813305397411 ) ) ;
#85732=EDGE_LOOP ( 'NONE', ( #5460, #4690, #26712, #62927 ) ) ;
#85733=CARTESIAN_POINT ( 'NONE',  ( 115.8731522275743941, -31.19128430790902584, 34.27276813305396530 ) ) ;
#85734=CARTESIAN_POINT ( 'NONE',  ( 102.6743760996991597, -27.25069970728465307, 176.4213395616249898 ) ) ;
#85735=EDGE_CURVE ( 'NONE', #76359, #16547, #14109, .T. ) ;
#85738=CARTESIAN_POINT ( 'NONE',  ( 114.0809025726587436, -44.48955379074138961, 129.1613395616249704 ) ) ;
#85739=VECTOR ( 'NONE', #89709, 1000.000000000000000 ) ;
#85740=CARTESIAN_POINT ( 'NONE',  ( 182.5667039024459939, -19.82844715994031048, -5.074374724088000832 ) ) ;
#85744=CIRCLE ( 'NONE', #32019, 10.00000000000000711 ) ;
#85747=CARTESIAN_POINT ( 'NONE',  ( 108.3338899180770625, -46.73481428249178293, 133.6785589755952799 ) ) ;
#85750=VECTOR ( 'NONE', #17603, 1000.000000000000000 ) ;
#85751=DIRECTION ( 'NONE',  ( 0.7071067811865473507, 0.000000000000000000, -0.7071067811865476838 ) ) ;
#85752=CARTESIAN_POINT ( 'NONE',  ( 112.5942678722098123, -28.35481117739004731, 130.6124851771425881 ) ) ;
#85753=CARTESIAN_POINT ( 'NONE',  ( 106.9273489086460387, -26.26968863985776537, 60.08705384733897858 ) ) ;
#85757=CARTESIAN_POINT ( 'NONE',  ( 112.5987260342905358, -28.66361022110268308, 44.59848241876795782 ) ) ;
#85758=CARTESIAN_POINT ( 'NONE',  ( 72.06648329127402519, -45.72944715994106701, -4.824374724089063982 ) ) ;
#85759=CARTESIAN_POINT ( 'NONE',  ( 108.8451227504523189, -46.97957433935474825, 163.7127681330539701 ) ) ;
#85763=VECTOR ( 'NONE', #77459, 1000.000000000000000 ) ;
#85764=CARTESIAN_POINT ( 'NONE',  ( 19.56648329127303043, -71.37844715994266664, 361.9756252759109998 ) ) ;
#85767=CIRCLE ( 'NONE', #78505, 4.750000000000000888 ) ;
#85768=PLANE ( 'NONE',  #89790 ) ;
#85769=CARTESIAN_POINT ( 'NONE',  ( 112.2268274879326668, -45.83864656583022423, 212.9870538473389558 ) ) ;
#85771=CARTESIAN_POINT ( 'NONE',  ( 109.7247347643963167, -27.00076673087112766, 144.8648027181440909 ) ) ;
#85772=CARTESIAN_POINT ( 'NONE',  ( 105.6290766085263044, -47.07696477925017575, 253.4670538473393719 ) ) ;
#85773=CARTESIAN_POINT ( 'NONE',  ( 102.9539626486510713, -46.35650038051790744, 88.25562527591095829 ) ) ;
#85774=CARTESIAN_POINT ( 'NONE',  ( 33.78309357196401663, -29.99615139349950965, -5.074374724088000832 ) ) ;
#85775=CARTESIAN_POINT ( 'NONE',  ( 97.06112902794230024, -37.99671193374311429, 192.4271787320971043 ) ) ;
#85777=ORIENTED_EDGE ( 'NONE', *, *, #69793, .T. ) ;
#85783=CARTESIAN_POINT ( 'NONE',  ( 110.9930042498355363, -46.38681234365495953, 278.8841967044824059 ) ) ;
#85785=CARTESIAN_POINT ( 'NONE',  ( 132.7641780748886049, -34.30680158339101382, 1.893168945965612471 ) ) ;
#85787=FACE_OUTER_BOUND ( 'NONE', #26009, .T. ) ;
#85788=FACE_OUTER_BOUND ( 'NONE', #26443, .T. ) ;
#85790=CARTESIAN_POINT ( 'NONE',  ( 97.51448592794399417, -38.47012922887837760, 200.8924198280769815 ) ) ;
#85792=ORIENTED_EDGE ( 'NONE', *, *, #6307, .T. ) ;
#85794=AXIS2_PLACEMENT_3D ( 'NONE', #60328, #73520, #32179 ) ;
#85798=EDGE_CURVE ( 'NONE', #2462, #1233, #83169, .T. ) ;
#85799=CARTESIAN_POINT ( 'NONE',  ( 109.8085987287837213, -27.34093086507540704, 255.8499109901960367 ) ) ;
#85800=DIRECTION ( 'NONE',  ( -0.7071067811865794361, 0.7071067811865157093, -7.071067811865803697E-16 ) ) ;
#85801=EDGE_CURVE ( 'NONE', #26492, #28372, #34086, .T. ) ;
#85802=DIRECTION ( 'NONE',  ( 0.000000000000000000, 2.135044278125299371E-15, -1.000000000000000000 ) ) ;
#85803=CARTESIAN_POINT ( 'NONE',  ( 165.6738106836030227, -28.98061976758901892, 117.4678068554150627 ) ) ;
#85804=EDGE_CURVE ( 'NONE', #83210, #8807, #6393, .T. ) ;
#85805=VECTOR ( 'NONE', #83333, 1000.000000000000000 ) ;
#85807=ADVANCED_FACE ( 'NONE', ( #5515 ), #33656, .T. ) ;
#85808=CARTESIAN_POINT ( 'NONE',  ( 77.49614765539782013, -35.75123073100116500, 2.855912073278434438 ) ) ;
#85809=VERTEX_POINT ( 'NONE', #60909 ) ;
#85810=DIRECTION ( 'NONE',  ( 0.9068632946707806397, -0.4214249218767879279, 9.068632946707804446E-16 ) ) ;
#85811=CARTESIAN_POINT ( 'NONE',  ( 103.6908924260029607, -28.08645471411401928, 18.19094751244793073 ) ) ;
#85812=CIRCLE ( 'NONE', #1700, 0.5000000000000004441 ) ;
#85813=EDGE_CURVE ( 'NONE', #80451, #18492, #27285, .T. ) ;
#85814=CARTESIAN_POINT ( 'NONE',  ( 136.8000579002609811, -18.42904715602391263, 6.774297104452461582 ) ) ;
#85815=EDGE_CURVE ( 'NONE', #52459, #44341, #11170, .T. ) ;
#85816=DIRECTION ( 'NONE',  ( 1.639958061481212836E-42, -4.100000000000000342E-29, -1.000000000000000000 ) ) ;
#85818=CARTESIAN_POINT ( 'NONE',  ( 107.0664832912739968, -36.72944715994100306, 9.635625275910941312 ) ) ;
#85823=CARTESIAN_POINT ( 'NONE',  ( 115.1669806615814622, -43.29214270484202132, 88.28419670448195689 ) ) ;
#85824=ORIENTED_EDGE ( 'NONE', *, *, #23972, .F. ) ;
#85825=CARTESIAN_POINT ( 'NONE',  ( 114.2970346969270565, -32.18244176163005221, 33.69527697093299423 ) ) ;
#85826=ADVANCED_FACE ( 'NONE', ( #82725, #26392, #46808 ), #74541, .T. ) ;
#85828=CARTESIAN_POINT ( 'NONE',  ( 101.9660762386545514, -28.83879614530413704, 66.97682140113498406 ) ) ;
#85829=CARTESIAN_POINT ( 'NONE',  ( 116.7946685605787849, -39.38945716434293587, 14.61465845921219575 ) ) ;
#85831=DIRECTION ( 'NONE',  ( 1.000000000000000000, 4.163336342344333240E-14, 0.000000000000000000 ) ) ;
#85832=CARTESIAN_POINT ( 'NONE',  ( 97.78987344453990715, -29.31549002224505429, 41.78991099019596334 ) ) ;
#85834=EDGE_LOOP ( 'NONE', ( #35690, #31946, #52150, #77504 ) ) ;
#85835=LINE ( 'NONE', #79007, #87932 ) ;
#85837=CARTESIAN_POINT ( 'NONE',  ( 102.3735796352302714, -26.67091080359734434, 131.4118157521009778 ) ) ;
#85839=ORIENTED_EDGE ( 'NONE', *, *, #39487, .T. ) ;
#85840=VERTEX_POINT ( 'NONE', #20489 ) ;
#85841=AXIS2_PLACEMENT_3D ( 'NONE', #37050, #16172, #43851 ) ;
#85844=CARTESIAN_POINT ( 'NONE',  ( 104.6152064257953498, -27.26083179018618452, 200.2784824187689310 ) ) ;
#85846=FACE_OUTER_BOUND ( 'NONE', #55457, .T. ) ;
#85847=FACE_OUTER_BOUND ( 'NONE', #46721, .T. ) ;
#85848=CARTESIAN_POINT ( 'NONE',  ( 97.10477362122047396, -39.80301782323012105, 17.56419670448195092 ) ) ;
#85849=CARTESIAN_POINT ( 'NONE',  ( 127.0664832912740110, -54.72944906728950798, 14.67562527591099197 ) ) ;
#85850=EDGE_CURVE ( 'NONE', #30894, #13404, #48897, .T. ) ;
#85851=ORIENTED_EDGE ( 'NONE', *, *, #38752, .F. ) ;
#85853=EDGE_CURVE ( 'NONE', #20676, #40647, #28554, .T. ) ;
#85854=DIRECTION ( 'NONE',  ( 0.000000000000000000, 0.000000000000000000, 1.000000000000000000 ) ) ;
#85855=AXIS2_PLACEMENT_3D ( 'NONE', #54, #500, #14134 ) ;
#85857=AXIS2_PLACEMENT_3D ( 'NONE', #85633, #56085, #35206 ) ;
#85860=CARTESIAN_POINT ( 'NONE',  ( 101.3060704567421197, -26.40153104436172526, 255.4813395616251626 ) ) ;
#85862=CARTESIAN_POINT ( 'NONE',  ( 41.56648329127499153, -32.07844715994070839, 258.9256252759120116 ) ) ;
#85863=CARTESIAN_POINT ( 'NONE',  ( 98.70294500015674544, -34.99527330041078699, 215.5867055423629779 ) ) ;
#85864=DIRECTION ( 'NONE',  ( -1.000000000000000078E-15, 1.000000000000000083E-30, 1.000000000000000000 ) ) ;
#85865=CARTESIAN_POINT ( 'NONE',  ( 105.4244226815142298, -47.00233879195495490, 33.44991099019695469 ) ) ;
#85866=DIRECTION ( 'NONE',  ( 0.000000000000000000, 0.000000000000000000, -1.000000000000000000 ) ) ;
#85867=CARTESIAN_POINT ( 'NONE',  ( 113.3579092357397542, -45.09751872455207433, 143.0899109901969553 ) ) ;
#85868=ORIENTED_EDGE ( 'NONE', *, *, #86231, .F. ) ;
#85869=CARTESIAN_POINT ( 'NONE',  ( 131.4143329470395827, -19.45719076514318502, 6.889371645759392315 ) ) ;
#85870=ORIENTED_EDGE ( 'NONE', *, *, #84039, .F. ) ;
#85872=DIRECTION ( 'NONE',  ( 1.000000000000000000, 1.261617073437676668E-15, 9.462128050782575008E-16 ) ) ;
#85873=ORIENTED_EDGE ( 'NONE', *, *, #15010, .F. ) ;
#85875=DIRECTION ( 'NONE',  ( -0.7071067811865279218, 0.7071067811865670016, -6.612322855859973915E-17 ) ) ;
#85878=DIRECTION ( 'NONE',  ( -1.000000000000000000, 1.271620792853953879E-14, 0.000000000000000000 ) ) ;
#85879=DIRECTION ( 'NONE',  ( 2.900000000000000265E-14, -2.000000000000000155E-15, 1.000000000000000000 ) ) ;
#85880=ORIENTED_EDGE ( 'NONE', *, *, #6345, .T. ) ;
#85881=VECTOR ( 'NONE', #51262, 999.9999999999998863 ) ;
#85882=CARTESIAN_POINT ( 'NONE',  ( 107.2325596213128875, -25.65389481303129315, 80.07657765686299456 ) ) ;
#85884=CARTESIAN_POINT ( 'NONE',  ( 97.06384678839589242, -37.34232347881079761, 166.3752407659725918 ) ) ;
#85885=DIRECTION ( 'NONE',  ( 0.000000000000000000, 0.000000000000000000, 1.000000000000000000 ) ) ;
#85887=VERTEX_POINT ( 'NONE', #19573 ) ;
#85890=CARTESIAN_POINT ( 'NONE',  ( 107.0664832912739399, -36.72944715994096754, 298.1356252759109680 ) ) ;
#85894=CARTESIAN_POINT ( 'NONE',  ( 97.81169461453751524, -40.51741999607308742, 142.6356648221729131 ) ) ;
#85895=CARTESIAN_POINT ( 'NONE',  ( 163.0664832912739826, -18.82844715994099971, 333.4006252759120343 ) ) ;
#85896=CARTESIAN_POINT ( 'NONE',  ( 162.8913605087221868, -31.76306994223289948, 237.4678068554150059 ) ) ;
#85897=VERTEX_POINT ( 'NONE', #14114 ) ;
#85898=ADVANCED_FACE ( 'NONE', ( #74992 ), #12775, .T. ) ;
#85899=FACE_OUTER_BOUND ( 'NONE', #19939, .T. ) ;
#85900=ADVANCED_FACE ( 'NONE', ( #28631 ), #49506, .T. ) ;
#85901=CARTESIAN_POINT ( 'NONE',  ( 109.6835627966674878, -27.30531164764932939, 170.8613395616249591 ) ) ;
#85904=EDGE_CURVE ( 'NONE', #78471, #25006, #57608, .T. ) ;
#85905=CARTESIAN_POINT ( 'NONE',  ( 100.8736165617014677, -44.32606212243579336, 8.032768133052980986 ) ) ;
#85906=DIRECTION ( 'NONE',  ( 1.175184669632759901E-16, -1.000000000000000000, -2.000000000000003705E-15 ) ) ;
#85907=LINE ( 'NONE', #37744, #38590 ) ;
#85908=CARTESIAN_POINT ( 'NONE',  ( 117.0603303411406984, -38.08442816249873886, 13.71933068259133748 ) ) ;
#85910=VERTEX_POINT ( 'NONE', #1385 ) ;
#85911=CARTESIAN_POINT ( 'NONE',  ( 104.4908855836804236, -26.97855169986425494, 30.28161050152675315 ) ) ;
#85912=CARTESIAN_POINT ( 'NONE',  ( 115.9419818307744663, -40.91744192719425399, 228.4756252759109714 ) ) ;
#85913=ORIENTED_EDGE ( 'NONE', *, *, #16010, .F. ) ;
#85915=VERTEX_POINT ( 'NONE', #29089 ) ;
#85916=CARTESIAN_POINT ( 'NONE',  ( 113.0661788413732580, -30.20779614827405624, 195.9158690201829529 ) ) ;
#85917=ADVANCED_FACE ( 'NONE', ( #57218 ), #63605, .F. ) ;
#85918=CIRCLE ( 'NONE', #11983, 2.117000000000007987 ) ;
#85919=LINE ( 'NONE', #59057, #2311 ) ;
#85920=CARTESIAN_POINT ( 'NONE',  ( 115.9247622085524085, -36.97270265434710979, 40.23586902018294609 ) ) ;
#85926=CARTESIAN_POINT ( 'NONE',  ( 83.06670390244806867, -51.22944715994108122, 207.5838068554169809 ) ) ;
#85927=CYLINDRICAL_SURFACE ( 'NONE', #24143, 3.000000000000002665 ) ;
#85928=ORIENTED_EDGE ( 'NONE', *, *, #41483, .F. ) ;
#85929=CARTESIAN_POINT ( 'NONE',  ( 108.0121126588926046, -24.94157235513505100, 265.0127681330535552 ) ) ;
#85930=CARTESIAN_POINT ( 'NONE',  ( 152.0371591254583450, -47.82818131005588214, 249.9678068554149490 ) ) ;
#85932=AXIS2_PLACEMENT_3D ( 'NONE', #5247, #32486, #82018 ) ;
#85935=DIRECTION ( 'NONE',  ( -0.7071067811567310901, 0.7071067812163639443, 0.000000000000000000 ) ) ;
#85936=PLANE ( 'NONE',  #14264 ) ;
#85938=CARTESIAN_POINT ( 'NONE',  ( 100.2135729606528685, -43.75450166055420453, 17.96133956162493206 ) ) ;
#85941=VECTOR ( 'NONE', #4392, 1000.000000000000000 ) ;
#85942=CARTESIAN_POINT ( 'NONE',  ( 96.91449086013869874, -32.24229349230230923, 51.98324432352996638 ) ) ;
#85943=CARTESIAN_POINT ( 'NONE',  ( 80.06648329127399677, -36.72944715994107412, 14.92562527591094224 ) ) ;
#85944=CARTESIAN_POINT ( 'NONE',  ( 117.4299418851264818, -35.59553461117717887, 278.9127681330539872 ) ) ;
#85947=CARTESIAN_POINT ( 'NONE',  ( 78.94219388974352114, -39.23922437001928643, 8.028287874532400892 ) ) ;
#85948=DIRECTION ( 'NONE',  ( 0.7071067811566161820, 0.7071067812164789634, 0.000000000000000000 ) ) ;
#85949=PLANE ( 'NONE',  #37859 ) ;
#85950=CARTESIAN_POINT ( 'NONE',  ( 115.5296723907996039, -38.53924143319417794, 106.4890427505429642 ) ) ;
#85951=CARTESIAN_POINT ( 'NONE',  ( 117.4343095520634108, -35.18433407802718449, 214.9441967044829767 ) ) ;
#85953=DIRECTION ( 'NONE',  ( 1.000000000000000078E-15, -1.000000000000000000, 0.000000000000000000 ) ) ;
#85955=EDGE_CURVE ( 'NONE', #41740, #4309, #74986, .T. ) ;
#85957=ORIENTED_EDGE ( 'NONE', *, *, #13077, .T. ) ;
#85958=ORIENTED_EDGE ( 'NONE', *, *, #39825, .F. ) ;
#85959=DIRECTION ( 'NONE',  ( 0.000000000000000000, 1.000000000000000000, 2.000000000000000155E-15 ) ) ;
#85961=EDGE_LOOP ( 'NONE', ( #88741, #1087 ) ) ;
#85963=CARTESIAN_POINT ( 'NONE',  ( 110.1026808908064680, -27.16648640359800382, 40.83168070709650976 ) ) ;
#85964=CARTESIAN_POINT ( 'NONE',  ( 108.3145574644059224, -45.20850512633867169, 142.1152769709339907 ) ) ;
#85965=CARTESIAN_POINT ( 'NONE',  ( 96.86726761138238828, -30.64586122335317953, 280.8984824187682534 ) ) ;
#85966=AXIS2_PLACEMENT_3D ( 'NONE', #5786, #81208, #39394 ) ;
#85969=EDGE_CURVE ( 'NONE', #32919, #4843, #43520, .T. ) ;
#85970=CARTESIAN_POINT ( 'NONE',  ( 103.4484542752979053, -27.40651198025439328, 136.3710560532725253 ) ) ;
#85971=ORIENTED_EDGE ( 'NONE', *, *, #33629, .T. ) ;
#85973=CARTESIAN_POINT ( 'NONE',  ( 112.0646398527721317, -45.48910543467338385, 32.98989392684662647 ) ) ;
#85976=EDGE_CURVE ( 'NONE', #241, #48806, #70658, .T. ) ;
#85977=CARTESIAN_POINT ( 'NONE',  ( 149.4409906032288404, -0.9156555935619370423, 361.9756252759100335 ) ) ;
#85978=EDGE_LOOP ( 'NONE', ( #58918, #33469, #28606, #9800 ) ) ;
#85979=CARTESIAN_POINT ( 'NONE',  ( 109.9893001866846163, -26.72224116339410571, 259.8499109901965767 ) ) ;
#85980=CARTESIAN_POINT ( 'NONE',  ( 118.1215414109737196, -37.72100569522838498, 29.74324432352998215 ) ) ;
#85982=CARTESIAN_POINT ( 'NONE',  ( 115.0372575041536578, -42.90846256976404760, 119.3022919422766392 ) ) ;
#85984=DIRECTION ( 'NONE',  ( 0.000000000000000000, -1.000000000000000000, 0.000000000000000000 ) ) ;
#85985=DIRECTION ( 'NONE',  ( 0.000000000000000000, 1.000000000000000000, 0.000000000000000000 ) ) ;
#85986=FACE_OUTER_BOUND ( 'NONE', #89931, .T. ) ;
#85987=CARTESIAN_POINT ( 'NONE',  ( 131.8668787344651037, -38.38871026388260077, 7.389079501614427947 ) ) ;
#85988=CARTESIAN_POINT ( 'NONE',  ( 115.8254323908514323, -31.73001882614791214, 10.23979194279731075 ) ) ;
#85991=CARTESIAN_POINT ( 'NONE',  ( 102.4390861222961888, -38.62343645255491253, 9.635625275910941312 ) ) ;
#85993=CARTESIAN_POINT ( 'NONE',  ( 100.0090739042524604, -28.97838942479177149, 285.6641967044823787 ) ) ;
#85994=CARTESIAN_POINT ( 'NONE',  ( 96.61884675261427446, -36.21154414529181764, 167.2870538473399620 ) ) ;
#85995=CARTESIAN_POINT ( 'NONE',  ( 115.6290845971308414, -28.50119646097363812, 35.43562527591098643 ) ) ;
#85996=CARTESIAN_POINT ( 'NONE',  ( 41.56648329127398966, -18.82844715994071194, 15.92562527591207022 ) ) ;
#85997=DIRECTION ( 'NONE',  ( 0.000000000000000000, 1.000000000000000000, 0.000000000000000000 ) ) ;
#85998=DIRECTION ( 'NONE',  ( 0.9825752044328147639, 0.1858654557302462929, 0.000000000000000000 ) ) ;
#85999=AXIS2_PLACEMENT_3D ( 'NONE', #67843, #33323, #46483 ) ;
#86000=ORIENTED_EDGE ( 'NONE', *, *, #75330, .T. ) ;
#86001=ADVANCED_FACE ( 'NONE', ( #30870 ), #51733, .F. ) ;
#86002=DIRECTION ( 'NONE',  ( 0.000000000000000000, -1.000000000000000000, 0.000000000000000000 ) ) ;
#86003=ORIENTED_EDGE ( 'NONE', *, *, #76437, .T. ) ;
#86006=CARTESIAN_POINT ( 'NONE',  ( 107.3052971647831697, -26.36210646096938959, 71.04610146638695767 ) ) ;
#86009=CARTESIAN_POINT ( 'NONE',  ( 98.30751720600149213, -41.72883398697895529, 47.73978837389122987 ) ) ;
#86011=CARTESIAN_POINT ( 'NONE',  ( 107.2427983594548948, -47.16656068249876910, 208.5899109901969837 ) ) ;
#86013=DIRECTION ( 'NONE',  ( 0.000000000000000000, 1.000000000000000000, 0.000000000000000000 ) ) ;
#86015=CARTESIAN_POINT ( 'NONE',  ( 97.33784130656839295, -34.07106454601533585, 47.11479194387641201 ) ) ;
#86017=EDGE_CURVE ( 'NONE', #829, #43762, #4050, .T. ) ;
#86018=CARTESIAN_POINT ( 'NONE',  ( 113.3725682976012052, -44.50658906070807319, 98.11867516117681021 ) ) ;
#86019=CARTESIAN_POINT ( 'NONE',  ( 108.2420053567034017, -46.43931755893584779, 117.6727681330539639 ) ) ;
#86021=ORIENTED_EDGE ( 'NONE', *, *, #72155, .F. ) ;
#86022=CARTESIAN_POINT ( 'NONE',  ( 115.8258230018156354, -33.33084548093709287, 90.54063092494496345 ) ) ;
#86023=EDGE_CURVE ( 'NONE', #68920, #70782, #24504, .T. ) ;
#86025=CARTESIAN_POINT ( 'NONE',  ( 99.34779341711927714, -29.80408710710938891, 231.7565776568629587 ) ) ;
#86026=CYLINDRICAL_SURFACE ( 'NONE', #10023, 2.116999999999993776 ) ;
#86027=CARTESIAN_POINT ( 'NONE',  ( 188.5667039024485518, -48.82844715993430640, 173.2178068554150059 ) ) ;
#86029=EDGE_CURVE ( 'NONE', #52709, #2908, #65390, .T. ) ;
#86030=DIRECTION ( 'NONE',  ( 1.000000000000000000, 4.299999999999999979E-14, 1.000000000000000078E-15 ) ) ;
#86031=CARTESIAN_POINT ( 'NONE',  ( 107.0664832912739257, -50.72944715994095333, 312.1356252759112522 ) ) ;
#86032=AXIS2_PLACEMENT_3D ( 'NONE', #38835, #33368, #67432 ) ;
#86034=LINE ( 'NONE', #44207, #3777 ) ;
#86035=CARTESIAN_POINT ( 'NONE',  ( 101.9826776100855454, -46.51815199768669373, 167.1832443235299763 ) ) ;
#86039=DIRECTION ( 'NONE',  ( -0.0001713722456129692653, 0.9999999853157764962, 0.000000000000000000 ) ) ;
#86040=CARTESIAN_POINT ( 'NONE',  ( 99.04406184703033489, -42.84125762489144051, 77.84395860774790776 ) ) ;
#86041=CARTESIAN_POINT ( 'NONE',  ( 115.0371094337952940, -42.90866003816787355, 104.3022725537445297 ) ) ;
#86042=CARTESIAN_POINT ( 'NONE',  ( 112.9694095044039841, -31.09161174735247002, 232.2509475124489597 ) ) ;
#86043=CONICAL_SURFACE ( 'NONE', #25066, 13.31607168056649826, 0.1047197551196538678 ) ;
#86044=DIRECTION ( 'NONE',  ( -4.237773401492740281E-14, 1.000000000000000000, 0.000000000000000000 ) ) ;
#86045=CARTESIAN_POINT ( 'NONE',  ( 107.5657785589506688, -47.77162953885341778, 192.6003871806729535 ) ) ;
#86046=DIRECTION ( 'NONE',  ( 0.000000000000000000, 1.000000000000000000, 0.000000000000000000 ) ) ;
#86047=EDGE_LOOP ( 'NONE', ( #46140, #25737 ) ) ;
#86049=ORIENTED_EDGE ( 'NONE', *, *, #84039, .T. ) ;
#86050=CARTESIAN_POINT ( 'NONE',  ( 112.4825976992256074, -45.17049497366694766, 64.03124135276239315 ) ) ;
#86053=CARTESIAN_POINT ( 'NONE',  ( 106.8709381294020488, -45.58890767966684621, 268.9901547344683763 ) ) ;
#86054=CARTESIAN_POINT ( 'NONE',  ( 115.0372572128023450, -42.90846295832322710, 273.3022919040415672 ) ) ;
#86057=CARTESIAN_POINT ( 'NONE',  ( 116.3481150955673087, -39.37902819411457500, 9.635625275910941312 ) ) ;
#86058=FACE_OUTER_BOUND ( 'NONE', #68183, .T. ) ;
#86059=ORIENTED_EDGE ( 'NONE', *, *, #42568, .F. ) ;
#86060=EDGE_LOOP ( 'NONE', ( #66043, #52092, #52498, #42543 ) ) ;
#86062=DIRECTION ( 'NONE',  ( -0.9254794337955620787, -0.3787978585227822492, 0.000000000000000000 ) ) ;
#86067=CARTESIAN_POINT ( 'NONE',  ( 98.53948418117370522, -33.67937232826720617, 25.48765792331497693 ) ) ;
#86068=CARTESIAN_POINT ( 'NONE',  ( 116.6812525300504291, -40.81632573062672265, 168.5070538473399608 ) ) ;
#86069=CARTESIAN_POINT ( 'NONE',  ( 117.2009162446675390, -42.82382785266567993, 128.3956252759109873 ) ) ;
#86071=CARTESIAN_POINT ( 'NONE',  ( 115.9068016902149907, -30.09448287295081670, 260.3508633711493871 ) ) ;
#86072=CARTESIAN_POINT ( 'NONE',  ( 108.3335911829770453, -46.73484319673156762, 98.67887531062980599 ) ) ;
#86073=CARTESIAN_POINT ( 'NONE',  ( 75.31670390244798341, -50.82844715994100682, 58.80080685541479824 ) ) ;
#86075=ORIENTED_EDGE ( 'NONE', *, *, #23035, .F. ) ;
#86078=CARTESIAN_POINT ( 'NONE',  ( 117.4703304800641206, -30.95114626853415984, 179.2299109901959753 ) ) ;
#86079=ORIENTED_EDGE ( 'NONE', *, *, #69904, .F. ) ;
#86080=CARTESIAN_POINT ( 'NONE',  ( 96.74292298454378169, -35.27647329413149890, 181.2156252759109805 ) ) ;
#86081=CARTESIAN_POINT ( 'NONE',  ( 164.9190312289450162, -35.91149509760580116, 117.4678068554150485 ) ) ;
#86082=AXIS2_PLACEMENT_3D ( 'NONE', #26990, #1422, #8231 ) ;
#86083=CARTESIAN_POINT ( 'NONE',  ( 25.56670390244731550, -48.82844715994178841, 175.7178068554150627 ) ) ;
#86087=CARTESIAN_POINT ( 'NONE',  ( 99.39760893136107711, -29.69972230079153519, 271.7356252759109907 ) ) ;
#86088=CARTESIAN_POINT ( 'NONE',  ( 182.5667039024469886, -33.35206098992650681, -5.074374724088000832 ) ) ;
#86089=CARTESIAN_POINT ( 'NONE',  ( 107.0664832912739399, -36.72944715994095333, 293.6369201390379544 ) ) ;
#86090=CARTESIAN_POINT ( 'NONE',  ( 80.06648329127399677, -8.350947159940998787, 306.1181252759120071 ) ) ;
#86091=AXIS2_PLACEMENT_3D ( 'NONE', #3223, #9586, #9146 ) ;
#86095=CARTESIAN_POINT ( 'NONE',  ( 102.5058979696208041, -43.38806787210953786, 195.5838068554170661 ) ) ;
#86097=CARTESIAN_POINT ( 'NONE',  ( 135.3099415725432095, -21.18303583363543297, 7.982915248818459375 ) ) ;
#86098=CARTESIAN_POINT ( 'NONE',  ( 99.99311136543857970, -27.18998042936580362, 185.5841967044829630 ) ) ;
#86099=CARTESIAN_POINT ( 'NONE',  ( 98.59006141831567049, -43.82340604873675716, 67.86895860924497015 ) ) ;
#86100=CARTESIAN_POINT ( 'NONE',  ( 100.7971853062899896, -45.88878125878837011, 238.1108633711489517 ) ) ;
#86105=DIRECTION ( 'NONE',  ( -0.7071067811865187069, -0.7071067811865764385, -7.071067811865181482E-16 ) ) ;
#86108=VECTOR ( 'NONE', #76500, 1000.000000000000000 ) ;
#86109=DIRECTION ( 'NONE',  ( -0.9254794337955620787, -0.3787978585227822492, 0.000000000000000000 ) ) ;
#86111=ORIENTED_EDGE ( 'NONE', *, *, #81304, .T. ) ;
#86112=EDGE_CURVE ( 'NONE', #80585, #62559, #52167, .T. ) ;
#86113=CARTESIAN_POINT ( 'NONE',  ( 107.7867742379091567, -27.70205266993799142, 114.4476579233149636 ) ) ;
#86115=ORIENTED_EDGE ( 'NONE', *, *, #57465, .F. ) ;
#86116=EDGE_CURVE ( 'NONE', #67833, #68744, #32640, .T. ) ;
#86117=CARTESIAN_POINT ( 'NONE',  ( 116.5135284680787322, -32.37261310794437463, 100.1699109901969535 ) ) ;
#86119=EDGE_CURVE ( 'NONE', #84817, #2920, #10423, .T. ) ;
#86120=CARTESIAN_POINT ( 'NONE',  ( 77.55659459556460433, -17.60518703966017640, 7.068229416970193135 ) ) ;
#86121=CARTESIAN_POINT ( 'NONE',  ( 142.8832909413445122, -79.11588146349311046, 361.9756252759100335 ) ) ;
#86122=EDGE_CURVE ( 'NONE', #74315, #71626, #89524, .T. ) ;
#86123=CARTESIAN_POINT ( 'NONE',  ( 111.8803212371932148, -27.54331830560560590, 14.68038718067299442 ) ) ;
#86125=VERTEX_POINT ( 'NONE', #65818 ) ;
#86127=CARTESIAN_POINT ( 'NONE',  ( 57.56670390244747892, -48.82844715994040286, 137.2178068554150911 ) ) ;
#86130=CARTESIAN_POINT ( 'NONE',  ( 46.03715912545343514, -48.62818131006090283, 180.4678068554150911 ) ) ;
#86131=PLANE ( 'NONE',  #24767 ) ;
#86136=CARTESIAN_POINT ( 'NONE',  ( 103.9639062230918825, -47.31423993612443724, 62.33753003781600199 ) ) ;
#86137=EDGE_LOOP ( 'NONE', ( #64084, #80015, #63012, #41116 ) ) ;
#86140=DIRECTION ( 'NONE',  ( 1.000000000000000000, 4.237773401492740281E-14, 0.000000000000000000 ) ) ;
#86141=CARTESIAN_POINT ( 'NONE',  ( 108.0140583617620820, -28.59404368299928123, 127.8023760838769505 ) ) ;
#86142=AXIS2_PLACEMENT_3D ( 'NONE', #77649, #65350, #71728 ) ;
#86143=VECTOR ( 'NONE', #72141, 1000.000000000000000 ) ;
#86144=CARTESIAN_POINT ( 'NONE',  ( 107.0664832912739257, -52.72944715994094622, 302.7856252759109452 ) ) ;
#86145=CARTESIAN_POINT ( 'NONE',  ( 107.0664832912740110, -46.47944715994103149, 14.92562527591097066 ) ) ;
#86146=ORIENTED_EDGE ( 'NONE', *, *, #7663, .T. ) ;
#86147=VERTEX_POINT ( 'NONE', #73986 ) ;
#86152=CARTESIAN_POINT ( 'NONE',  ( 116.1908163682739712, -34.48822628859398520, 160.4377737820879588 ) ) ;
#86154=CARTESIAN_POINT ( 'NONE',  ( 99.40614514399899804, -27.65486269830070398, 146.6356252759109395 ) ) ;
#86157=CARTESIAN_POINT ( 'NONE',  ( 99.04406183952015397, -42.84125761515226571, 82.84395860677673795 ) ) ;
#86160=B_SPLINE_CURVE_WITH_KNOTS ( 'NONE', 3,
 ( #30088, #56879, #84623, #22381, #58234, #42344, #50060, #52714, #3280, #11423, #37795, #39567, #60452, #66372, #24172, #79592, #32297, #45032 ),
 .UNSPECIFIED., .F., .F.,
 ( 4, 2, 2, 2, 2, 2, 2, 2, 4 ),
 ( 0.000000000000000000, 0.06249555305220369505, 0.1249911061044073901, 0.1874866591566110852, 0.2499822122088147802, 0.3124777652610184475, 0.3749733183132221703, 0.4374688713654258931, 0.4999644244176295604 ),
 .UNSPECIFIED. ) ;
#86163=CARTESIAN_POINT ( 'NONE',  ( 107.5268921225462719, -45.37172398690709230, 195.4490427505439811 ) ) ;
#86164=CARTESIAN_POINT ( 'NONE',  ( 115.0395865772315034, -43.53517906860128051, 63.26419670448196797 ) ) ;
#86165=ORIENTED_EDGE ( 'NONE', *, *, #45922, .F. ) ;
#86166=CARTESIAN_POINT ( 'NONE',  ( 99.77739493559400330, -44.20163642594134501, 21.96133956162593748 ) ) ;
#86167=DIRECTION ( 'NONE',  ( -4.012088370409549976E-14, 1.000000000000000000, 0.000000000000000000 ) ) ;
#86169=CARTESIAN_POINT ( 'NONE',  ( 83.06670390244796920, -58.72944715994093912, 207.5838068554149913 ) ) ;
#86170=CARTESIAN_POINT ( 'NONE',  ( 97.79428472817266993, -42.74653246722733257, 142.7965776568629508 ) ) ;
#86172=VERTEX_POINT ( 'NONE', #87178 ) ;
#86174=ORIENTED_EDGE ( 'NONE', *, *, #78243, .F. ) ;
#86178=CONICAL_SURFACE ( 'NONE', #84776, 11.57110091390434192, 0.7853981633974471688 ) ;
#86180=ADVANCED_FACE ( 'NONE', ( #80370 ), #58555, .F. ) ;
#86181=DIRECTION ( 'NONE',  ( 1.000000000000000078E-15, -1.000000000000000000, 0.000000000000000000 ) ) ;
#86182=CARTESIAN_POINT ( 'NONE',  ( 111.9289591080100053, -27.50755150920414849, 59.68991099019693536 ) ) ;
#86183=DIRECTION ( 'NONE',  ( -0.4214249218767882055, -0.9068632946707806397, -4.214249218767890910E-16 ) ) ;
#86187=CARTESIAN_POINT ( 'NONE',  ( 97.55373691267104164, -39.00345059616621768, 56.51276813305494784 ) ) ;
#86189=CARTESIAN_POINT ( 'NONE',  ( 102.6926969729870507, -27.29023857175978662, 176.4213395616249898 ) ) ;
#86190=CARTESIAN_POINT ( 'NONE',  ( 165.9667039024459996, -26.71338133339301635, -5.074374724088000832 ) ) ;
#86191=DIRECTION ( 'NONE',  ( 1.000000000000000000, 3.999999999999999995E-14, 1.000000000000000078E-15 ) ) ;
#86192=ORIENTED_EDGE ( 'NONE', *, *, #51452, .F. ) ;
#86193=DIRECTION ( 'NONE',  ( 3.999999999999999995E-14, -1.000000000000000000, 4.100000000000000342E-29 ) ) ;
#86194=DIRECTION ( 'NONE',  ( 4.299999999999999979E-14, -1.000000000000000000, 4.400000000000000367E-29 ) ) ;
#86197=DIRECTION ( 'NONE',  ( -2.106816776397999944E-14, 1.000000000000000000, -2.206816776398000223E-29 ) ) ;
#86198=CARTESIAN_POINT ( 'NONE',  ( 97.05395071892901626, -41.52132310946490890, 216.6937205140059461 ) ) ;
#86200=CARTESIAN_POINT ( 'NONE',  ( 172.5664832912729878, -27.57844715994070484, 258.9256252759120116 ) ) ;
#86201=CARTESIAN_POINT ( 'NONE',  ( 115.0714481855697926, -30.01693675811307571, 265.3813395616251682 ) ) ;
#86202=CARTESIAN_POINT ( 'NONE',  ( 114.7393473568293700, -44.74971245420289279, 109.1718157521009687 ) ) ;
#86204=CARTESIAN_POINT ( 'NONE',  ( 57.56670390244718760, -42.82844715994040996, 173.2178068554150911 ) ) ;
#86207=ORIENTED_EDGE ( 'NONE', *, *, #67549, .F. ) ;
#86212=VERTEX_POINT ( 'NONE', #12211 ) ;
#86213=CIRCLE ( 'NONE', #60045, 7.499999999999992895 ) ;
#86214=EDGE_LOOP ( 'NONE', ( #54424, #73973, #49739, #70900, #14966, #29952, #17240, #5494 ) ) ;
#86215=DIRECTION ( 'NONE',  ( 0.7071067811865491270, -0.7071067811865459074, 7.071067811865492096E-16 ) ) ;
#86216=CARTESIAN_POINT ( 'NONE',  ( 116.5364499171840720, -42.42977282487416346, 274.3832443235299365 ) ) ;
#86217=DIRECTION ( 'NONE',  ( -0.08544974978095701279, -0.9963424814100680926, 0.000000000000000000 ) ) ;
#86220=CARTESIAN_POINT ( 'NONE',  ( 172.5667039024480687, -42.82844715993500273, 300.4678068554149490 ) ) ;
#86222=CARTESIAN_POINT ( 'NONE',  ( 87.31648329127401098, -36.72944715994105991, 14.92562527591095112 ) ) ;
#86223=CARTESIAN_POINT ( 'NONE',  ( 98.52747904795083400, -36.52563780154032003, 195.7295626852199462 ) ) ;
#86224=EDGE_LOOP ( 'NONE', ( #12774, #74600 ) ) ;
#86227=FACE_BOUND ( 'NONE', #9322, .T. ) ;
#86228=CARTESIAN_POINT ( 'NONE',  ( 108.3331741162412811, -46.73489075662012482, 182.6773131391069853 ) ) ;
#86229=CARTESIAN_POINT ( 'NONE',  ( 100.6696166679599713, -29.33055989933774299, 256.6441967044817147 ) ) ;
#86230=DIRECTION ( 'NONE',  ( -0.7071067811861110330, -0.7071067811869841124, 0.000000000000000000 ) ) ;
#86231=EDGE_CURVE ( 'NONE', #59341, #87723, #40799, .T. ) ;
#86232=PLANE ( 'NONE',  #62166 ) ;
#86234=CARTESIAN_POINT ( 'NONE',  ( 25.56670390244797275, -67.87844715994100397, 142.0928068554150059 ) ) ;
#86236=CARTESIAN_POINT ( 'NONE',  ( 104.0201293345620286, -27.19852536998958925, 56.32266916734289453 ) ) ;
#86237=EDGE_LOOP ( 'NONE', ( #71162, #32159, #17319, #64328, #24704, #58332 ) ) ;
#86239=CARTESIAN_POINT ( 'NONE',  ( 111.0677264286952521, -45.23305914580045339, 284.3463452106589102 ) ) ;
#86240=AXIS2_PLACEMENT_3D ( 'NONE', #40935, #13687, #47295 ) ;
#86243=CARTESIAN_POINT ( 'NONE',  ( 194.0371591254575492, -24.42818131005417115, 117.4678068554150627 ) ) ;
#86246=FACE_OUTER_BOUND ( 'NONE', #45872, .T. ) ;
#86247=CARTESIAN_POINT ( 'NONE',  ( 151.0371591254585155, -46.82818131005592477, 129.9678068554149775 ) ) ;
#86248=ORIENTED_EDGE ( 'NONE', *, *, #46823, .F. ) ;
#86249=CARTESIAN_POINT ( 'NONE',  ( 112.7599586733956727, -27.95389904326713904, 69.61848241876793963 ) ) ;
#86251=CARTESIAN_POINT ( 'NONE',  ( 114.1634876701351402, -42.35485373834646339, 47.72765792331495760 ) ) ;
#86252=CARTESIAN_POINT ( 'NONE',  ( 116.3228127852087113, -32.93589129790882453, 90.13562527591095375 ) ) ;
#86253=CARTESIAN_POINT ( 'NONE',  ( 116.3620231750148406, -38.09673052741934640, 70.15396425827796634 ) ) ;
#86254=CARTESIAN_POINT ( 'NONE',  ( 104.4075039567214134, -46.45791419004698497, 13.36474276782575465 ) ) ;
#86257=CARTESIAN_POINT ( 'NONE',  ( 115.7467025339723250, -43.60978142820201242, 44.30514908543492680 ) ) ;
#86258=LINE ( 'NONE', #17225, #62827 ) ;
#86259=ORIENTED_EDGE ( 'NONE', *, *, #3466, .F. ) ;
#86262=ORIENTED_EDGE ( 'NONE', *, *, #71175, .T. ) ;
#86263=CARTESIAN_POINT ( 'NONE',  ( 99.06808600115306263, -45.54042523694053557, 152.9899109901969894 ) ) ;
#86264=CARTESIAN_POINT ( 'NONE',  ( 78.98444042533783715, -21.25772566032899746, 1.807989669955657019 ) ) ;
#86265=AXIS2_PLACEMENT_3D ( 'NONE', #83204, #77731, #43179 ) ;
#86266=AXIS2_PLACEMENT_3D ( 'NONE', #2217, #84456, #64889 ) ;
#86268=ORIENTED_EDGE ( 'NONE', *, *, #18411, .F. ) ;
#86269=VERTEX_POINT ( 'NONE', #69416 ) ;
#86270=EDGE_CURVE ( 'NONE', #39062, #71292, #48048, .T. ) ;
#86272=AXIS2_PLACEMENT_3D ( 'NONE', #3663, #79538, #31359 ) ;
#86274=CARTESIAN_POINT ( 'NONE',  ( 114.9410966442422648, -29.98191058901448969, 229.4022919425779605 ) ) ;
#86275=CARTESIAN_POINT ( 'NONE',  ( 97.50743367704620823, -39.67470400402397246, 126.5637992372244156 ) ) ;
#86277=CARTESIAN_POINT ( 'NONE',  ( 104.4907123320104461, -46.86782655419724364, 43.37848241876896083 ) ) ;
#86278=CARTESIAN_POINT ( 'NONE',  ( 108.3330981890487550, -46.73490692371524347, 43.67726424760522264 ) ) ;
#86279=EDGE_LOOP ( 'NONE', ( #61328, #10491, #21080, #45693 ) ) ;
#86280=CARTESIAN_POINT ( 'NONE',  ( 114.7582354846073827, -30.31413633156125087, 170.3796143784777257 ) ) ;
#86281=CARTESIAN_POINT ( 'NONE',  ( 107.0664832912739399, -50.04691774669244353, 305.7008218191032256 ) ) ;
#86283=CARTESIAN_POINT ( 'NONE',  ( 107.0667039024479834, -36.72944715994099596, 239.5838068554170093 ) ) ;
#86284=EDGE_CURVE ( 'NONE', #2245, #79375, #62141, .T. ) ;
#86285=FACE_OUTER_BOUND ( 'NONE', #19898, .T. ) ;
#86286=CARTESIAN_POINT ( 'NONE',  ( 113.2071528006340628, -45.12711609280825087, 228.0784824187679760 ) ) ;
#86287=VECTOR ( 'NONE', #7533, 1000.000000000000000 ) ;
#86289=FACE_BOUND ( 'NONE', #26511, .T. ) ;
#86290=DIRECTION ( 'NONE',  ( 0.000000000000000000, 0.000000000000000000, -1.000000000000000000 ) ) ;
#86291=CARTESIAN_POINT ( 'NONE',  ( 98.63544605819593869, -40.03554478408833006, 246.0343245899819919 ) ) ;
#86293=CARTESIAN_POINT ( 'NONE',  ( 103.6060256796756960, -46.54035428658114171, 53.30705384733997221 ) ) ;
#86295=CARTESIAN_POINT ( 'NONE',  ( 107.9493508131109962, -25.66448314884807047, 115.0251490854349612 ) ) ;
#86297=PLANE ( 'NONE',  #4617 ) ;
#86300=LINE ( 'NONE', #58569, #56925 ) ;
#86301=CARTESIAN_POINT ( 'NONE',  ( 172.5664832912729878, -27.82844715994070484, 318.9256252759120116 ) ) ;
#86302=DIRECTION ( 'NONE',  ( 0.000000000000000000, 0.000000000000000000, -1.000000000000000000 ) ) ;
#86305=EDGE_CURVE ( 'NONE', #39081, #75765, #26280, .T. ) ;
#86309=CARTESIAN_POINT ( 'NONE',  ( 167.6524903400756159, -49.32844715993520879, 129.9678068554150059 ) ) ;
#86312=EDGE_CURVE ( 'NONE', #18344, #42921, #79421, .T. ) ;
#86314=CARTESIAN_POINT ( 'NONE',  ( 112.8139912305532704, -47.12176010715679553, 102.9784824187679817 ) ) ;
#86316=AXIS2_PLACEMENT_3D ( 'NONE', #85654, #9333, #42934 ) ;
#86317=ADVANCED_FACE ( 'NONE', ( #75336 ), #5399, .F. ) ;
#86318=DIRECTION ( 'NONE',  ( 0.8571673007021115565, -0.5150380749100554878, 7.521945815882500121E-16 ) ) ;
#86319=CARTESIAN_POINT ( 'NONE',  ( 134.0664832912740110, -41.22944715994101017, 4.925625275910997303 ) ) ;
#86322=DIRECTION ( 'NONE',  ( 1.000000000000000000, 4.163336342344333240E-14, 0.000000000000000000 ) ) ;
#86324=EDGE_CURVE ( 'NONE', #55190, #86673, #60794, .T. ) ;
#86326=CARTESIAN_POINT ( 'NONE',  ( 41.56648329127398966, -27.57844715994070484, 18.92562527591200094 ) ) ;
#86333=CARTESIAN_POINT ( 'NONE',  ( 115.7831077080300304, -41.80230944217467481, 34.40645861541539574 ) ) ;
#86334=CARTESIAN_POINT ( 'NONE',  ( 116.8431970675091662, -40.18699730018602168, 174.5680062282909546 ) ) ;
#86336=LINE ( 'NONE', #79083, #51567 ) ;
#86338=CIRCLE ( 'NONE', #45709, 10.00000000000000355 ) ;
#86340=CARTESIAN_POINT ( 'NONE',  ( 112.3272512417296554, -28.22507648531182056, 285.6356252759109680 ) ) ;
#86341=DIRECTION ( 'NONE',  ( -0.7071067811864613084, 0.7071067811866338371, -7.071067811864621391E-16 ) ) ;
#86342=CARTESIAN_POINT ( 'NONE',  ( 19.56648329127400032, 25.62155284005901379, 323.8756252759109202 ) ) ;
#86343=EDGE_CURVE ( 'NONE', #8253, #26639, #8343, .T. ) ;
#86344=FACE_OUTER_BOUND ( 'NONE', #16551, .T. ) ;
#86346=AXIS2_PLACEMENT_3D ( 'NONE', #9920, #58059, #78530 ) ;
#86347=ORIENTED_EDGE ( 'NONE', *, *, #66782, .T. ) ;
#86348=CARTESIAN_POINT ( 'NONE',  ( 112.1405701860857675, -28.01352448884034985, 29.65657790821143891 ) ) ;
#86353=CARTESIAN_POINT ( 'NONE',  ( 104.9381124493903457, -46.57529615900893560, 178.8387261630399507 ) ) ;
#86354=DIRECTION ( 'NONE',  ( 1.000000000000000078E-15, 1.000000000000000083E-30, -1.000000000000000000 ) ) ;
#86355=CARTESIAN_POINT ( 'NONE',  ( 109.2565852557048629, -45.31616550848684000, 44.20729759161095984 ) ) ;
#86357=AXIS2_PLACEMENT_3D ( 'NONE', #77828, #44171, #71470 ) ;
#86358=DIRECTION ( 'NONE',  ( 0.000000000000000000, 0.000000000000000000, -1.000000000000000000 ) ) ;
#86362=CARTESIAN_POINT ( 'NONE',  ( 66.21896343372186777, -72.55791859125355359, 542.9756252759101471 ) ) ;
#86363=EDGE_LOOP ( 'NONE', ( #2667, #88135, #3821, #682 ) ) ;
#86364=CARTESIAN_POINT ( 'NONE',  ( 97.24442698086039627, -40.26379795196659472, 266.6013395616254797 ) ) ;
#86365=FACE_OUTER_BOUND ( 'NONE', #85282, .T. ) ;
#86366=ORIENTED_EDGE ( 'NONE', *, *, #54565, .F. ) ;
#86367=CARTESIAN_POINT ( 'NONE',  ( 117.0718954855324228, -35.46248235742579880, 83.92729194248475721 ) ) ;
#86369=DIRECTION ( 'NONE',  ( -6.524622321627019585E-16, -4.013151879589939944E-16, -1.000000000000000000 ) ) ;
#86371=CARTESIAN_POINT ( 'NONE',  ( 97.99904154034810233, -44.43610744809739543, 222.8870538473399563 ) ) ;
#86374=CARTESIAN_POINT ( 'NONE',  ( 101.1169593292293598, -28.07258979649007102, 46.55562527591094835 ) ) ;
#86376=VECTOR ( 'NONE', #81309, 1000.000000000000000 ) ;
#86377=CARTESIAN_POINT ( 'NONE',  ( 105.8935610739654010, -47.12417332243212087, 282.4870538473394390 ) ) ;
#86378=ORIENTED_EDGE ( 'NONE', *, *, #32449, .F. ) ;
#86379=PLANE ( 'NONE',  #24539 ) ;
#86381=DIRECTION ( 'NONE',  ( 1.000000000000000078E-15, -1.000000000000000000, 0.000000000000000000 ) ) ;
#86382=CARTESIAN_POINT ( 'NONE',  ( 114.7830339860594364, -33.98399025413122843, 111.9166617981629486 ) ) ;
#86383=CARTESIAN_POINT ( 'NONE',  ( 101.9739164908862961, -45.89159533563675808, 183.1727681330539781 ) ) ;
#86388=ORIENTED_EDGE ( 'NONE', *, *, #29735, .T. ) ;
#86390=CIRCLE ( 'NONE', #19660, 0.5000000000000004441 ) ;
#86392=VECTOR ( 'NONE', #9262, 1000.000000000000000 ) ;
#86393=ORIENTED_EDGE ( 'NONE', *, *, #26423, .T. ) ;
#86395=DIRECTION ( 'NONE',  ( 0.000000000000000000, 0.000000000000000000, 1.000000000000000000 ) ) ;
#86396=CARTESIAN_POINT ( 'NONE',  ( 116.5791382887796175, -39.71887157413915759, 249.5838068554168672 ) ) ;
#86400=CARTESIAN_POINT ( 'NONE',  ( 97.80494057462277624, -40.50090208643202772, 42.63420498255158009 ) ) ;
#86401=CARTESIAN_POINT ( 'NONE',  ( 101.0184087763112757, -44.32493413285080663, 121.4638483995059630 ) ) ;
#86402=AXIS2_PLACEMENT_3D ( 'NONE', #45500, #79626, #9673 ) ;
#86403=CARTESIAN_POINT ( 'NONE',  ( 118.6196304926710212, -33.88663714441439367, 14.01848241876796308 ) ) ;
#86404=EDGE_CURVE ( 'NONE', #8253, #72194, #49844, .T. ) ;
#86406=DIRECTION ( 'NONE',  ( -4.299999999999999979E-14, 1.000000000000000000, -4.128053709984630540E-29 ) ) ;
#86407=ORIENTED_EDGE ( 'NONE', *, *, #74601, .T. ) ;
#86408=TOROIDAL_SURFACE ( 'NONE', #87827, 15.69999999999999929, 0.2999999999999999889 ) ;
#86410=ADVANCED_FACE ( 'NONE', ( #56664 ), #83952, .T. ) ;
#86411=CARTESIAN_POINT ( 'NONE',  ( 100.9542024942777090, -28.70739358321760903, 136.5939626800898736 ) ) ;
#86412=ORIENTED_EDGE ( 'NONE', *, *, #28165, .F. ) ;
#86414=CARTESIAN_POINT ( 'NONE',  ( 107.0667039024479834, -48.82844715994099971, 160.9178068554150229 ) ) ;
#86415=DIRECTION ( 'NONE',  ( 1.000000000000000078E-15, -1.000000000000000000, 0.000000000000000000 ) ) ;
#86417=EDGE_CURVE ( 'NONE', #60267, #18060, #21723, .T. ) ;
#86421=CARTESIAN_POINT ( 'NONE',  ( 110.9930863310008959, -46.38701419431276207, 282.8841967044824628 ) ) ;
#86422=CARTESIAN_POINT ( 'NONE',  ( 96.79082665085387305, -38.90864320302405588, 27.49276813305395706 ) ) ;
#86427=CARTESIAN_POINT ( 'NONE',  ( 107.0664832912739968, -0.7548456658612000547, 333.4006252759120343 ) ) ;
#86430=CARTESIAN_POINT ( 'NONE',  ( 131.4308125312103357, -37.51428458727104953, 6.911392308671625351 ) ) ;
#86431=DIRECTION ( 'NONE',  ( 4.299999999999999979E-14, -1.000000000000000000, 0.000000000000000000 ) ) ;
#86432=DIRECTION ( 'NONE',  ( 0.04216478779797398074, -0.9991106698809455455, 0.000000000000000000 ) ) ;
#86434=DIRECTION ( 'NONE',  ( 0.000000000000000000, 0.000000000000000000, 1.000000000000000000 ) ) ;
#86435=CARTESIAN_POINT ( 'NONE',  ( 117.4518178387850895, -35.59314106485747686, 278.9127681330539872 ) ) ;
#86436=CARTESIAN_POINT ( 'NONE',  ( 108.6750115452441747, -26.42919841034747819, 185.9527681330539792 ) ) ;
#86437=CARTESIAN_POINT ( 'NONE',  ( 103.4696982656617479, -25.41196563057017244, 51.32133956162493149 ) ) ;
#86438=PLANE ( 'NONE',  #55146 ) ;
#86439=CARTESIAN_POINT ( 'NONE',  ( 113.1782937727292335, -44.75186859144043439, 48.09395860939415002 ) ) ;
#86440=CARTESIAN_POINT ( 'NONE',  ( 81.48703104221002036, -34.36767655967705792, 1.942446731264919402 ) ) ;
#86442=AXIS2_PLACEMENT_3D ( 'NONE', #64506, #56776, #8655 ) ;
#86443=VECTOR ( 'NONE', #45231, 1000.000000000000000 ) ;
#86445=CARTESIAN_POINT ( 'NONE',  ( 116.3137647483393806, -32.94861263809731611, 185.1356252759109680 ) ) ;
#86447=CARTESIAN_POINT ( 'NONE',  ( 117.3137205126583211, -38.32096045344800928, 64.69181575210097890 ) ) ;
#86450=CARTESIAN_POINT ( 'NONE',  ( 117.0720146172106695, -35.46346990303036506, 49.92721339702549699 ) ) ;
#86451=CARTESIAN_POINT ( 'NONE',  ( 106.4848323041101850, -24.91801670280283787, 191.1156252759109861 ) ) ;
#86454=DIRECTION ( 'NONE',  ( -0.0001484127181978378183, 0.8660253910675245193, -0.5000000000000061062 ) ) ;
#86457=FACE_OUTER_BOUND ( 'NONE', #13765, .T. ) ;
#86458=CARTESIAN_POINT ( 'NONE',  ( 116.3247715116346939, -32.94624160847306626, 99.13562527591096796 ) ) ;
#86460=CARTESIAN_POINT ( 'NONE',  ( 116.5825849560772411, -39.12894369053753252, 123.6299109901969615 ) ) ;
#86462=VERTEX_POINT ( 'NONE', #35321 ) ;
#86464=CARTESIAN_POINT ( 'NONE',  ( 114.0372341014417543, -43.02906291645705039, 79.68539282970694160 ) ) ;
#86466=DIRECTION ( 'NONE',  ( -0.9254794337955620787, -0.3787978585227822492, 0.000000000000000000 ) ) ;
#86467=VECTOR ( 'NONE', #64564, 1000.000000000000000 ) ;
#86468=CARTESIAN_POINT ( 'NONE',  ( 98.59486473514179750, -43.92970144294050527, 222.8870538473389615 ) ) ;
#86470=VECTOR ( 'NONE', #69371, 1000.000000000000000 ) ;
#86471=DIRECTION ( 'NONE',  ( 0.7071067811865171526, 0.7071067811865779928, 7.071067811865162747E-16 ) ) ;
#86475=CARTESIAN_POINT ( 'NONE',  ( 21.03715912545744615, -47.82818131006197149, 129.9678068554150627 ) ) ;
#86476=CARTESIAN_POINT ( 'NONE',  ( 119.2637946045970097, -42.39761235918182791, 9.425625275910983092 ) ) ;
#86477=CARTESIAN_POINT ( 'NONE',  ( 109.8501361970267425, -26.70547878262030395, 174.8613395616249591 ) ) ;
#86478=ORIENTED_EDGE ( 'NONE', *, *, #68041, .T. ) ;
#86479=ORIENTED_EDGE ( 'NONE', *, *, #60209, .F. ) ;
#86480=CARTESIAN_POINT ( 'NONE',  ( 142.8821648370248170, -72.54478064608022692, 396.9756252759102040 ) ) ;
#86481=CARTESIAN_POINT ( 'NONE',  ( 97.06107108145566542, -37.99641183283564772, 152.4272919321757627 ) ) ;
#86483=CARTESIAN_POINT ( 'NONE',  ( 163.2449138993009115, -32.11662333284039761, 117.4678068554150485 ) ) ;
#86486=VECTOR ( 'NONE', #16181, 1000.000000000000000 ) ;
#86487=CARTESIAN_POINT ( 'NONE',  ( 95.90979441981569664, -32.73335165780250122, 176.0527681330539735 ) ) ;
#86488=CYLINDRICAL_SURFACE ( 'NONE', #29918, 2.117000000000007987 ) ;
#86490=ORIENTED_EDGE ( 'NONE', *, *, #68606, .F. ) ;
#86491=ORIENTED_EDGE ( 'NONE', *, *, #49672, .F. ) ;
#86492=CARTESIAN_POINT ( 'NONE',  ( 98.00184567357263177, -40.95613624034808709, 62.67415154770495889 ) ) ;
#86493=DIRECTION ( 'NONE',  ( -3.999999999999999995E-14, 1.000000000000000000, -4.100000000000000342E-29 ) ) ;
#86494=CARTESIAN_POINT ( 'NONE',  ( 137.8897065959776000, -5.906223855237799469, -5.074374724088998256 ) ) ;
#86495=CARTESIAN_POINT ( 'NONE',  ( 107.8719782714504873, -26.68843711164719323, 261.4444404487539941 ) ) ;
#86496=CARTESIAN_POINT ( 'NONE',  ( 188.5667039024479834, -67.87844715994100397, 137.2178068554150059 ) ) ;
#86498=CARTESIAN_POINT ( 'NONE',  ( 111.6189197817724335, -43.97823206604638813, 9.635625275910941312 ) ) ;
#86502=ORIENTED_EDGE ( 'NONE', *, *, #39245, .F. ) ;
#86505=ORIENTED_EDGE ( 'NONE', *, *, #63061, .F. ) ;
#86506=PLANE ( 'NONE',  #846 ) ;
#86508=ADVANCED_FACE ( 'NONE', ( #65714 ), #86627, .F. ) ;
#86509=CARTESIAN_POINT ( 'NONE',  ( 98.88061221520823096, -34.29066745521690507, 30.51813411379100671 ) ) ;
#86510=CARTESIAN_POINT ( 'NONE',  ( 96.11487883884397831, -35.06878432418778146, 221.1946728949589840 ) ) ;
#86512=CARTESIAN_POINT ( 'NONE',  ( 116.7751801856528147, -32.99181816784836485, 139.1184824187679396 ) ) ;
#86514=CARTESIAN_POINT ( 'NONE',  ( 106.2269110120561635, -47.75074920971118075, 263.5280062282920994 ) ) ;
#86515=CARTESIAN_POINT ( 'NONE',  ( 116.7952009943650324, -39.38756004681069101, 99.61577355868260497 ) ) ;
#86517=ORIENTED_EDGE ( 'NONE', *, *, #55286, .F. ) ;
#86518=ADVANCED_FACE ( 'NONE', ( #23522 ), #72147, .T. ) ;
#86519=ORIENTED_EDGE ( 'NONE', *, *, #79148, .T. ) ;
#86520=AXIS2_PLACEMENT_3D ( 'NONE', #10837, #43567, #38107 ) ;
#86521=AXIS2_PLACEMENT_3D ( 'NONE', #24132, #51803, #22803 ) ;
#86522=EDGE_CURVE ( 'NONE', #87708, #23215, #27201, .T. ) ;
#86524=CARTESIAN_POINT ( 'NONE',  ( 96.60014388984734524, -36.47963607454698831, 196.3070538473399438 ) ) ;
#86525=ORIENTED_EDGE ( 'NONE', *, *, #85707, .T. ) ;
#86527=CARTESIAN_POINT ( 'NONE',  ( 107.9182787209079919, -47.15539321873765743, 177.6413395616249886 ) ) ;
#86528=CARTESIAN_POINT ( 'NONE',  ( 109.7235518845913731, -27.00045683443076783, 264.8648104959339094 ) ) ;
#86535=CARTESIAN_POINT ( 'NONE',  ( 105.0259480979001552, -25.88970440745778134, 276.2365776568634033 ) ) ;
#86536=DIRECTION ( 'NONE',  ( 1.000000000000000000, -9.073094938289460781E-13, 0.000000000000000000 ) ) ;
#86538=ADVANCED_FACE ( 'NONE', ( #30761 ), #31640, .T. ) ;
#86539=FACE_OUTER_BOUND ( 'NONE', #20845, .T. ) ;
#86541=DIRECTION ( 'NONE',  ( -1.000000000000000000, 0.000000000000000000, 0.000000000000000000 ) ) ;
#86543=CARTESIAN_POINT ( 'NONE',  ( 105.3826699058209329, -44.58506565010721800, 195.5838068554169809 ) ) ;
#86544=ORIENTED_EDGE ( 'NONE', *, *, #34124, .T. ) ;
#86545=CARTESIAN_POINT ( 'NONE',  ( 164.9667039024459996, -26.71338133339301635, -5.074374724088000832 ) ) ;
#86546=CARTESIAN_POINT ( 'NONE',  ( 96.72113125116129595, -35.27340624960861959, 181.2156252759109805 ) ) ;
#86547=CARTESIAN_POINT ( 'NONE',  ( 117.9246037767874498, -41.47663949653230020, 54.49848241876792088 ) ) ;
#86548=CARTESIAN_POINT ( 'NONE',  ( 104.3994723555534989, -25.95519307775132134, 236.2575300378159682 ) ) ;
#86550=CARTESIAN_POINT ( 'NONE',  ( 51.23005224011598102, -33.89581943344511217, -5.074374724088000832 ) ) ;
#86551=AXIS2_PLACEMENT_3D ( 'NONE', #35536, #63257, #28739 ) ;
#86552=DIRECTION ( 'NONE',  ( 0.000000000000000000, 0.000000000000000000, -1.000000000000000000 ) ) ;
#86556=CYLINDRICAL_SURFACE ( 'NONE', #5052, 9.999999999999998224 ) ;
#86557=ORIENTED_EDGE ( 'NONE', *, *, #4777, .F. ) ;
#86559=CARTESIAN_POINT ( 'NONE',  ( 108.0930535991856800, -45.20896867503704897, 117.0952769709339663 ) ) ;
#86561=VERTEX_POINT ( 'NONE', #52502 ) ;
#86562=CARTESIAN_POINT ( 'NONE',  ( 117.8338636819850365, -39.12263375953639155, 99.64038718067195077 ) ) ;
#86563=CARTESIAN_POINT ( 'NONE',  ( 188.5667039024479834, -48.82844715994099971, 293.2178068554150627 ) ) ;
#86564=CARTESIAN_POINT ( 'NONE',  ( 78.42773927738372208, -16.51875925606581319, 7.791169830165904031 ) ) ;
#86565=LINE ( 'NONE', #86121, #57758 ) ;
#86566=ADVANCED_FACE ( 'NONE', ( #30322 ), #69285, .T. ) ;
#86567=CARTESIAN_POINT ( 'NONE',  ( 114.9268010244043978, -42.60560063232861694, 28.31562527591097123 ) ) ;
#86568=ORIENTED_EDGE ( 'NONE', *, *, #56129, .T. ) ;
#86572=CARTESIAN_POINT ( 'NONE',  ( 41.56648329127398966, -27.57844715994070484, 81.92562527591199739 ) ) ;
#86573=CARTESIAN_POINT ( 'NONE',  ( 142.8824340801164965, -74.11588153691423031, 540.9756252759101471 ) ) ;
#86574=CARTESIAN_POINT ( 'NONE',  ( 53.56670390244743629, -48.82844715994058049, 180.4678068554151196 ) ) ;
#86575=DIRECTION ( 'NONE',  ( 0.000000000000000000, 1.000000000000000000, 0.000000000000000000 ) ) ;
#86576=CARTESIAN_POINT ( 'NONE',  ( 97.70648437022691724, -40.25111366377705480, 52.61248643207778741 ) ) ;
#86579=CARTESIAN_POINT ( 'NONE',  ( 106.6078071710152244, -25.70885557892963647, 40.09753003781596448 ) ) ;
#86580=ORIENTED_EDGE ( 'NONE', *, *, #53663, .T. ) ;
#86581=VERTEX_POINT ( 'NONE', #59343 ) ;
#86586=CARTESIAN_POINT ( 'NONE',  ( 114.5787023362084085, -39.92261033116096058, 166.3252332267339852 ) ) ;
#86589=CIRCLE ( 'NONE', #85176, 3.299999999999997158 ) ;
#86590=VECTOR ( 'NONE', #37546, 1000.000000000000000 ) ;
#86591=CARTESIAN_POINT ( 'NONE',  ( 41.56648329127398966, -27.57844715994070484, 78.92562527591199739 ) ) ;
#86593=ORIENTED_EDGE ( 'NONE', *, *, #46720, .T. ) ;
#86596=VERTEX_POINT ( 'NONE', #2618 ) ;
#86598=CARTESIAN_POINT ( 'NONE',  ( 103.5819202103828474, -28.00394742224748157, 171.8225356868499603 ) ) ;
#86601=CARTESIAN_POINT ( 'NONE',  ( 112.1393456749956101, -28.01282280174694606, 119.6564586061650886 ) ) ;
#86602=CARTESIAN_POINT ( 'NONE',  ( 97.86672898778118679, -40.64958093551612706, 16.64701983854467571 ) ) ;
#86604=CLOSED_SHELL ( 'NONE', ( #81892, #4816, #25784, #75272, #40256, #84847, #11749, #62500, #46697, #25786, #61370, #8583, #478, #64772, #17083, #7435, #57868, #37236, #57048, #46383, #30114, #87787, #1926, #11895, #54160, #14841, #43945, #41060, #45385, #49246, #83736, #31865, #28047, #78454, #36254, #88597, #6959, #63760, #17620, #79155, #4159, #89903, #59094, #21048, #43720, #47817, #39935, #75225, #27864, #31838, #56080, #31767, #84482, #89199, #775, #56471, #73082, #89178, #30818, #60151, #82417, #53440, #38815, #88376, #3264, #12954, #18297, #81735, #36187, #10814, #34084, #32485, #34212, #47396, #15617, #13518, #34989, #59593, #88770, #52551, #32530, #54184, #27534, #8494, #55700, #79669, #63461, #7401, #34571, #10703, #58246, #63857, #47546, #50285, #45156, #82861, #13372, #47058, #58801, #54064, #2576, #46293, #44848, #58298, #40360, #85618, #33583, #2063, #42905, #74731, #45851, #44626, #85917, #67215, #1420, #75836, #86566, #16975, #40861, #38881, #56346, #13717, #14033, #62254, #84098, #37201, #56433, #74268, #11126, #88422, #9715, #30809, #57762, #44236, #85389, #48007, #69713, #77411, #36405, #62717, #68998, #40419, #36292, #68785, #72481, #80150, #1688, #12065, #43732, #63641, #83040, #14869, #80087, #80536, #61834, #56969, #16467, #61369, #34411, #76965, #33621, #59923, #60733, #67734, #50691, #31503, #89440, #14596, #73496, #56891, #17641, #48813, #37191, #45059, #21571, #7990, #57372, #36352, #51844, #65814, #30813, #77800, #31063, #76261, #266, #9093, #67506, #59861, #56658, #42986, #2546, #60249, #70198, #8928, #46376, #8797, #3238, #34123, #85418, #26962, #24173, #41758, #88882, #33275, #35327, #18838, #43842, #35235, #69496, #80353, #33193, #24784, #65806, #5380, #5578, #1290, #41254, #60203, #34920, #13915, #71352, #9159, #78946, #2465, #11509, #78544, #48732, #47100, #53035, #15242, #47038, #74633, #40333, #1109, #7757, #89719, #89088, #77244, #18087, #59412, #2967, #13580, #69108, #4768, #3761, #50498, #30909, #47953, #81599, #19168, #68456, #11290, #65261, #31621, #19340, #82195, #5962, #37425, #6935, #14611, #47515, #53069, #59109, #59992, #23236, #65685, #15230, #31940, #27582, #21022, #45472, #30064, #41511, #72762, #18712, #561, #69291, #87952, #42392, #81832, #693, #30257, #84052, #6409, #18429, #7666, #79120, #89448, #87009, #12602, #58163, #81149, #28241, #43548, #52123, #24249, #71673, #22838, #39552, #24330, #88571, #56442, #29554, #55012, #18540, #22144, #26601, #83135, #5728, #7148, #19308, #41559, #21912, #58764, #49658, #57882, #15290, #6955, #26115, #70466, #12208, #81912, #34092, #10805, #26019, #68879, #45764, #24986, #44632, #19853, #59284, #41365, #81676, #53139, #25352, #35587, #16249, #39724, #25319, #68554, #79070, #18162, #74630, #52615, #89905, #66587, #22074, #88449, #50605, #68758, #25501, #47500, #66316, #74860, #29350, #63912, #58925, #81663, #75509, #72441, #51342, #28558, #75317, #19169, #11864, #60337, #48148, #18612, #79238, #30915, #5109, #71514, #79102, #81223, #31526, #76276, #73694, #43320, #26410, #47899, #12911, #57472, #54433, #64367, #69698, #19860, #10857, #57459, #1041, #44771, #77200, #10295, #70596, #36873, #18194, #6724, #12755, #2335, #69110, #11039, #54852, #89829, #72399, #33065, #56643, #65676, #47096, #60650, #35195, #19240, #76795, #18076, #35218, #55453, #55983, #64156, #20276, #35349, #51326, #36363, #83055, #46199, #51533, #30315, #83750, #89108, #4871, #54992, #9902, #16264, #28584, #73750, #11646, #7746, #34645, #1446, #21382, #80811, #16483, #14854, #115, #64593, #62587, #76881, #52428, #78189, #80754, #41233, #11085, #33781, #47333, #25403, #22817, #72564, #86538, #88104, #16973, #56353, #49714, #32401, #34394, #32239, #23167, #6142, #28889, #41746, #31245, #46120, #63103, #85807, #48901, #31231, #85404, #88271, #60081, #29127, #26846, #35947, #8180, #62724, #78194, #81226, #81329, #14777, #36686, #35766, #85304, #85826, #82560, #57921, #29080, #12268, #73743, #21578, #20924, #6416, #71645, #38596, #79857, #36733, #75780, #52843, #89824, #3141, #10959, #38538, #5290, #50425, #74100, #7531, #7259, #47150, #48952, #7710, #392, #3292, #30866, #9343, #4267, #77948, #6911, #38039, #27954, #81506, #37471, #40336, #12077, #84691, #43376, #79345, #16913, #86508, #82082, #31032, #23374, #37928, #42345, #35933, #27750, #2842, #66845, #13133, #77701, #73462, #41693, #15395, #44509, #9131, #3546, #81414, #69859, #79011, #41266, #8911, #11527, #87812, #63246, #52823, #17318, #57978, #62413, #44064, #88665, #27935, #89272, #85520, #74294, #52013, #53991, #53366, #27945, #66815, #73728, #86001, #40218, #42798, #78806, #39100, #83642, #75457, #7036, #38809, #16569, #15966, #40041, #28550, #87239, #66715, #3344, #69053, #71193, #22051, #41172, #28677, #10022, #65701, #18874, #55398, #1255, #19004, #87518, #78004, #4200, #80423, #20472, #58006, #22752, #54106, #28696, #17747, #32767, #62731, #57565, #17595, #82980, #50496, #22660, #62246, #40927, #21435, #49772, #25025, #71249, #46611, #74715, #43988, #81731, #36519, #50445, #69160, #6306, #56370, #56765, #38801, #57591, #26406, #8806, #16982, #35017, #78730, #28540, #24798, #32367, #43259, #29011, #68730, #89287, #24864, #6230, #15864, #12841, #80240, #42651, #74483, #39765, #89173, #84206, #42419, #33382, #47912, #9077, #3349, #62199, #3819, #79646, #85243, #17135, #36858, #47956, #56832, #10025, #68025, #85458, #66322, #30701, #26014, #8314, #8737, #62605, #2840, #25708, #81946, #1310, #41863, #85900, #9569, #18630, #79974, #12372, #62030, #82283, #33177, #40898, #39663, #6127, #25795, #74694, #6938, #56959, #9198, #58526, #74834, #51505, #19113, #67023, #876, #66082, #24179, #21878, #37188, #27338, #47560, #32458, #54553, #50401, #66259, #24779, #23051, #44926, #35259, #84696, #22028, #36589, #27415, #27792, #76663, #60486, #53439, #19768, #72679, #51005, #43616, #4561, #57072, #43216, #59137, #66087, #87554, #84541, #79514, #48930, #76520, #51063, #56436, #75967, #32136, #43805, #33699, #10728, #35519, #21414, #23995, #78540, #5902, #17026, #42005, #58483, #75108, #64763, #71621, #54212, #35316, #54988, #54373, #33581, #24659, #20977, #28467, #86928, #33071, #85898, #62669, #32432, #15667, #5912, #41880, #60905, #23548, #56096, #8783, #28887, #65887, #45236, #67236, #22735, #7801, #69177, #5688, #27837, #84391, #73912, #62489, #17982, #69164, #59406, #20360, #51851, #44656, #10812, #62763, #66517, #25082, #69917, #8617, #22045, #45654, #26229, #18929, #52016, #6905, #30756, #65767, #47114, #83648, #67121, #3536, #89308, #49460, #49342, #25755, #59097, #8171, #35747, #7138, #73390, #25235, #49087, #73161, #60511, #39656, #42750, #38508, #57156, #79072, #9809, #5160, #81701, #88210, #72817, #83574, #49671, #84300, #88389, #19327, #61443, #63636, #63188, #54605, #66318, #897, #11238, #71828, #7719, #88260, #56328, #16491, #65532, #29198, #20883, #16183, #55397, #39608, #45012, #85368, #40850, #9735, #59234, #48347, #15245, #20068, #53238, #22616, #83646, #87979, #15792, #2654, #40163, #9471, #65866, #79529, #28598, #85240, #19783, #4285, #76584, #12617, #52425, #73077, #7567, #21108, #84608, #18715, #66913, #31334, #17899, #3771, #15289, #22900, #35494, #10310, #61463, #33592, #56707, #52352, #6024, #41360, #4763, #18488, #45678, #41380, #21774, #19285, #89684, #13575, #33685, #21497, #79796, #72581, #8541, #5331, #63800, #2735, #87988, #78907, #51748, #21705, #17818, #997, #22623, #21550, #55554, #74607, #16983, #71450, #33943, #13723, #56853, #35340, #8700, #56316, #22578, #18931, #88555, #41832, #84783, #22439, #15349, #36812, #56070, #76349, #38083, #47779, #28031, #54387, #4841, #67929, #71861, #15455, #65966, #26335, #60782, #15148, #85349, #46984, #64678, #86180, #42095, #50829, #52453, #28237, #4596, #3645, #13686, #47180, #63853, #25211, #13793, #89057, #16677, #28442, #44223, #4702, #42194, #48072, #82348, #81948, #39617, #77588, #48647, #34349, #12558, #39555, #49895, #21136, #67973, #1897, #16558, #86317, #47511, #70958, #40246, #22650, #43741, #14126, #70874, #40619, #464, #32460, #59476, #24290, #77749, #34533, #17274, #13171, #83883, #88227, #3537, #71155, #59754, #33298, #85003, #10418, #69681, #3154, #49892, #88946, #39290, #86938, #11885, #84572, #73264, #61876, #14662, #362, #35177, #37698, #17797, #82274, #42423, #36410, #39012, #28188, #1580, #62169, #58190, #21198, #45255, #28658, #23488, #86518, #29068, #78857, #54362, #30639, #4679, #48658, #52960, #81258, #38409, #18144, #19843, #25272, #68259, #18497, #41973, #40787, #2626, #43652, #20482, #1790, #23213, #26162, #71973, #69592, #88498, #79693, #7565, #30170, #37095, #62390, #8431, #51626, #23557, #32036, #84163, #42793, #89682, #58029, #43042, #58868, #67795, #11619, #11436, #19734, #44863, #59921, #48699, #24197, #10358, #59830, #60954, #67862, #36901, #44964, #6507, #38197, #14145, #45984, #6832, #84962, #10205, #35521, #44901, #80884, #9838, #68868, #86410, #72099, #29091, #20247, #88284, #88320, #75600, #75668, #48719, #68265, #27866, #83551, #55077, #35718, #83117, #60219, #81906, #38726, #50091, #77368, #21847, #6406, #20993, #78142, #83495, #29905, #52919, #62951, #73619, #63444, #81777, #64544, #5266, #33280, #72686, #87981, #19131, #23763, #19745, #40055, #70846, #37197, #71702, #11961, #79855, #63303, #74594, #22952, #52405, #82228, #81890, #32476, #22383, #11425, #31416, #27976, #54826, #41661, #1509, #64357, #42404, #8381, #84438, #55289, #21393, #58168, #38697, #2134, #26006, #19084, #88793, #70718, #11480, #37312, #42912, #10410 ) ) ;
#86607=EDGE_CURVE ( 'NONE', #64435, #34773, #78926, .T. ) ;
#86608=CARTESIAN_POINT ( 'NONE',  ( 103.2852591291245830, -43.96353797031052579, 210.0109475124489506 ) ) ;
#86609=CARTESIAN_POINT ( 'NONE',  ( 116.1429853652930149, -29.07104484579759784, 74.38419670448293175 ) ) ;
#86610=EDGE_CURVE ( 'NONE', #43140, #25043, #37383, .T. ) ;
#86611=CARTESIAN_POINT ( 'NONE',  ( 97.82856912889580769, -29.34641599088746133, 45.78991099019697231 ) ) ;
#86612=DIRECTION ( 'NONE',  ( 0.000000000000000000, 0.000000000000000000, -1.000000000000000000 ) ) ;
#86613=PLANE ( 'NONE',  #65534 ) ;
#86614=CARTESIAN_POINT ( 'NONE',  ( 107.7967913059082576, -25.29348262043577478, 322.9250063603933540 ) ) ;
#86616=CARTESIAN_POINT ( 'NONE',  ( 107.6529936739636639, -47.12767891731729009, 148.6213395616249784 ) ) ;
#86617=LINE ( 'NONE', #78918, #4490 ) ;
#86621=EDGE_CURVE ( 'NONE', #7066, #81364, #38448, .T. ) ;
#86623=CARTESIAN_POINT ( 'NONE',  ( 116.7802871385218282, -39.10473973501323286, 9.635625275910941312 ) ) ;
#86625=EDGE_LOOP ( 'NONE', ( #37072, #67428, #54683, #72609 ) ) ;
#86627=CYLINDRICAL_SURFACE ( 'NONE', #9765, 3.000000000000002665 ) ;
#86628=CARTESIAN_POINT ( 'NONE',  ( 41.56648329127399677, -18.82844715994099971, 261.0426252759119734 ) ) ;
#86629=CARTESIAN_POINT ( 'NONE',  ( 110.3541591212943445, -25.34385655279935534, 64.85276813305395649 ) ) ;
#86630=DIRECTION ( 'NONE',  ( 0.000000000000000000, 0.000000000000000000, 1.000000000000000000 ) ) ;
#86632=DIRECTION ( 'NONE',  ( 1.000000000000000000, 4.163336342344333240E-14, 0.000000000000000000 ) ) ;
#86633=CARTESIAN_POINT ( 'NONE',  ( 116.9446180447427821, -41.83184233209006209, 93.44705384733997278 ) ) ;
#86635=CARTESIAN_POINT ( 'NONE',  ( 114.9613132280021830, -29.02649429439055595, 190.4537205140059655 ) ) ;
#86636=CARTESIAN_POINT ( 'NONE',  ( 87.31648329127403940, -54.62589567669624557, -5.074374724089048883 ) ) ;
#86638=EDGE_CURVE ( 'NONE', #17228, #25149, #17031, .T. ) ;
#86639=ORIENTED_EDGE ( 'NONE', *, *, #33467, .T. ) ;
#86641=CARTESIAN_POINT ( 'NONE',  ( 41.56670390244718050, -42.82844715994109208, 180.4678068554150911 ) ) ;
#86642=CARTESIAN_POINT ( 'NONE',  ( 97.78523098987417939, -40.45222676762392666, 136.6304043995652080 ) ) ;
#86644=CARTESIAN_POINT ( 'NONE',  ( 117.9946794957619431, -34.78331989172042427, 198.9546728949589749 ) ) ;
#86645=EDGE_LOOP ( 'NONE', ( #21704, #30621, #9562, #63695 ) ) ;
#86647=CARTESIAN_POINT ( 'NONE',  ( 104.4050232528787774, -25.97761772452189888, 236.2575300378159682 ) ) ;
#86648=CARTESIAN_POINT ( 'NONE',  ( 97.94860405783340696, -41.87310908463563663, 132.7356252759109623 ) ) ;
#86649=CIRCLE ( 'NONE', #76449, 13.44999999999999396 ) ;
#86650=FACE_OUTER_BOUND ( 'NONE', #38000, .T. ) ;
#86651=CARTESIAN_POINT ( 'NONE',  ( 82.16007929299428270, -38.51483178663178819, 7.477467810852441055 ) ) ;
#86656=VECTOR ( 'NONE', #80339, 1000.000000000000000 ) ;
#86658=EDGE_LOOP ( 'NONE', ( #66572, #30057, #5699, #74524 ) ) ;
#86659=EDGE_LOOP ( 'NONE', ( #19956, #75645, #49969, #69537 ) ) ;
#86661=DIRECTION ( 'NONE',  ( 1.387778780781444492E-15, 0.000000000000000000, -1.000000000000000000 ) ) ;
#86662=CARTESIAN_POINT ( 'NONE',  ( 115.9068016902149907, -30.09448287295081670, 260.3508633711493871 ) ) ;
#86664=CARTESIAN_POINT ( 'NONE',  ( 132.3549177284975826, -34.56918551488095659, 2.099346190922506405 ) ) ;
#86665=CIRCLE ( 'NONE', #56161, 0.5000000000000031086 ) ;
#86667=CARTESIAN_POINT ( 'NONE',  ( 180.2121375201585636, -29.73316016638864312, 237.4678068554150059 ) ) ;
#86669=VECTOR ( 'NONE', #20815, 1000.000000000000000 ) ;
#86671=CARTESIAN_POINT ( 'NONE',  ( 111.9460571495898620, -43.77514521526708080, 202.4809912566479397 ) ) ;
#86673=VERTEX_POINT ( 'NONE', #58888 ) ;
#86674=ORIENTED_EDGE ( 'NONE', *, *, #67402, .F. ) ;
#86675=VECTOR ( 'NONE', #5588, 999.9999999999998863 ) ;
#86677=LINE ( 'NONE', #72153, #39034 ) ;
#86679=CARTESIAN_POINT ( 'NONE',  ( 188.5667039024479834, -65.37844715994100397, 257.2178068554150059 ) ) ;
#86680=CARTESIAN_POINT ( 'NONE',  ( 106.6757791475081376, -27.34201535943007499, 36.52920235351597711 ) ) ;
#86683=FACE_OUTER_BOUND ( 'NONE', #52179, .T. ) ;
#86684=VERTEX_POINT ( 'NONE', #44372 ) ;
#86685=CARTESIAN_POINT ( 'NONE',  ( 102.0651407823954884, -27.97162049558258445, 56.48994194808369684 ) ) ;
#86687=CARTESIAN_POINT ( 'NONE',  ( 172.5664832912740110, -18.82844715994099971, 261.0426252759119734 ) ) ;
#86688=CARTESIAN_POINT ( 'NONE',  ( 110.2473415405206083, -44.77823998140315354, 20.70618560768600247 ) ) ;
#86689=CIRCLE ( 'NONE', #30082, 0.5000000000000004441 ) ;
#86691=CARTESIAN_POINT ( 'NONE',  ( 31.90335556477745627, -33.89581943344423109, 193.9678068554150911 ) ) ;
#86693=DIRECTION ( 'NONE',  ( -0.7071067811865434649, -0.7071067811865516806, -7.071067811865440820E-16 ) ) ;
#86694=ORIENTED_EDGE ( 'NONE', *, *, #18270, .T. ) ;
#86695=LINE ( 'NONE', #67583, #36374 ) ;
#86698=CARTESIAN_POINT ( 'NONE',  ( 114.0222564360173720, -28.96386602133403798, 114.4956252759109816 ) ) ;
#86699=ORIENTED_EDGE ( 'NONE', *, *, #75883, .T. ) ;
#86700=CARTESIAN_POINT ( 'NONE',  ( 113.9308110932664704, -41.86102644448636312, 27.73813411379200033 ) ) ;
#86701=CARTESIAN_POINT ( 'NONE',  ( 100.5671124743891909, -44.38319045565923204, 88.01544400472339191 ) ) ;
#86702=CARTESIAN_POINT ( 'NONE',  ( 104.4236822747140678, -45.74566190472552307, 58.76920235351595778 ) ) ;
#86703=CARTESIAN_POINT ( 'NONE',  ( 46.03715912545425937, -48.62818131006086020, 313.9678068554150059 ) ) ;
#86705=CIRCLE ( 'NONE', #78027, 3.249999999999975131 ) ;
#86707=CARTESIAN_POINT ( 'NONE',  ( 109.6172575917244529, -25.13135243900233817, 25.90419670448196143 ) ) ;
#86708=DIRECTION ( 'NONE',  ( -1.000000000000000078E-15, 1.000000000000000000, 0.000000000000000000 ) ) ;
#86709=ORIENTED_EDGE ( 'NONE', *, *, #23831, .F. ) ;
#86710=LINE ( 'NONE', #52149, #8191 ) ;
#86712=ORIENTED_EDGE ( 'NONE', *, *, #62438, .T. ) ;
#86713=CIRCLE ( 'NONE', #25818, 3.250000000000002665 ) ;
#86716=VERTEX_POINT ( 'NONE', #68858 ) ;
#86719=AXIS2_PLACEMENT_3D ( 'NONE', #17539, #67017, #58848 ) ;
#86720=CARTESIAN_POINT ( 'NONE',  ( 97.31640351007376921, -35.61153895465465524, 206.2356252759109623 ) ) ;
#86721=LINE ( 'NONE', #18110, #66953 ) ;
#86724=CARTESIAN_POINT ( 'NONE',  ( 112.7416762643710229, -27.24439759747685486, 50.65943479972101215 ) ) ;
#86725=CARTESIAN_POINT ( 'NONE',  ( 97.81339943497903278, -40.52160296963607777, 42.63598487163911699 ) ) ;
#86726=VERTEX_POINT ( 'NONE', #20272 ) ;
#86727=CARTESIAN_POINT ( 'NONE',  ( 104.6139328008865448, -27.02899419139365733, 171.2735265809598957 ) ) ;
#86728=AXIS2_PLACEMENT_3D ( 'NONE', #51357, #79103, #65011 ) ;
#86729=AXIS2_PLACEMENT_3D ( 'NONE', #25965, #40026, #53630 ) ;
#86730=CYLINDRICAL_SURFACE ( 'NONE', #75265, 10.00000000000002487 ) ;
#86732=AXIS2_PLACEMENT_3D ( 'NONE', #84113, #28223, #20089 ) ;
#86733=DIRECTION ( 'NONE',  ( -1.000000000000000000, 0.000000000000000000, -1.000000000000000078E-15 ) ) ;
#86734=CARTESIAN_POINT ( 'NONE',  ( 115.7813355090083860, -41.80530075443426341, 114.4070842759231681 ) ) ;
#86735=CARTESIAN_POINT ( 'NONE',  ( 111.5990003564989905, -46.09347164638234062, 247.9356252759109509 ) ) ;
#86736=DIRECTION ( 'NONE',  ( 0.000000000000000000, 0.000000000000000000, 1.000000000000000000 ) ) ;
#86738=CARTESIAN_POINT ( 'NONE',  ( 79.00802158143601162, -39.26771232012922042, 1.799893082726616855 ) ) ;
#86739=CARTESIAN_POINT ( 'NONE',  ( 110.7878219579318255, -44.41760495294317934, 247.3581341137909533 ) ) ;
#86741=CARTESIAN_POINT ( 'NONE',  ( 98.87507392487052016, -43.19978241230791838, 87.85848241876792031 ) ) ;
#86743=CARTESIAN_POINT ( 'NONE',  ( 117.2525043769621362, -39.29786468180206782, 123.6299109901969615 ) ) ;
#86744=ORIENTED_EDGE ( 'NONE', *, *, #29172, .T. ) ;
#86745=DIRECTION ( 'NONE',  ( 0.000000000000000000, 1.000000000000000000, 0.000000000000000000 ) ) ;
#86749=LINE ( 'NONE', #49967, #17467 ) ;
#86751=LINE ( 'NONE', #24519, #54300 ) ;
#86752=ORIENTED_EDGE ( 'NONE', *, *, #70183, .F. ) ;
#86753=CARTESIAN_POINT ( 'NONE',  ( 97.78493946438445050, -40.45149985807169202, 51.62996325680755660 ) ) ;
#86754=CARTESIAN_POINT ( 'NONE',  ( 98.80516515778722919, -28.16326830255935221, 115.6870538473389587 ) ) ;
#86755=ORIENTED_EDGE ( 'NONE', *, *, #43007, .F. ) ;
#86757=CARTESIAN_POINT ( 'NONE',  ( 172.5664832912729878, -18.82844715994071194, 138.9256252759119832 ) ) ;
#86758=AXIS2_PLACEMENT_3D ( 'NONE', #63684, #77765, #14190 ) ;
#86759=AXIS2_PLACEMENT_3D ( 'NONE', #35129, #63298, #70113 ) ;
#86761=ORIENTED_EDGE ( 'NONE', *, *, #66138, .T. ) ;
#86762=CARTESIAN_POINT ( 'NONE',  ( 98.44037697964694189, -30.83566621160791144, 120.8499109901969604 ) ) ;
#86763=( NAMED_UNIT ( * ) PLANE_ANGLE_UNIT ( ) SI_UNIT ( $, .RADIAN. ) );
#86764=LINE ( 'NONE', #57246, #72436 ) ;
#86765=CARTESIAN_POINT ( 'NONE',  ( 131.0667039024480118, -64.87844715994098976, 231.5838068554150198 ) ) ;
#86768=ORIENTED_EDGE ( 'NONE', *, *, #9797, .T. ) ;
#86769=DIRECTION ( 'NONE',  ( -4.237773401492740281E-14, 1.000000000000000000, 0.000000000000000000 ) ) ;
#86770=FACE_OUTER_BOUND ( 'NONE', #26124, .T. ) ;
#86772=AXIS2_PLACEMENT_3D ( 'NONE', #16359, #64065, #1840 ) ;
#86773=CARTESIAN_POINT ( 'NONE',  ( 117.0099953369308281, -35.16094053785537454, 249.9518134712358801 ) ) ;
#86778=VECTOR ( 'NONE', #71350, 1000.000000000000000 ) ;
#86779=CARTESIAN_POINT ( 'NONE',  ( 116.8171228623376265, -34.15291831040233461, 35.03145861012588824 ) ) ;
#86780=EDGE_CURVE ( 'NONE', #51570, #74209, #87962, .T. ) ;
#86781=CARTESIAN_POINT ( 'NONE',  ( 96.69720940280909360, -36.59277893904148726, 152.3280062282909739 ) ) ;
#86782=DIRECTION ( 'NONE',  ( 4.299999999999999979E-14, -1.000000000000000000, 4.400000000000000367E-29 ) ) ;
#86784=AXIS2_PLACEMENT_3D ( 'NONE', #25680, #68374, #54249 ) ;
#86785=CARTESIAN_POINT ( 'NONE',  ( 106.9359508110862578, -26.91635713860572920, 56.08705384733897148 ) ) ;
#86786=CARTESIAN_POINT ( 'NONE',  ( 131.0667039024480118, -58.72944715994092491, 204.3338068554149913 ) ) ;
#86787=DIRECTION ( 'NONE',  ( 1.000000000000000078E-15, -1.000000000000000083E-30, -1.000000000000000000 ) ) ;
#86788=VECTOR ( 'NONE', #11608, 1000.000000000000000 ) ;
#86791=AXIS2_PLACEMENT_3D ( 'NONE', #73492, #38970, #66678 ) ;
#86792=CIRCLE ( 'NONE', #37521, 4.750000000000004441 ) ;
#86793=ORIENTED_EDGE ( 'NONE', *, *, #2813, .F. ) ;
#86795=CARTESIAN_POINT ( 'NONE',  ( 99.82831888057269509, -43.73513634207608902, 188.3701547344689686 ) ) ;
#86796=CYLINDRICAL_SURFACE ( 'NONE', #6694, 2.030000000001807248 ) ;
#86797=EDGE_CURVE ( 'NONE', #2880, #23552, #26179, .T. ) ;
#86799=CARTESIAN_POINT ( 'NONE',  ( 134.0664832912740110, -8.350947159940998787, 4.925625275911999168 ) ) ;
#86801=CARTESIAN_POINT ( 'NONE',  ( 42.66648329127298922, 12.92155284005730387, 355.9756252759109998 ) ) ;
#86803=DIRECTION ( 'NONE',  ( 9.351236661543306751E-17, -3.725950533538267725E-29, -1.000000000000000000 ) ) ;
#86804=CARTESIAN_POINT ( 'NONE',  ( 194.5664832912739826, -18.82844715994099971, 342.9256252759119548 ) ) ;
#86805=VERTEX_POINT ( 'NONE', #11662 ) ;
#86806=CARTESIAN_POINT ( 'NONE',  ( 117.4688788178166732, -35.86077403649778006, 253.8927681330538348 ) ) ;
#86807=CARTESIAN_POINT ( 'NONE',  ( 131.0667039024480118, -64.87844715994098976, 207.5838068554149913 ) ) ;
#86808=ORIENTED_EDGE ( 'NONE', *, *, #72891, .T. ) ;
#86809=EDGE_CURVE ( 'NONE', #783, #5130, #28692, .T. ) ;
#86810=EDGE_CURVE ( 'NONE', #26375, #20111, #68273, .T. ) ;
#86811=CARTESIAN_POINT ( 'NONE',  ( 31.78666935232898894, -29.62846900982320264, -5.074374724088000832 ) ) ;
#86812=CARTESIAN_POINT ( 'NONE',  ( 168.0371591254543944, -48.62818131005519717, 249.9678068554149775 ) ) ;
#86813=FACE_OUTER_BOUND ( 'NONE', #35709, .T. ) ;
#86817=CARTESIAN_POINT ( 'NONE',  ( 97.01638781908712872, -41.44040028630095662, 207.6632443235299661 ) ) ;
#86819=ORIENTED_EDGE ( 'NONE', *, *, #12726, .T. ) ;
#86820=CARTESIAN_POINT ( 'NONE',  ( 107.6091111025649809, -48.61711588689897212, 38.61276813305397582 ) ) ;
#86822=EDGE_CURVE ( 'NONE', #41258, #50227, #82953, .T. ) ;
#86823=ORIENTED_EDGE ( 'NONE', *, *, #15043, .T. ) ;
#86824=CARTESIAN_POINT ( 'NONE',  ( 81.77561474849751733, -16.57277681850257878, 2.101554741567897011 ) ) ;
#86828=CARTESIAN_POINT ( 'NONE',  ( 104.2492358271959603, -44.39057208814350020, 140.1138046553059837 ) ) ;
#86829=CARTESIAN_POINT ( 'NONE',  ( 98.82211989244140682, -29.33244250316893087, 231.7565776568629587 ) ) ;
#86833=ORIENTED_EDGE ( 'NONE', *, *, #9279, .T. ) ;
#86840=ORIENTED_EDGE ( 'NONE', *, *, #37798, .T. ) ;
#86841=DIRECTION ( 'NONE',  ( 0.9242245927363033076, 0.3818493186865918876, 0.000000000000000000 ) ) ;
#86843=CARTESIAN_POINT ( 'NONE',  ( 163.0664832912739826, -8.350947159940998787, 330.8831252759119934 ) ) ;
#86844=CARTESIAN_POINT ( 'NONE',  ( 97.73346832622766556, -34.05261013000342274, 140.5267055423629756 ) ) ;
#86845=CARTESIAN_POINT ( 'NONE',  ( 114.1203865811702087, -46.31439608500644312, 33.08133956162495792 ) ) ;
#86846=EDGE_CURVE ( 'NONE', #25435, #40826, #6967, .T. ) ;
#86850=CYLINDRICAL_SURFACE ( 'NONE', #70234, 2.500000000000002220 ) ;
#86851=EDGE_LOOP ( 'NONE', ( #56531, #86192, #5055, #59854, #46527, #12305 ) ) ;
#86855=ORIENTED_EDGE ( 'NONE', *, *, #44350, .T. ) ;
#86856=CARTESIAN_POINT ( 'NONE',  ( 130.5667039024479834, -40.02944715994100022, 239.5838068554162987 ) ) ;
#86857=EDGE_CURVE ( 'NONE', #51387, #70197, #27516, .T. ) ;
#86858=VECTOR ( 'NONE', #79392, 1000.000000000000000 ) ;
#86860=LINE ( 'NONE', #58671, #51856 ) ;
#86862=ORIENTED_EDGE ( 'NONE', *, *, #9012, .T. ) ;
#86863=CARTESIAN_POINT ( 'NONE',  ( 97.77253489752784787, -40.53345146323919579, 11.63562527591094309 ) ) ;
#86864=CARTESIAN_POINT ( 'NONE',  ( 99.03245663461365211, -44.38790092286875932, 32.92038718067297509 ) ) ;
#86867=DIRECTION ( 'NONE',  ( -4.299999999999999979E-14, 1.000000000000000000, -4.400000000000000367E-29 ) ) ;
#86868=DIRECTION ( 'NONE',  ( 0.000000000000000000, 0.000000000000000000, -1.000000000000000000 ) ) ;
#86869=FACE_BOUND ( 'NONE', #29071, .T. ) ;
#86870=AXIS2_PLACEMENT_3D ( 'NONE', #40797, #67613, #13994 ) ;
#86872=CARTESIAN_POINT ( 'NONE',  ( 104.4083387335005426, -46.45815895792671313, 162.3646280642559816 ) ) ;
#86874=CARTESIAN_POINT ( 'NONE',  ( 101.0739185617116078, -45.28721829360737416, 282.0899109901967563 ) ) ;
#86875=CARTESIAN_POINT ( 'NONE',  ( 115.5173804941753133, -29.60510038635626273, 220.3718157521019521 ) ) ;
#86876=CARTESIAN_POINT ( 'NONE',  ( 97.75304581901603740, -31.99688534799786765, 46.95276813305393659 ) ) ;
#86879=DIRECTION ( 'NONE',  ( -0.7071067811861110330, -0.7071067811869841124, 0.000000000000000000 ) ) ;
#86881=ORIENTED_EDGE ( 'NONE', *, *, #64888, .F. ) ;
#86882=DIRECTION ( 'NONE',  ( 0.000000000000000000, 0.000000000000000000, -1.000000000000000000 ) ) ;
#86883=VERTEX_POINT ( 'NONE', #54296 ) ;
#86884=CARTESIAN_POINT ( 'NONE',  ( 107.8187922529720026, -26.97765417004757538, 66.01562527591097762 ) ) ;
#86885=DIRECTION ( 'NONE',  ( 0.000000000000000000, 0.000000000000000000, 1.000000000000000000 ) ) ;
#86886=ORIENTED_EDGE ( 'NONE', *, *, #64091, .T. ) ;
#86888=CARTESIAN_POINT ( 'NONE',  ( 106.9407056411434951, -47.75886249174716625, 228.5794347997199907 ) ) ;
#86889=LINE ( 'NONE', #80986, #38218 ) ;
#86890=CARTESIAN_POINT ( 'NONE',  ( 172.5664832912728457, -27.82844715994070484, 261.9256252759120116 ) ) ;
#86891=DIRECTION ( 'NONE',  ( -1.000000000000000078E-15, 1.000000000000000083E-30, 1.000000000000000000 ) ) ;
#86895=CARTESIAN_POINT ( 'NONE',  ( 48.45959712127340424, -26.00627455219079209, 237.4678068554150059 ) ) ;
#86896=CARTESIAN_POINT ( 'NONE',  ( 97.98063455390165188, -41.72806076336413383, 176.7146728949589658 ) ) ;
#86897=VERTEX_POINT ( 'NONE', #18913 ) ;
#86898=ORIENTED_EDGE ( 'NONE', *, *, #11974, .T. ) ;
#86899=AXIS2_PLACEMENT_3D ( 'NONE', #35722, #56150, #49793 ) ;
#86900=CARTESIAN_POINT ( 'NONE',  ( 112.5403241924349942, -29.76056314593741803, 75.97872616303996551 ) ) ;
#86903=EDGE_CURVE ( 'NONE', #17773, #28811, #27047, .T. ) ;
#86904=CARTESIAN_POINT ( 'NONE',  ( 106.9482321581270270, -47.09886382165559127, 228.5794347997199907 ) ) ;
#86905=CARTESIAN_POINT ( 'NONE',  ( 130.3998166246059895, 12.92155284005730387, 358.9756252759109998 ) ) ;
#86907=DIRECTION ( 'NONE',  ( 0.000000000000000000, 0.000000000000000000, 1.000000000000000000 ) ) ;
#86908=EDGE_CURVE ( 'NONE', #49561, #24002, #88232, .T. ) ;
#86910=AXIS2_PLACEMENT_3D ( 'NONE', #30516, #33194, #75876 ) ;
#86915=CARTESIAN_POINT ( 'NONE',  ( 101.7806060443208480, -45.68981339355064364, 162.1527681330539679 ) ) ;
#86919=EDGE_CURVE ( 'NONE', #84782, #79006, #35219, .T. ) ;
#86920=CARTESIAN_POINT ( 'NONE',  ( 182.2420472961728137, -31.76306994223174840, 237.4678068554150059 ) ) ;
#86925=EDGE_CURVE ( 'NONE', #30791, #40389, #46104, .T. ) ;
#86926=EDGE_CURVE ( 'NONE', #82549, #73698, #30187, .T. ) ;
#86927=CARTESIAN_POINT ( 'NONE',  ( 156.5667039024485803, -48.82844715993568485, 137.2178068554149775 ) ) ;
#86928=ADVANCED_FACE ( 'NONE', ( #12333 ), #80486, .F. ) ;
#86929=CARTESIAN_POINT ( 'NONE',  ( 96.74292298454378169, -35.27647329413149890, 181.2156252759109805 ) ) ;
#86930=CARTESIAN_POINT ( 'NONE',  ( 20.03715912545732891, -24.95799193693189721, 300.4678068554150059 ) ) ;
#86931=ORIENTED_EDGE ( 'NONE', *, *, #58920, .T. ) ;
#86932=ORIENTED_EDGE ( 'NONE', *, *, #32043, .F. ) ;
#86933=ORIENTED_EDGE ( 'NONE', *, *, #36902, .T. ) ;
#86934=AXIS2_PLACEMENT_3D ( 'NONE', #42688, #62704, #40912 ) ;
#86937=CARTESIAN_POINT ( 'NONE',  ( 117.0720925080216404, -35.46411601386796519, 164.9271620083415826 ) ) ;
#86938=ADVANCED_FACE ( 'NONE', ( #31871 ), #45042, .T. ) ;
#86939=CARTESIAN_POINT ( 'NONE',  ( 112.7530619618799932, -30.23101651580132199, 285.9349166392303800 ) ) ;
#86940=CARTESIAN_POINT ( 'NONE',  ( 125.0664851986225443, -56.72944715994101728, -4.824374724089012467 ) ) ;
#86941=ORIENTED_EDGE ( 'NONE', *, *, #20811, .F. ) ;
#86944=DIRECTION ( 'NONE',  ( 1.000000000000000078E-15, 1.000000000000000083E-30, -1.000000000000000000 ) ) ;
#86945=ORIENTED_EDGE ( 'NONE', *, *, #11843, .F. ) ;
#86948=ORIENTED_EDGE ( 'NONE', *, *, #35363, .F. ) ;
#86950=CARTESIAN_POINT ( 'NONE',  ( 116.3215253324775773, -32.93968801256757217, 155.1356252759109680 ) ) ;
#86951=CARTESIAN_POINT ( 'NONE',  ( 110.6296508234850222, -44.49217663217273611, 27.34099125664796048 ) ) ;
#86952=CARTESIAN_POINT ( 'NONE',  ( 116.3700403630726612, -44.11035778917459993, 198.2927681330539542 ) ) ;
#86953=CARTESIAN_POINT ( 'NONE',  ( 117.4654710391980217, -40.40706546494233464, 178.5680062282919778 ) ) ;
#86955=CARTESIAN_POINT ( 'NONE',  ( 116.5364499171840720, -42.42977282487416346, 274.3832443235299365 ) ) ;
#86957=LINE ( 'NONE', #80596, #55473 ) ;
#86958=ORIENTED_EDGE ( 'NONE', *, *, #63125, .F. ) ;
#86959=EDGE_CURVE ( 'NONE', #70182, #59657, #5530, .T. ) ;
#86960=CIRCLE ( 'NONE', #68088, 2.500000000000002220 ) ;
#86961=ORIENTED_EDGE ( 'NONE', *, *, #9284, .F. ) ;
#86965=DIRECTION ( 'NONE',  ( 0.7071067811865614505, -0.7071067811865336949, 0.000000000000000000 ) ) ;
#86966=CARTESIAN_POINT ( 'NONE',  ( 118.0872578842352993, -35.40452791748241879, 238.9337205140059552 ) ) ;
#86967=VERTEX_POINT ( 'NONE', #79601 ) ;
#86968=CARTESIAN_POINT ( 'NONE',  ( 107.6530059321349455, -47.12789624220987150, 152.6213395616249500 ) ) ;
#86969=FACE_OUTER_BOUND ( 'NONE', #27996, .T. ) ;
#86970=FACE_OUTER_BOUND ( 'NONE', #14058, .T. ) ;
#86972=FACE_OUTER_BOUND ( 'NONE', #45259, .T. ) ;
#86973=DIRECTION ( 'NONE',  ( 5.512527431108029424E-15, -1.000000000000000000, 0.000000000000000000 ) ) ;
#86975=CARTESIAN_POINT ( 'NONE',  ( 116.5620552962770802, -42.34175257684895399, 279.4137205140061724 ) ) ;
#86976=DIRECTION ( 'NONE',  ( 0.000000000000000000, -1.000000000000000000, 0.000000000000000000 ) ) ;
#86977=CARTESIAN_POINT ( 'NONE',  ( 107.0664832912739968, -36.72944715994100306, -2.364374724089013391 ) ) ;
#86978=CARTESIAN_POINT ( 'NONE',  ( 193.0371591254583450, -47.82818131005411999, 249.9678068554149775 ) ) ;
#86979=VECTOR ( 'NONE', #21671, 1000.000000000000000 ) ;
#86982=CARTESIAN_POINT ( 'NONE',  ( 128.0667039024480118, -58.72944715994110254, 310.9178068554150514 ) ) ;
#86983=CARTESIAN_POINT ( 'NONE',  ( 109.5808203229745743, -44.32760431976820570, 195.5838068554168103 ) ) ;
#86984=EDGE_LOOP ( 'NONE', ( #27207, #94, #49912, #44994 ) ) ;
#86985=CARTESIAN_POINT ( 'NONE',  ( 151.0371591254573787, -24.95799193692592866, 249.9678068554149490 ) ) ;
#86986=CARTESIAN_POINT ( 'NONE',  ( 97.38146765292194118, -40.64695096355149673, 206.6327681330539860 ) ) ;
#86987=CARTESIAN_POINT ( 'NONE',  ( 113.8563929230154912, -44.64017497981368621, 104.1413395616249744 ) ) ;
#86988=CARTESIAN_POINT ( 'NONE',  ( 107.5118819425545951, -47.18863449879560079, 233.6099109901969655 ) ) ;
#86989=CARTESIAN_POINT ( 'NONE',  ( 128.0667039024480118, -58.72944715994112386, 198.9178068554149945 ) ) ;
#86990=AXIS2_PLACEMENT_3D ( 'NONE', #28854, #7064, #7510 ) ;
#86991=CARTESIAN_POINT ( 'NONE',  ( 107.0664832912739257, -52.72944715994095333, 311.3356252759109566 ) ) ;
#86993=CARTESIAN_POINT ( 'NONE',  ( 104.7197490991536881, -46.50674210198418734, 38.38840247910224690 ) ) ;
#86994=DIRECTION ( 'NONE',  ( 0.000000000000000000, 0.000000000000000000, 1.000000000000000000 ) ) ;
#86995=LINE ( 'NONE', #37501, #17551 ) ;
#86997=EDGE_LOOP ( 'NONE', ( #5305, #20138, #53287, #87444, #12198 ) ) ;
#86998=ORIENTED_EDGE ( 'NONE', *, *, #50973, .F. ) ;
#86999=CARTESIAN_POINT ( 'NONE',  ( 102.5065049712838601, -29.50707016595331567, 109.9467055423629631 ) ) ;
#87000=DIRECTION ( 'NONE',  ( 0.000000000000000000, 0.000000000000000000, 1.000000000000000000 ) ) ;
#87002=CARTESIAN_POINT ( 'NONE',  ( 98.87507392487052016, -43.19978241230791838, 87.85848241876792031 ) ) ;
#87003=LINE ( 'NONE', #81987, #43908 ) ;
#87004=CARTESIAN_POINT ( 'NONE',  ( 78.98444042533766662, -16.20116865955368723, 8.043260881866178380 ) ) ;
#87005=CARTESIAN_POINT ( 'NONE',  ( 109.7248659318316868, -27.00080518283870035, 175.8647919417129231 ) ) ;
#87006=CARTESIAN_POINT ( 'NONE',  ( 116.1300133678986413, -31.69047823903573047, 29.24229194257799236 ) ) ;
#87007=ORIENTED_EDGE ( 'NONE', *, *, #65264, .F. ) ;
#87009=ADVANCED_FACE ( 'NONE', ( #3725 ), #24181, .F. ) ;
#87010=ORIENTED_EDGE ( 'NONE', *, *, #61869, .F. ) ;
#87011=ORIENTED_EDGE ( 'NONE', *, *, #764, .F. ) ;
#87013=CARTESIAN_POINT ( 'NONE',  ( 102.9676436823274202, -46.25511244710193637, 133.2651490854339613 ) ) ;
#87015=CARTESIAN_POINT ( 'NONE',  ( 179.4595971212720258, -26.00627455219131789, -5.074374724088000832 ) ) ;
#87019=CYLINDRICAL_SURFACE ( 'NONE', #78120, 0.2500000000000002220 ) ;
#87020=VECTOR ( 'NONE', #39188, 1000.000000000000000 ) ;
#87021=EDGE_CURVE ( 'NONE', #20859, #58541, #65003, .T. ) ;
#87023=DIRECTION ( 'NONE',  ( 0.000000000000000000, 0.000000000000000000, -1.000000000000000000 ) ) ;
#87024=CARTESIAN_POINT ( 'NONE',  ( 112.7479404651554376, -27.97242311821432992, 69.61848241876793963 ) ) ;
#87025=ORIENTED_EDGE ( 'NONE', *, *, #82614, .F. ) ;
#87026=ORIENTED_EDGE ( 'NONE', *, *, #8109, .F. ) ;
#87030=FACE_OUTER_BOUND ( 'NONE', #58049, .T. ) ;
#87032=CARTESIAN_POINT ( 'NONE',  ( 108.5374814027631203, -28.67222352762033211, 162.7509475124489597 ) ) ;
#87034=EDGE_CURVE ( 'NONE', #51043, #29395, #4176, .T. ) ;
#87040=DIRECTION ( 'NONE',  ( 1.000000000000000078E-15, 1.000000000000000083E-30, -1.000000000000000000 ) ) ;
#87041=ORIENTED_EDGE ( 'NONE', *, *, #22329, .T. ) ;
#87045=EDGE_CURVE ( 'NONE', #87386, #4730, #33224, .T. ) ;
#87046=CARTESIAN_POINT ( 'NONE',  ( 115.2219208674478352, -40.19601845633869175, 164.9387261630399450 ) ) ;
#87047=CARTESIAN_POINT ( 'NONE',  ( 163.2569089553700223, -33.54226604285010893, -5.074374724088000832 ) ) ;
#87048=DIRECTION ( 'NONE',  ( 0.000000000000000000, 0.000000000000000000, 1.000000000000000000 ) ) ;
#87049=CARTESIAN_POINT ( 'NONE',  ( 188.5667039024479834, -62.87844715994099687, 293.2178068554150627 ) ) ;
#87053=VERTEX_POINT ( 'NONE', #31417 ) ;
#87054=AXIS2_PLACEMENT_3D ( 'NONE', #60124, #18810, #38353 ) ;
#87055=CARTESIAN_POINT ( 'NONE',  ( 99.07378970379950545, -35.07216769230775810, 213.9823760838769715 ) ) ;
#87056=CARTESIAN_POINT ( 'NONE',  ( 98.82253044624914651, -28.18127440817969287, 115.6870538473389587 ) ) ;
#87057=CARTESIAN_POINT ( 'NONE',  ( 110.5478855402368197, -46.57039549162855963, 37.84705384733994293 ) ) ;
#87059=LINE ( 'NONE', #3483, #61117 ) ;
#87060=DIRECTION ( 'NONE',  ( -1.175184669632759901E-16, 1.000000000000000000, 2.000000000000003705E-15 ) ) ;
#87061=CARTESIAN_POINT ( 'NONE',  ( 111.4172602844868862, -47.75239391268459599, 168.8756252759109486 ) ) ;
#87063=VERTEX_POINT ( 'NONE', #17801 ) ;
#87064=CARTESIAN_POINT ( 'NONE',  ( 194.5664832912739826, -18.82844715994099971, -5.074374724088000832 ) ) ;
#87065=ORIENTED_EDGE ( 'NONE', *, *, #85515, .F. ) ;
#87066=ORIENTED_EDGE ( 'NONE', *, *, #48121, .F. ) ;
#87067=CARTESIAN_POINT ( 'NONE',  ( 51.42025729302798709, -31.94127993907680718, -5.074374724088000832 ) ) ;
#87070=AXIS2_PLACEMENT_3D ( 'NONE', #30496, #50929, #57288 ) ;
#87071=ORIENTED_EDGE ( 'NONE', *, *, #72869, .T. ) ;
#87075=CARTESIAN_POINT ( 'NONE',  ( 97.62219055090962172, -32.23153194184447301, 75.97276813305397525 ) ) ;
#87077=CARTESIAN_POINT ( 'NONE',  ( 163.0664832912739826, 0.2215528400590083269, 333.4006252759110112 ) ) ;
#87079=CARTESIAN_POINT ( 'NONE',  ( 96.07333748454163924, -35.06730156692549372, 71.20705384733993526 ) ) ;
#87080=CARTESIAN_POINT ( 'NONE',  ( 72.31648329127401098, -45.62589376934781882, 14.92562527591093691 ) ) ;
#87081=CARTESIAN_POINT ( 'NONE',  ( 96.66614461754338095, -36.48121138304695421, 192.3070538473399438 ) ) ;
#87082=CARTESIAN_POINT ( 'NONE',  ( 109.7211212765799786, -26.99981308150919546, 59.86509729586450135 ) ) ;
#87084=VERTEX_POINT ( 'NONE', #32769 ) ;
#87088=DIRECTION ( 'NONE',  ( 1.000000000000000000, 4.299999999999999979E-14, 1.000000000000000078E-15 ) ) ;
#87089=CYLINDRICAL_SURFACE ( 'NONE', #50597, 13.16666666666670160 ) ;
#87090=EDGE_CURVE ( 'NONE', #20391, #42590, #75111, .T. ) ;
#87091=CARTESIAN_POINT ( 'NONE',  ( 104.1736071946568103, -26.63078081164005440, 225.2984824187679749 ) ) ;
#87094=CARTESIAN_POINT ( 'NONE',  ( 96.75463230179867935, -40.77307608890721013, 242.6118157521009664 ) ) ;
#87095=CARTESIAN_POINT ( 'NONE',  ( 102.5975616584704966, -46.88947854763195267, 128.2346728949589760 ) ) ;
#87096=DIRECTION ( 'NONE',  ( -1.000000000000000078E-15, 1.000000000000000083E-30, 1.000000000000000000 ) ) ;
#87097=CARTESIAN_POINT ( 'NONE',  ( 82.41057659162468951, -38.17027654744429555, 7.249284792661043753 ) ) ;
#87099=CARTESIAN_POINT ( 'NONE',  ( 117.0607235903083705, -38.08165846641635000, 264.7191046043259917 ) ) ;
#87102=EDGE_CURVE ( 'NONE', #89625, #45788, #32499, .T. ) ;
#87104=ORIENTED_EDGE ( 'NONE', *, *, #36572, .F. ) ;
#87106=EDGE_LOOP ( 'NONE', ( #30081, #22228, #88417, #10069, #36725 ) ) ;
#87108=CARTESIAN_POINT ( 'NONE',  ( 99.38154727845876835, -29.68499927947409489, 271.7356252759109907 ) ) ;
#87110=CARTESIAN_POINT ( 'NONE',  ( 132.0298243561165918, -34.87939921900699147, 2.327894594454071875 ) ) ;
#87113=CARTESIAN_POINT ( 'NONE',  ( 115.0894713190635628, -30.61837156327993625, 149.3442108353245317 ) ) ;
#87114=CARTESIAN_POINT ( 'NONE',  ( 112.8494018163660968, -30.44343212223953543, 198.9067055423629711 ) ) ;
#87116=ORIENTED_EDGE ( 'NONE', *, *, #68497, .F. ) ;
#87122=CARTESIAN_POINT ( 'NONE',  ( 101.4552306925257454, -43.61128330217721327, 8.464440448754938728 ) ) ;
#87123=EDGE_CURVE ( 'NONE', #77666, #78013, #40922, .T. ) ;
#87126=AXIS2_PLACEMENT_3D ( 'NONE', #68780, #40617, #25645 ) ;
#87127=EDGE_CURVE ( 'NONE', #47902, #85594, #50754, .T. ) ;
#87128=LINE ( 'NONE', #63661, #78210 ) ;
#87132=CARTESIAN_POINT ( 'NONE',  ( 103.3524915959513351, -27.44467182146633277, 56.37927426770519901 ) ) ;
#87133=EDGE_LOOP ( 'NONE', ( #11588, #47903 ) ) ;
#87134=AXIS2_PLACEMENT_3D ( 'NONE', #1795, #84924, #78559 ) ;
#87135=LINE ( 'NONE', #37195, #81524 ) ;
#87136=CARTESIAN_POINT ( 'NONE',  ( 98.54061126669880366, -38.21619907818254802, 44.26999513149598897 ) ) ;
#87137=CARTESIAN_POINT ( 'NONE',  ( 135.7892066358463410, -16.57943358559917613, 7.744922197151018040 ) ) ;
#87145=CARTESIAN_POINT ( 'NONE',  ( 116.9219696586192754, -33.22298239640010564, 114.0984824187679720 ) ) ;
#87147=CARTESIAN_POINT ( 'NONE',  ( 113.0365282982730264, -42.83802263516175657, 72.61527697093394806 ) ) ;
#87149=AXIS2_PLACEMENT_3D ( 'NONE', #50443, #58164, #2771 ) ;
#87152=CARTESIAN_POINT ( 'NONE',  ( 115.8905597133153549, -37.54428082998141747, 75.18444044875394638 ) ) ;
#87153=CARTESIAN_POINT ( 'NONE',  ( 136.8005346357622329, -19.07423037056981840, 3.076719480830218068 ) ) ;
#87156=CARTESIAN_POINT ( 'NONE',  ( 104.4853289249099362, -46.88901594738546663, 43.37848241876896083 ) ) ;
#87159=ORIENTED_EDGE ( 'NONE', *, *, #41175, .F. ) ;
#87160=DIRECTION ( 'NONE',  ( 0.0001713722456120069274, -0.9999999853157766072, 0.000000000000000000 ) ) ;
#87161=ORIENTED_EDGE ( 'NONE', *, *, #9405, .T. ) ;
#87162=DIRECTION ( 'NONE',  ( -1.000000000000000078E-15, 0.000000000000000000, 1.000000000000000000 ) ) ;
#87163=ORIENTED_EDGE ( 'NONE', *, *, #20529, .F. ) ;
#87165=AXIS2_PLACEMENT_3D ( 'NONE', #63477, #1264, #28970 ) ;
#87167=CARTESIAN_POINT ( 'NONE',  ( 96.81359797424451585, -35.17473563989037899, 221.1946728949589840 ) ) ;
#87168=CARTESIAN_POINT ( 'NONE',  ( 116.3201495438094923, -32.94088975182634726, 124.1356252759109537 ) ) ;
#87169=CARTESIAN_POINT ( 'NONE',  ( 115.0372574793866818, -42.90846260279429458, 189.3022919390266168 ) ) ;
#87170=CARTESIAN_POINT ( 'NONE',  ( 111.9288574835248511, -27.50774424443475397, 55.68991099019693536 ) ) ;
#87171=VECTOR ( 'NONE', #10327, 1000.000000000000000 ) ;
#87172=CARTESIAN_POINT ( 'NONE',  ( 194.0371591254573218, -24.42818131005407878, 237.4678068554150059 ) ) ;
#87173=ORIENTED_EDGE ( 'NONE', *, *, #4579, .T. ) ;
#87174=CYLINDRICAL_SURFACE ( 'NONE', #3627, 4.750000000000004441 ) ;
#87176=EDGE_CURVE ( 'NONE', #10820, #79159, #6858, .T. ) ;
#87178=CARTESIAN_POINT ( 'NONE',  ( 163.0664832912739826, 0.2215528400590083269, 330.1506252759110680 ) ) ;
#87180=CARTESIAN_POINT ( 'NONE',  ( 96.79764630557882299, -40.75620882907056597, 246.6118157521009664 ) ) ;
#87181=CYLINDRICAL_SURFACE ( 'NONE', #44330, 0.4999999999999982236 ) ;
#87184=CARTESIAN_POINT ( 'NONE',  ( 182.5667039024476139, -32.29483332967956954, 313.9678068554149490 ) ) ;
#87186=CARTESIAN_POINT ( 'NONE',  ( 110.1391594044062003, -28.21056625751448976, 249.2114674471249600 ) ) ;
#87187=DIRECTION ( 'NONE',  ( -0.9242245927363026414, -0.3818493186865932754, 0.000000000000000000 ) ) ;
#87188=CARTESIAN_POINT ( 'NONE',  ( 97.56228874418796693, -32.49873190831186776, 96.99276813305395706 ) ) ;
#87190=CARTESIAN_POINT ( 'NONE',  ( 109.2104764766756517, -26.48201038666214657, 139.9127681330539872 ) ) ;
#87191=ORIENTED_EDGE ( 'NONE', *, *, #11468, .T. ) ;
#87192=CARTESIAN_POINT ( 'NONE',  ( 132.8222787434353620, -21.18254450372675279, 7.982620440117798921 ) ) ;
#87193=ORIENTED_EDGE ( 'NONE', *, *, #83743, .F. ) ;
#87194=CARTESIAN_POINT ( 'NONE',  ( 41.56670390244718050, -42.82844715994109208, 180.4678068554150911 ) ) ;
#87196=DIRECTION ( 'NONE',  ( 0.000000000000000000, 1.000000000000000000, 0.000000000000000000 ) ) ;
#87200=CARTESIAN_POINT ( 'NONE',  ( 96.59500279541983048, -37.56604165528066375, 101.3899109901969524 ) ) ;
#87203=DIRECTION ( 'NONE',  ( -4.237773401492740281E-14, 1.000000000000000000, 0.000000000000000000 ) ) ;
#87205=DIRECTION ( 'NONE',  ( 2.056463827196271584E-15, -0.8571673007021100021, 0.5150380749100580413 ) ) ;
#87206=ORIENTED_EDGE ( 'NONE', *, *, #87356, .T. ) ;
#87207=VECTOR ( 'NONE', #36448, 1000.000000000000000 ) ;
#87209=CARTESIAN_POINT ( 'NONE',  ( 97.55101884832849635, -31.05922868340991627, 130.9108633711489915 ) ) ;
#87211=DIRECTION ( 'NONE',  ( -1.000000000000000000, 0.000000000000000000, 0.000000000000000000 ) ) ;
#87216=CARTESIAN_POINT ( 'NONE',  ( 116.3212776292296127, -32.94146857471318413, 287.6356252759109680 ) ) ;
#87217=DIRECTION ( 'NONE',  ( -4.237773401492740281E-14, 1.000000000000000000, 0.000000000000000000 ) ) ;
#87219=CARTESIAN_POINT ( 'NONE',  ( 72.06648329127399677, -9.729447159941065237, -4.824374724089063982 ) ) ;
#87221=CARTESIAN_POINT ( 'NONE',  ( 100.9544813764768634, -28.70716881530696796, 180.5939773098653234 ) ) ;
#87222=VECTOR ( 'NONE', #40263, 1000.000000000000000 ) ;
#87223=ORIENTED_EDGE ( 'NONE', *, *, #80199, .T. ) ;
#87224=CARTESIAN_POINT ( 'NONE',  ( 99.04406200859183684, -42.84125783440281054, 32.84395862863929239 ) ) ;
#87225=CARTESIAN_POINT ( 'NONE',  ( 104.0204373342842814, -47.42213563049708824, 213.3556252759109668 ) ) ;
#87227=VECTOR ( 'NONE', #83177, 1000.000000000000114 ) ;
#87229=ORIENTED_EDGE ( 'NONE', *, *, #86959, .T. ) ;
#87230=CARTESIAN_POINT ( 'NONE',  ( 115.0479362680065663, -42.38275094372907859, 49.33562527591095659 ) ) ;
#87232=CARTESIAN_POINT ( 'NONE',  ( 98.15100249062076898, -41.26166231382807581, 51.70074165506993324 ) ) ;
#87234=DIRECTION ( 'NONE',  ( 1.000000000000000000, 1.000000000000000078E-15, 1.000000000000000078E-15 ) ) ;
#87237=ORIENTED_EDGE ( 'NONE', *, *, #30816, .T. ) ;
#87239=ADVANCED_FACE ( 'NONE', ( #33671 ), #23214, .T. ) ;
#87240=ORIENTED_EDGE ( 'NONE', *, *, #54779, .F. ) ;
#87242=CARTESIAN_POINT ( 'NONE',  ( 115.4123442176498173, -41.04489973583525142, 239.8663452106589773 ) ) ;
#87243=CARTESIAN_POINT ( 'NONE',  ( 180.1667039024460166, -26.71338133339240528, 342.9256252759119548 ) ) ;
#87246=EDGE_CURVE ( 'NONE', #64215, #7655, #70441, .T. ) ;
#87247=CARTESIAN_POINT ( 'NONE',  ( 82.62351725430391980, -37.74149216370238946, 2.839569540204898157 ) ) ;
#87248=CIRCLE ( 'NONE', #48063, 0.5000000000000004441 ) ;
#87249=ORIENTED_EDGE ( 'NONE', *, *, #82217, .T. ) ;
#87252=EDGE_CURVE ( 'NONE', #89686, #68890, #30261, .T. ) ;
#87253=VERTEX_POINT ( 'NONE', #2301 ) ;
#87254=CARTESIAN_POINT ( 'NONE',  ( 102.3890460933095170, -47.58756240099349100, 287.2527681330536780 ) ) ;
#87255=DIRECTION ( 'NONE',  ( 0.000000000000000000, 1.000000000000000000, 0.000000000000000000 ) ) ;
#87259=FACE_OUTER_BOUND ( 'NONE', #16060, .T. ) ;
#87261=AXIS2_PLACEMENT_3D ( 'NONE', #69547, #26853, #68651 ) ;
#87262=CARTESIAN_POINT ( 'NONE',  ( 117.2699639542694001, -41.09825485984158178, 209.5165776568640013 ) ) ;
#87265=AXIS2_PLACEMENT_3D ( 'NONE', #22718, #50851, #50394 ) ;
#87266=CARTESIAN_POINT ( 'NONE',  ( 113.5330014162060195, -28.49676089798827405, 75.54705384733995288 ) ) ;
#87267=LINE ( 'NONE', #81801, #4785 ) ;
#87268=ORIENTED_EDGE ( 'NONE', *, *, #261, .F. ) ;
#87271=CARTESIAN_POINT ( 'NONE',  ( 81.14852608520887145, -16.20116861175210587, 1.807989644435677778 ) ) ;
#87273=FACE_OUTER_BOUND ( 'NONE', #79815, .T. ) ;
#87274=CARTESIAN_POINT ( 'NONE',  ( 115.0083044075158654, -38.73198694842640322, 121.4480903695919807 ) ) ;
#87275=CARTESIAN_POINT ( 'NONE',  ( 115.4773891788847067, -29.52237647247901009, 225.4022919425769658 ) ) ;
#87277=ORIENTED_EDGE ( 'NONE', *, *, #29104, .T. ) ;
#87278=DIRECTION ( 'NONE',  ( 1.000000000000000000, 4.299999999999999979E-14, 1.000000000000000078E-15 ) ) ;
#87281=ORIENTED_EDGE ( 'NONE', *, *, #49035, .T. ) ;
#87282=DIRECTION ( 'NONE',  ( 1.000000000000000078E-15, 0.000000000000000000, -1.000000000000000000 ) ) ;
#87283=ORIENTED_EDGE ( 'NONE', *, *, #18113, .F. ) ;
#87284=ORIENTED_EDGE ( 'NONE', *, *, #67745, .T. ) ;
#87285=CARTESIAN_POINT ( 'NONE',  ( 116.9610908827738882, -34.94244874878751972, 9.968958609244259250 ) ) ;
#87289=CARTESIAN_POINT ( 'NONE',  ( 98.34938918086412230, -31.65742736436922300, 25.90653489524752118 ) ) ;
#87290=CARTESIAN_POINT ( 'NONE',  ( 105.9636396274569137, -27.08297541922676643, 159.5895626852199598 ) ) ;
#87292=CARTESIAN_POINT ( 'NONE',  ( 110.2977701465690643, -46.68767980799292872, 12.82705384733995402 ) ) ;
#87295=VECTOR ( 'NONE', #88766, 1000.000000000000000 ) ;
#87296=ORIENTED_EDGE ( 'NONE', *, *, #82005, .F. ) ;
#87297=CARTESIAN_POINT ( 'NONE',  ( 62.03715912545824551, -47.82818131006021645, 300.4678068554150627 ) ) ;
#87298=ORIENTED_EDGE ( 'NONE', *, *, #48678, .T. ) ;
#87299=CARTESIAN_POINT ( 'NONE',  ( 97.20990489797566170, -38.46844655478637520, 167.4655669962249078 ) ) ;
#87303=VERTEX_POINT ( 'NONE', #29106 ) ;
#87305=CARTESIAN_POINT ( 'NONE',  ( 105.1595199372206793, -47.03071207059073799, 12.42991099019596923 ) ) ;
#87306=CARTESIAN_POINT ( 'NONE',  ( 112.9878179797879909, -28.09632633057573159, 40.59848241876795782 ) ) ;
#87310=DIRECTION ( 'NONE',  ( -0.7071067811865483499, -0.7071067811865466846, -7.071067811865491110E-16 ) ) ;
#87311=DIRECTION ( 'NONE',  ( 0.000000000000000000, 0.000000000000000000, 1.000000000000000000 ) ) ;
#87313=AXIS2_PLACEMENT_3D ( 'NONE', #38374, #44289, #2980 ) ;
#87317=CARTESIAN_POINT ( 'NONE',  ( 99.26081945853924537, -43.75962541195023903, 56.90991099019593236 ) ) ;
#87318=CARTESIAN_POINT ( 'NONE',  ( 97.09625178000921153, -41.50107833764869980, 212.6937205140059461 ) ) ;
#87319=CARTESIAN_POINT ( 'NONE',  ( 118.0115981831179113, -38.42934884787886318, 64.69181575210097890 ) ) ;
#87321=AXIS2_PLACEMENT_3D ( 'NONE', #81305, #53077, #80848 ) ;
#87324=DIRECTION ( 'NONE',  ( 0.000000000000000000, 0.000000000000000000, -1.000000000000000000 ) ) ;
#87325=AXIS2_PLACEMENT_3D ( 'NONE', #42461, #35661, #22063 ) ;
#87326=EDGE_CURVE ( 'NONE', #42151, #75837, #18635, .T. ) ;
#87328=DIRECTION ( 'NONE',  ( 0.000000000000000000, 0.000000000000000000, -1.000000000000000000 ) ) ;
#87329=ORIENTED_EDGE ( 'NONE', *, *, #12913, .T. ) ;
#87330=CARTESIAN_POINT ( 'NONE',  ( 109.5220866130624700, -46.80460460589462457, 83.75467289495797729 ) ) ;
#87332=ORIENTED_EDGE ( 'NONE', *, *, #70814, .F. ) ;
#87333=PLANE ( 'NONE',  #71748 ) ;
#87334=CARTESIAN_POINT ( 'NONE',  ( 100.6697571656888499, -44.93374849542860971, 228.0499109901969348 ) ) ;
#87337=CARTESIAN_POINT ( 'NONE',  ( 115.9432244607059204, -41.40609373283200512, 148.4407487842870808 ) ) ;
#87338=DIRECTION ( 'NONE',  ( 0.7071067811868666508, 0.7071067811862283836, 7.071067811868659373E-16 ) ) ;
#87339=EDGE_CURVE ( 'NONE', #7800, #42450, #27324, .T. ) ;
#87340=DIRECTION ( 'NONE',  ( 0.000000000000000000, 0.000000000000000000, -1.000000000000000000 ) ) ;
#87341=CIRCLE ( 'NONE', #19192, 4.749999999999976907 ) ;
#87342=CARTESIAN_POINT ( 'NONE',  ( 132.4277392773765030, -38.94013506380868961, 2.060080721660203729 ) ) ;
#87344=CARTESIAN_POINT ( 'NONE',  ( 116.6595528204499601, -34.65899032542078118, 183.9956252759109532 ) ) ;
#87346=ORIENTED_EDGE ( 'NONE', *, *, #57682, .T. ) ;
#87347=CARTESIAN_POINT ( 'NONE',  ( 112.4011824308993397, -28.99526907646757934, 86.03967854399191140 ) ) ;
#87348=VECTOR ( 'NONE', #5850, 1000.000000000000000 ) ;
#87350=CARTESIAN_POINT ( 'NONE',  ( 99.87094702832897042, -29.26198151734326203, 261.6746728949581779 ) ) ;
#87352=DIRECTION ( 'NONE',  ( 0.02150753337723862457, 0.0009076677972192722819, 0.9997682742251809973 ) ) ;
#87354=AXIS2_PLACEMENT_3D ( 'NONE', #45595, #30225, #10219 ) ;
#87356=EDGE_CURVE ( 'NONE', #17228, #2012, #64078, .T. ) ;
#87359=FACE_OUTER_BOUND ( 'NONE', #69398, .T. ) ;
#87360=EDGE_CURVE ( 'NONE', #15908, #50719, #9555, .T. ) ;
#87361=CARTESIAN_POINT ( 'NONE',  ( 102.8528367378537496, -46.24122135049443472, 177.2441967044819648 ) ) ;
#87362=ORIENTED_EDGE ( 'NONE', *, *, #85194, .T. ) ;
#87363=EDGE_LOOP ( 'NONE', ( #20667, #8252, #10135, #2464 ) ) ;
#87367=CARTESIAN_POINT ( 'NONE',  ( 107.0664832912748068, -36.72944715993923381, 14.92562527591097066 ) ) ;
#87371=CARTESIAN_POINT ( 'NONE',  ( 115.0397999656063917, -29.07403674218411638, 189.4232443235299570 ) ) ;
#87376=VECTOR ( 'NONE', #89455, 1000.000000000000000 ) ;
#87377=CARTESIAN_POINT ( 'NONE',  ( 105.3030533616251319, -46.61669885714199779, 63.43686953697783082 ) ) ;
#87380=CARTESIAN_POINT ( 'NONE',  ( 113.1369140564456615, -42.18651563507969371, 36.06237608387696980 ) ) ;
#87381=DIRECTION ( 'NONE',  ( 1.000000000000000078E-15, -1.000000000000000083E-30, -1.000000000000000000 ) ) ;
#87383=CARTESIAN_POINT ( 'NONE',  ( 90.44969454456405344, -20.11243780205715481, 218.8274735512160589 ) ) ;
#87384=CARTESIAN_POINT ( 'NONE',  ( 82.54568444100624447, -17.53793914063253112, 7.103892432653575284 ) ) ;
#87385=ORIENTED_EDGE ( 'NONE', *, *, #24481, .F. ) ;
#87386=VERTEX_POINT ( 'NONE', #30449 ) ;
#87390=ORIENTED_EDGE ( 'NONE', *, *, #7431, .F. ) ;
#87392=CARTESIAN_POINT ( 'NONE',  ( 115.5775591941339542, -37.73626844564258676, 53.15527697093397563 ) ) ;
#87393=CARTESIAN_POINT ( 'NONE',  ( 113.7648918053778715, -44.74678383396227588, 193.1299109901969757 ) ) ;
#87394=CARTESIAN_POINT ( 'NONE',  ( 112.4747680694540861, -26.21285726233885427, 169.6984824187679521 ) ) ;
#87395=DIRECTION ( 'NONE',  ( -1.000000000000000078E-15, 1.000000000000000000, 0.000000000000000000 ) ) ;
#87396=CARTESIAN_POINT ( 'NONE',  ( 112.6636929512762180, -45.52454417301038347, 259.0270538473393458 ) ) ;
#87397=CYLINDRICAL_SURFACE ( 'NONE', #15867, 1.499999999999987788 ) ;
#87403=CARTESIAN_POINT ( 'NONE',  ( 96.73248008985177648, -40.78176272772311250, 246.6118157521009664 ) ) ;
#87404=ORIENTED_EDGE ( 'NONE', *, *, #61530, .T. ) ;
#87405=EDGE_CURVE ( 'NONE', #54125, #13421, #17165, .T. ) ;
#87406=CARTESIAN_POINT ( 'NONE',  ( 107.2431713256043224, -47.18863871633809026, 212.5899109901969837 ) ) ;
#87407=CARTESIAN_POINT ( 'NONE',  ( 100.9540432848167200, -28.70751825032547799, 265.5939957159569076 ) ) ;
#87409=DIRECTION ( 'NONE',  ( 1.000000000000000078E-15, -1.000000000000000083E-30, -1.000000000000000000 ) ) ;
#87411=EDGE_CURVE ( 'NONE', #11589, #64922, #84980, .T. ) ;
#87412=FACE_OUTER_BOUND ( 'NONE', #9699, .T. ) ;
#87413=CARTESIAN_POINT ( 'NONE',  ( 107.0664832912750057, -36.72944715993903486, 9.125625275910969947 ) ) ;
#87414=CARTESIAN_POINT ( 'NONE',  ( 116.1206117333611019, -31.56300607074032882, 285.2384824187680579 ) ) ;
#87415=CARTESIAN_POINT ( 'NONE',  ( 163.0664832912739826, -0.2185775633789972805, 333.4006252759120343 ) ) ;
#87416=CYLINDRICAL_SURFACE ( 'NONE', #20695, 6.571100913904384555 ) ;
#87418=CARTESIAN_POINT ( 'NONE',  ( 149.4512091874902922, -60.54365471797113685, 361.9756252759100335 ) ) ;
#87419=EDGE_CURVE ( 'NONE', #42151, #45558, #43606, .T. ) ;
#87420=DIRECTION ( 'NONE',  ( -4.496403249731880833E-15, 0.000000000000000000, -1.000000000000000000 ) ) ;
#87423=CARTESIAN_POINT ( 'NONE',  ( 177.0664832912730162, 12.92155284005730387, 358.9756252759109998 ) ) ;
#87426=EDGE_CURVE ( 'NONE', #26963, #83074, #30004, .T. ) ;
#87427=DIRECTION ( 'NONE',  ( 0.000000000000000000, 0.000000000000000000, -1.000000000000000000 ) ) ;
#87428=CARTESIAN_POINT ( 'NONE',  ( 100.6239562591623695, -26.75308202300568539, 220.5327681330539633 ) ) ;
#87429=CARTESIAN_POINT ( 'NONE',  ( 104.1078173601787995, -46.72588569351386667, 103.3470538473389411 ) ) ;
#87430=CARTESIAN_POINT ( 'NONE',  ( 115.4227270478554317, -30.42340481720227885, 215.3413395616249773 ) ) ;
#87431=CARTESIAN_POINT ( 'NONE',  ( 83.06670390244796920, -61.87844715994100397, 207.5838068554149913 ) ) ;
#87432=LINE ( 'NONE', #39273, #70740 ) ;
#87433=CARTESIAN_POINT ( 'NONE',  ( 97.81169536214920868, -40.51742132101362870, 146.6356105553879274 ) ) ;
#87435=LINE ( 'NONE', #30680, #24931 ) ;
#87436=EDGE_CURVE ( 'NONE', #76720, #87084, #68239, .T. ) ;
#87437=CARTESIAN_POINT ( 'NONE',  ( 143.0664832912740110, -18.82844715994099971, 323.8756252759120002 ) ) ;
#87438=EDGE_CURVE ( 'NONE', #9653, #75243, #45823, .T. ) ;
#87440=ORIENTED_EDGE ( 'NONE', *, *, #89512, .T. ) ;
#87442=CARTESIAN_POINT ( 'NONE',  ( 113.1794296094924874, -30.05060732774411036, 153.8971817328389875 ) ) ;
#87444=ORIENTED_EDGE ( 'NONE', *, *, #22707, .T. ) ;
#87446=CARTESIAN_POINT ( 'NONE',  ( 117.2167691715782070, -39.01263929987993606, 144.6499109901969859 ) ) ;
#87447=EDGE_CURVE ( 'NONE', #13942, #87997, #17707, .T. ) ;
#87448=CARTESIAN_POINT ( 'NONE',  ( 107.0664832912739968, -36.72944715994100306, 287.6356252759109680 ) ) ;
#87452=DIRECTION ( 'NONE',  ( 0.000000000000000000, 0.000000000000000000, 1.000000000000000000 ) ) ;
#87453=CARTESIAN_POINT ( 'NONE',  ( 106.8551140066829817, -47.84553036069068099, 77.56133956162591403 ) ) ;
#87455=ORIENTED_EDGE ( 'NONE', *, *, #85194, .F. ) ;
#87456=VERTEX_POINT ( 'NONE', #73553 ) ;
#87458=CARTESIAN_POINT ( 'NONE',  ( 86.06670390244796920, -58.35344715994099829, 310.9178068554150514 ) ) ;
#87459=CARTESIAN_POINT ( 'NONE',  ( 105.8036208730406003, -25.68330614324009886, 156.1670538473389627 ) ) ;
#87460=DIRECTION ( 'NONE',  ( -4.299999999999999979E-14, 1.000000000000000000, -4.400000000000000367E-29 ) ) ;
#87461=CARTESIAN_POINT ( 'NONE',  ( 106.5462518941686909, -24.40236651281373526, 322.0356252759110021 ) ) ;
#87462=CARTESIAN_POINT ( 'NONE',  ( 188.5667039024479834, -65.37844715994100397, 168.3428068554150059 ) ) ;
#87463=LINE ( 'NONE', #53348, #45971 ) ;
#87466=CYLINDRICAL_SURFACE ( 'NONE', #11028, 0.2500000000000002220 ) ;
#87467=EDGE_CURVE ( 'NONE', #47446, #48239, #86792, .T. ) ;
#87468=CARTESIAN_POINT ( 'NONE',  ( 95.37363933861277587, -34.96150835630652409, 71.20705384733993526 ) ) ;
#87470=ORIENTED_EDGE ( 'NONE', *, *, #5919, .F. ) ;
#87475=FACE_OUTER_BOUND ( 'NONE', #19071, .T. ) ;
#87476=CARTESIAN_POINT ( 'NONE',  ( 100.0385306026334717, -40.93546354753772221, 159.5738046553059917 ) ) ;
#87478=AXIS2_PLACEMENT_3D ( 'NONE', #10529, #51839, #16908 ) ;
#87479=CIRCLE ( 'NONE', #62639, 2.500000000000002220 ) ;
#87480=CYLINDRICAL_SURFACE ( 'NONE', #82319, 3.000000000000002665 ) ;
#87481=VERTEX_POINT ( 'NONE', #87641 ) ;
#87482=ORIENTED_EDGE ( 'NONE', *, *, #70327, .F. ) ;
#87487=CARTESIAN_POINT ( 'NONE',  ( 98.59150690531237160, -40.78546747480537249, 213.1253928297069535 ) ) ;
#87488=DIRECTION ( 'NONE',  ( 4.299999999999999979E-14, -1.000000000000000000, 0.000000000000000000 ) ) ;
#87493=CIRCLE ( 'NONE', #55557, 2.517499999999998739 ) ;
#87496=CARTESIAN_POINT ( 'NONE',  ( 115.4521610479674081, -32.75750308622325946, 211.9966617981629611 ) ) ;
#87497=AXIS2_PLACEMENT_3D ( 'NONE', #43752, #51015, #79199 ) ;
#87498=CARTESIAN_POINT ( 'NONE',  ( 101.6994268497411724, -27.72483345503921370, 85.50419670448295051 ) ) ;
#87499=CARTESIAN_POINT ( 'NONE',  ( 104.7644060343265409, -46.87484541886973943, 72.39848241876795498 ) ) ;
#87500=CARTESIAN_POINT ( 'NONE',  ( 182.5667039024459939, -19.82844715994031048, 342.9256252759119548 ) ) ;
#87503=CARTESIAN_POINT ( 'NONE',  ( 97.95649862111255857, -30.46988169760521359, 161.8594347997199918 ) ) ;
#87504=DIRECTION ( 'NONE',  ( 0.000000000000000000, 0.000000000000000000, 1.000000000000000000 ) ) ;
#87505=ORIENTED_EDGE ( 'NONE', *, *, #384, .T. ) ;
#87507=ORIENTED_EDGE ( 'NONE', *, *, #44128, .T. ) ;
#87508=ORIENTED_EDGE ( 'NONE', *, *, #70053, .F. ) ;
#87509=PLANE ( 'NONE',  #44773 ) ;
#87512=AXIS2_PLACEMENT_3D ( 'NONE', #42850, #36061, #7011 ) ;
#87513=DIRECTION ( 'NONE',  ( 1.000000000000000078E-15, 1.000000000000000083E-30, -1.000000000000000000 ) ) ;
#87516=CARTESIAN_POINT ( 'NONE',  ( 96.79149040999978126, -38.49340627261485537, 91.46133956162493917 ) ) ;
#87517=CARTESIAN_POINT ( 'NONE',  ( 69.68306499799194853, -72.55732494038082336, 540.9756252759101471 ) ) ;
#87518=ADVANCED_FACE ( 'NONE', ( #30889 ), #18140, .F. ) ;
#87519=CARTESIAN_POINT ( 'NONE',  ( 168.3595971214164422, -48.62134037890297833, 180.4678068554150059 ) ) ;
#87520=DIRECTION ( 'NONE',  ( -9.073094938289460781E-13, -1.000000000000000000, 0.000000000000000000 ) ) ;
#87522=CARTESIAN_POINT ( 'NONE',  ( 112.1775644307544013, -28.39036538331624726, 94.63848241876893042 ) ) ;
#87524=CARTESIAN_POINT ( 'NONE',  ( 106.4848323041101850, -24.91801670280283787, 191.1156252759109861 ) ) ;
#87525=CARTESIAN_POINT ( 'NONE',  ( 98.34908471767082005, -31.65797358294662089, 60.90658434867807358 ) ) ;
#87526=CARTESIAN_POINT ( 'NONE',  ( 33.91903122894440514, -35.91149509761246605, 193.9678068554150911 ) ) ;
#87527=ORIENTED_EDGE ( 'NONE', *, *, #49837, .T. ) ;
#87528=CYLINDRICAL_SURFACE ( 'NONE', #19396, 0.4999999999999982236 ) ;
#87531=CARTESIAN_POINT ( 'NONE',  ( 107.0667039024482818, -36.72944715994102438, 249.5838068554170093 ) ) ;
#87533=DIRECTION ( 'NONE',  ( 0.9999999853157766072, 0.0001713722456134502174, 0.000000000000000000 ) ) ;
#87534=CARTESIAN_POINT ( 'NONE',  ( 98.80440911621268185, -29.31655204712020080, 235.7565776568629872 ) ) ;
#87535=ORIENTED_EDGE ( 'NONE', *, *, #11444, .F. ) ;
#87537=CARTESIAN_POINT ( 'NONE',  ( 116.5562423158612972, -42.44168660689859962, 274.3832443235299365 ) ) ;
#87538=CARTESIAN_POINT ( 'NONE',  ( 102.2928874563330055, -26.70895414482565045, 136.4422919425779526 ) ) ;
#87539=PLANE ( 'NONE',  #2683 ) ;
#87540=CARTESIAN_POINT ( 'NONE',  ( 82.77657790094494317, -37.19711456031350849, 6.808568500764617504 ) ) ;
#87542=CYLINDRICAL_SURFACE ( 'NONE', #88753, 2.500000000000002220 ) ;
#87543=ORIENTED_EDGE ( 'NONE', *, *, #67334, .F. ) ;
#87546=VECTOR ( 'NONE', #27288, 999.9999999999998863 ) ;
#87548=ORIENTED_EDGE ( 'NONE', *, *, #43835, .F. ) ;
#87550=ORIENTED_EDGE ( 'NONE', *, *, #67396, .T. ) ;
#87552=CARTESIAN_POINT ( 'NONE',  ( 106.6078071710152244, -25.70885557892973949, 36.09753003781596448 ) ) ;
#87554=ADVANCED_FACE ( 'NONE', ( #13134 ), #41701, .T. ) ;
#87555=DIRECTION ( 'NONE',  ( 0.000000000000000000, 0.000000000000000000, 1.000000000000000000 ) ) ;
#87556=DIRECTION ( 'NONE',  ( 1.027984282060330356E-15, 1.000000000000000000, 0.000000000000000000 ) ) ;
#87557=CARTESIAN_POINT ( 'NONE',  ( 107.2162147037312678, -27.02129552338790575, 229.4867055423629836 ) ) ;
#87559=EDGE_CURVE ( 'NONE', #44745, #82826, #73522, .T. ) ;
#87560=ORIENTED_EDGE ( 'NONE', *, *, #55902, .T. ) ;
#87561=VERTEX_POINT ( 'NONE', #60813 ) ;
#87562=AXIS2_PLACEMENT_3D ( 'NONE', #24571, #88598, #52239 ) ;
#87563=DIRECTION ( 'NONE',  ( -0.7071067811866279529, 0.7071067811864671926, -7.071067811865978232E-16 ) ) ;
#87564=CIRCLE ( 'NONE', #51286, 0.9999999999999731326 ) ;
#87565=CARTESIAN_POINT ( 'NONE',  ( 165.2725846195388328, -35.55794170701241796, 237.4678068554150059 ) ) ;
#87566=DIRECTION ( 'NONE',  ( -4.237773401492740281E-14, 1.000000000000000000, 0.000000000000000000 ) ) ;
#87567=CARTESIAN_POINT ( 'NONE',  ( 112.0788320361856307, -29.42159941445254390, 41.03015473446897232 ) ) ;
#87569=VECTOR ( 'NONE', #86341, 999.9999999999998863 ) ;
#87570=LINE ( 'NONE', #3550, #79628 ) ;
#87571=CARTESIAN_POINT ( 'NONE',  ( 97.78144721833423603, -39.80378292816726571, 241.5813395616259811 ) ) ;
#87572=CARTESIAN_POINT ( 'NONE',  ( 34.96670390244647564, -26.71338133339322951, 193.9678068554150911 ) ) ;
#87573=EDGE_LOOP ( 'NONE', ( #24364, #30297, #11653, #73117 ) ) ;
#87574=EDGE_CURVE ( 'NONE', #41295, #55881, #2701, .T. ) ;
#87575=DIRECTION ( 'NONE',  ( 0.7071067811866377228, -0.7071067811864573116, 0.000000000000000000 ) ) ;
#87577=FACE_OUTER_BOUND ( 'NONE', #35889, .T. ) ;
#87578=CARTESIAN_POINT ( 'NONE',  ( 107.4895849179006575, -45.99858499349326735, 40.43094751244896656 ) ) ;
#87580=CARTESIAN_POINT ( 'NONE',  ( 135.6073602527844457, -16.45223222829654475, 7.843813999037777762 ) ) ;
#87581=DIRECTION ( 'NONE',  ( 0.000000000000000000, 0.000000000000000000, -1.000000000000000000 ) ) ;
#87584=CARTESIAN_POINT ( 'NONE',  ( 97.81168895331838087, -40.51742574516882200, 287.6356252759109680 ) ) ;
#87587=CARTESIAN_POINT ( 'NONE',  ( 96.63902489370863691, -37.56252461247890295, 101.3899109901969524 ) ) ;
#87589=CARTESIAN_POINT ( 'NONE',  ( 110.1208792074641991, -44.70608788829420632, 62.28956268521896078 ) ) ;
#87590=LINE ( 'NONE', #67137, #40198 ) ;
#87591=CARTESIAN_POINT ( 'NONE',  ( 99.03873739112161445, -32.90617299384241790, 72.40444044875393104 ) ) ;
#87595=CARTESIAN_POINT ( 'NONE',  ( 97.33132060198839497, -32.84282867815538509, 37.02419670448292521 ) ) ;
#87596=CARTESIAN_POINT ( 'NONE',  ( 116.3214902495786873, -32.94210931476069248, 180.1356252759109680 ) ) ;
#87599=CARTESIAN_POINT ( 'NONE',  ( 116.3135889066590636, -32.94480564983713577, 259.1356252759109680 ) ) ;
#87602=VECTOR ( 'NONE', #55075, 1000.000000000000000 ) ;
#87604=VERTEX_POINT ( 'NONE', #48500 ) ;
#87606=ORIENTED_EDGE ( 'NONE', *, *, #19893, .F. ) ;
#87607=CARTESIAN_POINT ( 'NONE',  ( 112.0813997088635858, -45.80630777137071874, 252.9661014663878689 ) ) ;
#87608=CARTESIAN_POINT ( 'NONE',  ( 97.26831979079280188, -34.56112429623405546, 126.1522026196660278 ) ) ;
#87609=CARTESIAN_POINT ( 'NONE',  ( 104.4081005686254571, -46.45808911557011101, 188.3647919350316897 ) ) ;
#87610=CARTESIAN_POINT ( 'NONE',  ( 110.3540904097210387, -25.34409450869410563, 60.85276813305395649 ) ) ;
#87611=DIRECTION ( 'NONE',  ( 1.000000000000000078E-15, -1.000000000000000083E-30, -1.000000000000000000 ) ) ;
#87612=ORIENTED_EDGE ( 'NONE', *, *, #35202, .T. ) ;
#87613=CARTESIAN_POINT ( 'NONE',  ( 112.1394879536045011, -28.01289599002803499, 114.6579011162244939 ) ) ;
#87614=DIRECTION ( 'NONE',  ( 0.000000000000000000, -1.000000000000000000, 0.000000000000000000 ) ) ;
#87615=ORIENTED_EDGE ( 'NONE', *, *, #23387, .F. ) ;
#87619=DIRECTION ( 'NONE',  ( 0.000000000000000000, 1.000000000000000000, 0.000000000000000000 ) ) ;
#87620=CARTESIAN_POINT ( 'NONE',  ( 100.6697571656888073, -44.93374849542868787, 232.0499109901969632 ) ) ;
#87621=DIRECTION ( 'NONE',  ( 0.000000000000000000, 0.000000000000000000, -1.000000000000000000 ) ) ;
#87622=AXIS2_PLACEMENT_3D ( 'NONE', #22181, #78494, #29885 ) ;
#87623=EDGE_CURVE ( 'NONE', #9653, #44627, #88984, .T. ) ;
#87624=DIRECTION ( 'NONE',  ( 0.000000000000000000, 0.000000000000000000, -1.000000000000000000 ) ) ;
#87625=CARTESIAN_POINT ( 'NONE',  ( 77.71552635664728825, -38.16021090637489976, 2.608895778946703992 ) ) ;
#87627=CARTESIAN_POINT ( 'NONE',  ( 98.20387719113243463, -34.86749027545791080, 260.5962293518865636 ) ) ;
#87629=CARTESIAN_POINT ( 'NONE',  ( 96.11054930851091171, -38.00668368623056637, 82.43086337114895912 ) ) ;
#87631=CARTESIAN_POINT ( 'NONE',  ( 114.8040440383551157, -44.68828107661028781, 118.2022919425779719 ) ) ;
#87632=VERTEX_POINT ( 'NONE', #20398 ) ;
#87633=CARTESIAN_POINT ( 'NONE',  ( 133.6896269580626040, -21.47945062089170776, 8.225625248534988998 ) ) ;
#87636=CIRCLE ( 'NONE', #89127, 2.517500000000005844 ) ;
#87637=EDGE_CURVE ( 'NONE', #83459, #54780, #48068, .T. ) ;
#87638=FACE_OUTER_BOUND ( 'NONE', #87820, .T. ) ;
#87639=LINE ( 'NONE', #53067, #83331 ) ;
#87640=ORIENTED_EDGE ( 'NONE', *, *, #27538, .T. ) ;
#87641=CARTESIAN_POINT ( 'NONE',  ( 42.66648329127298922, 12.92155284005730387, 361.9756252759109998 ) ) ;
#87642=EDGE_CURVE ( 'NONE', #81179, #26477, #88546, .T. ) ;
#87643=CARTESIAN_POINT ( 'NONE',  ( 95.98894329157613470, -41.07880401750329469, 96.62419670448197451 ) ) ;
#87645=LINE ( 'NONE', #38583, #79854 ) ;
#87646=DIRECTION ( 'NONE',  ( -0.000000000000000000, -0.000000000000000000, -1.000000000000000000 ) ) ;
#87647=DIRECTION ( 'NONE',  ( 0.000000000000000000, 1.000000000000000000, 0.000000000000000000 ) ) ;
#87648=CARTESIAN_POINT ( 'NONE',  ( 97.81170495107971874, -40.51745053935989915, 26.63526479160227112 ) ) ;
#87649=VERTEX_POINT ( 'NONE', #53978 ) ;
#87650=EDGE_CURVE ( 'NONE', #85451, #67349, #35089, .T. ) ;
#87651=CARTESIAN_POINT ( 'NONE',  ( 104.1015100224914960, -46.74719628246504044, 107.3470538473389411 ) ) ;
#87654=CARTESIAN_POINT ( 'NONE',  ( 116.8171228670854447, -34.15291832200010447, 144.0314586091287197 ) ) ;
#87658=DIRECTION ( 'NONE',  ( 0.000000000000000000, 1.000000000000000000, 0.000000000000000000 ) ) ;
#87662=DIRECTION ( 'NONE',  ( 0.000000000000000000, 0.000000000000000000, 1.000000000000000000 ) ) ;
#87663=DIRECTION ( 'NONE',  ( 9.351236661543306751E-17, -3.725950533538267725E-29, -1.000000000000000000 ) ) ;
#87664=PLANE ( 'NONE',  #49490 ) ;
#87666=CIRCLE ( 'NONE', #76058, 5.599999999999994316 ) ;
#87667=CARTESIAN_POINT ( 'NONE',  ( 98.30753431935190179, -41.72887571374209159, 32.73979196285422688 ) ) ;
#87668=CARTESIAN_POINT ( 'NONE',  ( 115.7764676695377517, -43.63945112744033850, 194.2927681330539542 ) ) ;
#87669=ORIENTED_EDGE ( 'NONE', *, *, #1227, .F. ) ;
#87670=CARTESIAN_POINT ( 'NONE',  ( 97.58158007118578325, -32.53714515026965870, 51.98324432352896451 ) ) ;
#87673=CARTESIAN_POINT ( 'NONE',  ( 87.31648329127403940, -46.72944715994105280, -5.074374724089048883 ) ) ;
#87676=VERTEX_POINT ( 'NONE', #63966 ) ;
#87677=ORIENTED_EDGE ( 'NONE', *, *, #19603, .F. ) ;
#87679=CARTESIAN_POINT ( 'NONE',  ( 115.1079044709731676, -40.52387399376650734, 224.9072975916109840 ) ) ;
#87680=VECTOR ( 'NONE', #15092, 1000.000000000000000 ) ;
#87683=VECTOR ( 'NONE', #75384, 1000.000000000000000 ) ;
#87685=CIRCLE ( 'NONE', #25306, 2.117000000000007987 ) ;
#87686=DIRECTION ( 'NONE',  ( 1.000000000000000000, 4.163336342344333240E-14, 0.000000000000000000 ) ) ;
#87687=CARTESIAN_POINT ( 'NONE',  ( 82.32434691320904108, -38.30306751046272495, 2.518077574344857350 ) ) ;
#87688=CIRCLE ( 'NONE', #48495, 10.00000000000000711 ) ;
#87690=CARTESIAN_POINT ( 'NONE',  ( 73.24325998657060666, -46.55267046464442160, 14.92562527591093868 ) ) ;
#87692=ORIENTED_EDGE ( 'NONE', *, *, #68561, .T. ) ;
#87693=CARTESIAN_POINT ( 'NONE',  ( 118.5710604172009965, -33.89858672578665733, 14.01848241876796308 ) ) ;
#87694=EDGE_LOOP ( 'NONE', ( #41660, #77771 ) ) ;
#87696=CARTESIAN_POINT ( 'NONE',  ( 107.8084489643801334, -27.48037055177216104, 262.8309475124484038 ) ) ;
#87697=CARTESIAN_POINT ( 'NONE',  ( 177.0664832912730162, 12.92155284005730387, 355.9756252759109998 ) ) ;
#87699=FACE_OUTER_BOUND ( 'NONE', #82891, .T. ) ;
#87701=CARTESIAN_POINT ( 'NONE',  ( 98.34346157482828232, -29.86603762143552032, 196.8080062282919869 ) ) ;
#87704=EDGE_CURVE ( 'NONE', #61739, #53210, #2188, .T. ) ;
#87705=CARTESIAN_POINT ( 'NONE',  ( 113.4418579183357849, -27.64362872000679516, 80.57753003781597556 ) ) ;
#87707=ORIENTED_EDGE ( 'NONE', *, *, #32998, .F. ) ;
#87708=VERTEX_POINT ( 'NONE', #35341 ) ;
#87709=ORIENTED_EDGE ( 'NONE', *, *, #21092, .F. ) ;
#87710=CARTESIAN_POINT ( 'NONE',  ( 102.0657985602851596, -27.97123491610403434, 160.4896842913302066 ) ) ;
#87711=PLANE ( 'NONE',  #41301 ) ;
#87712=CARTESIAN_POINT ( 'NONE',  ( 97.81170238817014706, -40.51743819009087844, 137.6355114220584994 ) ) ;
#87713=CARTESIAN_POINT ( 'NONE',  ( 105.6960798208838384, -45.90617939248504342, 145.2766617981629622 ) ) ;
#87714=CARTESIAN_POINT ( 'NONE',  ( 98.88183825371838509, -29.26641886349639066, 226.7261014663869503 ) ) ;
#87715=CARTESIAN_POINT ( 'NONE',  ( 168.3595971214446934, -48.62134037892948157, 249.9678068554149775 ) ) ;
#87716=VERTEX_POINT ( 'NONE', #50311 ) ;
#87718=DIRECTION ( 'NONE',  ( -4.237773401492740281E-14, 1.000000000000000000, 0.000000000000000000 ) ) ;
#87720=VERTEX_POINT ( 'NONE', #43043 ) ;
#87723=VERTEX_POINT ( 'NONE', #42592 ) ;
#87724=ORIENTED_EDGE ( 'NONE', *, *, #70395, .F. ) ;
#87725=LINE ( 'NONE', #17350, #32336 ) ;
#87726=AXIS2_PLACEMENT_3D ( 'NONE', #42046, #30227, #29781 ) ;
#87728=CARTESIAN_POINT ( 'NONE',  ( 102.0657424188261899, -27.97126782499678299, 25.48991181321247268 ) ) ;
#87729=EDGE_CURVE ( 'NONE', #37766, #85594, #78055, .T. ) ;
#87730=CARTESIAN_POINT ( 'NONE',  ( 97.64684354035226477, -39.08338314719364348, 165.9438483995059528 ) ) ;
#87731=CARTESIAN_POINT ( 'NONE',  ( 96.64524470886469487, -32.90705862865544162, 21.03467289495897319 ) ) ;
#87734=EDGE_CURVE ( 'NONE', #21614, #58445, #49861, .T. ) ;
#87735=LINE ( 'NONE', #24615, #18016 ) ;
#87736=EDGE_CURVE ( 'NONE', #75279, #78504, #71678, .T. ) ;
#87740=ORIENTED_EDGE ( 'NONE', *, *, #81484, .F. ) ;
#87743=CARTESIAN_POINT ( 'NONE',  ( 116.9280472011850520, -38.65089867813137658, 133.6735763414937423 ) ) ;
#87745=AXIS2_PLACEMENT_3D ( 'NONE', #56602, #71157, #30258 ) ;
#87746=ORIENTED_EDGE ( 'NONE', *, *, #4979, .T. ) ;
#87747=CARTESIAN_POINT ( 'NONE',  ( 116.7906267970580103, -31.42506456344890964, 24.21181575210196257 ) ) ;
#87749=CARTESIAN_POINT ( 'NONE',  ( 115.7648065088891371, -43.62413145733483333, 44.30514908543492680 ) ) ;
#87750=AXIS2_PLACEMENT_3D ( 'NONE', #86127, #9819, #37526 ) ;
#87753=DIRECTION ( 'NONE',  ( 1.000000000000000078E-15, 0.000000000000000000, 1.000000000000000000 ) ) ;
#87756=CARTESIAN_POINT ( 'NONE',  ( 176.7669697523291461, -48.62818131005482059, 249.9678068554149775 ) ) ;
#87758=EDGE_CURVE ( 'NONE', #35953, #67515, #23099, .T. ) ;
#87760=CARTESIAN_POINT ( 'NONE',  ( 46.48091746482047171, -48.32844715994088602, 129.9678068554150911 ) ) ;
#87762=VERTEX_POINT ( 'NONE', #43493 ) ;
#87763=CARTESIAN_POINT ( 'NONE',  ( 118.7820429505835733, -34.63792632846725184, 48.96705384733895983 ) ) ;
#87764=CARTESIAN_POINT ( 'NONE',  ( 98.03678599612689482, -44.40402742967116723, 222.8870538473399563 ) ) ;
#87765=CARTESIAN_POINT ( 'NONE',  ( 117.1124756048696440, -32.06433792440376607, 55.16038718067301261 ) ) ;
#87766=CARTESIAN_POINT ( 'NONE',  ( 97.81555608408764613, -40.52686364465421320, 171.6367057649424623 ) ) ;
#87767=FACE_OUTER_BOUND ( 'NONE', #17129, .T. ) ;
#87769=VECTOR ( 'NONE', #80521, 1000.000000000000000 ) ;
#87770=VECTOR ( 'NONE', #49632, 1000.000000000000000 ) ;
#87771=ORIENTED_EDGE ( 'NONE', *, *, #7022, .F. ) ;
#87772=CARTESIAN_POINT ( 'NONE',  ( 112.1393456656949041, -28.01282279600963676, 185.6564586070249447 ) ) ;
#87773=ORIENTED_EDGE ( 'NONE', *, *, #23826, .T. ) ;
#87774=CARTESIAN_POINT ( 'NONE',  ( 97.83387747045378546, -32.00739517038279303, 91.96229194257693962 ) ) ;
#87776=ORIENTED_EDGE ( 'NONE', *, *, #68228, .F. ) ;
#87777=CARTESIAN_POINT ( 'NONE',  ( 110.2492204789523100, -26.78788743924354065, 230.8299109901969643 ) ) ;
#87779=DIRECTION ( 'NONE',  ( -0.000000000000000000, -0.000000000000000000, 1.000000000000000000 ) ) ;
#87781=CARTESIAN_POINT ( 'NONE',  ( 188.5667039024479834, -62.87844715994099687, 293.2178068554150627 ) ) ;
#87782=CARTESIAN_POINT ( 'NONE',  ( 133.4132809338130699, -39.40256188477528099, 1.689562700881797053 ) ) ;
#87784=CARTESIAN_POINT ( 'NONE',  ( 116.8150918559700813, -40.26546416881835455, 173.5375300378159693 ) ) ;
#87785=EDGE_LOOP ( 'NONE', ( #47152, #34424, #39443, #85604 ) ) ;
#87786=ORIENTED_EDGE ( 'NONE', *, *, #57790, .T. ) ;
#87787=ADVANCED_FACE ( 'NONE', ( #9442 ), #1743, .F. ) ;
#87788=CARTESIAN_POINT ( 'NONE',  ( 108.7714652236932835, -45.96901220096565055, 124.1653928297069882 ) ) ;
#87789=LINE ( 'NONE', #82339, #44295 ) ;
#87790=CARTESIAN_POINT ( 'NONE',  ( 101.9853755998761500, -45.08682593082387058, 243.1413395616249886 ) ) ;
#87791=CARTESIAN_POINT ( 'NONE',  ( 107.0667039024468039, -54.72944715994100306, 199.5838068554169809 ) ) ;
#87793=CARTESIAN_POINT ( 'NONE',  ( 194.5667039024479834, -40.82844715993405771, 300.4678068554149490 ) ) ;
#87799=LINE ( 'NONE', #46880, #35670 ) ;
#87800=CARTESIAN_POINT ( 'NONE',  ( 117.0473132972741865, -39.66401662079137225, 183.5984824187679578 ) ) ;
#87801=CARTESIAN_POINT ( 'NONE',  ( 100.9548448467986219, -28.70687276283804934, 170.5930046438545276 ) ) ;
#87802=VERTEX_POINT ( 'NONE', #37151 ) ;
#87803=VERTEX_POINT ( 'NONE', #71239 ) ;
#87804=FACE_OUTER_BOUND ( 'NONE', #31534, .T. ) ;
#87805=CARTESIAN_POINT ( 'NONE',  ( 81.55977255149463190, -21.04085022825163520, 7.869587501197700341 ) ) ;
#87806=B_SPLINE_CURVE_WITH_KNOTS ( 'NONE', 3,
 ( #78680, #17323, #4127, #9170, #10938, #71844, #15990, #37316, #9607, #43670, #17762, #72291, #71406, #66342, #31378, #86367, #3251, #23272 ),
 .UNSPECIFIED., .F., .F.,
 ( 4, 2, 2, 2, 2, 2, 2, 2, 4 ),
 ( 0.4999999997770634419, 0.5624999998049304839, 0.6249999998327975259, 0.6874999998606646789, 0.7499999998885317209, 0.8124999999163987630, 0.8749999999442659160, 0.9374999999721329580, 1.000000000000000000 ),
 .UNSPECIFIED. ) ;
#87808=LINE ( 'NONE', #88718, #74371 ) ;
#87809=AXIS2_PLACEMENT_3D ( 'NONE', #26452, #46422, #32807 ) ;
#87810=CARTESIAN_POINT ( 'NONE',  ( 97.70670343771699606, -40.25169526565032641, 96.61288812823406147 ) ) ;
#87811=VERTEX_POINT ( 'NONE', #63055 ) ;
#87812=ADVANCED_FACE ( 'NONE', ( #78506 ), #85768, .F. ) ;
#87813=CONICAL_SURFACE ( 'NONE', #15331, 1.258750000000002922, 1.029744258676650093 ) ;
#87815=VECTOR ( 'NONE', #37408, 1000.000000000000000 ) ;
#87816=AXIS2_PLACEMENT_3D ( 'NONE', #45316, #73482, #52121 ) ;
#87817=CARTESIAN_POINT ( 'NONE',  ( 115.8553914792215380, -44.67901184617146981, 233.2413395616259493 ) ) ;
#87818=DIRECTION ( 'NONE',  ( 3.999999999999999995E-14, -1.000000000000000000, 4.100000000000000342E-29 ) ) ;
#87820=EDGE_LOOP ( 'NONE', ( #11345, #62326, #29921, #9242 ) ) ;
#87821=AXIS2_PLACEMENT_3D ( 'NONE', #53879, #12583, #8002 ) ;
#87822=CARTESIAN_POINT ( 'NONE',  ( 116.6612529692701230, -33.83881916766647180, 65.05964535752768541 ) ) ;
#87823=PLANE ( 'NONE',  #71029 ) ;
#87824=CARTESIAN_POINT ( 'NONE',  ( 98.54779198038390575, -41.97720663294746402, 166.7658525804957890 ) ) ;
#87825=CARTESIAN_POINT ( 'NONE',  ( 110.3993955946342993, -29.27817736879564237, 22.55951894101998434 ) ) ;
#87826=CARTESIAN_POINT ( 'NONE',  ( 113.9312237880395600, -28.03689036367077492, 120.5565776568639507 ) ) ;
#87827=AXIS2_PLACEMENT_3D ( 'NONE', #62634, #13591, #6774 ) ;
#87830=ORIENTED_EDGE ( 'NONE', *, *, #82165, .T. ) ;
#87831=AXIS2_PLACEMENT_3D ( 'NONE', #32240, #67212, #74486 ) ;
#87833=CARTESIAN_POINT ( 'NONE',  ( 106.5394234437989667, -24.24056378642895737, 322.0356252759110021 ) ) ;
#87835=EDGE_LOOP ( 'NONE', ( #56495, #79410, #77345, #79144, #84534, #17453 ) ) ;
#87837=EDGE_LOOP ( 'NONE', ( #44646, #71640 ) ) ;
#87839=CARTESIAN_POINT ( 'NONE',  ( 105.7976818973216666, -26.72428486692717797, 156.1772091278820653 ) ) ;
#87840=AXIS2_PLACEMENT_3D ( 'NONE', #9220, #596, #42812 ) ;
#87841=CARTESIAN_POINT ( 'NONE',  ( 106.1832117796525807, -28.23380338452170335, 49.58099125664799800 ) ) ;
#87842=CARTESIAN_POINT ( 'NONE',  ( 116.8782924623045290, -40.31758940317881468, 218.5470538473399529 ) ) ;
#87843=CARTESIAN_POINT ( 'NONE',  ( 102.0615167388204725, -46.55869598106830409, 172.2137205140059564 ) ) ;
#87844=DIRECTION ( 'NONE',  ( 0.000000000000000000, 0.000000000000000000, -1.000000000000000000 ) ) ;
#87845=CARTESIAN_POINT ( 'NONE',  ( 101.0866664386429647, -45.26901348810219616, 278.0899109901965858 ) ) ;
#87848=DIRECTION ( 'NONE',  ( 0.7071067811865779928, -0.7071067811865171526, 7.071067811865475333E-16 ) ) ;
#87849=ORIENTED_EDGE ( 'NONE', *, *, #29455, .F. ) ;
#87850=ORIENTED_EDGE ( 'NONE', *, *, #35212, .T. ) ;
#87851=CIRCLE ( 'NONE', #47238, 3.000000000000002665 ) ;
#87853=CARTESIAN_POINT ( 'NONE',  ( 103.2876017065440664, -26.96590681778891252, 215.3699109901969848 ) ) ;
#87854=ORIENTED_EDGE ( 'NONE', *, *, #36470, .F. ) ;
#87855=CARTESIAN_POINT ( 'NONE',  ( 95.40772882630993479, -38.85404833720006224, 201.4699109901969791 ) ) ;
#87856=CARTESIAN_POINT ( 'NONE',  ( 115.0878329645725131, -30.61624704198809610, 264.3439639102033425 ) ) ;
#87857=VECTOR ( 'NONE', #60586, 1000.000000000000000 ) ;
#87858=DIRECTION ( 'NONE',  ( 0.1858654558203329255, -0.9825752044157738396, 0.000000000000000000 ) ) ;
#87860=CARTESIAN_POINT ( 'NONE',  ( 100.6116892621281949, -31.39203453219122864, 277.6356252759112522 ) ) ;
#87861=LINE ( 'NONE', #54643, #31145 ) ;
#87862=CARTESIAN_POINT ( 'NONE',  ( 109.6428154823273644, -46.48014078660262527, 173.7814426156472223 ) ) ;
#87864=CARTESIAN_POINT ( 'NONE',  ( 19.56648329127400032, 25.62155284005901379, 323.8756252759109202 ) ) ;
#87867=EDGE_CURVE ( 'NONE', #19753, #47917, #77148, .T. ) ;
#87868=DIRECTION ( 'NONE',  ( -0.7071067811985214391, 0.7071067811745735954, 0.000000000000000000 ) ) ;
#87870=CARTESIAN_POINT ( 'NONE',  ( 99.69663197418856271, -31.46466773810444906, 195.5838068554171230 ) ) ;
#87871=VERTEX_POINT ( 'NONE', #4857 ) ;
#87872=FACE_OUTER_BOUND ( 'NONE', #16549, .T. ) ;
#87873=CARTESIAN_POINT ( 'NONE',  ( 113.0381276193345883, -46.05869713813741129, 218.0175300378159591 ) ) ;
#87874=CARTESIAN_POINT ( 'NONE',  ( 97.93258204476157402, -31.63109636822184711, 106.9213395616259703 ) ) ;
#87875=CARTESIAN_POINT ( 'NONE',  ( 97.12841500021716001, -40.02000613830777098, 237.5813395616249579 ) ) ;
#87876=CARTESIAN_POINT ( 'NONE',  ( 49.16670390244701139, -28.27351298637340093, -5.074374724088000832 ) ) ;
#87877=CARTESIAN_POINT ( 'NONE',  ( 80.06648329127398256, -9.029447159941060619, 4.925625275910944012 ) ) ;
#87878=CARTESIAN_POINT ( 'NONE',  ( 34.33598329127477911, -36.32844715994133367, 300.4678068554150059 ) ) ;
#87879=FACE_OUTER_BOUND ( 'NONE', #42669, .T. ) ;
#87880=PLANE ( 'NONE',  #66811 ) ;
#87881=LINE ( 'NONE', #25646, #83387 ) ;
#87882=VECTOR ( 'NONE', #15416, 1000.000000000000114 ) ;
#87883=AXIS2_PLACEMENT_3D ( 'NONE', #77628, #84462, #89929 ) ;
#87884=CIRCLE ( 'NONE', #31331, 4.750000000000004441 ) ;
#87885=AXIS2_PLACEMENT_3D ( 'NONE', #7592, #35279, #68473 ) ;
#87887=ORIENTED_EDGE ( 'NONE', *, *, #81101, .F. ) ;
#87888=CARTESIAN_POINT ( 'NONE',  ( 112.8906599442021275, -43.66427313951261624, 147.5428960185529661 ) ) ;
#87890=ORIENTED_EDGE ( 'NONE', *, *, #35027, .T. ) ;
#87891=CARTESIAN_POINT ( 'NONE',  ( 179.1667039024473809, -26.71338133338671739, 313.9678068554149490 ) ) ;
#87892=CARTESIAN_POINT ( 'NONE',  ( 107.3333893024683903, -26.32957087652229689, 116.0556252759109555 ) ) ;
#87894=CARTESIAN_POINT ( 'NONE',  ( 152.0368932755773130, -23.42844715993587812, 129.9678068554149775 ) ) ;
#87898=CARTESIAN_POINT ( 'NONE',  ( 99.16769444712198833, -43.44866735504071187, 76.89943479972100704 ) ) ;
#87899=ORIENTED_EDGE ( 'NONE', *, *, #65870, .T. ) ;
#87900=EDGE_LOOP ( 'NONE', ( #35192, #87332, #29013, #57631 ) ) ;
#87902=DIRECTION ( 'NONE',  ( 1.000000000000000078E-15, 1.000000000000000083E-30, -1.000000000000000000 ) ) ;
#87904=CARTESIAN_POINT ( 'NONE',  ( 116.8150918559699818, -40.26546416881831192, 169.5375300378149745 ) ) ;
#87905=CARTESIAN_POINT ( 'NONE',  ( 36.65249034007441509, -48.32844715994130524, 180.4678068554150911 ) ) ;
#87907=DIRECTION ( 'NONE',  ( -1.000000000000000000, 1.000000000000000078E-15, 0.000000000000000000 ) ) ;
#87908=DIRECTION ( 'NONE',  ( 4.299999999999999979E-14, -1.000000000000000000, 0.000000000000000000 ) ) ;
#87909=CYLINDRICAL_SURFACE ( 'NONE', #54657, 1.000000000000000888 ) ;
#87910=DIRECTION ( 'NONE',  ( 0.000000000000000000, 1.000000000000000000, 0.000000000000000000 ) ) ;
#87912=CARTESIAN_POINT ( 'NONE',  ( 103.8480726019013218, -46.65951555449696997, 82.32705384733995402 ) ) ;
#87916=DIRECTION ( 'NONE',  ( -0.9254794337955620787, -0.3787978585227822492, 0.000000000000000000 ) ) ;
#87917=CARTESIAN_POINT ( 'NONE',  ( 180.2121375201597004, -29.73316016638962722, 193.9678068554150059 ) ) ;
#87918=CARTESIAN_POINT ( 'NONE',  ( 100.8299159177638984, -43.59960581930123880, 154.8080903695919801 ) ) ;
#87919=EDGE_CURVE ( 'NONE', #7620, #73802, #44839, .T. ) ;
#87921=ORIENTED_EDGE ( 'NONE', *, *, #44750, .T. ) ;
#87923=ADVANCED_FACE ( 'NONE', ( #72117 ), #87089, .F. ) ;
#87924=CARTESIAN_POINT ( 'NONE',  ( 141.8664832912729992, -71.52944715994142655, 361.9756252759109998 ) ) ;
#87925=VERTEX_POINT ( 'NONE', #3511 ) ;
#87926=VERTEX_POINT ( 'NONE', #87982 ) ;
#87928=EDGE_CURVE ( 'NONE', #61077, #37281, #38040, .T. ) ;
#87929=CARTESIAN_POINT ( 'NONE',  ( 107.5663136956459738, -46.11170142552477813, 194.0625356868489462 ) ) ;
#87930=EDGE_CURVE ( 'NONE', #54590, #24712, #44760, .T. ) ;
#87931=CARTESIAN_POINT ( 'NONE',  ( 112.2214490935429438, -49.20647916188104887, 293.6356252759106837 ) ) ;
#87932=VECTOR ( 'NONE', #16776, 1000.000000000000000 ) ;
#87936=CIRCLE ( 'NONE', #61788, 2.116999999999993776 ) ;
#87937=VERTEX_POINT ( 'NONE', #58466 ) ;
#87938=ORIENTED_EDGE ( 'NONE', *, *, #48176, .F. ) ;
#87939=AXIS2_PLACEMENT_3D ( 'NONE', #60008, #68201, #20509 ) ;
#87942=ORIENTED_EDGE ( 'NONE', *, *, #1554, .F. ) ;
#87943=EDGE_CURVE ( 'NONE', #13404, #30894, #37577, .T. ) ;
#87944=CARTESIAN_POINT ( 'NONE',  ( 114.5355946289170390, -40.02218186577253789, 251.3138046553057734 ) ) ;
#87945=CARTESIAN_POINT ( 'NONE',  ( 117.1278252906914048, -39.54294340788323581, 98.60991099019594230 ) ) ;
#87946=CARTESIAN_POINT ( 'NONE',  ( 117.9791962420231073, -38.33460093242097599, 73.72229194257801055 ) ) ;
#87947=CARTESIAN_POINT ( 'NONE',  ( 104.6193894214979707, -44.52608570832915547, 249.5838068554171798 ) ) ;
#87948=PRODUCT ( 'Feed Lead', 'Feed Lead', '', ( #88992 ) ) ;
#87950=DIRECTION ( 'NONE',  ( 0.000000000000000000, 0.000000000000000000, 1.000000000000000000 ) ) ;
#87951=CARTESIAN_POINT ( 'NONE',  ( 99.42212199502026237, -27.67378918447352731, 146.6356252759109395 ) ) ;
#87952=ADVANCED_FACE ( 'NONE', ( #17600 ), #45279, .F. ) ;
#87956=ORIENTED_EDGE ( 'NONE', *, *, #62939, .F. ) ;
#87957=ORIENTED_EDGE ( 'NONE', *, *, #24898, .F. ) ;
#87959=CARTESIAN_POINT ( 'NONE',  ( 165.6738106836199904, -26.00627455219321860, -5.074374724088000832 ) ) ;
#87960=AXIS2_PLACEMENT_3D ( 'NONE', #70985, #63710, #44134 ) ;
#87962=LINE ( 'NONE', #19814, #27259 ) ;
#87963=EDGE_LOOP ( 'NONE', ( #74377, #66988, #62168, #26300 ) ) ;
#87964=CARTESIAN_POINT ( 'NONE',  ( 105.7154773057149839, -46.72385838908932953, 177.4689586075003547 ) ) ;
#87965=CARTESIAN_POINT ( 'NONE',  ( 97.54218415029114908, -32.48978251111615378, 100.9927681330539713 ) ) ;
#87969=CYLINDRICAL_SURFACE ( 'NONE', #47003, 9.999999999999998224 ) ;
#87970=CARTESIAN_POINT ( 'NONE',  ( 105.7154773207258813, -46.72385839099544569, 143.4689586084740824 ) ) ;
#87972=CARTESIAN_POINT ( 'NONE',  ( 97.69433714244412670, -41.24514667321082584, 167.6841967044829573 ) ) ;
#87973=DIRECTION ( 'NONE',  ( 0.000000000000000000, 0.000000000000000000, 1.000000000000000000 ) ) ;
#87975=ORIENTED_EDGE ( 'NONE', *, *, #40964, .T. ) ;
#87976=PLANE ( 'NONE',  #44006 ) ;
#87977=EDGE_CURVE ( 'NONE', #42544, #41323, #44388, .T. ) ;
#87978=CARTESIAN_POINT ( 'NONE',  ( 116.3212776292296127, -32.94146857471318413, 287.6356252759109680 ) ) ;
#87979=ADVANCED_FACE ( 'NONE', ( #10763 ), #9893, .T. ) ;
#87980=CARTESIAN_POINT ( 'NONE',  ( 105.8009397366041497, -26.72383029953164524, 135.1771514046403411 ) ) ;
#87981=ADVANCED_FACE ( 'NONE', ( #17156 ), #45712, .F. ) ;
#87982=CARTESIAN_POINT ( 'NONE',  ( 176.5667039024390306, -48.82844715994099971, 249.9678068554149775 ) ) ;
#87983=CARTESIAN_POINT ( 'NONE',  ( 96.72907894039983034, -34.86132901292410224, 241.1841967044819626 ) ) ;
#87985=CARTESIAN_POINT ( 'NONE',  ( 194.0371591254575776, -24.42818131005417115, 116.4678068554150201 ) ) ;
#87986=CARTESIAN_POINT ( 'NONE',  ( 96.51501197915654018, -40.09867661842082498, 277.5603871806729899 ) ) ;
#87987=CARTESIAN_POINT ( 'NONE',  ( 96.56348986465089013, -36.88801538493378018, 132.3384824187679669 ) ) ;
#87988=ADVANCED_FACE ( 'NONE', ( #3961 ), #80725, .F. ) ;
#87989=DIRECTION ( 'NONE',  ( 4.299999999999999979E-14, -1.000000000000000000, 4.400000000000000367E-29 ) ) ;
#87991=AXIS2_PLACEMENT_3D ( 'NONE', #9068, #36768, #23600 ) ;
#87994=DIRECTION ( 'NONE',  ( 1.000000000000000078E-15, -1.000000000000000083E-30, -1.000000000000000000 ) ) ;
#87995=VERTEX_POINT ( 'NONE', #66628 ) ;
#87996=ORIENTED_EDGE ( 'NONE', *, *, #85239, .T. ) ;
#87997=VERTEX_POINT ( 'NONE', #11681 ) ;
#88000=CARTESIAN_POINT ( 'NONE',  ( 97.37192905580968727, -32.85904099757684804, 37.02419670448292521 ) ) ;
#88001=DIRECTION ( 'NONE',  ( 0.000000000000000000, 1.000000000000000000, 0.000000000000000000 ) ) ;
#88004=CARTESIAN_POINT ( 'NONE',  ( 48.45959712127293528, -26.00627455219328610, 117.4678068554150485 ) ) ;
#88006=CARTESIAN_POINT ( 'NONE',  ( 110.1391594044062003, -28.21056625751448976, 249.2114674471249600 ) ) ;
#88009=VERTEX_POINT ( 'NONE', #39374 ) ;
#88010=VECTOR ( 'NONE', #57813, 1000.000000000000000 ) ;
#88011=AXIS2_PLACEMENT_3D ( 'NONE', #52685, #59072, #30944 ) ;
#88013=AXIS2_PLACEMENT_3D ( 'NONE', #40312, #54363, #61207 ) ;
#88014=CARTESIAN_POINT ( 'NONE',  ( 115.9448851316561928, -41.40291037483353875, 183.4410333944183549 ) ) ;
#88015=LINE ( 'NONE', #19867, #54200 ) ;
#88017=CARTESIAN_POINT ( 'NONE',  ( 114.7948027157550399, -42.07682430429896669, 9.788249972563944468 ) ) ;
#88018=CARTESIAN_POINT ( 'NONE',  ( 41.56648329127398966, -27.82844715994070484, 198.9256252759119832 ) ) ;
#88020=CARTESIAN_POINT ( 'NONE',  ( 109.0793648114890715, -47.66380995969711876, 277.7213395616258822 ) ) ;
#88023=CARTESIAN_POINT ( 'NONE',  ( 97.07198842992696086, -35.37925190007393894, 57.21895314611191452 ) ) ;
#88024=VECTOR ( 'NONE', #86733, 1000.000000000000000 ) ;
#88025=FACE_OUTER_BOUND ( 'NONE', #44567, .T. ) ;
#88026=CARTESIAN_POINT ( 'NONE',  ( 98.55283614654496205, -38.28467619158744384, 49.30047132197196191 ) ) ;
#88029=CARTESIAN_POINT ( 'NONE',  ( 136.5762189171834962, -17.60488046388850591, 7.068409955833985236 ) ) ;
#88033=CARTESIAN_POINT ( 'NONE',  ( 113.1781950736253748, -44.75194242080101503, 194.0939235927813513 ) ) ;
#88035=LINE ( 'NONE', #74400, #11721 ) ;
#88036=EDGE_CURVE ( 'NONE', #69124, #66137, #69325, .T. ) ;
#88038=EDGE_LOOP ( 'NONE', ( #69278, #64561 ) ) ;
#88039=CARTESIAN_POINT ( 'NONE',  ( 104.1077555235347631, -46.72609462085661391, 107.3470538473389411 ) ) ;
#88041=B_SPLINE_CURVE_WITH_KNOTS ( 'NONE', 3,
 ( #26445, #40059, #18732, #11924, #67318, #26000, #53669, #81436, #46858, #67777, #74590, #5566, #33258, #54118, #17399, #65976, #31456, #59161, #19625, #35484, #6891, #69126, #6448, #55010, #68680, #48653, #76384, #12831, #47312, #41397, #14619 ),
 .UNSPECIFIED., .F., .F.,
 ( 4, 2, 2, 2, 2, 2, 2, 2, 2, 2, 1, 1, 1, 1, 1, 1, 1, 2, 4 ),
 ( 0.000000000000000000, 0.06250382389165948238, 0.1250076477833189648, 0.1875114716749784471, 0.2500152955666379295, 0.3125191194582974119, 0.3750229433499568943, 0.4375267672416163767, 0.4687786791874462566, 0.4844046351603611411, 0.4922176131468187776, 0.4961241021400474849, 0.4980773466366619773, 0.4990539688849690014, 0.4995422800091225413, 0.4997864355711990614, 0.4999085133522373492, 0.4999695522427566319, 0.5000305911332758591 ),
 .UNSPECIFIED. ) ;
#88042=CARTESIAN_POINT ( 'NONE',  ( 108.6385355886969108, -45.12496878139073431, 82.14670554236298017 ) ) ;
#88043=EDGE_CURVE ( 'NONE', #39062, #2317, #41149, .T. ) ;
#88044=CARTESIAN_POINT ( 'NONE',  ( 98.98640610341819013, -42.64021795225433209, 87.82849860576001788 ) ) ;
#88045=CARTESIAN_POINT ( 'NONE',  ( 97.22447099779657265, -34.58340453033963513, 102.5872975916109482 ) ) ;
#88046=EDGE_CURVE ( 'NONE', #33376, #39081, #34794, .T. ) ;
#88049=CARTESIAN_POINT ( 'NONE',  ( 99.48587976144928291, -43.91775078298940116, 77.92991099019597812 ) ) ;
#88050=AXIS2_PLACEMENT_3D ( 'NONE', #600, #22860, #29219 ) ;
#88051=CARTESIAN_POINT ( 'NONE',  ( 112.1398324001274887, -28.01310167226245085, 180.6568491273569350 ) ) ;
#88052=EDGE_CURVE ( 'NONE', #32467, #59850, #34341, .T. ) ;
#88053=ORIENTED_EDGE ( 'NONE', *, *, #17243, .T. ) ;
#88057=VERTEX_POINT ( 'NONE', #47057 ) ;
#88058=EDGE_LOOP ( 'NONE', ( #89631, #32161, #10701, #25569 ) ) ;
#88059=EDGE_CURVE ( 'NONE', #72562, #17905, #2770, .T. ) ;
#88060=PLANE ( 'NONE',  #65884 ) ;
#88062=CARTESIAN_POINT ( 'NONE',  ( 104.4938967476557536, -26.68352342390101128, 245.2880062282919482 ) ) ;
#88063=CARTESIAN_POINT ( 'NONE',  ( 113.7362177204465041, -29.20338847083969114, 124.4983641739881506 ) ) ;
#88065=CARTESIAN_POINT ( 'NONE',  ( 117.4876440797474828, -37.01562065295904347, 39.80419670448193159 ) ) ;
#88067=CARTESIAN_POINT ( 'NONE',  ( 107.0664832912739968, -36.72944715994100306, 394.9756252759102040 ) ) ;
#88068=EDGE_LOOP ( 'NONE', ( #42393, #58216, #44585, #82200 ) ) ;
#88069=CARTESIAN_POINT ( 'NONE',  ( 116.3212776292296127, -32.94146857471318413, 287.6356252759109680 ) ) ;
#88070=VECTOR ( 'NONE', #44734, 999.9999999999998863 ) ;
#88071=CIRCLE ( 'NONE', #21346, 0.5000000000000004441 ) ;
#88072=CARTESIAN_POINT ( 'NONE',  ( 182.5667039024469886, -33.35206098992650681, -5.074374724088000832 ) ) ;
#88074=CIRCLE ( 'NONE', #9748, 4.875000000000017764 ) ;
#88075=CARTESIAN_POINT ( 'NONE',  ( 138.8545562996767444, -1.932463243632620342, 361.9756252759100335 ) ) ;
#88076=VECTOR ( 'NONE', #82437, 1000.000000000000000 ) ;
#88077=DIRECTION ( 'NONE',  ( -0.0001211784769804366042, 0.7071067708032299226, 0.7071067811865512365 ) ) ;
#88078=CARTESIAN_POINT ( 'NONE',  ( 116.2977993645976227, -41.52656014244018223, 288.4441967044823514 ) ) ;
#88079=DIRECTION ( 'NONE',  ( 0.7071067811868710917, -0.7071067811862240537, 0.000000000000000000 ) ) ;
#88080=CIRCLE ( 'NONE', #72134, 4.875000000000017764 ) ;
#88081=LINE ( 'NONE', #53962, #73825 ) ;
#88082=CARTESIAN_POINT ( 'NONE',  ( 97.81375517989221180, -40.51659548082960072, 91.63516306087667829 ) ) ;
#88083=CARTESIAN_POINT ( 'NONE',  ( 98.62497865991430501, -35.42670724699001283, 265.6267055423624583 ) ) ;
#88085=CARTESIAN_POINT ( 'NONE',  ( 96.10063762778156615, -37.91858611869021445, 77.40038718067299328 ) ) ;
#88087=CARTESIAN_POINT ( 'NONE',  ( 114.5591802247839865, -28.54312911867770808, 154.4746728949589851 ) ) ;
#88088=ORIENTED_EDGE ( 'NONE', *, *, #62139, .F. ) ;
#88089=DIRECTION ( 'NONE',  ( 1.000000000000000078E-15, -1.000000000000000083E-30, -1.000000000000000000 ) ) ;
#88090=ORIENTED_EDGE ( 'NONE', *, *, #36008, .F. ) ;
#88093=CARTESIAN_POINT ( 'NONE',  ( 29.56648329127400388, 25.62155284005901379, 323.8756252759109202 ) ) ;
#88095=CARTESIAN_POINT ( 'NONE',  ( 134.4427611689536093, -33.99866847873244069, 1.641799428525427151 ) ) ;
#88096=ORIENTED_EDGE ( 'NONE', *, *, #53097, .F. ) ;
#88097=EDGE_CURVE ( 'NONE', #24965, #73817, #10026, .T. ) ;
#88098=DIRECTION ( 'NONE',  ( -9.351236661543306751E-17, 3.725950533538267165E-29, 1.000000000000000000 ) ) ;
#88099=CARTESIAN_POINT ( 'NONE',  ( 114.5437501075917481, -29.39581020157643110, 149.4441967044819819 ) ) ;
#88100=ORIENTED_EDGE ( 'NONE', *, *, #3317, .T. ) ;
#88102=CARTESIAN_POINT ( 'NONE',  ( 71.06648329127399677, -18.82844715994099971, 323.8756252759120002 ) ) ;
#88104=ADVANCED_FACE ( 'NONE', ( #33001 ), #88884, .T. ) ;
#88105=DIRECTION ( 'NONE',  ( -2.279500465453769633E-16, 0.000000000000000000, 1.000000000000000000 ) ) ;
#88108=DIRECTION ( 'NONE',  ( 0.1811243268507065352, -0.9834602067307444129, 0.000000000000000000 ) ) ;
#88110=CIRCLE ( 'NONE', #75057, 11.45913725231036118 ) ;
#88112=DIRECTION ( 'NONE',  ( -1.000000000000000078E-15, 1.000000000000000083E-30, 1.000000000000000000 ) ) ;
#88113=CARTESIAN_POINT ( 'NONE',  ( 41.56648329127381203, -27.82844715994070484, 81.92562527591199739 ) ) ;
#88114=ORIENTED_EDGE ( 'NONE', *, *, #64916, .F. ) ;
#88115=ORIENTED_EDGE ( 'NONE', *, *, #19617, .F. ) ;
#88116=PLANE ( 'NONE',  #71351 ) ;
#88120=CARTESIAN_POINT ( 'NONE',  ( 115.0886908286442605, -30.61735931247813625, 104.3439862672049969 ) ) ;
#88122=FACE_OUTER_BOUND ( 'NONE', #1721, .T. ) ;
#88123=VECTOR ( 'NONE', #12634, 999.9999999999998863 ) ;
#88124=VECTOR ( 'NONE', #46514, 1000.000000000000114 ) ;
#88128=CARTESIAN_POINT ( 'NONE',  ( 102.5357197525642192, -45.39752751535328201, 208.1927681330529651 ) ) ;
#88131=CARTESIAN_POINT ( 'NONE',  ( 96.07333748454176714, -35.06730156692550793, 67.20705384733894050 ) ) ;
#88132=CARTESIAN_POINT ( 'NONE',  ( 115.0672684967225479, -42.78377500417700929, 53.31083235052207669 ) ) ;
#88133=DIRECTION ( 'NONE',  ( 0.000000000000000000, 1.000000000000000000, 0.000000000000000000 ) ) ;
#88134=DIRECTION ( 'NONE',  ( -1.346944695195362088E-15, 1.000000000000000000, -3.469446951953620425E-31 ) ) ;
#88135=ORIENTED_EDGE ( 'NONE', *, *, #38969, .T. ) ;
#88137=VECTOR ( 'NONE', #67490, 1000.000000000000114 ) ;
#88138=ORIENTED_EDGE ( 'NONE', *, *, #25897, .T. ) ;
#88139=ORIENTED_EDGE ( 'NONE', *, *, #25806, .T. ) ;
#88140=EDGE_CURVE ( 'NONE', #89690, #54987, #53417, .T. ) ;
#88141=CARTESIAN_POINT ( 'NONE',  ( 112.1951879357659152, -44.60173489647391420, 219.4796785439919802 ) ) ;
#88143=CARTESIAN_POINT ( 'NONE',  ( 97.86646836935159399, -40.64896943459201140, 52.64654800080118235 ) ) ;
#88148=CARTESIAN_POINT ( 'NONE',  ( 69.26949937496598864, -71.54137415153812185, 361.9756252759101471 ) ) ;
#88152=CIRCLE ( 'NONE', #6956, 0.5000000000000007772 ) ;
#88153=EDGE_CURVE ( 'NONE', #12031, #78421, #54911, .T. ) ;
#88154=CARTESIAN_POINT ( 'NONE',  ( 115.0821730991288376, -30.60891592853656817, 35.34399340870037065 ) ) ;
#88155=ORIENTED_EDGE ( 'NONE', *, *, #80064, .F. ) ;
#88156=CARTESIAN_POINT ( 'NONE',  ( 111.4155313275575168, -46.20429869645016652, 27.91848241876792969 ) ) ;
#88157=VERTEX_POINT ( 'NONE', #47958 ) ;
#88158=ORIENTED_EDGE ( 'NONE', *, *, #22683, .F. ) ;
#88159=CARTESIAN_POINT ( 'NONE',  ( 99.00663190570655559, -35.27291570150341471, 239.0023760838769817 ) ) ;
#88160=VECTOR ( 'NONE', #41683, 1000.000000000000000 ) ;
#88162=CARTESIAN_POINT ( 'NONE',  ( 105.8036208730406003, -25.68330614323999228, 160.1670538473399574 ) ) ;
#88164=DIRECTION ( 'NONE',  ( -1.000000000000000000, -3.360405532702990443E-14, 0.000000000000000000 ) ) ;
#88165=AXIS2_PLACEMENT_3D ( 'NONE', #86799, #73149, #30493 ) ;
#88166=LINE ( 'NONE', #47236, #57905 ) ;
#88168=CARTESIAN_POINT ( 'NONE',  ( 118.8391071721064662, -38.46623720595516005, 219.7099109901969882 ) ) ;
#88171=EDGE_CURVE ( 'NONE', #53148, #79585, #75696, .T. ) ;
#88172=VERTEX_POINT ( 'NONE', #6647 ) ;
#88173=CARTESIAN_POINT ( 'NONE',  ( 115.3013748915712711, -44.17149383341634206, 79.25372051400697160 ) ) ;
#88174=DIRECTION ( 'NONE',  ( 0.000000000000000000, 0.000000000000000000, -1.000000000000000000 ) ) ;
#88175=ORIENTED_EDGE ( 'NONE', *, *, #66836, .T. ) ;
#88176=VERTEX_POINT ( 'NONE', #82973 ) ;
#88177=ORIENTED_EDGE ( 'NONE', *, *, #62063, .F. ) ;
#88179=DIRECTION ( 'NONE',  ( 0.000000000000000000, -1.000000000000000000, 0.000000000000000000 ) ) ;
#88181=CARTESIAN_POINT ( 'NONE',  ( 109.6408758491008655, -46.48062444223011624, 152.7819551027729688 ) ) ;
#88182=CARTESIAN_POINT ( 'NONE',  ( 102.2276451341571999, -43.90295244235954897, 149.9099951314959753 ) ) ;
#88183=CARTESIAN_POINT ( 'NONE',  ( 113.8133276556114595, -26.95691720032833416, 235.5956252759109759 ) ) ;
#88185=DIRECTION ( 'NONE',  ( 0.000000000000000000, 1.000000000000000000, 0.000000000000000000 ) ) ;
#88186=ORIENTED_EDGE ( 'NONE', *, *, #6318, .F. ) ;
#88188=LINE ( 'NONE', #24165, #66484 ) ;
#88189=ORIENTED_EDGE ( 'NONE', *, *, #24809, .T. ) ;
#88191=ORIENTED_EDGE ( 'NONE', *, *, #16027, .T. ) ;
#88192=LINE ( 'NONE', #81383, #47411 ) ;
#88194=ORIENTED_EDGE ( 'NONE', *, *, #20668, .F. ) ;
#88195=DIRECTION ( 'NONE',  ( 0.000000000000000000, -1.000000000000000000, 0.000000000000000000 ) ) ;
#88198=CARTESIAN_POINT ( 'NONE',  ( 103.6069473157389922, -44.53891209398362605, 176.6667055423629620 ) ) ;
#88199=CARTESIAN_POINT ( 'NONE',  ( 115.4801557161918311, -43.01927310766588874, 28.31562527591097123 ) ) ;
#88200=ORIENTED_EDGE ( 'NONE', *, *, #13290, .F. ) ;
#88202=EDGE_LOOP ( 'NONE', ( #24538, #36989, #89602, #28542 ) ) ;
#88206=ORIENTED_EDGE ( 'NONE', *, *, #14633, .T. ) ;
#88207=CARTESIAN_POINT ( 'NONE',  ( 100.7142663445133763, -28.97135979089331315, 166.6218790464526194 ) ) ;
#88208=CIRCLE ( 'NONE', #72249, 3.299999999999997158 ) ;
#88210=ADVANCED_FACE ( 'NONE', ( #35236, #29783 ), #63401, .F. ) ;
#88211=CARTESIAN_POINT ( 'NONE',  ( 110.8533328532906665, -45.98470352573126974, 132.8855273142165458 ) ) ;
#88212=AXIS2_PLACEMENT_3D ( 'NONE', #58273, #8351, #63308 ) ;
#88214=ORIENTED_EDGE ( 'NONE', *, *, #60790, .T. ) ;
#88216=CARTESIAN_POINT ( 'NONE',  ( 117.4065409050533617, -38.22262247076111663, 28.71276813305395592 ) ) ;
#88217=CARTESIAN_POINT ( 'NONE',  ( 112.7836381133937067, -27.91740111342080866, 65.61848241876793963 ) ) ;
#88218=LINE ( 'NONE', #47292, #36125 ) ;
#88220=CYLINDRICAL_SURFACE ( 'NONE', #71367, 0.2500000000000046074 ) ;
#88221=DIRECTION ( 'NONE',  ( 0.000000000000000000, 0.000000000000000000, -1.000000000000000000 ) ) ;
#88223=CARTESIAN_POINT ( 'NONE',  ( 99.32888008572089689, -30.27953731386449476, 121.7710324745360566 ) ) ;
#88224=CIRCLE ( 'NONE', #47594, 0.4999999999999933387 ) ;
#88227=ADVANCED_FACE ( 'NONE', ( #36608 ), #43389, .T. ) ;
#88228=CARTESIAN_POINT ( 'NONE',  ( 117.9706719164645250, -41.49678058079525300, 58.49848241876792798 ) ) ;
#88229=CARTESIAN_POINT ( 'NONE',  ( 96.64436219916188975, -36.48069147925158262, 192.3070538473399438 ) ) ;
#88230=CARTESIAN_POINT ( 'NONE',  ( 116.5531001583795216, -32.35436324414348519, 100.1699109901969535 ) ) ;
#88232=CIRCLE ( 'NONE', #5486, 3.250000000000002665 ) ;
#88233=CARTESIAN_POINT ( 'NONE',  ( 113.1798327254349346, -44.75071842742295303, 173.0900461106986086 ) ) ;
#88234=CARTESIAN_POINT ( 'NONE',  ( 118.4837085360594671, -37.70862757085654238, 300.2406250056037038 ) ) ;
#88235=LINE ( 'NONE', #18722, #19035 ) ;
#88236=EDGE_CURVE ( 'NONE', #3377, #1830, #2078, .T. ) ;
#88237=FACE_OUTER_BOUND ( 'NONE', #11529, .T. ) ;
#88239=CARTESIAN_POINT ( 'NONE',  ( 112.1775644307543587, -28.39036538331633963, 90.63848241876793566 ) ) ;
#88242=ORIENTED_EDGE ( 'NONE', *, *, #24672, .F. ) ;
#88243=CARTESIAN_POINT ( 'NONE',  ( 106.5683798796750779, -47.15615894637585370, 243.5384824187679556 ) ) ;
#88244=DIRECTION ( 'NONE',  ( -0.04216478779797398074, 0.9991106698809455455, 0.000000000000000000 ) ) ;
#88245=CARTESIAN_POINT ( 'NONE',  ( 116.3423118429748797, -40.59191411747055156, 148.5122355737231317 ) ) ;
#88247=DIRECTION ( 'NONE',  ( -0.000000000000000000, 1.000000000000000000, 0.000000000000000000 ) ) ;
#88248=CARTESIAN_POINT ( 'NONE',  ( 132.2214349158035418, -38.77077206072119964, 2.188418444516419203 ) ) ;
#88250=CARTESIAN_POINT ( 'NONE',  ( 112.4269750522866502, -44.91043508143939533, 178.0384824187689503 ) ) ;
#88254=VECTOR ( 'NONE', #8361, 1000.000000000000000 ) ;
#88255=CARTESIAN_POINT ( 'NONE',  ( 103.7844689056781675, -44.99325446404193940, 113.7072975916109669 ) ) ;
#88256=DIRECTION ( 'NONE',  ( 0.000000000000000000, 0.000000000000000000, -1.000000000000000000 ) ) ;
#88257=CARTESIAN_POINT ( 'NONE',  ( 97.54182784564409303, -34.36413255805981493, 272.1327681330532755 ) ) ;
#88260=ADVANCED_FACE ( 'NONE', ( #71130 ), #57021, .T. ) ;
#88262=CARTESIAN_POINT ( 'NONE',  ( 107.0664832912739399, -36.72944715994095333, 293.6356252759109680 ) ) ;
#88263=CARTESIAN_POINT ( 'NONE',  ( 188.5667039024484382, -42.82844715993430640, 175.7178068554150343 ) ) ;
#88266=CARTESIAN_POINT ( 'NONE',  ( 115.0229693000241156, -29.09019634776596419, 189.4232443235299570 ) ) ;
#88268=VERTEX_POINT ( 'NONE', #14821 ) ;
#88269=ORIENTED_EDGE ( 'NONE', *, *, #73346, .F. ) ;
#88271=ADVANCED_FACE ( 'NONE', ( #9335 ), #8907, .F. ) ;
#88273=CARTESIAN_POINT ( 'NONE',  ( 78.92334784197174713, -16.22821065591839584, 1.829869330582365228 ) ) ;
#88275=CARTESIAN_POINT ( 'NONE',  ( 172.5664832912740110, -36.32844715994070839, 254.1756252759120400 ) ) ;
#88276=AXIS2_PLACEMENT_3D ( 'NONE', #25432, #44972, #37283 ) ;
#88277=CARTESIAN_POINT ( 'NONE',  ( 163.1543517358360020, -31.62489322948790971, 193.9678068554150059 ) ) ;
#88278=ORIENTED_EDGE ( 'NONE', *, *, #3570, .T. ) ;
#88279=CIRCLE ( 'NONE', #21481, 11.45913725231036118 ) ;
#88280=DIRECTION ( 'NONE',  ( -0.9254794337955620787, -0.3787978585227822492, 0.000000000000000000 ) ) ;
#88281=CARTESIAN_POINT ( 'NONE',  ( 110.2559530472221923, -26.76685766971437630, 234.8299109901969643 ) ) ;
#88282=CARTESIAN_POINT ( 'NONE',  ( 135.3099415725499455, -39.18303583363249487, 7.982915248815769971 ) ) ;
#88283=VERTEX_POINT ( 'NONE', #28892 ) ;
#88284=ADVANCED_FACE ( 'NONE', ( #42489 ), #50658, .T. ) ;
#88285=AXIS2_PLACEMENT_3D ( 'NONE', #13630, #41315, #34512 ) ;
#88287=CARTESIAN_POINT ( 'NONE',  ( 107.0667039024479834, -48.82844715994099971, 160.9178068554150229 ) ) ;
#88289=CARTESIAN_POINT ( 'NONE',  ( 100.8021347340043690, -42.70095134221056554, 34.73856656006796584 ) ) ;
#88290=CIRCLE ( 'NONE', #49088, 3.000000000000002665 ) ;
#88291=CARTESIAN_POINT ( 'NONE',  ( 97.72691728231733066, -42.68408598780226271, 137.7661014663869992 ) ) ;
#88292=DIRECTION ( 'NONE',  ( 0.000000000000000000, 0.000000000000000000, -1.000000000000000000 ) ) ;
#88293=EDGE_LOOP ( 'NONE', ( #23702, #80151, #31703, #48788 ) ) ;
#88294=VECTOR ( 'NONE', #78618, 1000.000000000000000 ) ;
#88295=DIRECTION ( 'NONE',  ( 0.000000000000000000, -1.000000000000000000, 0.000000000000000000 ) ) ;
#88297=EDGE_LOOP ( 'NONE', ( #76345, #24693 ) ) ;
#88298=ORIENTED_EDGE ( 'NONE', *, *, #3051, .F. ) ;
#88300=ORIENTED_EDGE ( 'NONE', *, *, #80669, .T. ) ;
#88303=CARTESIAN_POINT ( 'NONE',  ( 102.2116477823090293, -29.08462914334738869, 64.93718173283896533 ) ) ;
#88304=CARTESIAN_POINT ( 'NONE',  ( 95.38311866650811055, -38.85853310224461410, 201.4699109901969791 ) ) ;
#88305=CARTESIAN_POINT ( 'NONE',  ( 113.6005200848514676, -45.61596423689133672, 183.0689586092439640 ) ) ;
#88306=CARTESIAN_POINT ( 'NONE',  ( 77.31648329127399677, -18.72944715994106346, -5.074374724089059541 ) ) ;
#88307=CARTESIAN_POINT ( 'NONE',  ( 118.3409026158823281, -33.07932318167559060, 280.0756252759109657 ) ) ;
#88310=ORIENTED_EDGE ( 'NONE', *, *, #84507, .T. ) ;
#88315=CARTESIAN_POINT ( 'NONE',  ( 100.6103855434584631, -26.73206753375993827, 220.5327681330539633 ) ) ;
#88317=CARTESIAN_POINT ( 'NONE',  ( 103.3034881226635946, -27.00695273605797908, 215.3699109901969848 ) ) ;
#88318=CARTESIAN_POINT ( 'NONE',  ( 107.0664832912750057, -36.72944715993903486, 9.125625275910969947 ) ) ;
#88319=DIRECTION ( 'NONE',  ( 1.000000000000000000, 0.000000000000000000, -2.089354330573420398E-14 ) ) ;
#88320=ADVANCED_FACE ( 'NONE', ( #48851 ), #69774, .T. ) ;
#88321=CARTESIAN_POINT ( 'NONE',  ( 116.7947957127217222, -39.38901390484394227, 24.61469397140603732 ) ) ;
#88322=CARTESIAN_POINT ( 'NONE',  ( 116.7833380721246641, -34.07052967118504938, 30.03894244259582180 ) ) ;
#88323=CARTESIAN_POINT ( 'NONE',  ( 105.6833081684227835, -28.74817111171022788, 277.6356252759111953 ) ) ;
#88324=DIRECTION ( 'NONE',  ( -0.7071067811987160612, -0.7071067811743789733, 0.000000000000000000 ) ) ;
#88325=CARTESIAN_POINT ( 'NONE',  ( 97.81930885783896201, -40.53600329143382908, 172.6372235601638465 ) ) ;
#88328=DIRECTION ( 'NONE',  ( 0.000000000000000000, 1.000000000000000000, 0.000000000000000000 ) ) ;
#88329=DIRECTION ( 'NONE',  ( 4.299999999999999979E-14, -1.000000000000000000, 4.400000000000000367E-29 ) ) ;
#88330=CARTESIAN_POINT ( 'NONE',  ( 41.56648329127499153, -36.32844715994070839, 194.1756252759119832 ) ) ;
#88332=ORIENTED_EDGE ( 'NONE', *, *, #57495, .F. ) ;
#88333=VECTOR ( 'NONE', #10549, 999.9999999999998863 ) ;
#88334=CARTESIAN_POINT ( 'NONE',  ( 136.8164806451551669, -18.72944715939129523, 6.749772901088581634 ) ) ;
#88335=CARTESIAN_POINT ( 'NONE',  ( 98.88149684619317270, -29.26610755689610599, 230.7261014663869503 ) ) ;
#88336=CARTESIAN_POINT ( 'NONE',  ( 113.3146854497373965, -28.34009065521201265, 100.5670538473389684 ) ) ;
#88337=CARTESIAN_POINT ( 'NONE',  ( 100.1098231460999841, -44.55235322945014076, 262.9984824187678782 ) ) ;
#88339=CARTESIAN_POINT ( 'NONE',  ( 31.85959712127300847, -23.19206098994050436, -5.074374724088000832 ) ) ;
#88340=DIRECTION ( 'NONE',  ( 0.7071067811864677477, 0.7071067811866272868, 7.071067811864671681E-16 ) ) ;
#88343=CARTESIAN_POINT ( 'NONE',  ( 133.4132809338025254, -21.40256188477528099, 1.689562700883915136 ) ) ;
#88345=CIRCLE ( 'NONE', #10010, 4.749999999999976907 ) ;
#88347=ORIENTED_EDGE ( 'NONE', *, *, #71521, .T. ) ;
#88349=CARTESIAN_POINT ( 'NONE',  ( 108.7098619460078481, -45.63517435782368636, 127.1562293518869780 ) ) ;
#88351=DIRECTION ( 'NONE',  ( 0.000000000000000000, 0.000000000000000000, 1.000000000000000000 ) ) ;
#88354=CARTESIAN_POINT ( 'NONE',  ( 95.80265872640110558, -40.33145541733360773, 127.5727681330539554 ) ) ;
#88356=CIRCLE ( 'NONE', #27378, 2.517499999999998739 ) ;
#88358=CARTESIAN_POINT ( 'NONE',  ( 188.5667039024479834, -67.87844715994100397, 142.0928068554150059 ) ) ;
#88359=CARTESIAN_POINT ( 'NONE',  ( 131.3164832912740110, -36.72944715994100306, -5.074374724089004474 ) ) ;
#88360=AXIS2_PLACEMENT_3D ( 'NONE', #80286, #37601, #51649 ) ;
#88361=CARTESIAN_POINT ( 'NONE',  ( 98.84777479348167617, -29.24180311599940651, 80.73848241876795839 ) ) ;
#88363=ORIENTED_EDGE ( 'NONE', *, *, #24559, .F. ) ;
#88366=CARTESIAN_POINT ( 'NONE',  ( 113.7965574739370140, -44.62378898692899298, 149.1508633711479774 ) ) ;
#88370=EDGE_CURVE ( 'NONE', #733, #86726, #58367, .T. ) ;
#88371=CARTESIAN_POINT ( 'NONE',  ( 25.56670390244797275, -67.87844715994100397, 173.2178068554149775 ) ) ;
#88374=CARTESIAN_POINT ( 'NONE',  ( 117.3319688044107920, -38.62265419183311366, 88.68133956162493803 ) ) ;
#88375=ORIENTED_EDGE ( 'NONE', *, *, #27705, .F. ) ;
#88376=ADVANCED_FACE ( 'NONE', ( #31102 ), #30230, .T. ) ;
#88382=CARTESIAN_POINT ( 'NONE',  ( 112.6324121799619462, -43.35677846492738041, 145.9385665600669881 ) ) ;
#88386=CARTESIAN_POINT ( 'NONE',  ( 34.33598329127384829, -36.32844715994141893, 193.9678068554150911 ) ) ;
#88387=ORIENTED_EDGE ( 'NONE', *, *, #83725, .F. ) ;
#88389=ADVANCED_FACE ( 'NONE', ( #17046 ), #46051, .F. ) ;
#88390=CARTESIAN_POINT ( 'NONE',  ( 77.55551418448884249, -19.85480617635147027, 7.067502061099748545 ) ) ;
#88391=CARTESIAN_POINT ( 'NONE',  ( 115.6778139412940192, -34.63821234579798158, 205.4472975916109476 ) ) ;
#88392=CARTESIAN_POINT ( 'NONE',  ( 51.42025729304100423, -33.70561438051981185, -5.074374724088000832 ) ) ;
#88393=CARTESIAN_POINT ( 'NONE',  ( 20.03715912545732891, -24.95799193693189721, 300.4678068554150059 ) ) ;
#88394=AXIS2_PLACEMENT_3D ( 'NONE', #19514, #19971, #47651 ) ;
#88395=ORIENTED_EDGE ( 'NONE', *, *, #10720, .F. ) ;
#88396=AXIS2_PLACEMENT_3D ( 'NONE', #49477, #11166, #66125 ) ;
#88399=VERTEX_POINT ( 'NONE', #72014 ) ;
#88400=ORIENTED_EDGE ( 'NONE', *, *, #82529, .F. ) ;
#88401=CARTESIAN_POINT ( 'NONE',  ( 99.03493788190004921, -39.95360648959476180, 249.4604713219719656 ) ) ;
#88402=VECTOR ( 'NONE', #35269, 1000.000000000000000 ) ;
#88403=CARTESIAN_POINT ( 'NONE',  ( 103.3545649297684577, -47.16578287771347533, 102.3165776568629752 ) ) ;
#88404=CARTESIAN_POINT ( 'NONE',  ( 96.36089708107958529, -41.75325360632975702, 61.67562527591097421 ) ) ;
#88405=CARTESIAN_POINT ( 'NONE',  ( 107.2533376234434570, -45.00125912700468689, 249.5838068554171230 ) ) ;
#88408=MECHANICAL_DESIGN_GEOMETRIC_PRESENTATION_REPRESENTATION('',(#55034),#34769);
#88409=CARTESIAN_POINT ( 'NONE',  ( 101.2007021600770855, -45.34774740814643934, 193.1013395616249682 ) ) ;
#88410=CARTESIAN_POINT ( 'NONE',  ( 107.0664832912739399, -36.72944715994095333, 293.6356252759109680 ) ) ;
#88413=VERTEX_POINT ( 'NONE', #51100 ) ;
#88414=ORIENTED_EDGE ( 'NONE', *, *, #54678, .T. ) ;
#88416=DIRECTION ( 'NONE',  ( 1.000000000000000078E-15, -1.000000000000000083E-30, -1.000000000000000000 ) ) ;
#88417=ORIENTED_EDGE ( 'NONE', *, *, #11007, .F. ) ;
#88420=CARTESIAN_POINT ( 'NONE',  ( 96.03551326368828711, -41.06051932364815826, 96.62419670448197451 ) ) ;
#88422=ADVANCED_FACE ( 'NONE', ( #30668 ), #38363, .F. ) ;
#88423=DIRECTION ( 'NONE',  ( -0.7071067811865192621, -0.7071067811865758834, 2.899137802864845566E-29 ) ) ;
#88425=CARTESIAN_POINT ( 'NONE',  ( 130.0664832912740110, -18.82844715994099971, 284.9256252759119548 ) ) ;
#88427=CARTESIAN_POINT ( 'NONE',  ( 102.2473430764597282, -45.94923854148469644, 208.1927681330539599 ) ) ;
#88430=VERTEX_POINT ( 'NONE', #66063 ) ;
#88431=VECTOR ( 'NONE', #12108, 1000.000000000000000 ) ;
#88432=DIRECTION ( 'NONE',  ( 0.000000000000000000, 1.000000000000000000, 0.000000000000000000 ) ) ;
#88433=CARTESIAN_POINT ( 'NONE',  ( 41.56648329127499153, -27.82844715994070484, 323.6756252759119548 ) ) ;
#88435=CARTESIAN_POINT ( 'NONE',  ( 107.0664832912739399, -36.72944715994095333, 302.7856252759109452 ) ) ;
#88436=CARTESIAN_POINT ( 'NONE',  ( 115.8924960319658055, -44.71257290243538307, 233.2413395616259493 ) ) ;
#88437=VERTEX_POINT ( 'NONE', #4306 ) ;
#88438=CARTESIAN_POINT ( 'NONE',  ( 183.6524903400784012, -49.32844715993451956, 249.9678068554149775 ) ) ;
#88439=CARTESIAN_POINT ( 'NONE',  ( 101.0741685120301412, -45.28686133165523131, 278.0899109901965858 ) ) ;
#88440=CARTESIAN_POINT ( 'NONE',  ( 109.5186955991938191, -46.90685520642291806, 128.7641967044819751 ) ) ;
#88441=DIRECTION ( 'NONE',  ( 0.000000000000000000, 0.000000000000000000, 1.000000000000000000 ) ) ;
#88443=VECTOR ( 'NONE', #84133, 1000.000000000000000 ) ;
#88444=LINE ( 'NONE', #54321, #53524 ) ;
#88445=FACE_OUTER_BOUND ( 'NONE', #71750, .T. ) ;
#88446=CARTESIAN_POINT ( 'NONE',  ( 104.4899545095031925, -26.97880757019963127, 190.2814586045716396 ) ) ;
#88447=LINE ( 'NONE', #69339, #24808 ) ;
#88449=ADVANCED_FACE ( 'NONE', ( #31995 ), #59688, .F. ) ;
#88450=ORIENTED_EDGE ( 'NONE', *, *, #26660, .T. ) ;
#88451=VERTEX_POINT ( 'NONE', #2530 ) ;
#88453=ORIENTED_EDGE ( 'NONE', *, *, #3749, .F. ) ;
#88454=LINE ( 'NONE', #26655, #55414 ) ;
#88455=CARTESIAN_POINT ( 'NONE',  ( 116.7496603916996207, -31.44741115753631178, 20.21181575210195902 ) ) ;
#88456=DIRECTION ( 'NONE',  ( 9.030537910253610117E-13, -1.000000000000000000, 8.600537910253610331E-28 ) ) ;
#88457=AXIS2_PLACEMENT_3D ( 'NONE', #48748, #28788, #34687 ) ;
#88458=CARTESIAN_POINT ( 'NONE',  ( 71.25416588882602298, -72.55705569728901594, 542.9756252759101471 ) ) ;
#88460=DIRECTION ( 'NONE',  ( 0.000000000000000000, 2.135044278125299371E-15, -1.000000000000000000 ) ) ;
#88462=CARTESIAN_POINT ( 'NONE',  ( 100.3746636439974935, -30.62762610928201568, 230.1486103042669811 ) ) ;
#88463=ORIENTED_EDGE ( 'NONE', *, *, #39603, .F. ) ;
#88465=AXIS2_PLACEMENT_3D ( 'NONE', #9373, #42355, #36909 ) ;
#88467=VERTEX_POINT ( 'NONE', #23866 ) ;
#88468=CARTESIAN_POINT ( 'NONE',  ( 97.81169585860149596, -40.51742224678086046, 106.6356332503197137 ) ) ;
#88469=CARTESIAN_POINT ( 'NONE',  ( 97.94027119124240244, -40.81832795154717530, 101.6620931678271376 ) ) ;
#88470=EDGE_CURVE ( 'NONE', #60843, #57623, #11572, .T. ) ;
#88471=DIRECTION ( 'NONE',  ( 0.9068632946707807507, -0.4214249218767880945, 8.673617379884035472E-16 ) ) ;
#88473=CARTESIAN_POINT ( 'NONE',  ( 105.5822692374337777, -27.99308443639166555, 11.64158330589692980 ) ) ;
#88475=AXIS2_PLACEMENT_3D ( 'NONE', #63252, #43236, #37336 ) ;
#88476=DIRECTION ( 'NONE',  ( -2.900000000000000265E-14, 2.000000000000000155E-15, -1.000000000000000000 ) ) ;
#88477=CARTESIAN_POINT ( 'NONE',  ( 117.6440887749188846, -33.30491810902906735, 284.0756252759109657 ) ) ;
#88479=DIRECTION ( 'NONE',  ( 1.000000000000000000, 0.000000000000000000, 0.000000000000000000 ) ) ;
#88480=ORIENTED_EDGE ( 'NONE', *, *, #1399, .T. ) ;
#88482=VECTOR ( 'NONE', #73071, 1000.000000000000000 ) ;
#88483=DIRECTION ( 'NONE',  ( 0.000000000000000000, 0.000000000000000000, 1.000000000000000000 ) ) ;
#88484=CARTESIAN_POINT ( 'NONE',  ( 115.2001725772484662, -37.69162533786680314, 51.55094751244793372 ) ) ;
#88485=FACE_OUTER_BOUND ( 'NONE', #4913, .T. ) ;
#88486=DIRECTION ( 'NONE',  ( -2.999999999999999839E-15, 1.000000000000000000, -2.999999999999999900E-30 ) ) ;
#88489=ORIENTED_EDGE ( 'NONE', *, *, #47667, .F. ) ;
#88491=EDGE_CURVE ( 'NONE', #60263, #10962, #3801, .T. ) ;
#88493=ORIENTED_EDGE ( 'NONE', *, *, #41453, .T. ) ;
#88494=CARTESIAN_POINT ( 'NONE',  ( 108.5379876179846264, -26.40851185940291046, 104.9641967044819779 ) ) ;
#88496=EDGE_CURVE ( 'NONE', #20192, #81785, #21589, .T. ) ;
#88497=CARTESIAN_POINT ( 'NONE',  ( 115.4947688602672997, -38.28382951093581710, 88.10384839950596358 ) ) ;
#88498=ADVANCED_FACE ( 'NONE', ( #41045 ), #76022, .F. ) ;
#88500=CARTESIAN_POINT ( 'NONE',  ( 107.8890265924388814, -27.36996276949999185, 106.4263452106589654 ) ) ;
#88501=CARTESIAN_POINT ( 'NONE',  ( 86.98314995793998605, 12.92155284005730387, 355.9756252759109998 ) ) ;
#88503=CARTESIAN_POINT ( 'NONE',  ( 107.0664832912739968, -36.72944715994100306, 287.6356252759109680 ) ) ;
#88505=CARTESIAN_POINT ( 'NONE',  ( 103.9509101786591287, -47.35857741242491414, 58.33753003781600199 ) ) ;
#88507=CARTESIAN_POINT ( 'NONE',  ( 70.06202783732101125, -36.73691869758536654, 361.9756252759101471 ) ) ;
#88509=CARTESIAN_POINT ( 'NONE',  ( 77.33253953643577461, -19.07457063615845883, 3.076560393663061443 ) ) ;
#88511=ORIENTED_EDGE ( 'NONE', *, *, #80802, .T. ) ;
#88512=CIRCLE ( 'NONE', #58028, 3.000000000000002665 ) ;
#88515=CARTESIAN_POINT ( 'NONE',  ( 115.3604274781777264, -30.50455558986040572, 264.3508633711496714 ) ) ;
#88516=CARTESIAN_POINT ( 'NONE',  ( 96.64920772548965999, -35.94453432339758336, 142.2670538473399517 ) ) ;
#88517=LINE ( 'NONE', #14449, #24888 ) ;
#88518=CARTESIAN_POINT ( 'NONE',  ( 104.4068591371749761, -46.45772509445649234, 128.3646896267844966 ) ) ;
#88519=CARTESIAN_POINT ( 'NONE',  ( 96.63924282488838458, -37.56250720137591514, 97.38991099019594344 ) ) ;
#88520=CARTESIAN_POINT ( 'NONE',  ( 31.89136050872224004, -31.76306994223876501, 313.9678068554150059 ) ) ;
#88522=LINE ( 'NONE', #88069, #48284 ) ;
#88523=AXIS2_PLACEMENT_3D ( 'NONE', #63299, #16057, #617 ) ;
#88524=CARTESIAN_POINT ( 'NONE',  ( 115.0375705353306586, -42.90806541145470732, 159.3021678111343817 ) ) ;
#88525=ORIENTED_EDGE ( 'NONE', *, *, #68524, .F. ) ;
#88526=CIRCLE ( 'NONE', #49340, 2.116999999999993776 ) ;
#88527=CARTESIAN_POINT ( 'NONE',  ( 37.36643805256657913, -48.62818131006120836, 249.9678068554150343 ) ) ;
#88528=CARTESIAN_POINT ( 'NONE',  ( 134.0664832912740110, -8.350947159940998787, 306.1181252759120071 ) ) ;
#88529=CARTESIAN_POINT ( 'NONE',  ( 111.4711666614669099, -26.61707918639087822, 284.7375300378156453 ) ) ;
#88531=LINE ( 'NONE', #60798, #23147 ) ;
#88532=CARTESIAN_POINT ( 'NONE',  ( 77.45242755740703444, -37.60567372264567609, 2.908038864009608648 ) ) ;
#88533=CARTESIAN_POINT ( 'NONE',  ( 106.0094748626272434, -28.25366608065910157, 269.5981341137911613 ) ) ;
#88534=DIRECTION ( 'NONE',  ( 0.000000000000000000, 1.000000000000000000, 1.914177628664063178E-15 ) ) ;
#88535=CARTESIAN_POINT ( 'NONE',  ( 112.7479404651553949, -27.97242311821442584, 65.61848241876793963 ) ) ;
#88536=DIRECTION ( 'NONE',  ( 9.351236661543306751E-17, -3.725950533538267725E-29, -1.000000000000000000 ) ) ;
#88537=CARTESIAN_POINT ( 'NONE',  ( 95.52074050172029729, -39.61468907688732344, 166.5213395616259788 ) ) ;
#88539=CARTESIAN_POINT ( 'NONE',  ( 118.5256205435843100, -36.72944715994100306, 305.0306255462182321 ) ) ;
#88540=VERTEX_POINT ( 'NONE', #46505 ) ;
#88541=VECTOR ( 'NONE', #61892, 1000.000000000000000 ) ;
#88543=DIRECTION ( 'NONE',  ( 0.000000000000000000, 1.000000000000000000, 0.000000000000000000 ) ) ;
#88544=CARTESIAN_POINT ( 'NONE',  ( 188.5667039024479834, -48.82844715994099971, 173.2178068554149775 ) ) ;
#88546=LINE ( 'NONE', #13567, #53424 ) ;
#88547=CARTESIAN_POINT ( 'NONE',  ( 117.1686558484209826, -33.85615284218268073, 149.0470538473389581 ) ) ;
#88548=ORIENTED_EDGE ( 'NONE', *, *, #41004, .F. ) ;
#88549=CARTESIAN_POINT ( 'NONE',  ( 182.2300522401149863, -33.89581943344511217, -5.074374724088000832 ) ) ;
#88551=LINE ( 'NONE', #44160, #11137 ) ;
#88552=LINE ( 'NONE', #34460, #80070 ) ;
#88555=ADVANCED_FACE ( 'NONE', ( #68321 ), #81523, .F. ) ;
#88556=DIRECTION ( 'NONE',  ( 0.000000000000000000, 0.000000000000000000, -1.000000000000000000 ) ) ;
#88557=ORIENTED_EDGE ( 'NONE', *, *, #71219, .T. ) ;
#88558=CIRCLE ( 'NONE', #49362, 3.000000000000002665 ) ;
#88560=EDGE_LOOP ( 'NONE', ( #77430, #11218, #59505, #27958, #30041, #7608 ) ) ;
#88561=PLANE ( 'NONE',  #24968 ) ;
#88564=DIRECTION ( 'NONE',  ( 0.000000000000000000, 0.000000000000000000, -1.000000000000000000 ) ) ;
#88566=EDGE_CURVE ( 'NONE', #82149, #41571, #46295, .T. ) ;
#88567=DIRECTION ( 'NONE',  ( 1.000000000000000078E-15, -1.000000000000000000, 0.000000000000000000 ) ) ;
#88568=CYLINDRICAL_SURFACE ( 'NONE', #47132, 9.999999999999998224 ) ;
#88569=DIRECTION ( 'NONE',  ( 9.032638163712999905E-13, -1.000000000000000000, 1.217258424823508649E-28 ) ) ;
#88570=VECTOR ( 'NONE', #31713, 1000.000000000000000 ) ;
#88571=ADVANCED_FACE ( 'NONE', ( #20175 ), #33345, .F. ) ;
#88572=VERTEX_POINT ( 'NONE', #88330 ) ;
#88573=CARTESIAN_POINT ( 'NONE',  ( 34.67381068360400320, -28.98061976758901892, -5.074374724088000832 ) ) ;
#88575=CARTESIAN_POINT ( 'NONE',  ( 116.7732407090125690, -35.28285290846963562, 214.9441967044819819 ) ) ;
#88577=ORIENTED_EDGE ( 'NONE', *, *, #14837, .F. ) ;
#88578=CARTESIAN_POINT ( 'NONE',  ( 98.34688518126465340, -32.29864090244033292, 46.95276813305293473 ) ) ;
#88579=EDGE_CURVE ( 'NONE', #69807, #88931, #74680, .T. ) ;
#88580=CARTESIAN_POINT ( 'NONE',  ( 133.5842039024480243, -43.72944715994092491, 231.5838068554170093 ) ) ;
#88581=FACE_OUTER_BOUND ( 'NONE', #23676, .T. ) ;
#88587=ORIENTED_EDGE ( 'NONE', *, *, #36633, .T. ) ;
#88588=CARTESIAN_POINT ( 'NONE',  ( 98.31940232332729579, -40.15947632561638869, 243.0434880678019738 ) ) ;
#88589=VECTOR ( 'NONE', #20941, 1000.000000000000000 ) ;
#88590=DIRECTION ( 'NONE',  ( 1.000000000000000078E-15, -1.000000000000000083E-30, -1.000000000000000000 ) ) ;
#88592=CARTESIAN_POINT ( 'NONE',  ( 98.30753412158296101, -41.72887537170915095, 152.7397919317029960 ) ) ;
#88594=CARTESIAN_POINT ( 'NONE',  ( 107.0664832912739968, -36.72944715994100306, 287.6356252759109680 ) ) ;
#88595=ORIENTED_EDGE ( 'NONE', *, *, #45188, .T. ) ;
#88597=ADVANCED_FACE ( 'NONE', ( #64195 ), #69212, .F. ) ;
#88598=DIRECTION ( 'NONE',  ( 0.000000000000000000, 0.000000000000000000, -1.000000000000000000 ) ) ;
#88599=ORIENTED_EDGE ( 'NONE', *, *, #87419, .F. ) ;
#88600=CARTESIAN_POINT ( 'NONE',  ( 96.65879732087768161, -33.00665786158104709, 26.06514908543494613 ) ) ;
#88604=CARTESIAN_POINT ( 'NONE',  ( 109.9373871219287082, -28.56496087843131448, 252.6376141791152747 ) ) ;
#88606=FACE_BOUND ( 'NONE', #81765, .T. ) ;
#88607=CARTESIAN_POINT ( 'NONE',  ( 99.36405074150913208, -30.70139697576582805, 155.7984824187689412 ) ) ;
#88610=DIRECTION ( 'NONE',  ( 0.000000000000000000, 0.000000000000000000, 1.000000000000000000 ) ) ;
#88611=EDGE_CURVE ( 'NONE', #29809, #1463, #21523, .T. ) ;
#88612=LINE ( 'NONE', #54487, #21840 ) ;
#88613=CARTESIAN_POINT ( 'NONE',  ( 105.6260786687505657, -47.09854616955767881, 253.4670538473393719 ) ) ;
#88615=ORIENTED_EDGE ( 'NONE', *, *, #12240, .T. ) ;
#88616=CARTESIAN_POINT ( 'NONE',  ( 98.82360578189442890, -43.24043672769812474, 87.85848241876792031 ) ) ;
#88617=LINE ( 'NONE', #10947, #46765 ) ;
#88620=ORIENTED_EDGE ( 'NONE', *, *, #35935, .F. ) ;
#88623=LINE ( 'NONE', #11407, #13768 ) ;
#88624=CARTESIAN_POINT ( 'NONE',  ( 167.2371591254545535, -47.82818131005522133, 117.4678068554150485 ) ) ;
#88625=LINE ( 'NONE', #25, #4075 ) ;
#88627=CARTESIAN_POINT ( 'NONE',  ( 107.5257129551532813, -44.87112140103544533, 150.4395189410199407 ) ) ;
#88628=CARTESIAN_POINT ( 'NONE',  ( 96.95773401446056994, -39.36581715674629578, 272.5299109901966972 ) ) ;
#88629=CARTESIAN_POINT ( 'NONE',  ( 126.0667039024479266, -14.72944715994094977, 239.5838068554170377 ) ) ;
#88632=FACE_OUTER_BOUND ( 'NONE', #16096, .T. ) ;
#88633=AXIS2_PLACEMENT_3D ( 'NONE', #86927, #17870, #51049 ) ;
#88634=ORIENTED_EDGE ( 'NONE', *, *, #21602, .T. ) ;
#88635=ORIENTED_EDGE ( 'NONE', *, *, #41069, .T. ) ;
#88636=VECTOR ( 'NONE', #12763, 1000.000000000000000 ) ;
#88637=CARTESIAN_POINT ( 'NONE',  ( 180.1667039024473809, -26.71338133338667831, 313.9678068554149490 ) ) ;
#88638=ORIENTED_EDGE ( 'NONE', *, *, #27135, .T. ) ;
#88639=VERTEX_POINT ( 'NONE', #34678 ) ;
#88640=LINE ( 'NONE', #26396, #62888 ) ;
#88642=CARTESIAN_POINT ( 'NONE',  ( 130.5667039024482960, -36.72944715994102438, 249.5838068554162987 ) ) ;
#88644=CARTESIAN_POINT ( 'NONE',  ( 100.5405518937255209, -43.91836718856000488, 156.4124198280769917 ) ) ;
#88645=CARTESIAN_POINT ( 'NONE',  ( 112.9881877051661263, -28.09578728253486446, 44.59848241876795782 ) ) ;
#88650=AXIS2_PLACEMENT_3D ( 'NONE', #49349, #7139, #62541 ) ;
#88651=DIRECTION ( 'NONE',  ( 0.000000000000000000, -1.000000000000000000, 0.000000000000000000 ) ) ;
#88652=ORIENTED_EDGE ( 'NONE', *, *, #30399, .F. ) ;
#88655=CARTESIAN_POINT ( 'NONE',  ( 100.8871001369827809, -44.69991734071174250, 132.0523233816342952 ) ) ;
#88657=DIRECTION ( 'NONE',  ( -1.000000000000000078E-15, 0.000000000000000000, -1.000000000000000000 ) ) ;
#88659=CARTESIAN_POINT ( 'NONE',  ( 96.56351739100374232, -40.17746103522156176, 286.5908633711491120 ) ) ;
#88660=CARTESIAN_POINT ( 'NONE',  ( 107.3220933465437810, -25.63295393647281628, 71.04610146638795243 ) ) ;
#88661=EDGE_CURVE ( 'NONE', #38273, #7861, #7432, .T. ) ;
#88662=CARTESIAN_POINT ( 'NONE',  ( 107.0664832912750057, -36.72944715993903486, 9.125625275910969947 ) ) ;
#88664=CARTESIAN_POINT ( 'NONE',  ( 97.07207306401238611, -35.37843331541325398, 147.2194715753597904 ) ) ;
#88665=ADVANCED_FACE ( 'NONE', ( #62387 ), #43277, .F. ) ;
#88666=DIRECTION ( 'NONE',  ( 1.000000000000000078E-15, -1.000000000000000083E-30, -1.000000000000000000 ) ) ;
#88667=AXIS2_PLACEMENT_3D ( 'NONE', #26275, #47592, #75327 ) ;
#88668=EDGE_CURVE ( 'NONE', #34865, #62712, #41482, .T. ) ;
#88669=CARTESIAN_POINT ( 'NONE',  ( 107.0667039024482818, -36.72944715994102438, 249.5838068554170093 ) ) ;
#88672=DIRECTION ( 'NONE',  ( -1.000000000000000000, -4.299999999999999979E-14, -9.351236661543306751E-17 ) ) ;
#88675=CARTESIAN_POINT ( 'NONE',  ( 118.1298445534695531, -37.63217702543061449, 38.77372051400595865 ) ) ;
#88676=CARTESIAN_POINT ( 'NONE',  ( 109.9169591795599388, -46.81676508990216234, 68.79562527591099297 ) ) ;
#88677=DIRECTION ( 'NONE',  ( -0.9963424814100663163, 0.08544974978097671925, 0.000000000000000000 ) ) ;
#88682=ORIENTED_EDGE ( 'NONE', *, *, #43889, .T. ) ;
#88684=CARTESIAN_POINT ( 'NONE',  ( 116.7039036015865037, -32.90075090702275418, 95.13943479971997874 ) ) ;
#88685=CARTESIAN_POINT ( 'NONE',  ( 41.56648329127398966, -27.57844715994070484, 321.9256252759120116 ) ) ;
#88686=ORIENTED_EDGE ( 'NONE', *, *, #81317, .T. ) ;
#88687=CIRCLE ( 'NONE', #78520, 15.69999999999999929 ) ;
#88688=CARTESIAN_POINT ( 'NONE',  ( 118.7655994573050577, -38.45539276985793720, 219.7099109901969882 ) ) ;
#88691=DIRECTION ( 'NONE',  ( 0.000000000000000000, 1.000000000000000000, 0.000000000000000000 ) ) ;
#88692=CARTESIAN_POINT ( 'NONE',  ( 113.2454987024005106, -28.75867294838092647, 80.55229194212900268 ) ) ;
#88693=EDGE_CURVE ( 'NONE', #33706, #75087, #15603, .T. ) ;
#88694=CARTESIAN_POINT ( 'NONE',  ( 132.8008218761673902, -39.17731672736219650, 1.873071027760403240 ) ) ;
#88696=CARTESIAN_POINT ( 'NONE',  ( 109.2982854457139581, -26.60236246699145113, 179.8918157521019339 ) ) ;
#88697=EDGE_LOOP ( 'NONE', ( #39266, #85417 ) ) ;
#88698=VECTOR ( 'NONE', #73559, 1000.000000000000114 ) ;
#88699=ORIENTED_EDGE ( 'NONE', *, *, #67549, .T. ) ;
#88700=CARTESIAN_POINT ( 'NONE',  ( 99.59846494627726088, -31.90336481815605296, 142.3015833058969974 ) ) ;
#88701=VECTOR ( 'NONE', #71204, 1000.000000000000000 ) ;
#88702=DIRECTION ( 'NONE',  ( 0.000000000000000000, 0.000000000000000000, 1.000000000000000000 ) ) ;
#88703=CARTESIAN_POINT ( 'NONE',  ( 112.3177584634462534, -44.98096486020153151, 259.0270538473389479 ) ) ;
#88704=CARTESIAN_POINT ( 'NONE',  ( 181.9694315774059987, -34.03355364505895864, 237.4678068554150059 ) ) ;
#88706=CARTESIAN_POINT ( 'NONE',  ( 135.9998166246059839, 12.92155284005730387, 358.9756252759109998 ) ) ;
#88707=DIRECTION ( 'NONE',  ( 0.000000000000000000, 0.000000000000000000, -1.000000000000000000 ) ) ;
#88708=CYLINDRICAL_SURFACE ( 'NONE', #27545, 2.750000000000002665 ) ;
#88710=CARTESIAN_POINT ( 'NONE',  ( 96.07698540226623152, -35.78353028925530310, 186.2461014663869889 ) ) ;
#88711=LINE ( 'NONE', #89601, #85199 ) ;
#88713=ORIENTED_EDGE ( 'NONE', *, *, #55087, .F. ) ;
#88714=AXIS2_PLACEMENT_3D ( 'NONE', #53346, #87908, #25670 ) ;
#88715=CARTESIAN_POINT ( 'NONE',  ( 107.0664832912739968, -36.72944715994100306, 287.6356252759109680 ) ) ;
#88716=CARTESIAN_POINT ( 'NONE',  ( 78.76417807489981726, -16.30680158338988761, 1.893168945960760796 ) ) ;
#88717=DIRECTION ( 'NONE',  ( -0.7071067811892205457, 0.7071067811838745998, -7.071067811892213774E-16 ) ) ;
#88718=CARTESIAN_POINT ( 'NONE',  ( 105.7809510460201210, -24.27257308096163868, 321.6188579224977389 ) ) ;
#88719=EDGE_CURVE ( 'NONE', #58657, #35463, #21699, .T. ) ;
#88721=ORIENTED_EDGE ( 'NONE', *, *, #23143, .F. ) ;
#88722=CARTESIAN_POINT ( 'NONE',  ( 105.7141979885323906, -46.72366441306870399, 62.46885673744021972 ) ) ;
#88723=CARTESIAN_POINT ( 'NONE',  ( 99.08584233156592802, -29.96666100724374715, 215.7670538473399517 ) ) ;
#88724=EDGE_LOOP ( 'NONE', ( #77585, #31492, #36865, #6330, #83555, #67936, #28793, #59283, #72779, #50624, #22039, #35773, #46577, #9518, #46822, #44940, #81337, #55003, #35407, #38635, #45737, #89444, #78842, #35068, #54364, #80576, #33824, #81148, #39578, #5470, #6081, #81201, #32209, #52708, #20447, #11272, #32933, #88910, #65918, #39428, #19239, #78938, #5419, #1682, #11630, #47712, #43896, #77294 ) ) ;
#88727=DIRECTION ( 'NONE',  ( -1.000000000000000000, -4.299999999999999979E-14, -1.000000000000000078E-15 ) ) ;
#88728=CARTESIAN_POINT ( 'NONE',  ( 134.0664828118826506, -39.47944715903992829, 8.225259175038003079 ) ) ;
#88730=CARTESIAN_POINT ( 'NONE',  ( 106.6371065190374452, -28.08557299187883061, 42.94618560768698501 ) ) ;
#88731=CARTESIAN_POINT ( 'NONE',  ( 113.3444227873369243, -45.07958072982976461, 139.0899109901969553 ) ) ;
#88732=LINE ( 'NONE', #26487, #66734 ) ;
#88733=ORIENTED_EDGE ( 'NONE', *, *, #42063, .T. ) ;
#88734=EDGE_CURVE ( 'NONE', #16097, #12031, #72466, .T. ) ;
#88735=DIRECTION ( 'NONE',  ( 1.000000000000000000, 4.299999999999999979E-14, 1.000000000000000078E-15 ) ) ;
#88736=CARTESIAN_POINT ( 'NONE',  ( 97.91842249762910910, -40.76970847486229843, 66.65793780748323627 ) ) ;
#88737=ORIENTED_EDGE ( 'NONE', *, *, #60442, .F. ) ;
#88740=DIRECTION ( 'NONE',  ( 1.000000000000000078E-15, -1.000000000000000083E-30, -1.000000000000000000 ) ) ;
#88741=ORIENTED_EDGE ( 'NONE', *, *, #54718, .T. ) ;
#88742=ORIENTED_EDGE ( 'NONE', *, *, #89515, .T. ) ;
#88743=CARTESIAN_POINT ( 'NONE',  ( 32.15435173583699680, -31.62489322948790971, -5.074374724088000832 ) ) ;
#88744=CARTESIAN_POINT ( 'NONE',  ( 114.0365971503568119, -41.66641429710976752, 52.75813411379098739 ) ) ;
#88745=CARTESIAN_POINT ( 'NONE',  ( 96.99510461011969653, -33.95209312647379818, 251.1127681330538337 ) ) ;
#88747=CARTESIAN_POINT ( 'NONE',  ( 102.9757002774701959, -26.48594595611781344, 175.3908633711489813 ) ) ;
#88748=CARTESIAN_POINT ( 'NONE',  ( 74.56648329127402519, -41.22944715994105991, 4.925625275910938683 ) ) ;
#88749=CARTESIAN_POINT ( 'NONE',  ( 96.68076663292312389, -33.01451620012166899, 22.06514908543494258 ) ) ;
#88750=CYLINDRICAL_SURFACE ( 'NONE', #27460, 0.5000000000000073275 ) ;
#88752=EDGE_LOOP ( 'NONE', ( #923, #20421, #63256, #43668, #12976, #48904, #62622, #73132, #66742, #73127, #84630, #86744, #60084, #24915 ) ) ;
#88753=AXIS2_PLACEMENT_3D ( 'NONE', #51659, #31221, #16718 ) ;
#88755=CARTESIAN_POINT ( 'NONE',  ( 97.86673394820853389, -40.64959261906454202, 111.6470208298959363 ) ) ;
#88756=CARTESIAN_POINT ( 'NONE',  ( 96.81521419041753518, -34.60385362728553815, 216.1641967044819808 ) ) ;
#88758=CARTESIAN_POINT ( 'NONE',  ( 109.6058900474308757, -26.58167301968400764, 199.8813395616249977 ) ) ;
#88759=CARTESIAN_POINT ( 'NONE',  ( 63.03715912545735023, -24.42818131006017879, 249.9678068554150343 ) ) ;
#88761=LINE ( 'NONE', #5643, #74020 ) ;
#88762=LINE ( 'NONE', #82851, #67374 ) ;
#88764=CARTESIAN_POINT ( 'NONE',  ( 98.99084639576925326, -33.78646765538439922, 277.6356252759111385 ) ) ;
#88765=CARTESIAN_POINT ( 'NONE',  ( 172.5664832912729878, -27.82844715994070484, 18.92562527591200094 ) ) ;
#88766=DIRECTION ( 'NONE',  ( 0.000000000000000000, 1.000000000000000000, 0.000000000000000000 ) ) ;
#88768=FACE_OUTER_BOUND ( 'NONE', #47973, .T. ) ;
#88770=ADVANCED_FACE ( 'NONE', ( #70561 ), #8333, .T. ) ;
#88771=DIRECTION ( 'NONE',  ( 0.000000000000000000, 0.000000000000000000, 1.000000000000000000 ) ) ;
#88772=LINE ( 'NONE', #55543, #63364 ) ;
#88774=AXIS2_PLACEMENT_3D ( 'NONE', #6791, #62203, #34491 ) ;
#88776=ORIENTED_EDGE ( 'NONE', *, *, #14038, .F. ) ;
#88777=EDGE_CURVE ( 'NONE', #47693, #49134, #50092, .T. ) ;
#88779=CARTESIAN_POINT ( 'NONE',  ( 115.4056828889858650, -30.43626719779562251, 219.3413395616249773 ) ) ;
#88780=CARTESIAN_POINT ( 'NONE',  ( 117.8753414029365842, -39.04084647772175032, 104.6708633711489824 ) ) ;
#88781=CARTESIAN_POINT ( 'NONE',  ( 96.72029611048706954, -35.13276604965626859, 262.2041967044821149 ) ) ;
#88783=CARTESIAN_POINT ( 'NONE',  ( 131.0667039024480118, -58.72944715994093912, 210.8338068554149913 ) ) ;
#88785=CARTESIAN_POINT ( 'NONE',  ( 89.06648138392553449, -56.72944715994104570, -4.824374724089047106 ) ) ;
#88786=LINE ( 'NONE', #47862, #21903 ) ;
#88787=CIRCLE ( 'NONE', #68479, 1.000000000000000888 ) ;
#88788=CARTESIAN_POINT ( 'NONE',  ( 131.8552587341735318, -20.37463194332409699, 2.472581811075852176 ) ) ;
#88789=EDGE_CURVE ( 'NONE', #38331, #15124, #80480, .T. ) ;
#88790=CIRCLE ( 'NONE', #13429, 2.116999999999993776 ) ;
#88792=ORIENTED_EDGE ( 'NONE', *, *, #61668, .F. ) ;
#88793=ADVANCED_FACE ( 'NONE', ( #65524 ), #16936, .T. ) ;
#88794=AXIS2_PLACEMENT_3D ( 'NONE', #48492, #68081, #81730 ) ;
#88795=CARTESIAN_POINT ( 'NONE',  ( 103.4870123794286059, -45.04810440550495798, 136.6876579233149300 ) ) ;
#88797=ORIENTED_EDGE ( 'NONE', *, *, #61403, .F. ) ;
#88798=CARTESIAN_POINT ( 'NONE',  ( 112.1392171050070345, -28.01274908269051167, 89.65543061173896433 ) ) ;
#88799=CARTESIAN_POINT ( 'NONE',  ( 109.1969564574039282, -26.54663071456431211, 135.9127681330539872 ) ) ;
#88800=CARTESIAN_POINT ( 'NONE',  ( 162.9033555647770015, -33.89581943344391135, -5.074374724088000832 ) ) ;
#88803=CARTESIAN_POINT ( 'NONE',  ( 48.86082318535673608, -35.55794170701784651, 313.9678068554150059 ) ) ;
#88805=LINE ( 'NONE', #38838, #33826 ) ;
#88806=CARTESIAN_POINT ( 'NONE',  ( 116.1466984671188385, -33.09446055034462120, 54.12991099019798469 ) ) ;
#88808=ORIENTED_EDGE ( 'NONE', *, *, #52291, .F. ) ;
#88809=ORIENTED_EDGE ( 'NONE', *, *, #28511, .F. ) ;
#88811=CARTESIAN_POINT ( 'NONE',  ( 96.59955023297828802, -32.98040794253982000, 172.0527681330529788 ) ) ;
#88812=CARTESIAN_POINT ( 'NONE',  ( 143.9834832912729894, -1.929447159941392931, 361.9756252759109998 ) ) ;
#88813=CARTESIAN_POINT ( 'NONE',  ( 150.5667039024475571, -25.42844715993593852, 180.4678068554149775 ) ) ;
#88815=CYLINDRICAL_SURFACE ( 'NONE', #61942, 11.45913725231036118 ) ;
#88816=DIRECTION ( 'NONE',  ( 1.000000000000000000, 0.000000000000000000, 0.000000000000000000 ) ) ;
#88817=CARTESIAN_POINT ( 'NONE',  ( 41.56648329127398966, -18.82844715994071194, 255.9256252759120684 ) ) ;
#88818=CARTESIAN_POINT ( 'NONE',  ( 111.0741232671659304, -25.60348521778444209, 99.80133956162498521 ) ) ;
#88819=ORIENTED_EDGE ( 'NONE', *, *, #28672, .T. ) ;
#88821=ORIENTED_EDGE ( 'NONE', *, *, #6909, .F. ) ;
#88822=CARTESIAN_POINT ( 'NONE',  ( 49.35031423293201414, -29.99615139349890569, -5.074374724088000832 ) ) ;
#88823=FACE_OUTER_BOUND ( 'NONE', #78693, .T. ) ;
#88824=AXIS2_PLACEMENT_3D ( 'NONE', #48408, #54775, #61168 ) ;
#88827=CARTESIAN_POINT ( 'NONE',  ( 100.4889591185686015, -31.84898980388015843, 178.6366617981629474 ) ) ;
#88830=CARTESIAN_POINT ( 'NONE',  ( 41.56648329127398966, -27.82844715994070484, 254.1756252759120400 ) ) ;
#88831=ORIENTED_EDGE ( 'NONE', *, *, #64256, .T. ) ;
#88833=ORIENTED_EDGE ( 'NONE', *, *, #9850, .T. ) ;
#88835=DIRECTION ( 'NONE',  ( 5.512527431108029424E-15, -1.000000000000000000, 0.000000000000000000 ) ) ;
#88836=ORIENTED_EDGE ( 'NONE', *, *, #8151, .T. ) ;
#88837=EDGE_LOOP ( 'NONE', ( #50351, #71542, #78533, #18598 ) ) ;
#88839=AXIS2_PLACEMENT_3D ( 'NONE', #45218, #80222, #86140 ) ;
#88840=CARTESIAN_POINT ( 'NONE',  ( 110.1519232268686181, -46.31854332990749867, 204.2558690201829847 ) ) ;
#88841=CARTESIAN_POINT ( 'NONE',  ( 25.56670390244797275, -48.82844715994099971, 295.9678068554150059 ) ) ;
#88842=DIRECTION ( 'NONE',  ( 1.000000000000000078E-15, -1.000000000000000000, 0.000000000000000000 ) ) ;
#88849=ORIENTED_EDGE ( 'NONE', *, *, #59032, .T. ) ;
#88850=VECTOR ( 'NONE', #17916, 1000.000000000000000 ) ;
#88851=CARTESIAN_POINT ( 'NONE',  ( 107.4137727038933150, -44.88475929872373626, 235.4280903695919562 ) ) ;
#88852=CARTESIAN_POINT ( 'NONE',  ( 114.7236970816665860, -44.73335358772728654, 113.1718157521009687 ) ) ;
#88853=CARTESIAN_POINT ( 'NONE',  ( 96.10063762778146668, -37.91858611869022866, 81.40038718067299328 ) ) ;
#88854=CARTESIAN_POINT ( 'NONE',  ( 105.4761177374140999, -44.76735112088204005, 249.5838068554172082 ) ) ;
#88855=CARTESIAN_POINT ( 'NONE',  ( 131.8552587341665969, -17.08426237657134905, 7.378668740739960263 ) ) ;
#88856=CARTESIAN_POINT ( 'NONE',  ( 31.71315051186898870, -31.94127993907790852, 313.9678068554150059 ) ) ;
#88857=CARTESIAN_POINT ( 'NONE',  ( 113.6855667929701923, -45.58166236755234024, 184.0994347997199725 ) ) ;
#88858=CARTESIAN_POINT ( 'NONE',  ( 102.6998691488477249, -45.78651595893203563, 277.2188344857675020 ) ) ;
#88859=ORIENTED_EDGE ( 'NONE', *, *, #15240, .F. ) ;
#88861=ORIENTED_EDGE ( 'NONE', *, *, #78519, .F. ) ;
#88862=VERTEX_POINT ( 'NONE', #72350 ) ;
#88865=DIRECTION ( 'NONE',  ( -1.000000000000000078E-15, 1.000000000000000083E-30, 1.000000000000000000 ) ) ;
#88866=CARTESIAN_POINT ( 'NONE',  ( 113.2424586320066169, -28.75634830710533407, 90.55259365063709254 ) ) ;
#88867=CARTESIAN_POINT ( 'NONE',  ( 103.3623838164489541, -47.14379949381606849, 102.3165776568629752 ) ) ;
#88869=CARTESIAN_POINT ( 'NONE',  ( 136.7978637535026678, -36.40984252624616602, 6.777538624683693058 ) ) ;
#88873=CARTESIAN_POINT ( 'NONE',  ( 115.4997179687694171, -29.61999039777962039, 220.3718157521019521 ) ) ;
#88874=CARTESIAN_POINT ( 'NONE',  ( 107.0667039024479834, -48.82844715994099971, 160.9178068554150229 ) ) ;
#88876=LINE ( 'NONE', #53411, #81600 ) ;
#88878=DIRECTION ( 'NONE',  ( 1.000000000000000078E-15, -1.000000000000000083E-30, -1.000000000000000000 ) ) ;
#88879=VECTOR ( 'NONE', #34822, 1000.000000000000000 ) ;
#88881=DIRECTION ( 'NONE',  ( 0.7071067811861728725, -0.7071067811869222730, 0.000000000000000000 ) ) ;
#88882=ADVANCED_FACE ( 'NONE', ( #52300 ), #69961, .T. ) ;
#88883=CARTESIAN_POINT ( 'NONE',  ( 126.8164832912740394, -46.47944715994101017, -5.074374724089010691 ) ) ;
#88884=CYLINDRICAL_SURFACE ( 'NONE', #53483, 0.5000000000000172085 ) ;
#88885=CARTESIAN_POINT ( 'NONE',  ( 101.2695147780440266, -26.33598991146258328, 255.4813395616251626 ) ) ;
#88887=EDGE_CURVE ( 'NONE', #79111, #41648, #15933, .T. ) ;
#88889=CARTESIAN_POINT ( 'NONE',  ( 116.4744410436840383, -32.23804052137624865, 15.18133956162492915 ) ) ;
#88890=CARTESIAN_POINT ( 'NONE',  ( 98.13109353019112291, -31.27492705589930821, 166.8899109901969950 ) ) ;
#88891=DIRECTION ( 'NONE',  ( 1.000000000000000078E-15, 0.000000000000000000, -1.000000000000000000 ) ) ;
#88892=CARTESIAN_POINT ( 'NONE',  ( 97.07207337491342969, -35.37841122429128404, 102.2188882665558083 ) ) ;
#88894=CYLINDRICAL_SURFACE ( 'NONE', #76206, 9.999999999999998224 ) ;
#88895=PLANE ( 'NONE',  #45210 ) ;
#88896=CARTESIAN_POINT ( 'NONE',  ( 20.03715912545820288, -46.82818131006190043, 300.4678068554150059 ) ) ;
#88897=ORIENTED_EDGE ( 'NONE', *, *, #41219, .T. ) ;
#88898=VECTOR ( 'NONE', #52253, 1000.000000000000000 ) ;
#88903=DIRECTION ( 'NONE',  ( 0.000000000000000000, 1.000000000000000000, 0.000000000000000000 ) ) ;
#88904=CARTESIAN_POINT ( 'NONE',  ( 118.0600790064083299, -37.62648441163795354, 34.77372051400695341 ) ) ;
#88906=CARTESIAN_POINT ( 'NONE',  ( 71.24189083761808661, -0.9290567490904538817, 394.9756252759101471 ) ) ;
#88908=CARTESIAN_POINT ( 'NONE',  ( 98.42407572851979580, -32.30458340910843162, 245.3724198280769428 ) ) ;
#88909=ORIENTED_EDGE ( 'NONE', *, *, #56847, .T. ) ;
#88910=ORIENTED_EDGE ( 'NONE', *, *, #82632, .F. ) ;
#88911=ORIENTED_EDGE ( 'NONE', *, *, #7044, .T. ) ;
#88912=AXIS2_PLACEMENT_3D ( 'NONE', #11780, #41248, #19936 ) ;
#88913=LINE ( 'NONE', #33928, #45635 ) ;
#88914=CARTESIAN_POINT ( 'NONE',  ( 98.54785118950427147, -41.97730404426498296, 101.7661766900147597 ) ) ;
#88915=CARTESIAN_POINT ( 'NONE',  ( 107.0664832912739541, -20.72944715994095333, 311.3356252759109566 ) ) ;
#88916=DIRECTION ( 'NONE',  ( 1.000000000000000078E-15, 0.000000000000000000, 1.000000000000000000 ) ) ;
#88920=CARTESIAN_POINT ( 'NONE',  ( 112.0813997088635858, -45.80630777137071874, 252.9661014663878689 ) ) ;
#88922=ORIENTED_EDGE ( 'NONE', *, *, #41193, .F. ) ;
#88926=CARTESIAN_POINT ( 'NONE',  ( 113.1369140564456615, -42.18651563507969371, 36.06237608387696980 ) ) ;
#88927=CARTESIAN_POINT ( 'NONE',  ( 97.81067182961875517, -40.51494070217739107, 131.6354111825010307 ) ) ;
#88928=EDGE_CURVE ( 'NONE', #82506, #56272, #40545, .T. ) ;
#88930=CARTESIAN_POINT ( 'NONE',  ( 179.8585841295807484, -30.08671355699668126, 193.9678068554150059 ) ) ;
#88931=VERTEX_POINT ( 'NONE', #76769 ) ;
#88932=CARTESIAN_POINT ( 'NONE',  ( 79.69020591997146141, -33.99866847873249043, 8.209451181319794344 ) ) ;
#88933=AXIS2_PLACEMENT_3D ( 'NONE', #77963, #79310, #57946 ) ;
#88935=CARTESIAN_POINT ( 'NONE',  ( 117.2382404677042729, -39.01746902538002360, 148.6499109901969859 ) ) ;
#88937=CARTESIAN_POINT ( 'NONE',  ( 98.71159061831248493, -42.24584867631038065, 87.79035904436562987 ) ) ;
#88938=CARTESIAN_POINT ( 'NONE',  ( 108.6971488411468414, -45.98241724535997577, 119.1349166392299566 ) ) ;
#88941=CARTESIAN_POINT ( 'NONE',  ( 110.8022603587792219, -46.48553390388831019, 58.86705384733998159 ) ) ;
#88942=CARTESIAN_POINT ( 'NONE',  ( 100.9549047852691785, -28.70684421539622377, 181.5944067750197064 ) ) ;
#88943=VECTOR ( 'NONE', #11599, 1000.000000000000000 ) ;
#88945=VERTEX_POINT ( 'NONE', #49491 ) ;
#88946=ADVANCED_FACE ( 'NONE', ( #78136 ), #23178, .T. ) ;
#88947=CARTESIAN_POINT ( 'NONE',  ( 162.7131505118539962, -33.70561438052090608, -5.074374724088000832 ) ) ;
#88948=ORIENTED_EDGE ( 'NONE', *, *, #89482, .F. ) ;
#88951=EDGE_LOOP ( 'NONE', ( #69896, #85870, #82661, #55185 ) ) ;
#88952=CARTESIAN_POINT ( 'NONE',  ( 99.34779341711919187, -29.80408710710932496, 235.7565776568639819 ) ) ;
#88953=CARTESIAN_POINT ( 'NONE',  ( 97.77490566832175034, -42.75910828249967466, 142.7965776568629508 ) ) ;
#88954=CARTESIAN_POINT ( 'NONE',  ( 165.9667039024459996, -28.27351298637401200, 342.9256252759119548 ) ) ;
#88955=LINE ( 'NONE', #82159, #56139 ) ;
#88956=CARTESIAN_POINT ( 'NONE',  ( 109.6838526317122273, -47.46831852615197533, 83.75467289495897205 ) ) ;
#88957=CARTESIAN_POINT ( 'NONE',  ( 115.0918025260861555, -30.62139641523929967, 95.34367351736931084 ) ) ;
#88958=EDGE_LOOP ( 'NONE', ( #32296, #21009, #66950, #26110 ) ) ;
#88959=CARTESIAN_POINT ( 'NONE',  ( 48.79742451362075428, -36.32844715994075813, 313.9678068554150059 ) ) ;
#88960=EDGE_CURVE ( 'NONE', #6301, #82784, #43619, .T. ) ;
#88962=VERTEX_POINT ( 'NONE', #7288 ) ;
#88963=CIRCLE ( 'NONE', #38247, 0.3000000000000016542 ) ;
#88965=CARTESIAN_POINT ( 'NONE',  ( 142.8682495647594521, 8.654319075478440482, 542.9756252759101471 ) ) ;
#88966=CARTESIAN_POINT ( 'NONE',  ( 106.2286657330468103, -47.72771449247521502, 267.5280062282920994 ) ) ;
#88967=DIRECTION ( 'NONE',  ( 0.000000000000000000, 0.000000000000000000, 1.000000000000000000 ) ) ;
#88969=DIRECTION ( 'NONE',  ( 9.351236661543306751E-17, -3.725950533538267725E-29, -1.000000000000000000 ) ) ;
#88970=CARTESIAN_POINT ( 'NONE',  ( 107.0664832912739968, -36.72944715994100306, 287.6356252759109680 ) ) ;
#88971=CARTESIAN_POINT ( 'NONE',  ( 97.32756240343553600, -42.09278592120095652, 26.72705384733997747 ) ) ;
#88972=DIRECTION ( 'NONE',  ( 0.000000000000000000, 0.000000000000000000, -1.000000000000000000 ) ) ;
#88973=CARTESIAN_POINT ( 'NONE',  ( 118.8789388927531974, -36.16900092901214947, 114.8641967044819694 ) ) ;
#88974=DIRECTION ( 'NONE',  ( 2.999999999999999839E-15, -1.000000000000000000, 2.999999999999999900E-30 ) ) ;
#88975=CARTESIAN_POINT ( 'NONE',  ( 117.0653594338693892, -39.95035295773606521, 158.5784824187679476 ) ) ;
#88978=ORIENTED_EDGE ( 'NONE', *, *, #79312, .T. ) ;
#88981=CARTESIAN_POINT ( 'NONE',  ( 135.9759635523953420, -34.74831825237850325, 2.232988539019887142 ) ) ;
#88984=LINE ( 'NONE', #54871, #12820 ) ;
#88985=CARTESIAN_POINT ( 'NONE',  ( 108.7503283313270543, -25.75779200005056779, 144.9432443235299672 ) ) ;
#88986=VERTEX_POINT ( 'NONE', #43575 ) ;
#88987=LINE ( 'NONE', #26746, #65433 ) ;
#88990=DIRECTION ( 'NONE',  ( 0.000000000000000000, 0.000000000000000000, 1.000000000000000000 ) ) ;
#88992=PRODUCT_CONTEXT ( 'NONE', #13854, 'mechanical' ) ;
#88994=ORIENTED_EDGE ( 'NONE', *, *, #33806, .F. ) ;
#88995=VERTEX_POINT ( 'NONE', #71314 ) ;
#88997=EDGE_CURVE ( 'NONE', #66809, #11502, #463, .T. ) ;
#88998=VECTOR ( 'NONE', #9251, 999.9999999999998863 ) ;
#88999=ORIENTED_EDGE ( 'NONE', *, *, #13908, .T. ) ;
#89000=CARTESIAN_POINT ( 'NONE',  ( 163.1639762274590169, -34.03355364505800651, 117.4678068554150485 ) ) ;
#89001=CARTESIAN_POINT ( 'NONE',  ( 104.6691943795874096, -26.96177962471290002, 250.2678212403098712 ) ) ;
#89002=EDGE_CURVE ( 'NONE', #67994, #24090, #63777, .T. ) ;
#89003=DIRECTION ( 'NONE',  ( 0.000000000000000000, 0.000000000000000000, -1.000000000000000000 ) ) ;
#89004=DIRECTION ( 'NONE',  ( -0.7071067811865165975, -0.7071067811865784369, -7.071067811865158803E-16 ) ) ;
#89005=LINE ( 'NONE', #26759, #75543 ) ;
#89006=DIRECTION ( 'NONE',  ( -1.000000000000000078E-15, 0.000000000000000000, 1.000000000000000000 ) ) ;
#89007=CARTESIAN_POINT ( 'NONE',  ( 97.60796736720944011, -39.98265213332607004, 181.5900836763981943 ) ) ;
#89009=ORIENTED_EDGE ( 'NONE', *, *, #4054, .F. ) ;
#89010=CARTESIAN_POINT ( 'NONE',  ( 57.56670390244747892, -48.82844715994040286, 137.2178068554150911 ) ) ;
#89011=CARTESIAN_POINT ( 'NONE',  ( 172.5664832912740110, -32.07844715994070839, 83.67562527591201160 ) ) ;
#89012=CARTESIAN_POINT ( 'NONE',  ( 112.8396959964675972, -44.62460075896464673, 224.0784824187679476 ) ) ;
#89013=LINE ( 'NONE', #54454, #80646 ) ;
#89014=ORIENTED_EDGE ( 'NONE', *, *, #88153, .F. ) ;
#89015=CARTESIAN_POINT ( 'NONE',  ( 96.76615086495803553, -37.93025403122315709, 82.43086337114895912 ) ) ;
#89016=DIRECTION ( 'NONE',  ( 1.000000000000000000, -6.938893903907222067E-14, 0.000000000000000000 ) ) ;
#89018=DIRECTION ( 'NONE',  ( 1.639958061481212836E-42, -4.100000000000000342E-29, -1.000000000000000000 ) ) ;
#89019=ORIENTED_EDGE ( 'NONE', *, *, #24837, .T. ) ;
#89023=CARTESIAN_POINT ( 'NONE',  ( 98.91186986371705814, -40.27407823153063759, 228.0844404487539805 ) ) ;
#89025=CARTESIAN_POINT ( 'NONE',  ( 98.38035888927598194, -41.69516708799280735, 52.73934900735942932 ) ) ;
#89027=AXIS2_PLACEMENT_3D ( 'NONE', #77242, #21380, #42248 ) ;
#89028=EDGE_CURVE ( 'NONE', #68284, #79540, #37718, .T. ) ;
#89029=CARTESIAN_POINT ( 'NONE',  ( 104.4081005625954361, -46.45808911397131169, 153.3647919345398236 ) ) ;
#89031=DIRECTION ( 'NONE',  ( 4.299999999999999979E-14, -1.000000000000000000, 0.000000000000000000 ) ) ;
#89034=LINE ( 'NONE', #26795, #41181 ) ;
#89036=CARTESIAN_POINT ( 'NONE',  ( 110.2841844748215578, -46.64581212076017636, 12.82705384733995402 ) ) ;
#89037=VERTEX_POINT ( 'NONE', #1821 ) ;
#89038=CARTESIAN_POINT ( 'NONE',  ( 115.2289877667042930, -36.78642703073501252, 261.6395189410197872 ) ) ;
#89039=CARTESIAN_POINT ( 'NONE',  ( 41.56648329127398966, -27.82844715994070484, 75.92562527591199739 ) ) ;
#89040=CARTESIAN_POINT ( 'NONE',  ( 108.6395843534182291, -26.47938140272615470, 144.9432443235309904 ) ) ;
#89042=DIRECTION ( 'NONE',  ( 0.000000000000000000, 1.000000000000000000, 0.000000000000000000 ) ) ;
#89043=DIRECTION ( 'NONE',  ( 1.639958061481212836E-42, -4.100000000000000342E-29, -1.000000000000000000 ) ) ;
#89045=CARTESIAN_POINT ( 'NONE',  ( 106.5652502036378593, -47.22167190867460818, 243.5384824187679556 ) ) ;
#89047=ORIENTED_EDGE ( 'NONE', *, *, #4090, .F. ) ;
#89049=CARTESIAN_POINT ( 'NONE',  ( 104.7499416563296961, -46.93859083614567140, 68.39848241876794077 ) ) ;
#89050=EDGE_CURVE ( 'NONE', #73456, #52361, #73942, .T. ) ;
#89052=VECTOR ( 'NONE', #37621, 1000.000000000000000 ) ;
#89053=ORIENTED_EDGE ( 'NONE', *, *, #80773, .F. ) ;
#89056=ORIENTED_EDGE ( 'NONE', *, *, #52291, .T. ) ;
#89057=ADVANCED_FACE ( 'NONE', ( #10409 ), #31286, .F. ) ;
#89058=TOROIDAL_SURFACE ( 'NONE', #13581, 13.50000000000000000, 0.5000000000000000000 ) ;
#89059=CARTESIAN_POINT ( 'NONE',  ( 97.06112134132980884, -37.99667316087749924, 161.4271097635434558 ) ) ;
#89061=PLANE ( 'NONE',  #49440 ) ;
#89062=DIRECTION ( 'NONE',  ( 0.000000000000000000, 0.000000000000000000, 1.000000000000000000 ) ) ;
#89063=CARTESIAN_POINT ( 'NONE',  ( 103.8567473457716375, -28.69212669812176841, 173.2090427505439720 ) ) ;
#89064=CARTESIAN_POINT ( 'NONE',  ( 115.7133342524696360, -42.59197454220085177, 269.3527681330536439 ) ) ;
#89066=DIRECTION ( 'NONE',  ( 0.000000000000000000, 0.000000000000000000, 1.000000000000000000 ) ) ;
#89070=CARTESIAN_POINT ( 'NONE',  ( 131.0667039024480687, -51.22944715994093201, 207.5838068554170377 ) ) ;
#89071=EDGE_LOOP ( 'NONE', ( #6665, #54682, #13004, #36670 ) ) ;
#89073=EDGE_CURVE ( 'NONE', #61623, #75367, #81595, .T. ) ;
#89075=ORIENTED_EDGE ( 'NONE', *, *, #45610, .F. ) ;
#89076=ORIENTED_EDGE ( 'NONE', *, *, #88236, .F. ) ;
#89077=DIRECTION ( 'NONE',  ( 0.9242245927363033076, 0.3818493186865917766, 0.000000000000000000 ) ) ;
#89082=CARTESIAN_POINT ( 'NONE',  ( 98.53214291706959216, -37.07752924029257713, 160.7809912566479511 ) ) ;
#89083=CARTESIAN_POINT ( 'NONE',  ( 112.8421283165351809, -27.25026954951128388, 49.62895860924498947 ) ) ;
#89085=FACE_OUTER_BOUND ( 'NONE', #55282, .T. ) ;
#89086=ORIENTED_EDGE ( 'NONE', *, *, #14063, .F. ) ;
#89088=ADVANCED_FACE ( 'NONE', ( #38549 ), #65375, .F. ) ;
#89091=ORIENTED_EDGE ( 'NONE', *, *, #72210, .T. ) ;
#89092=CARTESIAN_POINT ( 'NONE',  ( 114.2890383888417034, -29.74243919954670190, 165.4383927227787296 ) ) ;
#89094=CYLINDRICAL_SURFACE ( 'NONE', #35931, 3.250000000000002665 ) ;
#89095=VECTOR ( 'NONE', #21519, 1000.000000000000000 ) ;
#89096=CARTESIAN_POINT ( 'NONE',  ( 163.1543517358360020, -31.62489322948790971, 117.4678068554150485 ) ) ;
#89098=CARTESIAN_POINT ( 'NONE',  ( 115.5918606122963439, -42.76801532637115599, 53.33562527591095659 ) ) ;
#89099=CARTESIAN_POINT ( 'NONE',  ( 117.0955297935745705, -31.97384786926005873, 60.19086337114898555 ) ) ;
#89100=VECTOR ( 'NONE', #40919, 1000.000000000000000 ) ;
#89101=CARTESIAN_POINT ( 'NONE',  ( 29.56670390244797630, -67.87844715994100397, 10.91780685541479734 ) ) ;
#89103=CARTESIAN_POINT ( 'NONE',  ( 105.7995310142117660, -26.72403331909748303, 146.1777001516798862 ) ) ;
#89105=ORIENTED_EDGE ( 'NONE', *, *, #53565, .T. ) ;
#89108=ADVANCED_FACE ( 'NONE', ( #37224 ), #64929, .T. ) ;
#89112=EDGE_LOOP ( 'NONE', ( #67937, #14800, #68591, #24083 ) ) ;
#89113=CARTESIAN_POINT ( 'NONE',  ( 112.8137514937528891, -47.12132662887700008, 98.97848241876793907 ) ) ;
#89115=CARTESIAN_POINT ( 'NONE',  ( 97.82528869122914728, -40.55050793170509849, 171.6387267483714254 ) ) ;
#89118=AXIS2_PLACEMENT_3D ( 'NONE', #63453, #76639, #13515 ) ;
#89120=AXIS2_PLACEMENT_3D ( 'NONE', #58379, #30242, #54102 ) ;
#89121=CIRCLE ( 'NONE', #44095, 2.500000000000002220 ) ;
#89123=ORIENTED_EDGE ( 'NONE', *, *, #87467, .F. ) ;
#89124=CARTESIAN_POINT ( 'NONE',  ( 116.4859054502388744, -39.36344060769043551, 94.60991099019594230 ) ) ;
#89126=VERTEX_POINT ( 'NONE', #67938 ) ;
#89127=AXIS2_PLACEMENT_3D ( 'NONE', #63394, #14812, #36598 ) ;
#89129=CARTESIAN_POINT ( 'NONE',  ( 96.29057984255084079, -34.37493501460200207, 252.1432443235302969 ) ) ;
#89130=CARTESIAN_POINT ( 'NONE',  ( 125.9611475301394847, -58.72944715994102438, 249.5838068554163840 ) ) ;
#89131=DIRECTION ( 'NONE',  ( 0.000000000000000000, 1.000000000000000000, 0.000000000000000000 ) ) ;
#89133=CARTESIAN_POINT ( 'NONE',  ( 112.1393456378820446, -28.01282277885371030, 45.65645860958608893 ) ) ;
#89136=CARTESIAN_POINT ( 'NONE',  ( 111.8874393434638250, -45.23954810143646910, 212.9870538473399506 ) ) ;
#89138=EDGE_LOOP ( 'NONE', ( #24576, #64410, #12589, #52602 ) ) ;
#89139=CARTESIAN_POINT ( 'NONE',  ( 103.3528332358002331, -45.35993549251112711, 133.6968214011349403 ) ) ;
#89140=LINE ( 'NONE', #32815, #29856 ) ;
#89141=CARTESIAN_POINT ( 'NONE',  ( 97.44287158780967673, -40.59272077381804422, 247.6422919425769749 ) ) ;
#89143=DIRECTION ( 'NONE',  ( 0.000000000000000000, 0.000000000000000000, -1.000000000000000000 ) ) ;
#89145=CYLINDRICAL_SURFACE ( 'NONE', #21167, 9.999999999999998224 ) ;
#89146=DIRECTION ( 'NONE',  ( -4.237773401492740281E-14, 1.000000000000000000, 0.000000000000000000 ) ) ;
#89147=CARTESIAN_POINT ( 'NONE',  ( 21.03689327557711763, -23.42844715994186089, 249.9678068554150059 ) ) ;
#89148=CARTESIAN_POINT ( 'NONE',  ( 106.9751875180390641, -47.13234726572967759, 187.5699109901969734 ) ) ;
#89150=EDGE_LOOP ( 'NONE', ( #40811, #33744 ) ) ;
#89151=ORIENTED_EDGE ( 'NONE', *, *, #81334, .F. ) ;
#89153=CARTESIAN_POINT ( 'NONE',  ( 81.30994157256897381, -21.18303583361772269, 7.982915248808116537 ) ) ;
#89154=CARTESIAN_POINT ( 'NONE',  ( 116.8164492606990308, -34.15029442158964201, 125.0311193818890416 ) ) ;
#89155=DIRECTION ( 'NONE',  ( 0.000000000000000000, 0.000000000000000000, -1.000000000000000000 ) ) ;
#89159=CARTESIAN_POINT ( 'NONE',  ( 116.3283240494693160, -32.94276334974209419, 64.13562527591099638 ) ) ;
#89160=AXIS2_PLACEMENT_3D ( 'NONE', #86641, #86194, #51647 ) ;
#89161=CARTESIAN_POINT ( 'NONE',  ( 104.1857688441879191, -26.67323559945603151, 225.2984824187679749 ) ) ;
#89162=EDGE_CURVE ( 'NONE', #41446, #88268, #7231, .T. ) ;
#89166=FACE_OUTER_BOUND ( 'NONE', #66123, .T. ) ;
#89168=CARTESIAN_POINT ( 'NONE',  ( 98.93870468184483968, -41.20551083899233902, 24.54523322673496466 ) ) ;
#89169=CARTESIAN_POINT ( 'NONE',  ( 98.83948440537673719, -30.29086274794821065, 151.7984824187679465 ) ) ;
#89171=CARTESIAN_POINT ( 'NONE',  ( 123.6837132603318707, -22.62993780205694705, 219.5838068554170093 ) ) ;
#89172=EDGE_LOOP ( 'NONE', ( #20344, #13255, #89091, #50506 ) ) ;
#89173=ADVANCED_FACE ( 'NONE', ( #54277 ), #44016, .T. ) ;
#89175=CARTESIAN_POINT ( 'NONE',  ( 117.0385479230201327, -38.27385465322490887, 68.70451315128531178 ) ) ;
#89176=ORIENTED_EDGE ( 'NONE', *, *, #8575, .T. ) ;
#89177=ORIENTED_EDGE ( 'NONE', *, *, #63864, .T. ) ;
#89178=ADVANCED_FACE ( 'NONE', ( #23614 ), #51272, .F. ) ;
#89179=AXIS2_PLACEMENT_3D ( 'NONE', #26808, #13197, #39990 ) ;
#89180=VECTOR ( 'NONE', #62739, 999.9999999999998863 ) ;
#89181=FACE_BOUND ( 'NONE', #83424, .T. ) ;
#89182=CIRCLE ( 'NONE', #74648, 0.9999999999992039701 ) ;
#89183=ORIENTED_EDGE ( 'NONE', *, *, #1334, .F. ) ;
#89184=ORIENTED_EDGE ( 'NONE', *, *, #82329, .T. ) ;
#89186=CIRCLE ( 'NONE', #10843, 13.31747058675099815 ) ;
#89188=CARTESIAN_POINT ( 'NONE',  ( 111.7311378220509255, -29.53965576977622831, 69.04099125664797043 ) ) ;
#89189=CIRCLE ( 'NONE', #38402, 4.750000000000000888 ) ;
#89190=CARTESIAN_POINT ( 'NONE',  ( 98.92532678050559980, -30.18208626920050719, 240.7870538473399620 ) ) ;
#89191=AXIS2_PLACEMENT_3D ( 'NONE', #982, #44529, #58608 ) ;
#89192=CARTESIAN_POINT ( 'NONE',  ( 106.3035372762157351, -47.10473409126657174, 222.5184824187679453 ) ) ;
#89193=DIRECTION ( 'NONE',  ( 0.000000000000000000, 1.000000000000000000, 0.000000000000000000 ) ) ;
#89194=CARTESIAN_POINT ( 'NONE',  ( 96.56373827543593791, -40.17738982329606046, 282.5908633711490552 ) ) ;
#89195=DIRECTION ( 'NONE',  ( -4.237773401492740281E-14, 1.000000000000000000, 0.000000000000000000 ) ) ;
#89196=CARTESIAN_POINT ( 'NONE',  ( 57.56670390244747892, -48.82844715994040286, 137.2178068554150911 ) ) ;
#89197=EDGE_CURVE ( 'NONE', #3936, #52361, #85577, .T. ) ;
#89199=ADVANCED_FACE ( 'NONE', ( #69740 ), #34760, .T. ) ;
#89200=CARTESIAN_POINT ( 'NONE',  ( 103.5913876162975527, -46.49993820617282125, 102.3165776568639700 ) ) ;
#89201=CARTESIAN_POINT ( 'NONE',  ( 118.8926602832294037, -35.39890769255473657, 83.91562527591095488 ) ) ;
#89202=CARTESIAN_POINT ( 'NONE',  ( 96.87130625142565066, -34.19761792387945576, 276.1327681330536734 ) ) ;
#89204=CARTESIAN_POINT ( 'NONE',  ( 117.0684261367714072, -39.67022423017687771, 183.5984824187679578 ) ) ;
#89205=CARTESIAN_POINT ( 'NONE',  ( 115.8254323898935496, -31.73001882380996364, 34.23979194300372342 ) ) ;
#89206=CARTESIAN_POINT ( 'NONE',  ( 165.3359832912740046, -36.32844715994100682, 342.9256252759109884 ) ) ;
#89207=CARTESIAN_POINT ( 'NONE',  ( 141.0664832912740394, -46.72944715994099596, -4.824374724088994704 ) ) ;
#89208=CARTESIAN_POINT ( 'NONE',  ( 104.8437968989451861, -46.57283331671013116, 28.40163825079190474 ) ) ;
#89209=AXIS2_PLACEMENT_3D ( 'NONE', #88318, #13345, #41032 ) ;
#89210=CARTESIAN_POINT ( 'NONE',  ( 110.4749035026220554, -45.11497559619134279, 277.6356252759110816 ) ) ;
#89212=CARTESIAN_POINT ( 'NONE',  ( 115.0371819524543326, -42.90856332754897551, 174.3022820718215655 ) ) ;
#89213=DIRECTION ( 'NONE',  ( 0.03970846417641692161, -0.4987692715698832657, 0.8658247233767341067 ) ) ;
#89216=DIRECTION ( 'NONE',  ( -1.000000000000000000, 0.000000000000000000, -9.974659986866630932E-16 ) ) ;
#89217=CARTESIAN_POINT ( 'NONE',  ( 51.06648329127400388, 22.62155284005901024, 327.8006252759110453 ) ) ;
#89218=CARTESIAN_POINT ( 'NONE',  ( 109.7248659271630800, -27.00080518147012043, 75.86479194210151888 ) ) ;
#89220=DIRECTION ( 'NONE',  ( 1.000000000000000000, 2.999999999999999839E-15, 1.000000000000000078E-15 ) ) ;
#89221=ORIENTED_EDGE ( 'NONE', *, *, #49272, .F. ) ;
#89223=CARTESIAN_POINT ( 'NONE',  ( 110.5061846383585475, -26.86461981176654845, 209.8099109901969541 ) ) ;
#89224=CARTESIAN_POINT ( 'NONE',  ( 109.2014185099688603, -26.52530387367253795, 135.9127681330539872 ) ) ;
#89225=CARTESIAN_POINT ( 'NONE',  ( 108.0180542234412684, -24.86750695335871697, 261.0127681330534415 ) ) ;
#89226=CARTESIAN_POINT ( 'NONE',  ( 99.09570913299437223, -30.55043168099339823, 155.8022919353178395 ) ) ;
#89227=EDGE_CURVE ( 'NONE', #30095, #48357, #57987, .T. ) ;
#89228=CARTESIAN_POINT ( 'NONE',  ( 49.35211078756498893, -35.65087443492551245, 237.4678068554150059 ) ) ;
#89229=LINE ( 'NONE', #81083, #75415 ) ;
#89230=CARTESIAN_POINT ( 'NONE',  ( 182.2300522401149863, -33.89581943344511217, 117.4678068554150627 ) ) ;
#89231=CARTESIAN_POINT ( 'NONE',  ( 107.0664832912739541, -36.72944715994095333, 305.0306255462182321 ) ) ;
#89232=AXIS2_PLACEMENT_3D ( 'NONE', #61948, #48751, #27881 ) ;
#89234=AXIS2_PLACEMENT_3D ( 'NONE', #63399, #49307, #14818 ) ;
#89235=ORIENTED_EDGE ( 'NONE', *, *, #27052, .F. ) ;
#89236=ORIENTED_EDGE ( 'NONE', *, *, #42250, .F. ) ;
#89237=CARTESIAN_POINT ( 'NONE',  ( 99.28690145085043639, -32.09363259137744251, 130.3333722090289655 ) ) ;
#89239=ORIENTED_EDGE ( 'NONE', *, *, #21734, .T. ) ;
#89240=LINE ( 'NONE', #27005, #38774 ) ;
#89241=CARTESIAN_POINT ( 'NONE',  ( 117.5589153096731110, -33.32758106675091625, 130.0880062282919880 ) ) ;
#89242=CARTESIAN_POINT ( 'NONE',  ( 101.9927089507507816, -45.44550910856975889, 148.1569819098927780 ) ) ;
#89245=DIRECTION ( 'NONE',  ( 1.000000000000000078E-15, -1.000000000000000083E-30, -1.000000000000000000 ) ) ;
#89246=CARTESIAN_POINT ( 'NONE',  ( 107.3052971647831555, -26.36210646096926524, 75.04610146638796664 ) ) ;
#89248=ORIENTED_EDGE ( 'NONE', *, *, #34753, .F. ) ;
#89252=AXIS2_PLACEMENT_3D ( 'NONE', #33264, #60967, #81880 ) ;
#89254=CARTESIAN_POINT ( 'NONE',  ( 179.8608231853570487, -35.55794170701178558, 117.4678068554150627 ) ) ;
#89255=CARTESIAN_POINT ( 'NONE',  ( 102.3899016914588884, -28.13915478247121271, 141.4727681330539895 ) ) ;
#89256=CARTESIAN_POINT ( 'NONE',  ( 184.5667039024480118, -48.82844715994099971, 20.91780685541479912 ) ) ;
#89258=DIRECTION ( 'NONE',  ( 1.000000000000000000, 6.145690160522439356E-16, 0.000000000000000000 ) ) ;
#89261=CARTESIAN_POINT ( 'NONE',  ( 194.0667039024475287, -24.92844715993407334, 180.4678068554150343 ) ) ;
#89262=CARTESIAN_POINT ( 'NONE',  ( 95.51222647996974047, -34.21005103128000968, 106.1556252759109640 ) ) ;
#89264=VERTEX_POINT ( 'NONE', #55618 ) ;
#89266=AXIS2_PLACEMENT_3D ( 'NONE', #25880, #24989, #46748 ) ;
#89267=DIRECTION ( 'NONE',  ( 0.000000000000000000, -1.000000000000000000, 0.000000000000000000 ) ) ;
#89270=CIRCLE ( 'NONE', #22560, 3.000000000000002665 ) ;
#89271=CARTESIAN_POINT ( 'NONE',  ( 112.5929834642309117, -30.72215809952430376, 197.3023760838769647 ) ) ;
#89272=ADVANCED_FACE ( 'NONE', ( #83370 ), #6608, .F. ) ;
#89274=EDGE_CURVE ( 'NONE', #69124, #77884, #27942, .T. ) ;
#89275=EDGE_CURVE ( 'NONE', #83807, #44910, #42029, .T. ) ;
#89276=CARTESIAN_POINT ( 'NONE',  ( 115.0897088867533569, -30.61867969486051066, 25.34382189988804157 ) ) ;
#89277=VERTEX_POINT ( 'NONE', #21142 ) ;
#89279=VERTEX_POINT ( 'NONE', #35196 ) ;
#89280=DIRECTION ( 'NONE',  ( -1.000000000000000078E-15, 1.000000000000000083E-30, 1.000000000000000000 ) ) ;
#89281=EDGE_CURVE ( 'NONE', #48706, #57647, #13873, .T. ) ;
#89282=DIRECTION ( 'NONE',  ( 1.000000000000000078E-15, 0.000000000000000000, -1.000000000000000000 ) ) ;
#89283=ORIENTED_EDGE ( 'NONE', *, *, #40414, .F. ) ;
#89284=ORIENTED_EDGE ( 'NONE', *, *, #65190, .T. ) ;
#89285=DIRECTION ( 'NONE',  ( -4.237773401492740281E-14, 1.000000000000000000, 0.000000000000000000 ) ) ;
#89286=CARTESIAN_POINT ( 'NONE',  ( 102.9614994733801439, -44.58294233512814486, 208.6244404487539725 ) ) ;
#89287=ADVANCED_FACE ( 'NONE', ( #239 ), #19794, .F. ) ;
#89288=CARTESIAN_POINT ( 'NONE',  ( 180.1667039024460166, -26.71338133339240528, -5.074374724088000832 ) ) ;
#89291=EDGE_LOOP ( 'NONE', ( #37986, #69831, #56308, #58008, #56049, #38499 ) ) ;
#89292=EDGE_CURVE ( 'NONE', #48257, #31385, #21764, .T. ) ;
#89293=DIRECTION ( 'NONE',  ( 0.000000000000000000, 0.000000000000000000, -1.000000000000000000 ) ) ;
#89294=AXIS2_PLACEMENT_3D ( 'NONE', #61484, #34676, #62384 ) ;
#89295=VERTEX_POINT ( 'NONE', #21598 ) ;
#89297=EDGE_CURVE ( 'NONE', #61357, #45558, #5811, .T. ) ;
#89298=CARTESIAN_POINT ( 'NONE',  ( 105.5353399150147737, -28.71163411781831698, 233.0452332267339841 ) ) ;
#89299=CARTESIAN_POINT ( 'NONE',  ( 117.2597117638302393, -39.02229875088008981, 148.6499109901969859 ) ) ;
#89300=CARTESIAN_POINT ( 'NONE',  ( 117.0705705820184477, -32.08379757587633208, 59.16038718067295576 ) ) ;
#89301=CARTESIAN_POINT ( 'NONE',  ( 115.3486850554863707, -40.94587795544506292, 249.5838068554168103 ) ) ;
#89302=CARTESIAN_POINT ( 'NONE',  ( 131.9645448811557742, -16.94667115355465725, 7.474641677900195624 ) ) ;
#89303=CARTESIAN_POINT ( 'NONE',  ( 109.3584748782654401, -25.91645705315499981, 180.9222919425779708 ) ) ;
#89305=ORIENTED_EDGE ( 'NONE', *, *, #20635, .F. ) ;
#89307=EDGE_LOOP ( 'NONE', ( #6211, #61159, #19781, #68851 ) ) ;
#89308=ADVANCED_FACE ( 'NONE', ( #77004 ), #14787, .F. ) ;
#89309=VERTEX_POINT ( 'NONE', #47918 ) ;
#89311=ORIENTED_EDGE ( 'NONE', *, *, #26310, .T. ) ;
#89312=CIRCLE ( 'NONE', #42856, 5.599999999999994316 ) ;
#89315=CARTESIAN_POINT ( 'NONE',  ( 114.7075677164476986, -44.71649393962480445, 113.1718157521009687 ) ) ;
#89320=CARTESIAN_POINT ( 'NONE',  ( 108.3334480864761957, -46.73485935512827183, 143.6772919419037180 ) ) ;
#89321=LINE ( 'NONE', #39794, #55694 ) ;
#89322=CARTESIAN_POINT ( 'NONE',  ( 96.87985868497426623, -34.61725761836213167, 212.1641967044819808 ) ) ;
#89326=DIRECTION ( 'NONE',  ( 4.299999999999999979E-14, -1.000000000000000000, 4.400000000000000367E-29 ) ) ;
#89328=DIRECTION ( 'NONE',  ( 0.000000000000000000, 0.000000000000000000, 1.000000000000000000 ) ) ;
#89329=PLANE ( 'NONE',  #6762 ) ;
#89330=AXIS2_PLACEMENT_3D ( 'NONE', #64655, #23787, #45519 ) ;
#89332=CARTESIAN_POINT ( 'NONE',  ( 109.9724474192709351, -48.26999177473817326, 242.7727681330539724 ) ) ;
#89333=ORIENTED_EDGE ( 'NONE', *, *, #31428, .F. ) ;
#89334=CARTESIAN_POINT ( 'NONE',  ( 106.7561181679527209, -26.70555286918040139, 195.1009897130665252 ) ) ;
#89335=CARTESIAN_POINT ( 'NONE',  ( 102.6883137591737665, -46.90427260131782106, 137.2651490854349561 ) ) ;
#89336=CARTESIAN_POINT ( 'NONE',  ( 101.6089948421187898, -47.24856100052405594, 13.19562527591094891 ) ) ;
#89337=CARTESIAN_POINT ( 'NONE',  ( 117.0586869608412286, -33.60713302236428746, 170.0670538473399631 ) ) ;
#89341=AXIS2_PLACEMENT_3D ( 'NONE', #47654, #89466, #24009 ) ;
#89343=CARTESIAN_POINT ( 'NONE',  ( 194.0371591254575208, -24.42818131005407167, 180.4678068554150343 ) ) ;
#89344=FACE_BOUND ( 'NONE', #13610, .T. ) ;
#89345=DIRECTION ( 'NONE',  ( -0.7071067811865784369, 0.7071067811865165975, -7.071067811865791864E-16 ) ) ;
#89348=VERTEX_POINT ( 'NONE', #50877 ) ;
#89350=ORIENTED_EDGE ( 'NONE', *, *, #11710, .T. ) ;
#89352=CARTESIAN_POINT ( 'NONE',  ( 96.70769389551976758, -42.43415482991306220, 22.72705384733997391 ) ) ;
#89355=LINE ( 'NONE', #54793, #83889 ) ;
#89356=CARTESIAN_POINT ( 'NONE',  ( 106.9632158956753756, -45.78494306966059924, 232.0019436376009594 ) ) ;
#89358=VERTEX_POINT ( 'NONE', #15485 ) ;
#89359=ORIENTED_EDGE ( 'NONE', *, *, #39155, .F. ) ;
#89360=EDGE_CURVE ( 'NONE', #19378, #48818, #43154, .T. ) ;
#89363=CARTESIAN_POINT ( 'NONE',  ( 180.3164832912740110, 12.92155284005802507, 349.2756252759111248 ) ) ;
#89364=LINE ( 'NONE', #82565, #87569 ) ;
#89366=DIRECTION ( 'NONE',  ( 1.000000000000000000, 0.000000000000000000, 0.000000000000000000 ) ) ;
#89368=CARTESIAN_POINT ( 'NONE',  ( 97.83217745605946902, -40.05230289513916375, 266.6013395616258776 ) ) ;
#89369=FACE_OUTER_BOUND ( 'NONE', #70271, .T. ) ;
#89371=ORIENTED_EDGE ( 'NONE', *, *, #80199, .F. ) ;
#89372=CYLINDRICAL_SURFACE ( 'NONE', #54783, 2.749999999999974687 ) ;
#89373=AXIS2_PLACEMENT_3D ( 'NONE', #83147, #5601, #49929 ) ;
#89375=CARTESIAN_POINT ( 'NONE',  ( 98.42956409136928642, -40.12054696651731689, 94.44237608387695104 ) ) ;
#89378=AXIS2_PLACEMENT_3D ( 'NONE', #87243, #54018, #74498 ) ;
#89380=EDGE_CURVE ( 'NONE', #46099, #56697, #17262, .T. ) ;
#89382=EDGE_LOOP ( 'NONE', ( #87830, #82336, #28170, #2139 ) ) ;
#89386=CARTESIAN_POINT ( 'NONE',  ( 96.60699139826044757, -36.88735862350505101, 136.3384824187679385 ) ) ;
#89388=EDGE_CURVE ( 'NONE', #23038, #59691, #43516, .T. ) ;
#89390=CARTESIAN_POINT ( 'NONE',  ( 107.2938360571228600, -27.87074582556254398, 116.4872975916119771 ) ) ;
#89391=EDGE_CURVE ( 'NONE', #21258, #30095, #37257, .T. ) ;
#89394=AXIS2_PLACEMENT_3D ( 'NONE', #14410, #82568, #34381 ) ;
#89395=CARTESIAN_POINT ( 'NONE',  ( 116.7650972879214919, -32.84690348374694224, 50.12991099019698282 ) ) ;
#89397=VERTEX_POINT ( 'NONE', #58571 ) ;
#89400=ORIENTED_EDGE ( 'NONE', *, *, #35881, .F. ) ;
#89403=EDGE_CURVE ( 'NONE', #28049, #3581, #51751, .T. ) ;
#89404=CYLINDRICAL_SURFACE ( 'NONE', #13702, 5.599999999999994316 ) ;
#89405=ORIENTED_EDGE ( 'NONE', *, *, #87123, .F. ) ;
#89406=CARTESIAN_POINT ( 'NONE',  ( 100.5669465097397506, -44.03830869352251653, 266.9984824187685604 ) ) ;
#89407=CARTESIAN_POINT ( 'NONE',  ( 99.08473320778040261, -45.52208679145996939, 152.9899109901969894 ) ) ;
#89410=CARTESIAN_POINT ( 'NONE',  ( 102.5581934769535906, -27.32956362888499768, 91.43276813305395478 ) ) ;
#89411=DIRECTION ( 'NONE',  ( 0.8660254037844359321, 0.000000000000000000, 0.5000000000000046629 ) ) ;
#89412=ORIENTED_EDGE ( 'NONE', *, *, #32732, .T. ) ;
#89414=DIRECTION ( 'NONE',  ( 1.000000000000000078E-15, 1.000000000000000083E-30, -1.000000000000000000 ) ) ;
#89417=DIRECTION ( 'NONE',  ( -0.7071067811865743291, 0.7071067811865207053, -7.071067811865750448E-16 ) ) ;
#89418=FACE_OUTER_BOUND ( 'NONE', #38833, .T. ) ;
#89419=CARTESIAN_POINT ( 'NONE',  ( 98.42358855985509081, -42.06826316073455274, 11.76800622829193799 ) ) ;
#89422=FACE_OUTER_BOUND ( 'NONE', #66086, .T. ) ;
#89423=CARTESIAN_POINT ( 'NONE',  ( 114.9268010244043978, -42.60560063232861694, 28.31562527591097123 ) ) ;
#89424=CARTESIAN_POINT ( 'NONE',  ( 97.78574527986302201, -40.45344939432850140, 101.6305854416151675 ) ) ;
#89425=CARTESIAN_POINT ( 'NONE',  ( 102.3703197837810848, -46.01248081495474906, 123.2041967044829818 ) ) ;
#89426=FACE_OUTER_BOUND ( 'NONE', #34588, .T. ) ;
#89427=CARTESIAN_POINT ( 'NONE',  ( 117.2811830599562057, -39.02712847638015603, 148.6499109901969859 ) ) ;
#89429=ORIENTED_EDGE ( 'NONE', *, *, #66905, .T. ) ;
#89430=DIRECTION ( 'NONE',  ( -4.237773401492740281E-14, 1.000000000000000000, 0.000000000000000000 ) ) ;
#89431=DIRECTION ( 'NONE',  ( 0.000000000000000000, 1.000000000000000000, 0.000000000000000000 ) ) ;
#89432=PLANE ( 'NONE',  #71723 ) ;
#89433=EDGE_LOOP ( 'NONE', ( #9201, #59022 ) ) ;
#89434=CARTESIAN_POINT ( 'NONE',  ( 108.4200078917168639, -26.73535838700381362, 60.96903794334217963 ) ) ;
#89435=CARTESIAN_POINT ( 'NONE',  ( 102.5972826210866060, -46.89011293525640411, 132.2346728949579528 ) ) ;
#89436=ORIENTED_EDGE ( 'NONE', *, *, #55044, .F. ) ;
#89437=DIRECTION ( 'NONE',  ( 0.000000000000000000, 0.000000000000000000, 1.000000000000000000 ) ) ;
#89440=ADVANCED_FACE ( 'NONE', ( #3187 ), #59010, .T. ) ;
#89441=CARTESIAN_POINT ( 'NONE',  ( 184.5667039024483245, -48.82844715993448403, 300.4678068554149490 ) ) ;
#89442=DIRECTION ( 'NONE',  ( -0.7071067811567310901, 0.7071067812163639443, 0.000000000000000000 ) ) ;
#89444=ORIENTED_EDGE ( 'NONE', *, *, #59574, .F. ) ;
#89445=VECTOR ( 'NONE', #45711, 1000.000000000000000 ) ;
#89447=VECTOR ( 'NONE', #37759, 1000.000000000000000 ) ;
#89448=ADVANCED_FACE ( 'NONE', ( #22748, #79500 ), #44047, .F. ) ;
#89449=VERTEX_POINT ( 'NONE', #36365 ) ;
#89452=CARTESIAN_POINT ( 'NONE',  ( 172.5664832912740110, -18.82844715994099971, 258.9256252759120116 ) ) ;
#89453=CARTESIAN_POINT ( 'NONE',  ( 100.0143388906741393, -29.55856279621482585, 250.6953418232228898 ) ) ;
#89455=DIRECTION ( 'NONE',  ( 1.000000000000000000, 0.000000000000000000, 0.000000000000000000 ) ) ;
#89457=CARTESIAN_POINT ( 'NONE',  ( 151.0371591254573502, -24.42818131005592974, 249.9678068554149490 ) ) ;
#89459=ORIENTED_EDGE ( 'NONE', *, *, #87360, .F. ) ;
#89461=CLOSED_SHELL ( 'NONE', ( #7640, #34210, #83276, #5987, #78115, #55814, #87923 ) ) ;
#89463=DIRECTION ( 'NONE',  ( -0.9254794337955620787, -0.3787978585227822492, 0.000000000000000000 ) ) ;
#89465=CARTESIAN_POINT ( 'NONE',  ( 106.5981863181247604, -46.53222597210204725, 243.5384824187679556 ) ) ;
#89466=DIRECTION ( 'NONE',  ( -1.000000000000000078E-15, -1.000000000000000083E-30, 1.000000000000000000 ) ) ;
#89467=CARTESIAN_POINT ( 'NONE',  ( 112.9285164932675514, -28.85859325239454165, 100.5670538473389684 ) ) ;
#89469=CARTESIAN_POINT ( 'NONE',  ( 103.7104750361727383, -27.30776277115187156, 21.34877412902993399 ) ) ;
#89470=ORIENTED_CLOSED_SHELL ( 'NONE', *, #11119, .F. );
#89471=VERTEX_POINT ( 'NONE', #10439 ) ;
#89472=DIRECTION ( 'NONE',  ( 2.900000000000000265E-14, -2.000000000000000155E-15, 1.000000000000000000 ) ) ;
#89473=VERTEX_POINT ( 'NONE', #51303 ) ;
#89474=ORIENTED_EDGE ( 'NONE', *, *, #10297, .F. ) ;
#89477=CARTESIAN_POINT ( 'NONE',  ( 111.1445474647120051, -44.63080920614596181, 269.3872975916115706 ) ) ;
#89479=DIRECTION ( 'NONE',  ( 0.000000000000000000, 0.000000000000000000, -1.000000000000000000 ) ) ;
#89482=EDGE_CURVE ( 'NONE', #63259, #49134, #37769, .T. ) ;
#89485=CARTESIAN_POINT ( 'NONE',  ( 142.0664832912740110, -9.729447159941040368, 14.82207188531770115 ) ) ;
#89486=CYLINDRICAL_SURFACE ( 'NONE', #23772, 3.000000000000002665 ) ;
#89488=CARTESIAN_POINT ( 'NONE',  ( 117.2669906530413186, -38.88274231480306042, 63.66133956162494911 ) ) ;
#89489=EDGE_LOOP ( 'NONE', ( #63712, #32830, #87277, #47245 ) ) ;
#89490=EDGE_CURVE ( 'NONE', #85218, #42076, #86749, .T. ) ;
#89491=CARTESIAN_POINT ( 'NONE',  ( 115.6911714722407396, -33.30735935496929301, 246.9452332267339614 ) ) ;
#89492=FACE_OUTER_BOUND ( 'NONE', #33677, .T. ) ;
#89493=CARTESIAN_POINT ( 'NONE',  ( 117.1372161989437899, -34.25576096370539148, 164.0061014663879746 ) ) ;
#89495=EDGE_CURVE ( 'NONE', #35560, #26742, #39280, .T. ) ;
#89497=CARTESIAN_POINT ( 'NONE',  ( 163.0664832912739826, -18.82844715994099971, 333.4006252759120343 ) ) ;
#89499=CYLINDRICAL_SURFACE ( 'NONE', #29094, 2.500000000000002220 ) ;
#89500=CARTESIAN_POINT ( 'NONE',  ( 118.7023651333632159, -39.22291191012653400, 254.6584824187681022 ) ) ;
#89503=CIRCLE ( 'NONE', #79335, 2.500000000000002220 ) ;
#89505=CARTESIAN_POINT ( 'NONE',  ( 98.11234142011190329, -43.28847465721014487, 102.8175300378159847 ) ) ;
#89510=EDGE_LOOP ( 'NONE', ( #4930, #40189, #22801, #57497, #63927 ) ) ;
#89511=VERTEX_POINT ( 'NONE', #46723 ) ;
#89512=EDGE_CURVE ( 'NONE', #74550, #40777, #8734, .T. ) ;
#89513=CARTESIAN_POINT ( 'NONE',  ( 164.9667039024459996, -28.27351298637401200, 342.9256252759119548 ) ) ;
#89515=EDGE_CURVE ( 'NONE', #83508, #67349, #12680, .T. ) ;
#89516=CARTESIAN_POINT ( 'NONE',  ( 140.9629299006806491, -8.979447159940995959, 14.92562527591100618 ) ) ;
#89518=CARTESIAN_POINT ( 'NONE',  ( 103.0775956431641305, -44.40992243120454930, 165.0014237029239439 ) ) ;
#89519=CARTESIAN_POINT ( 'NONE',  ( 96.89316087236547048, -34.20304521249558150, 272.1327681330539576 ) ) ;
#89521=ORIENTED_EDGE ( 'NONE', *, *, #69182, .F. ) ;
#89523=AXIS2_PLACEMENT_3D ( 'NONE', #85589, #22018, #15187 ) ;
#89524=CIRCLE ( 'NONE', #32900, 2.029999999999997140 ) ;
#89525=DIRECTION ( 'NONE',  ( 0.000000000000000000, 0.000000000000000000, -1.000000000000000000 ) ) ;
#89526=ORIENTED_EDGE ( 'NONE', *, *, #16178, .T. ) ;
#89527=VERTEX_POINT ( 'NONE', #39024 ) ;
#89528=AXIS2_PLACEMENT_3D ( 'NONE', #76408, #1003, #76859 ) ;
#89529=DIRECTION ( 'NONE',  ( 4.237773401492740281E-14, -1.000000000000000000, 0.000000000000000000 ) ) ;
#89530=ORIENTED_EDGE ( 'NONE', *, *, #23285, .F. ) ;
#89532=DIRECTION ( 'NONE',  ( -0.7071067811865274777, 0.7071067811865675568, -7.071067811865283048E-16 ) ) ;
#89533=CARTESIAN_POINT ( 'NONE',  ( 115.8254304378072987, -31.73001405447006817, 14.23979235309599289 ) ) ;
#89534=CYLINDRICAL_SURFACE ( 'NONE', #78262, 3.250000000000002665 ) ;
#89535=CARTESIAN_POINT ( 'NONE',  ( 182.2300522401171179, -33.89581943343741699, 313.9678068554149490 ) ) ;
#89536=CARTESIAN_POINT ( 'NONE',  ( 104.2579841207466984, -28.11985932224000351, 209.7619436376009787 ) ) ;
#89537=CARTESIAN_POINT ( 'NONE',  ( 97.73303842741869119, -31.98671872394393034, 50.95276813305294183 ) ) ;
#89538=CARTESIAN_POINT ( 'NONE',  ( 141.0235900724605642, -46.62589376934778329, -5.074374724089071087 ) ) ;
#89540=DIRECTION ( 'NONE',  ( -0.7071067811578587436, 0.7071067812152364018, 0.000000000000000000 ) ) ;
#89542=CARTESIAN_POINT ( 'NONE',  ( 115.0878329645715468, -30.61624704198585434, 260.3439639102809338 ) ) ;
#89544=DIRECTION ( 'NONE',  ( -0.7071067811865462405, 0.000000000000000000, 0.7071067811865486830 ) ) ;
#89546=PLANE ( 'NONE',  #54778 ) ;
#89548=DIRECTION ( 'NONE',  ( -1.000000000000000078E-15, 1.000000000000000083E-30, 1.000000000000000000 ) ) ;
#89550=CARTESIAN_POINT ( 'NONE',  ( 110.8024161898992190, -46.48594086123524960, 62.86705384733992474 ) ) ;
#89553=ADVANCED_FACE ( 'NONE', ( #25856 ), #45820, .F. ) ;
#89555=DIRECTION ( 'NONE',  ( 0.000000000000000000, 0.000000000000000000, -1.000000000000000000 ) ) ;
#89556=VERTEX_POINT ( 'NONE', #88093 ) ;
#89557=CARTESIAN_POINT ( 'NONE',  ( 98.01104804690241679, -32.31685915242277929, 121.9642353160954684 ) ) ;
#89558=CARTESIAN_POINT ( 'NONE',  ( 48.79742451362098166, -36.32844715994040996, -5.074374724088000832 ) ) ;
#89560=ORIENTED_EDGE ( 'NONE', *, *, #2239, .F. ) ;
#89561=CARTESIAN_POINT ( 'NONE',  ( 100.2845952792443569, -46.47769036989463132, 83.09276813305294240 ) ) ;
#89563=CARTESIAN_POINT ( 'NONE',  ( 105.7165518034377811, -46.72402163992320823, 172.4654686376170218 ) ) ;
#89564=DIRECTION ( 'NONE',  ( -0.0001713722456127401463, 0.9999999853157766072, 1.713722456137401502E-19 ) ) ;
#89565=CARTESIAN_POINT ( 'NONE',  ( 71.23990787207000608, 10.64204399490126463, 540.9756252759101471 ) ) ;
#89567=EDGE_CURVE ( 'NONE', #17862, #67541, #62395, .T. ) ;
#89568=AXIS2_PLACEMENT_3D ( 'NONE', #80670, #67468, #39755 ) ;
#89570=ORIENTED_EDGE ( 'NONE', *, *, #48109, .F. ) ;
#89571=CARTESIAN_POINT ( 'NONE',  ( 117.0231039428182385, -39.62849705588580917, 134.5889586092439743 ) ) ;
#89573=VERTEX_POINT ( 'NONE', #39916 ) ;
#89574=CARTESIAN_POINT ( 'NONE',  ( 109.9831304889622743, -26.74336511273928707, 255.8499109901966051 ) ) ;
#89575=DIRECTION ( 'NONE',  ( -1.000000000000000000, 0.000000000000000000, 0.000000000000000000 ) ) ;
#89577=CYLINDRICAL_SURFACE ( 'NONE', #47262, 0.5000000000000197620 ) ;
#89578=DIRECTION ( 'NONE',  ( 1.000000000000000000, 0.000000000000000000, 0.000000000000000000 ) ) ;
#89579=EDGE_CURVE ( 'NONE', #22726, #6301, #11782, .T. ) ;
#89580=AXIS2_PLACEMENT_3D ( 'NONE', #26723, #19924, #75339 ) ;
#89583=CARTESIAN_POINT ( 'NONE',  ( 124.0664832912757021, -36.72944715993921960, 14.92562527591098842 ) ) ;
#89584=AXIS2_PLACEMENT_3D ( 'NONE', #63672, #36424, #35499 ) ;
#89585=AXIS2_PLACEMENT_3D ( 'NONE', #55305, #83062, #50753 ) ;
#89586=CARTESIAN_POINT ( 'NONE',  ( 97.99937763885726838, -40.39701179870337455, 206.6327681330539860 ) ) ;
#89589=CARTESIAN_POINT ( 'NONE',  ( 99.74964917879287896, -31.73022550229359595, 117.2815833058969446 ) ) ;
#89592=CARTESIAN_POINT ( 'NONE',  ( 97.95230308628410398, -39.01119097033267025, 12.96539282970593554 ) ) ;
#89593=CARTESIAN_POINT ( 'NONE',  ( 78.64819577385250682, -34.37139167075708457, 1.944749297858806125 ) ) ;
#89594=CARTESIAN_POINT ( 'NONE',  ( 19.56648329127303043, 25.62155284005700295, 342.9256252759109884 ) ) ;
#89597=CARTESIAN_POINT ( 'NONE',  ( 50.87649884952465840, -33.54226604284966839, 313.9678068554150059 ) ) ;
#89598=CARTESIAN_POINT ( 'NONE',  ( 181.8764988495240118, -33.54226604284930602, -5.074374724088000832 ) ) ;
#89599=CARTESIAN_POINT ( 'NONE',  ( 93.47673478713714701, -35.56394370010534800, 302.6356252759109680 ) ) ;
#89600=CARTESIAN_POINT ( 'NONE',  ( 106.3035372762157351, -47.10473409126657174, 222.5184824187679453 ) ) ;
#89601=CARTESIAN_POINT ( 'NONE',  ( 63.56670390244745050, -47.82844715994014706, 129.9678068554150911 ) ) ;
#89602=ORIENTED_EDGE ( 'NONE', *, *, #44758, .T. ) ;
#89604=ORIENTED_EDGE ( 'NONE', *, *, #57985, .T. ) ;
#89605=CARTESIAN_POINT ( 'NONE',  ( 45.56670390244500624, -48.82844715994099971, 249.9678068554150343 ) ) ;
#89606=CARTESIAN_POINT ( 'NONE',  ( 82.26793483429007381, -20.38027623202287586, 7.385026757025396016 ) ) ;
#89607=CARTESIAN_POINT ( 'NONE',  ( 104.4905352225451054, -26.97864795354891854, 185.2818706022724768 ) ) ;
#89608=CARTESIAN_POINT ( 'NONE',  ( 19.56648329127400032, -18.82844715994099971, -5.074374724088000832 ) ) ;
#89609=AXIS2_PLACEMENT_3D ( 'NONE', #20349, #339, #75758 ) ;
#89610=VECTOR ( 'NONE', #53767, 1000.000000000000000 ) ;
#89612=ORIENTED_EDGE ( 'NONE', *, *, #3644, .F. ) ;
#89613=CARTESIAN_POINT ( 'NONE',  ( 117.5558648759066926, -37.28717672647940873, 14.78419670448294454 ) ) ;
#89614=CARTESIAN_POINT ( 'NONE',  ( 117.2277029493381377, -41.08016003417893103, 213.5165776568629781 ) ) ;
#89617=FACE_OUTER_BOUND ( 'NONE', #52373, .T. ) ;
#89618=CYLINDRICAL_SURFACE ( 'NONE', #3655, 9.999999999999998224 ) ;
#89619=EDGE_CURVE ( 'NONE', #18344, #1069, #13067, .T. ) ;
#89621=EDGE_CURVE ( 'NONE', #15468, #33306, #46423, .T. ) ;
#89622=CARTESIAN_POINT ( 'NONE',  ( 100.9805754248354788, -42.21072563198327998, 54.72809036959092310 ) ) ;
#89623=CARTESIAN_POINT ( 'NONE',  ( 97.98816800684205930, -30.38363046389439859, 156.8289586092439549 ) ) ;
#89625=VERTEX_POINT ( 'NONE', #59905 ) ;
#89627=VECTOR ( 'NONE', #76341, 1000.000000000000000 ) ;
#89628=FACE_OUTER_BOUND ( 'NONE', #14628, .T. ) ;
#89629=CARTESIAN_POINT ( 'NONE',  ( 97.81315821180474757, -40.51681016098617505, 66.63608906629065132 ) ) ;
#89630=ORIENTED_EDGE ( 'NONE', *, *, #31487, .F. ) ;
#89631=ORIENTED_EDGE ( 'NONE', *, *, #47795, .F. ) ;
#89632=AXIS2_PLACEMENT_3D ( 'NONE', #69237, #48764, #3765 ) ;
#89633=FACE_OUTER_BOUND ( 'NONE', #50165, .T. ) ;
#89634=ORIENTED_EDGE ( 'NONE', *, *, #56835, .T. ) ;
#89636=CARTESIAN_POINT ( 'NONE',  ( 165.2725846195380086, -35.55794170701810941, -5.074374724088000832 ) ) ;
#89637=CARTESIAN_POINT ( 'NONE',  ( 102.6518059180641416, -28.82227990381128180, 104.9162293518859599 ) ) ;
#89638=CARTESIAN_POINT ( 'NONE',  ( 118.0743634110212383, -35.49574686983337557, 233.9032443235299752 ) ) ;
#89640=CARTESIAN_POINT ( 'NONE',  ( 107.5647246096319236, -47.74832088493825211, 192.6003871806729535 ) ) ;
#89642=CARTESIAN_POINT ( 'NONE',  ( 116.3171286962602267, -41.53660429022799150, 284.4441967044824082 ) ) ;
#89644=CARTESIAN_POINT ( 'NONE',  ( 172.5664832912740110, -9.303447159940999356, 78.92562527591199739 ) ) ;
#89645=AXIS2_PLACEMENT_3D ( 'NONE', #51294, #13330, #6509 ) ;
#89647=CIRCLE ( 'NONE', #62076, 1.000000000000000888 ) ;
#89648=AXIS2_PLACEMENT_3D ( 'NONE', #51848, #10539, #52283 ) ;
#89649=VECTOR ( 'NONE', #88916, 1000.000000000000000 ) ;
#89650=CARTESIAN_POINT ( 'NONE',  ( 98.20607846729126322, -32.50961293922092210, 75.97276813305397525 ) ) ;
#89651=CARTESIAN_POINT ( 'NONE',  ( 101.9388778781502509, -27.60177885026046596, 60.48419670448296159 ) ) ;
#89652=CARTESIAN_POINT ( 'NONE',  ( 109.2210686807619453, -48.43357285789136313, 277.7213395616254843 ) ) ;
#89653=ORIENTED_EDGE ( 'NONE', *, *, #54667, .T. ) ;
#89654=CARTESIAN_POINT ( 'NONE',  ( 106.9404395787681352, -47.78219344473501451, 232.5794347997199907 ) ) ;
#89656=CARTESIAN_POINT ( 'NONE',  ( 0.000000000000000000, 0.000000000000000000, 0.000000000000000000 ) ) ;
#89657=CARTESIAN_POINT ( 'NONE',  ( 117.0607179957026176, -38.08171581397471073, 24.71885727970600755 ) ) ;
#89658=CARTESIAN_POINT ( 'NONE',  ( 188.5667039024479834, -58.35344715994099829, 139.9678068554150059 ) ) ;
#89659=CARTESIAN_POINT ( 'NONE',  ( 114.6549693520563835, -40.28990096540307775, 277.6356252759109111 ) ) ;
#89660=DIRECTION ( 'NONE',  ( 0.000000000000000000, 1.000000000000000000, 0.000000000000000000 ) ) ;
#89661=EDGE_CURVE ( 'NONE', #83042, #6555, #31766, .T. ) ;
#89662=CARTESIAN_POINT ( 'NONE',  ( 99.08963683242468790, -42.79560731373364035, 172.8439316841160291 ) ) ;
#89663=CARTESIAN_POINT ( 'NONE',  ( 41.56670390244695312, -36.32844715994109208, 129.9678068554150911 ) ) ;
#89665=CIRCLE ( 'NONE', #79551, 2.500000000000002220 ) ;
#89666=LINE ( 'NONE', #20172, #61710 ) ;
#89667=CARTESIAN_POINT ( 'NONE',  ( 102.0623058274917696, -27.97328479470368379, 40.48947073801728180 ) ) ;
#89668=DIRECTION ( 'NONE',  ( 0.000000000000000000, 0.000000000000000000, 1.000000000000000000 ) ) ;
#89669=FACE_OUTER_BOUND ( 'NONE', #27264, .T. ) ;
#89670=EDGE_LOOP ( 'NONE', ( #297, #83371, #69505, #54260 ) ) ;
#89671=CARTESIAN_POINT ( 'NONE',  ( 107.0664832912740110, -46.47944715994103149, 14.92562527591097066 ) ) ;
#89672=CARTESIAN_POINT ( 'NONE',  ( 103.0820296961932456, -47.91685729158425744, 252.3041967044823366 ) ) ;
#89673=CARTESIAN_POINT ( 'NONE',  ( 114.5121600660089030, -29.42679343410769377, 145.4441967044819819 ) ) ;
#89674=CARTESIAN_POINT ( 'NONE',  ( 116.2568870038579547, -41.81614494787783798, 259.4241967044827106 ) ) ;
#89675=LINE ( 'NONE', #26992, #31615 ) ;
#89677=DIRECTION ( 'NONE',  ( 0.000000000000000000, 0.000000000000000000, 1.000000000000000000 ) ) ;
#89678=LINE ( 'NONE', #5663, #19468 ) ;
#89680=AXIS2_PLACEMENT_3D ( 'NONE', #64495, #2271, #29973 ) ;
#89682=ADVANCED_FACE ( 'NONE', ( #87638 ), #53066, .F. ) ;
#89683=ORIENTED_EDGE ( 'NONE', *, *, #52841, .F. ) ;
#89684=ADVANCED_FACE ( 'NONE', ( #21276, #7649, #82633, #33996, #28521, #34895, #62156, #89888, #61697, #35337, #63051, #6748, #62606, #27641, #55321, #48950, #831, #34446, #83076 ), #26739, .T. ) ;
#89686=VERTEX_POINT ( 'NONE', #20394 ) ;
#89687=CARTESIAN_POINT ( 'NONE',  ( 109.0154912191213583, -27.88557705556195998, 179.3143245899819647 ) ) ;
#89690=VERTEX_POINT ( 'NONE', #20830 ) ;
#89692=CARTESIAN_POINT ( 'NONE',  ( 114.9485010938853122, -29.93956786141553295, 180.3927681330539770 ) ) ;
#89693=DIRECTION ( 'NONE',  ( -0.7071067708032283683, -0.0001211784769705719365, 0.7071067811865527908 ) ) ;
#89694=DIRECTION ( 'NONE',  ( 0.7071067811862239427, 0.7071067811868709807, 0.000000000000000000 ) ) ;
#89695=EDGE_CURVE ( 'NONE', #1618, #65123, #380, .T. ) ;
#89699=CARTESIAN_POINT ( 'NONE',  ( 118.1148702536304427, -35.48641528967804248, 83.91562527591095488 ) ) ;
#89701=EDGE_LOOP ( 'NONE', ( #46125, #63381, #61848, #63312 ) ) ;
#89702=VERTEX_POINT ( 'NONE', #28075 ) ;
#89705=AXIS2_PLACEMENT_3D ( 'NONE', #44502, #30892, #72234 ) ;
#89706=DIRECTION ( 'NONE',  ( -0.9999999853157766072, -0.0001713722456134502174, 0.000000000000000000 ) ) ;
#89707=CARTESIAN_POINT ( 'NONE',  ( 113.6884830475838442, -29.53135334845051574, 195.4841967044819739 ) ) ;
#89709=DIRECTION ( 'NONE',  ( -1.000000000000000000, 0.000000000000000000, 0.000000000000000000 ) ) ;
#89711=CARTESIAN_POINT ( 'NONE',  ( 163.5667039024461360, -18.82844715994099971, 335.8679285791478719 ) ) ;
#89713=VECTOR ( 'NONE', #4128, 1000.000000000000000 ) ;
#89714=DIRECTION ( 'NONE',  ( -4.554376769437570034E-14, 1.000000000000000000, 0.000000000000000000 ) ) ;
#89716=CARTESIAN_POINT ( 'NONE',  ( 116.5783909117432842, -29.70293872869703833, 109.3327681330539605 ) ) ;
#89719=ADVANCED_FACE ( 'NONE', ( #8098 ), #75798, .F. ) ;
#89720=ORIENTED_EDGE ( 'NONE', *, *, #971, .F. ) ;
#89722=DIRECTION ( 'NONE',  ( 1.000000000000000000, 4.272717921125132861E-14, 0.000000000000000000 ) ) ;
#89724=AXIS2_PLACEMENT_3D ( 'NONE', #57061, #84805, #77981 ) ;
#89727=CARTESIAN_POINT ( 'NONE',  ( 98.90610402553750191, -36.53467484046868208, 194.1252332267349630 ) ) ;
#89730=ORIENTED_EDGE ( 'NONE', *, *, #76253, .F. ) ;
#89731=VERTEX_POINT ( 'NONE', #47619 ) ;
#89734=ORIENTED_EDGE ( 'NONE', *, *, #642, .T. ) ;
#89737=EDGE_CURVE ( 'NONE', #73246, #86684, #13130, .T. ) ;
#89738=CARTESIAN_POINT ( 'NONE',  ( 109.5509076938284068, -28.22321920626787062, 256.2815833058970725 ) ) ;
#89739=ORIENTED_EDGE ( 'NONE', *, *, #66737, .F. ) ;
#89740=EDGE_CURVE ( 'NONE', #78028, #13668, #30503, .T. ) ;
#89741=VECTOR ( 'NONE', #48125, 1000.000000000000000 ) ;
#89742=CYLINDRICAL_SURFACE ( 'NONE', #37780, 1.000000000002049694 ) ;
#89743=AXIS2_PLACEMENT_3D ( 'NONE', #43303, #24223, #10579 ) ;
#89747=DIRECTION ( 'NONE',  ( 1.000000000000000000, -1.040834085586083310E-14, 0.000000000000000000 ) ) ;
#89748=ORIENTED_EDGE ( 'NONE', *, *, #54366, .T. ) ;
#89749=ORIENTED_EDGE ( 'NONE', *, *, #68561, .F. ) ;
#89750=CARTESIAN_POINT ( 'NONE',  ( 111.8846140958497273, -43.31847907419767552, 225.8966617981629668 ) ) ;
#89751=CARTESIAN_POINT ( 'NONE',  ( 99.66888285774223277, -46.01973906766702527, 122.0413395616249659 ) ) ;
#89752=CARTESIAN_POINT ( 'NONE',  ( 106.0785370228624913, -48.51385081415340750, 112.5099109901969712 ) ) ;
#89753=CARTESIAN_POINT ( 'NONE',  ( 99.04337972803247681, -36.17635250646264922, 249.5838068554172935 ) ) ;
#89754=CARTESIAN_POINT ( 'NONE',  ( 133.1188885517785252, -16.14703303315377525, 8.087249882924000488 ) ) ;
#89755=CARTESIAN_POINT ( 'NONE',  ( 102.6835365363430981, -27.27046913952221985, 176.4213395616249898 ) ) ;
#89756=CARTESIAN_POINT ( 'NONE',  ( 179.1667039024460166, -26.71338133339251542, -5.074374724088000832 ) ) ;
#89757=CARTESIAN_POINT ( 'NONE',  ( 97.31588835286031269, -39.30608500589924148, 127.5314679824783894 ) ) ;
#89763=CARTESIAN_POINT ( 'NONE',  ( 33.78129701732998313, -35.65087443492610930, 313.9678068554150059 ) ) ;
#89764=ORIENTED_EDGE ( 'NONE', *, *, #62679, .T. ) ;
#89768=CARTESIAN_POINT ( 'NONE',  ( 117.6081704542122282, -33.40500446796587397, 129.0575300378159795 ) ) ;
#89771=LINE ( 'NONE', #5299, #13643 ) ;
#89772=CARTESIAN_POINT ( 'NONE',  ( 100.8874678748097296, -44.70022136769403431, 143.0522919416148966 ) ) ;
#89774=CARTESIAN_POINT ( 'NONE',  ( 97.42226921825846375, -40.63044708855864684, 202.6327681330539860 ) ) ;
#89775=DIRECTION ( 'NONE',  ( 4.299999999999999979E-14, -1.000000000000000000, 4.400000000000000367E-29 ) ) ;
#89777=ORIENTED_EDGE ( 'NONE', *, *, #11254, .F. ) ;
#89779=DIRECTION ( 'NONE',  ( -0.9999999853157766072, -0.0001713722456143218888, 0.000000000000000000 ) ) ;
#89780=CARTESIAN_POINT ( 'NONE',  ( 184.5664832912729878, -71.37844715994266664, 342.9256252759109884 ) ) ;
#89781=AXIS2_PLACEMENT_3D ( 'NONE', #23797, #44201, #59175 ) ;
#89782=DIRECTION ( 'NONE',  ( 0.9834602067019604377, 0.1811243270069963496, 0.000000000000000000 ) ) ;
#89783=CARTESIAN_POINT ( 'NONE',  ( 95.18116725028646385, -37.33612674980418689, 271.3670538473392639 ) ) ;
#89784=ORIENTED_EDGE ( 'NONE', *, *, #87252, .F. ) ;
#89786=CARTESIAN_POINT ( 'NONE',  ( 96.61975328461473111, -36.61901104994432643, 111.3184824187679567 ) ) ;
#89787=CARTESIAN_POINT ( 'NONE',  ( 103.4771999316985500, -25.43557003456049870, 51.32133956162493149 ) ) ;
#89788=CARTESIAN_POINT ( 'NONE',  ( 95.86339321018937198, -32.71673170297378164, 172.0527681330539735 ) ) ;
#89789=DIRECTION ( 'NONE',  ( -0.9254794337955620787, -0.3787978585227822492, 0.000000000000000000 ) ) ;
#89790=AXIS2_PLACEMENT_3D ( 'NONE', #8555, #36709, #2640 ) ;
#89793=PLANE ( 'NONE',  #5718 ) ;
#89795=LINE ( 'NONE', #13038, #68450 ) ;
#89796=DIRECTION ( 'NONE',  ( 9.912705577010326536E-16, 1.000000000000000000, 0.000000000000000000 ) ) ;
#89797=ORIENTED_EDGE ( 'NONE', *, *, #62383, .F. ) ;
#89798=EDGE_CURVE ( 'NONE', #3392, #3093, #47858, .T. ) ;
#89800=EDGE_CURVE ( 'NONE', #53148, #45118, #60015, .T. ) ;
#89802=VECTOR ( 'NONE', #51628, 1000.000000000000000 ) ;
#89805=CARTESIAN_POINT ( 'NONE',  ( 97.81168148112675453, -40.51739256386586163, 162.6360428395636859 ) ) ;
#89806=CARTESIAN_POINT ( 'NONE',  ( 96.10063762778156615, -37.91858611869021445, 77.40038718067299328 ) ) ;
#89807=B_SPLINE_CURVE_WITH_KNOTS ( 'NONE', 3,
 ( #74987, #41339, #47257, #69071, #15007, #44028, #22725, #9533, #64055, #22275, #70422, #9094, #49950, #77236, #64942, #15907, #64500, #35431 ),
 .UNSPECIFIED., .F., .F.,
 ( 4, 2, 2, 2, 2, 2, 2, 2, 4 ),
 ( 0.4999048021866459024, 0.5624167019133151646, 0.6249286016399844268, 0.6874405013666536890, 0.7499524010933229512, 0.8124643008199922134, 0.8749762005466614756, 0.9374881002733307378, 1.000000000000000000 ),
 .UNSPECIFIED. ) ;
#89808=DIRECTION ( 'NONE',  ( 0.000000000000000000, 0.000000000000000000, -1.000000000000000000 ) ) ;
#89809=CARTESIAN_POINT ( 'NONE',  ( 114.2868575967315223, -43.69575777765361124, 118.2174201252820751 ) ) ;
#89810=EDGE_CURVE ( 'NONE', #61107, #31976, #71113, .T. ) ;
#89811=CARTESIAN_POINT ( 'NONE',  ( 97.63545021146504155, -41.27351965004424983, 167.6841967044829573 ) ) ;
#89812=DIRECTION ( 'NONE',  ( -0.7071067811865765496, 0.7071067811865185959, -7.071067811865773128E-16 ) ) ;
#89813=CARTESIAN_POINT ( 'NONE',  ( 115.6077113496922948, -36.78907078068826308, 263.2438483995052820 ) ) ;
#89814=ORIENTED_EDGE ( 'NONE', *, *, #55706, .T. ) ;
#89815=AXIS2_PLACEMENT_3D ( 'NONE', #38507, #18066, #38956 ) ;
#89816=ORIENTED_EDGE ( 'NONE', *, *, #74025, .F. ) ;
#89817=ORIENTED_EDGE ( 'NONE', *, *, #59260, .T. ) ;
#89819=DIRECTION ( 'NONE',  ( -1.000000000000000078E-15, 1.000000000000000083E-30, 1.000000000000000000 ) ) ;
#89821=CARTESIAN_POINT ( 'NONE',  ( 104.4909048318107381, -26.97854783814448965, 20.28044007747010014 ) ) ;
#89822=CARTESIAN_POINT ( 'NONE',  ( 97.07198150990170404, -35.37932431885595008, 276.2185944750585236 ) ) ;
#89824=ADVANCED_FACE ( 'NONE', ( #86970 ), #73319, .F. ) ;
#89826=CARTESIAN_POINT ( 'NONE',  ( 106.5394234437989667, -24.24056378642895737, 322.0356252759110021 ) ) ;
#89827=CARTESIAN_POINT ( 'NONE',  ( 106.2788006184939888, -47.06957971430152554, 267.5280062282925542 ) ) ;
#89828=DIRECTION ( 'NONE',  ( -0.7071067811865476838, -0.7071067811865473507, 0.000000000000000000 ) ) ;
#89829=ADVANCED_FACE ( 'NONE', ( #11093, #36706, #31091 ), #1287, .F. ) ;
#89830=ORIENTED_EDGE ( 'NONE', *, *, #56240, .F. ) ;
#89832=LINE ( 'NONE', #81673, #57724 ) ;
#89834=CARTESIAN_POINT ( 'NONE',  ( 111.3320211711901067, -29.76992759232029329, 92.45666179816296903 ) ) ;
#89835=CIRCLE ( 'NONE', #50640, 2.117000000000007987 ) ;
#89836=AXIS2_PLACEMENT_3D ( 'NONE', #52035, #50373, #17550 ) ;
#89837=CARTESIAN_POINT ( 'NONE',  ( 46.32460016641643108, -48.34074026909789268, 129.9678068554150911 ) ) ;
#89838=DIRECTION ( 'NONE',  ( 0.000000000000000000, 0.000000000000000000, -1.000000000000000000 ) ) ;
#89840=AXIS2_PLACEMENT_3D ( 'NONE', #39999, #74529, #75435 ) ;
#89841=CARTESIAN_POINT ( 'NONE',  ( 77.40046754268342966, -36.03188136815408171, 6.871351212842532696 ) ) ;
#89843=CARTESIAN_POINT ( 'NONE',  ( 109.2014631304945027, -26.52509060526352869, 139.9127681330539872 ) ) ;
#89845=DIRECTION ( 'NONE',  ( 3.339108161477000479E-13, -1.000000000000000000, 6.848429599184487071E-29 ) ) ;
#89846=CARTESIAN_POINT ( 'NONE',  ( 115.4287739208600527, -39.66208659201188880, 129.9901547344679500 ) ) ;
#89847=FACE_OUTER_BOUND ( 'NONE', #59281, .T. ) ;
#89848=EDGE_CURVE ( 'NONE', #26191, #71530, #34706, .T. ) ;
#89849=DIRECTION ( 'NONE',  ( -1.000000000000000000, -4.299999999999999979E-14, -1.000000000000000078E-15 ) ) ;
#89850=CARTESIAN_POINT ( 'NONE',  ( 118.0249073071387471, -38.34132458482030614, 69.72229194257801055 ) ) ;
#89851=CARTESIAN_POINT ( 'NONE',  ( 151.0371591254582313, -46.82818131005593187, 313.9678068554149490 ) ) ;
#89853=LINE ( 'NONE', #88947, #51245 ) ;
#89854=ORIENTED_EDGE ( 'NONE', *, *, #29375, .F. ) ;
#89855=EDGE_LOOP ( 'NONE', ( #79305, #12085 ) ) ;
#89857=VECTOR ( 'NONE', #56320, 1000.000000000000000 ) ;
#89858=DIRECTION ( 'NONE',  ( 1.000000000000000078E-15, 0.000000000000000000, -1.000000000000000000 ) ) ;
#89860=CARTESIAN_POINT ( 'NONE',  ( 106.8506556707805260, -46.50783423188027399, 272.5584824187685626 ) ) ;
#89861=CARTESIAN_POINT ( 'NONE',  ( 95.54549022710490647, -39.60850420455695087, 162.5213395616259788 ) ) ;
#89863=CARTESIAN_POINT ( 'NONE',  ( 109.6410330058590716, -46.48058483609847968, 128.7812978340938912 ) ) ;
#89864=CARTESIAN_POINT ( 'NONE',  ( 117.5953528424095254, -42.16796915894857278, 89.44705384733997278 ) ) ;
#89865=DIRECTION ( 'NONE',  ( 1.000000000000000000, 0.000000000000000000, 0.000000000000000000 ) ) ;
#89866=EDGE_LOOP ( 'NONE', ( #69823, #34715, #53157, #30743 ) ) ;
#89869=DIRECTION ( 'NONE',  ( 0.000000000000000000, 0.000000000000000000, -1.000000000000000000 ) ) ;
#89870=AXIS2_PLACEMENT_3D ( 'NONE', #82459, #75630, #12505 ) ;
#89871=VERTEX_POINT ( 'NONE', #17909 ) ;
#89875=DIRECTION ( 'NONE',  ( 0.000000000000000000, 0.000000000000000000, -1.000000000000000000 ) ) ;
#89876=CARTESIAN_POINT ( 'NONE',  ( 105.0259480979001410, -25.88970440745768542, 280.2365776568631759 ) ) ;
#89877=LINE ( 'NONE', #12665, #34449 ) ;
#89878=CARTESIAN_POINT ( 'NONE',  ( 188.5667039024479834, -62.87844715994099687, 178.0928068554149775 ) ) ;
#89879=CARTESIAN_POINT ( 'NONE',  ( 101.9945362158859155, -45.44663583214662594, 92.15693711078462513 ) ) ;
#89880=CARTESIAN_POINT ( 'NONE',  ( 105.4283229756613309, -27.08692670426131954, 15.20991099019697401 ) ) ;
#89881=FACE_OUTER_BOUND ( 'NONE', #21325, .T. ) ;
#89882=CARTESIAN_POINT ( 'NONE',  ( 112.7897778137181746, -47.07797880090539167, 98.97848241876793907 ) ) ;
#89883=CARTESIAN_POINT ( 'NONE',  ( 57.56670390244829605, -48.82844715994039575, 293.2178068554150627 ) ) ;
#89884=CARTESIAN_POINT ( 'NONE',  ( 108.0109225731970213, -26.30163847990888826, 155.0041967044819557 ) ) ;
#89887=CARTESIAN_POINT ( 'NONE',  ( 25.56670390244797275, -48.82844715994099971, 173.2178068554149775 ) ) ;
#89888=FACE_BOUND ( 'NONE', #11852, .T. ) ;
#89889=CARTESIAN_POINT ( 'NONE',  ( 136.5183630979163638, -35.48272428400311895, 2.716753546981010903 ) ) ;
#89891=VECTOR ( 'NONE', #79961, 1000.000000000000114 ) ;
#89892=CARTESIAN_POINT ( 'NONE',  ( 48.86082318535681424, -35.55794170701784651, 237.4678068554150059 ) ) ;
#89893=CARTESIAN_POINT ( 'NONE',  ( 99.38968898744698777, -27.63536841754259044, 150.6356252759109680 ) ) ;
#89894=VERTEX_POINT ( 'NONE', #20163 ) ;
#89897=CARTESIAN_POINT ( 'NONE',  ( 110.1438736645959580, -26.08919931346192911, 210.8403871806729626 ) ) ;
#89899=LINE ( 'NONE', #13140, #79376 ) ;
#89900=VECTOR ( 'NONE', #8771, 999.9999999999998863 ) ;
#89903=ADVANCED_FACE ( 'NONE', ( #40592 ), #26973, .F. ) ;
#89905=ADVANCED_FACE ( 'NONE', ( #19703 ), #53297, .F. ) ;
#89907=CIRCLE ( 'NONE', #42016, 5.035202529042049235 ) ;
#89909=VERTEX_POINT ( 'NONE', #89206 ) ;
#89910=CYLINDRICAL_SURFACE ( 'NONE', #35066, 13.44999999999999396 ) ;
#89911=CARTESIAN_POINT ( 'NONE',  ( 108.1817661827909376, -47.09470796318245078, 198.6613395616249989 ) ) ;
#89912=CARTESIAN_POINT ( 'NONE',  ( 98.10600417527815864, -32.16171936412747101, 250.9518541729705987 ) ) ;
#89913=DIRECTION ( 'NONE',  ( -1.000000000000000000, 6.036837696399451257E-13, 0.000000000000000000 ) ) ;
#89916=AXIS2_PLACEMENT_3D ( 'NONE', #36782, #43124, #8638 ) ;
#89918=CARTESIAN_POINT ( 'NONE',  ( 188.5667039024479834, -67.87844715994100397, 252.3428068554150059 ) ) ;
#89922=AXIS2_PLACEMENT_3D ( 'NONE', #67778, #17839, #60962 ) ;
#89924=CARTESIAN_POINT ( 'NONE',  ( 87.06648329127403940, -54.72944906728955061, -4.824374724089049771 ) ) ;
#89925=CARTESIAN_POINT ( 'NONE',  ( 117.3624379696766198, -35.49166588079122420, 234.9337205140059552 ) ) ;
#89926=EDGE_CURVE ( 'NONE', #12869, #10387, #32419, .T. ) ;
#89927=DIRECTION ( 'NONE',  ( 0.9242245927363026414, 0.3818493186865932754, 0.000000000000000000 ) ) ;
#89928=CARTESIAN_POINT ( 'NONE',  ( 102.8368274790083490, -27.91052165842139487, 91.43276813305296002 ) ) ;
#89929=DIRECTION ( 'NONE',  ( -2.081668171172166620E-14, -1.000000000000000000, 0.000000000000000000 ) ) ;
#89930=CARTESIAN_POINT ( 'NONE',  ( 113.5912987900053110, -29.06716993070983435, 20.51551907639133887 ) ) ;
#89931=EDGE_LOOP ( 'NONE', ( #81527, #31745, #12519, #18581 ) ) ;
#89932=VERTEX_POINT ( 'NONE', #76010 ) ;
ENDSEC;
END-ISO-10303-21;
